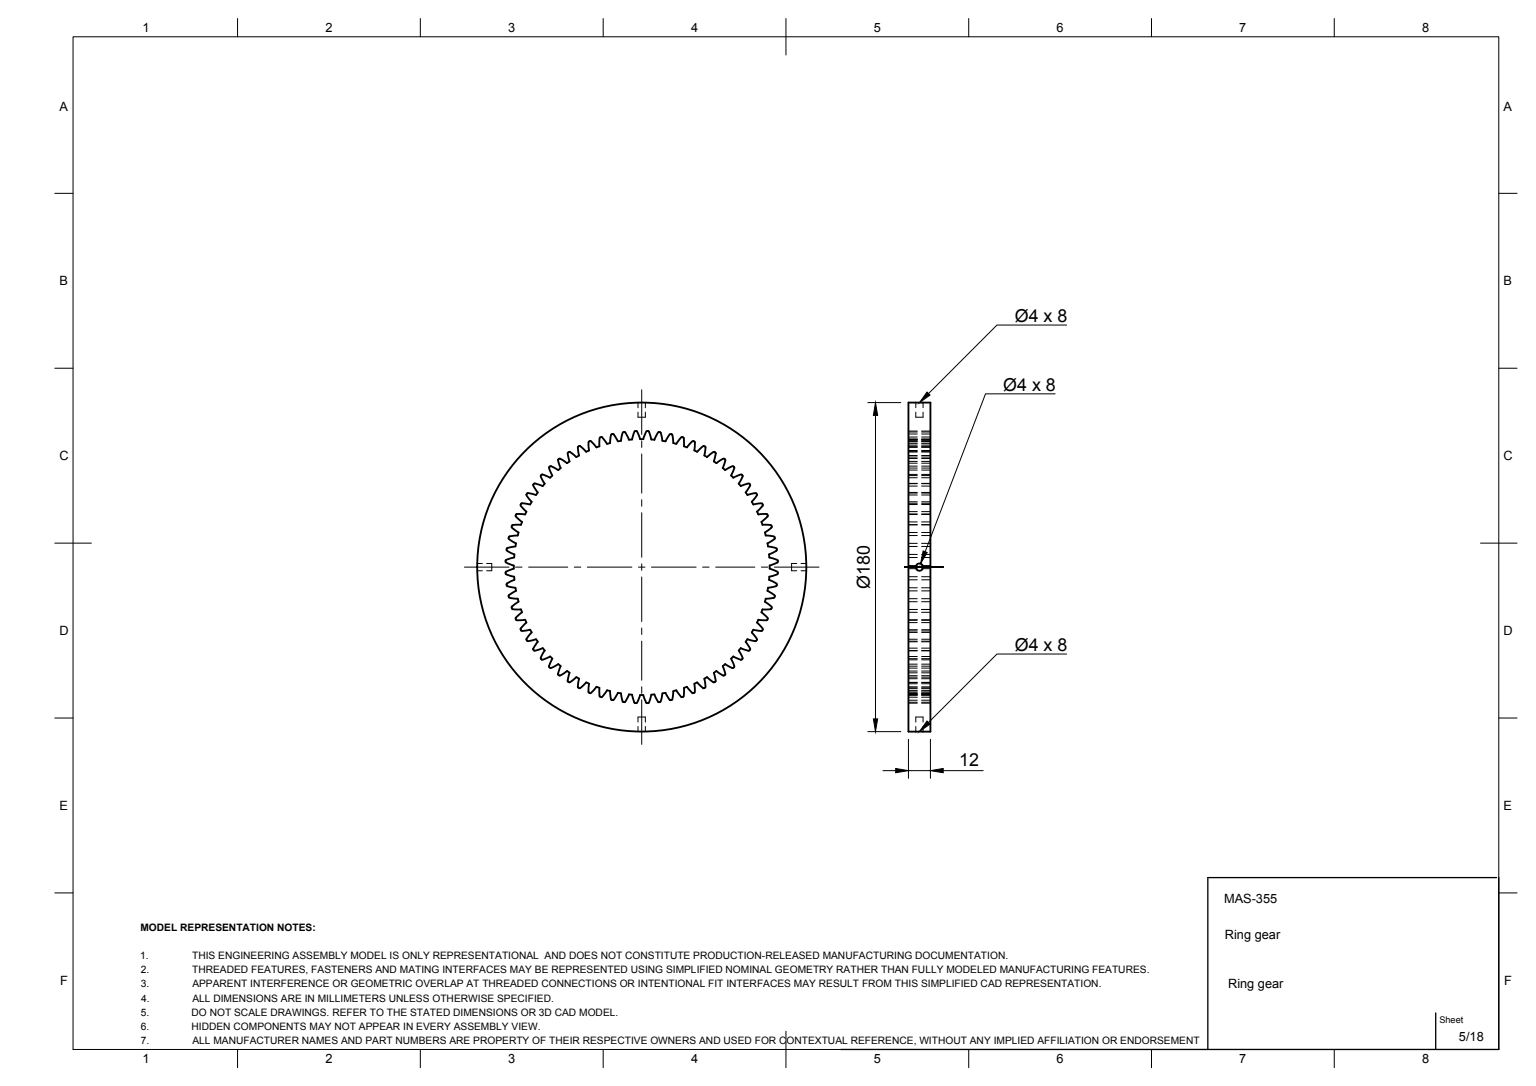
ISO-10303-21;
HEADER;
/* Generated by software containing ST-Developer
 * from STEP Tools, Inc. (www.steptools.com) 
 */

FILE_DESCRIPTION(
/* description */ ('Independent two-stage fixed-ring planetary gearbox,24/24/72 teeth,mod
ule2,20deg involutes,three planets per stage,4:1 x4:1=16:1. Native cut
-space/fillet/pattern tooth profiles derived from reusable gear blanks
; shared sun/planet/ring/carrier parts across both stages. Captured br
onze-journal input/carriers, headed retained planet pins, keyed inters
tage drive and modular keyed output interface. Native ideal gear links
; no torque, precision grade, production backlash/fits, lubrication, s
peed or life rating.'),
/* implementation_level */ '2;1');

FILE_NAME(
/* name */ 'Ring gear.step',
/* time_stamp */ '2026-11-08T19:10:00-08:00',
/* author */ (''),
/* organization */ (''),
/* preprocessor_version */ 'ST-DEVELOPER v20.2',
/* originating_system */ 'Autodesk Translation Framework v15.17.0.0',
/* authorisation */ '');

FILE_SCHEMA (('AUTOMOTIVE_DESIGN { 1 0 10303 214 3 1 1 }'));
ENDSEC;

DATA;
#10=MECHANICAL_DESIGN_GEOMETRIC_PRESENTATION_REPRESENTATION('',(#1167),#259224);
#403=(
BOUNDED_CURVE()
B_SPLINE_CURVE(5,(#53033,#53034,#53035,#53036,#53037,#53038,#53039,#53040,
#53041,#53042,#53043,#53044,#53045,#53046,#53047,#53048,#53049,#53050,#53051,
#53052,#53053,#53054,#53055,#53056,#53057,#53058,#53059,#53060,#53061,#53062,
#53063,#53064,#53065,#53066,#53067,#53068,#53069,#53070,#53071,#53072,#53073,
#53074,#53075,#53076,#53077,#53078,#53079,#53080,#53081,#53082,#53083,#53084,
#53085,#53086,#53087,#53088,#53089,#53090,#53091,#53092,#53093,#53094,#53095,
#53096,#53097,#53098,#53099,#53100,#53101,#53102,#53103,#53104,#53105,#53106,
#53107,#53108,#53109,#53110,#53111,#53112,#53113,#53114,#53115,#53116,#53117,
#53118,#53119,#53120,#53121,#53122,#53123,#53124,#53125,#53126,#53127,#53128,
#53129,#53130,#53131,#53132,#53133,#53134,#53135,#53136,#53137,#53138,#53139,
#53140,#53141,#53142,#53143,#53144,#53145,#53146,#53147,#53148,#53149,#53150,
#53151,#53152,#53153,#53154,#53155,#53156,#53157,#53158,#53159,#53160,#53161,
#53162,#53163,#53164,#53165,#53166,#53167,#53168,#53169,#53170,#53171,#53172,
#53173,#53174,#53175,#53176,#53177,#53178,#53179,#53180,#53181,#53182,#53183,
#53184,#53185,#53186,#53187,#53188,#53189,#53190,#53191,#53192,#53193,#53194,
#53195,#53196,#53197,#53198,#53199,#53200,#53201,#53202,#53203,#53204,#53205,
#53206,#53207,#53208,#53209,#53210,#53211,#53212,#53213,#53214,#53215,#53216,
#53217,#53218,#53219,#53220,#53221,#53222,#53223,#53224,#53225,#53226),
 .UNSPECIFIED.,.F.,.F.)
B_SPLINE_CURVE_WITH_KNOTS((6,1,1,1,1,1,1,1,1,1,1,1,1,1,1,1,1,1,1,1,1,1,
1,1,1,1,1,1,1,1,1,1,1,1,1,1,1,1,1,1,1,1,1,1,1,1,1,1,1,1,1,1,1,1,1,1,1,1,
1,1,1,1,1,1,1,1,1,1,1,1,1,1,1,1,1,1,1,1,1,1,1,1,1,1,1,1,1,1,1,1,1,1,1,1,
1,1,1,1,1,1,1,1,1,1,1,1,1,1,1,1,1,1,1,1,1,1,1,1,1,1,1,1,1,1,1,1,1,1,1,1,
1,1,1,1,1,1,1,1,1,1,1,1,1,1,1,1,1,1,1,1,1,1,1,1,1,1,1,1,1,1,1,1,1,1,1,1,
1,1,1,1,1,1,1,1,1,1,1,1,1,1,1,1,1,1,1,1,1,1,1,6),(0.,0.005,0.01,0.015,0.02,
0.025,0.03,0.035,0.04,0.045,0.05,0.055,0.06,0.065,0.07,0.075,0.08,0.085,
0.09,0.095,0.1,0.105,0.11,0.115,0.12,0.125,0.13,0.135,0.14,0.145,0.15,0.155,
0.16,0.165,0.17,0.175,0.18,0.185,0.19,0.195,0.2,0.205,0.21,0.215,0.22,0.225,
0.23,0.235,0.24,0.245,0.25,0.255,0.26,0.265,0.27,0.275,0.28,0.285,0.29,
0.295,0.3,0.305,0.31,0.315,0.32,0.325,0.33,0.335,0.34,0.345,0.35,0.355,
0.36,0.365,0.37,0.375,0.38,0.385,0.39,0.395,0.4,0.405,0.41,0.415,0.42,0.425,
0.43,0.435,0.44,0.445,0.45,0.455,0.46,0.465,0.47,0.475,0.48,0.485,0.49,
0.495,0.5,0.505,0.51,0.515,0.52,0.525,0.53,0.535,0.54,0.545,0.55,0.555,
0.56,0.565,0.57,0.575,0.58,0.585,0.59,0.595,0.6,0.605,0.61,0.615,0.62,0.625,
0.63,0.635,0.64,0.645,0.65,0.655,0.66,0.665,0.67,0.675,0.68,0.685,0.690000000000001,
0.695000000000001,0.700000000000001,0.705000000000001,0.710000000000001,
0.715000000000001,0.720000000000001,0.725000000000001,0.730000000000001,
0.735000000000001,0.740000000000001,0.745000000000001,0.750000000000001,
0.755000000000001,0.760000000000001,0.765000000000001,0.770000000000001,
0.775000000000001,0.780000000000001,0.785000000000001,0.790000000000001,
0.795000000000001,0.800000000000001,0.805000000000001,0.810000000000001,
0.815000000000001,0.820000000000001,0.825000000000001,0.830000000000001,
0.835000000000001,0.840000000000001,0.845000000000001,0.850000000000001,
0.855000000000001,0.860000000000001,0.865000000000001,0.870000000000001,
0.875000000000001,0.880000000000001,0.885000000000001,0.890000000000001,
0.895000000000001,0.900000000000001,0.905000000000001,0.910000000000001,
0.915000000000001,0.920000000000001,0.925000000000001,0.930000000000001,
0.935000000000001,0.940000000000001,0.941429844431396),.UNSPECIFIED.)
CURVE()
GEOMETRIC_REPRESENTATION_ITEM()
RATIONAL_B_SPLINE_CURVE((1.,1.,1.,1.,1.,1.,1.,1.,1.,1.,1.,1.,1.,1.,1.,1.,
1.,1.,1.,1.,1.,1.,1.,1.,1.,1.,1.,1.,1.,1.,1.,1.,1.,1.,1.,1.,1.,1.,1.,1.,
1.,1.,1.,1.,1.,1.,1.,1.,1.,1.,1.,1.,1.,1.,1.,1.,1.,1.,1.,1.,1.,1.,1.,1.,
1.,1.,1.,1.,1.,1.,1.,1.,1.,1.,1.,1.,1.,1.,1.,1.,1.,1.,1.,1.,1.,1.,1.,1.,
1.,1.,1.,1.,1.,1.,1.,1.,1.,1.,1.,1.,1.,1.,1.,1.,1.,1.,1.,1.,1.,1.,1.,1.,
1.,1.,1.,1.,1.,1.,1.,1.,1.,1.,1.,1.,1.,1.,1.,1.,1.,1.,1.,1.,1.,1.,1.,1.,
1.,1.,1.,1.,1.,1.,1.,1.,1.,1.,1.,1.,1.,1.,1.,1.,1.,1.,1.,1.,1.,1.,1.,1.,
1.,1.,1.,1.,1.,1.,1.,1.,1.,1.,1.,1.,1.,1.,1.,1.,1.,1.,1.,1.,1.,1.,1.,1.,
1.,1.,1.,1.,1.,1.,1.,1.,1.,1.))
REPRESENTATION_ITEM('')
);
#404=(
BOUNDED_CURVE()
B_SPLINE_CURVE(5,(#53229,#53230,#53231,#53232,#53233,#53234,#53235,#53236,
#53237,#53238,#53239,#53240,#53241,#53242,#53243,#53244,#53245,#53246,#53247,
#53248,#53249,#53250,#53251,#53252,#53253,#53254,#53255,#53256,#53257,#53258,
#53259,#53260,#53261,#53262,#53263,#53264,#53265,#53266,#53267,#53268,#53269,
#53270,#53271,#53272,#53273,#53274,#53275,#53276,#53277,#53278,#53279,#53280,
#53281,#53282,#53283,#53284,#53285,#53286,#53287,#53288,#53289,#53290,#53291,
#53292,#53293,#53294,#53295,#53296,#53297,#53298,#53299,#53300,#53301,#53302,
#53303,#53304,#53305,#53306,#53307,#53308,#53309,#53310,#53311,#53312,#53313,
#53314,#53315,#53316,#53317,#53318,#53319,#53320,#53321,#53322,#53323,#53324,
#53325,#53326,#53327,#53328,#53329,#53330,#53331,#53332,#53333,#53334,#53335,
#53336,#53337,#53338,#53339,#53340,#53341,#53342,#53343,#53344,#53345,#53346,
#53347,#53348,#53349,#53350,#53351,#53352,#53353,#53354,#53355,#53356,#53357,
#53358,#53359,#53360,#53361,#53362,#53363,#53364,#53365,#53366,#53367,#53368,
#53369,#53370,#53371,#53372,#53373,#53374,#53375,#53376,#53377,#53378,#53379,
#53380,#53381,#53382,#53383,#53384,#53385,#53386,#53387,#53388,#53389,#53390,
#53391,#53392,#53393,#53394,#53395,#53396,#53397,#53398,#53399,#53400,#53401,
#53402,#53403,#53404,#53405,#53406,#53407,#53408,#53409,#53410,#53411,#53412,
#53413,#53414,#53415,#53416,#53417,#53418,#53419,#53420,#53421,#53422),
 .UNSPECIFIED.,.F.,.F.)
B_SPLINE_CURVE_WITH_KNOTS((6,1,1,1,1,1,1,1,1,1,1,1,1,1,1,1,1,1,1,1,1,1,
1,1,1,1,1,1,1,1,1,1,1,1,1,1,1,1,1,1,1,1,1,1,1,1,1,1,1,1,1,1,1,1,1,1,1,1,
1,1,1,1,1,1,1,1,1,1,1,1,1,1,1,1,1,1,1,1,1,1,1,1,1,1,1,1,1,1,1,1,1,1,1,1,
1,1,1,1,1,1,1,1,1,1,1,1,1,1,1,1,1,1,1,1,1,1,1,1,1,1,1,1,1,1,1,1,1,1,1,1,
1,1,1,1,1,1,1,1,1,1,1,1,1,1,1,1,1,1,1,1,1,1,1,1,1,1,1,1,1,1,1,1,1,1,1,1,
1,1,1,1,1,1,1,1,1,1,1,1,1,1,1,1,1,1,1,1,1,1,1,6),(-0.941429844431396,-0.940000000000001,
-0.935000000000001,-0.930000000000001,-0.925000000000001,-0.920000000000001,
-0.915000000000001,-0.910000000000001,-0.905000000000001,-0.900000000000001,
-0.895000000000001,-0.890000000000001,-0.885000000000001,-0.880000000000001,
-0.875000000000001,-0.870000000000001,-0.865000000000001,-0.860000000000001,
-0.855000000000001,-0.850000000000001,-0.845000000000001,-0.840000000000001,
-0.835000000000001,-0.830000000000001,-0.825000000000001,-0.820000000000001,
-0.815000000000001,-0.810000000000001,-0.805000000000001,-0.800000000000001,
-0.795000000000001,-0.790000000000001,-0.785000000000001,-0.780000000000001,
-0.775000000000001,-0.770000000000001,-0.765000000000001,-0.760000000000001,
-0.755000000000001,-0.750000000000001,-0.745000000000001,-0.740000000000001,
-0.735000000000001,-0.730000000000001,-0.725000000000001,-0.720000000000001,
-0.715000000000001,-0.710000000000001,-0.705000000000001,-0.700000000000001,
-0.695000000000001,-0.690000000000001,-0.685,-0.68,-0.675,-0.67,-0.665,
-0.66,-0.655,-0.65,-0.645,-0.64,-0.635,-0.63,-0.625,-0.62,-0.615,-0.61,
-0.605,-0.6,-0.595,-0.59,-0.585,-0.58,-0.575,-0.57,-0.565,-0.56,-0.555,
-0.55,-0.545,-0.54,-0.535,-0.53,-0.525,-0.52,-0.515,-0.51,-0.505,-0.5,-0.495,
-0.49,-0.485,-0.48,-0.475,-0.47,-0.465,-0.46,-0.455,-0.45,-0.445,-0.44,
-0.435,-0.43,-0.425,-0.42,-0.415,-0.41,-0.405,-0.4,-0.395,-0.39,-0.385,
-0.38,-0.375,-0.37,-0.365,-0.36,-0.355,-0.35,-0.345,-0.34,-0.335,-0.33,
-0.325,-0.32,-0.315,-0.31,-0.305,-0.3,-0.295,-0.29,-0.285,-0.28,-0.275,
-0.27,-0.265,-0.26,-0.255,-0.25,-0.245,-0.24,-0.235,-0.23,-0.225,-0.22,
-0.215,-0.21,-0.205,-0.2,-0.195,-0.19,-0.185,-0.18,-0.175,-0.17,-0.165,
-0.16,-0.155,-0.15,-0.145,-0.14,-0.135,-0.13,-0.125,-0.12,-0.115,-0.11,
-0.105,-0.1,-0.095,-0.09,-0.085,-0.08,-0.075,-0.07,-0.065,-0.06,-0.055,
-0.05,-0.045,-0.04,-0.035,-0.03,-0.025,-0.02,-0.015,-0.01,-0.005,0.),
 .UNSPECIFIED.)
CURVE()
GEOMETRIC_REPRESENTATION_ITEM()
RATIONAL_B_SPLINE_CURVE((1.,1.,1.,1.,1.,1.,1.,1.,1.,1.,1.,1.,1.,1.,1.,1.,
1.,1.,1.,1.,1.,1.,1.,1.,1.,1.,1.,1.,1.,1.,1.,1.,1.,1.,1.,1.,1.,1.,1.,1.,
1.,1.,1.,1.,1.,1.,1.,1.,1.,1.,1.,1.,1.,1.,1.,1.,1.,1.,1.,1.,1.,1.,1.,1.,
1.,1.,1.,1.,1.,1.,1.,1.,1.,1.,1.,1.,1.,1.,1.,1.,1.,1.,1.,1.,1.,1.,1.,1.,
1.,1.,1.,1.,1.,1.,1.,1.,1.,1.,1.,1.,1.,1.,1.,1.,1.,1.,1.,1.,1.,1.,1.,1.,
1.,1.,1.,1.,1.,1.,1.,1.,1.,1.,1.,1.,1.,1.,1.,1.,1.,1.,1.,1.,1.,1.,1.,1.,
1.,1.,1.,1.,1.,1.,1.,1.,1.,1.,1.,1.,1.,1.,1.,1.,1.,1.,1.,1.,1.,1.,1.,1.,
1.,1.,1.,1.,1.,1.,1.,1.,1.,1.,1.,1.,1.,1.,1.,1.,1.,1.,1.,1.,1.,1.,1.,1.,
1.,1.,1.,1.,1.,1.,1.,1.,1.,1.))
REPRESENTATION_ITEM('')
);
#405=(
BOUNDED_CURVE()
B_SPLINE_CURVE(5,(#53929,#53930,#53931,#53932,#53933,#53934,#53935,#53936,
#53937,#53938,#53939,#53940,#53941,#53942,#53943,#53944,#53945,#53946,#53947,
#53948,#53949,#53950,#53951,#53952,#53953,#53954,#53955,#53956,#53957,#53958,
#53959,#53960,#53961,#53962,#53963,#53964,#53965,#53966,#53967,#53968,#53969,
#53970,#53971,#53972,#53973,#53974,#53975,#53976,#53977,#53978,#53979,#53980,
#53981,#53982,#53983,#53984,#53985,#53986,#53987,#53988,#53989,#53990,#53991,
#53992,#53993,#53994,#53995,#53996,#53997,#53998,#53999,#54000,#54001,#54002,
#54003,#54004,#54005,#54006,#54007,#54008,#54009,#54010,#54011,#54012,#54013,
#54014,#54015,#54016,#54017,#54018,#54019,#54020,#54021,#54022,#54023,#54024,
#54025,#54026,#54027,#54028,#54029,#54030,#54031,#54032,#54033,#54034,#54035,
#54036,#54037,#54038,#54039,#54040,#54041,#54042,#54043,#54044,#54045,#54046,
#54047,#54048,#54049,#54050,#54051,#54052,#54053,#54054,#54055,#54056,#54057,
#54058,#54059,#54060,#54061,#54062,#54063,#54064,#54065,#54066,#54067,#54068,
#54069,#54070,#54071,#54072,#54073,#54074,#54075,#54076,#54077,#54078,#54079,
#54080,#54081,#54082,#54083,#54084,#54085,#54086,#54087,#54088,#54089,#54090,
#54091,#54092,#54093,#54094,#54095,#54096,#54097,#54098,#54099,#54100,#54101,
#54102,#54103,#54104,#54105,#54106,#54107,#54108,#54109,#54110,#54111,#54112,
#54113,#54114,#54115,#54116,#54117,#54118,#54119,#54120,#54121,#54122),
 .UNSPECIFIED.,.F.,.F.)
B_SPLINE_CURVE_WITH_KNOTS((6,1,1,1,1,1,1,1,1,1,1,1,1,1,1,1,1,1,1,1,1,1,
1,1,1,1,1,1,1,1,1,1,1,1,1,1,1,1,1,1,1,1,1,1,1,1,1,1,1,1,1,1,1,1,1,1,1,1,
1,1,1,1,1,1,1,1,1,1,1,1,1,1,1,1,1,1,1,1,1,1,1,1,1,1,1,1,1,1,1,1,1,1,1,1,
1,1,1,1,1,1,1,1,1,1,1,1,1,1,1,1,1,1,1,1,1,1,1,1,1,1,1,1,1,1,1,1,1,1,1,1,
1,1,1,1,1,1,1,1,1,1,1,1,1,1,1,1,1,1,1,1,1,1,1,1,1,1,1,1,1,1,1,1,1,1,1,1,
1,1,1,1,1,1,1,1,1,1,1,1,1,1,1,1,1,1,1,1,1,1,1,6),(0.,0.005,0.01,0.015,0.02,
0.025,0.03,0.035,0.04,0.045,0.05,0.055,0.06,0.065,0.07,0.075,0.08,0.085,
0.09,0.095,0.1,0.105,0.11,0.115,0.12,0.125,0.13,0.135,0.14,0.145,0.15,0.155,
0.16,0.165,0.17,0.175,0.18,0.185,0.19,0.195,0.2,0.205,0.21,0.215,0.22,0.225,
0.23,0.235,0.24,0.245,0.25,0.255,0.26,0.265,0.27,0.275,0.28,0.285,0.29,
0.295,0.3,0.305,0.31,0.315,0.32,0.325,0.33,0.335,0.34,0.345,0.35,0.355,
0.36,0.365,0.37,0.375,0.38,0.385,0.39,0.395,0.4,0.405,0.41,0.415,0.42,0.425,
0.43,0.435,0.44,0.445,0.45,0.455,0.46,0.465,0.47,0.475,0.48,0.485,0.49,
0.495,0.5,0.505,0.51,0.515,0.52,0.525,0.53,0.535,0.54,0.545,0.55,0.555,
0.56,0.565,0.57,0.575,0.58,0.585,0.59,0.595,0.6,0.605,0.61,0.615,0.62,0.625,
0.63,0.635,0.64,0.645,0.65,0.655,0.66,0.665,0.67,0.675,0.68,0.685,0.690000000000001,
0.695000000000001,0.700000000000001,0.705000000000001,0.710000000000001,
0.715000000000001,0.720000000000001,0.725000000000001,0.730000000000001,
0.735000000000001,0.740000000000001,0.745000000000001,0.750000000000001,
0.755000000000001,0.760000000000001,0.765000000000001,0.770000000000001,
0.775000000000001,0.780000000000001,0.785000000000001,0.790000000000001,
0.795000000000001,0.800000000000001,0.805000000000001,0.810000000000001,
0.815000000000001,0.820000000000001,0.825000000000001,0.830000000000001,
0.835000000000001,0.840000000000001,0.845000000000001,0.850000000000001,
0.855000000000001,0.860000000000001,0.865000000000001,0.870000000000001,
0.875000000000001,0.880000000000001,0.885000000000001,0.890000000000001,
0.895000000000001,0.900000000000001,0.905000000000001,0.910000000000001,
0.915000000000001,0.920000000000001,0.925000000000001,0.930000000000001,
0.935000000000001,0.940000000000001,0.941429844431388),.UNSPECIFIED.)
CURVE()
GEOMETRIC_REPRESENTATION_ITEM()
RATIONAL_B_SPLINE_CURVE((1.,1.,1.,1.,1.,1.,1.,1.,1.,1.,1.,1.,1.,1.,1.,1.,
1.,1.,1.,1.,1.,1.,1.,1.,1.,1.,1.,1.,1.,1.,1.,1.,1.,1.,1.,1.,1.,1.,1.,1.,
1.,1.,1.,1.,1.,1.,1.,1.,1.,1.,1.,1.,1.,1.,1.,1.,1.,1.,1.,1.,1.,1.,1.,1.,
1.,1.,1.,1.,1.,1.,1.,1.,1.,1.,1.,1.,1.,1.,1.,1.,1.,1.,1.,1.,1.,1.,1.,1.,
1.,1.,1.,1.,1.,1.,1.,1.,1.,1.,1.,1.,1.,1.,1.,1.,1.,1.,1.,1.,1.,1.,1.,1.,
1.,1.,1.,1.,1.,1.,1.,1.,1.,1.,1.,1.,1.,1.,1.,1.,1.,1.,1.,1.,1.,1.,1.,1.,
1.,1.,1.,1.,1.,1.,1.,1.,1.,1.,1.,1.,1.,1.,1.,1.,1.,1.,1.,1.,1.,1.,1.,1.,
1.,1.,1.,1.,1.,1.,1.,1.,1.,1.,1.,1.,1.,1.,1.,1.,1.,1.,1.,1.,1.,1.,1.,1.,
1.,1.,1.,1.,1.,1.,1.,1.,1.,1.))
REPRESENTATION_ITEM('')
);
#406=(
BOUNDED_CURVE()
B_SPLINE_CURVE(5,(#54125,#54126,#54127,#54128,#54129,#54130,#54131,#54132,
#54133,#54134,#54135,#54136,#54137,#54138,#54139,#54140,#54141,#54142,#54143,
#54144,#54145,#54146,#54147,#54148,#54149,#54150,#54151,#54152,#54153,#54154,
#54155,#54156,#54157,#54158,#54159,#54160,#54161,#54162,#54163,#54164,#54165,
#54166,#54167,#54168,#54169,#54170,#54171,#54172,#54173,#54174,#54175,#54176,
#54177,#54178,#54179,#54180,#54181,#54182,#54183,#54184,#54185,#54186,#54187,
#54188,#54189,#54190,#54191,#54192,#54193,#54194,#54195,#54196,#54197,#54198,
#54199,#54200,#54201,#54202,#54203,#54204,#54205,#54206,#54207,#54208,#54209,
#54210,#54211,#54212,#54213,#54214,#54215,#54216,#54217,#54218,#54219,#54220,
#54221,#54222,#54223,#54224,#54225,#54226,#54227,#54228,#54229,#54230,#54231,
#54232,#54233,#54234,#54235,#54236,#54237,#54238,#54239,#54240,#54241,#54242,
#54243,#54244,#54245,#54246,#54247,#54248,#54249,#54250,#54251,#54252,#54253,
#54254,#54255,#54256,#54257,#54258,#54259,#54260,#54261,#54262,#54263,#54264,
#54265,#54266,#54267,#54268,#54269,#54270,#54271,#54272,#54273,#54274,#54275,
#54276,#54277,#54278,#54279,#54280,#54281,#54282,#54283,#54284,#54285,#54286,
#54287,#54288,#54289,#54290,#54291,#54292,#54293,#54294,#54295,#54296,#54297,
#54298,#54299,#54300,#54301,#54302,#54303,#54304,#54305,#54306,#54307,#54308,
#54309,#54310,#54311,#54312,#54313,#54314,#54315,#54316,#54317,#54318),
 .UNSPECIFIED.,.F.,.F.)
B_SPLINE_CURVE_WITH_KNOTS((6,1,1,1,1,1,1,1,1,1,1,1,1,1,1,1,1,1,1,1,1,1,
1,1,1,1,1,1,1,1,1,1,1,1,1,1,1,1,1,1,1,1,1,1,1,1,1,1,1,1,1,1,1,1,1,1,1,1,
1,1,1,1,1,1,1,1,1,1,1,1,1,1,1,1,1,1,1,1,1,1,1,1,1,1,1,1,1,1,1,1,1,1,1,1,
1,1,1,1,1,1,1,1,1,1,1,1,1,1,1,1,1,1,1,1,1,1,1,1,1,1,1,1,1,1,1,1,1,1,1,1,
1,1,1,1,1,1,1,1,1,1,1,1,1,1,1,1,1,1,1,1,1,1,1,1,1,1,1,1,1,1,1,1,1,1,1,1,
1,1,1,1,1,1,1,1,1,1,1,1,1,1,1,1,1,1,1,1,1,1,1,6),(-0.941429844431391,-0.940000000000001,
-0.935000000000001,-0.930000000000001,-0.925000000000001,-0.920000000000001,
-0.915000000000001,-0.910000000000001,-0.905000000000001,-0.900000000000001,
-0.895000000000001,-0.890000000000001,-0.885000000000001,-0.880000000000001,
-0.875000000000001,-0.870000000000001,-0.865000000000001,-0.860000000000001,
-0.855000000000001,-0.850000000000001,-0.845000000000001,-0.840000000000001,
-0.835000000000001,-0.830000000000001,-0.825000000000001,-0.820000000000001,
-0.815000000000001,-0.810000000000001,-0.805000000000001,-0.800000000000001,
-0.795000000000001,-0.790000000000001,-0.785000000000001,-0.780000000000001,
-0.775000000000001,-0.770000000000001,-0.765000000000001,-0.760000000000001,
-0.755000000000001,-0.750000000000001,-0.745000000000001,-0.740000000000001,
-0.735000000000001,-0.730000000000001,-0.725000000000001,-0.720000000000001,
-0.715000000000001,-0.710000000000001,-0.705000000000001,-0.700000000000001,
-0.695000000000001,-0.690000000000001,-0.685,-0.68,-0.675,-0.67,-0.665,
-0.66,-0.655,-0.65,-0.645,-0.64,-0.635,-0.63,-0.625,-0.62,-0.615,-0.61,
-0.605,-0.6,-0.595,-0.59,-0.585,-0.58,-0.575,-0.57,-0.565,-0.56,-0.555,
-0.55,-0.545,-0.54,-0.535,-0.53,-0.525,-0.52,-0.515,-0.51,-0.505,-0.5,-0.495,
-0.49,-0.485,-0.48,-0.475,-0.47,-0.465,-0.46,-0.455,-0.45,-0.445,-0.44,
-0.435,-0.43,-0.425,-0.42,-0.415,-0.41,-0.405,-0.4,-0.395,-0.39,-0.385,
-0.38,-0.375,-0.37,-0.365,-0.36,-0.355,-0.35,-0.345,-0.34,-0.335,-0.33,
-0.325,-0.32,-0.315,-0.31,-0.305,-0.3,-0.295,-0.29,-0.285,-0.28,-0.275,
-0.27,-0.265,-0.26,-0.255,-0.25,-0.245,-0.24,-0.235,-0.23,-0.225,-0.22,
-0.215,-0.21,-0.205,-0.2,-0.195,-0.19,-0.185,-0.18,-0.175,-0.17,-0.165,
-0.16,-0.155,-0.15,-0.145,-0.14,-0.135,-0.13,-0.125,-0.12,-0.115,-0.11,
-0.105,-0.1,-0.095,-0.09,-0.085,-0.08,-0.075,-0.07,-0.065,-0.06,-0.055,
-0.05,-0.045,-0.04,-0.035,-0.03,-0.025,-0.02,-0.015,-0.01,-0.005,0.),
 .UNSPECIFIED.)
CURVE()
GEOMETRIC_REPRESENTATION_ITEM()
RATIONAL_B_SPLINE_CURVE((1.,1.,1.,1.,1.,1.,1.,1.,1.,1.,1.,1.,1.,1.,1.,1.,
1.,1.,1.,1.,1.,1.,1.,1.,1.,1.,1.,1.,1.,1.,1.,1.,1.,1.,1.,1.,1.,1.,1.,1.,
1.,1.,1.,1.,1.,1.,1.,1.,1.,1.,1.,1.,1.,1.,1.,1.,1.,1.,1.,1.,1.,1.,1.,1.,
1.,1.,1.,1.,1.,1.,1.,1.,1.,1.,1.,1.,1.,1.,1.,1.,1.,1.,1.,1.,1.,1.,1.,1.,
1.,1.,1.,1.,1.,1.,1.,1.,1.,1.,1.,1.,1.,1.,1.,1.,1.,1.,1.,1.,1.,1.,1.,1.,
1.,1.,1.,1.,1.,1.,1.,1.,1.,1.,1.,1.,1.,1.,1.,1.,1.,1.,1.,1.,1.,1.,1.,1.,
1.,1.,1.,1.,1.,1.,1.,1.,1.,1.,1.,1.,1.,1.,1.,1.,1.,1.,1.,1.,1.,1.,1.,1.,
1.,1.,1.,1.,1.,1.,1.,1.,1.,1.,1.,1.,1.,1.,1.,1.,1.,1.,1.,1.,1.,1.,1.,1.,
1.,1.,1.,1.,1.,1.,1.,1.,1.,1.))
REPRESENTATION_ITEM('')
);
#407=(
BOUNDED_CURVE()
B_SPLINE_CURVE(5,(#54825,#54826,#54827,#54828,#54829,#54830,#54831,#54832,
#54833,#54834,#54835,#54836,#54837,#54838,#54839,#54840,#54841,#54842,#54843,
#54844,#54845,#54846,#54847,#54848,#54849,#54850,#54851,#54852,#54853,#54854,
#54855,#54856,#54857,#54858,#54859,#54860,#54861,#54862,#54863,#54864,#54865,
#54866,#54867,#54868,#54869,#54870,#54871,#54872,#54873,#54874,#54875,#54876,
#54877,#54878,#54879,#54880,#54881,#54882,#54883,#54884,#54885,#54886,#54887,
#54888,#54889,#54890,#54891,#54892,#54893,#54894,#54895,#54896,#54897,#54898,
#54899,#54900,#54901,#54902,#54903,#54904,#54905,#54906,#54907,#54908,#54909,
#54910,#54911,#54912,#54913,#54914,#54915,#54916,#54917,#54918,#54919,#54920,
#54921,#54922,#54923,#54924,#54925,#54926,#54927,#54928,#54929,#54930,#54931,
#54932,#54933,#54934,#54935,#54936,#54937,#54938,#54939,#54940,#54941,#54942,
#54943,#54944,#54945,#54946,#54947,#54948,#54949,#54950,#54951,#54952,#54953,
#54954,#54955,#54956,#54957,#54958,#54959,#54960,#54961,#54962,#54963,#54964,
#54965,#54966,#54967,#54968,#54969,#54970,#54971,#54972,#54973,#54974,#54975,
#54976,#54977,#54978,#54979,#54980,#54981,#54982,#54983,#54984,#54985,#54986,
#54987,#54988,#54989,#54990,#54991,#54992,#54993,#54994,#54995,#54996,#54997,
#54998,#54999,#55000,#55001,#55002,#55003,#55004,#55005,#55006,#55007,#55008,
#55009,#55010,#55011,#55012,#55013,#55014,#55015,#55016,#55017,#55018),
 .UNSPECIFIED.,.F.,.F.)
B_SPLINE_CURVE_WITH_KNOTS((6,1,1,1,1,1,1,1,1,1,1,1,1,1,1,1,1,1,1,1,1,1,
1,1,1,1,1,1,1,1,1,1,1,1,1,1,1,1,1,1,1,1,1,1,1,1,1,1,1,1,1,1,1,1,1,1,1,1,
1,1,1,1,1,1,1,1,1,1,1,1,1,1,1,1,1,1,1,1,1,1,1,1,1,1,1,1,1,1,1,1,1,1,1,1,
1,1,1,1,1,1,1,1,1,1,1,1,1,1,1,1,1,1,1,1,1,1,1,1,1,1,1,1,1,1,1,1,1,1,1,1,
1,1,1,1,1,1,1,1,1,1,1,1,1,1,1,1,1,1,1,1,1,1,1,1,1,1,1,1,1,1,1,1,1,1,1,1,
1,1,1,1,1,1,1,1,1,1,1,1,1,1,1,1,1,1,1,1,1,1,1,6),(0.,0.005,0.01,0.015,0.02,
0.025,0.03,0.035,0.04,0.045,0.05,0.055,0.06,0.065,0.07,0.075,0.08,0.085,
0.09,0.095,0.1,0.105,0.11,0.115,0.12,0.125,0.13,0.135,0.14,0.145,0.15,0.155,
0.16,0.165,0.17,0.175,0.18,0.185,0.19,0.195,0.2,0.205,0.21,0.215,0.22,0.225,
0.23,0.235,0.24,0.245,0.25,0.255,0.26,0.265,0.27,0.275,0.28,0.285,0.29,
0.295,0.3,0.305,0.31,0.315,0.32,0.325,0.33,0.335,0.34,0.345,0.35,0.355,
0.36,0.365,0.37,0.375,0.38,0.385,0.39,0.395,0.4,0.405,0.41,0.415,0.42,0.425,
0.43,0.435,0.44,0.445,0.45,0.455,0.46,0.465,0.47,0.475,0.48,0.485,0.49,
0.495,0.5,0.505,0.51,0.515,0.52,0.525,0.53,0.535,0.54,0.545,0.55,0.555,
0.56,0.565,0.57,0.575,0.58,0.585,0.59,0.595,0.6,0.605,0.61,0.615,0.62,0.625,
0.63,0.635,0.64,0.645,0.65,0.655,0.66,0.665,0.67,0.675,0.68,0.685,0.690000000000001,
0.695000000000001,0.700000000000001,0.705000000000001,0.710000000000001,
0.715000000000001,0.720000000000001,0.725000000000001,0.730000000000001,
0.735000000000001,0.740000000000001,0.745000000000001,0.750000000000001,
0.755000000000001,0.760000000000001,0.765000000000001,0.770000000000001,
0.775000000000001,0.780000000000001,0.785000000000001,0.790000000000001,
0.795000000000001,0.800000000000001,0.805000000000001,0.810000000000001,
0.815000000000001,0.820000000000001,0.825000000000001,0.830000000000001,
0.835000000000001,0.840000000000001,0.845000000000001,0.850000000000001,
0.855000000000001,0.860000000000001,0.865000000000001,0.870000000000001,
0.875000000000001,0.880000000000001,0.885000000000001,0.890000000000001,
0.895000000000001,0.900000000000001,0.905000000000001,0.910000000000001,
0.915000000000001,0.920000000000001,0.925000000000001,0.930000000000001,
0.935000000000001,0.940000000000001,0.941429844431439),.UNSPECIFIED.)
CURVE()
GEOMETRIC_REPRESENTATION_ITEM()
RATIONAL_B_SPLINE_CURVE((1.,1.,1.,1.,1.,1.,1.,1.,1.,1.,1.,1.,1.,1.,1.,1.,
1.,1.,1.,1.,1.,1.,1.,1.,1.,1.,1.,1.,1.,1.,1.,1.,1.,1.,1.,1.,1.,1.,1.,1.,
1.,1.,1.,1.,1.,1.,1.,1.,1.,1.,1.,1.,1.,1.,1.,1.,1.,1.,1.,1.,1.,1.,1.,1.,
1.,1.,1.,1.,1.,1.,1.,1.,1.,1.,1.,1.,1.,1.,1.,1.,1.,1.,1.,1.,1.,1.,1.,1.,
1.,1.,1.,1.,1.,1.,1.,1.,1.,1.,1.,1.,1.,1.,1.,1.,1.,1.,1.,1.,1.,1.,1.,1.,
1.,1.,1.,1.,1.,1.,1.,1.,1.,1.,1.,1.,1.,1.,1.,1.,1.,1.,1.,1.,1.,1.,1.,1.,
1.,1.,1.,1.,1.,1.,1.,1.,1.,1.,1.,1.,1.,1.,1.,1.,1.,1.,1.,1.,1.,1.,1.,1.,
1.,1.,1.,1.,1.,1.,1.,1.,1.,1.,1.,1.,1.,1.,1.,1.,1.,1.,1.,1.,1.,1.,1.,1.,
1.,1.,1.,1.,1.,1.,1.,1.,1.,1.))
REPRESENTATION_ITEM('')
);
#408=(
BOUNDED_CURVE()
B_SPLINE_CURVE(5,(#55021,#55022,#55023,#55024,#55025,#55026,#55027,#55028,
#55029,#55030,#55031,#55032,#55033,#55034,#55035,#55036,#55037,#55038,#55039,
#55040,#55041,#55042,#55043,#55044,#55045,#55046,#55047,#55048,#55049,#55050,
#55051,#55052,#55053,#55054,#55055,#55056,#55057,#55058,#55059,#55060,#55061,
#55062,#55063,#55064,#55065,#55066,#55067,#55068,#55069,#55070,#55071,#55072,
#55073,#55074,#55075,#55076,#55077,#55078,#55079,#55080,#55081,#55082,#55083,
#55084,#55085,#55086,#55087,#55088,#55089,#55090,#55091,#55092,#55093,#55094,
#55095,#55096,#55097,#55098,#55099,#55100,#55101,#55102,#55103,#55104,#55105,
#55106,#55107,#55108,#55109,#55110,#55111,#55112,#55113,#55114,#55115,#55116,
#55117,#55118,#55119,#55120,#55121,#55122,#55123,#55124,#55125,#55126,#55127,
#55128,#55129,#55130,#55131,#55132,#55133,#55134,#55135,#55136,#55137,#55138,
#55139,#55140,#55141,#55142,#55143,#55144,#55145,#55146,#55147,#55148,#55149,
#55150,#55151,#55152,#55153,#55154,#55155,#55156,#55157,#55158,#55159,#55160,
#55161,#55162,#55163,#55164,#55165,#55166,#55167,#55168,#55169,#55170,#55171,
#55172,#55173,#55174,#55175,#55176,#55177,#55178,#55179,#55180,#55181,#55182,
#55183,#55184,#55185,#55186,#55187,#55188,#55189,#55190,#55191,#55192,#55193,
#55194,#55195,#55196,#55197,#55198,#55199,#55200,#55201,#55202,#55203,#55204,
#55205,#55206,#55207,#55208,#55209,#55210,#55211,#55212,#55213,#55214),
 .UNSPECIFIED.,.F.,.F.)
B_SPLINE_CURVE_WITH_KNOTS((6,1,1,1,1,1,1,1,1,1,1,1,1,1,1,1,1,1,1,1,1,1,
1,1,1,1,1,1,1,1,1,1,1,1,1,1,1,1,1,1,1,1,1,1,1,1,1,1,1,1,1,1,1,1,1,1,1,1,
1,1,1,1,1,1,1,1,1,1,1,1,1,1,1,1,1,1,1,1,1,1,1,1,1,1,1,1,1,1,1,1,1,1,1,1,
1,1,1,1,1,1,1,1,1,1,1,1,1,1,1,1,1,1,1,1,1,1,1,1,1,1,1,1,1,1,1,1,1,1,1,1,
1,1,1,1,1,1,1,1,1,1,1,1,1,1,1,1,1,1,1,1,1,1,1,1,1,1,1,1,1,1,1,1,1,1,1,1,
1,1,1,1,1,1,1,1,1,1,1,1,1,1,1,1,1,1,1,1,1,1,1,6),(-0.941429844431442,-0.940000000000001,
-0.935000000000001,-0.930000000000001,-0.925000000000001,-0.920000000000001,
-0.915000000000001,-0.910000000000001,-0.905000000000001,-0.900000000000001,
-0.895000000000001,-0.890000000000001,-0.885000000000001,-0.880000000000001,
-0.875000000000001,-0.870000000000001,-0.865000000000001,-0.860000000000001,
-0.855000000000001,-0.850000000000001,-0.845000000000001,-0.840000000000001,
-0.835000000000001,-0.830000000000001,-0.825000000000001,-0.820000000000001,
-0.815000000000001,-0.810000000000001,-0.805000000000001,-0.800000000000001,
-0.795000000000001,-0.790000000000001,-0.785000000000001,-0.780000000000001,
-0.775000000000001,-0.770000000000001,-0.765000000000001,-0.760000000000001,
-0.755000000000001,-0.750000000000001,-0.745000000000001,-0.740000000000001,
-0.735000000000001,-0.730000000000001,-0.725000000000001,-0.720000000000001,
-0.715000000000001,-0.710000000000001,-0.705000000000001,-0.700000000000001,
-0.695000000000001,-0.690000000000001,-0.685,-0.68,-0.675,-0.67,-0.665,
-0.66,-0.655,-0.65,-0.645,-0.64,-0.635,-0.63,-0.625,-0.62,-0.615,-0.61,
-0.605,-0.6,-0.595,-0.59,-0.585,-0.58,-0.575,-0.57,-0.565,-0.56,-0.555,
-0.55,-0.545,-0.54,-0.535,-0.53,-0.525,-0.52,-0.515,-0.51,-0.505,-0.5,-0.495,
-0.49,-0.485,-0.48,-0.475,-0.47,-0.465,-0.46,-0.455,-0.45,-0.445,-0.44,
-0.435,-0.43,-0.425,-0.42,-0.415,-0.41,-0.405,-0.4,-0.395,-0.39,-0.385,
-0.38,-0.375,-0.37,-0.365,-0.36,-0.355,-0.35,-0.345,-0.34,-0.335,-0.33,
-0.325,-0.32,-0.315,-0.31,-0.305,-0.3,-0.295,-0.29,-0.285,-0.28,-0.275,
-0.27,-0.265,-0.26,-0.255,-0.25,-0.245,-0.24,-0.235,-0.23,-0.225,-0.22,
-0.215,-0.21,-0.205,-0.2,-0.195,-0.19,-0.185,-0.18,-0.175,-0.17,-0.165,
-0.16,-0.155,-0.15,-0.145,-0.14,-0.135,-0.13,-0.125,-0.12,-0.115,-0.11,
-0.105,-0.1,-0.095,-0.09,-0.085,-0.08,-0.075,-0.07,-0.065,-0.06,-0.055,
-0.05,-0.045,-0.04,-0.035,-0.03,-0.025,-0.02,-0.015,-0.01,-0.005,0.),
 .UNSPECIFIED.)
CURVE()
GEOMETRIC_REPRESENTATION_ITEM()
RATIONAL_B_SPLINE_CURVE((1.,1.,1.,1.,1.,1.,1.,1.,1.,1.,1.,1.,1.,1.,1.,1.,
1.,1.,1.,1.,1.,1.,1.,1.,1.,1.,1.,1.,1.,1.,1.,1.,1.,1.,1.,1.,1.,1.,1.,1.,
1.,1.,1.,1.,1.,1.,1.,1.,1.,1.,1.,1.,1.,1.,1.,1.,1.,1.,1.,1.,1.,1.,1.,1.,
1.,1.,1.,1.,1.,1.,1.,1.,1.,1.,1.,1.,1.,1.,1.,1.,1.,1.,1.,1.,1.,1.,1.,1.,
1.,1.,1.,1.,1.,1.,1.,1.,1.,1.,1.,1.,1.,1.,1.,1.,1.,1.,1.,1.,1.,1.,1.,1.,
1.,1.,1.,1.,1.,1.,1.,1.,1.,1.,1.,1.,1.,1.,1.,1.,1.,1.,1.,1.,1.,1.,1.,1.,
1.,1.,1.,1.,1.,1.,1.,1.,1.,1.,1.,1.,1.,1.,1.,1.,1.,1.,1.,1.,1.,1.,1.,1.,
1.,1.,1.,1.,1.,1.,1.,1.,1.,1.,1.,1.,1.,1.,1.,1.,1.,1.,1.,1.,1.,1.,1.,1.,
1.,1.,1.,1.,1.,1.,1.,1.,1.,1.))
REPRESENTATION_ITEM('')
);
#409=(
BOUNDED_CURVE()
B_SPLINE_CURVE(5,(#55721,#55722,#55723,#55724,#55725,#55726,#55727,#55728,
#55729,#55730,#55731,#55732,#55733,#55734,#55735,#55736,#55737,#55738,#55739,
#55740,#55741,#55742,#55743,#55744,#55745,#55746,#55747,#55748,#55749,#55750,
#55751,#55752,#55753,#55754,#55755,#55756,#55757,#55758,#55759,#55760,#55761,
#55762,#55763,#55764,#55765,#55766,#55767,#55768,#55769,#55770,#55771,#55772,
#55773,#55774,#55775,#55776,#55777,#55778,#55779,#55780,#55781,#55782,#55783,
#55784,#55785,#55786,#55787,#55788,#55789,#55790,#55791,#55792,#55793,#55794,
#55795,#55796,#55797,#55798,#55799,#55800,#55801,#55802,#55803,#55804,#55805,
#55806,#55807,#55808,#55809,#55810,#55811,#55812,#55813,#55814,#55815,#55816,
#55817,#55818,#55819,#55820,#55821,#55822,#55823,#55824,#55825,#55826,#55827,
#55828,#55829,#55830,#55831,#55832,#55833,#55834,#55835,#55836,#55837,#55838,
#55839,#55840,#55841,#55842,#55843,#55844,#55845,#55846,#55847,#55848,#55849,
#55850,#55851,#55852,#55853,#55854,#55855,#55856,#55857,#55858,#55859,#55860,
#55861,#55862,#55863,#55864,#55865,#55866,#55867,#55868,#55869,#55870,#55871,
#55872,#55873,#55874,#55875,#55876,#55877,#55878,#55879,#55880,#55881,#55882,
#55883,#55884,#55885,#55886,#55887,#55888,#55889,#55890,#55891,#55892,#55893,
#55894,#55895,#55896,#55897,#55898,#55899,#55900,#55901,#55902,#55903,#55904,
#55905,#55906,#55907,#55908,#55909,#55910,#55911,#55912,#55913,#55914),
 .UNSPECIFIED.,.F.,.F.)
B_SPLINE_CURVE_WITH_KNOTS((6,1,1,1,1,1,1,1,1,1,1,1,1,1,1,1,1,1,1,1,1,1,
1,1,1,1,1,1,1,1,1,1,1,1,1,1,1,1,1,1,1,1,1,1,1,1,1,1,1,1,1,1,1,1,1,1,1,1,
1,1,1,1,1,1,1,1,1,1,1,1,1,1,1,1,1,1,1,1,1,1,1,1,1,1,1,1,1,1,1,1,1,1,1,1,
1,1,1,1,1,1,1,1,1,1,1,1,1,1,1,1,1,1,1,1,1,1,1,1,1,1,1,1,1,1,1,1,1,1,1,1,
1,1,1,1,1,1,1,1,1,1,1,1,1,1,1,1,1,1,1,1,1,1,1,1,1,1,1,1,1,1,1,1,1,1,1,1,
1,1,1,1,1,1,1,1,1,1,1,1,1,1,1,1,1,1,1,1,1,1,1,6),(0.,0.005,0.01,0.015,0.02,
0.025,0.03,0.035,0.04,0.045,0.05,0.055,0.06,0.065,0.07,0.075,0.08,0.085,
0.09,0.095,0.1,0.105,0.11,0.115,0.12,0.125,0.13,0.135,0.14,0.145,0.15,0.155,
0.16,0.165,0.17,0.175,0.18,0.185,0.19,0.195,0.2,0.205,0.21,0.215,0.22,0.225,
0.23,0.235,0.24,0.245,0.25,0.255,0.26,0.265,0.27,0.275,0.28,0.285,0.29,
0.295,0.3,0.305,0.31,0.315,0.32,0.325,0.33,0.335,0.34,0.345,0.35,0.355,
0.36,0.365,0.37,0.375,0.38,0.385,0.39,0.395,0.4,0.405,0.41,0.415,0.42,0.425,
0.43,0.435,0.44,0.445,0.45,0.455,0.46,0.465,0.47,0.475,0.48,0.485,0.49,
0.495,0.5,0.505,0.51,0.515,0.52,0.525,0.53,0.535,0.54,0.545,0.55,0.555,
0.56,0.565,0.57,0.575,0.58,0.585,0.59,0.595,0.6,0.605,0.61,0.615,0.62,0.625,
0.63,0.635,0.64,0.645,0.65,0.655,0.66,0.665,0.67,0.675,0.68,0.685,0.690000000000001,
0.695000000000001,0.700000000000001,0.705000000000001,0.710000000000001,
0.715000000000001,0.720000000000001,0.725000000000001,0.730000000000001,
0.735000000000001,0.740000000000001,0.745000000000001,0.750000000000001,
0.755000000000001,0.760000000000001,0.765000000000001,0.770000000000001,
0.775000000000001,0.780000000000001,0.785000000000001,0.790000000000001,
0.795000000000001,0.800000000000001,0.805000000000001,0.810000000000001,
0.815000000000001,0.820000000000001,0.825000000000001,0.830000000000001,
0.835000000000001,0.840000000000001,0.845000000000001,0.850000000000001,
0.855000000000001,0.860000000000001,0.865000000000001,0.870000000000001,
0.875000000000001,0.880000000000001,0.885000000000001,0.890000000000001,
0.895000000000001,0.900000000000001,0.905000000000001,0.910000000000001,
0.915000000000001,0.920000000000001,0.925000000000001,0.930000000000001,
0.935000000000001,0.940000000000001,0.941429844431425),.UNSPECIFIED.)
CURVE()
GEOMETRIC_REPRESENTATION_ITEM()
RATIONAL_B_SPLINE_CURVE((1.,1.,1.,1.,1.,1.,1.,1.,1.,1.,1.,1.,1.,1.,1.,1.,
1.,1.,1.,1.,1.,1.,1.,1.,1.,1.,1.,1.,1.,1.,1.,1.,1.,1.,1.,1.,1.,1.,1.,1.,
1.,1.,1.,1.,1.,1.,1.,1.,1.,1.,1.,1.,1.,1.,1.,1.,1.,1.,1.,1.,1.,1.,1.,1.,
1.,1.,1.,1.,1.,1.,1.,1.,1.,1.,1.,1.,1.,1.,1.,1.,1.,1.,1.,1.,1.,1.,1.,1.,
1.,1.,1.,1.,1.,1.,1.,1.,1.,1.,1.,1.,1.,1.,1.,1.,1.,1.,1.,1.,1.,1.,1.,1.,
1.,1.,1.,1.,1.,1.,1.,1.,1.,1.,1.,1.,1.,1.,1.,1.,1.,1.,1.,1.,1.,1.,1.,1.,
1.,1.,1.,1.,1.,1.,1.,1.,1.,1.,1.,1.,1.,1.,1.,1.,1.,1.,1.,1.,1.,1.,1.,1.,
1.,1.,1.,1.,1.,1.,1.,1.,1.,1.,1.,1.,1.,1.,1.,1.,1.,1.,1.,1.,1.,1.,1.,1.,
1.,1.,1.,1.,1.,1.,1.,1.,1.,1.))
REPRESENTATION_ITEM('')
);
#410=(
BOUNDED_CURVE()
B_SPLINE_CURVE(5,(#55917,#55918,#55919,#55920,#55921,#55922,#55923,#55924,
#55925,#55926,#55927,#55928,#55929,#55930,#55931,#55932,#55933,#55934,#55935,
#55936,#55937,#55938,#55939,#55940,#55941,#55942,#55943,#55944,#55945,#55946,
#55947,#55948,#55949,#55950,#55951,#55952,#55953,#55954,#55955,#55956,#55957,
#55958,#55959,#55960,#55961,#55962,#55963,#55964,#55965,#55966,#55967,#55968,
#55969,#55970,#55971,#55972,#55973,#55974,#55975,#55976,#55977,#55978,#55979,
#55980,#55981,#55982,#55983,#55984,#55985,#55986,#55987,#55988,#55989,#55990,
#55991,#55992,#55993,#55994,#55995,#55996,#55997,#55998,#55999,#56000,#56001,
#56002,#56003,#56004,#56005,#56006,#56007,#56008,#56009,#56010,#56011,#56012,
#56013,#56014,#56015,#56016,#56017,#56018,#56019,#56020,#56021,#56022,#56023,
#56024,#56025,#56026,#56027,#56028,#56029,#56030,#56031,#56032,#56033,#56034,
#56035,#56036,#56037,#56038,#56039,#56040,#56041,#56042,#56043,#56044,#56045,
#56046,#56047,#56048,#56049,#56050,#56051,#56052,#56053,#56054,#56055,#56056,
#56057,#56058,#56059,#56060,#56061,#56062,#56063,#56064,#56065,#56066,#56067,
#56068,#56069,#56070,#56071,#56072,#56073,#56074,#56075,#56076,#56077,#56078,
#56079,#56080,#56081,#56082,#56083,#56084,#56085,#56086,#56087,#56088,#56089,
#56090,#56091,#56092,#56093,#56094,#56095,#56096,#56097,#56098,#56099,#56100,
#56101,#56102,#56103,#56104,#56105,#56106,#56107,#56108,#56109,#56110),
 .UNSPECIFIED.,.F.,.F.)
B_SPLINE_CURVE_WITH_KNOTS((6,1,1,1,1,1,1,1,1,1,1,1,1,1,1,1,1,1,1,1,1,1,
1,1,1,1,1,1,1,1,1,1,1,1,1,1,1,1,1,1,1,1,1,1,1,1,1,1,1,1,1,1,1,1,1,1,1,1,
1,1,1,1,1,1,1,1,1,1,1,1,1,1,1,1,1,1,1,1,1,1,1,1,1,1,1,1,1,1,1,1,1,1,1,1,
1,1,1,1,1,1,1,1,1,1,1,1,1,1,1,1,1,1,1,1,1,1,1,1,1,1,1,1,1,1,1,1,1,1,1,1,
1,1,1,1,1,1,1,1,1,1,1,1,1,1,1,1,1,1,1,1,1,1,1,1,1,1,1,1,1,1,1,1,1,1,1,1,
1,1,1,1,1,1,1,1,1,1,1,1,1,1,1,1,1,1,1,1,1,1,1,6),(-0.941429844431423,-0.940000000000001,
-0.935000000000001,-0.930000000000001,-0.925000000000001,-0.920000000000001,
-0.915000000000001,-0.910000000000001,-0.905000000000001,-0.900000000000001,
-0.895000000000001,-0.890000000000001,-0.885000000000001,-0.880000000000001,
-0.875000000000001,-0.870000000000001,-0.865000000000001,-0.860000000000001,
-0.855000000000001,-0.850000000000001,-0.845000000000001,-0.840000000000001,
-0.835000000000001,-0.830000000000001,-0.825000000000001,-0.820000000000001,
-0.815000000000001,-0.810000000000001,-0.805000000000001,-0.800000000000001,
-0.795000000000001,-0.790000000000001,-0.785000000000001,-0.780000000000001,
-0.775000000000001,-0.770000000000001,-0.765000000000001,-0.760000000000001,
-0.755000000000001,-0.750000000000001,-0.745000000000001,-0.740000000000001,
-0.735000000000001,-0.730000000000001,-0.725000000000001,-0.720000000000001,
-0.715000000000001,-0.710000000000001,-0.705000000000001,-0.700000000000001,
-0.695000000000001,-0.690000000000001,-0.685,-0.68,-0.675,-0.67,-0.665,
-0.66,-0.655,-0.65,-0.645,-0.64,-0.635,-0.63,-0.625,-0.62,-0.615,-0.61,
-0.605,-0.6,-0.595,-0.59,-0.585,-0.58,-0.575,-0.57,-0.565,-0.56,-0.555,
-0.55,-0.545,-0.54,-0.535,-0.53,-0.525,-0.52,-0.515,-0.51,-0.505,-0.5,-0.495,
-0.49,-0.485,-0.48,-0.475,-0.47,-0.465,-0.46,-0.455,-0.45,-0.445,-0.44,
-0.435,-0.43,-0.425,-0.42,-0.415,-0.41,-0.405,-0.4,-0.395,-0.39,-0.385,
-0.38,-0.375,-0.37,-0.365,-0.36,-0.355,-0.35,-0.345,-0.34,-0.335,-0.33,
-0.325,-0.32,-0.315,-0.31,-0.305,-0.3,-0.295,-0.29,-0.285,-0.28,-0.275,
-0.27,-0.265,-0.26,-0.255,-0.25,-0.245,-0.24,-0.235,-0.23,-0.225,-0.22,
-0.215,-0.21,-0.205,-0.2,-0.195,-0.19,-0.185,-0.18,-0.175,-0.17,-0.165,
-0.16,-0.155,-0.15,-0.145,-0.14,-0.135,-0.13,-0.125,-0.12,-0.115,-0.11,
-0.105,-0.1,-0.095,-0.09,-0.085,-0.08,-0.075,-0.07,-0.065,-0.06,-0.055,
-0.05,-0.045,-0.04,-0.035,-0.03,-0.025,-0.02,-0.015,-0.01,-0.005,0.),
 .UNSPECIFIED.)
CURVE()
GEOMETRIC_REPRESENTATION_ITEM()
RATIONAL_B_SPLINE_CURVE((1.,1.,1.,1.,1.,1.,1.,1.,1.,1.,1.,1.,1.,1.,1.,1.,
1.,1.,1.,1.,1.,1.,1.,1.,1.,1.,1.,1.,1.,1.,1.,1.,1.,1.,1.,1.,1.,1.,1.,1.,
1.,1.,1.,1.,1.,1.,1.,1.,1.,1.,1.,1.,1.,1.,1.,1.,1.,1.,1.,1.,1.,1.,1.,1.,
1.,1.,1.,1.,1.,1.,1.,1.,1.,1.,1.,1.,1.,1.,1.,1.,1.,1.,1.,1.,1.,1.,1.,1.,
1.,1.,1.,1.,1.,1.,1.,1.,1.,1.,1.,1.,1.,1.,1.,1.,1.,1.,1.,1.,1.,1.,1.,1.,
1.,1.,1.,1.,1.,1.,1.,1.,1.,1.,1.,1.,1.,1.,1.,1.,1.,1.,1.,1.,1.,1.,1.,1.,
1.,1.,1.,1.,1.,1.,1.,1.,1.,1.,1.,1.,1.,1.,1.,1.,1.,1.,1.,1.,1.,1.,1.,1.,
1.,1.,1.,1.,1.,1.,1.,1.,1.,1.,1.,1.,1.,1.,1.,1.,1.,1.,1.,1.,1.,1.,1.,1.,
1.,1.,1.,1.,1.,1.,1.,1.,1.,1.))
REPRESENTATION_ITEM('')
);
#411=(
BOUNDED_CURVE()
B_SPLINE_CURVE(5,(#56617,#56618,#56619,#56620,#56621,#56622,#56623,#56624,
#56625,#56626,#56627,#56628,#56629,#56630,#56631,#56632,#56633,#56634,#56635,
#56636,#56637,#56638,#56639,#56640,#56641,#56642,#56643,#56644,#56645,#56646,
#56647,#56648,#56649,#56650,#56651,#56652,#56653,#56654,#56655,#56656,#56657,
#56658,#56659,#56660,#56661,#56662,#56663,#56664,#56665,#56666,#56667,#56668,
#56669,#56670,#56671,#56672,#56673,#56674,#56675,#56676,#56677,#56678,#56679,
#56680,#56681,#56682,#56683,#56684,#56685,#56686,#56687,#56688,#56689,#56690,
#56691,#56692,#56693,#56694,#56695,#56696,#56697,#56698,#56699,#56700,#56701,
#56702,#56703,#56704,#56705,#56706,#56707,#56708,#56709,#56710,#56711,#56712,
#56713,#56714,#56715,#56716,#56717,#56718,#56719,#56720,#56721,#56722,#56723,
#56724,#56725,#56726,#56727,#56728,#56729,#56730,#56731,#56732,#56733,#56734,
#56735,#56736,#56737,#56738,#56739,#56740,#56741,#56742,#56743,#56744,#56745,
#56746,#56747,#56748,#56749,#56750,#56751,#56752,#56753,#56754,#56755,#56756,
#56757,#56758,#56759,#56760,#56761,#56762,#56763,#56764,#56765,#56766,#56767,
#56768,#56769,#56770,#56771,#56772,#56773,#56774,#56775,#56776,#56777,#56778,
#56779,#56780,#56781,#56782,#56783,#56784,#56785,#56786,#56787,#56788,#56789,
#56790,#56791,#56792,#56793,#56794,#56795,#56796,#56797,#56798,#56799,#56800,
#56801,#56802,#56803,#56804,#56805,#56806,#56807,#56808,#56809,#56810),
 .UNSPECIFIED.,.F.,.F.)
B_SPLINE_CURVE_WITH_KNOTS((6,1,1,1,1,1,1,1,1,1,1,1,1,1,1,1,1,1,1,1,1,1,
1,1,1,1,1,1,1,1,1,1,1,1,1,1,1,1,1,1,1,1,1,1,1,1,1,1,1,1,1,1,1,1,1,1,1,1,
1,1,1,1,1,1,1,1,1,1,1,1,1,1,1,1,1,1,1,1,1,1,1,1,1,1,1,1,1,1,1,1,1,1,1,1,
1,1,1,1,1,1,1,1,1,1,1,1,1,1,1,1,1,1,1,1,1,1,1,1,1,1,1,1,1,1,1,1,1,1,1,1,
1,1,1,1,1,1,1,1,1,1,1,1,1,1,1,1,1,1,1,1,1,1,1,1,1,1,1,1,1,1,1,1,1,1,1,1,
1,1,1,1,1,1,1,1,1,1,1,1,1,1,1,1,1,1,1,1,1,1,1,6),(0.,0.005,0.01,0.015,0.02,
0.025,0.03,0.035,0.04,0.045,0.05,0.055,0.06,0.065,0.07,0.075,0.08,0.085,
0.09,0.095,0.1,0.105,0.11,0.115,0.12,0.125,0.13,0.135,0.14,0.145,0.15,0.155,
0.16,0.165,0.17,0.175,0.18,0.185,0.19,0.195,0.2,0.205,0.21,0.215,0.22,0.225,
0.23,0.235,0.24,0.245,0.25,0.255,0.26,0.265,0.27,0.275,0.28,0.285,0.29,
0.295,0.3,0.305,0.31,0.315,0.32,0.325,0.33,0.335,0.34,0.345,0.35,0.355,
0.36,0.365,0.37,0.375,0.38,0.385,0.39,0.395,0.4,0.405,0.41,0.415,0.42,0.425,
0.43,0.435,0.44,0.445,0.45,0.455,0.46,0.465,0.47,0.475,0.48,0.485,0.49,
0.495,0.5,0.505,0.51,0.515,0.52,0.525,0.53,0.535,0.54,0.545,0.55,0.555,
0.56,0.565,0.57,0.575,0.58,0.585,0.59,0.595,0.6,0.605,0.61,0.615,0.62,0.625,
0.63,0.635,0.64,0.645,0.65,0.655,0.66,0.665,0.67,0.675,0.68,0.685,0.690000000000001,
0.695000000000001,0.700000000000001,0.705000000000001,0.710000000000001,
0.715000000000001,0.720000000000001,0.725000000000001,0.730000000000001,
0.735000000000001,0.740000000000001,0.745000000000001,0.750000000000001,
0.755000000000001,0.760000000000001,0.765000000000001,0.770000000000001,
0.775000000000001,0.780000000000001,0.785000000000001,0.790000000000001,
0.795000000000001,0.800000000000001,0.805000000000001,0.810000000000001,
0.815000000000001,0.820000000000001,0.825000000000001,0.830000000000001,
0.835000000000001,0.840000000000001,0.845000000000001,0.850000000000001,
0.855000000000001,0.860000000000001,0.865000000000001,0.870000000000001,
0.875000000000001,0.880000000000001,0.885000000000001,0.890000000000001,
0.895000000000001,0.900000000000001,0.905000000000001,0.910000000000001,
0.915000000000001,0.920000000000001,0.925000000000001,0.930000000000001,
0.935000000000001,0.940000000000001,0.941429844431363),.UNSPECIFIED.)
CURVE()
GEOMETRIC_REPRESENTATION_ITEM()
RATIONAL_B_SPLINE_CURVE((1.,1.,1.,1.,1.,1.,1.,1.,1.,1.,1.,1.,1.,1.,1.,1.,
1.,1.,1.,1.,1.,1.,1.,1.,1.,1.,1.,1.,1.,1.,1.,1.,1.,1.,1.,1.,1.,1.,1.,1.,
1.,1.,1.,1.,1.,1.,1.,1.,1.,1.,1.,1.,1.,1.,1.,1.,1.,1.,1.,1.,1.,1.,1.,1.,
1.,1.,1.,1.,1.,1.,1.,1.,1.,1.,1.,1.,1.,1.,1.,1.,1.,1.,1.,1.,1.,1.,1.,1.,
1.,1.,1.,1.,1.,1.,1.,1.,1.,1.,1.,1.,1.,1.,1.,1.,1.,1.,1.,1.,1.,1.,1.,1.,
1.,1.,1.,1.,1.,1.,1.,1.,1.,1.,1.,1.,1.,1.,1.,1.,1.,1.,1.,1.,1.,1.,1.,1.,
1.,1.,1.,1.,1.,1.,1.,1.,1.,1.,1.,1.,1.,1.,1.,1.,1.,1.,1.,1.,1.,1.,1.,1.,
1.,1.,1.,1.,1.,1.,1.,1.,1.,1.,1.,1.,1.,1.,1.,1.,1.,1.,1.,1.,1.,1.,1.,1.,
1.,1.,1.,1.,1.,1.,1.,1.,1.,1.))
REPRESENTATION_ITEM('')
);
#412=(
BOUNDED_CURVE()
B_SPLINE_CURVE(5,(#56813,#56814,#56815,#56816,#56817,#56818,#56819,#56820,
#56821,#56822,#56823,#56824,#56825,#56826,#56827,#56828,#56829,#56830,#56831,
#56832,#56833,#56834,#56835,#56836,#56837,#56838,#56839,#56840,#56841,#56842,
#56843,#56844,#56845,#56846,#56847,#56848,#56849,#56850,#56851,#56852,#56853,
#56854,#56855,#56856,#56857,#56858,#56859,#56860,#56861,#56862,#56863,#56864,
#56865,#56866,#56867,#56868,#56869,#56870,#56871,#56872,#56873,#56874,#56875,
#56876,#56877,#56878,#56879,#56880,#56881,#56882,#56883,#56884,#56885,#56886,
#56887,#56888,#56889,#56890,#56891,#56892,#56893,#56894,#56895,#56896,#56897,
#56898,#56899,#56900,#56901,#56902,#56903,#56904,#56905,#56906,#56907,#56908,
#56909,#56910,#56911,#56912,#56913,#56914,#56915,#56916,#56917,#56918,#56919,
#56920,#56921,#56922,#56923,#56924,#56925,#56926,#56927,#56928,#56929,#56930,
#56931,#56932,#56933,#56934,#56935,#56936,#56937,#56938,#56939,#56940,#56941,
#56942,#56943,#56944,#56945,#56946,#56947,#56948,#56949,#56950,#56951,#56952,
#56953,#56954,#56955,#56956,#56957,#56958,#56959,#56960,#56961,#56962,#56963,
#56964,#56965,#56966,#56967,#56968,#56969,#56970,#56971,#56972,#56973,#56974,
#56975,#56976,#56977,#56978,#56979,#56980,#56981,#56982,#56983,#56984,#56985,
#56986,#56987,#56988,#56989,#56990,#56991,#56992,#56993,#56994,#56995,#56996,
#56997,#56998,#56999,#57000,#57001,#57002,#57003,#57004,#57005,#57006),
 .UNSPECIFIED.,.F.,.F.)
B_SPLINE_CURVE_WITH_KNOTS((6,1,1,1,1,1,1,1,1,1,1,1,1,1,1,1,1,1,1,1,1,1,
1,1,1,1,1,1,1,1,1,1,1,1,1,1,1,1,1,1,1,1,1,1,1,1,1,1,1,1,1,1,1,1,1,1,1,1,
1,1,1,1,1,1,1,1,1,1,1,1,1,1,1,1,1,1,1,1,1,1,1,1,1,1,1,1,1,1,1,1,1,1,1,1,
1,1,1,1,1,1,1,1,1,1,1,1,1,1,1,1,1,1,1,1,1,1,1,1,1,1,1,1,1,1,1,1,1,1,1,1,
1,1,1,1,1,1,1,1,1,1,1,1,1,1,1,1,1,1,1,1,1,1,1,1,1,1,1,1,1,1,1,1,1,1,1,1,
1,1,1,1,1,1,1,1,1,1,1,1,1,1,1,1,1,1,1,1,1,1,1,6),(-0.941429844431365,-0.940000000000001,
-0.935000000000001,-0.930000000000001,-0.925000000000001,-0.920000000000001,
-0.915000000000001,-0.910000000000001,-0.905000000000001,-0.900000000000001,
-0.895000000000001,-0.890000000000001,-0.885000000000001,-0.880000000000001,
-0.875000000000001,-0.870000000000001,-0.865000000000001,-0.860000000000001,
-0.855000000000001,-0.850000000000001,-0.845000000000001,-0.840000000000001,
-0.835000000000001,-0.830000000000001,-0.825000000000001,-0.820000000000001,
-0.815000000000001,-0.810000000000001,-0.805000000000001,-0.800000000000001,
-0.795000000000001,-0.790000000000001,-0.785000000000001,-0.780000000000001,
-0.775000000000001,-0.770000000000001,-0.765000000000001,-0.760000000000001,
-0.755000000000001,-0.750000000000001,-0.745000000000001,-0.740000000000001,
-0.735000000000001,-0.730000000000001,-0.725000000000001,-0.720000000000001,
-0.715000000000001,-0.710000000000001,-0.705000000000001,-0.700000000000001,
-0.695000000000001,-0.690000000000001,-0.685,-0.68,-0.675,-0.67,-0.665,
-0.66,-0.655,-0.65,-0.645,-0.64,-0.635,-0.63,-0.625,-0.62,-0.615,-0.61,
-0.605,-0.6,-0.595,-0.59,-0.585,-0.58,-0.575,-0.57,-0.565,-0.56,-0.555,
-0.55,-0.545,-0.54,-0.535,-0.53,-0.525,-0.52,-0.515,-0.51,-0.505,-0.5,-0.495,
-0.49,-0.485,-0.48,-0.475,-0.47,-0.465,-0.46,-0.455,-0.45,-0.445,-0.44,
-0.435,-0.43,-0.425,-0.42,-0.415,-0.41,-0.405,-0.4,-0.395,-0.39,-0.385,
-0.38,-0.375,-0.37,-0.365,-0.36,-0.355,-0.35,-0.345,-0.34,-0.335,-0.33,
-0.325,-0.32,-0.315,-0.31,-0.305,-0.3,-0.295,-0.29,-0.285,-0.28,-0.275,
-0.27,-0.265,-0.26,-0.255,-0.25,-0.245,-0.24,-0.235,-0.23,-0.225,-0.22,
-0.215,-0.21,-0.205,-0.2,-0.195,-0.19,-0.185,-0.18,-0.175,-0.17,-0.165,
-0.16,-0.155,-0.15,-0.145,-0.14,-0.135,-0.13,-0.125,-0.12,-0.115,-0.11,
-0.105,-0.1,-0.095,-0.09,-0.085,-0.08,-0.075,-0.07,-0.065,-0.06,-0.055,
-0.05,-0.045,-0.04,-0.035,-0.03,-0.025,-0.02,-0.015,-0.01,-0.005,0.),
 .UNSPECIFIED.)
CURVE()
GEOMETRIC_REPRESENTATION_ITEM()
RATIONAL_B_SPLINE_CURVE((1.,1.,1.,1.,1.,1.,1.,1.,1.,1.,1.,1.,1.,1.,1.,1.,
1.,1.,1.,1.,1.,1.,1.,1.,1.,1.,1.,1.,1.,1.,1.,1.,1.,1.,1.,1.,1.,1.,1.,1.,
1.,1.,1.,1.,1.,1.,1.,1.,1.,1.,1.,1.,1.,1.,1.,1.,1.,1.,1.,1.,1.,1.,1.,1.,
1.,1.,1.,1.,1.,1.,1.,1.,1.,1.,1.,1.,1.,1.,1.,1.,1.,1.,1.,1.,1.,1.,1.,1.,
1.,1.,1.,1.,1.,1.,1.,1.,1.,1.,1.,1.,1.,1.,1.,1.,1.,1.,1.,1.,1.,1.,1.,1.,
1.,1.,1.,1.,1.,1.,1.,1.,1.,1.,1.,1.,1.,1.,1.,1.,1.,1.,1.,1.,1.,1.,1.,1.,
1.,1.,1.,1.,1.,1.,1.,1.,1.,1.,1.,1.,1.,1.,1.,1.,1.,1.,1.,1.,1.,1.,1.,1.,
1.,1.,1.,1.,1.,1.,1.,1.,1.,1.,1.,1.,1.,1.,1.,1.,1.,1.,1.,1.,1.,1.,1.,1.,
1.,1.,1.,1.,1.,1.,1.,1.,1.,1.))
REPRESENTATION_ITEM('')
);
#413=(
BOUNDED_CURVE()
B_SPLINE_CURVE(5,(#57513,#57514,#57515,#57516,#57517,#57518,#57519,#57520,
#57521,#57522,#57523,#57524,#57525,#57526,#57527,#57528,#57529,#57530,#57531,
#57532,#57533,#57534,#57535,#57536,#57537,#57538,#57539,#57540,#57541,#57542,
#57543,#57544,#57545,#57546,#57547,#57548,#57549,#57550,#57551,#57552,#57553,
#57554,#57555,#57556,#57557,#57558,#57559,#57560,#57561,#57562,#57563,#57564,
#57565,#57566,#57567,#57568,#57569,#57570,#57571,#57572,#57573,#57574,#57575,
#57576,#57577,#57578,#57579,#57580,#57581,#57582,#57583,#57584,#57585,#57586,
#57587,#57588,#57589,#57590,#57591,#57592,#57593,#57594,#57595,#57596,#57597,
#57598,#57599,#57600,#57601,#57602,#57603,#57604,#57605,#57606,#57607,#57608,
#57609,#57610,#57611,#57612,#57613,#57614,#57615,#57616,#57617,#57618,#57619,
#57620,#57621,#57622,#57623,#57624,#57625,#57626,#57627,#57628,#57629,#57630,
#57631,#57632,#57633,#57634,#57635,#57636,#57637,#57638,#57639,#57640,#57641,
#57642,#57643,#57644,#57645,#57646,#57647,#57648,#57649,#57650,#57651,#57652,
#57653,#57654,#57655,#57656,#57657,#57658,#57659,#57660,#57661,#57662,#57663,
#57664,#57665,#57666,#57667,#57668,#57669,#57670,#57671,#57672,#57673,#57674,
#57675,#57676,#57677,#57678,#57679,#57680,#57681,#57682,#57683,#57684,#57685,
#57686,#57687,#57688,#57689,#57690,#57691,#57692,#57693,#57694,#57695,#57696,
#57697,#57698,#57699,#57700,#57701,#57702,#57703,#57704,#57705,#57706),
 .UNSPECIFIED.,.F.,.F.)
B_SPLINE_CURVE_WITH_KNOTS((6,1,1,1,1,1,1,1,1,1,1,1,1,1,1,1,1,1,1,1,1,1,
1,1,1,1,1,1,1,1,1,1,1,1,1,1,1,1,1,1,1,1,1,1,1,1,1,1,1,1,1,1,1,1,1,1,1,1,
1,1,1,1,1,1,1,1,1,1,1,1,1,1,1,1,1,1,1,1,1,1,1,1,1,1,1,1,1,1,1,1,1,1,1,1,
1,1,1,1,1,1,1,1,1,1,1,1,1,1,1,1,1,1,1,1,1,1,1,1,1,1,1,1,1,1,1,1,1,1,1,1,
1,1,1,1,1,1,1,1,1,1,1,1,1,1,1,1,1,1,1,1,1,1,1,1,1,1,1,1,1,1,1,1,1,1,1,1,
1,1,1,1,1,1,1,1,1,1,1,1,1,1,1,1,1,1,1,1,1,1,1,6),(0.,0.005,0.01,0.015,0.02,
0.025,0.03,0.035,0.04,0.045,0.05,0.055,0.06,0.065,0.07,0.075,0.08,0.085,
0.09,0.095,0.1,0.105,0.11,0.115,0.12,0.125,0.13,0.135,0.14,0.145,0.15,0.155,
0.16,0.165,0.17,0.175,0.18,0.185,0.19,0.195,0.2,0.205,0.21,0.215,0.22,0.225,
0.23,0.235,0.24,0.245,0.25,0.255,0.26,0.265,0.27,0.275,0.28,0.285,0.29,
0.295,0.3,0.305,0.31,0.315,0.32,0.325,0.33,0.335,0.34,0.345,0.35,0.355,
0.36,0.365,0.37,0.375,0.38,0.385,0.39,0.395,0.4,0.405,0.41,0.415,0.42,0.425,
0.43,0.435,0.44,0.445,0.45,0.455,0.46,0.465,0.47,0.475,0.48,0.485,0.49,
0.495,0.5,0.505,0.51,0.515,0.52,0.525,0.53,0.535,0.54,0.545,0.55,0.555,
0.56,0.565,0.57,0.575,0.58,0.585,0.59,0.595,0.6,0.605,0.61,0.615,0.62,0.625,
0.63,0.635,0.64,0.645,0.65,0.655,0.66,0.665,0.67,0.675,0.68,0.685,0.690000000000001,
0.695000000000001,0.700000000000001,0.705000000000001,0.710000000000001,
0.715000000000001,0.720000000000001,0.725000000000001,0.730000000000001,
0.735000000000001,0.740000000000001,0.745000000000001,0.750000000000001,
0.755000000000001,0.760000000000001,0.765000000000001,0.770000000000001,
0.775000000000001,0.780000000000001,0.785000000000001,0.790000000000001,
0.795000000000001,0.800000000000001,0.805000000000001,0.810000000000001,
0.815000000000001,0.820000000000001,0.825000000000001,0.830000000000001,
0.835000000000001,0.840000000000001,0.845000000000001,0.850000000000001,
0.855000000000001,0.860000000000001,0.865000000000001,0.870000000000001,
0.875000000000001,0.880000000000001,0.885000000000001,0.890000000000001,
0.895000000000001,0.900000000000001,0.905000000000001,0.910000000000001,
0.915000000000001,0.920000000000001,0.925000000000001,0.930000000000001,
0.935000000000001,0.940000000000001,0.941429844431354),.UNSPECIFIED.)
CURVE()
GEOMETRIC_REPRESENTATION_ITEM()
RATIONAL_B_SPLINE_CURVE((1.,1.,1.,1.,1.,1.,1.,1.,1.,1.,1.,1.,1.,1.,1.,1.,
1.,1.,1.,1.,1.,1.,1.,1.,1.,1.,1.,1.,1.,1.,1.,1.,1.,1.,1.,1.,1.,1.,1.,1.,
1.,1.,1.,1.,1.,1.,1.,1.,1.,1.,1.,1.,1.,1.,1.,1.,1.,1.,1.,1.,1.,1.,1.,1.,
1.,1.,1.,1.,1.,1.,1.,1.,1.,1.,1.,1.,1.,1.,1.,1.,1.,1.,1.,1.,1.,1.,1.,1.,
1.,1.,1.,1.,1.,1.,1.,1.,1.,1.,1.,1.,1.,1.,1.,1.,1.,1.,1.,1.,1.,1.,1.,1.,
1.,1.,1.,1.,1.,1.,1.,1.,1.,1.,1.,1.,1.,1.,1.,1.,1.,1.,1.,1.,1.,1.,1.,1.,
1.,1.,1.,1.,1.,1.,1.,1.,1.,1.,1.,1.,1.,1.,1.,1.,1.,1.,1.,1.,1.,1.,1.,1.,
1.,1.,1.,1.,1.,1.,1.,1.,1.,1.,1.,1.,1.,1.,1.,1.,1.,1.,1.,1.,1.,1.,1.,1.,
1.,1.,1.,1.,1.,1.,1.,1.,1.,1.))
REPRESENTATION_ITEM('')
);
#414=(
BOUNDED_CURVE()
B_SPLINE_CURVE(5,(#57709,#57710,#57711,#57712,#57713,#57714,#57715,#57716,
#57717,#57718,#57719,#57720,#57721,#57722,#57723,#57724,#57725,#57726,#57727,
#57728,#57729,#57730,#57731,#57732,#57733,#57734,#57735,#57736,#57737,#57738,
#57739,#57740,#57741,#57742,#57743,#57744,#57745,#57746,#57747,#57748,#57749,
#57750,#57751,#57752,#57753,#57754,#57755,#57756,#57757,#57758,#57759,#57760,
#57761,#57762,#57763,#57764,#57765,#57766,#57767,#57768,#57769,#57770,#57771,
#57772,#57773,#57774,#57775,#57776,#57777,#57778,#57779,#57780,#57781,#57782,
#57783,#57784,#57785,#57786,#57787,#57788,#57789,#57790,#57791,#57792,#57793,
#57794,#57795,#57796,#57797,#57798,#57799,#57800,#57801,#57802,#57803,#57804,
#57805,#57806,#57807,#57808,#57809,#57810,#57811,#57812,#57813,#57814,#57815,
#57816,#57817,#57818,#57819,#57820,#57821,#57822,#57823,#57824,#57825,#57826,
#57827,#57828,#57829,#57830,#57831,#57832,#57833,#57834,#57835,#57836,#57837,
#57838,#57839,#57840,#57841,#57842,#57843,#57844,#57845,#57846,#57847,#57848,
#57849,#57850,#57851,#57852,#57853,#57854,#57855,#57856,#57857,#57858,#57859,
#57860,#57861,#57862,#57863,#57864,#57865,#57866,#57867,#57868,#57869,#57870,
#57871,#57872,#57873,#57874,#57875,#57876,#57877,#57878,#57879,#57880,#57881,
#57882,#57883,#57884,#57885,#57886,#57887,#57888,#57889,#57890,#57891,#57892,
#57893,#57894,#57895,#57896,#57897,#57898,#57899,#57900,#57901,#57902),
 .UNSPECIFIED.,.F.,.F.)
B_SPLINE_CURVE_WITH_KNOTS((6,1,1,1,1,1,1,1,1,1,1,1,1,1,1,1,1,1,1,1,1,1,
1,1,1,1,1,1,1,1,1,1,1,1,1,1,1,1,1,1,1,1,1,1,1,1,1,1,1,1,1,1,1,1,1,1,1,1,
1,1,1,1,1,1,1,1,1,1,1,1,1,1,1,1,1,1,1,1,1,1,1,1,1,1,1,1,1,1,1,1,1,1,1,1,
1,1,1,1,1,1,1,1,1,1,1,1,1,1,1,1,1,1,1,1,1,1,1,1,1,1,1,1,1,1,1,1,1,1,1,1,
1,1,1,1,1,1,1,1,1,1,1,1,1,1,1,1,1,1,1,1,1,1,1,1,1,1,1,1,1,1,1,1,1,1,1,1,
1,1,1,1,1,1,1,1,1,1,1,1,1,1,1,1,1,1,1,1,1,1,1,6),(-0.941429844431354,-0.940000000000001,
-0.935000000000001,-0.930000000000001,-0.925000000000001,-0.920000000000001,
-0.915000000000001,-0.910000000000001,-0.905000000000001,-0.900000000000001,
-0.895000000000001,-0.890000000000001,-0.885000000000001,-0.880000000000001,
-0.875000000000001,-0.870000000000001,-0.865000000000001,-0.860000000000001,
-0.855000000000001,-0.850000000000001,-0.845000000000001,-0.840000000000001,
-0.835000000000001,-0.830000000000001,-0.825000000000001,-0.820000000000001,
-0.815000000000001,-0.810000000000001,-0.805000000000001,-0.800000000000001,
-0.795000000000001,-0.790000000000001,-0.785000000000001,-0.780000000000001,
-0.775000000000001,-0.770000000000001,-0.765000000000001,-0.760000000000001,
-0.755000000000001,-0.750000000000001,-0.745000000000001,-0.740000000000001,
-0.735000000000001,-0.730000000000001,-0.725000000000001,-0.720000000000001,
-0.715000000000001,-0.710000000000001,-0.705000000000001,-0.700000000000001,
-0.695000000000001,-0.690000000000001,-0.685,-0.68,-0.675,-0.67,-0.665,
-0.66,-0.655,-0.65,-0.645,-0.64,-0.635,-0.63,-0.625,-0.62,-0.615,-0.61,
-0.605,-0.6,-0.595,-0.59,-0.585,-0.58,-0.575,-0.57,-0.565,-0.56,-0.555,
-0.55,-0.545,-0.54,-0.535,-0.53,-0.525,-0.52,-0.515,-0.51,-0.505,-0.5,-0.495,
-0.49,-0.485,-0.48,-0.475,-0.47,-0.465,-0.46,-0.455,-0.45,-0.445,-0.44,
-0.435,-0.43,-0.425,-0.42,-0.415,-0.41,-0.405,-0.4,-0.395,-0.39,-0.385,
-0.38,-0.375,-0.37,-0.365,-0.36,-0.355,-0.35,-0.345,-0.34,-0.335,-0.33,
-0.325,-0.32,-0.315,-0.31,-0.305,-0.3,-0.295,-0.29,-0.285,-0.28,-0.275,
-0.27,-0.265,-0.26,-0.255,-0.25,-0.245,-0.24,-0.235,-0.23,-0.225,-0.22,
-0.215,-0.21,-0.205,-0.2,-0.195,-0.19,-0.185,-0.18,-0.175,-0.17,-0.165,
-0.16,-0.155,-0.15,-0.145,-0.14,-0.135,-0.13,-0.125,-0.12,-0.115,-0.11,
-0.105,-0.1,-0.095,-0.09,-0.085,-0.08,-0.075,-0.07,-0.065,-0.06,-0.055,
-0.05,-0.045,-0.04,-0.035,-0.03,-0.025,-0.02,-0.015,-0.01,-0.005,0.),
 .UNSPECIFIED.)
CURVE()
GEOMETRIC_REPRESENTATION_ITEM()
RATIONAL_B_SPLINE_CURVE((1.,1.,1.,1.,1.,1.,1.,1.,1.,1.,1.,1.,1.,1.,1.,1.,
1.,1.,1.,1.,1.,1.,1.,1.,1.,1.,1.,1.,1.,1.,1.,1.,1.,1.,1.,1.,1.,1.,1.,1.,
1.,1.,1.,1.,1.,1.,1.,1.,1.,1.,1.,1.,1.,1.,1.,1.,1.,1.,1.,1.,1.,1.,1.,1.,
1.,1.,1.,1.,1.,1.,1.,1.,1.,1.,1.,1.,1.,1.,1.,1.,1.,1.,1.,1.,1.,1.,1.,1.,
1.,1.,1.,1.,1.,1.,1.,1.,1.,1.,1.,1.,1.,1.,1.,1.,1.,1.,1.,1.,1.,1.,1.,1.,
1.,1.,1.,1.,1.,1.,1.,1.,1.,1.,1.,1.,1.,1.,1.,1.,1.,1.,1.,1.,1.,1.,1.,1.,
1.,1.,1.,1.,1.,1.,1.,1.,1.,1.,1.,1.,1.,1.,1.,1.,1.,1.,1.,1.,1.,1.,1.,1.,
1.,1.,1.,1.,1.,1.,1.,1.,1.,1.,1.,1.,1.,1.,1.,1.,1.,1.,1.,1.,1.,1.,1.,1.,
1.,1.,1.,1.,1.,1.,1.,1.,1.,1.))
REPRESENTATION_ITEM('')
);
#415=(
BOUNDED_CURVE()
B_SPLINE_CURVE(5,(#58409,#58410,#58411,#58412,#58413,#58414,#58415,#58416,
#58417,#58418,#58419,#58420,#58421,#58422,#58423,#58424,#58425,#58426,#58427,
#58428,#58429,#58430,#58431,#58432,#58433,#58434,#58435,#58436,#58437,#58438,
#58439,#58440,#58441,#58442,#58443,#58444,#58445,#58446,#58447,#58448,#58449,
#58450,#58451,#58452,#58453,#58454,#58455,#58456,#58457,#58458,#58459,#58460,
#58461,#58462,#58463,#58464,#58465,#58466,#58467,#58468,#58469,#58470,#58471,
#58472,#58473,#58474,#58475,#58476,#58477,#58478,#58479,#58480,#58481,#58482,
#58483,#58484,#58485,#58486,#58487,#58488,#58489,#58490,#58491,#58492,#58493,
#58494,#58495,#58496,#58497,#58498,#58499,#58500,#58501,#58502,#58503,#58504,
#58505,#58506,#58507,#58508,#58509,#58510,#58511,#58512,#58513,#58514,#58515,
#58516,#58517,#58518,#58519,#58520,#58521,#58522,#58523,#58524,#58525,#58526,
#58527,#58528,#58529,#58530,#58531,#58532,#58533,#58534,#58535,#58536,#58537,
#58538,#58539,#58540,#58541,#58542,#58543,#58544,#58545,#58546,#58547,#58548,
#58549,#58550,#58551,#58552,#58553,#58554,#58555,#58556,#58557,#58558,#58559,
#58560,#58561,#58562,#58563,#58564,#58565,#58566,#58567,#58568,#58569,#58570,
#58571,#58572,#58573,#58574,#58575,#58576,#58577,#58578,#58579,#58580,#58581,
#58582,#58583,#58584,#58585,#58586,#58587,#58588,#58589,#58590,#58591,#58592,
#58593,#58594,#58595,#58596,#58597,#58598,#58599,#58600,#58601,#58602),
 .UNSPECIFIED.,.F.,.F.)
B_SPLINE_CURVE_WITH_KNOTS((6,1,1,1,1,1,1,1,1,1,1,1,1,1,1,1,1,1,1,1,1,1,
1,1,1,1,1,1,1,1,1,1,1,1,1,1,1,1,1,1,1,1,1,1,1,1,1,1,1,1,1,1,1,1,1,1,1,1,
1,1,1,1,1,1,1,1,1,1,1,1,1,1,1,1,1,1,1,1,1,1,1,1,1,1,1,1,1,1,1,1,1,1,1,1,
1,1,1,1,1,1,1,1,1,1,1,1,1,1,1,1,1,1,1,1,1,1,1,1,1,1,1,1,1,1,1,1,1,1,1,1,
1,1,1,1,1,1,1,1,1,1,1,1,1,1,1,1,1,1,1,1,1,1,1,1,1,1,1,1,1,1,1,1,1,1,1,1,
1,1,1,1,1,1,1,1,1,1,1,1,1,1,1,1,1,1,1,1,1,1,1,6),(0.,0.005,0.01,0.015,0.02,
0.025,0.03,0.035,0.04,0.045,0.05,0.055,0.06,0.065,0.07,0.075,0.08,0.085,
0.09,0.095,0.1,0.105,0.11,0.115,0.12,0.125,0.13,0.135,0.14,0.145,0.15,0.155,
0.16,0.165,0.17,0.175,0.18,0.185,0.19,0.195,0.2,0.205,0.21,0.215,0.22,0.225,
0.23,0.235,0.24,0.245,0.25,0.255,0.26,0.265,0.27,0.275,0.28,0.285,0.29,
0.295,0.3,0.305,0.31,0.315,0.32,0.325,0.33,0.335,0.34,0.345,0.35,0.355,
0.36,0.365,0.37,0.375,0.38,0.385,0.39,0.395,0.4,0.405,0.41,0.415,0.42,0.425,
0.43,0.435,0.44,0.445,0.45,0.455,0.46,0.465,0.47,0.475,0.48,0.485,0.49,
0.495,0.5,0.505,0.51,0.515,0.52,0.525,0.53,0.535,0.54,0.545,0.55,0.555,
0.56,0.565,0.57,0.575,0.58,0.585,0.59,0.595,0.6,0.605,0.61,0.615,0.62,0.625,
0.63,0.635,0.64,0.645,0.65,0.655,0.66,0.665,0.67,0.675,0.68,0.685,0.690000000000001,
0.695000000000001,0.700000000000001,0.705000000000001,0.710000000000001,
0.715000000000001,0.720000000000001,0.725000000000001,0.730000000000001,
0.735000000000001,0.740000000000001,0.745000000000001,0.750000000000001,
0.755000000000001,0.760000000000001,0.765000000000001,0.770000000000001,
0.775000000000001,0.780000000000001,0.785000000000001,0.790000000000001,
0.795000000000001,0.800000000000001,0.805000000000001,0.810000000000001,
0.815000000000001,0.820000000000001,0.825000000000001,0.830000000000001,
0.835000000000001,0.840000000000001,0.845000000000001,0.850000000000001,
0.855000000000001,0.860000000000001,0.865000000000001,0.870000000000001,
0.875000000000001,0.880000000000001,0.885000000000001,0.890000000000001,
0.895000000000001,0.900000000000001,0.905000000000001,0.910000000000001,
0.915000000000001,0.920000000000001,0.925000000000001,0.930000000000001,
0.935000000000001,0.940000000000001,0.941429844431335),.UNSPECIFIED.)
CURVE()
GEOMETRIC_REPRESENTATION_ITEM()
RATIONAL_B_SPLINE_CURVE((1.,1.,1.,1.,1.,1.,1.,1.,1.,1.,1.,1.,1.,1.,1.,1.,
1.,1.,1.,1.,1.,1.,1.,1.,1.,1.,1.,1.,1.,1.,1.,1.,1.,1.,1.,1.,1.,1.,1.,1.,
1.,1.,1.,1.,1.,1.,1.,1.,1.,1.,1.,1.,1.,1.,1.,1.,1.,1.,1.,1.,1.,1.,1.,1.,
1.,1.,1.,1.,1.,1.,1.,1.,1.,1.,1.,1.,1.,1.,1.,1.,1.,1.,1.,1.,1.,1.,1.,1.,
1.,1.,1.,1.,1.,1.,1.,1.,1.,1.,1.,1.,1.,1.,1.,1.,1.,1.,1.,1.,1.,1.,1.,1.,
1.,1.,1.,1.,1.,1.,1.,1.,1.,1.,1.,1.,1.,1.,1.,1.,1.,1.,1.,1.,1.,1.,1.,1.,
1.,1.,1.,1.,1.,1.,1.,1.,1.,1.,1.,1.,1.,1.,1.,1.,1.,1.,1.,1.,1.,1.,1.,1.,
1.,1.,1.,1.,1.,1.,1.,1.,1.,1.,1.,1.,1.,1.,1.,1.,1.,1.,1.,1.,1.,1.,1.,1.,
1.,1.,1.,1.,1.,1.,1.,1.,1.,1.))
REPRESENTATION_ITEM('')
);
#416=(
BOUNDED_CURVE()
B_SPLINE_CURVE(5,(#58605,#58606,#58607,#58608,#58609,#58610,#58611,#58612,
#58613,#58614,#58615,#58616,#58617,#58618,#58619,#58620,#58621,#58622,#58623,
#58624,#58625,#58626,#58627,#58628,#58629,#58630,#58631,#58632,#58633,#58634,
#58635,#58636,#58637,#58638,#58639,#58640,#58641,#58642,#58643,#58644,#58645,
#58646,#58647,#58648,#58649,#58650,#58651,#58652,#58653,#58654,#58655,#58656,
#58657,#58658,#58659,#58660,#58661,#58662,#58663,#58664,#58665,#58666,#58667,
#58668,#58669,#58670,#58671,#58672,#58673,#58674,#58675,#58676,#58677,#58678,
#58679,#58680,#58681,#58682,#58683,#58684,#58685,#58686,#58687,#58688,#58689,
#58690,#58691,#58692,#58693,#58694,#58695,#58696,#58697,#58698,#58699,#58700,
#58701,#58702,#58703,#58704,#58705,#58706,#58707,#58708,#58709,#58710,#58711,
#58712,#58713,#58714,#58715,#58716,#58717,#58718,#58719,#58720,#58721,#58722,
#58723,#58724,#58725,#58726,#58727,#58728,#58729,#58730,#58731,#58732,#58733,
#58734,#58735,#58736,#58737,#58738,#58739,#58740,#58741,#58742,#58743,#58744,
#58745,#58746,#58747,#58748,#58749,#58750,#58751,#58752,#58753,#58754,#58755,
#58756,#58757,#58758,#58759,#58760,#58761,#58762,#58763,#58764,#58765,#58766,
#58767,#58768,#58769,#58770,#58771,#58772,#58773,#58774,#58775,#58776,#58777,
#58778,#58779,#58780,#58781,#58782,#58783,#58784,#58785,#58786,#58787,#58788,
#58789,#58790,#58791,#58792,#58793,#58794,#58795,#58796,#58797,#58798),
 .UNSPECIFIED.,.F.,.F.)
B_SPLINE_CURVE_WITH_KNOTS((6,1,1,1,1,1,1,1,1,1,1,1,1,1,1,1,1,1,1,1,1,1,
1,1,1,1,1,1,1,1,1,1,1,1,1,1,1,1,1,1,1,1,1,1,1,1,1,1,1,1,1,1,1,1,1,1,1,1,
1,1,1,1,1,1,1,1,1,1,1,1,1,1,1,1,1,1,1,1,1,1,1,1,1,1,1,1,1,1,1,1,1,1,1,1,
1,1,1,1,1,1,1,1,1,1,1,1,1,1,1,1,1,1,1,1,1,1,1,1,1,1,1,1,1,1,1,1,1,1,1,1,
1,1,1,1,1,1,1,1,1,1,1,1,1,1,1,1,1,1,1,1,1,1,1,1,1,1,1,1,1,1,1,1,1,1,1,1,
1,1,1,1,1,1,1,1,1,1,1,1,1,1,1,1,1,1,1,1,1,1,1,6),(-0.941429844431332,-0.940000000000001,
-0.935000000000001,-0.930000000000001,-0.925000000000001,-0.920000000000001,
-0.915000000000001,-0.910000000000001,-0.905000000000001,-0.900000000000001,
-0.895000000000001,-0.890000000000001,-0.885000000000001,-0.880000000000001,
-0.875000000000001,-0.870000000000001,-0.865000000000001,-0.860000000000001,
-0.855000000000001,-0.850000000000001,-0.845000000000001,-0.840000000000001,
-0.835000000000001,-0.830000000000001,-0.825000000000001,-0.820000000000001,
-0.815000000000001,-0.810000000000001,-0.805000000000001,-0.800000000000001,
-0.795000000000001,-0.790000000000001,-0.785000000000001,-0.780000000000001,
-0.775000000000001,-0.770000000000001,-0.765000000000001,-0.760000000000001,
-0.755000000000001,-0.750000000000001,-0.745000000000001,-0.740000000000001,
-0.735000000000001,-0.730000000000001,-0.725000000000001,-0.720000000000001,
-0.715000000000001,-0.710000000000001,-0.705000000000001,-0.700000000000001,
-0.695000000000001,-0.690000000000001,-0.685,-0.68,-0.675,-0.67,-0.665,
-0.66,-0.655,-0.65,-0.645,-0.64,-0.635,-0.63,-0.625,-0.62,-0.615,-0.61,
-0.605,-0.6,-0.595,-0.59,-0.585,-0.58,-0.575,-0.57,-0.565,-0.56,-0.555,
-0.55,-0.545,-0.54,-0.535,-0.53,-0.525,-0.52,-0.515,-0.51,-0.505,-0.5,-0.495,
-0.49,-0.485,-0.48,-0.475,-0.47,-0.465,-0.46,-0.455,-0.45,-0.445,-0.44,
-0.435,-0.43,-0.425,-0.42,-0.415,-0.41,-0.405,-0.4,-0.395,-0.39,-0.385,
-0.38,-0.375,-0.37,-0.365,-0.36,-0.355,-0.35,-0.345,-0.34,-0.335,-0.33,
-0.325,-0.32,-0.315,-0.31,-0.305,-0.3,-0.295,-0.29,-0.285,-0.28,-0.275,
-0.27,-0.265,-0.26,-0.255,-0.25,-0.245,-0.24,-0.235,-0.23,-0.225,-0.22,
-0.215,-0.21,-0.205,-0.2,-0.195,-0.19,-0.185,-0.18,-0.175,-0.17,-0.165,
-0.16,-0.155,-0.15,-0.145,-0.14,-0.135,-0.13,-0.125,-0.12,-0.115,-0.11,
-0.105,-0.1,-0.095,-0.09,-0.085,-0.08,-0.075,-0.07,-0.065,-0.06,-0.055,
-0.05,-0.045,-0.04,-0.035,-0.03,-0.025,-0.02,-0.015,-0.01,-0.005,0.),
 .UNSPECIFIED.)
CURVE()
GEOMETRIC_REPRESENTATION_ITEM()
RATIONAL_B_SPLINE_CURVE((1.,1.,1.,1.,1.,1.,1.,1.,1.,1.,1.,1.,1.,1.,1.,1.,
1.,1.,1.,1.,1.,1.,1.,1.,1.,1.,1.,1.,1.,1.,1.,1.,1.,1.,1.,1.,1.,1.,1.,1.,
1.,1.,1.,1.,1.,1.,1.,1.,1.,1.,1.,1.,1.,1.,1.,1.,1.,1.,1.,1.,1.,1.,1.,1.,
1.,1.,1.,1.,1.,1.,1.,1.,1.,1.,1.,1.,1.,1.,1.,1.,1.,1.,1.,1.,1.,1.,1.,1.,
1.,1.,1.,1.,1.,1.,1.,1.,1.,1.,1.,1.,1.,1.,1.,1.,1.,1.,1.,1.,1.,1.,1.,1.,
1.,1.,1.,1.,1.,1.,1.,1.,1.,1.,1.,1.,1.,1.,1.,1.,1.,1.,1.,1.,1.,1.,1.,1.,
1.,1.,1.,1.,1.,1.,1.,1.,1.,1.,1.,1.,1.,1.,1.,1.,1.,1.,1.,1.,1.,1.,1.,1.,
1.,1.,1.,1.,1.,1.,1.,1.,1.,1.,1.,1.,1.,1.,1.,1.,1.,1.,1.,1.,1.,1.,1.,1.,
1.,1.,1.,1.,1.,1.,1.,1.,1.,1.))
REPRESENTATION_ITEM('')
);
#417=(
BOUNDED_CURVE()
B_SPLINE_CURVE(5,(#59305,#59306,#59307,#59308,#59309,#59310,#59311,#59312,
#59313,#59314,#59315,#59316,#59317,#59318,#59319,#59320,#59321,#59322,#59323,
#59324,#59325,#59326,#59327,#59328,#59329,#59330,#59331,#59332,#59333,#59334,
#59335,#59336,#59337,#59338,#59339,#59340,#59341,#59342,#59343,#59344,#59345,
#59346,#59347,#59348,#59349,#59350,#59351,#59352,#59353,#59354,#59355,#59356,
#59357,#59358,#59359,#59360,#59361,#59362,#59363,#59364,#59365,#59366,#59367,
#59368,#59369,#59370,#59371,#59372,#59373,#59374,#59375,#59376,#59377,#59378,
#59379,#59380,#59381,#59382,#59383,#59384,#59385,#59386,#59387,#59388,#59389,
#59390,#59391,#59392,#59393,#59394,#59395,#59396,#59397,#59398,#59399,#59400,
#59401,#59402,#59403,#59404,#59405,#59406,#59407,#59408,#59409,#59410,#59411,
#59412,#59413,#59414,#59415,#59416,#59417,#59418,#59419,#59420,#59421,#59422,
#59423,#59424,#59425,#59426,#59427,#59428,#59429,#59430,#59431,#59432,#59433,
#59434,#59435,#59436,#59437,#59438,#59439,#59440,#59441,#59442,#59443,#59444,
#59445,#59446,#59447,#59448,#59449,#59450,#59451,#59452,#59453,#59454,#59455,
#59456,#59457,#59458,#59459,#59460,#59461,#59462,#59463,#59464,#59465,#59466,
#59467,#59468,#59469,#59470,#59471,#59472,#59473,#59474,#59475,#59476,#59477,
#59478,#59479,#59480,#59481,#59482,#59483,#59484,#59485,#59486,#59487,#59488,
#59489,#59490,#59491,#59492,#59493,#59494,#59495,#59496,#59497,#59498),
 .UNSPECIFIED.,.F.,.F.)
B_SPLINE_CURVE_WITH_KNOTS((6,1,1,1,1,1,1,1,1,1,1,1,1,1,1,1,1,1,1,1,1,1,
1,1,1,1,1,1,1,1,1,1,1,1,1,1,1,1,1,1,1,1,1,1,1,1,1,1,1,1,1,1,1,1,1,1,1,1,
1,1,1,1,1,1,1,1,1,1,1,1,1,1,1,1,1,1,1,1,1,1,1,1,1,1,1,1,1,1,1,1,1,1,1,1,
1,1,1,1,1,1,1,1,1,1,1,1,1,1,1,1,1,1,1,1,1,1,1,1,1,1,1,1,1,1,1,1,1,1,1,1,
1,1,1,1,1,1,1,1,1,1,1,1,1,1,1,1,1,1,1,1,1,1,1,1,1,1,1,1,1,1,1,1,1,1,1,1,
1,1,1,1,1,1,1,1,1,1,1,1,1,1,1,1,1,1,1,1,1,1,1,6),(0.,0.005,0.01,0.015,0.02,
0.025,0.03,0.035,0.04,0.045,0.05,0.055,0.06,0.065,0.07,0.075,0.08,0.085,
0.09,0.095,0.1,0.105,0.11,0.115,0.12,0.125,0.13,0.135,0.14,0.145,0.15,0.155,
0.16,0.165,0.17,0.175,0.18,0.185,0.19,0.195,0.2,0.205,0.21,0.215,0.22,0.225,
0.23,0.235,0.24,0.245,0.25,0.255,0.26,0.265,0.27,0.275,0.28,0.285,0.29,
0.295,0.3,0.305,0.31,0.315,0.32,0.325,0.33,0.335,0.34,0.345,0.35,0.355,
0.36,0.365,0.37,0.375,0.38,0.385,0.39,0.395,0.4,0.405,0.41,0.415,0.42,0.425,
0.43,0.435,0.44,0.445,0.45,0.455,0.46,0.465,0.47,0.475,0.48,0.485,0.49,
0.495,0.5,0.505,0.51,0.515,0.52,0.525,0.53,0.535,0.54,0.545,0.55,0.555,
0.56,0.565,0.57,0.575,0.58,0.585,0.59,0.595,0.6,0.605,0.61,0.615,0.62,0.625,
0.63,0.635,0.64,0.645,0.65,0.655,0.66,0.665,0.67,0.675,0.68,0.685,0.690000000000001,
0.695000000000001,0.700000000000001,0.705000000000001,0.710000000000001,
0.715000000000001,0.720000000000001,0.725000000000001,0.730000000000001,
0.735000000000001,0.740000000000001,0.745000000000001,0.750000000000001,
0.755000000000001,0.760000000000001,0.765000000000001,0.770000000000001,
0.775000000000001,0.780000000000001,0.785000000000001,0.790000000000001,
0.795000000000001,0.800000000000001,0.805000000000001,0.810000000000001,
0.815000000000001,0.820000000000001,0.825000000000001,0.830000000000001,
0.835000000000001,0.840000000000001,0.845000000000001,0.850000000000001,
0.855000000000001,0.860000000000001,0.865000000000001,0.870000000000001,
0.875000000000001,0.880000000000001,0.885000000000001,0.890000000000001,
0.895000000000001,0.900000000000001,0.905000000000001,0.910000000000001,
0.915000000000001,0.920000000000001,0.925000000000001,0.930000000000001,
0.935000000000001,0.940000000000001,0.941429844431367),.UNSPECIFIED.)
CURVE()
GEOMETRIC_REPRESENTATION_ITEM()
RATIONAL_B_SPLINE_CURVE((1.,1.,1.,1.,1.,1.,1.,1.,1.,1.,1.,1.,1.,1.,1.,1.,
1.,1.,1.,1.,1.,1.,1.,1.,1.,1.,1.,1.,1.,1.,1.,1.,1.,1.,1.,1.,1.,1.,1.,1.,
1.,1.,1.,1.,1.,1.,1.,1.,1.,1.,1.,1.,1.,1.,1.,1.,1.,1.,1.,1.,1.,1.,1.,1.,
1.,1.,1.,1.,1.,1.,1.,1.,1.,1.,1.,1.,1.,1.,1.,1.,1.,1.,1.,1.,1.,1.,1.,1.,
1.,1.,1.,1.,1.,1.,1.,1.,1.,1.,1.,1.,1.,1.,1.,1.,1.,1.,1.,1.,1.,1.,1.,1.,
1.,1.,1.,1.,1.,1.,1.,1.,1.,1.,1.,1.,1.,1.,1.,1.,1.,1.,1.,1.,1.,1.,1.,1.,
1.,1.,1.,1.,1.,1.,1.,1.,1.,1.,1.,1.,1.,1.,1.,1.,1.,1.,1.,1.,1.,1.,1.,1.,
1.,1.,1.,1.,1.,1.,1.,1.,1.,1.,1.,1.,1.,1.,1.,1.,1.,1.,1.,1.,1.,1.,1.,1.,
1.,1.,1.,1.,1.,1.,1.,1.,1.,1.))
REPRESENTATION_ITEM('')
);
#418=(
BOUNDED_CURVE()
B_SPLINE_CURVE(5,(#59501,#59502,#59503,#59504,#59505,#59506,#59507,#59508,
#59509,#59510,#59511,#59512,#59513,#59514,#59515,#59516,#59517,#59518,#59519,
#59520,#59521,#59522,#59523,#59524,#59525,#59526,#59527,#59528,#59529,#59530,
#59531,#59532,#59533,#59534,#59535,#59536,#59537,#59538,#59539,#59540,#59541,
#59542,#59543,#59544,#59545,#59546,#59547,#59548,#59549,#59550,#59551,#59552,
#59553,#59554,#59555,#59556,#59557,#59558,#59559,#59560,#59561,#59562,#59563,
#59564,#59565,#59566,#59567,#59568,#59569,#59570,#59571,#59572,#59573,#59574,
#59575,#59576,#59577,#59578,#59579,#59580,#59581,#59582,#59583,#59584,#59585,
#59586,#59587,#59588,#59589,#59590,#59591,#59592,#59593,#59594,#59595,#59596,
#59597,#59598,#59599,#59600,#59601,#59602,#59603,#59604,#59605,#59606,#59607,
#59608,#59609,#59610,#59611,#59612,#59613,#59614,#59615,#59616,#59617,#59618,
#59619,#59620,#59621,#59622,#59623,#59624,#59625,#59626,#59627,#59628,#59629,
#59630,#59631,#59632,#59633,#59634,#59635,#59636,#59637,#59638,#59639,#59640,
#59641,#59642,#59643,#59644,#59645,#59646,#59647,#59648,#59649,#59650,#59651,
#59652,#59653,#59654,#59655,#59656,#59657,#59658,#59659,#59660,#59661,#59662,
#59663,#59664,#59665,#59666,#59667,#59668,#59669,#59670,#59671,#59672,#59673,
#59674,#59675,#59676,#59677,#59678,#59679,#59680,#59681,#59682,#59683,#59684,
#59685,#59686,#59687,#59688,#59689,#59690,#59691,#59692,#59693,#59694),
 .UNSPECIFIED.,.F.,.F.)
B_SPLINE_CURVE_WITH_KNOTS((6,1,1,1,1,1,1,1,1,1,1,1,1,1,1,1,1,1,1,1,1,1,
1,1,1,1,1,1,1,1,1,1,1,1,1,1,1,1,1,1,1,1,1,1,1,1,1,1,1,1,1,1,1,1,1,1,1,1,
1,1,1,1,1,1,1,1,1,1,1,1,1,1,1,1,1,1,1,1,1,1,1,1,1,1,1,1,1,1,1,1,1,1,1,1,
1,1,1,1,1,1,1,1,1,1,1,1,1,1,1,1,1,1,1,1,1,1,1,1,1,1,1,1,1,1,1,1,1,1,1,1,
1,1,1,1,1,1,1,1,1,1,1,1,1,1,1,1,1,1,1,1,1,1,1,1,1,1,1,1,1,1,1,1,1,1,1,1,
1,1,1,1,1,1,1,1,1,1,1,1,1,1,1,1,1,1,1,1,1,1,1,6),(-0.941429844431342,-0.940000000000001,
-0.935000000000001,-0.930000000000001,-0.925000000000001,-0.920000000000001,
-0.915000000000001,-0.910000000000001,-0.905000000000001,-0.900000000000001,
-0.895000000000001,-0.890000000000001,-0.885000000000001,-0.880000000000001,
-0.875000000000001,-0.870000000000001,-0.865000000000001,-0.860000000000001,
-0.855000000000001,-0.850000000000001,-0.845000000000001,-0.840000000000001,
-0.835000000000001,-0.830000000000001,-0.825000000000001,-0.820000000000001,
-0.815000000000001,-0.810000000000001,-0.805000000000001,-0.800000000000001,
-0.795000000000001,-0.790000000000001,-0.785000000000001,-0.780000000000001,
-0.775000000000001,-0.770000000000001,-0.765000000000001,-0.760000000000001,
-0.755000000000001,-0.750000000000001,-0.745000000000001,-0.740000000000001,
-0.735000000000001,-0.730000000000001,-0.725000000000001,-0.720000000000001,
-0.715000000000001,-0.710000000000001,-0.705000000000001,-0.700000000000001,
-0.695000000000001,-0.690000000000001,-0.685,-0.68,-0.675,-0.67,-0.665,
-0.66,-0.655,-0.65,-0.645,-0.64,-0.635,-0.63,-0.625,-0.62,-0.615,-0.61,
-0.605,-0.6,-0.595,-0.59,-0.585,-0.58,-0.575,-0.57,-0.565,-0.56,-0.555,
-0.55,-0.545,-0.54,-0.535,-0.53,-0.525,-0.52,-0.515,-0.51,-0.505,-0.5,-0.495,
-0.49,-0.485,-0.48,-0.475,-0.47,-0.465,-0.46,-0.455,-0.45,-0.445,-0.44,
-0.435,-0.43,-0.425,-0.42,-0.415,-0.41,-0.405,-0.4,-0.395,-0.39,-0.385,
-0.38,-0.375,-0.37,-0.365,-0.36,-0.355,-0.35,-0.345,-0.34,-0.335,-0.33,
-0.325,-0.32,-0.315,-0.31,-0.305,-0.3,-0.295,-0.29,-0.285,-0.28,-0.275,
-0.27,-0.265,-0.26,-0.255,-0.25,-0.245,-0.24,-0.235,-0.23,-0.225,-0.22,
-0.215,-0.21,-0.205,-0.2,-0.195,-0.19,-0.185,-0.18,-0.175,-0.17,-0.165,
-0.16,-0.155,-0.15,-0.145,-0.14,-0.135,-0.13,-0.125,-0.12,-0.115,-0.11,
-0.105,-0.1,-0.095,-0.09,-0.085,-0.08,-0.075,-0.07,-0.065,-0.06,-0.055,
-0.05,-0.045,-0.04,-0.035,-0.03,-0.025,-0.02,-0.015,-0.01,-0.005,0.),
 .UNSPECIFIED.)
CURVE()
GEOMETRIC_REPRESENTATION_ITEM()
RATIONAL_B_SPLINE_CURVE((1.,1.,1.,1.,1.,1.,1.,1.,1.,1.,1.,1.,1.,1.,1.,1.,
1.,1.,1.,1.,1.,1.,1.,1.,1.,1.,1.,1.,1.,1.,1.,1.,1.,1.,1.,1.,1.,1.,1.,1.,
1.,1.,1.,1.,1.,1.,1.,1.,1.,1.,1.,1.,1.,1.,1.,1.,1.,1.,1.,1.,1.,1.,1.,1.,
1.,1.,1.,1.,1.,1.,1.,1.,1.,1.,1.,1.,1.,1.,1.,1.,1.,1.,1.,1.,1.,1.,1.,1.,
1.,1.,1.,1.,1.,1.,1.,1.,1.,1.,1.,1.,1.,1.,1.,1.,1.,1.,1.,1.,1.,1.,1.,1.,
1.,1.,1.,1.,1.,1.,1.,1.,1.,1.,1.,1.,1.,1.,1.,1.,1.,1.,1.,1.,1.,1.,1.,1.,
1.,1.,1.,1.,1.,1.,1.,1.,1.,1.,1.,1.,1.,1.,1.,1.,1.,1.,1.,1.,1.,1.,1.,1.,
1.,1.,1.,1.,1.,1.,1.,1.,1.,1.,1.,1.,1.,1.,1.,1.,1.,1.,1.,1.,1.,1.,1.,1.,
1.,1.,1.,1.,1.,1.,1.,1.,1.,1.))
REPRESENTATION_ITEM('')
);
#419=(
BOUNDED_CURVE()
B_SPLINE_CURVE(5,(#60201,#60202,#60203,#60204,#60205,#60206,#60207,#60208,
#60209,#60210,#60211,#60212,#60213,#60214,#60215,#60216,#60217,#60218,#60219,
#60220,#60221,#60222,#60223,#60224,#60225,#60226,#60227,#60228,#60229,#60230,
#60231,#60232,#60233,#60234,#60235,#60236,#60237,#60238,#60239,#60240,#60241,
#60242,#60243,#60244,#60245,#60246,#60247,#60248,#60249,#60250,#60251,#60252,
#60253,#60254,#60255,#60256,#60257,#60258,#60259,#60260,#60261,#60262,#60263,
#60264,#60265,#60266,#60267,#60268,#60269,#60270,#60271,#60272,#60273,#60274,
#60275,#60276,#60277,#60278,#60279,#60280,#60281,#60282,#60283,#60284,#60285,
#60286,#60287,#60288,#60289,#60290,#60291,#60292,#60293,#60294,#60295,#60296,
#60297,#60298,#60299,#60300,#60301,#60302,#60303,#60304,#60305,#60306,#60307,
#60308,#60309,#60310,#60311,#60312,#60313,#60314,#60315,#60316,#60317,#60318,
#60319,#60320,#60321,#60322,#60323,#60324,#60325,#60326,#60327,#60328,#60329,
#60330,#60331,#60332,#60333,#60334,#60335,#60336,#60337,#60338,#60339,#60340,
#60341,#60342,#60343,#60344,#60345,#60346,#60347,#60348,#60349,#60350,#60351,
#60352,#60353,#60354,#60355,#60356,#60357,#60358,#60359,#60360,#60361,#60362,
#60363,#60364,#60365,#60366,#60367,#60368,#60369,#60370,#60371,#60372,#60373,
#60374,#60375,#60376,#60377,#60378,#60379,#60380,#60381,#60382,#60383,#60384,
#60385,#60386,#60387,#60388,#60389,#60390,#60391,#60392,#60393,#60394),
 .UNSPECIFIED.,.F.,.F.)
B_SPLINE_CURVE_WITH_KNOTS((6,1,1,1,1,1,1,1,1,1,1,1,1,1,1,1,1,1,1,1,1,1,
1,1,1,1,1,1,1,1,1,1,1,1,1,1,1,1,1,1,1,1,1,1,1,1,1,1,1,1,1,1,1,1,1,1,1,1,
1,1,1,1,1,1,1,1,1,1,1,1,1,1,1,1,1,1,1,1,1,1,1,1,1,1,1,1,1,1,1,1,1,1,1,1,
1,1,1,1,1,1,1,1,1,1,1,1,1,1,1,1,1,1,1,1,1,1,1,1,1,1,1,1,1,1,1,1,1,1,1,1,
1,1,1,1,1,1,1,1,1,1,1,1,1,1,1,1,1,1,1,1,1,1,1,1,1,1,1,1,1,1,1,1,1,1,1,1,
1,1,1,1,1,1,1,1,1,1,1,1,1,1,1,1,1,1,1,1,1,1,1,6),(0.,0.005,0.01,0.015,0.02,
0.025,0.03,0.035,0.04,0.045,0.05,0.055,0.06,0.065,0.07,0.075,0.08,0.085,
0.09,0.095,0.1,0.105,0.11,0.115,0.12,0.125,0.13,0.135,0.14,0.145,0.15,0.155,
0.16,0.165,0.17,0.175,0.18,0.185,0.19,0.195,0.2,0.205,0.21,0.215,0.22,0.225,
0.23,0.235,0.24,0.245,0.25,0.255,0.26,0.265,0.27,0.275,0.28,0.285,0.29,
0.295,0.3,0.305,0.31,0.315,0.32,0.325,0.33,0.335,0.34,0.345,0.35,0.355,
0.36,0.365,0.37,0.375,0.38,0.385,0.39,0.395,0.4,0.405,0.41,0.415,0.42,0.425,
0.43,0.435,0.44,0.445,0.45,0.455,0.46,0.465,0.47,0.475,0.48,0.485,0.49,
0.495,0.5,0.505,0.51,0.515,0.52,0.525,0.53,0.535,0.54,0.545,0.55,0.555,
0.56,0.565,0.57,0.575,0.58,0.585,0.59,0.595,0.6,0.605,0.61,0.615,0.62,0.625,
0.63,0.635,0.64,0.645,0.65,0.655,0.66,0.665,0.67,0.675,0.68,0.685,0.690000000000001,
0.695000000000001,0.700000000000001,0.705000000000001,0.710000000000001,
0.715000000000001,0.720000000000001,0.725000000000001,0.730000000000001,
0.735000000000001,0.740000000000001,0.745000000000001,0.750000000000001,
0.755000000000001,0.760000000000001,0.765000000000001,0.770000000000001,
0.775000000000001,0.780000000000001,0.785000000000001,0.790000000000001,
0.795000000000001,0.800000000000001,0.805000000000001,0.810000000000001,
0.815000000000001,0.820000000000001,0.825000000000001,0.830000000000001,
0.835000000000001,0.840000000000001,0.845000000000001,0.850000000000001,
0.855000000000001,0.860000000000001,0.865000000000001,0.870000000000001,
0.875000000000001,0.880000000000001,0.885000000000001,0.890000000000001,
0.895000000000001,0.900000000000001,0.905000000000001,0.910000000000001,
0.915000000000001,0.920000000000001,0.925000000000001,0.930000000000001,
0.935000000000001,0.940000000000001,0.941429844431369),.UNSPECIFIED.)
CURVE()
GEOMETRIC_REPRESENTATION_ITEM()
RATIONAL_B_SPLINE_CURVE((1.,1.,1.,1.,1.,1.,1.,1.,1.,1.,1.,1.,1.,1.,1.,1.,
1.,1.,1.,1.,1.,1.,1.,1.,1.,1.,1.,1.,1.,1.,1.,1.,1.,1.,1.,1.,1.,1.,1.,1.,
1.,1.,1.,1.,1.,1.,1.,1.,1.,1.,1.,1.,1.,1.,1.,1.,1.,1.,1.,1.,1.,1.,1.,1.,
1.,1.,1.,1.,1.,1.,1.,1.,1.,1.,1.,1.,1.,1.,1.,1.,1.,1.,1.,1.,1.,1.,1.,1.,
1.,1.,1.,1.,1.,1.,1.,1.,1.,1.,1.,1.,1.,1.,1.,1.,1.,1.,1.,1.,1.,1.,1.,1.,
1.,1.,1.,1.,1.,1.,1.,1.,1.,1.,1.,1.,1.,1.,1.,1.,1.,1.,1.,1.,1.,1.,1.,1.,
1.,1.,1.,1.,1.,1.,1.,1.,1.,1.,1.,1.,1.,1.,1.,1.,1.,1.,1.,1.,1.,1.,1.,1.,
1.,1.,1.,1.,1.,1.,1.,1.,1.,1.,1.,1.,1.,1.,1.,1.,1.,1.,1.,1.,1.,1.,1.,1.,
1.,1.,1.,1.,1.,1.,1.,1.,1.,1.))
REPRESENTATION_ITEM('')
);
#420=(
BOUNDED_CURVE()
B_SPLINE_CURVE(5,(#60397,#60398,#60399,#60400,#60401,#60402,#60403,#60404,
#60405,#60406,#60407,#60408,#60409,#60410,#60411,#60412,#60413,#60414,#60415,
#60416,#60417,#60418,#60419,#60420,#60421,#60422,#60423,#60424,#60425,#60426,
#60427,#60428,#60429,#60430,#60431,#60432,#60433,#60434,#60435,#60436,#60437,
#60438,#60439,#60440,#60441,#60442,#60443,#60444,#60445,#60446,#60447,#60448,
#60449,#60450,#60451,#60452,#60453,#60454,#60455,#60456,#60457,#60458,#60459,
#60460,#60461,#60462,#60463,#60464,#60465,#60466,#60467,#60468,#60469,#60470,
#60471,#60472,#60473,#60474,#60475,#60476,#60477,#60478,#60479,#60480,#60481,
#60482,#60483,#60484,#60485,#60486,#60487,#60488,#60489,#60490,#60491,#60492,
#60493,#60494,#60495,#60496,#60497,#60498,#60499,#60500,#60501,#60502,#60503,
#60504,#60505,#60506,#60507,#60508,#60509,#60510,#60511,#60512,#60513,#60514,
#60515,#60516,#60517,#60518,#60519,#60520,#60521,#60522,#60523,#60524,#60525,
#60526,#60527,#60528,#60529,#60530,#60531,#60532,#60533,#60534,#60535,#60536,
#60537,#60538,#60539,#60540,#60541,#60542,#60543,#60544,#60545,#60546,#60547,
#60548,#60549,#60550,#60551,#60552,#60553,#60554,#60555,#60556,#60557,#60558,
#60559,#60560,#60561,#60562,#60563,#60564,#60565,#60566,#60567,#60568,#60569,
#60570,#60571,#60572,#60573,#60574,#60575,#60576,#60577,#60578,#60579,#60580,
#60581,#60582,#60583,#60584,#60585,#60586,#60587,#60588,#60589,#60590),
 .UNSPECIFIED.,.F.,.F.)
B_SPLINE_CURVE_WITH_KNOTS((6,1,1,1,1,1,1,1,1,1,1,1,1,1,1,1,1,1,1,1,1,1,
1,1,1,1,1,1,1,1,1,1,1,1,1,1,1,1,1,1,1,1,1,1,1,1,1,1,1,1,1,1,1,1,1,1,1,1,
1,1,1,1,1,1,1,1,1,1,1,1,1,1,1,1,1,1,1,1,1,1,1,1,1,1,1,1,1,1,1,1,1,1,1,1,
1,1,1,1,1,1,1,1,1,1,1,1,1,1,1,1,1,1,1,1,1,1,1,1,1,1,1,1,1,1,1,1,1,1,1,1,
1,1,1,1,1,1,1,1,1,1,1,1,1,1,1,1,1,1,1,1,1,1,1,1,1,1,1,1,1,1,1,1,1,1,1,1,
1,1,1,1,1,1,1,1,1,1,1,1,1,1,1,1,1,1,1,1,1,1,1,6),(-0.941429844431369,-0.940000000000001,
-0.935000000000001,-0.930000000000001,-0.925000000000001,-0.920000000000001,
-0.915000000000001,-0.910000000000001,-0.905000000000001,-0.900000000000001,
-0.895000000000001,-0.890000000000001,-0.885000000000001,-0.880000000000001,
-0.875000000000001,-0.870000000000001,-0.865000000000001,-0.860000000000001,
-0.855000000000001,-0.850000000000001,-0.845000000000001,-0.840000000000001,
-0.835000000000001,-0.830000000000001,-0.825000000000001,-0.820000000000001,
-0.815000000000001,-0.810000000000001,-0.805000000000001,-0.800000000000001,
-0.795000000000001,-0.790000000000001,-0.785000000000001,-0.780000000000001,
-0.775000000000001,-0.770000000000001,-0.765000000000001,-0.760000000000001,
-0.755000000000001,-0.750000000000001,-0.745000000000001,-0.740000000000001,
-0.735000000000001,-0.730000000000001,-0.725000000000001,-0.720000000000001,
-0.715000000000001,-0.710000000000001,-0.705000000000001,-0.700000000000001,
-0.695000000000001,-0.690000000000001,-0.685,-0.68,-0.675,-0.67,-0.665,
-0.66,-0.655,-0.65,-0.645,-0.64,-0.635,-0.63,-0.625,-0.62,-0.615,-0.61,
-0.605,-0.6,-0.595,-0.59,-0.585,-0.58,-0.575,-0.57,-0.565,-0.56,-0.555,
-0.55,-0.545,-0.54,-0.535,-0.53,-0.525,-0.52,-0.515,-0.51,-0.505,-0.5,-0.495,
-0.49,-0.485,-0.48,-0.475,-0.47,-0.465,-0.46,-0.455,-0.45,-0.445,-0.44,
-0.435,-0.43,-0.425,-0.42,-0.415,-0.41,-0.405,-0.4,-0.395,-0.39,-0.385,
-0.38,-0.375,-0.37,-0.365,-0.36,-0.355,-0.35,-0.345,-0.34,-0.335,-0.33,
-0.325,-0.32,-0.315,-0.31,-0.305,-0.3,-0.295,-0.29,-0.285,-0.28,-0.275,
-0.27,-0.265,-0.26,-0.255,-0.25,-0.245,-0.24,-0.235,-0.23,-0.225,-0.22,
-0.215,-0.21,-0.205,-0.2,-0.195,-0.19,-0.185,-0.18,-0.175,-0.17,-0.165,
-0.16,-0.155,-0.15,-0.145,-0.14,-0.135,-0.13,-0.125,-0.12,-0.115,-0.11,
-0.105,-0.1,-0.095,-0.09,-0.085,-0.08,-0.075,-0.07,-0.065,-0.06,-0.055,
-0.05,-0.045,-0.04,-0.035,-0.03,-0.025,-0.02,-0.015,-0.01,-0.005,0.),
 .UNSPECIFIED.)
CURVE()
GEOMETRIC_REPRESENTATION_ITEM()
RATIONAL_B_SPLINE_CURVE((1.,1.,1.,1.,1.,1.,1.,1.,1.,1.,1.,1.,1.,1.,1.,1.,
1.,1.,1.,1.,1.,1.,1.,1.,1.,1.,1.,1.,1.,1.,1.,1.,1.,1.,1.,1.,1.,1.,1.,1.,
1.,1.,1.,1.,1.,1.,1.,1.,1.,1.,1.,1.,1.,1.,1.,1.,1.,1.,1.,1.,1.,1.,1.,1.,
1.,1.,1.,1.,1.,1.,1.,1.,1.,1.,1.,1.,1.,1.,1.,1.,1.,1.,1.,1.,1.,1.,1.,1.,
1.,1.,1.,1.,1.,1.,1.,1.,1.,1.,1.,1.,1.,1.,1.,1.,1.,1.,1.,1.,1.,1.,1.,1.,
1.,1.,1.,1.,1.,1.,1.,1.,1.,1.,1.,1.,1.,1.,1.,1.,1.,1.,1.,1.,1.,1.,1.,1.,
1.,1.,1.,1.,1.,1.,1.,1.,1.,1.,1.,1.,1.,1.,1.,1.,1.,1.,1.,1.,1.,1.,1.,1.,
1.,1.,1.,1.,1.,1.,1.,1.,1.,1.,1.,1.,1.,1.,1.,1.,1.,1.,1.,1.,1.,1.,1.,1.,
1.,1.,1.,1.,1.,1.,1.,1.,1.,1.))
REPRESENTATION_ITEM('')
);
#421=(
BOUNDED_CURVE()
B_SPLINE_CURVE(5,(#61097,#61098,#61099,#61100,#61101,#61102,#61103,#61104,
#61105,#61106,#61107,#61108,#61109,#61110,#61111,#61112,#61113,#61114,#61115,
#61116,#61117,#61118,#61119,#61120,#61121,#61122,#61123,#61124,#61125,#61126,
#61127,#61128,#61129,#61130,#61131,#61132,#61133,#61134,#61135,#61136,#61137,
#61138,#61139,#61140,#61141,#61142,#61143,#61144,#61145,#61146,#61147,#61148,
#61149,#61150,#61151,#61152,#61153,#61154,#61155,#61156,#61157,#61158,#61159,
#61160,#61161,#61162,#61163,#61164,#61165,#61166,#61167,#61168,#61169,#61170,
#61171,#61172,#61173,#61174,#61175,#61176,#61177,#61178,#61179,#61180,#61181,
#61182,#61183,#61184,#61185,#61186,#61187,#61188,#61189,#61190,#61191,#61192,
#61193,#61194,#61195,#61196,#61197,#61198,#61199,#61200,#61201,#61202,#61203,
#61204,#61205,#61206,#61207,#61208,#61209,#61210,#61211,#61212,#61213,#61214,
#61215,#61216,#61217,#61218,#61219,#61220,#61221,#61222,#61223,#61224,#61225,
#61226,#61227,#61228,#61229,#61230,#61231,#61232,#61233,#61234,#61235,#61236,
#61237,#61238,#61239,#61240,#61241,#61242,#61243,#61244,#61245,#61246,#61247,
#61248,#61249,#61250,#61251,#61252,#61253,#61254,#61255,#61256,#61257,#61258,
#61259,#61260,#61261,#61262,#61263,#61264,#61265,#61266,#61267,#61268,#61269,
#61270,#61271,#61272,#61273,#61274,#61275,#61276,#61277,#61278,#61279,#61280,
#61281,#61282,#61283,#61284,#61285,#61286,#61287,#61288,#61289,#61290),
 .UNSPECIFIED.,.F.,.F.)
B_SPLINE_CURVE_WITH_KNOTS((6,1,1,1,1,1,1,1,1,1,1,1,1,1,1,1,1,1,1,1,1,1,
1,1,1,1,1,1,1,1,1,1,1,1,1,1,1,1,1,1,1,1,1,1,1,1,1,1,1,1,1,1,1,1,1,1,1,1,
1,1,1,1,1,1,1,1,1,1,1,1,1,1,1,1,1,1,1,1,1,1,1,1,1,1,1,1,1,1,1,1,1,1,1,1,
1,1,1,1,1,1,1,1,1,1,1,1,1,1,1,1,1,1,1,1,1,1,1,1,1,1,1,1,1,1,1,1,1,1,1,1,
1,1,1,1,1,1,1,1,1,1,1,1,1,1,1,1,1,1,1,1,1,1,1,1,1,1,1,1,1,1,1,1,1,1,1,1,
1,1,1,1,1,1,1,1,1,1,1,1,1,1,1,1,1,1,1,1,1,1,1,6),(0.,0.005,0.01,0.015,0.02,
0.025,0.03,0.035,0.04,0.045,0.05,0.055,0.06,0.065,0.07,0.075,0.08,0.085,
0.09,0.095,0.1,0.105,0.11,0.115,0.12,0.125,0.13,0.135,0.14,0.145,0.15,0.155,
0.16,0.165,0.17,0.175,0.18,0.185,0.19,0.195,0.2,0.205,0.21,0.215,0.22,0.225,
0.23,0.235,0.24,0.245,0.25,0.255,0.26,0.265,0.27,0.275,0.28,0.285,0.29,
0.295,0.3,0.305,0.31,0.315,0.32,0.325,0.33,0.335,0.34,0.345,0.35,0.355,
0.36,0.365,0.37,0.375,0.38,0.385,0.39,0.395,0.4,0.405,0.41,0.415,0.42,0.425,
0.43,0.435,0.44,0.445,0.45,0.455,0.46,0.465,0.47,0.475,0.48,0.485,0.49,
0.495,0.5,0.505,0.51,0.515,0.52,0.525,0.53,0.535,0.54,0.545,0.55,0.555,
0.56,0.565,0.57,0.575,0.58,0.585,0.59,0.595,0.6,0.605,0.61,0.615,0.62,0.625,
0.63,0.635,0.64,0.645,0.65,0.655,0.66,0.665,0.67,0.675,0.68,0.685,0.690000000000001,
0.695000000000001,0.700000000000001,0.705000000000001,0.710000000000001,
0.715000000000001,0.720000000000001,0.725000000000001,0.730000000000001,
0.735000000000001,0.740000000000001,0.745000000000001,0.750000000000001,
0.755000000000001,0.760000000000001,0.765000000000001,0.770000000000001,
0.775000000000001,0.780000000000001,0.785000000000001,0.790000000000001,
0.795000000000001,0.800000000000001,0.805000000000001,0.810000000000001,
0.815000000000001,0.820000000000001,0.825000000000001,0.830000000000001,
0.835000000000001,0.840000000000001,0.845000000000001,0.850000000000001,
0.855000000000001,0.860000000000001,0.865000000000001,0.870000000000001,
0.875000000000001,0.880000000000001,0.885000000000001,0.890000000000001,
0.895000000000001,0.900000000000001,0.905000000000001,0.910000000000001,
0.915000000000001,0.920000000000001,0.925000000000001,0.930000000000001,
0.935000000000001,0.940000000000001,0.941429844431463),.UNSPECIFIED.)
CURVE()
GEOMETRIC_REPRESENTATION_ITEM()
RATIONAL_B_SPLINE_CURVE((1.,1.,1.,1.,1.,1.,1.,1.,1.,1.,1.,1.,1.,1.,1.,1.,
1.,1.,1.,1.,1.,1.,1.,1.,1.,1.,1.,1.,1.,1.,1.,1.,1.,1.,1.,1.,1.,1.,1.,1.,
1.,1.,1.,1.,1.,1.,1.,1.,1.,1.,1.,1.,1.,1.,1.,1.,1.,1.,1.,1.,1.,1.,1.,1.,
1.,1.,1.,1.,1.,1.,1.,1.,1.,1.,1.,1.,1.,1.,1.,1.,1.,1.,1.,1.,1.,1.,1.,1.,
1.,1.,1.,1.,1.,1.,1.,1.,1.,1.,1.,1.,1.,1.,1.,1.,1.,1.,1.,1.,1.,1.,1.,1.,
1.,1.,1.,1.,1.,1.,1.,1.,1.,1.,1.,1.,1.,1.,1.,1.,1.,1.,1.,1.,1.,1.,1.,1.,
1.,1.,1.,1.,1.,1.,1.,1.,1.,1.,1.,1.,1.,1.,1.,1.,1.,1.,1.,1.,1.,1.,1.,1.,
1.,1.,1.,1.,1.,1.,1.,1.,1.,1.,1.,1.,1.,1.,1.,1.,1.,1.,1.,1.,1.,1.,1.,1.,
1.,1.,1.,1.,1.,1.,1.,1.,1.,1.))
REPRESENTATION_ITEM('')
);
#422=(
BOUNDED_CURVE()
B_SPLINE_CURVE(5,(#61293,#61294,#61295,#61296,#61297,#61298,#61299,#61300,
#61301,#61302,#61303,#61304,#61305,#61306,#61307,#61308,#61309,#61310,#61311,
#61312,#61313,#61314,#61315,#61316,#61317,#61318,#61319,#61320,#61321,#61322,
#61323,#61324,#61325,#61326,#61327,#61328,#61329,#61330,#61331,#61332,#61333,
#61334,#61335,#61336,#61337,#61338,#61339,#61340,#61341,#61342,#61343,#61344,
#61345,#61346,#61347,#61348,#61349,#61350,#61351,#61352,#61353,#61354,#61355,
#61356,#61357,#61358,#61359,#61360,#61361,#61362,#61363,#61364,#61365,#61366,
#61367,#61368,#61369,#61370,#61371,#61372,#61373,#61374,#61375,#61376,#61377,
#61378,#61379,#61380,#61381,#61382,#61383,#61384,#61385,#61386,#61387,#61388,
#61389,#61390,#61391,#61392,#61393,#61394,#61395,#61396,#61397,#61398,#61399,
#61400,#61401,#61402,#61403,#61404,#61405,#61406,#61407,#61408,#61409,#61410,
#61411,#61412,#61413,#61414,#61415,#61416,#61417,#61418,#61419,#61420,#61421,
#61422,#61423,#61424,#61425,#61426,#61427,#61428,#61429,#61430,#61431,#61432,
#61433,#61434,#61435,#61436,#61437,#61438,#61439,#61440,#61441,#61442,#61443,
#61444,#61445,#61446,#61447,#61448,#61449,#61450,#61451,#61452,#61453,#61454,
#61455,#61456,#61457,#61458,#61459,#61460,#61461,#61462,#61463,#61464,#61465,
#61466,#61467,#61468,#61469,#61470,#61471,#61472,#61473,#61474,#61475,#61476,
#61477,#61478,#61479,#61480,#61481,#61482,#61483,#61484,#61485,#61486),
 .UNSPECIFIED.,.F.,.F.)
B_SPLINE_CURVE_WITH_KNOTS((6,1,1,1,1,1,1,1,1,1,1,1,1,1,1,1,1,1,1,1,1,1,
1,1,1,1,1,1,1,1,1,1,1,1,1,1,1,1,1,1,1,1,1,1,1,1,1,1,1,1,1,1,1,1,1,1,1,1,
1,1,1,1,1,1,1,1,1,1,1,1,1,1,1,1,1,1,1,1,1,1,1,1,1,1,1,1,1,1,1,1,1,1,1,1,
1,1,1,1,1,1,1,1,1,1,1,1,1,1,1,1,1,1,1,1,1,1,1,1,1,1,1,1,1,1,1,1,1,1,1,1,
1,1,1,1,1,1,1,1,1,1,1,1,1,1,1,1,1,1,1,1,1,1,1,1,1,1,1,1,1,1,1,1,1,1,1,1,
1,1,1,1,1,1,1,1,1,1,1,1,1,1,1,1,1,1,1,1,1,1,1,6),(-0.941429844431463,-0.940000000000001,
-0.935000000000001,-0.930000000000001,-0.925000000000001,-0.920000000000001,
-0.915000000000001,-0.910000000000001,-0.905000000000001,-0.900000000000001,
-0.895000000000001,-0.890000000000001,-0.885000000000001,-0.880000000000001,
-0.875000000000001,-0.870000000000001,-0.865000000000001,-0.860000000000001,
-0.855000000000001,-0.850000000000001,-0.845000000000001,-0.840000000000001,
-0.835000000000001,-0.830000000000001,-0.825000000000001,-0.820000000000001,
-0.815000000000001,-0.810000000000001,-0.805000000000001,-0.800000000000001,
-0.795000000000001,-0.790000000000001,-0.785000000000001,-0.780000000000001,
-0.775000000000001,-0.770000000000001,-0.765000000000001,-0.760000000000001,
-0.755000000000001,-0.750000000000001,-0.745000000000001,-0.740000000000001,
-0.735000000000001,-0.730000000000001,-0.725000000000001,-0.720000000000001,
-0.715000000000001,-0.710000000000001,-0.705000000000001,-0.700000000000001,
-0.695000000000001,-0.690000000000001,-0.685,-0.68,-0.675,-0.67,-0.665,
-0.66,-0.655,-0.65,-0.645,-0.64,-0.635,-0.63,-0.625,-0.62,-0.615,-0.61,
-0.605,-0.6,-0.595,-0.59,-0.585,-0.58,-0.575,-0.57,-0.565,-0.56,-0.555,
-0.55,-0.545,-0.54,-0.535,-0.53,-0.525,-0.52,-0.515,-0.51,-0.505,-0.5,-0.495,
-0.49,-0.485,-0.48,-0.475,-0.47,-0.465,-0.46,-0.455,-0.45,-0.445,-0.44,
-0.435,-0.43,-0.425,-0.42,-0.415,-0.41,-0.405,-0.4,-0.395,-0.39,-0.385,
-0.38,-0.375,-0.37,-0.365,-0.36,-0.355,-0.35,-0.345,-0.34,-0.335,-0.33,
-0.325,-0.32,-0.315,-0.31,-0.305,-0.3,-0.295,-0.29,-0.285,-0.28,-0.275,
-0.27,-0.265,-0.26,-0.255,-0.25,-0.245,-0.24,-0.235,-0.23,-0.225,-0.22,
-0.215,-0.21,-0.205,-0.2,-0.195,-0.19,-0.185,-0.18,-0.175,-0.17,-0.165,
-0.16,-0.155,-0.15,-0.145,-0.14,-0.135,-0.13,-0.125,-0.12,-0.115,-0.11,
-0.105,-0.1,-0.095,-0.09,-0.085,-0.08,-0.075,-0.07,-0.065,-0.06,-0.055,
-0.05,-0.045,-0.04,-0.035,-0.03,-0.025,-0.02,-0.015,-0.01,-0.005,0.),
 .UNSPECIFIED.)
CURVE()
GEOMETRIC_REPRESENTATION_ITEM()
RATIONAL_B_SPLINE_CURVE((1.,1.,1.,1.,1.,1.,1.,1.,1.,1.,1.,1.,1.,1.,1.,1.,
1.,1.,1.,1.,1.,1.,1.,1.,1.,1.,1.,1.,1.,1.,1.,1.,1.,1.,1.,1.,1.,1.,1.,1.,
1.,1.,1.,1.,1.,1.,1.,1.,1.,1.,1.,1.,1.,1.,1.,1.,1.,1.,1.,1.,1.,1.,1.,1.,
1.,1.,1.,1.,1.,1.,1.,1.,1.,1.,1.,1.,1.,1.,1.,1.,1.,1.,1.,1.,1.,1.,1.,1.,
1.,1.,1.,1.,1.,1.,1.,1.,1.,1.,1.,1.,1.,1.,1.,1.,1.,1.,1.,1.,1.,1.,1.,1.,
1.,1.,1.,1.,1.,1.,1.,1.,1.,1.,1.,1.,1.,1.,1.,1.,1.,1.,1.,1.,1.,1.,1.,1.,
1.,1.,1.,1.,1.,1.,1.,1.,1.,1.,1.,1.,1.,1.,1.,1.,1.,1.,1.,1.,1.,1.,1.,1.,
1.,1.,1.,1.,1.,1.,1.,1.,1.,1.,1.,1.,1.,1.,1.,1.,1.,1.,1.,1.,1.,1.,1.,1.,
1.,1.,1.,1.,1.,1.,1.,1.,1.,1.))
REPRESENTATION_ITEM('')
);
#423=(
BOUNDED_CURVE()
B_SPLINE_CURVE(5,(#61993,#61994,#61995,#61996,#61997,#61998,#61999,#62000,
#62001,#62002,#62003,#62004,#62005,#62006,#62007,#62008,#62009,#62010,#62011,
#62012,#62013,#62014,#62015,#62016,#62017,#62018,#62019,#62020,#62021,#62022,
#62023,#62024,#62025,#62026,#62027,#62028,#62029,#62030,#62031,#62032,#62033,
#62034,#62035,#62036,#62037,#62038,#62039,#62040,#62041,#62042,#62043,#62044,
#62045,#62046,#62047,#62048,#62049,#62050,#62051,#62052,#62053,#62054,#62055,
#62056,#62057,#62058,#62059,#62060,#62061,#62062,#62063,#62064,#62065,#62066,
#62067,#62068,#62069,#62070,#62071,#62072,#62073,#62074,#62075,#62076,#62077,
#62078,#62079,#62080,#62081,#62082,#62083,#62084,#62085,#62086,#62087,#62088,
#62089,#62090,#62091,#62092,#62093,#62094,#62095,#62096,#62097,#62098,#62099,
#62100,#62101,#62102,#62103,#62104,#62105,#62106,#62107,#62108,#62109,#62110,
#62111,#62112,#62113,#62114,#62115,#62116,#62117,#62118,#62119,#62120,#62121,
#62122,#62123,#62124,#62125,#62126,#62127,#62128,#62129,#62130,#62131,#62132,
#62133,#62134,#62135,#62136,#62137,#62138,#62139,#62140,#62141,#62142,#62143,
#62144,#62145,#62146,#62147,#62148,#62149,#62150,#62151,#62152,#62153,#62154,
#62155,#62156,#62157,#62158,#62159,#62160,#62161,#62162,#62163,#62164,#62165,
#62166,#62167,#62168,#62169,#62170,#62171,#62172,#62173,#62174,#62175,#62176,
#62177,#62178,#62179,#62180,#62181,#62182,#62183,#62184,#62185,#62186),
 .UNSPECIFIED.,.F.,.F.)
B_SPLINE_CURVE_WITH_KNOTS((6,1,1,1,1,1,1,1,1,1,1,1,1,1,1,1,1,1,1,1,1,1,
1,1,1,1,1,1,1,1,1,1,1,1,1,1,1,1,1,1,1,1,1,1,1,1,1,1,1,1,1,1,1,1,1,1,1,1,
1,1,1,1,1,1,1,1,1,1,1,1,1,1,1,1,1,1,1,1,1,1,1,1,1,1,1,1,1,1,1,1,1,1,1,1,
1,1,1,1,1,1,1,1,1,1,1,1,1,1,1,1,1,1,1,1,1,1,1,1,1,1,1,1,1,1,1,1,1,1,1,1,
1,1,1,1,1,1,1,1,1,1,1,1,1,1,1,1,1,1,1,1,1,1,1,1,1,1,1,1,1,1,1,1,1,1,1,1,
1,1,1,1,1,1,1,1,1,1,1,1,1,1,1,1,1,1,1,1,1,1,1,6),(0.,0.005,0.01,0.015,0.02,
0.025,0.03,0.035,0.04,0.045,0.05,0.055,0.06,0.065,0.07,0.075,0.08,0.085,
0.09,0.095,0.1,0.105,0.11,0.115,0.12,0.125,0.13,0.135,0.14,0.145,0.15,0.155,
0.16,0.165,0.17,0.175,0.18,0.185,0.19,0.195,0.2,0.205,0.21,0.215,0.22,0.225,
0.23,0.235,0.24,0.245,0.25,0.255,0.26,0.265,0.27,0.275,0.28,0.285,0.29,
0.295,0.3,0.305,0.31,0.315,0.32,0.325,0.33,0.335,0.34,0.345,0.35,0.355,
0.36,0.365,0.37,0.375,0.38,0.385,0.39,0.395,0.4,0.405,0.41,0.415,0.42,0.425,
0.43,0.435,0.44,0.445,0.45,0.455,0.46,0.465,0.47,0.475,0.48,0.485,0.49,
0.495,0.5,0.505,0.51,0.515,0.52,0.525,0.53,0.535,0.54,0.545,0.55,0.555,
0.56,0.565,0.57,0.575,0.58,0.585,0.59,0.595,0.6,0.605,0.61,0.615,0.62,0.625,
0.63,0.635,0.64,0.645,0.65,0.655,0.66,0.665,0.67,0.675,0.68,0.685,0.690000000000001,
0.695000000000001,0.700000000000001,0.705000000000001,0.710000000000001,
0.715000000000001,0.720000000000001,0.725000000000001,0.730000000000001,
0.735000000000001,0.740000000000001,0.745000000000001,0.750000000000001,
0.755000000000001,0.760000000000001,0.765000000000001,0.770000000000001,
0.775000000000001,0.780000000000001,0.785000000000001,0.790000000000001,
0.795000000000001,0.800000000000001,0.805000000000001,0.810000000000001,
0.815000000000001,0.820000000000001,0.825000000000001,0.830000000000001,
0.835000000000001,0.840000000000001,0.845000000000001,0.850000000000001,
0.855000000000001,0.860000000000001,0.865000000000001,0.870000000000001,
0.875000000000001,0.880000000000001,0.885000000000001,0.890000000000001,
0.895000000000001,0.900000000000001,0.905000000000001,0.910000000000001,
0.915000000000001,0.920000000000001,0.925000000000001,0.930000000000001,
0.935000000000001,0.940000000000001,0.941429844431297),.UNSPECIFIED.)
CURVE()
GEOMETRIC_REPRESENTATION_ITEM()
RATIONAL_B_SPLINE_CURVE((1.,1.,1.,1.,1.,1.,1.,1.,1.,1.,1.,1.,1.,1.,1.,1.,
1.,1.,1.,1.,1.,1.,1.,1.,1.,1.,1.,1.,1.,1.,1.,1.,1.,1.,1.,1.,1.,1.,1.,1.,
1.,1.,1.,1.,1.,1.,1.,1.,1.,1.,1.,1.,1.,1.,1.,1.,1.,1.,1.,1.,1.,1.,1.,1.,
1.,1.,1.,1.,1.,1.,1.,1.,1.,1.,1.,1.,1.,1.,1.,1.,1.,1.,1.,1.,1.,1.,1.,1.,
1.,1.,1.,1.,1.,1.,1.,1.,1.,1.,1.,1.,1.,1.,1.,1.,1.,1.,1.,1.,1.,1.,1.,1.,
1.,1.,1.,1.,1.,1.,1.,1.,1.,1.,1.,1.,1.,1.,1.,1.,1.,1.,1.,1.,1.,1.,1.,1.,
1.,1.,1.,1.,1.,1.,1.,1.,1.,1.,1.,1.,1.,1.,1.,1.,1.,1.,1.,1.,1.,1.,1.,1.,
1.,1.,1.,1.,1.,1.,1.,1.,1.,1.,1.,1.,1.,1.,1.,1.,1.,1.,1.,1.,1.,1.,1.,1.,
1.,1.,1.,1.,1.,1.,1.,1.,1.,1.))
REPRESENTATION_ITEM('')
);
#424=(
BOUNDED_CURVE()
B_SPLINE_CURVE(5,(#62189,#62190,#62191,#62192,#62193,#62194,#62195,#62196,
#62197,#62198,#62199,#62200,#62201,#62202,#62203,#62204,#62205,#62206,#62207,
#62208,#62209,#62210,#62211,#62212,#62213,#62214,#62215,#62216,#62217,#62218,
#62219,#62220,#62221,#62222,#62223,#62224,#62225,#62226,#62227,#62228,#62229,
#62230,#62231,#62232,#62233,#62234,#62235,#62236,#62237,#62238,#62239,#62240,
#62241,#62242,#62243,#62244,#62245,#62246,#62247,#62248,#62249,#62250,#62251,
#62252,#62253,#62254,#62255,#62256,#62257,#62258,#62259,#62260,#62261,#62262,
#62263,#62264,#62265,#62266,#62267,#62268,#62269,#62270,#62271,#62272,#62273,
#62274,#62275,#62276,#62277,#62278,#62279,#62280,#62281,#62282,#62283,#62284,
#62285,#62286,#62287,#62288,#62289,#62290,#62291,#62292,#62293,#62294,#62295,
#62296,#62297,#62298,#62299,#62300,#62301,#62302,#62303,#62304,#62305,#62306,
#62307,#62308,#62309,#62310,#62311,#62312,#62313,#62314,#62315,#62316,#62317,
#62318,#62319,#62320,#62321,#62322,#62323,#62324,#62325,#62326,#62327,#62328,
#62329,#62330,#62331,#62332,#62333,#62334,#62335,#62336,#62337,#62338,#62339,
#62340,#62341,#62342,#62343,#62344,#62345,#62346,#62347,#62348,#62349,#62350,
#62351,#62352,#62353,#62354,#62355,#62356,#62357,#62358,#62359,#62360,#62361,
#62362,#62363,#62364,#62365,#62366,#62367,#62368,#62369,#62370,#62371,#62372,
#62373,#62374,#62375,#62376,#62377,#62378,#62379,#62380,#62381,#62382),
 .UNSPECIFIED.,.F.,.F.)
B_SPLINE_CURVE_WITH_KNOTS((6,1,1,1,1,1,1,1,1,1,1,1,1,1,1,1,1,1,1,1,1,1,
1,1,1,1,1,1,1,1,1,1,1,1,1,1,1,1,1,1,1,1,1,1,1,1,1,1,1,1,1,1,1,1,1,1,1,1,
1,1,1,1,1,1,1,1,1,1,1,1,1,1,1,1,1,1,1,1,1,1,1,1,1,1,1,1,1,1,1,1,1,1,1,1,
1,1,1,1,1,1,1,1,1,1,1,1,1,1,1,1,1,1,1,1,1,1,1,1,1,1,1,1,1,1,1,1,1,1,1,1,
1,1,1,1,1,1,1,1,1,1,1,1,1,1,1,1,1,1,1,1,1,1,1,1,1,1,1,1,1,1,1,1,1,1,1,1,
1,1,1,1,1,1,1,1,1,1,1,1,1,1,1,1,1,1,1,1,1,1,1,6),(-0.941429844431289,-0.940000000000001,
-0.935000000000001,-0.930000000000001,-0.925000000000001,-0.920000000000001,
-0.915000000000001,-0.910000000000001,-0.905000000000001,-0.900000000000001,
-0.895000000000001,-0.890000000000001,-0.885000000000001,-0.880000000000001,
-0.875000000000001,-0.870000000000001,-0.865000000000001,-0.860000000000001,
-0.855000000000001,-0.850000000000001,-0.845000000000001,-0.840000000000001,
-0.835000000000001,-0.830000000000001,-0.825000000000001,-0.820000000000001,
-0.815000000000001,-0.810000000000001,-0.805000000000001,-0.800000000000001,
-0.795000000000001,-0.790000000000001,-0.785000000000001,-0.780000000000001,
-0.775000000000001,-0.770000000000001,-0.765000000000001,-0.760000000000001,
-0.755000000000001,-0.750000000000001,-0.745000000000001,-0.740000000000001,
-0.735000000000001,-0.730000000000001,-0.725000000000001,-0.720000000000001,
-0.715000000000001,-0.710000000000001,-0.705000000000001,-0.700000000000001,
-0.695000000000001,-0.690000000000001,-0.685,-0.68,-0.675,-0.67,-0.665,
-0.66,-0.655,-0.65,-0.645,-0.64,-0.635,-0.63,-0.625,-0.62,-0.615,-0.61,
-0.605,-0.6,-0.595,-0.59,-0.585,-0.58,-0.575,-0.57,-0.565,-0.56,-0.555,
-0.55,-0.545,-0.54,-0.535,-0.53,-0.525,-0.52,-0.515,-0.51,-0.505,-0.5,-0.495,
-0.49,-0.485,-0.48,-0.475,-0.47,-0.465,-0.46,-0.455,-0.45,-0.445,-0.44,
-0.435,-0.43,-0.425,-0.42,-0.415,-0.41,-0.405,-0.4,-0.395,-0.39,-0.385,
-0.38,-0.375,-0.37,-0.365,-0.36,-0.355,-0.35,-0.345,-0.34,-0.335,-0.33,
-0.325,-0.32,-0.315,-0.31,-0.305,-0.3,-0.295,-0.29,-0.285,-0.28,-0.275,
-0.27,-0.265,-0.26,-0.255,-0.25,-0.245,-0.24,-0.235,-0.23,-0.225,-0.22,
-0.215,-0.21,-0.205,-0.2,-0.195,-0.19,-0.185,-0.18,-0.175,-0.17,-0.165,
-0.16,-0.155,-0.15,-0.145,-0.14,-0.135,-0.13,-0.125,-0.12,-0.115,-0.11,
-0.105,-0.1,-0.095,-0.09,-0.085,-0.08,-0.075,-0.07,-0.065,-0.06,-0.055,
-0.05,-0.045,-0.04,-0.035,-0.03,-0.025,-0.02,-0.015,-0.01,-0.005,0.),
 .UNSPECIFIED.)
CURVE()
GEOMETRIC_REPRESENTATION_ITEM()
RATIONAL_B_SPLINE_CURVE((1.,1.,1.,1.,1.,1.,1.,1.,1.,1.,1.,1.,1.,1.,1.,1.,
1.,1.,1.,1.,1.,1.,1.,1.,1.,1.,1.,1.,1.,1.,1.,1.,1.,1.,1.,1.,1.,1.,1.,1.,
1.,1.,1.,1.,1.,1.,1.,1.,1.,1.,1.,1.,1.,1.,1.,1.,1.,1.,1.,1.,1.,1.,1.,1.,
1.,1.,1.,1.,1.,1.,1.,1.,1.,1.,1.,1.,1.,1.,1.,1.,1.,1.,1.,1.,1.,1.,1.,1.,
1.,1.,1.,1.,1.,1.,1.,1.,1.,1.,1.,1.,1.,1.,1.,1.,1.,1.,1.,1.,1.,1.,1.,1.,
1.,1.,1.,1.,1.,1.,1.,1.,1.,1.,1.,1.,1.,1.,1.,1.,1.,1.,1.,1.,1.,1.,1.,1.,
1.,1.,1.,1.,1.,1.,1.,1.,1.,1.,1.,1.,1.,1.,1.,1.,1.,1.,1.,1.,1.,1.,1.,1.,
1.,1.,1.,1.,1.,1.,1.,1.,1.,1.,1.,1.,1.,1.,1.,1.,1.,1.,1.,1.,1.,1.,1.,1.,
1.,1.,1.,1.,1.,1.,1.,1.,1.,1.))
REPRESENTATION_ITEM('')
);
#425=(
BOUNDED_CURVE()
B_SPLINE_CURVE(5,(#62889,#62890,#62891,#62892,#62893,#62894,#62895,#62896,
#62897,#62898,#62899,#62900,#62901,#62902,#62903,#62904,#62905,#62906,#62907,
#62908,#62909,#62910,#62911,#62912,#62913,#62914,#62915,#62916,#62917,#62918,
#62919,#62920,#62921,#62922,#62923,#62924,#62925,#62926,#62927,#62928,#62929,
#62930,#62931,#62932,#62933,#62934,#62935,#62936,#62937,#62938,#62939,#62940,
#62941,#62942,#62943,#62944,#62945,#62946,#62947,#62948,#62949,#62950,#62951,
#62952,#62953,#62954,#62955,#62956,#62957,#62958,#62959,#62960,#62961,#62962,
#62963,#62964,#62965,#62966,#62967,#62968,#62969,#62970,#62971,#62972,#62973,
#62974,#62975,#62976,#62977,#62978,#62979,#62980,#62981,#62982,#62983,#62984,
#62985,#62986,#62987,#62988,#62989,#62990,#62991,#62992,#62993,#62994,#62995,
#62996,#62997,#62998,#62999,#63000,#63001,#63002,#63003,#63004,#63005,#63006,
#63007,#63008,#63009,#63010,#63011,#63012,#63013,#63014,#63015,#63016,#63017,
#63018,#63019,#63020,#63021,#63022,#63023,#63024,#63025,#63026,#63027,#63028,
#63029,#63030,#63031,#63032,#63033,#63034,#63035,#63036,#63037,#63038,#63039,
#63040,#63041,#63042,#63043,#63044,#63045,#63046,#63047,#63048,#63049,#63050,
#63051,#63052,#63053,#63054,#63055,#63056,#63057,#63058,#63059,#63060,#63061,
#63062,#63063,#63064,#63065,#63066,#63067,#63068,#63069,#63070,#63071,#63072,
#63073,#63074,#63075,#63076,#63077,#63078,#63079,#63080,#63081,#63082),
 .UNSPECIFIED.,.F.,.F.)
B_SPLINE_CURVE_WITH_KNOTS((6,1,1,1,1,1,1,1,1,1,1,1,1,1,1,1,1,1,1,1,1,1,
1,1,1,1,1,1,1,1,1,1,1,1,1,1,1,1,1,1,1,1,1,1,1,1,1,1,1,1,1,1,1,1,1,1,1,1,
1,1,1,1,1,1,1,1,1,1,1,1,1,1,1,1,1,1,1,1,1,1,1,1,1,1,1,1,1,1,1,1,1,1,1,1,
1,1,1,1,1,1,1,1,1,1,1,1,1,1,1,1,1,1,1,1,1,1,1,1,1,1,1,1,1,1,1,1,1,1,1,1,
1,1,1,1,1,1,1,1,1,1,1,1,1,1,1,1,1,1,1,1,1,1,1,1,1,1,1,1,1,1,1,1,1,1,1,1,
1,1,1,1,1,1,1,1,1,1,1,1,1,1,1,1,1,1,1,1,1,1,1,6),(0.,0.005,0.01,0.015,0.02,
0.025,0.03,0.035,0.04,0.045,0.05,0.055,0.06,0.065,0.07,0.075,0.08,0.085,
0.09,0.095,0.1,0.105,0.11,0.115,0.12,0.125,0.13,0.135,0.14,0.145,0.15,0.155,
0.16,0.165,0.17,0.175,0.18,0.185,0.19,0.195,0.2,0.205,0.21,0.215,0.22,0.225,
0.23,0.235,0.24,0.245,0.25,0.255,0.26,0.265,0.27,0.275,0.28,0.285,0.29,
0.295,0.3,0.305,0.31,0.315,0.32,0.325,0.33,0.335,0.34,0.345,0.35,0.355,
0.36,0.365,0.37,0.375,0.38,0.385,0.39,0.395,0.4,0.405,0.41,0.415,0.42,0.425,
0.43,0.435,0.44,0.445,0.45,0.455,0.46,0.465,0.47,0.475,0.48,0.485,0.49,
0.495,0.5,0.505,0.51,0.515,0.52,0.525,0.53,0.535,0.54,0.545,0.55,0.555,
0.56,0.565,0.57,0.575,0.58,0.585,0.59,0.595,0.6,0.605,0.61,0.615,0.62,0.625,
0.63,0.635,0.64,0.645,0.65,0.655,0.66,0.665,0.67,0.675,0.68,0.685,0.690000000000001,
0.695000000000001,0.700000000000001,0.705000000000001,0.710000000000001,
0.715000000000001,0.720000000000001,0.725000000000001,0.730000000000001,
0.735000000000001,0.740000000000001,0.745000000000001,0.750000000000001,
0.755000000000001,0.760000000000001,0.765000000000001,0.770000000000001,
0.775000000000001,0.780000000000001,0.785000000000001,0.790000000000001,
0.795000000000001,0.800000000000001,0.805000000000001,0.810000000000001,
0.815000000000001,0.820000000000001,0.825000000000001,0.830000000000001,
0.835000000000001,0.840000000000001,0.845000000000001,0.850000000000001,
0.855000000000001,0.860000000000001,0.865000000000001,0.870000000000001,
0.875000000000001,0.880000000000001,0.885000000000001,0.890000000000001,
0.895000000000001,0.900000000000001,0.905000000000001,0.910000000000001,
0.915000000000001,0.920000000000001,0.925000000000001,0.930000000000001,
0.935000000000001,0.940000000000001,0.941429844431249),.UNSPECIFIED.)
CURVE()
GEOMETRIC_REPRESENTATION_ITEM()
RATIONAL_B_SPLINE_CURVE((1.,1.,1.,1.,1.,1.,1.,1.,1.,1.,1.,1.,1.,1.,1.,1.,
1.,1.,1.,1.,1.,1.,1.,1.,1.,1.,1.,1.,1.,1.,1.,1.,1.,1.,1.,1.,1.,1.,1.,1.,
1.,1.,1.,1.,1.,1.,1.,1.,1.,1.,1.,1.,1.,1.,1.,1.,1.,1.,1.,1.,1.,1.,1.,1.,
1.,1.,1.,1.,1.,1.,1.,1.,1.,1.,1.,1.,1.,1.,1.,1.,1.,1.,1.,1.,1.,1.,1.,1.,
1.,1.,1.,1.,1.,1.,1.,1.,1.,1.,1.,1.,1.,1.,1.,1.,1.,1.,1.,1.,1.,1.,1.,1.,
1.,1.,1.,1.,1.,1.,1.,1.,1.,1.,1.,1.,1.,1.,1.,1.,1.,1.,1.,1.,1.,1.,1.,1.,
1.,1.,1.,1.,1.,1.,1.,1.,1.,1.,1.,1.,1.,1.,1.,1.,1.,1.,1.,1.,1.,1.,1.,1.,
1.,1.,1.,1.,1.,1.,1.,1.,1.,1.,1.,1.,1.,1.,1.,1.,1.,1.,1.,1.,1.,1.,1.,1.,
1.,1.,1.,1.,1.,1.,1.,1.,1.,1.))
REPRESENTATION_ITEM('')
);
#426=(
BOUNDED_CURVE()
B_SPLINE_CURVE(5,(#63085,#63086,#63087,#63088,#63089,#63090,#63091,#63092,
#63093,#63094,#63095,#63096,#63097,#63098,#63099,#63100,#63101,#63102,#63103,
#63104,#63105,#63106,#63107,#63108,#63109,#63110,#63111,#63112,#63113,#63114,
#63115,#63116,#63117,#63118,#63119,#63120,#63121,#63122,#63123,#63124,#63125,
#63126,#63127,#63128,#63129,#63130,#63131,#63132,#63133,#63134,#63135,#63136,
#63137,#63138,#63139,#63140,#63141,#63142,#63143,#63144,#63145,#63146,#63147,
#63148,#63149,#63150,#63151,#63152,#63153,#63154,#63155,#63156,#63157,#63158,
#63159,#63160,#63161,#63162,#63163,#63164,#63165,#63166,#63167,#63168,#63169,
#63170,#63171,#63172,#63173,#63174,#63175,#63176,#63177,#63178,#63179,#63180,
#63181,#63182,#63183,#63184,#63185,#63186,#63187,#63188,#63189,#63190,#63191,
#63192,#63193,#63194,#63195,#63196,#63197,#63198,#63199,#63200,#63201,#63202,
#63203,#63204,#63205,#63206,#63207,#63208,#63209,#63210,#63211,#63212,#63213,
#63214,#63215,#63216,#63217,#63218,#63219,#63220,#63221,#63222,#63223,#63224,
#63225,#63226,#63227,#63228,#63229,#63230,#63231,#63232,#63233,#63234,#63235,
#63236,#63237,#63238,#63239,#63240,#63241,#63242,#63243,#63244,#63245,#63246,
#63247,#63248,#63249,#63250,#63251,#63252,#63253,#63254,#63255,#63256,#63257,
#63258,#63259,#63260,#63261,#63262,#63263,#63264,#63265,#63266,#63267,#63268,
#63269,#63270,#63271,#63272,#63273,#63274,#63275,#63276,#63277,#63278),
 .UNSPECIFIED.,.F.,.F.)
B_SPLINE_CURVE_WITH_KNOTS((6,1,1,1,1,1,1,1,1,1,1,1,1,1,1,1,1,1,1,1,1,1,
1,1,1,1,1,1,1,1,1,1,1,1,1,1,1,1,1,1,1,1,1,1,1,1,1,1,1,1,1,1,1,1,1,1,1,1,
1,1,1,1,1,1,1,1,1,1,1,1,1,1,1,1,1,1,1,1,1,1,1,1,1,1,1,1,1,1,1,1,1,1,1,1,
1,1,1,1,1,1,1,1,1,1,1,1,1,1,1,1,1,1,1,1,1,1,1,1,1,1,1,1,1,1,1,1,1,1,1,1,
1,1,1,1,1,1,1,1,1,1,1,1,1,1,1,1,1,1,1,1,1,1,1,1,1,1,1,1,1,1,1,1,1,1,1,1,
1,1,1,1,1,1,1,1,1,1,1,1,1,1,1,1,1,1,1,1,1,1,1,6),(-0.94142984443124,-0.940000000000001,
-0.935000000000001,-0.930000000000001,-0.925000000000001,-0.920000000000001,
-0.915000000000001,-0.910000000000001,-0.905000000000001,-0.900000000000001,
-0.895000000000001,-0.890000000000001,-0.885000000000001,-0.880000000000001,
-0.875000000000001,-0.870000000000001,-0.865000000000001,-0.860000000000001,
-0.855000000000001,-0.850000000000001,-0.845000000000001,-0.840000000000001,
-0.835000000000001,-0.830000000000001,-0.825000000000001,-0.820000000000001,
-0.815000000000001,-0.810000000000001,-0.805000000000001,-0.800000000000001,
-0.795000000000001,-0.790000000000001,-0.785000000000001,-0.780000000000001,
-0.775000000000001,-0.770000000000001,-0.765000000000001,-0.760000000000001,
-0.755000000000001,-0.750000000000001,-0.745000000000001,-0.740000000000001,
-0.735000000000001,-0.730000000000001,-0.725000000000001,-0.720000000000001,
-0.715000000000001,-0.710000000000001,-0.705000000000001,-0.700000000000001,
-0.695000000000001,-0.690000000000001,-0.685,-0.68,-0.675,-0.67,-0.665,
-0.66,-0.655,-0.65,-0.645,-0.64,-0.635,-0.63,-0.625,-0.62,-0.615,-0.61,
-0.605,-0.6,-0.595,-0.59,-0.585,-0.58,-0.575,-0.57,-0.565,-0.56,-0.555,
-0.55,-0.545,-0.54,-0.535,-0.53,-0.525,-0.52,-0.515,-0.51,-0.505,-0.5,-0.495,
-0.49,-0.485,-0.48,-0.475,-0.47,-0.465,-0.46,-0.455,-0.45,-0.445,-0.44,
-0.435,-0.43,-0.425,-0.42,-0.415,-0.41,-0.405,-0.4,-0.395,-0.39,-0.385,
-0.38,-0.375,-0.37,-0.365,-0.36,-0.355,-0.35,-0.345,-0.34,-0.335,-0.33,
-0.325,-0.32,-0.315,-0.31,-0.305,-0.3,-0.295,-0.29,-0.285,-0.28,-0.275,
-0.27,-0.265,-0.26,-0.255,-0.25,-0.245,-0.24,-0.235,-0.23,-0.225,-0.22,
-0.215,-0.21,-0.205,-0.2,-0.195,-0.19,-0.185,-0.18,-0.175,-0.17,-0.165,
-0.16,-0.155,-0.15,-0.145,-0.14,-0.135,-0.13,-0.125,-0.12,-0.115,-0.11,
-0.105,-0.1,-0.095,-0.09,-0.085,-0.08,-0.075,-0.07,-0.065,-0.06,-0.055,
-0.05,-0.045,-0.04,-0.035,-0.03,-0.025,-0.02,-0.015,-0.01,-0.005,0.),
 .UNSPECIFIED.)
CURVE()
GEOMETRIC_REPRESENTATION_ITEM()
RATIONAL_B_SPLINE_CURVE((1.,1.,1.,1.,1.,1.,1.,1.,1.,1.,1.,1.,1.,1.,1.,1.,
1.,1.,1.,1.,1.,1.,1.,1.,1.,1.,1.,1.,1.,1.,1.,1.,1.,1.,1.,1.,1.,1.,1.,1.,
1.,1.,1.,1.,1.,1.,1.,1.,1.,1.,1.,1.,1.,1.,1.,1.,1.,1.,1.,1.,1.,1.,1.,1.,
1.,1.,1.,1.,1.,1.,1.,1.,1.,1.,1.,1.,1.,1.,1.,1.,1.,1.,1.,1.,1.,1.,1.,1.,
1.,1.,1.,1.,1.,1.,1.,1.,1.,1.,1.,1.,1.,1.,1.,1.,1.,1.,1.,1.,1.,1.,1.,1.,
1.,1.,1.,1.,1.,1.,1.,1.,1.,1.,1.,1.,1.,1.,1.,1.,1.,1.,1.,1.,1.,1.,1.,1.,
1.,1.,1.,1.,1.,1.,1.,1.,1.,1.,1.,1.,1.,1.,1.,1.,1.,1.,1.,1.,1.,1.,1.,1.,
1.,1.,1.,1.,1.,1.,1.,1.,1.,1.,1.,1.,1.,1.,1.,1.,1.,1.,1.,1.,1.,1.,1.,1.,
1.,1.,1.,1.,1.,1.,1.,1.,1.,1.))
REPRESENTATION_ITEM('')
);
#427=(
BOUNDED_CURVE()
B_SPLINE_CURVE(5,(#63785,#63786,#63787,#63788,#63789,#63790,#63791,#63792,
#63793,#63794,#63795,#63796,#63797,#63798,#63799,#63800,#63801,#63802,#63803,
#63804,#63805,#63806,#63807,#63808,#63809,#63810,#63811,#63812,#63813,#63814,
#63815,#63816,#63817,#63818,#63819,#63820,#63821,#63822,#63823,#63824,#63825,
#63826,#63827,#63828,#63829,#63830,#63831,#63832,#63833,#63834,#63835,#63836,
#63837,#63838,#63839,#63840,#63841,#63842,#63843,#63844,#63845,#63846,#63847,
#63848,#63849,#63850,#63851,#63852,#63853,#63854,#63855,#63856,#63857,#63858,
#63859,#63860,#63861,#63862,#63863,#63864,#63865,#63866,#63867,#63868,#63869,
#63870,#63871,#63872,#63873,#63874,#63875,#63876,#63877,#63878,#63879,#63880,
#63881,#63882,#63883,#63884,#63885,#63886,#63887,#63888,#63889,#63890,#63891,
#63892,#63893,#63894,#63895,#63896,#63897,#63898,#63899,#63900,#63901,#63902,
#63903,#63904,#63905,#63906,#63907,#63908,#63909,#63910,#63911,#63912,#63913,
#63914,#63915,#63916,#63917,#63918,#63919,#63920,#63921,#63922,#63923,#63924,
#63925,#63926,#63927,#63928,#63929,#63930,#63931,#63932,#63933,#63934,#63935,
#63936,#63937,#63938,#63939,#63940,#63941,#63942,#63943,#63944,#63945,#63946,
#63947,#63948,#63949,#63950,#63951,#63952,#63953,#63954,#63955,#63956,#63957,
#63958,#63959,#63960,#63961,#63962,#63963,#63964,#63965,#63966,#63967,#63968,
#63969,#63970,#63971,#63972,#63973,#63974,#63975,#63976,#63977,#63978),
 .UNSPECIFIED.,.F.,.F.)
B_SPLINE_CURVE_WITH_KNOTS((6,1,1,1,1,1,1,1,1,1,1,1,1,1,1,1,1,1,1,1,1,1,
1,1,1,1,1,1,1,1,1,1,1,1,1,1,1,1,1,1,1,1,1,1,1,1,1,1,1,1,1,1,1,1,1,1,1,1,
1,1,1,1,1,1,1,1,1,1,1,1,1,1,1,1,1,1,1,1,1,1,1,1,1,1,1,1,1,1,1,1,1,1,1,1,
1,1,1,1,1,1,1,1,1,1,1,1,1,1,1,1,1,1,1,1,1,1,1,1,1,1,1,1,1,1,1,1,1,1,1,1,
1,1,1,1,1,1,1,1,1,1,1,1,1,1,1,1,1,1,1,1,1,1,1,1,1,1,1,1,1,1,1,1,1,1,1,1,
1,1,1,1,1,1,1,1,1,1,1,1,1,1,1,1,1,1,1,1,1,1,1,6),(0.,0.005,0.01,0.015,0.02,
0.025,0.03,0.035,0.04,0.045,0.05,0.055,0.06,0.065,0.07,0.075,0.08,0.085,
0.09,0.095,0.1,0.105,0.11,0.115,0.12,0.125,0.13,0.135,0.14,0.145,0.15,0.155,
0.16,0.165,0.17,0.175,0.18,0.185,0.19,0.195,0.2,0.205,0.21,0.215,0.22,0.225,
0.23,0.235,0.24,0.245,0.25,0.255,0.26,0.265,0.27,0.275,0.28,0.285,0.29,
0.295,0.3,0.305,0.31,0.315,0.32,0.325,0.33,0.335,0.34,0.345,0.35,0.355,
0.36,0.365,0.37,0.375,0.38,0.385,0.39,0.395,0.4,0.405,0.41,0.415,0.42,0.425,
0.43,0.435,0.44,0.445,0.45,0.455,0.46,0.465,0.47,0.475,0.48,0.485,0.49,
0.495,0.5,0.505,0.51,0.515,0.52,0.525,0.53,0.535,0.54,0.545,0.55,0.555,
0.56,0.565,0.57,0.575,0.58,0.585,0.59,0.595,0.6,0.605,0.61,0.615,0.62,0.625,
0.63,0.635,0.64,0.645,0.65,0.655,0.66,0.665,0.67,0.675,0.68,0.685,0.690000000000001,
0.695000000000001,0.700000000000001,0.705000000000001,0.710000000000001,
0.715000000000001,0.720000000000001,0.725000000000001,0.730000000000001,
0.735000000000001,0.740000000000001,0.745000000000001,0.750000000000001,
0.755000000000001,0.760000000000001,0.765000000000001,0.770000000000001,
0.775000000000001,0.780000000000001,0.785000000000001,0.790000000000001,
0.795000000000001,0.800000000000001,0.805000000000001,0.810000000000001,
0.815000000000001,0.820000000000001,0.825000000000001,0.830000000000001,
0.835000000000001,0.840000000000001,0.845000000000001,0.850000000000001,
0.855000000000001,0.860000000000001,0.865000000000001,0.870000000000001,
0.875000000000001,0.880000000000001,0.885000000000001,0.890000000000001,
0.895000000000001,0.900000000000001,0.905000000000001,0.910000000000001,
0.915000000000001,0.920000000000001,0.925000000000001,0.930000000000001,
0.935000000000001,0.940000000000001,0.941429844431314),.UNSPECIFIED.)
CURVE()
GEOMETRIC_REPRESENTATION_ITEM()
RATIONAL_B_SPLINE_CURVE((1.,1.,1.,1.,1.,1.,1.,1.,1.,1.,1.,1.,1.,1.,1.,1.,
1.,1.,1.,1.,1.,1.,1.,1.,1.,1.,1.,1.,1.,1.,1.,1.,1.,1.,1.,1.,1.,1.,1.,1.,
1.,1.,1.,1.,1.,1.,1.,1.,1.,1.,1.,1.,1.,1.,1.,1.,1.,1.,1.,1.,1.,1.,1.,1.,
1.,1.,1.,1.,1.,1.,1.,1.,1.,1.,1.,1.,1.,1.,1.,1.,1.,1.,1.,1.,1.,1.,1.,1.,
1.,1.,1.,1.,1.,1.,1.,1.,1.,1.,1.,1.,1.,1.,1.,1.,1.,1.,1.,1.,1.,1.,1.,1.,
1.,1.,1.,1.,1.,1.,1.,1.,1.,1.,1.,1.,1.,1.,1.,1.,1.,1.,1.,1.,1.,1.,1.,1.,
1.,1.,1.,1.,1.,1.,1.,1.,1.,1.,1.,1.,1.,1.,1.,1.,1.,1.,1.,1.,1.,1.,1.,1.,
1.,1.,1.,1.,1.,1.,1.,1.,1.,1.,1.,1.,1.,1.,1.,1.,1.,1.,1.,1.,1.,1.,1.,1.,
1.,1.,1.,1.,1.,1.,1.,1.,1.,1.))
REPRESENTATION_ITEM('')
);
#428=(
BOUNDED_CURVE()
B_SPLINE_CURVE(5,(#63981,#63982,#63983,#63984,#63985,#63986,#63987,#63988,
#63989,#63990,#63991,#63992,#63993,#63994,#63995,#63996,#63997,#63998,#63999,
#64000,#64001,#64002,#64003,#64004,#64005,#64006,#64007,#64008,#64009,#64010,
#64011,#64012,#64013,#64014,#64015,#64016,#64017,#64018,#64019,#64020,#64021,
#64022,#64023,#64024,#64025,#64026,#64027,#64028,#64029,#64030,#64031,#64032,
#64033,#64034,#64035,#64036,#64037,#64038,#64039,#64040,#64041,#64042,#64043,
#64044,#64045,#64046,#64047,#64048,#64049,#64050,#64051,#64052,#64053,#64054,
#64055,#64056,#64057,#64058,#64059,#64060,#64061,#64062,#64063,#64064,#64065,
#64066,#64067,#64068,#64069,#64070,#64071,#64072,#64073,#64074,#64075,#64076,
#64077,#64078,#64079,#64080,#64081,#64082,#64083,#64084,#64085,#64086,#64087,
#64088,#64089,#64090,#64091,#64092,#64093,#64094,#64095,#64096,#64097,#64098,
#64099,#64100,#64101,#64102,#64103,#64104,#64105,#64106,#64107,#64108,#64109,
#64110,#64111,#64112,#64113,#64114,#64115,#64116,#64117,#64118,#64119,#64120,
#64121,#64122,#64123,#64124,#64125,#64126,#64127,#64128,#64129,#64130,#64131,
#64132,#64133,#64134,#64135,#64136,#64137,#64138,#64139,#64140,#64141,#64142,
#64143,#64144,#64145,#64146,#64147,#64148,#64149,#64150,#64151,#64152,#64153,
#64154,#64155,#64156,#64157,#64158,#64159,#64160,#64161,#64162,#64163,#64164,
#64165,#64166,#64167,#64168,#64169,#64170,#64171,#64172,#64173,#64174),
 .UNSPECIFIED.,.F.,.F.)
B_SPLINE_CURVE_WITH_KNOTS((6,1,1,1,1,1,1,1,1,1,1,1,1,1,1,1,1,1,1,1,1,1,
1,1,1,1,1,1,1,1,1,1,1,1,1,1,1,1,1,1,1,1,1,1,1,1,1,1,1,1,1,1,1,1,1,1,1,1,
1,1,1,1,1,1,1,1,1,1,1,1,1,1,1,1,1,1,1,1,1,1,1,1,1,1,1,1,1,1,1,1,1,1,1,1,
1,1,1,1,1,1,1,1,1,1,1,1,1,1,1,1,1,1,1,1,1,1,1,1,1,1,1,1,1,1,1,1,1,1,1,1,
1,1,1,1,1,1,1,1,1,1,1,1,1,1,1,1,1,1,1,1,1,1,1,1,1,1,1,1,1,1,1,1,1,1,1,1,
1,1,1,1,1,1,1,1,1,1,1,1,1,1,1,1,1,1,1,1,1,1,1,6),(-0.941429844431327,-0.940000000000001,
-0.935000000000001,-0.930000000000001,-0.925000000000001,-0.920000000000001,
-0.915000000000001,-0.910000000000001,-0.905000000000001,-0.900000000000001,
-0.895000000000001,-0.890000000000001,-0.885000000000001,-0.880000000000001,
-0.875000000000001,-0.870000000000001,-0.865000000000001,-0.860000000000001,
-0.855000000000001,-0.850000000000001,-0.845000000000001,-0.840000000000001,
-0.835000000000001,-0.830000000000001,-0.825000000000001,-0.820000000000001,
-0.815000000000001,-0.810000000000001,-0.805000000000001,-0.800000000000001,
-0.795000000000001,-0.790000000000001,-0.785000000000001,-0.780000000000001,
-0.775000000000001,-0.770000000000001,-0.765000000000001,-0.760000000000001,
-0.755000000000001,-0.750000000000001,-0.745000000000001,-0.740000000000001,
-0.735000000000001,-0.730000000000001,-0.725000000000001,-0.720000000000001,
-0.715000000000001,-0.710000000000001,-0.705000000000001,-0.700000000000001,
-0.695000000000001,-0.690000000000001,-0.685,-0.68,-0.675,-0.67,-0.665,
-0.66,-0.655,-0.65,-0.645,-0.64,-0.635,-0.63,-0.625,-0.62,-0.615,-0.61,
-0.605,-0.6,-0.595,-0.59,-0.585,-0.58,-0.575,-0.57,-0.565,-0.56,-0.555,
-0.55,-0.545,-0.54,-0.535,-0.53,-0.525,-0.52,-0.515,-0.51,-0.505,-0.5,-0.495,
-0.49,-0.485,-0.48,-0.475,-0.47,-0.465,-0.46,-0.455,-0.45,-0.445,-0.44,
-0.435,-0.43,-0.425,-0.42,-0.415,-0.41,-0.405,-0.4,-0.395,-0.39,-0.385,
-0.38,-0.375,-0.37,-0.365,-0.36,-0.355,-0.35,-0.345,-0.34,-0.335,-0.33,
-0.325,-0.32,-0.315,-0.31,-0.305,-0.3,-0.295,-0.29,-0.285,-0.28,-0.275,
-0.27,-0.265,-0.26,-0.255,-0.25,-0.245,-0.24,-0.235,-0.23,-0.225,-0.22,
-0.215,-0.21,-0.205,-0.2,-0.195,-0.19,-0.185,-0.18,-0.175,-0.17,-0.165,
-0.16,-0.155,-0.15,-0.145,-0.14,-0.135,-0.13,-0.125,-0.12,-0.115,-0.11,
-0.105,-0.1,-0.095,-0.09,-0.085,-0.08,-0.075,-0.07,-0.065,-0.06,-0.055,
-0.05,-0.045,-0.04,-0.035,-0.03,-0.025,-0.02,-0.015,-0.01,-0.005,0.),
 .UNSPECIFIED.)
CURVE()
GEOMETRIC_REPRESENTATION_ITEM()
RATIONAL_B_SPLINE_CURVE((1.,1.,1.,1.,1.,1.,1.,1.,1.,1.,1.,1.,1.,1.,1.,1.,
1.,1.,1.,1.,1.,1.,1.,1.,1.,1.,1.,1.,1.,1.,1.,1.,1.,1.,1.,1.,1.,1.,1.,1.,
1.,1.,1.,1.,1.,1.,1.,1.,1.,1.,1.,1.,1.,1.,1.,1.,1.,1.,1.,1.,1.,1.,1.,1.,
1.,1.,1.,1.,1.,1.,1.,1.,1.,1.,1.,1.,1.,1.,1.,1.,1.,1.,1.,1.,1.,1.,1.,1.,
1.,1.,1.,1.,1.,1.,1.,1.,1.,1.,1.,1.,1.,1.,1.,1.,1.,1.,1.,1.,1.,1.,1.,1.,
1.,1.,1.,1.,1.,1.,1.,1.,1.,1.,1.,1.,1.,1.,1.,1.,1.,1.,1.,1.,1.,1.,1.,1.,
1.,1.,1.,1.,1.,1.,1.,1.,1.,1.,1.,1.,1.,1.,1.,1.,1.,1.,1.,1.,1.,1.,1.,1.,
1.,1.,1.,1.,1.,1.,1.,1.,1.,1.,1.,1.,1.,1.,1.,1.,1.,1.,1.,1.,1.,1.,1.,1.,
1.,1.,1.,1.,1.,1.,1.,1.,1.,1.))
REPRESENTATION_ITEM('')
);
#429=(
BOUNDED_CURVE()
B_SPLINE_CURVE(5,(#64681,#64682,#64683,#64684,#64685,#64686,#64687,#64688,
#64689,#64690,#64691,#64692,#64693,#64694,#64695,#64696,#64697,#64698,#64699,
#64700,#64701,#64702,#64703,#64704,#64705,#64706,#64707,#64708,#64709,#64710,
#64711,#64712,#64713,#64714,#64715,#64716,#64717,#64718,#64719,#64720,#64721,
#64722,#64723,#64724,#64725,#64726,#64727,#64728,#64729,#64730,#64731,#64732,
#64733,#64734,#64735,#64736,#64737,#64738,#64739,#64740,#64741,#64742,#64743,
#64744,#64745,#64746,#64747,#64748,#64749,#64750,#64751,#64752,#64753,#64754,
#64755,#64756,#64757,#64758,#64759,#64760,#64761,#64762,#64763,#64764,#64765,
#64766,#64767,#64768,#64769,#64770,#64771,#64772,#64773,#64774,#64775,#64776,
#64777,#64778,#64779,#64780,#64781,#64782,#64783,#64784,#64785,#64786,#64787,
#64788,#64789,#64790,#64791,#64792,#64793,#64794,#64795,#64796,#64797,#64798,
#64799,#64800,#64801,#64802,#64803,#64804,#64805,#64806,#64807,#64808,#64809,
#64810,#64811,#64812,#64813,#64814,#64815,#64816,#64817,#64818,#64819,#64820,
#64821,#64822,#64823,#64824,#64825,#64826,#64827,#64828,#64829,#64830,#64831,
#64832,#64833,#64834,#64835,#64836,#64837,#64838,#64839,#64840,#64841,#64842,
#64843,#64844,#64845,#64846,#64847,#64848,#64849,#64850,#64851,#64852,#64853,
#64854,#64855,#64856,#64857,#64858,#64859,#64860,#64861,#64862,#64863,#64864,
#64865,#64866,#64867,#64868,#64869,#64870,#64871,#64872,#64873,#64874),
 .UNSPECIFIED.,.F.,.F.)
B_SPLINE_CURVE_WITH_KNOTS((6,1,1,1,1,1,1,1,1,1,1,1,1,1,1,1,1,1,1,1,1,1,
1,1,1,1,1,1,1,1,1,1,1,1,1,1,1,1,1,1,1,1,1,1,1,1,1,1,1,1,1,1,1,1,1,1,1,1,
1,1,1,1,1,1,1,1,1,1,1,1,1,1,1,1,1,1,1,1,1,1,1,1,1,1,1,1,1,1,1,1,1,1,1,1,
1,1,1,1,1,1,1,1,1,1,1,1,1,1,1,1,1,1,1,1,1,1,1,1,1,1,1,1,1,1,1,1,1,1,1,1,
1,1,1,1,1,1,1,1,1,1,1,1,1,1,1,1,1,1,1,1,1,1,1,1,1,1,1,1,1,1,1,1,1,1,1,1,
1,1,1,1,1,1,1,1,1,1,1,1,1,1,1,1,1,1,1,1,1,1,1,6),(0.,0.005,0.01,0.015,0.02,
0.025,0.03,0.035,0.04,0.045,0.05,0.055,0.06,0.065,0.07,0.075,0.08,0.085,
0.09,0.095,0.1,0.105,0.11,0.115,0.12,0.125,0.13,0.135,0.14,0.145,0.15,0.155,
0.16,0.165,0.17,0.175,0.18,0.185,0.19,0.195,0.2,0.205,0.21,0.215,0.22,0.225,
0.23,0.235,0.24,0.245,0.25,0.255,0.26,0.265,0.27,0.275,0.28,0.285,0.29,
0.295,0.3,0.305,0.31,0.315,0.32,0.325,0.33,0.335,0.34,0.345,0.35,0.355,
0.36,0.365,0.37,0.375,0.38,0.385,0.39,0.395,0.4,0.405,0.41,0.415,0.42,0.425,
0.43,0.435,0.44,0.445,0.45,0.455,0.46,0.465,0.47,0.475,0.48,0.485,0.49,
0.495,0.5,0.505,0.51,0.515,0.52,0.525,0.53,0.535,0.54,0.545,0.55,0.555,
0.56,0.565,0.57,0.575,0.58,0.585,0.59,0.595,0.6,0.605,0.61,0.615,0.62,0.625,
0.63,0.635,0.64,0.645,0.65,0.655,0.66,0.665,0.67,0.675,0.68,0.685,0.690000000000001,
0.695000000000001,0.700000000000001,0.705000000000001,0.710000000000001,
0.715000000000001,0.720000000000001,0.725000000000001,0.730000000000001,
0.735000000000001,0.740000000000001,0.745000000000001,0.750000000000001,
0.755000000000001,0.760000000000001,0.765000000000001,0.770000000000001,
0.775000000000001,0.780000000000001,0.785000000000001,0.790000000000001,
0.795000000000001,0.800000000000001,0.805000000000001,0.810000000000001,
0.815000000000001,0.820000000000001,0.825000000000001,0.830000000000001,
0.835000000000001,0.840000000000001,0.845000000000001,0.850000000000001,
0.855000000000001,0.860000000000001,0.865000000000001,0.870000000000001,
0.875000000000001,0.880000000000001,0.885000000000001,0.890000000000001,
0.895000000000001,0.900000000000001,0.905000000000001,0.910000000000001,
0.915000000000001,0.920000000000001,0.925000000000001,0.930000000000001,
0.935000000000001,0.940000000000001,0.941429844431384),.UNSPECIFIED.)
CURVE()
GEOMETRIC_REPRESENTATION_ITEM()
RATIONAL_B_SPLINE_CURVE((1.,1.,1.,1.,1.,1.,1.,1.,1.,1.,1.,1.,1.,1.,1.,1.,
1.,1.,1.,1.,1.,1.,1.,1.,1.,1.,1.,1.,1.,1.,1.,1.,1.,1.,1.,1.,1.,1.,1.,1.,
1.,1.,1.,1.,1.,1.,1.,1.,1.,1.,1.,1.,1.,1.,1.,1.,1.,1.,1.,1.,1.,1.,1.,1.,
1.,1.,1.,1.,1.,1.,1.,1.,1.,1.,1.,1.,1.,1.,1.,1.,1.,1.,1.,1.,1.,1.,1.,1.,
1.,1.,1.,1.,1.,1.,1.,1.,1.,1.,1.,1.,1.,1.,1.,1.,1.,1.,1.,1.,1.,1.,1.,1.,
1.,1.,1.,1.,1.,1.,1.,1.,1.,1.,1.,1.,1.,1.,1.,1.,1.,1.,1.,1.,1.,1.,1.,1.,
1.,1.,1.,1.,1.,1.,1.,1.,1.,1.,1.,1.,1.,1.,1.,1.,1.,1.,1.,1.,1.,1.,1.,1.,
1.,1.,1.,1.,1.,1.,1.,1.,1.,1.,1.,1.,1.,1.,1.,1.,1.,1.,1.,1.,1.,1.,1.,1.,
1.,1.,1.,1.,1.,1.,1.,1.,1.,1.))
REPRESENTATION_ITEM('')
);
#430=(
BOUNDED_CURVE()
B_SPLINE_CURVE(5,(#64877,#64878,#64879,#64880,#64881,#64882,#64883,#64884,
#64885,#64886,#64887,#64888,#64889,#64890,#64891,#64892,#64893,#64894,#64895,
#64896,#64897,#64898,#64899,#64900,#64901,#64902,#64903,#64904,#64905,#64906,
#64907,#64908,#64909,#64910,#64911,#64912,#64913,#64914,#64915,#64916,#64917,
#64918,#64919,#64920,#64921,#64922,#64923,#64924,#64925,#64926,#64927,#64928,
#64929,#64930,#64931,#64932,#64933,#64934,#64935,#64936,#64937,#64938,#64939,
#64940,#64941,#64942,#64943,#64944,#64945,#64946,#64947,#64948,#64949,#64950,
#64951,#64952,#64953,#64954,#64955,#64956,#64957,#64958,#64959,#64960,#64961,
#64962,#64963,#64964,#64965,#64966,#64967,#64968,#64969,#64970,#64971,#64972,
#64973,#64974,#64975,#64976,#64977,#64978,#64979,#64980,#64981,#64982,#64983,
#64984,#64985,#64986,#64987,#64988,#64989,#64990,#64991,#64992,#64993,#64994,
#64995,#64996,#64997,#64998,#64999,#65000,#65001,#65002,#65003,#65004,#65005,
#65006,#65007,#65008,#65009,#65010,#65011,#65012,#65013,#65014,#65015,#65016,
#65017,#65018,#65019,#65020,#65021,#65022,#65023,#65024,#65025,#65026,#65027,
#65028,#65029,#65030,#65031,#65032,#65033,#65034,#65035,#65036,#65037,#65038,
#65039,#65040,#65041,#65042,#65043,#65044,#65045,#65046,#65047,#65048,#65049,
#65050,#65051,#65052,#65053,#65054,#65055,#65056,#65057,#65058,#65059,#65060,
#65061,#65062,#65063,#65064,#65065,#65066,#65067,#65068,#65069,#65070),
 .UNSPECIFIED.,.F.,.F.)
B_SPLINE_CURVE_WITH_KNOTS((6,1,1,1,1,1,1,1,1,1,1,1,1,1,1,1,1,1,1,1,1,1,
1,1,1,1,1,1,1,1,1,1,1,1,1,1,1,1,1,1,1,1,1,1,1,1,1,1,1,1,1,1,1,1,1,1,1,1,
1,1,1,1,1,1,1,1,1,1,1,1,1,1,1,1,1,1,1,1,1,1,1,1,1,1,1,1,1,1,1,1,1,1,1,1,
1,1,1,1,1,1,1,1,1,1,1,1,1,1,1,1,1,1,1,1,1,1,1,1,1,1,1,1,1,1,1,1,1,1,1,1,
1,1,1,1,1,1,1,1,1,1,1,1,1,1,1,1,1,1,1,1,1,1,1,1,1,1,1,1,1,1,1,1,1,1,1,1,
1,1,1,1,1,1,1,1,1,1,1,1,1,1,1,1,1,1,1,1,1,1,1,6),(-0.941429844431384,-0.940000000000001,
-0.935000000000001,-0.930000000000001,-0.925000000000001,-0.920000000000001,
-0.915000000000001,-0.910000000000001,-0.905000000000001,-0.900000000000001,
-0.895000000000001,-0.890000000000001,-0.885000000000001,-0.880000000000001,
-0.875000000000001,-0.870000000000001,-0.865000000000001,-0.860000000000001,
-0.855000000000001,-0.850000000000001,-0.845000000000001,-0.840000000000001,
-0.835000000000001,-0.830000000000001,-0.825000000000001,-0.820000000000001,
-0.815000000000001,-0.810000000000001,-0.805000000000001,-0.800000000000001,
-0.795000000000001,-0.790000000000001,-0.785000000000001,-0.780000000000001,
-0.775000000000001,-0.770000000000001,-0.765000000000001,-0.760000000000001,
-0.755000000000001,-0.750000000000001,-0.745000000000001,-0.740000000000001,
-0.735000000000001,-0.730000000000001,-0.725000000000001,-0.720000000000001,
-0.715000000000001,-0.710000000000001,-0.705000000000001,-0.700000000000001,
-0.695000000000001,-0.690000000000001,-0.685,-0.68,-0.675,-0.67,-0.665,
-0.66,-0.655,-0.65,-0.645,-0.64,-0.635,-0.63,-0.625,-0.62,-0.615,-0.61,
-0.605,-0.6,-0.595,-0.59,-0.585,-0.58,-0.575,-0.57,-0.565,-0.56,-0.555,
-0.55,-0.545,-0.54,-0.535,-0.53,-0.525,-0.52,-0.515,-0.51,-0.505,-0.5,-0.495,
-0.49,-0.485,-0.48,-0.475,-0.47,-0.465,-0.46,-0.455,-0.45,-0.445,-0.44,
-0.435,-0.43,-0.425,-0.42,-0.415,-0.41,-0.405,-0.4,-0.395,-0.39,-0.385,
-0.38,-0.375,-0.37,-0.365,-0.36,-0.355,-0.35,-0.345,-0.34,-0.335,-0.33,
-0.325,-0.32,-0.315,-0.31,-0.305,-0.3,-0.295,-0.29,-0.285,-0.28,-0.275,
-0.27,-0.265,-0.26,-0.255,-0.25,-0.245,-0.24,-0.235,-0.23,-0.225,-0.22,
-0.215,-0.21,-0.205,-0.2,-0.195,-0.19,-0.185,-0.18,-0.175,-0.17,-0.165,
-0.16,-0.155,-0.15,-0.145,-0.14,-0.135,-0.13,-0.125,-0.12,-0.115,-0.11,
-0.105,-0.1,-0.095,-0.09,-0.085,-0.08,-0.075,-0.07,-0.065,-0.06,-0.055,
-0.05,-0.045,-0.04,-0.035,-0.03,-0.025,-0.02,-0.015,-0.01,-0.005,0.),
 .UNSPECIFIED.)
CURVE()
GEOMETRIC_REPRESENTATION_ITEM()
RATIONAL_B_SPLINE_CURVE((1.,1.,1.,1.,1.,1.,1.,1.,1.,1.,1.,1.,1.,1.,1.,1.,
1.,1.,1.,1.,1.,1.,1.,1.,1.,1.,1.,1.,1.,1.,1.,1.,1.,1.,1.,1.,1.,1.,1.,1.,
1.,1.,1.,1.,1.,1.,1.,1.,1.,1.,1.,1.,1.,1.,1.,1.,1.,1.,1.,1.,1.,1.,1.,1.,
1.,1.,1.,1.,1.,1.,1.,1.,1.,1.,1.,1.,1.,1.,1.,1.,1.,1.,1.,1.,1.,1.,1.,1.,
1.,1.,1.,1.,1.,1.,1.,1.,1.,1.,1.,1.,1.,1.,1.,1.,1.,1.,1.,1.,1.,1.,1.,1.,
1.,1.,1.,1.,1.,1.,1.,1.,1.,1.,1.,1.,1.,1.,1.,1.,1.,1.,1.,1.,1.,1.,1.,1.,
1.,1.,1.,1.,1.,1.,1.,1.,1.,1.,1.,1.,1.,1.,1.,1.,1.,1.,1.,1.,1.,1.,1.,1.,
1.,1.,1.,1.,1.,1.,1.,1.,1.,1.,1.,1.,1.,1.,1.,1.,1.,1.,1.,1.,1.,1.,1.,1.,
1.,1.,1.,1.,1.,1.,1.,1.,1.,1.))
REPRESENTATION_ITEM('')
);
#431=(
BOUNDED_CURVE()
B_SPLINE_CURVE(5,(#65577,#65578,#65579,#65580,#65581,#65582,#65583,#65584,
#65585,#65586,#65587,#65588,#65589,#65590,#65591,#65592,#65593,#65594,#65595,
#65596,#65597,#65598,#65599,#65600,#65601,#65602,#65603,#65604,#65605,#65606,
#65607,#65608,#65609,#65610,#65611,#65612,#65613,#65614,#65615,#65616,#65617,
#65618,#65619,#65620,#65621,#65622,#65623,#65624,#65625,#65626,#65627,#65628,
#65629,#65630,#65631,#65632,#65633,#65634,#65635,#65636,#65637,#65638,#65639,
#65640,#65641,#65642,#65643,#65644,#65645,#65646,#65647,#65648,#65649,#65650,
#65651,#65652,#65653,#65654,#65655,#65656,#65657,#65658,#65659,#65660,#65661,
#65662,#65663,#65664,#65665,#65666,#65667,#65668,#65669,#65670,#65671,#65672,
#65673,#65674,#65675,#65676,#65677,#65678,#65679,#65680,#65681,#65682,#65683,
#65684,#65685,#65686,#65687,#65688,#65689,#65690,#65691,#65692,#65693,#65694,
#65695,#65696,#65697,#65698,#65699,#65700,#65701,#65702,#65703,#65704,#65705,
#65706,#65707,#65708,#65709,#65710,#65711,#65712,#65713,#65714,#65715,#65716,
#65717,#65718,#65719,#65720,#65721,#65722,#65723,#65724,#65725,#65726,#65727,
#65728,#65729,#65730,#65731,#65732,#65733,#65734,#65735,#65736,#65737,#65738,
#65739,#65740,#65741,#65742,#65743,#65744,#65745,#65746,#65747,#65748,#65749,
#65750,#65751,#65752,#65753,#65754,#65755,#65756,#65757,#65758,#65759,#65760,
#65761,#65762,#65763,#65764,#65765,#65766,#65767,#65768,#65769,#65770),
 .UNSPECIFIED.,.F.,.F.)
B_SPLINE_CURVE_WITH_KNOTS((6,1,1,1,1,1,1,1,1,1,1,1,1,1,1,1,1,1,1,1,1,1,
1,1,1,1,1,1,1,1,1,1,1,1,1,1,1,1,1,1,1,1,1,1,1,1,1,1,1,1,1,1,1,1,1,1,1,1,
1,1,1,1,1,1,1,1,1,1,1,1,1,1,1,1,1,1,1,1,1,1,1,1,1,1,1,1,1,1,1,1,1,1,1,1,
1,1,1,1,1,1,1,1,1,1,1,1,1,1,1,1,1,1,1,1,1,1,1,1,1,1,1,1,1,1,1,1,1,1,1,1,
1,1,1,1,1,1,1,1,1,1,1,1,1,1,1,1,1,1,1,1,1,1,1,1,1,1,1,1,1,1,1,1,1,1,1,1,
1,1,1,1,1,1,1,1,1,1,1,1,1,1,1,1,1,1,1,1,1,1,1,6),(0.,0.005,0.01,0.015,0.02,
0.025,0.03,0.035,0.04,0.045,0.05,0.055,0.06,0.065,0.07,0.075,0.08,0.085,
0.09,0.095,0.1,0.105,0.11,0.115,0.12,0.125,0.13,0.135,0.14,0.145,0.15,0.155,
0.16,0.165,0.17,0.175,0.18,0.185,0.19,0.195,0.2,0.205,0.21,0.215,0.22,0.225,
0.23,0.235,0.24,0.245,0.25,0.255,0.26,0.265,0.27,0.275,0.28,0.285,0.29,
0.295,0.3,0.305,0.31,0.315,0.32,0.325,0.33,0.335,0.34,0.345,0.35,0.355,
0.36,0.365,0.37,0.375,0.38,0.385,0.39,0.395,0.4,0.405,0.41,0.415,0.42,0.425,
0.43,0.435,0.44,0.445,0.45,0.455,0.46,0.465,0.47,0.475,0.48,0.485,0.49,
0.495,0.5,0.505,0.51,0.515,0.52,0.525,0.53,0.535,0.54,0.545,0.55,0.555,
0.56,0.565,0.57,0.575,0.58,0.585,0.59,0.595,0.6,0.605,0.61,0.615,0.62,0.625,
0.63,0.635,0.64,0.645,0.65,0.655,0.66,0.665,0.67,0.675,0.68,0.685,0.690000000000001,
0.695000000000001,0.700000000000001,0.705000000000001,0.710000000000001,
0.715000000000001,0.720000000000001,0.725000000000001,0.730000000000001,
0.735000000000001,0.740000000000001,0.745000000000001,0.750000000000001,
0.755000000000001,0.760000000000001,0.765000000000001,0.770000000000001,
0.775000000000001,0.780000000000001,0.785000000000001,0.790000000000001,
0.795000000000001,0.800000000000001,0.805000000000001,0.810000000000001,
0.815000000000001,0.820000000000001,0.825000000000001,0.830000000000001,
0.835000000000001,0.840000000000001,0.845000000000001,0.850000000000001,
0.855000000000001,0.860000000000001,0.865000000000001,0.870000000000001,
0.875000000000001,0.880000000000001,0.885000000000001,0.890000000000001,
0.895000000000001,0.900000000000001,0.905000000000001,0.910000000000001,
0.915000000000001,0.920000000000001,0.925000000000001,0.930000000000001,
0.935000000000001,0.940000000000001,0.941429844431397),.UNSPECIFIED.)
CURVE()
GEOMETRIC_REPRESENTATION_ITEM()
RATIONAL_B_SPLINE_CURVE((1.,1.,1.,1.,1.,1.,1.,1.,1.,1.,1.,1.,1.,1.,1.,1.,
1.,1.,1.,1.,1.,1.,1.,1.,1.,1.,1.,1.,1.,1.,1.,1.,1.,1.,1.,1.,1.,1.,1.,1.,
1.,1.,1.,1.,1.,1.,1.,1.,1.,1.,1.,1.,1.,1.,1.,1.,1.,1.,1.,1.,1.,1.,1.,1.,
1.,1.,1.,1.,1.,1.,1.,1.,1.,1.,1.,1.,1.,1.,1.,1.,1.,1.,1.,1.,1.,1.,1.,1.,
1.,1.,1.,1.,1.,1.,1.,1.,1.,1.,1.,1.,1.,1.,1.,1.,1.,1.,1.,1.,1.,1.,1.,1.,
1.,1.,1.,1.,1.,1.,1.,1.,1.,1.,1.,1.,1.,1.,1.,1.,1.,1.,1.,1.,1.,1.,1.,1.,
1.,1.,1.,1.,1.,1.,1.,1.,1.,1.,1.,1.,1.,1.,1.,1.,1.,1.,1.,1.,1.,1.,1.,1.,
1.,1.,1.,1.,1.,1.,1.,1.,1.,1.,1.,1.,1.,1.,1.,1.,1.,1.,1.,1.,1.,1.,1.,1.,
1.,1.,1.,1.,1.,1.,1.,1.,1.,1.))
REPRESENTATION_ITEM('')
);
#432=(
BOUNDED_CURVE()
B_SPLINE_CURVE(5,(#65773,#65774,#65775,#65776,#65777,#65778,#65779,#65780,
#65781,#65782,#65783,#65784,#65785,#65786,#65787,#65788,#65789,#65790,#65791,
#65792,#65793,#65794,#65795,#65796,#65797,#65798,#65799,#65800,#65801,#65802,
#65803,#65804,#65805,#65806,#65807,#65808,#65809,#65810,#65811,#65812,#65813,
#65814,#65815,#65816,#65817,#65818,#65819,#65820,#65821,#65822,#65823,#65824,
#65825,#65826,#65827,#65828,#65829,#65830,#65831,#65832,#65833,#65834,#65835,
#65836,#65837,#65838,#65839,#65840,#65841,#65842,#65843,#65844,#65845,#65846,
#65847,#65848,#65849,#65850,#65851,#65852,#65853,#65854,#65855,#65856,#65857,
#65858,#65859,#65860,#65861,#65862,#65863,#65864,#65865,#65866,#65867,#65868,
#65869,#65870,#65871,#65872,#65873,#65874,#65875,#65876,#65877,#65878,#65879,
#65880,#65881,#65882,#65883,#65884,#65885,#65886,#65887,#65888,#65889,#65890,
#65891,#65892,#65893,#65894,#65895,#65896,#65897,#65898,#65899,#65900,#65901,
#65902,#65903,#65904,#65905,#65906,#65907,#65908,#65909,#65910,#65911,#65912,
#65913,#65914,#65915,#65916,#65917,#65918,#65919,#65920,#65921,#65922,#65923,
#65924,#65925,#65926,#65927,#65928,#65929,#65930,#65931,#65932,#65933,#65934,
#65935,#65936,#65937,#65938,#65939,#65940,#65941,#65942,#65943,#65944,#65945,
#65946,#65947,#65948,#65949,#65950,#65951,#65952,#65953,#65954,#65955,#65956,
#65957,#65958,#65959,#65960,#65961,#65962,#65963,#65964,#65965,#65966),
 .UNSPECIFIED.,.F.,.F.)
B_SPLINE_CURVE_WITH_KNOTS((6,1,1,1,1,1,1,1,1,1,1,1,1,1,1,1,1,1,1,1,1,1,
1,1,1,1,1,1,1,1,1,1,1,1,1,1,1,1,1,1,1,1,1,1,1,1,1,1,1,1,1,1,1,1,1,1,1,1,
1,1,1,1,1,1,1,1,1,1,1,1,1,1,1,1,1,1,1,1,1,1,1,1,1,1,1,1,1,1,1,1,1,1,1,1,
1,1,1,1,1,1,1,1,1,1,1,1,1,1,1,1,1,1,1,1,1,1,1,1,1,1,1,1,1,1,1,1,1,1,1,1,
1,1,1,1,1,1,1,1,1,1,1,1,1,1,1,1,1,1,1,1,1,1,1,1,1,1,1,1,1,1,1,1,1,1,1,1,
1,1,1,1,1,1,1,1,1,1,1,1,1,1,1,1,1,1,1,1,1,1,1,6),(-0.941429844431399,-0.940000000000001,
-0.935000000000001,-0.930000000000001,-0.925000000000001,-0.920000000000001,
-0.915000000000001,-0.910000000000001,-0.905000000000001,-0.900000000000001,
-0.895000000000001,-0.890000000000001,-0.885000000000001,-0.880000000000001,
-0.875000000000001,-0.870000000000001,-0.865000000000001,-0.860000000000001,
-0.855000000000001,-0.850000000000001,-0.845000000000001,-0.840000000000001,
-0.835000000000001,-0.830000000000001,-0.825000000000001,-0.820000000000001,
-0.815000000000001,-0.810000000000001,-0.805000000000001,-0.800000000000001,
-0.795000000000001,-0.790000000000001,-0.785000000000001,-0.780000000000001,
-0.775000000000001,-0.770000000000001,-0.765000000000001,-0.760000000000001,
-0.755000000000001,-0.750000000000001,-0.745000000000001,-0.740000000000001,
-0.735000000000001,-0.730000000000001,-0.725000000000001,-0.720000000000001,
-0.715000000000001,-0.710000000000001,-0.705000000000001,-0.700000000000001,
-0.695000000000001,-0.690000000000001,-0.685,-0.68,-0.675,-0.67,-0.665,
-0.66,-0.655,-0.65,-0.645,-0.64,-0.635,-0.63,-0.625,-0.62,-0.615,-0.61,
-0.605,-0.6,-0.595,-0.59,-0.585,-0.58,-0.575,-0.57,-0.565,-0.56,-0.555,
-0.55,-0.545,-0.54,-0.535,-0.53,-0.525,-0.52,-0.515,-0.51,-0.505,-0.5,-0.495,
-0.49,-0.485,-0.48,-0.475,-0.47,-0.465,-0.46,-0.455,-0.45,-0.445,-0.44,
-0.435,-0.43,-0.425,-0.42,-0.415,-0.41,-0.405,-0.4,-0.395,-0.39,-0.385,
-0.38,-0.375,-0.37,-0.365,-0.36,-0.355,-0.35,-0.345,-0.34,-0.335,-0.33,
-0.325,-0.32,-0.315,-0.31,-0.305,-0.3,-0.295,-0.29,-0.285,-0.28,-0.275,
-0.27,-0.265,-0.26,-0.255,-0.25,-0.245,-0.24,-0.235,-0.23,-0.225,-0.22,
-0.215,-0.21,-0.205,-0.2,-0.195,-0.19,-0.185,-0.18,-0.175,-0.17,-0.165,
-0.16,-0.155,-0.15,-0.145,-0.14,-0.135,-0.13,-0.125,-0.12,-0.115,-0.11,
-0.105,-0.1,-0.095,-0.09,-0.085,-0.08,-0.075,-0.07,-0.065,-0.06,-0.055,
-0.05,-0.045,-0.04,-0.035,-0.03,-0.025,-0.02,-0.015,-0.01,-0.005,0.),
 .UNSPECIFIED.)
CURVE()
GEOMETRIC_REPRESENTATION_ITEM()
RATIONAL_B_SPLINE_CURVE((1.,1.,1.,1.,1.,1.,1.,1.,1.,1.,1.,1.,1.,1.,1.,1.,
1.,1.,1.,1.,1.,1.,1.,1.,1.,1.,1.,1.,1.,1.,1.,1.,1.,1.,1.,1.,1.,1.,1.,1.,
1.,1.,1.,1.,1.,1.,1.,1.,1.,1.,1.,1.,1.,1.,1.,1.,1.,1.,1.,1.,1.,1.,1.,1.,
1.,1.,1.,1.,1.,1.,1.,1.,1.,1.,1.,1.,1.,1.,1.,1.,1.,1.,1.,1.,1.,1.,1.,1.,
1.,1.,1.,1.,1.,1.,1.,1.,1.,1.,1.,1.,1.,1.,1.,1.,1.,1.,1.,1.,1.,1.,1.,1.,
1.,1.,1.,1.,1.,1.,1.,1.,1.,1.,1.,1.,1.,1.,1.,1.,1.,1.,1.,1.,1.,1.,1.,1.,
1.,1.,1.,1.,1.,1.,1.,1.,1.,1.,1.,1.,1.,1.,1.,1.,1.,1.,1.,1.,1.,1.,1.,1.,
1.,1.,1.,1.,1.,1.,1.,1.,1.,1.,1.,1.,1.,1.,1.,1.,1.,1.,1.,1.,1.,1.,1.,1.,
1.,1.,1.,1.,1.,1.,1.,1.,1.,1.))
REPRESENTATION_ITEM('')
);
#433=(
BOUNDED_CURVE()
B_SPLINE_CURVE(5,(#66473,#66474,#66475,#66476,#66477,#66478,#66479,#66480,
#66481,#66482,#66483,#66484,#66485,#66486,#66487,#66488,#66489,#66490,#66491,
#66492,#66493,#66494,#66495,#66496,#66497,#66498,#66499,#66500,#66501,#66502,
#66503,#66504,#66505,#66506,#66507,#66508,#66509,#66510,#66511,#66512,#66513,
#66514,#66515,#66516,#66517,#66518,#66519,#66520,#66521,#66522,#66523,#66524,
#66525,#66526,#66527,#66528,#66529,#66530,#66531,#66532,#66533,#66534,#66535,
#66536,#66537,#66538,#66539,#66540,#66541,#66542,#66543,#66544,#66545,#66546,
#66547,#66548,#66549,#66550,#66551,#66552,#66553,#66554,#66555,#66556,#66557,
#66558,#66559,#66560,#66561,#66562,#66563,#66564,#66565,#66566,#66567,#66568,
#66569,#66570,#66571,#66572,#66573,#66574,#66575,#66576,#66577,#66578,#66579,
#66580,#66581,#66582,#66583,#66584,#66585,#66586,#66587,#66588,#66589,#66590,
#66591,#66592,#66593,#66594,#66595,#66596,#66597,#66598,#66599,#66600,#66601,
#66602,#66603,#66604,#66605,#66606,#66607,#66608,#66609,#66610,#66611,#66612,
#66613,#66614,#66615,#66616,#66617,#66618,#66619,#66620,#66621,#66622,#66623,
#66624,#66625,#66626,#66627,#66628,#66629,#66630,#66631,#66632,#66633,#66634,
#66635,#66636,#66637,#66638,#66639,#66640,#66641,#66642,#66643,#66644,#66645,
#66646,#66647,#66648,#66649,#66650,#66651,#66652,#66653,#66654,#66655,#66656,
#66657,#66658,#66659,#66660,#66661,#66662,#66663,#66664,#66665,#66666),
 .UNSPECIFIED.,.F.,.F.)
B_SPLINE_CURVE_WITH_KNOTS((6,1,1,1,1,1,1,1,1,1,1,1,1,1,1,1,1,1,1,1,1,1,
1,1,1,1,1,1,1,1,1,1,1,1,1,1,1,1,1,1,1,1,1,1,1,1,1,1,1,1,1,1,1,1,1,1,1,1,
1,1,1,1,1,1,1,1,1,1,1,1,1,1,1,1,1,1,1,1,1,1,1,1,1,1,1,1,1,1,1,1,1,1,1,1,
1,1,1,1,1,1,1,1,1,1,1,1,1,1,1,1,1,1,1,1,1,1,1,1,1,1,1,1,1,1,1,1,1,1,1,1,
1,1,1,1,1,1,1,1,1,1,1,1,1,1,1,1,1,1,1,1,1,1,1,1,1,1,1,1,1,1,1,1,1,1,1,1,
1,1,1,1,1,1,1,1,1,1,1,1,1,1,1,1,1,1,1,1,1,1,1,6),(0.,0.005,0.01,0.015,0.02,
0.025,0.03,0.035,0.04,0.045,0.05,0.055,0.06,0.065,0.07,0.075,0.08,0.085,
0.09,0.095,0.1,0.105,0.11,0.115,0.12,0.125,0.13,0.135,0.14,0.145,0.15,0.155,
0.16,0.165,0.17,0.175,0.18,0.185,0.19,0.195,0.2,0.205,0.21,0.215,0.22,0.225,
0.23,0.235,0.24,0.245,0.25,0.255,0.26,0.265,0.27,0.275,0.28,0.285,0.29,
0.295,0.3,0.305,0.31,0.315,0.32,0.325,0.33,0.335,0.34,0.345,0.35,0.355,
0.36,0.365,0.37,0.375,0.38,0.385,0.39,0.395,0.4,0.405,0.41,0.415,0.42,0.425,
0.43,0.435,0.44,0.445,0.45,0.455,0.46,0.465,0.47,0.475,0.48,0.485,0.49,
0.495,0.5,0.505,0.51,0.515,0.52,0.525,0.53,0.535,0.54,0.545,0.55,0.555,
0.56,0.565,0.57,0.575,0.58,0.585,0.59,0.595,0.6,0.605,0.61,0.615,0.62,0.625,
0.63,0.635,0.64,0.645,0.65,0.655,0.66,0.665,0.67,0.675,0.68,0.685,0.690000000000001,
0.695000000000001,0.700000000000001,0.705000000000001,0.710000000000001,
0.715000000000001,0.720000000000001,0.725000000000001,0.730000000000001,
0.735000000000001,0.740000000000001,0.745000000000001,0.750000000000001,
0.755000000000001,0.760000000000001,0.765000000000001,0.770000000000001,
0.775000000000001,0.780000000000001,0.785000000000001,0.790000000000001,
0.795000000000001,0.800000000000001,0.805000000000001,0.810000000000001,
0.815000000000001,0.820000000000001,0.825000000000001,0.830000000000001,
0.835000000000001,0.840000000000001,0.845000000000001,0.850000000000001,
0.855000000000001,0.860000000000001,0.865000000000001,0.870000000000001,
0.875000000000001,0.880000000000001,0.885000000000001,0.890000000000001,
0.895000000000001,0.900000000000001,0.905000000000001,0.910000000000001,
0.915000000000001,0.920000000000001,0.925000000000001,0.930000000000001,
0.935000000000001,0.940000000000001,0.941429844431383),.UNSPECIFIED.)
CURVE()
GEOMETRIC_REPRESENTATION_ITEM()
RATIONAL_B_SPLINE_CURVE((1.,1.,1.,1.,1.,1.,1.,1.,1.,1.,1.,1.,1.,1.,1.,1.,
1.,1.,1.,1.,1.,1.,1.,1.,1.,1.,1.,1.,1.,1.,1.,1.,1.,1.,1.,1.,1.,1.,1.,1.,
1.,1.,1.,1.,1.,1.,1.,1.,1.,1.,1.,1.,1.,1.,1.,1.,1.,1.,1.,1.,1.,1.,1.,1.,
1.,1.,1.,1.,1.,1.,1.,1.,1.,1.,1.,1.,1.,1.,1.,1.,1.,1.,1.,1.,1.,1.,1.,1.,
1.,1.,1.,1.,1.,1.,1.,1.,1.,1.,1.,1.,1.,1.,1.,1.,1.,1.,1.,1.,1.,1.,1.,1.,
1.,1.,1.,1.,1.,1.,1.,1.,1.,1.,1.,1.,1.,1.,1.,1.,1.,1.,1.,1.,1.,1.,1.,1.,
1.,1.,1.,1.,1.,1.,1.,1.,1.,1.,1.,1.,1.,1.,1.,1.,1.,1.,1.,1.,1.,1.,1.,1.,
1.,1.,1.,1.,1.,1.,1.,1.,1.,1.,1.,1.,1.,1.,1.,1.,1.,1.,1.,1.,1.,1.,1.,1.,
1.,1.,1.,1.,1.,1.,1.,1.,1.,1.))
REPRESENTATION_ITEM('')
);
#434=(
BOUNDED_CURVE()
B_SPLINE_CURVE(5,(#66669,#66670,#66671,#66672,#66673,#66674,#66675,#66676,
#66677,#66678,#66679,#66680,#66681,#66682,#66683,#66684,#66685,#66686,#66687,
#66688,#66689,#66690,#66691,#66692,#66693,#66694,#66695,#66696,#66697,#66698,
#66699,#66700,#66701,#66702,#66703,#66704,#66705,#66706,#66707,#66708,#66709,
#66710,#66711,#66712,#66713,#66714,#66715,#66716,#66717,#66718,#66719,#66720,
#66721,#66722,#66723,#66724,#66725,#66726,#66727,#66728,#66729,#66730,#66731,
#66732,#66733,#66734,#66735,#66736,#66737,#66738,#66739,#66740,#66741,#66742,
#66743,#66744,#66745,#66746,#66747,#66748,#66749,#66750,#66751,#66752,#66753,
#66754,#66755,#66756,#66757,#66758,#66759,#66760,#66761,#66762,#66763,#66764,
#66765,#66766,#66767,#66768,#66769,#66770,#66771,#66772,#66773,#66774,#66775,
#66776,#66777,#66778,#66779,#66780,#66781,#66782,#66783,#66784,#66785,#66786,
#66787,#66788,#66789,#66790,#66791,#66792,#66793,#66794,#66795,#66796,#66797,
#66798,#66799,#66800,#66801,#66802,#66803,#66804,#66805,#66806,#66807,#66808,
#66809,#66810,#66811,#66812,#66813,#66814,#66815,#66816,#66817,#66818,#66819,
#66820,#66821,#66822,#66823,#66824,#66825,#66826,#66827,#66828,#66829,#66830,
#66831,#66832,#66833,#66834,#66835,#66836,#66837,#66838,#66839,#66840,#66841,
#66842,#66843,#66844,#66845,#66846,#66847,#66848,#66849,#66850,#66851,#66852,
#66853,#66854,#66855,#66856,#66857,#66858,#66859,#66860,#66861,#66862),
 .UNSPECIFIED.,.F.,.F.)
B_SPLINE_CURVE_WITH_KNOTS((6,1,1,1,1,1,1,1,1,1,1,1,1,1,1,1,1,1,1,1,1,1,
1,1,1,1,1,1,1,1,1,1,1,1,1,1,1,1,1,1,1,1,1,1,1,1,1,1,1,1,1,1,1,1,1,1,1,1,
1,1,1,1,1,1,1,1,1,1,1,1,1,1,1,1,1,1,1,1,1,1,1,1,1,1,1,1,1,1,1,1,1,1,1,1,
1,1,1,1,1,1,1,1,1,1,1,1,1,1,1,1,1,1,1,1,1,1,1,1,1,1,1,1,1,1,1,1,1,1,1,1,
1,1,1,1,1,1,1,1,1,1,1,1,1,1,1,1,1,1,1,1,1,1,1,1,1,1,1,1,1,1,1,1,1,1,1,1,
1,1,1,1,1,1,1,1,1,1,1,1,1,1,1,1,1,1,1,1,1,1,1,6),(-0.941429844431371,-0.940000000000001,
-0.935000000000001,-0.930000000000001,-0.925000000000001,-0.920000000000001,
-0.915000000000001,-0.910000000000001,-0.905000000000001,-0.900000000000001,
-0.895000000000001,-0.890000000000001,-0.885000000000001,-0.880000000000001,
-0.875000000000001,-0.870000000000001,-0.865000000000001,-0.860000000000001,
-0.855000000000001,-0.850000000000001,-0.845000000000001,-0.840000000000001,
-0.835000000000001,-0.830000000000001,-0.825000000000001,-0.820000000000001,
-0.815000000000001,-0.810000000000001,-0.805000000000001,-0.800000000000001,
-0.795000000000001,-0.790000000000001,-0.785000000000001,-0.780000000000001,
-0.775000000000001,-0.770000000000001,-0.765000000000001,-0.760000000000001,
-0.755000000000001,-0.750000000000001,-0.745000000000001,-0.740000000000001,
-0.735000000000001,-0.730000000000001,-0.725000000000001,-0.720000000000001,
-0.715000000000001,-0.710000000000001,-0.705000000000001,-0.700000000000001,
-0.695000000000001,-0.690000000000001,-0.685,-0.68,-0.675,-0.67,-0.665,
-0.66,-0.655,-0.65,-0.645,-0.64,-0.635,-0.63,-0.625,-0.62,-0.615,-0.61,
-0.605,-0.6,-0.595,-0.59,-0.585,-0.58,-0.575,-0.57,-0.565,-0.56,-0.555,
-0.55,-0.545,-0.54,-0.535,-0.53,-0.525,-0.52,-0.515,-0.51,-0.505,-0.5,-0.495,
-0.49,-0.485,-0.48,-0.475,-0.47,-0.465,-0.46,-0.455,-0.45,-0.445,-0.44,
-0.435,-0.43,-0.425,-0.42,-0.415,-0.41,-0.405,-0.4,-0.395,-0.39,-0.385,
-0.38,-0.375,-0.37,-0.365,-0.36,-0.355,-0.35,-0.345,-0.34,-0.335,-0.33,
-0.325,-0.32,-0.315,-0.31,-0.305,-0.3,-0.295,-0.29,-0.285,-0.28,-0.275,
-0.27,-0.265,-0.26,-0.255,-0.25,-0.245,-0.24,-0.235,-0.23,-0.225,-0.22,
-0.215,-0.21,-0.205,-0.2,-0.195,-0.19,-0.185,-0.18,-0.175,-0.17,-0.165,
-0.16,-0.155,-0.15,-0.145,-0.14,-0.135,-0.13,-0.125,-0.12,-0.115,-0.11,
-0.105,-0.1,-0.095,-0.09,-0.085,-0.08,-0.075,-0.07,-0.065,-0.06,-0.055,
-0.05,-0.045,-0.04,-0.035,-0.03,-0.025,-0.02,-0.015,-0.01,-0.005,0.),
 .UNSPECIFIED.)
CURVE()
GEOMETRIC_REPRESENTATION_ITEM()
RATIONAL_B_SPLINE_CURVE((1.,1.,1.,1.,1.,1.,1.,1.,1.,1.,1.,1.,1.,1.,1.,1.,
1.,1.,1.,1.,1.,1.,1.,1.,1.,1.,1.,1.,1.,1.,1.,1.,1.,1.,1.,1.,1.,1.,1.,1.,
1.,1.,1.,1.,1.,1.,1.,1.,1.,1.,1.,1.,1.,1.,1.,1.,1.,1.,1.,1.,1.,1.,1.,1.,
1.,1.,1.,1.,1.,1.,1.,1.,1.,1.,1.,1.,1.,1.,1.,1.,1.,1.,1.,1.,1.,1.,1.,1.,
1.,1.,1.,1.,1.,1.,1.,1.,1.,1.,1.,1.,1.,1.,1.,1.,1.,1.,1.,1.,1.,1.,1.,1.,
1.,1.,1.,1.,1.,1.,1.,1.,1.,1.,1.,1.,1.,1.,1.,1.,1.,1.,1.,1.,1.,1.,1.,1.,
1.,1.,1.,1.,1.,1.,1.,1.,1.,1.,1.,1.,1.,1.,1.,1.,1.,1.,1.,1.,1.,1.,1.,1.,
1.,1.,1.,1.,1.,1.,1.,1.,1.,1.,1.,1.,1.,1.,1.,1.,1.,1.,1.,1.,1.,1.,1.,1.,
1.,1.,1.,1.,1.,1.,1.,1.,1.,1.))
REPRESENTATION_ITEM('')
);
#435=(
BOUNDED_CURVE()
B_SPLINE_CURVE(5,(#67369,#67370,#67371,#67372,#67373,#67374,#67375,#67376,
#67377,#67378,#67379,#67380,#67381,#67382,#67383,#67384,#67385,#67386,#67387,
#67388,#67389,#67390,#67391,#67392,#67393,#67394,#67395,#67396,#67397,#67398,
#67399,#67400,#67401,#67402,#67403,#67404,#67405,#67406,#67407,#67408,#67409,
#67410,#67411,#67412,#67413,#67414,#67415,#67416,#67417,#67418,#67419,#67420,
#67421,#67422,#67423,#67424,#67425,#67426,#67427,#67428,#67429,#67430,#67431,
#67432,#67433,#67434,#67435,#67436,#67437,#67438,#67439,#67440,#67441,#67442,
#67443,#67444,#67445,#67446,#67447,#67448,#67449,#67450,#67451,#67452,#67453,
#67454,#67455,#67456,#67457,#67458,#67459,#67460,#67461,#67462,#67463,#67464,
#67465,#67466,#67467,#67468,#67469,#67470,#67471,#67472,#67473,#67474,#67475,
#67476,#67477,#67478,#67479,#67480,#67481,#67482,#67483,#67484,#67485,#67486,
#67487,#67488,#67489,#67490,#67491,#67492,#67493,#67494,#67495,#67496,#67497,
#67498,#67499,#67500,#67501,#67502,#67503,#67504,#67505,#67506,#67507,#67508,
#67509,#67510,#67511,#67512,#67513,#67514,#67515,#67516,#67517,#67518,#67519,
#67520,#67521,#67522,#67523,#67524,#67525,#67526,#67527,#67528,#67529,#67530,
#67531,#67532,#67533,#67534,#67535,#67536,#67537,#67538,#67539,#67540,#67541,
#67542,#67543,#67544,#67545,#67546,#67547,#67548,#67549,#67550,#67551,#67552,
#67553,#67554,#67555,#67556,#67557,#67558,#67559,#67560,#67561,#67562),
 .UNSPECIFIED.,.F.,.F.)
B_SPLINE_CURVE_WITH_KNOTS((6,1,1,1,1,1,1,1,1,1,1,1,1,1,1,1,1,1,1,1,1,1,
1,1,1,1,1,1,1,1,1,1,1,1,1,1,1,1,1,1,1,1,1,1,1,1,1,1,1,1,1,1,1,1,1,1,1,1,
1,1,1,1,1,1,1,1,1,1,1,1,1,1,1,1,1,1,1,1,1,1,1,1,1,1,1,1,1,1,1,1,1,1,1,1,
1,1,1,1,1,1,1,1,1,1,1,1,1,1,1,1,1,1,1,1,1,1,1,1,1,1,1,1,1,1,1,1,1,1,1,1,
1,1,1,1,1,1,1,1,1,1,1,1,1,1,1,1,1,1,1,1,1,1,1,1,1,1,1,1,1,1,1,1,1,1,1,1,
1,1,1,1,1,1,1,1,1,1,1,1,1,1,1,1,1,1,1,1,1,1,1,6),(0.,0.005,0.01,0.015,0.02,
0.025,0.03,0.035,0.04,0.045,0.05,0.055,0.06,0.065,0.07,0.075,0.08,0.085,
0.09,0.095,0.1,0.105,0.11,0.115,0.12,0.125,0.13,0.135,0.14,0.145,0.15,0.155,
0.16,0.165,0.17,0.175,0.18,0.185,0.19,0.195,0.2,0.205,0.21,0.215,0.22,0.225,
0.23,0.235,0.24,0.245,0.25,0.255,0.26,0.265,0.27,0.275,0.28,0.285,0.29,
0.295,0.3,0.305,0.31,0.315,0.32,0.325,0.33,0.335,0.34,0.345,0.35,0.355,
0.36,0.365,0.37,0.375,0.38,0.385,0.39,0.395,0.4,0.405,0.41,0.415,0.42,0.425,
0.43,0.435,0.44,0.445,0.45,0.455,0.46,0.465,0.47,0.475,0.48,0.485,0.49,
0.495,0.5,0.505,0.51,0.515,0.52,0.525,0.53,0.535,0.54,0.545,0.55,0.555,
0.56,0.565,0.57,0.575,0.58,0.585,0.59,0.595,0.6,0.605,0.61,0.615,0.62,0.625,
0.63,0.635,0.64,0.645,0.65,0.655,0.66,0.665,0.67,0.675,0.68,0.685,0.690000000000001,
0.695000000000001,0.700000000000001,0.705000000000001,0.710000000000001,
0.715000000000001,0.720000000000001,0.725000000000001,0.730000000000001,
0.735000000000001,0.740000000000001,0.745000000000001,0.750000000000001,
0.755000000000001,0.760000000000001,0.765000000000001,0.770000000000001,
0.775000000000001,0.780000000000001,0.785000000000001,0.790000000000001,
0.795000000000001,0.800000000000001,0.805000000000001,0.810000000000001,
0.815000000000001,0.820000000000001,0.825000000000001,0.830000000000001,
0.835000000000001,0.840000000000001,0.845000000000001,0.850000000000001,
0.855000000000001,0.860000000000001,0.865000000000001,0.870000000000001,
0.875000000000001,0.880000000000001,0.885000000000001,0.890000000000001,
0.895000000000001,0.900000000000001,0.905000000000001,0.910000000000001,
0.915000000000001,0.920000000000001,0.925000000000001,0.930000000000001,
0.935000000000001,0.940000000000001,0.941429844431383),.UNSPECIFIED.)
CURVE()
GEOMETRIC_REPRESENTATION_ITEM()
RATIONAL_B_SPLINE_CURVE((1.,1.,1.,1.,1.,1.,1.,1.,1.,1.,1.,1.,1.,1.,1.,1.,
1.,1.,1.,1.,1.,1.,1.,1.,1.,1.,1.,1.,1.,1.,1.,1.,1.,1.,1.,1.,1.,1.,1.,1.,
1.,1.,1.,1.,1.,1.,1.,1.,1.,1.,1.,1.,1.,1.,1.,1.,1.,1.,1.,1.,1.,1.,1.,1.,
1.,1.,1.,1.,1.,1.,1.,1.,1.,1.,1.,1.,1.,1.,1.,1.,1.,1.,1.,1.,1.,1.,1.,1.,
1.,1.,1.,1.,1.,1.,1.,1.,1.,1.,1.,1.,1.,1.,1.,1.,1.,1.,1.,1.,1.,1.,1.,1.,
1.,1.,1.,1.,1.,1.,1.,1.,1.,1.,1.,1.,1.,1.,1.,1.,1.,1.,1.,1.,1.,1.,1.,1.,
1.,1.,1.,1.,1.,1.,1.,1.,1.,1.,1.,1.,1.,1.,1.,1.,1.,1.,1.,1.,1.,1.,1.,1.,
1.,1.,1.,1.,1.,1.,1.,1.,1.,1.,1.,1.,1.,1.,1.,1.,1.,1.,1.,1.,1.,1.,1.,1.,
1.,1.,1.,1.,1.,1.,1.,1.,1.,1.))
REPRESENTATION_ITEM('')
);
#436=(
BOUNDED_CURVE()
B_SPLINE_CURVE(5,(#67565,#67566,#67567,#67568,#67569,#67570,#67571,#67572,
#67573,#67574,#67575,#67576,#67577,#67578,#67579,#67580,#67581,#67582,#67583,
#67584,#67585,#67586,#67587,#67588,#67589,#67590,#67591,#67592,#67593,#67594,
#67595,#67596,#67597,#67598,#67599,#67600,#67601,#67602,#67603,#67604,#67605,
#67606,#67607,#67608,#67609,#67610,#67611,#67612,#67613,#67614,#67615,#67616,
#67617,#67618,#67619,#67620,#67621,#67622,#67623,#67624,#67625,#67626,#67627,
#67628,#67629,#67630,#67631,#67632,#67633,#67634,#67635,#67636,#67637,#67638,
#67639,#67640,#67641,#67642,#67643,#67644,#67645,#67646,#67647,#67648,#67649,
#67650,#67651,#67652,#67653,#67654,#67655,#67656,#67657,#67658,#67659,#67660,
#67661,#67662,#67663,#67664,#67665,#67666,#67667,#67668,#67669,#67670,#67671,
#67672,#67673,#67674,#67675,#67676,#67677,#67678,#67679,#67680,#67681,#67682,
#67683,#67684,#67685,#67686,#67687,#67688,#67689,#67690,#67691,#67692,#67693,
#67694,#67695,#67696,#67697,#67698,#67699,#67700,#67701,#67702,#67703,#67704,
#67705,#67706,#67707,#67708,#67709,#67710,#67711,#67712,#67713,#67714,#67715,
#67716,#67717,#67718,#67719,#67720,#67721,#67722,#67723,#67724,#67725,#67726,
#67727,#67728,#67729,#67730,#67731,#67732,#67733,#67734,#67735,#67736,#67737,
#67738,#67739,#67740,#67741,#67742,#67743,#67744,#67745,#67746,#67747,#67748,
#67749,#67750,#67751,#67752,#67753,#67754,#67755,#67756,#67757,#67758),
 .UNSPECIFIED.,.F.,.F.)
B_SPLINE_CURVE_WITH_KNOTS((6,1,1,1,1,1,1,1,1,1,1,1,1,1,1,1,1,1,1,1,1,1,
1,1,1,1,1,1,1,1,1,1,1,1,1,1,1,1,1,1,1,1,1,1,1,1,1,1,1,1,1,1,1,1,1,1,1,1,
1,1,1,1,1,1,1,1,1,1,1,1,1,1,1,1,1,1,1,1,1,1,1,1,1,1,1,1,1,1,1,1,1,1,1,1,
1,1,1,1,1,1,1,1,1,1,1,1,1,1,1,1,1,1,1,1,1,1,1,1,1,1,1,1,1,1,1,1,1,1,1,1,
1,1,1,1,1,1,1,1,1,1,1,1,1,1,1,1,1,1,1,1,1,1,1,1,1,1,1,1,1,1,1,1,1,1,1,1,
1,1,1,1,1,1,1,1,1,1,1,1,1,1,1,1,1,1,1,1,1,1,1,6),(-0.941429844431383,-0.940000000000001,
-0.935000000000001,-0.930000000000001,-0.925000000000001,-0.920000000000001,
-0.915000000000001,-0.910000000000001,-0.905000000000001,-0.900000000000001,
-0.895000000000001,-0.890000000000001,-0.885000000000001,-0.880000000000001,
-0.875000000000001,-0.870000000000001,-0.865000000000001,-0.860000000000001,
-0.855000000000001,-0.850000000000001,-0.845000000000001,-0.840000000000001,
-0.835000000000001,-0.830000000000001,-0.825000000000001,-0.820000000000001,
-0.815000000000001,-0.810000000000001,-0.805000000000001,-0.800000000000001,
-0.795000000000001,-0.790000000000001,-0.785000000000001,-0.780000000000001,
-0.775000000000001,-0.770000000000001,-0.765000000000001,-0.760000000000001,
-0.755000000000001,-0.750000000000001,-0.745000000000001,-0.740000000000001,
-0.735000000000001,-0.730000000000001,-0.725000000000001,-0.720000000000001,
-0.715000000000001,-0.710000000000001,-0.705000000000001,-0.700000000000001,
-0.695000000000001,-0.690000000000001,-0.685,-0.68,-0.675,-0.67,-0.665,
-0.66,-0.655,-0.65,-0.645,-0.64,-0.635,-0.63,-0.625,-0.62,-0.615,-0.61,
-0.605,-0.6,-0.595,-0.59,-0.585,-0.58,-0.575,-0.57,-0.565,-0.56,-0.555,
-0.55,-0.545,-0.54,-0.535,-0.53,-0.525,-0.52,-0.515,-0.51,-0.505,-0.5,-0.495,
-0.49,-0.485,-0.48,-0.475,-0.47,-0.465,-0.46,-0.455,-0.45,-0.445,-0.44,
-0.435,-0.43,-0.425,-0.42,-0.415,-0.41,-0.405,-0.4,-0.395,-0.39,-0.385,
-0.38,-0.375,-0.37,-0.365,-0.36,-0.355,-0.35,-0.345,-0.34,-0.335,-0.33,
-0.325,-0.32,-0.315,-0.31,-0.305,-0.3,-0.295,-0.29,-0.285,-0.28,-0.275,
-0.27,-0.265,-0.26,-0.255,-0.25,-0.245,-0.24,-0.235,-0.23,-0.225,-0.22,
-0.215,-0.21,-0.205,-0.2,-0.195,-0.19,-0.185,-0.18,-0.175,-0.17,-0.165,
-0.16,-0.155,-0.15,-0.145,-0.14,-0.135,-0.13,-0.125,-0.12,-0.115,-0.11,
-0.105,-0.1,-0.095,-0.09,-0.085,-0.08,-0.075,-0.07,-0.065,-0.06,-0.055,
-0.05,-0.045,-0.04,-0.035,-0.03,-0.025,-0.02,-0.015,-0.01,-0.005,0.),
 .UNSPECIFIED.)
CURVE()
GEOMETRIC_REPRESENTATION_ITEM()
RATIONAL_B_SPLINE_CURVE((1.,1.,1.,1.,1.,1.,1.,1.,1.,1.,1.,1.,1.,1.,1.,1.,
1.,1.,1.,1.,1.,1.,1.,1.,1.,1.,1.,1.,1.,1.,1.,1.,1.,1.,1.,1.,1.,1.,1.,1.,
1.,1.,1.,1.,1.,1.,1.,1.,1.,1.,1.,1.,1.,1.,1.,1.,1.,1.,1.,1.,1.,1.,1.,1.,
1.,1.,1.,1.,1.,1.,1.,1.,1.,1.,1.,1.,1.,1.,1.,1.,1.,1.,1.,1.,1.,1.,1.,1.,
1.,1.,1.,1.,1.,1.,1.,1.,1.,1.,1.,1.,1.,1.,1.,1.,1.,1.,1.,1.,1.,1.,1.,1.,
1.,1.,1.,1.,1.,1.,1.,1.,1.,1.,1.,1.,1.,1.,1.,1.,1.,1.,1.,1.,1.,1.,1.,1.,
1.,1.,1.,1.,1.,1.,1.,1.,1.,1.,1.,1.,1.,1.,1.,1.,1.,1.,1.,1.,1.,1.,1.,1.,
1.,1.,1.,1.,1.,1.,1.,1.,1.,1.,1.,1.,1.,1.,1.,1.,1.,1.,1.,1.,1.,1.,1.,1.,
1.,1.,1.,1.,1.,1.,1.,1.,1.,1.))
REPRESENTATION_ITEM('')
);
#437=(
BOUNDED_CURVE()
B_SPLINE_CURVE(5,(#68265,#68266,#68267,#68268,#68269,#68270,#68271,#68272,
#68273,#68274,#68275,#68276,#68277,#68278,#68279,#68280,#68281,#68282,#68283,
#68284,#68285,#68286,#68287,#68288,#68289,#68290,#68291,#68292,#68293,#68294,
#68295,#68296,#68297,#68298,#68299,#68300,#68301,#68302,#68303,#68304,#68305,
#68306,#68307,#68308,#68309,#68310,#68311,#68312,#68313,#68314,#68315,#68316,
#68317,#68318,#68319,#68320,#68321,#68322,#68323,#68324,#68325,#68326,#68327,
#68328,#68329,#68330,#68331,#68332,#68333,#68334,#68335,#68336,#68337,#68338,
#68339,#68340,#68341,#68342,#68343,#68344,#68345,#68346,#68347,#68348,#68349,
#68350,#68351,#68352,#68353,#68354,#68355,#68356,#68357,#68358,#68359,#68360,
#68361,#68362,#68363,#68364,#68365,#68366,#68367,#68368,#68369,#68370,#68371,
#68372,#68373,#68374,#68375,#68376,#68377,#68378,#68379,#68380,#68381,#68382,
#68383,#68384,#68385,#68386,#68387,#68388,#68389,#68390,#68391,#68392,#68393,
#68394,#68395,#68396,#68397,#68398,#68399,#68400,#68401,#68402,#68403,#68404,
#68405,#68406,#68407,#68408,#68409,#68410,#68411,#68412,#68413,#68414,#68415,
#68416,#68417,#68418,#68419,#68420,#68421,#68422,#68423,#68424,#68425,#68426,
#68427,#68428,#68429,#68430,#68431,#68432,#68433,#68434,#68435,#68436,#68437,
#68438,#68439,#68440,#68441,#68442,#68443,#68444,#68445,#68446,#68447,#68448,
#68449,#68450,#68451,#68452,#68453,#68454,#68455,#68456,#68457,#68458),
 .UNSPECIFIED.,.F.,.F.)
B_SPLINE_CURVE_WITH_KNOTS((6,1,1,1,1,1,1,1,1,1,1,1,1,1,1,1,1,1,1,1,1,1,
1,1,1,1,1,1,1,1,1,1,1,1,1,1,1,1,1,1,1,1,1,1,1,1,1,1,1,1,1,1,1,1,1,1,1,1,
1,1,1,1,1,1,1,1,1,1,1,1,1,1,1,1,1,1,1,1,1,1,1,1,1,1,1,1,1,1,1,1,1,1,1,1,
1,1,1,1,1,1,1,1,1,1,1,1,1,1,1,1,1,1,1,1,1,1,1,1,1,1,1,1,1,1,1,1,1,1,1,1,
1,1,1,1,1,1,1,1,1,1,1,1,1,1,1,1,1,1,1,1,1,1,1,1,1,1,1,1,1,1,1,1,1,1,1,1,
1,1,1,1,1,1,1,1,1,1,1,1,1,1,1,1,1,1,1,1,1,1,1,6),(0.,0.005,0.01,0.015,0.02,
0.025,0.03,0.035,0.04,0.045,0.05,0.055,0.06,0.065,0.07,0.075,0.08,0.085,
0.09,0.095,0.1,0.105,0.11,0.115,0.12,0.125,0.13,0.135,0.14,0.145,0.15,0.155,
0.16,0.165,0.17,0.175,0.18,0.185,0.19,0.195,0.2,0.205,0.21,0.215,0.22,0.225,
0.23,0.235,0.24,0.245,0.25,0.255,0.26,0.265,0.27,0.275,0.28,0.285,0.29,
0.295,0.3,0.305,0.31,0.315,0.32,0.325,0.33,0.335,0.34,0.345,0.35,0.355,
0.36,0.365,0.37,0.375,0.38,0.385,0.39,0.395,0.4,0.405,0.41,0.415,0.42,0.425,
0.43,0.435,0.44,0.445,0.45,0.455,0.46,0.465,0.47,0.475,0.48,0.485,0.49,
0.495,0.5,0.505,0.51,0.515,0.52,0.525,0.53,0.535,0.54,0.545,0.55,0.555,
0.56,0.565,0.57,0.575,0.58,0.585,0.59,0.595,0.6,0.605,0.61,0.615,0.62,0.625,
0.63,0.635,0.64,0.645,0.65,0.655,0.66,0.665,0.67,0.675,0.68,0.685,0.690000000000001,
0.695000000000001,0.700000000000001,0.705000000000001,0.710000000000001,
0.715000000000001,0.720000000000001,0.725000000000001,0.730000000000001,
0.735000000000001,0.740000000000001,0.745000000000001,0.750000000000001,
0.755000000000001,0.760000000000001,0.765000000000001,0.770000000000001,
0.775000000000001,0.780000000000001,0.785000000000001,0.790000000000001,
0.795000000000001,0.800000000000001,0.805000000000001,0.810000000000001,
0.815000000000001,0.820000000000001,0.825000000000001,0.830000000000001,
0.835000000000001,0.840000000000001,0.845000000000001,0.850000000000001,
0.855000000000001,0.860000000000001,0.865000000000001,0.870000000000001,
0.875000000000001,0.880000000000001,0.885000000000001,0.890000000000001,
0.895000000000001,0.900000000000001,0.905000000000001,0.910000000000001,
0.915000000000001,0.920000000000001,0.925000000000001,0.930000000000001,
0.935000000000001,0.940000000000001,0.941429844431453),.UNSPECIFIED.)
CURVE()
GEOMETRIC_REPRESENTATION_ITEM()
RATIONAL_B_SPLINE_CURVE((1.,1.,1.,1.,1.,1.,1.,1.,1.,1.,1.,1.,1.,1.,1.,1.,
1.,1.,1.,1.,1.,1.,1.,1.,1.,1.,1.,1.,1.,1.,1.,1.,1.,1.,1.,1.,1.,1.,1.,1.,
1.,1.,1.,1.,1.,1.,1.,1.,1.,1.,1.,1.,1.,1.,1.,1.,1.,1.,1.,1.,1.,1.,1.,1.,
1.,1.,1.,1.,1.,1.,1.,1.,1.,1.,1.,1.,1.,1.,1.,1.,1.,1.,1.,1.,1.,1.,1.,1.,
1.,1.,1.,1.,1.,1.,1.,1.,1.,1.,1.,1.,1.,1.,1.,1.,1.,1.,1.,1.,1.,1.,1.,1.,
1.,1.,1.,1.,1.,1.,1.,1.,1.,1.,1.,1.,1.,1.,1.,1.,1.,1.,1.,1.,1.,1.,1.,1.,
1.,1.,1.,1.,1.,1.,1.,1.,1.,1.,1.,1.,1.,1.,1.,1.,1.,1.,1.,1.,1.,1.,1.,1.,
1.,1.,1.,1.,1.,1.,1.,1.,1.,1.,1.,1.,1.,1.,1.,1.,1.,1.,1.,1.,1.,1.,1.,1.,
1.,1.,1.,1.,1.,1.,1.,1.,1.,1.))
REPRESENTATION_ITEM('')
);
#438=(
BOUNDED_CURVE()
B_SPLINE_CURVE(5,(#68461,#68462,#68463,#68464,#68465,#68466,#68467,#68468,
#68469,#68470,#68471,#68472,#68473,#68474,#68475,#68476,#68477,#68478,#68479,
#68480,#68481,#68482,#68483,#68484,#68485,#68486,#68487,#68488,#68489,#68490,
#68491,#68492,#68493,#68494,#68495,#68496,#68497,#68498,#68499,#68500,#68501,
#68502,#68503,#68504,#68505,#68506,#68507,#68508,#68509,#68510,#68511,#68512,
#68513,#68514,#68515,#68516,#68517,#68518,#68519,#68520,#68521,#68522,#68523,
#68524,#68525,#68526,#68527,#68528,#68529,#68530,#68531,#68532,#68533,#68534,
#68535,#68536,#68537,#68538,#68539,#68540,#68541,#68542,#68543,#68544,#68545,
#68546,#68547,#68548,#68549,#68550,#68551,#68552,#68553,#68554,#68555,#68556,
#68557,#68558,#68559,#68560,#68561,#68562,#68563,#68564,#68565,#68566,#68567,
#68568,#68569,#68570,#68571,#68572,#68573,#68574,#68575,#68576,#68577,#68578,
#68579,#68580,#68581,#68582,#68583,#68584,#68585,#68586,#68587,#68588,#68589,
#68590,#68591,#68592,#68593,#68594,#68595,#68596,#68597,#68598,#68599,#68600,
#68601,#68602,#68603,#68604,#68605,#68606,#68607,#68608,#68609,#68610,#68611,
#68612,#68613,#68614,#68615,#68616,#68617,#68618,#68619,#68620,#68621,#68622,
#68623,#68624,#68625,#68626,#68627,#68628,#68629,#68630,#68631,#68632,#68633,
#68634,#68635,#68636,#68637,#68638,#68639,#68640,#68641,#68642,#68643,#68644,
#68645,#68646,#68647,#68648,#68649,#68650,#68651,#68652,#68653,#68654),
 .UNSPECIFIED.,.F.,.F.)
B_SPLINE_CURVE_WITH_KNOTS((6,1,1,1,1,1,1,1,1,1,1,1,1,1,1,1,1,1,1,1,1,1,
1,1,1,1,1,1,1,1,1,1,1,1,1,1,1,1,1,1,1,1,1,1,1,1,1,1,1,1,1,1,1,1,1,1,1,1,
1,1,1,1,1,1,1,1,1,1,1,1,1,1,1,1,1,1,1,1,1,1,1,1,1,1,1,1,1,1,1,1,1,1,1,1,
1,1,1,1,1,1,1,1,1,1,1,1,1,1,1,1,1,1,1,1,1,1,1,1,1,1,1,1,1,1,1,1,1,1,1,1,
1,1,1,1,1,1,1,1,1,1,1,1,1,1,1,1,1,1,1,1,1,1,1,1,1,1,1,1,1,1,1,1,1,1,1,1,
1,1,1,1,1,1,1,1,1,1,1,1,1,1,1,1,1,1,1,1,1,1,1,6),(-0.941429844431454,-0.940000000000001,
-0.935000000000001,-0.930000000000001,-0.925000000000001,-0.920000000000001,
-0.915000000000001,-0.910000000000001,-0.905000000000001,-0.900000000000001,
-0.895000000000001,-0.890000000000001,-0.885000000000001,-0.880000000000001,
-0.875000000000001,-0.870000000000001,-0.865000000000001,-0.860000000000001,
-0.855000000000001,-0.850000000000001,-0.845000000000001,-0.840000000000001,
-0.835000000000001,-0.830000000000001,-0.825000000000001,-0.820000000000001,
-0.815000000000001,-0.810000000000001,-0.805000000000001,-0.800000000000001,
-0.795000000000001,-0.790000000000001,-0.785000000000001,-0.780000000000001,
-0.775000000000001,-0.770000000000001,-0.765000000000001,-0.760000000000001,
-0.755000000000001,-0.750000000000001,-0.745000000000001,-0.740000000000001,
-0.735000000000001,-0.730000000000001,-0.725000000000001,-0.720000000000001,
-0.715000000000001,-0.710000000000001,-0.705000000000001,-0.700000000000001,
-0.695000000000001,-0.690000000000001,-0.685,-0.68,-0.675,-0.67,-0.665,
-0.66,-0.655,-0.65,-0.645,-0.64,-0.635,-0.63,-0.625,-0.62,-0.615,-0.61,
-0.605,-0.6,-0.595,-0.59,-0.585,-0.58,-0.575,-0.57,-0.565,-0.56,-0.555,
-0.55,-0.545,-0.54,-0.535,-0.53,-0.525,-0.52,-0.515,-0.51,-0.505,-0.5,-0.495,
-0.49,-0.485,-0.48,-0.475,-0.47,-0.465,-0.46,-0.455,-0.45,-0.445,-0.44,
-0.435,-0.43,-0.425,-0.42,-0.415,-0.41,-0.405,-0.4,-0.395,-0.39,-0.385,
-0.38,-0.375,-0.37,-0.365,-0.36,-0.355,-0.35,-0.345,-0.34,-0.335,-0.33,
-0.325,-0.32,-0.315,-0.31,-0.305,-0.3,-0.295,-0.29,-0.285,-0.28,-0.275,
-0.27,-0.265,-0.26,-0.255,-0.25,-0.245,-0.24,-0.235,-0.23,-0.225,-0.22,
-0.215,-0.21,-0.205,-0.2,-0.195,-0.19,-0.185,-0.18,-0.175,-0.17,-0.165,
-0.16,-0.155,-0.15,-0.145,-0.14,-0.135,-0.13,-0.125,-0.12,-0.115,-0.11,
-0.105,-0.1,-0.095,-0.09,-0.085,-0.08,-0.075,-0.07,-0.065,-0.06,-0.055,
-0.05,-0.045,-0.04,-0.035,-0.03,-0.025,-0.02,-0.015,-0.01,-0.005,0.),
 .UNSPECIFIED.)
CURVE()
GEOMETRIC_REPRESENTATION_ITEM()
RATIONAL_B_SPLINE_CURVE((1.,1.,1.,1.,1.,1.,1.,1.,1.,1.,1.,1.,1.,1.,1.,1.,
1.,1.,1.,1.,1.,1.,1.,1.,1.,1.,1.,1.,1.,1.,1.,1.,1.,1.,1.,1.,1.,1.,1.,1.,
1.,1.,1.,1.,1.,1.,1.,1.,1.,1.,1.,1.,1.,1.,1.,1.,1.,1.,1.,1.,1.,1.,1.,1.,
1.,1.,1.,1.,1.,1.,1.,1.,1.,1.,1.,1.,1.,1.,1.,1.,1.,1.,1.,1.,1.,1.,1.,1.,
1.,1.,1.,1.,1.,1.,1.,1.,1.,1.,1.,1.,1.,1.,1.,1.,1.,1.,1.,1.,1.,1.,1.,1.,
1.,1.,1.,1.,1.,1.,1.,1.,1.,1.,1.,1.,1.,1.,1.,1.,1.,1.,1.,1.,1.,1.,1.,1.,
1.,1.,1.,1.,1.,1.,1.,1.,1.,1.,1.,1.,1.,1.,1.,1.,1.,1.,1.,1.,1.,1.,1.,1.,
1.,1.,1.,1.,1.,1.,1.,1.,1.,1.,1.,1.,1.,1.,1.,1.,1.,1.,1.,1.,1.,1.,1.,1.,
1.,1.,1.,1.,1.,1.,1.,1.,1.,1.))
REPRESENTATION_ITEM('')
);
#439=(
BOUNDED_CURVE()
B_SPLINE_CURVE(5,(#69161,#69162,#69163,#69164,#69165,#69166,#69167,#69168,
#69169,#69170,#69171,#69172,#69173,#69174,#69175,#69176,#69177,#69178,#69179,
#69180,#69181,#69182,#69183,#69184,#69185,#69186,#69187,#69188,#69189,#69190,
#69191,#69192,#69193,#69194,#69195,#69196,#69197,#69198,#69199,#69200,#69201,
#69202,#69203,#69204,#69205,#69206,#69207,#69208,#69209,#69210,#69211,#69212,
#69213,#69214,#69215,#69216,#69217,#69218,#69219,#69220,#69221,#69222,#69223,
#69224,#69225,#69226,#69227,#69228,#69229,#69230,#69231,#69232,#69233,#69234,
#69235,#69236,#69237,#69238,#69239,#69240,#69241,#69242,#69243,#69244,#69245,
#69246,#69247,#69248,#69249,#69250,#69251,#69252,#69253,#69254,#69255,#69256,
#69257,#69258,#69259,#69260,#69261,#69262,#69263,#69264,#69265,#69266,#69267,
#69268,#69269,#69270,#69271,#69272,#69273,#69274,#69275,#69276,#69277,#69278,
#69279,#69280,#69281,#69282,#69283,#69284,#69285,#69286,#69287,#69288,#69289,
#69290,#69291,#69292,#69293,#69294,#69295,#69296,#69297,#69298,#69299,#69300,
#69301,#69302,#69303,#69304,#69305,#69306,#69307,#69308,#69309,#69310,#69311,
#69312,#69313,#69314,#69315,#69316,#69317,#69318,#69319,#69320,#69321,#69322,
#69323,#69324,#69325,#69326,#69327,#69328,#69329,#69330,#69331,#69332,#69333,
#69334,#69335,#69336,#69337,#69338,#69339,#69340,#69341,#69342,#69343,#69344,
#69345,#69346,#69347,#69348,#69349,#69350,#69351,#69352,#69353,#69354),
 .UNSPECIFIED.,.F.,.F.)
B_SPLINE_CURVE_WITH_KNOTS((6,1,1,1,1,1,1,1,1,1,1,1,1,1,1,1,1,1,1,1,1,1,
1,1,1,1,1,1,1,1,1,1,1,1,1,1,1,1,1,1,1,1,1,1,1,1,1,1,1,1,1,1,1,1,1,1,1,1,
1,1,1,1,1,1,1,1,1,1,1,1,1,1,1,1,1,1,1,1,1,1,1,1,1,1,1,1,1,1,1,1,1,1,1,1,
1,1,1,1,1,1,1,1,1,1,1,1,1,1,1,1,1,1,1,1,1,1,1,1,1,1,1,1,1,1,1,1,1,1,1,1,
1,1,1,1,1,1,1,1,1,1,1,1,1,1,1,1,1,1,1,1,1,1,1,1,1,1,1,1,1,1,1,1,1,1,1,1,
1,1,1,1,1,1,1,1,1,1,1,1,1,1,1,1,1,1,1,1,1,1,1,6),(0.,0.005,0.01,0.015,0.02,
0.025,0.03,0.035,0.04,0.045,0.05,0.055,0.06,0.065,0.07,0.075,0.08,0.085,
0.09,0.095,0.1,0.105,0.11,0.115,0.12,0.125,0.13,0.135,0.14,0.145,0.15,0.155,
0.16,0.165,0.17,0.175,0.18,0.185,0.19,0.195,0.2,0.205,0.21,0.215,0.22,0.225,
0.23,0.235,0.24,0.245,0.25,0.255,0.26,0.265,0.27,0.275,0.28,0.285,0.29,
0.295,0.3,0.305,0.31,0.315,0.32,0.325,0.33,0.335,0.34,0.345,0.35,0.355,
0.36,0.365,0.37,0.375,0.38,0.385,0.39,0.395,0.4,0.405,0.41,0.415,0.42,0.425,
0.43,0.435,0.44,0.445,0.45,0.455,0.46,0.465,0.47,0.475,0.48,0.485,0.49,
0.495,0.5,0.505,0.51,0.515,0.52,0.525,0.53,0.535,0.54,0.545,0.55,0.555,
0.56,0.565,0.57,0.575,0.58,0.585,0.59,0.595,0.6,0.605,0.61,0.615,0.62,0.625,
0.63,0.635,0.64,0.645,0.65,0.655,0.66,0.665,0.67,0.675,0.68,0.685,0.690000000000001,
0.695000000000001,0.700000000000001,0.705000000000001,0.710000000000001,
0.715000000000001,0.720000000000001,0.725000000000001,0.730000000000001,
0.735000000000001,0.740000000000001,0.745000000000001,0.750000000000001,
0.755000000000001,0.760000000000001,0.765000000000001,0.770000000000001,
0.775000000000001,0.780000000000001,0.785000000000001,0.790000000000001,
0.795000000000001,0.800000000000001,0.805000000000001,0.810000000000001,
0.815000000000001,0.820000000000001,0.825000000000001,0.830000000000001,
0.835000000000001,0.840000000000001,0.845000000000001,0.850000000000001,
0.855000000000001,0.860000000000001,0.865000000000001,0.870000000000001,
0.875000000000001,0.880000000000001,0.885000000000001,0.890000000000001,
0.895000000000001,0.900000000000001,0.905000000000001,0.910000000000001,
0.915000000000001,0.920000000000001,0.925000000000001,0.930000000000001,
0.935000000000001,0.940000000000001,0.941429844431382),.UNSPECIFIED.)
CURVE()
GEOMETRIC_REPRESENTATION_ITEM()
RATIONAL_B_SPLINE_CURVE((1.,1.,1.,1.,1.,1.,1.,1.,1.,1.,1.,1.,1.,1.,1.,1.,
1.,1.,1.,1.,1.,1.,1.,1.,1.,1.,1.,1.,1.,1.,1.,1.,1.,1.,1.,1.,1.,1.,1.,1.,
1.,1.,1.,1.,1.,1.,1.,1.,1.,1.,1.,1.,1.,1.,1.,1.,1.,1.,1.,1.,1.,1.,1.,1.,
1.,1.,1.,1.,1.,1.,1.,1.,1.,1.,1.,1.,1.,1.,1.,1.,1.,1.,1.,1.,1.,1.,1.,1.,
1.,1.,1.,1.,1.,1.,1.,1.,1.,1.,1.,1.,1.,1.,1.,1.,1.,1.,1.,1.,1.,1.,1.,1.,
1.,1.,1.,1.,1.,1.,1.,1.,1.,1.,1.,1.,1.,1.,1.,1.,1.,1.,1.,1.,1.,1.,1.,1.,
1.,1.,1.,1.,1.,1.,1.,1.,1.,1.,1.,1.,1.,1.,1.,1.,1.,1.,1.,1.,1.,1.,1.,1.,
1.,1.,1.,1.,1.,1.,1.,1.,1.,1.,1.,1.,1.,1.,1.,1.,1.,1.,1.,1.,1.,1.,1.,1.,
1.,1.,1.,1.,1.,1.,1.,1.,1.,1.))
REPRESENTATION_ITEM('')
);
#440=(
BOUNDED_CURVE()
B_SPLINE_CURVE(5,(#69357,#69358,#69359,#69360,#69361,#69362,#69363,#69364,
#69365,#69366,#69367,#69368,#69369,#69370,#69371,#69372,#69373,#69374,#69375,
#69376,#69377,#69378,#69379,#69380,#69381,#69382,#69383,#69384,#69385,#69386,
#69387,#69388,#69389,#69390,#69391,#69392,#69393,#69394,#69395,#69396,#69397,
#69398,#69399,#69400,#69401,#69402,#69403,#69404,#69405,#69406,#69407,#69408,
#69409,#69410,#69411,#69412,#69413,#69414,#69415,#69416,#69417,#69418,#69419,
#69420,#69421,#69422,#69423,#69424,#69425,#69426,#69427,#69428,#69429,#69430,
#69431,#69432,#69433,#69434,#69435,#69436,#69437,#69438,#69439,#69440,#69441,
#69442,#69443,#69444,#69445,#69446,#69447,#69448,#69449,#69450,#69451,#69452,
#69453,#69454,#69455,#69456,#69457,#69458,#69459,#69460,#69461,#69462,#69463,
#69464,#69465,#69466,#69467,#69468,#69469,#69470,#69471,#69472,#69473,#69474,
#69475,#69476,#69477,#69478,#69479,#69480,#69481,#69482,#69483,#69484,#69485,
#69486,#69487,#69488,#69489,#69490,#69491,#69492,#69493,#69494,#69495,#69496,
#69497,#69498,#69499,#69500,#69501,#69502,#69503,#69504,#69505,#69506,#69507,
#69508,#69509,#69510,#69511,#69512,#69513,#69514,#69515,#69516,#69517,#69518,
#69519,#69520,#69521,#69522,#69523,#69524,#69525,#69526,#69527,#69528,#69529,
#69530,#69531,#69532,#69533,#69534,#69535,#69536,#69537,#69538,#69539,#69540,
#69541,#69542,#69543,#69544,#69545,#69546,#69547,#69548,#69549,#69550),
 .UNSPECIFIED.,.F.,.F.)
B_SPLINE_CURVE_WITH_KNOTS((6,1,1,1,1,1,1,1,1,1,1,1,1,1,1,1,1,1,1,1,1,1,
1,1,1,1,1,1,1,1,1,1,1,1,1,1,1,1,1,1,1,1,1,1,1,1,1,1,1,1,1,1,1,1,1,1,1,1,
1,1,1,1,1,1,1,1,1,1,1,1,1,1,1,1,1,1,1,1,1,1,1,1,1,1,1,1,1,1,1,1,1,1,1,1,
1,1,1,1,1,1,1,1,1,1,1,1,1,1,1,1,1,1,1,1,1,1,1,1,1,1,1,1,1,1,1,1,1,1,1,1,
1,1,1,1,1,1,1,1,1,1,1,1,1,1,1,1,1,1,1,1,1,1,1,1,1,1,1,1,1,1,1,1,1,1,1,1,
1,1,1,1,1,1,1,1,1,1,1,1,1,1,1,1,1,1,1,1,1,1,1,6),(-0.941429844431382,-0.940000000000001,
-0.935000000000001,-0.930000000000001,-0.925000000000001,-0.920000000000001,
-0.915000000000001,-0.910000000000001,-0.905000000000001,-0.900000000000001,
-0.895000000000001,-0.890000000000001,-0.885000000000001,-0.880000000000001,
-0.875000000000001,-0.870000000000001,-0.865000000000001,-0.860000000000001,
-0.855000000000001,-0.850000000000001,-0.845000000000001,-0.840000000000001,
-0.835000000000001,-0.830000000000001,-0.825000000000001,-0.820000000000001,
-0.815000000000001,-0.810000000000001,-0.805000000000001,-0.800000000000001,
-0.795000000000001,-0.790000000000001,-0.785000000000001,-0.780000000000001,
-0.775000000000001,-0.770000000000001,-0.765000000000001,-0.760000000000001,
-0.755000000000001,-0.750000000000001,-0.745000000000001,-0.740000000000001,
-0.735000000000001,-0.730000000000001,-0.725000000000001,-0.720000000000001,
-0.715000000000001,-0.710000000000001,-0.705000000000001,-0.700000000000001,
-0.695000000000001,-0.690000000000001,-0.685,-0.68,-0.675,-0.67,-0.665,
-0.66,-0.655,-0.65,-0.645,-0.64,-0.635,-0.63,-0.625,-0.62,-0.615,-0.61,
-0.605,-0.6,-0.595,-0.59,-0.585,-0.58,-0.575,-0.57,-0.565,-0.56,-0.555,
-0.55,-0.545,-0.54,-0.535,-0.53,-0.525,-0.52,-0.515,-0.51,-0.505,-0.5,-0.495,
-0.49,-0.485,-0.48,-0.475,-0.47,-0.465,-0.46,-0.455,-0.45,-0.445,-0.44,
-0.435,-0.43,-0.425,-0.42,-0.415,-0.41,-0.405,-0.4,-0.395,-0.39,-0.385,
-0.38,-0.375,-0.37,-0.365,-0.36,-0.355,-0.35,-0.345,-0.34,-0.335,-0.33,
-0.325,-0.32,-0.315,-0.31,-0.305,-0.3,-0.295,-0.29,-0.285,-0.28,-0.275,
-0.27,-0.265,-0.26,-0.255,-0.25,-0.245,-0.24,-0.235,-0.23,-0.225,-0.22,
-0.215,-0.21,-0.205,-0.2,-0.195,-0.19,-0.185,-0.18,-0.175,-0.17,-0.165,
-0.16,-0.155,-0.15,-0.145,-0.14,-0.135,-0.13,-0.125,-0.12,-0.115,-0.11,
-0.105,-0.1,-0.095,-0.09,-0.085,-0.08,-0.075,-0.07,-0.065,-0.06,-0.055,
-0.05,-0.045,-0.04,-0.035,-0.03,-0.025,-0.02,-0.015,-0.01,-0.005,0.),
 .UNSPECIFIED.)
CURVE()
GEOMETRIC_REPRESENTATION_ITEM()
RATIONAL_B_SPLINE_CURVE((1.,1.,1.,1.,1.,1.,1.,1.,1.,1.,1.,1.,1.,1.,1.,1.,
1.,1.,1.,1.,1.,1.,1.,1.,1.,1.,1.,1.,1.,1.,1.,1.,1.,1.,1.,1.,1.,1.,1.,1.,
1.,1.,1.,1.,1.,1.,1.,1.,1.,1.,1.,1.,1.,1.,1.,1.,1.,1.,1.,1.,1.,1.,1.,1.,
1.,1.,1.,1.,1.,1.,1.,1.,1.,1.,1.,1.,1.,1.,1.,1.,1.,1.,1.,1.,1.,1.,1.,1.,
1.,1.,1.,1.,1.,1.,1.,1.,1.,1.,1.,1.,1.,1.,1.,1.,1.,1.,1.,1.,1.,1.,1.,1.,
1.,1.,1.,1.,1.,1.,1.,1.,1.,1.,1.,1.,1.,1.,1.,1.,1.,1.,1.,1.,1.,1.,1.,1.,
1.,1.,1.,1.,1.,1.,1.,1.,1.,1.,1.,1.,1.,1.,1.,1.,1.,1.,1.,1.,1.,1.,1.,1.,
1.,1.,1.,1.,1.,1.,1.,1.,1.,1.,1.,1.,1.,1.,1.,1.,1.,1.,1.,1.,1.,1.,1.,1.,
1.,1.,1.,1.,1.,1.,1.,1.,1.,1.))
REPRESENTATION_ITEM('')
);
#441=(
BOUNDED_CURVE()
B_SPLINE_CURVE(5,(#70057,#70058,#70059,#70060,#70061,#70062,#70063,#70064,
#70065,#70066,#70067,#70068,#70069,#70070,#70071,#70072,#70073,#70074,#70075,
#70076,#70077,#70078,#70079,#70080,#70081,#70082,#70083,#70084,#70085,#70086,
#70087,#70088,#70089,#70090,#70091,#70092,#70093,#70094,#70095,#70096,#70097,
#70098,#70099,#70100,#70101,#70102,#70103,#70104,#70105,#70106,#70107,#70108,
#70109,#70110,#70111,#70112,#70113,#70114,#70115,#70116,#70117,#70118,#70119,
#70120,#70121,#70122,#70123,#70124,#70125,#70126,#70127,#70128,#70129,#70130,
#70131,#70132,#70133,#70134,#70135,#70136,#70137,#70138,#70139,#70140,#70141,
#70142,#70143,#70144,#70145,#70146,#70147,#70148,#70149,#70150,#70151,#70152,
#70153,#70154,#70155,#70156,#70157,#70158,#70159,#70160,#70161,#70162,#70163,
#70164,#70165,#70166,#70167,#70168,#70169,#70170,#70171,#70172,#70173,#70174,
#70175,#70176,#70177,#70178,#70179,#70180,#70181,#70182,#70183,#70184,#70185,
#70186,#70187,#70188,#70189,#70190,#70191,#70192,#70193,#70194,#70195,#70196,
#70197,#70198,#70199,#70200,#70201,#70202,#70203,#70204,#70205,#70206,#70207,
#70208,#70209,#70210,#70211,#70212,#70213,#70214,#70215,#70216,#70217,#70218,
#70219,#70220,#70221,#70222,#70223,#70224,#70225,#70226,#70227,#70228,#70229,
#70230,#70231,#70232,#70233,#70234,#70235,#70236,#70237,#70238,#70239,#70240,
#70241,#70242,#70243,#70244,#70245,#70246,#70247,#70248,#70249,#70250),
 .UNSPECIFIED.,.F.,.F.)
B_SPLINE_CURVE_WITH_KNOTS((6,1,1,1,1,1,1,1,1,1,1,1,1,1,1,1,1,1,1,1,1,1,
1,1,1,1,1,1,1,1,1,1,1,1,1,1,1,1,1,1,1,1,1,1,1,1,1,1,1,1,1,1,1,1,1,1,1,1,
1,1,1,1,1,1,1,1,1,1,1,1,1,1,1,1,1,1,1,1,1,1,1,1,1,1,1,1,1,1,1,1,1,1,1,1,
1,1,1,1,1,1,1,1,1,1,1,1,1,1,1,1,1,1,1,1,1,1,1,1,1,1,1,1,1,1,1,1,1,1,1,1,
1,1,1,1,1,1,1,1,1,1,1,1,1,1,1,1,1,1,1,1,1,1,1,1,1,1,1,1,1,1,1,1,1,1,1,1,
1,1,1,1,1,1,1,1,1,1,1,1,1,1,1,1,1,1,1,1,1,1,1,6),(0.,0.005,0.01,0.015,0.02,
0.025,0.03,0.035,0.04,0.045,0.05,0.055,0.06,0.065,0.07,0.075,0.08,0.085,
0.09,0.095,0.1,0.105,0.11,0.115,0.12,0.125,0.13,0.135,0.14,0.145,0.15,0.155,
0.16,0.165,0.17,0.175,0.18,0.185,0.19,0.195,0.2,0.205,0.21,0.215,0.22,0.225,
0.23,0.235,0.24,0.245,0.25,0.255,0.26,0.265,0.27,0.275,0.28,0.285,0.29,
0.295,0.3,0.305,0.31,0.315,0.32,0.325,0.33,0.335,0.34,0.345,0.35,0.355,
0.36,0.365,0.37,0.375,0.38,0.385,0.39,0.395,0.4,0.405,0.41,0.415,0.42,0.425,
0.43,0.435,0.44,0.445,0.45,0.455,0.46,0.465,0.47,0.475,0.48,0.485,0.49,
0.495,0.5,0.505,0.51,0.515,0.52,0.525,0.53,0.535,0.54,0.545,0.55,0.555,
0.56,0.565,0.57,0.575,0.58,0.585,0.59,0.595,0.6,0.605,0.61,0.615,0.62,0.625,
0.63,0.635,0.64,0.645,0.65,0.655,0.66,0.665,0.67,0.675,0.68,0.685,0.690000000000001,
0.695000000000001,0.700000000000001,0.705000000000001,0.710000000000001,
0.715000000000001,0.720000000000001,0.725000000000001,0.730000000000001,
0.735000000000001,0.740000000000001,0.745000000000001,0.750000000000001,
0.755000000000001,0.760000000000001,0.765000000000001,0.770000000000001,
0.775000000000001,0.780000000000001,0.785000000000001,0.790000000000001,
0.795000000000001,0.800000000000001,0.805000000000001,0.810000000000001,
0.815000000000001,0.820000000000001,0.825000000000001,0.830000000000001,
0.835000000000001,0.840000000000001,0.845000000000001,0.850000000000001,
0.855000000000001,0.860000000000001,0.865000000000001,0.870000000000001,
0.875000000000001,0.880000000000001,0.885000000000001,0.890000000000001,
0.895000000000001,0.900000000000001,0.905000000000001,0.910000000000001,
0.915000000000001,0.920000000000001,0.925000000000001,0.930000000000001,
0.935000000000001,0.940000000000001,0.941429844431395),.UNSPECIFIED.)
CURVE()
GEOMETRIC_REPRESENTATION_ITEM()
RATIONAL_B_SPLINE_CURVE((1.,1.,1.,1.,1.,1.,1.,1.,1.,1.,1.,1.,1.,1.,1.,1.,
1.,1.,1.,1.,1.,1.,1.,1.,1.,1.,1.,1.,1.,1.,1.,1.,1.,1.,1.,1.,1.,1.,1.,1.,
1.,1.,1.,1.,1.,1.,1.,1.,1.,1.,1.,1.,1.,1.,1.,1.,1.,1.,1.,1.,1.,1.,1.,1.,
1.,1.,1.,1.,1.,1.,1.,1.,1.,1.,1.,1.,1.,1.,1.,1.,1.,1.,1.,1.,1.,1.,1.,1.,
1.,1.,1.,1.,1.,1.,1.,1.,1.,1.,1.,1.,1.,1.,1.,1.,1.,1.,1.,1.,1.,1.,1.,1.,
1.,1.,1.,1.,1.,1.,1.,1.,1.,1.,1.,1.,1.,1.,1.,1.,1.,1.,1.,1.,1.,1.,1.,1.,
1.,1.,1.,1.,1.,1.,1.,1.,1.,1.,1.,1.,1.,1.,1.,1.,1.,1.,1.,1.,1.,1.,1.,1.,
1.,1.,1.,1.,1.,1.,1.,1.,1.,1.,1.,1.,1.,1.,1.,1.,1.,1.,1.,1.,1.,1.,1.,1.,
1.,1.,1.,1.,1.,1.,1.,1.,1.,1.))
REPRESENTATION_ITEM('')
);
#442=(
BOUNDED_CURVE()
B_SPLINE_CURVE(5,(#70253,#70254,#70255,#70256,#70257,#70258,#70259,#70260,
#70261,#70262,#70263,#70264,#70265,#70266,#70267,#70268,#70269,#70270,#70271,
#70272,#70273,#70274,#70275,#70276,#70277,#70278,#70279,#70280,#70281,#70282,
#70283,#70284,#70285,#70286,#70287,#70288,#70289,#70290,#70291,#70292,#70293,
#70294,#70295,#70296,#70297,#70298,#70299,#70300,#70301,#70302,#70303,#70304,
#70305,#70306,#70307,#70308,#70309,#70310,#70311,#70312,#70313,#70314,#70315,
#70316,#70317,#70318,#70319,#70320,#70321,#70322,#70323,#70324,#70325,#70326,
#70327,#70328,#70329,#70330,#70331,#70332,#70333,#70334,#70335,#70336,#70337,
#70338,#70339,#70340,#70341,#70342,#70343,#70344,#70345,#70346,#70347,#70348,
#70349,#70350,#70351,#70352,#70353,#70354,#70355,#70356,#70357,#70358,#70359,
#70360,#70361,#70362,#70363,#70364,#70365,#70366,#70367,#70368,#70369,#70370,
#70371,#70372,#70373,#70374,#70375,#70376,#70377,#70378,#70379,#70380,#70381,
#70382,#70383,#70384,#70385,#70386,#70387,#70388,#70389,#70390,#70391,#70392,
#70393,#70394,#70395,#70396,#70397,#70398,#70399,#70400,#70401,#70402,#70403,
#70404,#70405,#70406,#70407,#70408,#70409,#70410,#70411,#70412,#70413,#70414,
#70415,#70416,#70417,#70418,#70419,#70420,#70421,#70422,#70423,#70424,#70425,
#70426,#70427,#70428,#70429,#70430,#70431,#70432,#70433,#70434,#70435,#70436,
#70437,#70438,#70439,#70440,#70441,#70442,#70443,#70444,#70445,#70446),
 .UNSPECIFIED.,.F.,.F.)
B_SPLINE_CURVE_WITH_KNOTS((6,1,1,1,1,1,1,1,1,1,1,1,1,1,1,1,1,1,1,1,1,1,
1,1,1,1,1,1,1,1,1,1,1,1,1,1,1,1,1,1,1,1,1,1,1,1,1,1,1,1,1,1,1,1,1,1,1,1,
1,1,1,1,1,1,1,1,1,1,1,1,1,1,1,1,1,1,1,1,1,1,1,1,1,1,1,1,1,1,1,1,1,1,1,1,
1,1,1,1,1,1,1,1,1,1,1,1,1,1,1,1,1,1,1,1,1,1,1,1,1,1,1,1,1,1,1,1,1,1,1,1,
1,1,1,1,1,1,1,1,1,1,1,1,1,1,1,1,1,1,1,1,1,1,1,1,1,1,1,1,1,1,1,1,1,1,1,1,
1,1,1,1,1,1,1,1,1,1,1,1,1,1,1,1,1,1,1,1,1,1,1,6),(-0.941429844431395,-0.940000000000001,
-0.935000000000001,-0.930000000000001,-0.925000000000001,-0.920000000000001,
-0.915000000000001,-0.910000000000001,-0.905000000000001,-0.900000000000001,
-0.895000000000001,-0.890000000000001,-0.885000000000001,-0.880000000000001,
-0.875000000000001,-0.870000000000001,-0.865000000000001,-0.860000000000001,
-0.855000000000001,-0.850000000000001,-0.845000000000001,-0.840000000000001,
-0.835000000000001,-0.830000000000001,-0.825000000000001,-0.820000000000001,
-0.815000000000001,-0.810000000000001,-0.805000000000001,-0.800000000000001,
-0.795000000000001,-0.790000000000001,-0.785000000000001,-0.780000000000001,
-0.775000000000001,-0.770000000000001,-0.765000000000001,-0.760000000000001,
-0.755000000000001,-0.750000000000001,-0.745000000000001,-0.740000000000001,
-0.735000000000001,-0.730000000000001,-0.725000000000001,-0.720000000000001,
-0.715000000000001,-0.710000000000001,-0.705000000000001,-0.700000000000001,
-0.695000000000001,-0.690000000000001,-0.685,-0.68,-0.675,-0.67,-0.665,
-0.66,-0.655,-0.65,-0.645,-0.64,-0.635,-0.63,-0.625,-0.62,-0.615,-0.61,
-0.605,-0.6,-0.595,-0.59,-0.585,-0.58,-0.575,-0.57,-0.565,-0.56,-0.555,
-0.55,-0.545,-0.54,-0.535,-0.53,-0.525,-0.52,-0.515,-0.51,-0.505,-0.5,-0.495,
-0.49,-0.485,-0.48,-0.475,-0.47,-0.465,-0.46,-0.455,-0.45,-0.445,-0.44,
-0.435,-0.43,-0.425,-0.42,-0.415,-0.41,-0.405,-0.4,-0.395,-0.39,-0.385,
-0.38,-0.375,-0.37,-0.365,-0.36,-0.355,-0.35,-0.345,-0.34,-0.335,-0.33,
-0.325,-0.32,-0.315,-0.31,-0.305,-0.3,-0.295,-0.29,-0.285,-0.28,-0.275,
-0.27,-0.265,-0.26,-0.255,-0.25,-0.245,-0.24,-0.235,-0.23,-0.225,-0.22,
-0.215,-0.21,-0.205,-0.2,-0.195,-0.19,-0.185,-0.18,-0.175,-0.17,-0.165,
-0.16,-0.155,-0.15,-0.145,-0.14,-0.135,-0.13,-0.125,-0.12,-0.115,-0.11,
-0.105,-0.1,-0.095,-0.09,-0.085,-0.08,-0.075,-0.07,-0.065,-0.06,-0.055,
-0.05,-0.045,-0.04,-0.035,-0.03,-0.025,-0.02,-0.015,-0.01,-0.005,0.),
 .UNSPECIFIED.)
CURVE()
GEOMETRIC_REPRESENTATION_ITEM()
RATIONAL_B_SPLINE_CURVE((1.,1.,1.,1.,1.,1.,1.,1.,1.,1.,1.,1.,1.,1.,1.,1.,
1.,1.,1.,1.,1.,1.,1.,1.,1.,1.,1.,1.,1.,1.,1.,1.,1.,1.,1.,1.,1.,1.,1.,1.,
1.,1.,1.,1.,1.,1.,1.,1.,1.,1.,1.,1.,1.,1.,1.,1.,1.,1.,1.,1.,1.,1.,1.,1.,
1.,1.,1.,1.,1.,1.,1.,1.,1.,1.,1.,1.,1.,1.,1.,1.,1.,1.,1.,1.,1.,1.,1.,1.,
1.,1.,1.,1.,1.,1.,1.,1.,1.,1.,1.,1.,1.,1.,1.,1.,1.,1.,1.,1.,1.,1.,1.,1.,
1.,1.,1.,1.,1.,1.,1.,1.,1.,1.,1.,1.,1.,1.,1.,1.,1.,1.,1.,1.,1.,1.,1.,1.,
1.,1.,1.,1.,1.,1.,1.,1.,1.,1.,1.,1.,1.,1.,1.,1.,1.,1.,1.,1.,1.,1.,1.,1.,
1.,1.,1.,1.,1.,1.,1.,1.,1.,1.,1.,1.,1.,1.,1.,1.,1.,1.,1.,1.,1.,1.,1.,1.,
1.,1.,1.,1.,1.,1.,1.,1.,1.,1.))
REPRESENTATION_ITEM('')
);
#443=(
BOUNDED_CURVE()
B_SPLINE_CURVE(5,(#70953,#70954,#70955,#70956,#70957,#70958,#70959,#70960,
#70961,#70962,#70963,#70964,#70965,#70966,#70967,#70968,#70969,#70970,#70971,
#70972,#70973,#70974,#70975,#70976,#70977,#70978,#70979,#70980,#70981,#70982,
#70983,#70984,#70985,#70986,#70987,#70988,#70989,#70990,#70991,#70992,#70993,
#70994,#70995,#70996,#70997,#70998,#70999,#71000,#71001,#71002,#71003,#71004,
#71005,#71006,#71007,#71008,#71009,#71010,#71011,#71012,#71013,#71014,#71015,
#71016,#71017,#71018,#71019,#71020,#71021,#71022,#71023,#71024,#71025,#71026,
#71027,#71028,#71029,#71030,#71031,#71032,#71033,#71034,#71035,#71036,#71037,
#71038,#71039,#71040,#71041,#71042,#71043,#71044,#71045,#71046,#71047,#71048,
#71049,#71050,#71051,#71052,#71053,#71054,#71055,#71056,#71057,#71058,#71059,
#71060,#71061,#71062,#71063,#71064,#71065,#71066,#71067,#71068,#71069,#71070,
#71071,#71072,#71073,#71074,#71075,#71076,#71077,#71078,#71079,#71080,#71081,
#71082,#71083,#71084,#71085,#71086,#71087,#71088,#71089,#71090,#71091,#71092,
#71093,#71094,#71095,#71096,#71097,#71098,#71099,#71100,#71101,#71102,#71103,
#71104,#71105,#71106,#71107,#71108,#71109,#71110,#71111,#71112,#71113,#71114,
#71115,#71116,#71117,#71118,#71119,#71120,#71121,#71122,#71123,#71124,#71125,
#71126,#71127,#71128,#71129,#71130,#71131,#71132,#71133,#71134,#71135,#71136,
#71137,#71138,#71139,#71140,#71141,#71142,#71143,#71144,#71145,#71146),
 .UNSPECIFIED.,.F.,.F.)
B_SPLINE_CURVE_WITH_KNOTS((6,1,1,1,1,1,1,1,1,1,1,1,1,1,1,1,1,1,1,1,1,1,
1,1,1,1,1,1,1,1,1,1,1,1,1,1,1,1,1,1,1,1,1,1,1,1,1,1,1,1,1,1,1,1,1,1,1,1,
1,1,1,1,1,1,1,1,1,1,1,1,1,1,1,1,1,1,1,1,1,1,1,1,1,1,1,1,1,1,1,1,1,1,1,1,
1,1,1,1,1,1,1,1,1,1,1,1,1,1,1,1,1,1,1,1,1,1,1,1,1,1,1,1,1,1,1,1,1,1,1,1,
1,1,1,1,1,1,1,1,1,1,1,1,1,1,1,1,1,1,1,1,1,1,1,1,1,1,1,1,1,1,1,1,1,1,1,1,
1,1,1,1,1,1,1,1,1,1,1,1,1,1,1,1,1,1,1,1,1,1,1,6),(0.,0.005,0.01,0.015,0.02,
0.025,0.03,0.035,0.04,0.045,0.05,0.055,0.06,0.065,0.07,0.075,0.08,0.085,
0.09,0.095,0.1,0.105,0.11,0.115,0.12,0.125,0.13,0.135,0.14,0.145,0.15,0.155,
0.16,0.165,0.17,0.175,0.18,0.185,0.19,0.195,0.2,0.205,0.21,0.215,0.22,0.225,
0.23,0.235,0.24,0.245,0.25,0.255,0.26,0.265,0.27,0.275,0.28,0.285,0.29,
0.295,0.3,0.305,0.31,0.315,0.32,0.325,0.33,0.335,0.34,0.345,0.35,0.355,
0.36,0.365,0.37,0.375,0.38,0.385,0.39,0.395,0.4,0.405,0.41,0.415,0.42,0.425,
0.43,0.435,0.44,0.445,0.45,0.455,0.46,0.465,0.47,0.475,0.48,0.485,0.49,
0.495,0.5,0.505,0.51,0.515,0.52,0.525,0.53,0.535,0.54,0.545,0.55,0.555,
0.56,0.565,0.57,0.575,0.58,0.585,0.59,0.595,0.6,0.605,0.61,0.615,0.62,0.625,
0.63,0.635,0.64,0.645,0.65,0.655,0.66,0.665,0.67,0.675,0.68,0.685,0.690000000000001,
0.695000000000001,0.700000000000001,0.705000000000001,0.710000000000001,
0.715000000000001,0.720000000000001,0.725000000000001,0.730000000000001,
0.735000000000001,0.740000000000001,0.745000000000001,0.750000000000001,
0.755000000000001,0.760000000000001,0.765000000000001,0.770000000000001,
0.775000000000001,0.780000000000001,0.785000000000001,0.790000000000001,
0.795000000000001,0.800000000000001,0.805000000000001,0.810000000000001,
0.815000000000001,0.820000000000001,0.825000000000001,0.830000000000001,
0.835000000000001,0.840000000000001,0.845000000000001,0.850000000000001,
0.855000000000001,0.860000000000001,0.865000000000001,0.870000000000001,
0.875000000000001,0.880000000000001,0.885000000000001,0.890000000000001,
0.895000000000001,0.900000000000001,0.905000000000001,0.910000000000001,
0.915000000000001,0.920000000000001,0.925000000000001,0.930000000000001,
0.935000000000001,0.940000000000001,0.941429844431403),.UNSPECIFIED.)
CURVE()
GEOMETRIC_REPRESENTATION_ITEM()
RATIONAL_B_SPLINE_CURVE((1.,1.,1.,1.,1.,1.,1.,1.,1.,1.,1.,1.,1.,1.,1.,1.,
1.,1.,1.,1.,1.,1.,1.,1.,1.,1.,1.,1.,1.,1.,1.,1.,1.,1.,1.,1.,1.,1.,1.,1.,
1.,1.,1.,1.,1.,1.,1.,1.,1.,1.,1.,1.,1.,1.,1.,1.,1.,1.,1.,1.,1.,1.,1.,1.,
1.,1.,1.,1.,1.,1.,1.,1.,1.,1.,1.,1.,1.,1.,1.,1.,1.,1.,1.,1.,1.,1.,1.,1.,
1.,1.,1.,1.,1.,1.,1.,1.,1.,1.,1.,1.,1.,1.,1.,1.,1.,1.,1.,1.,1.,1.,1.,1.,
1.,1.,1.,1.,1.,1.,1.,1.,1.,1.,1.,1.,1.,1.,1.,1.,1.,1.,1.,1.,1.,1.,1.,1.,
1.,1.,1.,1.,1.,1.,1.,1.,1.,1.,1.,1.,1.,1.,1.,1.,1.,1.,1.,1.,1.,1.,1.,1.,
1.,1.,1.,1.,1.,1.,1.,1.,1.,1.,1.,1.,1.,1.,1.,1.,1.,1.,1.,1.,1.,1.,1.,1.,
1.,1.,1.,1.,1.,1.,1.,1.,1.,1.))
REPRESENTATION_ITEM('')
);
#444=(
BOUNDED_CURVE()
B_SPLINE_CURVE(5,(#71149,#71150,#71151,#71152,#71153,#71154,#71155,#71156,
#71157,#71158,#71159,#71160,#71161,#71162,#71163,#71164,#71165,#71166,#71167,
#71168,#71169,#71170,#71171,#71172,#71173,#71174,#71175,#71176,#71177,#71178,
#71179,#71180,#71181,#71182,#71183,#71184,#71185,#71186,#71187,#71188,#71189,
#71190,#71191,#71192,#71193,#71194,#71195,#71196,#71197,#71198,#71199,#71200,
#71201,#71202,#71203,#71204,#71205,#71206,#71207,#71208,#71209,#71210,#71211,
#71212,#71213,#71214,#71215,#71216,#71217,#71218,#71219,#71220,#71221,#71222,
#71223,#71224,#71225,#71226,#71227,#71228,#71229,#71230,#71231,#71232,#71233,
#71234,#71235,#71236,#71237,#71238,#71239,#71240,#71241,#71242,#71243,#71244,
#71245,#71246,#71247,#71248,#71249,#71250,#71251,#71252,#71253,#71254,#71255,
#71256,#71257,#71258,#71259,#71260,#71261,#71262,#71263,#71264,#71265,#71266,
#71267,#71268,#71269,#71270,#71271,#71272,#71273,#71274,#71275,#71276,#71277,
#71278,#71279,#71280,#71281,#71282,#71283,#71284,#71285,#71286,#71287,#71288,
#71289,#71290,#71291,#71292,#71293,#71294,#71295,#71296,#71297,#71298,#71299,
#71300,#71301,#71302,#71303,#71304,#71305,#71306,#71307,#71308,#71309,#71310,
#71311,#71312,#71313,#71314,#71315,#71316,#71317,#71318,#71319,#71320,#71321,
#71322,#71323,#71324,#71325,#71326,#71327,#71328,#71329,#71330,#71331,#71332,
#71333,#71334,#71335,#71336,#71337,#71338,#71339,#71340,#71341,#71342),
 .UNSPECIFIED.,.F.,.F.)
B_SPLINE_CURVE_WITH_KNOTS((6,1,1,1,1,1,1,1,1,1,1,1,1,1,1,1,1,1,1,1,1,1,
1,1,1,1,1,1,1,1,1,1,1,1,1,1,1,1,1,1,1,1,1,1,1,1,1,1,1,1,1,1,1,1,1,1,1,1,
1,1,1,1,1,1,1,1,1,1,1,1,1,1,1,1,1,1,1,1,1,1,1,1,1,1,1,1,1,1,1,1,1,1,1,1,
1,1,1,1,1,1,1,1,1,1,1,1,1,1,1,1,1,1,1,1,1,1,1,1,1,1,1,1,1,1,1,1,1,1,1,1,
1,1,1,1,1,1,1,1,1,1,1,1,1,1,1,1,1,1,1,1,1,1,1,1,1,1,1,1,1,1,1,1,1,1,1,1,
1,1,1,1,1,1,1,1,1,1,1,1,1,1,1,1,1,1,1,1,1,1,1,6),(-0.941429844431403,-0.940000000000001,
-0.935000000000001,-0.930000000000001,-0.925000000000001,-0.920000000000001,
-0.915000000000001,-0.910000000000001,-0.905000000000001,-0.900000000000001,
-0.895000000000001,-0.890000000000001,-0.885000000000001,-0.880000000000001,
-0.875000000000001,-0.870000000000001,-0.865000000000001,-0.860000000000001,
-0.855000000000001,-0.850000000000001,-0.845000000000001,-0.840000000000001,
-0.835000000000001,-0.830000000000001,-0.825000000000001,-0.820000000000001,
-0.815000000000001,-0.810000000000001,-0.805000000000001,-0.800000000000001,
-0.795000000000001,-0.790000000000001,-0.785000000000001,-0.780000000000001,
-0.775000000000001,-0.770000000000001,-0.765000000000001,-0.760000000000001,
-0.755000000000001,-0.750000000000001,-0.745000000000001,-0.740000000000001,
-0.735000000000001,-0.730000000000001,-0.725000000000001,-0.720000000000001,
-0.715000000000001,-0.710000000000001,-0.705000000000001,-0.700000000000001,
-0.695000000000001,-0.690000000000001,-0.685,-0.68,-0.675,-0.67,-0.665,
-0.66,-0.655,-0.65,-0.645,-0.64,-0.635,-0.63,-0.625,-0.62,-0.615,-0.61,
-0.605,-0.6,-0.595,-0.59,-0.585,-0.58,-0.575,-0.57,-0.565,-0.56,-0.555,
-0.55,-0.545,-0.54,-0.535,-0.53,-0.525,-0.52,-0.515,-0.51,-0.505,-0.5,-0.495,
-0.49,-0.485,-0.48,-0.475,-0.47,-0.465,-0.46,-0.455,-0.45,-0.445,-0.44,
-0.435,-0.43,-0.425,-0.42,-0.415,-0.41,-0.405,-0.4,-0.395,-0.39,-0.385,
-0.38,-0.375,-0.37,-0.365,-0.36,-0.355,-0.35,-0.345,-0.34,-0.335,-0.33,
-0.325,-0.32,-0.315,-0.31,-0.305,-0.3,-0.295,-0.29,-0.285,-0.28,-0.275,
-0.27,-0.265,-0.26,-0.255,-0.25,-0.245,-0.24,-0.235,-0.23,-0.225,-0.22,
-0.215,-0.21,-0.205,-0.2,-0.195,-0.19,-0.185,-0.18,-0.175,-0.17,-0.165,
-0.16,-0.155,-0.15,-0.145,-0.14,-0.135,-0.13,-0.125,-0.12,-0.115,-0.11,
-0.105,-0.1,-0.095,-0.09,-0.085,-0.08,-0.075,-0.07,-0.065,-0.06,-0.055,
-0.05,-0.045,-0.04,-0.035,-0.03,-0.025,-0.02,-0.015,-0.01,-0.005,0.),
 .UNSPECIFIED.)
CURVE()
GEOMETRIC_REPRESENTATION_ITEM()
RATIONAL_B_SPLINE_CURVE((1.,1.,1.,1.,1.,1.,1.,1.,1.,1.,1.,1.,1.,1.,1.,1.,
1.,1.,1.,1.,1.,1.,1.,1.,1.,1.,1.,1.,1.,1.,1.,1.,1.,1.,1.,1.,1.,1.,1.,1.,
1.,1.,1.,1.,1.,1.,1.,1.,1.,1.,1.,1.,1.,1.,1.,1.,1.,1.,1.,1.,1.,1.,1.,1.,
1.,1.,1.,1.,1.,1.,1.,1.,1.,1.,1.,1.,1.,1.,1.,1.,1.,1.,1.,1.,1.,1.,1.,1.,
1.,1.,1.,1.,1.,1.,1.,1.,1.,1.,1.,1.,1.,1.,1.,1.,1.,1.,1.,1.,1.,1.,1.,1.,
1.,1.,1.,1.,1.,1.,1.,1.,1.,1.,1.,1.,1.,1.,1.,1.,1.,1.,1.,1.,1.,1.,1.,1.,
1.,1.,1.,1.,1.,1.,1.,1.,1.,1.,1.,1.,1.,1.,1.,1.,1.,1.,1.,1.,1.,1.,1.,1.,
1.,1.,1.,1.,1.,1.,1.,1.,1.,1.,1.,1.,1.,1.,1.,1.,1.,1.,1.,1.,1.,1.,1.,1.,
1.,1.,1.,1.,1.,1.,1.,1.,1.,1.))
REPRESENTATION_ITEM('')
);
#445=(
BOUNDED_CURVE()
B_SPLINE_CURVE(5,(#71849,#71850,#71851,#71852,#71853,#71854,#71855,#71856,
#71857,#71858,#71859,#71860,#71861,#71862,#71863,#71864,#71865,#71866,#71867,
#71868,#71869,#71870,#71871,#71872,#71873,#71874,#71875,#71876,#71877,#71878,
#71879,#71880,#71881,#71882,#71883,#71884,#71885,#71886,#71887,#71888,#71889,
#71890,#71891,#71892,#71893,#71894,#71895,#71896,#71897,#71898,#71899,#71900,
#71901,#71902,#71903,#71904,#71905,#71906,#71907,#71908,#71909,#71910,#71911,
#71912,#71913,#71914,#71915,#71916,#71917,#71918,#71919,#71920,#71921,#71922,
#71923,#71924,#71925,#71926,#71927,#71928,#71929,#71930,#71931,#71932,#71933,
#71934,#71935,#71936,#71937,#71938,#71939,#71940,#71941,#71942,#71943,#71944,
#71945,#71946,#71947,#71948,#71949,#71950,#71951,#71952,#71953,#71954,#71955,
#71956,#71957,#71958,#71959,#71960,#71961,#71962,#71963,#71964,#71965,#71966,
#71967,#71968,#71969,#71970,#71971,#71972,#71973,#71974,#71975,#71976,#71977,
#71978,#71979,#71980,#71981,#71982,#71983,#71984,#71985,#71986,#71987,#71988,
#71989,#71990,#71991,#71992,#71993,#71994,#71995,#71996,#71997,#71998,#71999,
#72000,#72001,#72002,#72003,#72004,#72005,#72006,#72007,#72008,#72009,#72010,
#72011,#72012,#72013,#72014,#72015,#72016,#72017,#72018,#72019,#72020,#72021,
#72022,#72023,#72024,#72025,#72026,#72027,#72028,#72029,#72030,#72031,#72032,
#72033,#72034,#72035,#72036,#72037,#72038,#72039,#72040,#72041,#72042),
 .UNSPECIFIED.,.F.,.F.)
B_SPLINE_CURVE_WITH_KNOTS((6,1,1,1,1,1,1,1,1,1,1,1,1,1,1,1,1,1,1,1,1,1,
1,1,1,1,1,1,1,1,1,1,1,1,1,1,1,1,1,1,1,1,1,1,1,1,1,1,1,1,1,1,1,1,1,1,1,1,
1,1,1,1,1,1,1,1,1,1,1,1,1,1,1,1,1,1,1,1,1,1,1,1,1,1,1,1,1,1,1,1,1,1,1,1,
1,1,1,1,1,1,1,1,1,1,1,1,1,1,1,1,1,1,1,1,1,1,1,1,1,1,1,1,1,1,1,1,1,1,1,1,
1,1,1,1,1,1,1,1,1,1,1,1,1,1,1,1,1,1,1,1,1,1,1,1,1,1,1,1,1,1,1,1,1,1,1,1,
1,1,1,1,1,1,1,1,1,1,1,1,1,1,1,1,1,1,1,1,1,1,1,6),(0.,0.005,0.01,0.015,0.02,
0.025,0.03,0.035,0.04,0.045,0.05,0.055,0.06,0.065,0.07,0.075,0.08,0.085,
0.09,0.095,0.1,0.105,0.11,0.115,0.12,0.125,0.13,0.135,0.14,0.145,0.15,0.155,
0.16,0.165,0.17,0.175,0.18,0.185,0.19,0.195,0.2,0.205,0.21,0.215,0.22,0.225,
0.23,0.235,0.24,0.245,0.25,0.255,0.26,0.265,0.27,0.275,0.28,0.285,0.29,
0.295,0.3,0.305,0.31,0.315,0.32,0.325,0.33,0.335,0.34,0.345,0.35,0.355,
0.36,0.365,0.37,0.375,0.38,0.385,0.39,0.395,0.4,0.405,0.41,0.415,0.42,0.425,
0.43,0.435,0.44,0.445,0.45,0.455,0.46,0.465,0.47,0.475,0.48,0.485,0.49,
0.495,0.5,0.505,0.51,0.515,0.52,0.525,0.53,0.535,0.54,0.545,0.55,0.555,
0.56,0.565,0.57,0.575,0.58,0.585,0.59,0.595,0.6,0.605,0.61,0.615,0.62,0.625,
0.63,0.635,0.64,0.645,0.65,0.655,0.66,0.665,0.67,0.675,0.68,0.685,0.690000000000001,
0.695000000000001,0.700000000000001,0.705000000000001,0.710000000000001,
0.715000000000001,0.720000000000001,0.725000000000001,0.730000000000001,
0.735000000000001,0.740000000000001,0.745000000000001,0.750000000000001,
0.755000000000001,0.760000000000001,0.765000000000001,0.770000000000001,
0.775000000000001,0.780000000000001,0.785000000000001,0.790000000000001,
0.795000000000001,0.800000000000001,0.805000000000001,0.810000000000001,
0.815000000000001,0.820000000000001,0.825000000000001,0.830000000000001,
0.835000000000001,0.840000000000001,0.845000000000001,0.850000000000001,
0.855000000000001,0.860000000000001,0.865000000000001,0.870000000000001,
0.875000000000001,0.880000000000001,0.885000000000001,0.890000000000001,
0.895000000000001,0.900000000000001,0.905000000000001,0.910000000000001,
0.915000000000001,0.920000000000001,0.925000000000001,0.930000000000001,
0.935000000000001,0.940000000000001,0.941429844431412),.UNSPECIFIED.)
CURVE()
GEOMETRIC_REPRESENTATION_ITEM()
RATIONAL_B_SPLINE_CURVE((1.,1.,1.,1.,1.,1.,1.,1.,1.,1.,1.,1.,1.,1.,1.,1.,
1.,1.,1.,1.,1.,1.,1.,1.,1.,1.,1.,1.,1.,1.,1.,1.,1.,1.,1.,1.,1.,1.,1.,1.,
1.,1.,1.,1.,1.,1.,1.,1.,1.,1.,1.,1.,1.,1.,1.,1.,1.,1.,1.,1.,1.,1.,1.,1.,
1.,1.,1.,1.,1.,1.,1.,1.,1.,1.,1.,1.,1.,1.,1.,1.,1.,1.,1.,1.,1.,1.,1.,1.,
1.,1.,1.,1.,1.,1.,1.,1.,1.,1.,1.,1.,1.,1.,1.,1.,1.,1.,1.,1.,1.,1.,1.,1.,
1.,1.,1.,1.,1.,1.,1.,1.,1.,1.,1.,1.,1.,1.,1.,1.,1.,1.,1.,1.,1.,1.,1.,1.,
1.,1.,1.,1.,1.,1.,1.,1.,1.,1.,1.,1.,1.,1.,1.,1.,1.,1.,1.,1.,1.,1.,1.,1.,
1.,1.,1.,1.,1.,1.,1.,1.,1.,1.,1.,1.,1.,1.,1.,1.,1.,1.,1.,1.,1.,1.,1.,1.,
1.,1.,1.,1.,1.,1.,1.,1.,1.,1.))
REPRESENTATION_ITEM('')
);
#446=(
BOUNDED_CURVE()
B_SPLINE_CURVE(5,(#72045,#72046,#72047,#72048,#72049,#72050,#72051,#72052,
#72053,#72054,#72055,#72056,#72057,#72058,#72059,#72060,#72061,#72062,#72063,
#72064,#72065,#72066,#72067,#72068,#72069,#72070,#72071,#72072,#72073,#72074,
#72075,#72076,#72077,#72078,#72079,#72080,#72081,#72082,#72083,#72084,#72085,
#72086,#72087,#72088,#72089,#72090,#72091,#72092,#72093,#72094,#72095,#72096,
#72097,#72098,#72099,#72100,#72101,#72102,#72103,#72104,#72105,#72106,#72107,
#72108,#72109,#72110,#72111,#72112,#72113,#72114,#72115,#72116,#72117,#72118,
#72119,#72120,#72121,#72122,#72123,#72124,#72125,#72126,#72127,#72128,#72129,
#72130,#72131,#72132,#72133,#72134,#72135,#72136,#72137,#72138,#72139,#72140,
#72141,#72142,#72143,#72144,#72145,#72146,#72147,#72148,#72149,#72150,#72151,
#72152,#72153,#72154,#72155,#72156,#72157,#72158,#72159,#72160,#72161,#72162,
#72163,#72164,#72165,#72166,#72167,#72168,#72169,#72170,#72171,#72172,#72173,
#72174,#72175,#72176,#72177,#72178,#72179,#72180,#72181,#72182,#72183,#72184,
#72185,#72186,#72187,#72188,#72189,#72190,#72191,#72192,#72193,#72194,#72195,
#72196,#72197,#72198,#72199,#72200,#72201,#72202,#72203,#72204,#72205,#72206,
#72207,#72208,#72209,#72210,#72211,#72212,#72213,#72214,#72215,#72216,#72217,
#72218,#72219,#72220,#72221,#72222,#72223,#72224,#72225,#72226,#72227,#72228,
#72229,#72230,#72231,#72232,#72233,#72234,#72235,#72236,#72237,#72238),
 .UNSPECIFIED.,.F.,.F.)
B_SPLINE_CURVE_WITH_KNOTS((6,1,1,1,1,1,1,1,1,1,1,1,1,1,1,1,1,1,1,1,1,1,
1,1,1,1,1,1,1,1,1,1,1,1,1,1,1,1,1,1,1,1,1,1,1,1,1,1,1,1,1,1,1,1,1,1,1,1,
1,1,1,1,1,1,1,1,1,1,1,1,1,1,1,1,1,1,1,1,1,1,1,1,1,1,1,1,1,1,1,1,1,1,1,1,
1,1,1,1,1,1,1,1,1,1,1,1,1,1,1,1,1,1,1,1,1,1,1,1,1,1,1,1,1,1,1,1,1,1,1,1,
1,1,1,1,1,1,1,1,1,1,1,1,1,1,1,1,1,1,1,1,1,1,1,1,1,1,1,1,1,1,1,1,1,1,1,1,
1,1,1,1,1,1,1,1,1,1,1,1,1,1,1,1,1,1,1,1,1,1,1,6),(-0.941429844431412,-0.940000000000001,
-0.935000000000001,-0.930000000000001,-0.925000000000001,-0.920000000000001,
-0.915000000000001,-0.910000000000001,-0.905000000000001,-0.900000000000001,
-0.895000000000001,-0.890000000000001,-0.885000000000001,-0.880000000000001,
-0.875000000000001,-0.870000000000001,-0.865000000000001,-0.860000000000001,
-0.855000000000001,-0.850000000000001,-0.845000000000001,-0.840000000000001,
-0.835000000000001,-0.830000000000001,-0.825000000000001,-0.820000000000001,
-0.815000000000001,-0.810000000000001,-0.805000000000001,-0.800000000000001,
-0.795000000000001,-0.790000000000001,-0.785000000000001,-0.780000000000001,
-0.775000000000001,-0.770000000000001,-0.765000000000001,-0.760000000000001,
-0.755000000000001,-0.750000000000001,-0.745000000000001,-0.740000000000001,
-0.735000000000001,-0.730000000000001,-0.725000000000001,-0.720000000000001,
-0.715000000000001,-0.710000000000001,-0.705000000000001,-0.700000000000001,
-0.695000000000001,-0.690000000000001,-0.685,-0.68,-0.675,-0.67,-0.665,
-0.66,-0.655,-0.65,-0.645,-0.64,-0.635,-0.63,-0.625,-0.62,-0.615,-0.61,
-0.605,-0.6,-0.595,-0.59,-0.585,-0.58,-0.575,-0.57,-0.565,-0.56,-0.555,
-0.55,-0.545,-0.54,-0.535,-0.53,-0.525,-0.52,-0.515,-0.51,-0.505,-0.5,-0.495,
-0.49,-0.485,-0.48,-0.475,-0.47,-0.465,-0.46,-0.455,-0.45,-0.445,-0.44,
-0.435,-0.43,-0.425,-0.42,-0.415,-0.41,-0.405,-0.4,-0.395,-0.39,-0.385,
-0.38,-0.375,-0.37,-0.365,-0.36,-0.355,-0.35,-0.345,-0.34,-0.335,-0.33,
-0.325,-0.32,-0.315,-0.31,-0.305,-0.3,-0.295,-0.29,-0.285,-0.28,-0.275,
-0.27,-0.265,-0.26,-0.255,-0.25,-0.245,-0.24,-0.235,-0.23,-0.225,-0.22,
-0.215,-0.21,-0.205,-0.2,-0.195,-0.19,-0.185,-0.18,-0.175,-0.17,-0.165,
-0.16,-0.155,-0.15,-0.145,-0.14,-0.135,-0.13,-0.125,-0.12,-0.115,-0.11,
-0.105,-0.1,-0.095,-0.09,-0.085,-0.08,-0.075,-0.07,-0.065,-0.06,-0.055,
-0.05,-0.045,-0.04,-0.035,-0.03,-0.025,-0.02,-0.015,-0.01,-0.005,0.),
 .UNSPECIFIED.)
CURVE()
GEOMETRIC_REPRESENTATION_ITEM()
RATIONAL_B_SPLINE_CURVE((1.,1.,1.,1.,1.,1.,1.,1.,1.,1.,1.,1.,1.,1.,1.,1.,
1.,1.,1.,1.,1.,1.,1.,1.,1.,1.,1.,1.,1.,1.,1.,1.,1.,1.,1.,1.,1.,1.,1.,1.,
1.,1.,1.,1.,1.,1.,1.,1.,1.,1.,1.,1.,1.,1.,1.,1.,1.,1.,1.,1.,1.,1.,1.,1.,
1.,1.,1.,1.,1.,1.,1.,1.,1.,1.,1.,1.,1.,1.,1.,1.,1.,1.,1.,1.,1.,1.,1.,1.,
1.,1.,1.,1.,1.,1.,1.,1.,1.,1.,1.,1.,1.,1.,1.,1.,1.,1.,1.,1.,1.,1.,1.,1.,
1.,1.,1.,1.,1.,1.,1.,1.,1.,1.,1.,1.,1.,1.,1.,1.,1.,1.,1.,1.,1.,1.,1.,1.,
1.,1.,1.,1.,1.,1.,1.,1.,1.,1.,1.,1.,1.,1.,1.,1.,1.,1.,1.,1.,1.,1.,1.,1.,
1.,1.,1.,1.,1.,1.,1.,1.,1.,1.,1.,1.,1.,1.,1.,1.,1.,1.,1.,1.,1.,1.,1.,1.,
1.,1.,1.,1.,1.,1.,1.,1.,1.,1.))
REPRESENTATION_ITEM('')
);
#447=(
BOUNDED_CURVE()
B_SPLINE_CURVE(5,(#72745,#72746,#72747,#72748,#72749,#72750,#72751,#72752,
#72753,#72754,#72755,#72756,#72757,#72758,#72759,#72760,#72761,#72762,#72763,
#72764,#72765,#72766,#72767,#72768,#72769,#72770,#72771,#72772,#72773,#72774,
#72775,#72776,#72777,#72778,#72779,#72780,#72781,#72782,#72783,#72784,#72785,
#72786,#72787,#72788,#72789,#72790,#72791,#72792,#72793,#72794,#72795,#72796,
#72797,#72798,#72799,#72800,#72801,#72802,#72803,#72804,#72805,#72806,#72807,
#72808,#72809,#72810,#72811,#72812,#72813,#72814,#72815,#72816,#72817,#72818,
#72819,#72820,#72821,#72822,#72823,#72824,#72825,#72826,#72827,#72828,#72829,
#72830,#72831,#72832,#72833,#72834,#72835,#72836,#72837,#72838,#72839,#72840,
#72841,#72842,#72843,#72844,#72845,#72846,#72847,#72848,#72849,#72850,#72851,
#72852,#72853,#72854,#72855,#72856,#72857,#72858,#72859,#72860,#72861,#72862,
#72863,#72864,#72865,#72866,#72867,#72868,#72869,#72870,#72871,#72872,#72873,
#72874,#72875,#72876,#72877,#72878,#72879,#72880,#72881,#72882,#72883,#72884,
#72885,#72886,#72887,#72888,#72889,#72890,#72891,#72892,#72893,#72894,#72895,
#72896,#72897,#72898,#72899,#72900,#72901,#72902,#72903,#72904,#72905,#72906,
#72907,#72908,#72909,#72910,#72911,#72912,#72913,#72914,#72915,#72916,#72917,
#72918,#72919,#72920,#72921,#72922,#72923,#72924,#72925,#72926,#72927,#72928,
#72929,#72930,#72931,#72932,#72933,#72934,#72935,#72936,#72937,#72938),
 .UNSPECIFIED.,.F.,.F.)
B_SPLINE_CURVE_WITH_KNOTS((6,1,1,1,1,1,1,1,1,1,1,1,1,1,1,1,1,1,1,1,1,1,
1,1,1,1,1,1,1,1,1,1,1,1,1,1,1,1,1,1,1,1,1,1,1,1,1,1,1,1,1,1,1,1,1,1,1,1,
1,1,1,1,1,1,1,1,1,1,1,1,1,1,1,1,1,1,1,1,1,1,1,1,1,1,1,1,1,1,1,1,1,1,1,1,
1,1,1,1,1,1,1,1,1,1,1,1,1,1,1,1,1,1,1,1,1,1,1,1,1,1,1,1,1,1,1,1,1,1,1,1,
1,1,1,1,1,1,1,1,1,1,1,1,1,1,1,1,1,1,1,1,1,1,1,1,1,1,1,1,1,1,1,1,1,1,1,1,
1,1,1,1,1,1,1,1,1,1,1,1,1,1,1,1,1,1,1,1,1,1,1,6),(0.,0.005,0.01,0.015,0.02,
0.025,0.03,0.035,0.04,0.045,0.05,0.055,0.06,0.065,0.07,0.075,0.08,0.085,
0.09,0.095,0.1,0.105,0.11,0.115,0.12,0.125,0.13,0.135,0.14,0.145,0.15,0.155,
0.16,0.165,0.17,0.175,0.18,0.185,0.19,0.195,0.2,0.205,0.21,0.215,0.22,0.225,
0.23,0.235,0.24,0.245,0.25,0.255,0.26,0.265,0.27,0.275,0.28,0.285,0.29,
0.295,0.3,0.305,0.31,0.315,0.32,0.325,0.33,0.335,0.34,0.345,0.35,0.355,
0.36,0.365,0.37,0.375,0.38,0.385,0.39,0.395,0.4,0.405,0.41,0.415,0.42,0.425,
0.43,0.435,0.44,0.445,0.45,0.455,0.46,0.465,0.47,0.475,0.48,0.485,0.49,
0.495,0.5,0.505,0.51,0.515,0.52,0.525,0.53,0.535,0.54,0.545,0.55,0.555,
0.56,0.565,0.57,0.575,0.58,0.585,0.59,0.595,0.6,0.605,0.61,0.615,0.62,0.625,
0.63,0.635,0.64,0.645,0.65,0.655,0.66,0.665,0.67,0.675,0.68,0.685,0.690000000000001,
0.695000000000001,0.700000000000001,0.705000000000001,0.710000000000001,
0.715000000000001,0.720000000000001,0.725000000000001,0.730000000000001,
0.735000000000001,0.740000000000001,0.745000000000001,0.750000000000001,
0.755000000000001,0.760000000000001,0.765000000000001,0.770000000000001,
0.775000000000001,0.780000000000001,0.785000000000001,0.790000000000001,
0.795000000000001,0.800000000000001,0.805000000000001,0.810000000000001,
0.815000000000001,0.820000000000001,0.825000000000001,0.830000000000001,
0.835000000000001,0.840000000000001,0.845000000000001,0.850000000000001,
0.855000000000001,0.860000000000001,0.865000000000001,0.870000000000001,
0.875000000000001,0.880000000000001,0.885000000000001,0.890000000000001,
0.895000000000001,0.900000000000001,0.905000000000001,0.910000000000001,
0.915000000000001,0.920000000000001,0.925000000000001,0.930000000000001,
0.935000000000001,0.940000000000001,0.941429844431353),.UNSPECIFIED.)
CURVE()
GEOMETRIC_REPRESENTATION_ITEM()
RATIONAL_B_SPLINE_CURVE((1.,1.,1.,1.,1.,1.,1.,1.,1.,1.,1.,1.,1.,1.,1.,1.,
1.,1.,1.,1.,1.,1.,1.,1.,1.,1.,1.,1.,1.,1.,1.,1.,1.,1.,1.,1.,1.,1.,1.,1.,
1.,1.,1.,1.,1.,1.,1.,1.,1.,1.,1.,1.,1.,1.,1.,1.,1.,1.,1.,1.,1.,1.,1.,1.,
1.,1.,1.,1.,1.,1.,1.,1.,1.,1.,1.,1.,1.,1.,1.,1.,1.,1.,1.,1.,1.,1.,1.,1.,
1.,1.,1.,1.,1.,1.,1.,1.,1.,1.,1.,1.,1.,1.,1.,1.,1.,1.,1.,1.,1.,1.,1.,1.,
1.,1.,1.,1.,1.,1.,1.,1.,1.,1.,1.,1.,1.,1.,1.,1.,1.,1.,1.,1.,1.,1.,1.,1.,
1.,1.,1.,1.,1.,1.,1.,1.,1.,1.,1.,1.,1.,1.,1.,1.,1.,1.,1.,1.,1.,1.,1.,1.,
1.,1.,1.,1.,1.,1.,1.,1.,1.,1.,1.,1.,1.,1.,1.,1.,1.,1.,1.,1.,1.,1.,1.,1.,
1.,1.,1.,1.,1.,1.,1.,1.,1.,1.))
REPRESENTATION_ITEM('')
);
#448=(
BOUNDED_CURVE()
B_SPLINE_CURVE(5,(#72941,#72942,#72943,#72944,#72945,#72946,#72947,#72948,
#72949,#72950,#72951,#72952,#72953,#72954,#72955,#72956,#72957,#72958,#72959,
#72960,#72961,#72962,#72963,#72964,#72965,#72966,#72967,#72968,#72969,#72970,
#72971,#72972,#72973,#72974,#72975,#72976,#72977,#72978,#72979,#72980,#72981,
#72982,#72983,#72984,#72985,#72986,#72987,#72988,#72989,#72990,#72991,#72992,
#72993,#72994,#72995,#72996,#72997,#72998,#72999,#73000,#73001,#73002,#73003,
#73004,#73005,#73006,#73007,#73008,#73009,#73010,#73011,#73012,#73013,#73014,
#73015,#73016,#73017,#73018,#73019,#73020,#73021,#73022,#73023,#73024,#73025,
#73026,#73027,#73028,#73029,#73030,#73031,#73032,#73033,#73034,#73035,#73036,
#73037,#73038,#73039,#73040,#73041,#73042,#73043,#73044,#73045,#73046,#73047,
#73048,#73049,#73050,#73051,#73052,#73053,#73054,#73055,#73056,#73057,#73058,
#73059,#73060,#73061,#73062,#73063,#73064,#73065,#73066,#73067,#73068,#73069,
#73070,#73071,#73072,#73073,#73074,#73075,#73076,#73077,#73078,#73079,#73080,
#73081,#73082,#73083,#73084,#73085,#73086,#73087,#73088,#73089,#73090,#73091,
#73092,#73093,#73094,#73095,#73096,#73097,#73098,#73099,#73100,#73101,#73102,
#73103,#73104,#73105,#73106,#73107,#73108,#73109,#73110,#73111,#73112,#73113,
#73114,#73115,#73116,#73117,#73118,#73119,#73120,#73121,#73122,#73123,#73124,
#73125,#73126,#73127,#73128,#73129,#73130,#73131,#73132,#73133,#73134),
 .UNSPECIFIED.,.F.,.F.)
B_SPLINE_CURVE_WITH_KNOTS((6,1,1,1,1,1,1,1,1,1,1,1,1,1,1,1,1,1,1,1,1,1,
1,1,1,1,1,1,1,1,1,1,1,1,1,1,1,1,1,1,1,1,1,1,1,1,1,1,1,1,1,1,1,1,1,1,1,1,
1,1,1,1,1,1,1,1,1,1,1,1,1,1,1,1,1,1,1,1,1,1,1,1,1,1,1,1,1,1,1,1,1,1,1,1,
1,1,1,1,1,1,1,1,1,1,1,1,1,1,1,1,1,1,1,1,1,1,1,1,1,1,1,1,1,1,1,1,1,1,1,1,
1,1,1,1,1,1,1,1,1,1,1,1,1,1,1,1,1,1,1,1,1,1,1,1,1,1,1,1,1,1,1,1,1,1,1,1,
1,1,1,1,1,1,1,1,1,1,1,1,1,1,1,1,1,1,1,1,1,1,1,6),(-0.941429844431353,-0.940000000000001,
-0.935000000000001,-0.930000000000001,-0.925000000000001,-0.920000000000001,
-0.915000000000001,-0.910000000000001,-0.905000000000001,-0.900000000000001,
-0.895000000000001,-0.890000000000001,-0.885000000000001,-0.880000000000001,
-0.875000000000001,-0.870000000000001,-0.865000000000001,-0.860000000000001,
-0.855000000000001,-0.850000000000001,-0.845000000000001,-0.840000000000001,
-0.835000000000001,-0.830000000000001,-0.825000000000001,-0.820000000000001,
-0.815000000000001,-0.810000000000001,-0.805000000000001,-0.800000000000001,
-0.795000000000001,-0.790000000000001,-0.785000000000001,-0.780000000000001,
-0.775000000000001,-0.770000000000001,-0.765000000000001,-0.760000000000001,
-0.755000000000001,-0.750000000000001,-0.745000000000001,-0.740000000000001,
-0.735000000000001,-0.730000000000001,-0.725000000000001,-0.720000000000001,
-0.715000000000001,-0.710000000000001,-0.705000000000001,-0.700000000000001,
-0.695000000000001,-0.690000000000001,-0.685,-0.68,-0.675,-0.67,-0.665,
-0.66,-0.655,-0.65,-0.645,-0.64,-0.635,-0.63,-0.625,-0.62,-0.615,-0.61,
-0.605,-0.6,-0.595,-0.59,-0.585,-0.58,-0.575,-0.57,-0.565,-0.56,-0.555,
-0.55,-0.545,-0.54,-0.535,-0.53,-0.525,-0.52,-0.515,-0.51,-0.505,-0.5,-0.495,
-0.49,-0.485,-0.48,-0.475,-0.47,-0.465,-0.46,-0.455,-0.45,-0.445,-0.44,
-0.435,-0.43,-0.425,-0.42,-0.415,-0.41,-0.405,-0.4,-0.395,-0.39,-0.385,
-0.38,-0.375,-0.37,-0.365,-0.36,-0.355,-0.35,-0.345,-0.34,-0.335,-0.33,
-0.325,-0.32,-0.315,-0.31,-0.305,-0.3,-0.295,-0.29,-0.285,-0.28,-0.275,
-0.27,-0.265,-0.26,-0.255,-0.25,-0.245,-0.24,-0.235,-0.23,-0.225,-0.22,
-0.215,-0.21,-0.205,-0.2,-0.195,-0.19,-0.185,-0.18,-0.175,-0.17,-0.165,
-0.16,-0.155,-0.15,-0.145,-0.14,-0.135,-0.13,-0.125,-0.12,-0.115,-0.11,
-0.105,-0.1,-0.095,-0.09,-0.085,-0.08,-0.075,-0.07,-0.065,-0.06,-0.055,
-0.05,-0.045,-0.04,-0.035,-0.03,-0.025,-0.02,-0.015,-0.01,-0.005,0.),
 .UNSPECIFIED.)
CURVE()
GEOMETRIC_REPRESENTATION_ITEM()
RATIONAL_B_SPLINE_CURVE((1.,1.,1.,1.,1.,1.,1.,1.,1.,1.,1.,1.,1.,1.,1.,1.,
1.,1.,1.,1.,1.,1.,1.,1.,1.,1.,1.,1.,1.,1.,1.,1.,1.,1.,1.,1.,1.,1.,1.,1.,
1.,1.,1.,1.,1.,1.,1.,1.,1.,1.,1.,1.,1.,1.,1.,1.,1.,1.,1.,1.,1.,1.,1.,1.,
1.,1.,1.,1.,1.,1.,1.,1.,1.,1.,1.,1.,1.,1.,1.,1.,1.,1.,1.,1.,1.,1.,1.,1.,
1.,1.,1.,1.,1.,1.,1.,1.,1.,1.,1.,1.,1.,1.,1.,1.,1.,1.,1.,1.,1.,1.,1.,1.,
1.,1.,1.,1.,1.,1.,1.,1.,1.,1.,1.,1.,1.,1.,1.,1.,1.,1.,1.,1.,1.,1.,1.,1.,
1.,1.,1.,1.,1.,1.,1.,1.,1.,1.,1.,1.,1.,1.,1.,1.,1.,1.,1.,1.,1.,1.,1.,1.,
1.,1.,1.,1.,1.,1.,1.,1.,1.,1.,1.,1.,1.,1.,1.,1.,1.,1.,1.,1.,1.,1.,1.,1.,
1.,1.,1.,1.,1.,1.,1.,1.,1.,1.))
REPRESENTATION_ITEM('')
);
#449=(
BOUNDED_CURVE()
B_SPLINE_CURVE(5,(#73641,#73642,#73643,#73644,#73645,#73646,#73647,#73648,
#73649,#73650,#73651,#73652,#73653,#73654,#73655,#73656,#73657,#73658,#73659,
#73660,#73661,#73662,#73663,#73664,#73665,#73666,#73667,#73668,#73669,#73670,
#73671,#73672,#73673,#73674,#73675,#73676,#73677,#73678,#73679,#73680,#73681,
#73682,#73683,#73684,#73685,#73686,#73687,#73688,#73689,#73690,#73691,#73692,
#73693,#73694,#73695,#73696,#73697,#73698,#73699,#73700,#73701,#73702,#73703,
#73704,#73705,#73706,#73707,#73708,#73709,#73710,#73711,#73712,#73713,#73714,
#73715,#73716,#73717,#73718,#73719,#73720,#73721,#73722,#73723,#73724,#73725,
#73726,#73727,#73728,#73729,#73730,#73731,#73732,#73733,#73734,#73735,#73736,
#73737,#73738,#73739,#73740,#73741,#73742,#73743,#73744,#73745,#73746,#73747,
#73748,#73749,#73750,#73751,#73752,#73753,#73754,#73755,#73756,#73757,#73758,
#73759,#73760,#73761,#73762,#73763,#73764,#73765,#73766,#73767,#73768,#73769,
#73770,#73771,#73772,#73773,#73774,#73775,#73776,#73777,#73778,#73779,#73780,
#73781,#73782,#73783,#73784,#73785,#73786,#73787,#73788,#73789,#73790,#73791,
#73792,#73793,#73794,#73795,#73796,#73797,#73798,#73799,#73800,#73801,#73802,
#73803,#73804,#73805,#73806,#73807,#73808,#73809,#73810,#73811,#73812,#73813,
#73814,#73815,#73816,#73817,#73818,#73819,#73820,#73821,#73822,#73823,#73824,
#73825,#73826,#73827,#73828,#73829,#73830,#73831,#73832,#73833,#73834),
 .UNSPECIFIED.,.F.,.F.)
B_SPLINE_CURVE_WITH_KNOTS((6,1,1,1,1,1,1,1,1,1,1,1,1,1,1,1,1,1,1,1,1,1,
1,1,1,1,1,1,1,1,1,1,1,1,1,1,1,1,1,1,1,1,1,1,1,1,1,1,1,1,1,1,1,1,1,1,1,1,
1,1,1,1,1,1,1,1,1,1,1,1,1,1,1,1,1,1,1,1,1,1,1,1,1,1,1,1,1,1,1,1,1,1,1,1,
1,1,1,1,1,1,1,1,1,1,1,1,1,1,1,1,1,1,1,1,1,1,1,1,1,1,1,1,1,1,1,1,1,1,1,1,
1,1,1,1,1,1,1,1,1,1,1,1,1,1,1,1,1,1,1,1,1,1,1,1,1,1,1,1,1,1,1,1,1,1,1,1,
1,1,1,1,1,1,1,1,1,1,1,1,1,1,1,1,1,1,1,1,1,1,1,6),(0.,0.005,0.01,0.015,0.02,
0.025,0.03,0.035,0.04,0.045,0.05,0.055,0.06,0.065,0.07,0.075,0.08,0.085,
0.09,0.095,0.1,0.105,0.11,0.115,0.12,0.125,0.13,0.135,0.14,0.145,0.15,0.155,
0.16,0.165,0.17,0.175,0.18,0.185,0.19,0.195,0.2,0.205,0.21,0.215,0.22,0.225,
0.23,0.235,0.24,0.245,0.25,0.255,0.26,0.265,0.27,0.275,0.28,0.285,0.29,
0.295,0.3,0.305,0.31,0.315,0.32,0.325,0.33,0.335,0.34,0.345,0.35,0.355,
0.36,0.365,0.37,0.375,0.38,0.385,0.39,0.395,0.4,0.405,0.41,0.415,0.42,0.425,
0.43,0.435,0.44,0.445,0.45,0.455,0.46,0.465,0.47,0.475,0.48,0.485,0.49,
0.495,0.5,0.505,0.51,0.515,0.52,0.525,0.53,0.535,0.54,0.545,0.55,0.555,
0.56,0.565,0.57,0.575,0.58,0.585,0.59,0.595,0.6,0.605,0.61,0.615,0.62,0.625,
0.63,0.635,0.64,0.645,0.65,0.655,0.66,0.665,0.67,0.675,0.68,0.685,0.690000000000001,
0.695000000000001,0.700000000000001,0.705000000000001,0.710000000000001,
0.715000000000001,0.720000000000001,0.725000000000001,0.730000000000001,
0.735000000000001,0.740000000000001,0.745000000000001,0.750000000000001,
0.755000000000001,0.760000000000001,0.765000000000001,0.770000000000001,
0.775000000000001,0.780000000000001,0.785000000000001,0.790000000000001,
0.795000000000001,0.800000000000001,0.805000000000001,0.810000000000001,
0.815000000000001,0.820000000000001,0.825000000000001,0.830000000000001,
0.835000000000001,0.840000000000001,0.845000000000001,0.850000000000001,
0.855000000000001,0.860000000000001,0.865000000000001,0.870000000000001,
0.875000000000001,0.880000000000001,0.885000000000001,0.890000000000001,
0.895000000000001,0.900000000000001,0.905000000000001,0.910000000000001,
0.915000000000001,0.920000000000001,0.925000000000001,0.930000000000001,
0.935000000000001,0.940000000000001,0.941429844431354),.UNSPECIFIED.)
CURVE()
GEOMETRIC_REPRESENTATION_ITEM()
RATIONAL_B_SPLINE_CURVE((1.,1.,1.,1.,1.,1.,1.,1.,1.,1.,1.,1.,1.,1.,1.,1.,
1.,1.,1.,1.,1.,1.,1.,1.,1.,1.,1.,1.,1.,1.,1.,1.,1.,1.,1.,1.,1.,1.,1.,1.,
1.,1.,1.,1.,1.,1.,1.,1.,1.,1.,1.,1.,1.,1.,1.,1.,1.,1.,1.,1.,1.,1.,1.,1.,
1.,1.,1.,1.,1.,1.,1.,1.,1.,1.,1.,1.,1.,1.,1.,1.,1.,1.,1.,1.,1.,1.,1.,1.,
1.,1.,1.,1.,1.,1.,1.,1.,1.,1.,1.,1.,1.,1.,1.,1.,1.,1.,1.,1.,1.,1.,1.,1.,
1.,1.,1.,1.,1.,1.,1.,1.,1.,1.,1.,1.,1.,1.,1.,1.,1.,1.,1.,1.,1.,1.,1.,1.,
1.,1.,1.,1.,1.,1.,1.,1.,1.,1.,1.,1.,1.,1.,1.,1.,1.,1.,1.,1.,1.,1.,1.,1.,
1.,1.,1.,1.,1.,1.,1.,1.,1.,1.,1.,1.,1.,1.,1.,1.,1.,1.,1.,1.,1.,1.,1.,1.,
1.,1.,1.,1.,1.,1.,1.,1.,1.,1.))
REPRESENTATION_ITEM('')
);
#450=(
BOUNDED_CURVE()
B_SPLINE_CURVE(5,(#73837,#73838,#73839,#73840,#73841,#73842,#73843,#73844,
#73845,#73846,#73847,#73848,#73849,#73850,#73851,#73852,#73853,#73854,#73855,
#73856,#73857,#73858,#73859,#73860,#73861,#73862,#73863,#73864,#73865,#73866,
#73867,#73868,#73869,#73870,#73871,#73872,#73873,#73874,#73875,#73876,#73877,
#73878,#73879,#73880,#73881,#73882,#73883,#73884,#73885,#73886,#73887,#73888,
#73889,#73890,#73891,#73892,#73893,#73894,#73895,#73896,#73897,#73898,#73899,
#73900,#73901,#73902,#73903,#73904,#73905,#73906,#73907,#73908,#73909,#73910,
#73911,#73912,#73913,#73914,#73915,#73916,#73917,#73918,#73919,#73920,#73921,
#73922,#73923,#73924,#73925,#73926,#73927,#73928,#73929,#73930,#73931,#73932,
#73933,#73934,#73935,#73936,#73937,#73938,#73939,#73940,#73941,#73942,#73943,
#73944,#73945,#73946,#73947,#73948,#73949,#73950,#73951,#73952,#73953,#73954,
#73955,#73956,#73957,#73958,#73959,#73960,#73961,#73962,#73963,#73964,#73965,
#73966,#73967,#73968,#73969,#73970,#73971,#73972,#73973,#73974,#73975,#73976,
#73977,#73978,#73979,#73980,#73981,#73982,#73983,#73984,#73985,#73986,#73987,
#73988,#73989,#73990,#73991,#73992,#73993,#73994,#73995,#73996,#73997,#73998,
#73999,#74000,#74001,#74002,#74003,#74004,#74005,#74006,#74007,#74008,#74009,
#74010,#74011,#74012,#74013,#74014,#74015,#74016,#74017,#74018,#74019,#74020,
#74021,#74022,#74023,#74024,#74025,#74026,#74027,#74028,#74029,#74030),
 .UNSPECIFIED.,.F.,.F.)
B_SPLINE_CURVE_WITH_KNOTS((6,1,1,1,1,1,1,1,1,1,1,1,1,1,1,1,1,1,1,1,1,1,
1,1,1,1,1,1,1,1,1,1,1,1,1,1,1,1,1,1,1,1,1,1,1,1,1,1,1,1,1,1,1,1,1,1,1,1,
1,1,1,1,1,1,1,1,1,1,1,1,1,1,1,1,1,1,1,1,1,1,1,1,1,1,1,1,1,1,1,1,1,1,1,1,
1,1,1,1,1,1,1,1,1,1,1,1,1,1,1,1,1,1,1,1,1,1,1,1,1,1,1,1,1,1,1,1,1,1,1,1,
1,1,1,1,1,1,1,1,1,1,1,1,1,1,1,1,1,1,1,1,1,1,1,1,1,1,1,1,1,1,1,1,1,1,1,1,
1,1,1,1,1,1,1,1,1,1,1,1,1,1,1,1,1,1,1,1,1,1,1,6),(-0.941429844431354,-0.940000000000001,
-0.935000000000001,-0.930000000000001,-0.925000000000001,-0.920000000000001,
-0.915000000000001,-0.910000000000001,-0.905000000000001,-0.900000000000001,
-0.895000000000001,-0.890000000000001,-0.885000000000001,-0.880000000000001,
-0.875000000000001,-0.870000000000001,-0.865000000000001,-0.860000000000001,
-0.855000000000001,-0.850000000000001,-0.845000000000001,-0.840000000000001,
-0.835000000000001,-0.830000000000001,-0.825000000000001,-0.820000000000001,
-0.815000000000001,-0.810000000000001,-0.805000000000001,-0.800000000000001,
-0.795000000000001,-0.790000000000001,-0.785000000000001,-0.780000000000001,
-0.775000000000001,-0.770000000000001,-0.765000000000001,-0.760000000000001,
-0.755000000000001,-0.750000000000001,-0.745000000000001,-0.740000000000001,
-0.735000000000001,-0.730000000000001,-0.725000000000001,-0.720000000000001,
-0.715000000000001,-0.710000000000001,-0.705000000000001,-0.700000000000001,
-0.695000000000001,-0.690000000000001,-0.685,-0.68,-0.675,-0.67,-0.665,
-0.66,-0.655,-0.65,-0.645,-0.64,-0.635,-0.63,-0.625,-0.62,-0.615,-0.61,
-0.605,-0.6,-0.595,-0.59,-0.585,-0.58,-0.575,-0.57,-0.565,-0.56,-0.555,
-0.55,-0.545,-0.54,-0.535,-0.53,-0.525,-0.52,-0.515,-0.51,-0.505,-0.5,-0.495,
-0.49,-0.485,-0.48,-0.475,-0.47,-0.465,-0.46,-0.455,-0.45,-0.445,-0.44,
-0.435,-0.43,-0.425,-0.42,-0.415,-0.41,-0.405,-0.4,-0.395,-0.39,-0.385,
-0.38,-0.375,-0.37,-0.365,-0.36,-0.355,-0.35,-0.345,-0.34,-0.335,-0.33,
-0.325,-0.32,-0.315,-0.31,-0.305,-0.3,-0.295,-0.29,-0.285,-0.28,-0.275,
-0.27,-0.265,-0.26,-0.255,-0.25,-0.245,-0.24,-0.235,-0.23,-0.225,-0.22,
-0.215,-0.21,-0.205,-0.2,-0.195,-0.19,-0.185,-0.18,-0.175,-0.17,-0.165,
-0.16,-0.155,-0.15,-0.145,-0.14,-0.135,-0.13,-0.125,-0.12,-0.115,-0.11,
-0.105,-0.1,-0.095,-0.09,-0.085,-0.08,-0.075,-0.07,-0.065,-0.06,-0.055,
-0.05,-0.045,-0.04,-0.035,-0.03,-0.025,-0.02,-0.015,-0.01,-0.005,0.),
 .UNSPECIFIED.)
CURVE()
GEOMETRIC_REPRESENTATION_ITEM()
RATIONAL_B_SPLINE_CURVE((1.,1.,1.,1.,1.,1.,1.,1.,1.,1.,1.,1.,1.,1.,1.,1.,
1.,1.,1.,1.,1.,1.,1.,1.,1.,1.,1.,1.,1.,1.,1.,1.,1.,1.,1.,1.,1.,1.,1.,1.,
1.,1.,1.,1.,1.,1.,1.,1.,1.,1.,1.,1.,1.,1.,1.,1.,1.,1.,1.,1.,1.,1.,1.,1.,
1.,1.,1.,1.,1.,1.,1.,1.,1.,1.,1.,1.,1.,1.,1.,1.,1.,1.,1.,1.,1.,1.,1.,1.,
1.,1.,1.,1.,1.,1.,1.,1.,1.,1.,1.,1.,1.,1.,1.,1.,1.,1.,1.,1.,1.,1.,1.,1.,
1.,1.,1.,1.,1.,1.,1.,1.,1.,1.,1.,1.,1.,1.,1.,1.,1.,1.,1.,1.,1.,1.,1.,1.,
1.,1.,1.,1.,1.,1.,1.,1.,1.,1.,1.,1.,1.,1.,1.,1.,1.,1.,1.,1.,1.,1.,1.,1.,
1.,1.,1.,1.,1.,1.,1.,1.,1.,1.,1.,1.,1.,1.,1.,1.,1.,1.,1.,1.,1.,1.,1.,1.,
1.,1.,1.,1.,1.,1.,1.,1.,1.,1.))
REPRESENTATION_ITEM('')
);
#451=(
BOUNDED_CURVE()
B_SPLINE_CURVE(5,(#74537,#74538,#74539,#74540,#74541,#74542,#74543,#74544,
#74545,#74546,#74547,#74548,#74549,#74550,#74551,#74552,#74553,#74554,#74555,
#74556,#74557,#74558,#74559,#74560,#74561,#74562,#74563,#74564,#74565,#74566,
#74567,#74568,#74569,#74570,#74571,#74572,#74573,#74574,#74575,#74576,#74577,
#74578,#74579,#74580,#74581,#74582,#74583,#74584,#74585,#74586,#74587,#74588,
#74589,#74590,#74591,#74592,#74593,#74594,#74595,#74596,#74597,#74598,#74599,
#74600,#74601,#74602,#74603,#74604,#74605,#74606,#74607,#74608,#74609,#74610,
#74611,#74612,#74613,#74614,#74615,#74616,#74617,#74618,#74619,#74620,#74621,
#74622,#74623,#74624,#74625,#74626,#74627,#74628,#74629,#74630,#74631,#74632,
#74633,#74634,#74635,#74636,#74637,#74638,#74639,#74640,#74641,#74642,#74643,
#74644,#74645,#74646,#74647,#74648,#74649,#74650,#74651,#74652,#74653,#74654,
#74655,#74656,#74657,#74658,#74659,#74660,#74661,#74662,#74663,#74664,#74665,
#74666,#74667,#74668,#74669,#74670,#74671,#74672,#74673,#74674,#74675,#74676,
#74677,#74678,#74679,#74680,#74681,#74682,#74683,#74684,#74685,#74686,#74687,
#74688,#74689,#74690,#74691,#74692,#74693,#74694,#74695,#74696,#74697,#74698,
#74699,#74700,#74701,#74702,#74703,#74704,#74705,#74706,#74707,#74708,#74709,
#74710,#74711,#74712,#74713,#74714,#74715,#74716,#74717,#74718,#74719,#74720,
#74721,#74722,#74723,#74724,#74725,#74726,#74727,#74728,#74729,#74730),
 .UNSPECIFIED.,.F.,.F.)
B_SPLINE_CURVE_WITH_KNOTS((6,1,1,1,1,1,1,1,1,1,1,1,1,1,1,1,1,1,1,1,1,1,
1,1,1,1,1,1,1,1,1,1,1,1,1,1,1,1,1,1,1,1,1,1,1,1,1,1,1,1,1,1,1,1,1,1,1,1,
1,1,1,1,1,1,1,1,1,1,1,1,1,1,1,1,1,1,1,1,1,1,1,1,1,1,1,1,1,1,1,1,1,1,1,1,
1,1,1,1,1,1,1,1,1,1,1,1,1,1,1,1,1,1,1,1,1,1,1,1,1,1,1,1,1,1,1,1,1,1,1,1,
1,1,1,1,1,1,1,1,1,1,1,1,1,1,1,1,1,1,1,1,1,1,1,1,1,1,1,1,1,1,1,1,1,1,1,1,
1,1,1,1,1,1,1,1,1,1,1,1,1,1,1,1,1,1,1,1,1,1,1,6),(0.,0.005,0.01,0.015,0.02,
0.025,0.03,0.035,0.04,0.045,0.05,0.055,0.06,0.065,0.07,0.075,0.08,0.085,
0.09,0.095,0.1,0.105,0.11,0.115,0.12,0.125,0.13,0.135,0.14,0.145,0.15,0.155,
0.16,0.165,0.17,0.175,0.18,0.185,0.19,0.195,0.2,0.205,0.21,0.215,0.22,0.225,
0.23,0.235,0.24,0.245,0.25,0.255,0.26,0.265,0.27,0.275,0.28,0.285,0.29,
0.295,0.3,0.305,0.31,0.315,0.32,0.325,0.33,0.335,0.34,0.345,0.35,0.355,
0.36,0.365,0.37,0.375,0.38,0.385,0.39,0.395,0.4,0.405,0.41,0.415,0.42,0.425,
0.43,0.435,0.44,0.445,0.45,0.455,0.46,0.465,0.47,0.475,0.48,0.485,0.49,
0.495,0.5,0.505,0.51,0.515,0.52,0.525,0.53,0.535,0.54,0.545,0.55,0.555,
0.56,0.565,0.57,0.575,0.58,0.585,0.59,0.595,0.6,0.605,0.61,0.615,0.62,0.625,
0.63,0.635,0.64,0.645,0.65,0.655,0.66,0.665,0.67,0.675,0.68,0.685,0.690000000000001,
0.695000000000001,0.700000000000001,0.705000000000001,0.710000000000001,
0.715000000000001,0.720000000000001,0.725000000000001,0.730000000000001,
0.735000000000001,0.740000000000001,0.745000000000001,0.750000000000001,
0.755000000000001,0.760000000000001,0.765000000000001,0.770000000000001,
0.775000000000001,0.780000000000001,0.785000000000001,0.790000000000001,
0.795000000000001,0.800000000000001,0.805000000000001,0.810000000000001,
0.815000000000001,0.820000000000001,0.825000000000001,0.830000000000001,
0.835000000000001,0.840000000000001,0.845000000000001,0.850000000000001,
0.855000000000001,0.860000000000001,0.865000000000001,0.870000000000001,
0.875000000000001,0.880000000000001,0.885000000000001,0.890000000000001,
0.895000000000001,0.900000000000001,0.905000000000001,0.910000000000001,
0.915000000000001,0.920000000000001,0.925000000000001,0.930000000000001,
0.935000000000001,0.940000000000001,0.94142984443138),.UNSPECIFIED.)
CURVE()
GEOMETRIC_REPRESENTATION_ITEM()
RATIONAL_B_SPLINE_CURVE((1.,1.,1.,1.,1.,1.,1.,1.,1.,1.,1.,1.,1.,1.,1.,1.,
1.,1.,1.,1.,1.,1.,1.,1.,1.,1.,1.,1.,1.,1.,1.,1.,1.,1.,1.,1.,1.,1.,1.,1.,
1.,1.,1.,1.,1.,1.,1.,1.,1.,1.,1.,1.,1.,1.,1.,1.,1.,1.,1.,1.,1.,1.,1.,1.,
1.,1.,1.,1.,1.,1.,1.,1.,1.,1.,1.,1.,1.,1.,1.,1.,1.,1.,1.,1.,1.,1.,1.,1.,
1.,1.,1.,1.,1.,1.,1.,1.,1.,1.,1.,1.,1.,1.,1.,1.,1.,1.,1.,1.,1.,1.,1.,1.,
1.,1.,1.,1.,1.,1.,1.,1.,1.,1.,1.,1.,1.,1.,1.,1.,1.,1.,1.,1.,1.,1.,1.,1.,
1.,1.,1.,1.,1.,1.,1.,1.,1.,1.,1.,1.,1.,1.,1.,1.,1.,1.,1.,1.,1.,1.,1.,1.,
1.,1.,1.,1.,1.,1.,1.,1.,1.,1.,1.,1.,1.,1.,1.,1.,1.,1.,1.,1.,1.,1.,1.,1.,
1.,1.,1.,1.,1.,1.,1.,1.,1.,1.))
REPRESENTATION_ITEM('')
);
#452=(
BOUNDED_CURVE()
B_SPLINE_CURVE(5,(#74733,#74734,#74735,#74736,#74737,#74738,#74739,#74740,
#74741,#74742,#74743,#74744,#74745,#74746,#74747,#74748,#74749,#74750,#74751,
#74752,#74753,#74754,#74755,#74756,#74757,#74758,#74759,#74760,#74761,#74762,
#74763,#74764,#74765,#74766,#74767,#74768,#74769,#74770,#74771,#74772,#74773,
#74774,#74775,#74776,#74777,#74778,#74779,#74780,#74781,#74782,#74783,#74784,
#74785,#74786,#74787,#74788,#74789,#74790,#74791,#74792,#74793,#74794,#74795,
#74796,#74797,#74798,#74799,#74800,#74801,#74802,#74803,#74804,#74805,#74806,
#74807,#74808,#74809,#74810,#74811,#74812,#74813,#74814,#74815,#74816,#74817,
#74818,#74819,#74820,#74821,#74822,#74823,#74824,#74825,#74826,#74827,#74828,
#74829,#74830,#74831,#74832,#74833,#74834,#74835,#74836,#74837,#74838,#74839,
#74840,#74841,#74842,#74843,#74844,#74845,#74846,#74847,#74848,#74849,#74850,
#74851,#74852,#74853,#74854,#74855,#74856,#74857,#74858,#74859,#74860,#74861,
#74862,#74863,#74864,#74865,#74866,#74867,#74868,#74869,#74870,#74871,#74872,
#74873,#74874,#74875,#74876,#74877,#74878,#74879,#74880,#74881,#74882,#74883,
#74884,#74885,#74886,#74887,#74888,#74889,#74890,#74891,#74892,#74893,#74894,
#74895,#74896,#74897,#74898,#74899,#74900,#74901,#74902,#74903,#74904,#74905,
#74906,#74907,#74908,#74909,#74910,#74911,#74912,#74913,#74914,#74915,#74916,
#74917,#74918,#74919,#74920,#74921,#74922,#74923,#74924,#74925,#74926),
 .UNSPECIFIED.,.F.,.F.)
B_SPLINE_CURVE_WITH_KNOTS((6,1,1,1,1,1,1,1,1,1,1,1,1,1,1,1,1,1,1,1,1,1,
1,1,1,1,1,1,1,1,1,1,1,1,1,1,1,1,1,1,1,1,1,1,1,1,1,1,1,1,1,1,1,1,1,1,1,1,
1,1,1,1,1,1,1,1,1,1,1,1,1,1,1,1,1,1,1,1,1,1,1,1,1,1,1,1,1,1,1,1,1,1,1,1,
1,1,1,1,1,1,1,1,1,1,1,1,1,1,1,1,1,1,1,1,1,1,1,1,1,1,1,1,1,1,1,1,1,1,1,1,
1,1,1,1,1,1,1,1,1,1,1,1,1,1,1,1,1,1,1,1,1,1,1,1,1,1,1,1,1,1,1,1,1,1,1,1,
1,1,1,1,1,1,1,1,1,1,1,1,1,1,1,1,1,1,1,1,1,1,1,6),(-0.941429844431407,-0.940000000000001,
-0.935000000000001,-0.930000000000001,-0.925000000000001,-0.920000000000001,
-0.915000000000001,-0.910000000000001,-0.905000000000001,-0.900000000000001,
-0.895000000000001,-0.890000000000001,-0.885000000000001,-0.880000000000001,
-0.875000000000001,-0.870000000000001,-0.865000000000001,-0.860000000000001,
-0.855000000000001,-0.850000000000001,-0.845000000000001,-0.840000000000001,
-0.835000000000001,-0.830000000000001,-0.825000000000001,-0.820000000000001,
-0.815000000000001,-0.810000000000001,-0.805000000000001,-0.800000000000001,
-0.795000000000001,-0.790000000000001,-0.785000000000001,-0.780000000000001,
-0.775000000000001,-0.770000000000001,-0.765000000000001,-0.760000000000001,
-0.755000000000001,-0.750000000000001,-0.745000000000001,-0.740000000000001,
-0.735000000000001,-0.730000000000001,-0.725000000000001,-0.720000000000001,
-0.715000000000001,-0.710000000000001,-0.705000000000001,-0.700000000000001,
-0.695000000000001,-0.690000000000001,-0.685,-0.68,-0.675,-0.67,-0.665,
-0.66,-0.655,-0.65,-0.645,-0.64,-0.635,-0.63,-0.625,-0.62,-0.615,-0.61,
-0.605,-0.6,-0.595,-0.59,-0.585,-0.58,-0.575,-0.57,-0.565,-0.56,-0.555,
-0.55,-0.545,-0.54,-0.535,-0.53,-0.525,-0.52,-0.515,-0.51,-0.505,-0.5,-0.495,
-0.49,-0.485,-0.48,-0.475,-0.47,-0.465,-0.46,-0.455,-0.45,-0.445,-0.44,
-0.435,-0.43,-0.425,-0.42,-0.415,-0.41,-0.405,-0.4,-0.395,-0.39,-0.385,
-0.38,-0.375,-0.37,-0.365,-0.36,-0.355,-0.35,-0.345,-0.34,-0.335,-0.33,
-0.325,-0.32,-0.315,-0.31,-0.305,-0.3,-0.295,-0.29,-0.285,-0.28,-0.275,
-0.27,-0.265,-0.26,-0.255,-0.25,-0.245,-0.24,-0.235,-0.23,-0.225,-0.22,
-0.215,-0.21,-0.205,-0.2,-0.195,-0.19,-0.185,-0.18,-0.175,-0.17,-0.165,
-0.16,-0.155,-0.15,-0.145,-0.14,-0.135,-0.13,-0.125,-0.12,-0.115,-0.11,
-0.105,-0.1,-0.095,-0.09,-0.085,-0.08,-0.075,-0.07,-0.065,-0.06,-0.055,
-0.05,-0.045,-0.04,-0.035,-0.03,-0.025,-0.02,-0.015,-0.01,-0.005,0.),
 .UNSPECIFIED.)
CURVE()
GEOMETRIC_REPRESENTATION_ITEM()
RATIONAL_B_SPLINE_CURVE((1.,1.,1.,1.,1.,1.,1.,1.,1.,1.,1.,1.,1.,1.,1.,1.,
1.,1.,1.,1.,1.,1.,1.,1.,1.,1.,1.,1.,1.,1.,1.,1.,1.,1.,1.,1.,1.,1.,1.,1.,
1.,1.,1.,1.,1.,1.,1.,1.,1.,1.,1.,1.,1.,1.,1.,1.,1.,1.,1.,1.,1.,1.,1.,1.,
1.,1.,1.,1.,1.,1.,1.,1.,1.,1.,1.,1.,1.,1.,1.,1.,1.,1.,1.,1.,1.,1.,1.,1.,
1.,1.,1.,1.,1.,1.,1.,1.,1.,1.,1.,1.,1.,1.,1.,1.,1.,1.,1.,1.,1.,1.,1.,1.,
1.,1.,1.,1.,1.,1.,1.,1.,1.,1.,1.,1.,1.,1.,1.,1.,1.,1.,1.,1.,1.,1.,1.,1.,
1.,1.,1.,1.,1.,1.,1.,1.,1.,1.,1.,1.,1.,1.,1.,1.,1.,1.,1.,1.,1.,1.,1.,1.,
1.,1.,1.,1.,1.,1.,1.,1.,1.,1.,1.,1.,1.,1.,1.,1.,1.,1.,1.,1.,1.,1.,1.,1.,
1.,1.,1.,1.,1.,1.,1.,1.,1.,1.))
REPRESENTATION_ITEM('')
);
#453=(
BOUNDED_CURVE()
B_SPLINE_CURVE(5,(#75433,#75434,#75435,#75436,#75437,#75438,#75439,#75440,
#75441,#75442,#75443,#75444,#75445,#75446,#75447,#75448,#75449,#75450,#75451,
#75452,#75453,#75454,#75455,#75456,#75457,#75458,#75459,#75460,#75461,#75462,
#75463,#75464,#75465,#75466,#75467,#75468,#75469,#75470,#75471,#75472,#75473,
#75474,#75475,#75476,#75477,#75478,#75479,#75480,#75481,#75482,#75483,#75484,
#75485,#75486,#75487,#75488,#75489,#75490,#75491,#75492,#75493,#75494,#75495,
#75496,#75497,#75498,#75499,#75500,#75501,#75502,#75503,#75504,#75505,#75506,
#75507,#75508,#75509,#75510,#75511,#75512,#75513,#75514,#75515,#75516,#75517,
#75518,#75519,#75520,#75521,#75522,#75523,#75524,#75525,#75526,#75527,#75528,
#75529,#75530,#75531,#75532,#75533,#75534,#75535,#75536,#75537,#75538,#75539,
#75540,#75541,#75542,#75543,#75544,#75545,#75546,#75547,#75548,#75549,#75550,
#75551,#75552,#75553,#75554,#75555,#75556,#75557,#75558,#75559,#75560,#75561,
#75562,#75563,#75564,#75565,#75566,#75567,#75568,#75569,#75570,#75571,#75572,
#75573,#75574,#75575,#75576,#75577,#75578,#75579,#75580,#75581,#75582,#75583,
#75584,#75585,#75586,#75587,#75588,#75589,#75590,#75591,#75592,#75593,#75594,
#75595,#75596,#75597,#75598,#75599,#75600,#75601,#75602,#75603,#75604,#75605,
#75606,#75607,#75608,#75609,#75610,#75611,#75612,#75613,#75614,#75615,#75616,
#75617,#75618,#75619,#75620,#75621,#75622,#75623,#75624,#75625,#75626),
 .UNSPECIFIED.,.F.,.F.)
B_SPLINE_CURVE_WITH_KNOTS((6,1,1,1,1,1,1,1,1,1,1,1,1,1,1,1,1,1,1,1,1,1,
1,1,1,1,1,1,1,1,1,1,1,1,1,1,1,1,1,1,1,1,1,1,1,1,1,1,1,1,1,1,1,1,1,1,1,1,
1,1,1,1,1,1,1,1,1,1,1,1,1,1,1,1,1,1,1,1,1,1,1,1,1,1,1,1,1,1,1,1,1,1,1,1,
1,1,1,1,1,1,1,1,1,1,1,1,1,1,1,1,1,1,1,1,1,1,1,1,1,1,1,1,1,1,1,1,1,1,1,1,
1,1,1,1,1,1,1,1,1,1,1,1,1,1,1,1,1,1,1,1,1,1,1,1,1,1,1,1,1,1,1,1,1,1,1,1,
1,1,1,1,1,1,1,1,1,1,1,1,1,1,1,1,1,1,1,1,1,1,1,6),(0.,0.005,0.01,0.015,0.02,
0.025,0.03,0.035,0.04,0.045,0.05,0.055,0.06,0.065,0.07,0.075,0.08,0.085,
0.09,0.095,0.1,0.105,0.11,0.115,0.12,0.125,0.13,0.135,0.14,0.145,0.15,0.155,
0.16,0.165,0.17,0.175,0.18,0.185,0.19,0.195,0.2,0.205,0.21,0.215,0.22,0.225,
0.23,0.235,0.24,0.245,0.25,0.255,0.26,0.265,0.27,0.275,0.28,0.285,0.29,
0.295,0.3,0.305,0.31,0.315,0.32,0.325,0.33,0.335,0.34,0.345,0.35,0.355,
0.36,0.365,0.37,0.375,0.38,0.385,0.39,0.395,0.4,0.405,0.41,0.415,0.42,0.425,
0.43,0.435,0.44,0.445,0.45,0.455,0.46,0.465,0.47,0.475,0.48,0.485,0.49,
0.495,0.5,0.505,0.51,0.515,0.52,0.525,0.53,0.535,0.54,0.545,0.55,0.555,
0.56,0.565,0.57,0.575,0.58,0.585,0.59,0.595,0.6,0.605,0.61,0.615,0.62,0.625,
0.63,0.635,0.64,0.645,0.65,0.655,0.66,0.665,0.67,0.675,0.68,0.685,0.690000000000001,
0.695000000000001,0.700000000000001,0.705000000000001,0.710000000000001,
0.715000000000001,0.720000000000001,0.725000000000001,0.730000000000001,
0.735000000000001,0.740000000000001,0.745000000000001,0.750000000000001,
0.755000000000001,0.760000000000001,0.765000000000001,0.770000000000001,
0.775000000000001,0.780000000000001,0.785000000000001,0.790000000000001,
0.795000000000001,0.800000000000001,0.805000000000001,0.810000000000001,
0.815000000000001,0.820000000000001,0.825000000000001,0.830000000000001,
0.835000000000001,0.840000000000001,0.845000000000001,0.850000000000001,
0.855000000000001,0.860000000000001,0.865000000000001,0.870000000000001,
0.875000000000001,0.880000000000001,0.885000000000001,0.890000000000001,
0.895000000000001,0.900000000000001,0.905000000000001,0.910000000000001,
0.915000000000001,0.920000000000001,0.925000000000001,0.930000000000001,
0.935000000000001,0.940000000000001,0.941429844431403),.UNSPECIFIED.)
CURVE()
GEOMETRIC_REPRESENTATION_ITEM()
RATIONAL_B_SPLINE_CURVE((1.,1.,1.,1.,1.,1.,1.,1.,1.,1.,1.,1.,1.,1.,1.,1.,
1.,1.,1.,1.,1.,1.,1.,1.,1.,1.,1.,1.,1.,1.,1.,1.,1.,1.,1.,1.,1.,1.,1.,1.,
1.,1.,1.,1.,1.,1.,1.,1.,1.,1.,1.,1.,1.,1.,1.,1.,1.,1.,1.,1.,1.,1.,1.,1.,
1.,1.,1.,1.,1.,1.,1.,1.,1.,1.,1.,1.,1.,1.,1.,1.,1.,1.,1.,1.,1.,1.,1.,1.,
1.,1.,1.,1.,1.,1.,1.,1.,1.,1.,1.,1.,1.,1.,1.,1.,1.,1.,1.,1.,1.,1.,1.,1.,
1.,1.,1.,1.,1.,1.,1.,1.,1.,1.,1.,1.,1.,1.,1.,1.,1.,1.,1.,1.,1.,1.,1.,1.,
1.,1.,1.,1.,1.,1.,1.,1.,1.,1.,1.,1.,1.,1.,1.,1.,1.,1.,1.,1.,1.,1.,1.,1.,
1.,1.,1.,1.,1.,1.,1.,1.,1.,1.,1.,1.,1.,1.,1.,1.,1.,1.,1.,1.,1.,1.,1.,1.,
1.,1.,1.,1.,1.,1.,1.,1.,1.,1.))
REPRESENTATION_ITEM('')
);
#454=(
BOUNDED_CURVE()
B_SPLINE_CURVE(5,(#75629,#75630,#75631,#75632,#75633,#75634,#75635,#75636,
#75637,#75638,#75639,#75640,#75641,#75642,#75643,#75644,#75645,#75646,#75647,
#75648,#75649,#75650,#75651,#75652,#75653,#75654,#75655,#75656,#75657,#75658,
#75659,#75660,#75661,#75662,#75663,#75664,#75665,#75666,#75667,#75668,#75669,
#75670,#75671,#75672,#75673,#75674,#75675,#75676,#75677,#75678,#75679,#75680,
#75681,#75682,#75683,#75684,#75685,#75686,#75687,#75688,#75689,#75690,#75691,
#75692,#75693,#75694,#75695,#75696,#75697,#75698,#75699,#75700,#75701,#75702,
#75703,#75704,#75705,#75706,#75707,#75708,#75709,#75710,#75711,#75712,#75713,
#75714,#75715,#75716,#75717,#75718,#75719,#75720,#75721,#75722,#75723,#75724,
#75725,#75726,#75727,#75728,#75729,#75730,#75731,#75732,#75733,#75734,#75735,
#75736,#75737,#75738,#75739,#75740,#75741,#75742,#75743,#75744,#75745,#75746,
#75747,#75748,#75749,#75750,#75751,#75752,#75753,#75754,#75755,#75756,#75757,
#75758,#75759,#75760,#75761,#75762,#75763,#75764,#75765,#75766,#75767,#75768,
#75769,#75770,#75771,#75772,#75773,#75774,#75775,#75776,#75777,#75778,#75779,
#75780,#75781,#75782,#75783,#75784,#75785,#75786,#75787,#75788,#75789,#75790,
#75791,#75792,#75793,#75794,#75795,#75796,#75797,#75798,#75799,#75800,#75801,
#75802,#75803,#75804,#75805,#75806,#75807,#75808,#75809,#75810,#75811,#75812,
#75813,#75814,#75815,#75816,#75817,#75818,#75819,#75820,#75821,#75822),
 .UNSPECIFIED.,.F.,.F.)
B_SPLINE_CURVE_WITH_KNOTS((6,1,1,1,1,1,1,1,1,1,1,1,1,1,1,1,1,1,1,1,1,1,
1,1,1,1,1,1,1,1,1,1,1,1,1,1,1,1,1,1,1,1,1,1,1,1,1,1,1,1,1,1,1,1,1,1,1,1,
1,1,1,1,1,1,1,1,1,1,1,1,1,1,1,1,1,1,1,1,1,1,1,1,1,1,1,1,1,1,1,1,1,1,1,1,
1,1,1,1,1,1,1,1,1,1,1,1,1,1,1,1,1,1,1,1,1,1,1,1,1,1,1,1,1,1,1,1,1,1,1,1,
1,1,1,1,1,1,1,1,1,1,1,1,1,1,1,1,1,1,1,1,1,1,1,1,1,1,1,1,1,1,1,1,1,1,1,1,
1,1,1,1,1,1,1,1,1,1,1,1,1,1,1,1,1,1,1,1,1,1,1,6),(-0.941429844431386,-0.940000000000001,
-0.935000000000001,-0.930000000000001,-0.925000000000001,-0.920000000000001,
-0.915000000000001,-0.910000000000001,-0.905000000000001,-0.900000000000001,
-0.895000000000001,-0.890000000000001,-0.885000000000001,-0.880000000000001,
-0.875000000000001,-0.870000000000001,-0.865000000000001,-0.860000000000001,
-0.855000000000001,-0.850000000000001,-0.845000000000001,-0.840000000000001,
-0.835000000000001,-0.830000000000001,-0.825000000000001,-0.820000000000001,
-0.815000000000001,-0.810000000000001,-0.805000000000001,-0.800000000000001,
-0.795000000000001,-0.790000000000001,-0.785000000000001,-0.780000000000001,
-0.775000000000001,-0.770000000000001,-0.765000000000001,-0.760000000000001,
-0.755000000000001,-0.750000000000001,-0.745000000000001,-0.740000000000001,
-0.735000000000001,-0.730000000000001,-0.725000000000001,-0.720000000000001,
-0.715000000000001,-0.710000000000001,-0.705000000000001,-0.700000000000001,
-0.695000000000001,-0.690000000000001,-0.685,-0.68,-0.675,-0.67,-0.665,
-0.66,-0.655,-0.65,-0.645,-0.64,-0.635,-0.63,-0.625,-0.62,-0.615,-0.61,
-0.605,-0.6,-0.595,-0.59,-0.585,-0.58,-0.575,-0.57,-0.565,-0.56,-0.555,
-0.55,-0.545,-0.54,-0.535,-0.53,-0.525,-0.52,-0.515,-0.51,-0.505,-0.5,-0.495,
-0.49,-0.485,-0.48,-0.475,-0.47,-0.465,-0.46,-0.455,-0.45,-0.445,-0.44,
-0.435,-0.43,-0.425,-0.42,-0.415,-0.41,-0.405,-0.4,-0.395,-0.39,-0.385,
-0.38,-0.375,-0.37,-0.365,-0.36,-0.355,-0.35,-0.345,-0.34,-0.335,-0.33,
-0.325,-0.32,-0.315,-0.31,-0.305,-0.3,-0.295,-0.29,-0.285,-0.28,-0.275,
-0.27,-0.265,-0.26,-0.255,-0.25,-0.245,-0.24,-0.235,-0.23,-0.225,-0.22,
-0.215,-0.21,-0.205,-0.2,-0.195,-0.19,-0.185,-0.18,-0.175,-0.17,-0.165,
-0.16,-0.155,-0.15,-0.145,-0.14,-0.135,-0.13,-0.125,-0.12,-0.115,-0.11,
-0.105,-0.1,-0.095,-0.09,-0.085,-0.08,-0.075,-0.07,-0.065,-0.06,-0.055,
-0.05,-0.045,-0.04,-0.035,-0.03,-0.025,-0.02,-0.015,-0.01,-0.005,0.),
 .UNSPECIFIED.)
CURVE()
GEOMETRIC_REPRESENTATION_ITEM()
RATIONAL_B_SPLINE_CURVE((1.,1.,1.,1.,1.,1.,1.,1.,1.,1.,1.,1.,1.,1.,1.,1.,
1.,1.,1.,1.,1.,1.,1.,1.,1.,1.,1.,1.,1.,1.,1.,1.,1.,1.,1.,1.,1.,1.,1.,1.,
1.,1.,1.,1.,1.,1.,1.,1.,1.,1.,1.,1.,1.,1.,1.,1.,1.,1.,1.,1.,1.,1.,1.,1.,
1.,1.,1.,1.,1.,1.,1.,1.,1.,1.,1.,1.,1.,1.,1.,1.,1.,1.,1.,1.,1.,1.,1.,1.,
1.,1.,1.,1.,1.,1.,1.,1.,1.,1.,1.,1.,1.,1.,1.,1.,1.,1.,1.,1.,1.,1.,1.,1.,
1.,1.,1.,1.,1.,1.,1.,1.,1.,1.,1.,1.,1.,1.,1.,1.,1.,1.,1.,1.,1.,1.,1.,1.,
1.,1.,1.,1.,1.,1.,1.,1.,1.,1.,1.,1.,1.,1.,1.,1.,1.,1.,1.,1.,1.,1.,1.,1.,
1.,1.,1.,1.,1.,1.,1.,1.,1.,1.,1.,1.,1.,1.,1.,1.,1.,1.,1.,1.,1.,1.,1.,1.,
1.,1.,1.,1.,1.,1.,1.,1.,1.,1.))
REPRESENTATION_ITEM('')
);
#455=(
BOUNDED_CURVE()
B_SPLINE_CURVE(5,(#76329,#76330,#76331,#76332,#76333,#76334,#76335,#76336,
#76337,#76338,#76339,#76340,#76341,#76342,#76343,#76344,#76345,#76346,#76347,
#76348,#76349,#76350,#76351,#76352,#76353,#76354,#76355,#76356,#76357,#76358,
#76359,#76360,#76361,#76362,#76363,#76364,#76365,#76366,#76367,#76368,#76369,
#76370,#76371,#76372,#76373,#76374,#76375,#76376,#76377,#76378,#76379,#76380,
#76381,#76382,#76383,#76384,#76385,#76386,#76387,#76388,#76389,#76390,#76391,
#76392,#76393,#76394,#76395,#76396,#76397,#76398,#76399,#76400,#76401,#76402,
#76403,#76404,#76405,#76406,#76407,#76408,#76409,#76410,#76411,#76412,#76413,
#76414,#76415,#76416,#76417,#76418,#76419,#76420,#76421,#76422,#76423,#76424,
#76425,#76426,#76427,#76428,#76429,#76430,#76431,#76432,#76433,#76434,#76435,
#76436,#76437,#76438,#76439,#76440,#76441,#76442,#76443,#76444,#76445,#76446,
#76447,#76448,#76449,#76450,#76451,#76452,#76453,#76454,#76455,#76456,#76457,
#76458,#76459,#76460,#76461,#76462,#76463,#76464,#76465,#76466,#76467,#76468,
#76469,#76470,#76471,#76472,#76473,#76474,#76475,#76476,#76477,#76478,#76479,
#76480,#76481,#76482,#76483,#76484,#76485,#76486,#76487,#76488,#76489,#76490,
#76491,#76492,#76493,#76494,#76495,#76496,#76497,#76498,#76499,#76500,#76501,
#76502,#76503,#76504,#76505,#76506,#76507,#76508,#76509,#76510,#76511,#76512,
#76513,#76514,#76515,#76516,#76517,#76518,#76519,#76520,#76521,#76522),
 .UNSPECIFIED.,.F.,.F.)
B_SPLINE_CURVE_WITH_KNOTS((6,1,1,1,1,1,1,1,1,1,1,1,1,1,1,1,1,1,1,1,1,1,
1,1,1,1,1,1,1,1,1,1,1,1,1,1,1,1,1,1,1,1,1,1,1,1,1,1,1,1,1,1,1,1,1,1,1,1,
1,1,1,1,1,1,1,1,1,1,1,1,1,1,1,1,1,1,1,1,1,1,1,1,1,1,1,1,1,1,1,1,1,1,1,1,
1,1,1,1,1,1,1,1,1,1,1,1,1,1,1,1,1,1,1,1,1,1,1,1,1,1,1,1,1,1,1,1,1,1,1,1,
1,1,1,1,1,1,1,1,1,1,1,1,1,1,1,1,1,1,1,1,1,1,1,1,1,1,1,1,1,1,1,1,1,1,1,1,
1,1,1,1,1,1,1,1,1,1,1,1,1,1,1,1,1,1,1,1,1,1,1,6),(0.,0.005,0.01,0.015,0.02,
0.025,0.03,0.035,0.04,0.045,0.05,0.055,0.06,0.065,0.07,0.075,0.08,0.085,
0.09,0.095,0.1,0.105,0.11,0.115,0.12,0.125,0.13,0.135,0.14,0.145,0.15,0.155,
0.16,0.165,0.17,0.175,0.18,0.185,0.19,0.195,0.2,0.205,0.21,0.215,0.22,0.225,
0.23,0.235,0.24,0.245,0.25,0.255,0.26,0.265,0.27,0.275,0.28,0.285,0.29,
0.295,0.3,0.305,0.31,0.315,0.32,0.325,0.33,0.335,0.34,0.345,0.35,0.355,
0.36,0.365,0.37,0.375,0.38,0.385,0.39,0.395,0.4,0.405,0.41,0.415,0.42,0.425,
0.43,0.435,0.44,0.445,0.45,0.455,0.46,0.465,0.47,0.475,0.48,0.485,0.49,
0.495,0.5,0.505,0.51,0.515,0.52,0.525,0.53,0.535,0.54,0.545,0.55,0.555,
0.56,0.565,0.57,0.575,0.58,0.585,0.59,0.595,0.6,0.605,0.61,0.615,0.62,0.625,
0.63,0.635,0.64,0.645,0.65,0.655,0.66,0.665,0.67,0.675,0.68,0.685,0.690000000000001,
0.695000000000001,0.700000000000001,0.705000000000001,0.710000000000001,
0.715000000000001,0.720000000000001,0.725000000000001,0.730000000000001,
0.735000000000001,0.740000000000001,0.745000000000001,0.750000000000001,
0.755000000000001,0.760000000000001,0.765000000000001,0.770000000000001,
0.775000000000001,0.780000000000001,0.785000000000001,0.790000000000001,
0.795000000000001,0.800000000000001,0.805000000000001,0.810000000000001,
0.815000000000001,0.820000000000001,0.825000000000001,0.830000000000001,
0.835000000000001,0.840000000000001,0.845000000000001,0.850000000000001,
0.855000000000001,0.860000000000001,0.865000000000001,0.870000000000001,
0.875000000000001,0.880000000000001,0.885000000000001,0.890000000000001,
0.895000000000001,0.900000000000001,0.905000000000001,0.910000000000001,
0.915000000000001,0.920000000000001,0.925000000000001,0.930000000000001,
0.935000000000001,0.940000000000001,0.941429844431507),.UNSPECIFIED.)
CURVE()
GEOMETRIC_REPRESENTATION_ITEM()
RATIONAL_B_SPLINE_CURVE((1.,1.,1.,1.,1.,1.,1.,1.,1.,1.,1.,1.,1.,1.,1.,1.,
1.,1.,1.,1.,1.,1.,1.,1.,1.,1.,1.,1.,1.,1.,1.,1.,1.,1.,1.,1.,1.,1.,1.,1.,
1.,1.,1.,1.,1.,1.,1.,1.,1.,1.,1.,1.,1.,1.,1.,1.,1.,1.,1.,1.,1.,1.,1.,1.,
1.,1.,1.,1.,1.,1.,1.,1.,1.,1.,1.,1.,1.,1.,1.,1.,1.,1.,1.,1.,1.,1.,1.,1.,
1.,1.,1.,1.,1.,1.,1.,1.,1.,1.,1.,1.,1.,1.,1.,1.,1.,1.,1.,1.,1.,1.,1.,1.,
1.,1.,1.,1.,1.,1.,1.,1.,1.,1.,1.,1.,1.,1.,1.,1.,1.,1.,1.,1.,1.,1.,1.,1.,
1.,1.,1.,1.,1.,1.,1.,1.,1.,1.,1.,1.,1.,1.,1.,1.,1.,1.,1.,1.,1.,1.,1.,1.,
1.,1.,1.,1.,1.,1.,1.,1.,1.,1.,1.,1.,1.,1.,1.,1.,1.,1.,1.,1.,1.,1.,1.,1.,
1.,1.,1.,1.,1.,1.,1.,1.,1.,1.))
REPRESENTATION_ITEM('')
);
#456=(
BOUNDED_CURVE()
B_SPLINE_CURVE(5,(#76525,#76526,#76527,#76528,#76529,#76530,#76531,#76532,
#76533,#76534,#76535,#76536,#76537,#76538,#76539,#76540,#76541,#76542,#76543,
#76544,#76545,#76546,#76547,#76548,#76549,#76550,#76551,#76552,#76553,#76554,
#76555,#76556,#76557,#76558,#76559,#76560,#76561,#76562,#76563,#76564,#76565,
#76566,#76567,#76568,#76569,#76570,#76571,#76572,#76573,#76574,#76575,#76576,
#76577,#76578,#76579,#76580,#76581,#76582,#76583,#76584,#76585,#76586,#76587,
#76588,#76589,#76590,#76591,#76592,#76593,#76594,#76595,#76596,#76597,#76598,
#76599,#76600,#76601,#76602,#76603,#76604,#76605,#76606,#76607,#76608,#76609,
#76610,#76611,#76612,#76613,#76614,#76615,#76616,#76617,#76618,#76619,#76620,
#76621,#76622,#76623,#76624,#76625,#76626,#76627,#76628,#76629,#76630,#76631,
#76632,#76633,#76634,#76635,#76636,#76637,#76638,#76639,#76640,#76641,#76642,
#76643,#76644,#76645,#76646,#76647,#76648,#76649,#76650,#76651,#76652,#76653,
#76654,#76655,#76656,#76657,#76658,#76659,#76660,#76661,#76662,#76663,#76664,
#76665,#76666,#76667,#76668,#76669,#76670,#76671,#76672,#76673,#76674,#76675,
#76676,#76677,#76678,#76679,#76680,#76681,#76682,#76683,#76684,#76685,#76686,
#76687,#76688,#76689,#76690,#76691,#76692,#76693,#76694,#76695,#76696,#76697,
#76698,#76699,#76700,#76701,#76702,#76703,#76704,#76705,#76706,#76707,#76708,
#76709,#76710,#76711,#76712,#76713,#76714,#76715,#76716,#76717,#76718),
 .UNSPECIFIED.,.F.,.F.)
B_SPLINE_CURVE_WITH_KNOTS((6,1,1,1,1,1,1,1,1,1,1,1,1,1,1,1,1,1,1,1,1,1,
1,1,1,1,1,1,1,1,1,1,1,1,1,1,1,1,1,1,1,1,1,1,1,1,1,1,1,1,1,1,1,1,1,1,1,1,
1,1,1,1,1,1,1,1,1,1,1,1,1,1,1,1,1,1,1,1,1,1,1,1,1,1,1,1,1,1,1,1,1,1,1,1,
1,1,1,1,1,1,1,1,1,1,1,1,1,1,1,1,1,1,1,1,1,1,1,1,1,1,1,1,1,1,1,1,1,1,1,1,
1,1,1,1,1,1,1,1,1,1,1,1,1,1,1,1,1,1,1,1,1,1,1,1,1,1,1,1,1,1,1,1,1,1,1,1,
1,1,1,1,1,1,1,1,1,1,1,1,1,1,1,1,1,1,1,1,1,1,1,6),(-0.9414298444315,-0.940000000000001,
-0.935000000000001,-0.930000000000001,-0.925000000000001,-0.920000000000001,
-0.915000000000001,-0.910000000000001,-0.905000000000001,-0.900000000000001,
-0.895000000000001,-0.890000000000001,-0.885000000000001,-0.880000000000001,
-0.875000000000001,-0.870000000000001,-0.865000000000001,-0.860000000000001,
-0.855000000000001,-0.850000000000001,-0.845000000000001,-0.840000000000001,
-0.835000000000001,-0.830000000000001,-0.825000000000001,-0.820000000000001,
-0.815000000000001,-0.810000000000001,-0.805000000000001,-0.800000000000001,
-0.795000000000001,-0.790000000000001,-0.785000000000001,-0.780000000000001,
-0.775000000000001,-0.770000000000001,-0.765000000000001,-0.760000000000001,
-0.755000000000001,-0.750000000000001,-0.745000000000001,-0.740000000000001,
-0.735000000000001,-0.730000000000001,-0.725000000000001,-0.720000000000001,
-0.715000000000001,-0.710000000000001,-0.705000000000001,-0.700000000000001,
-0.695000000000001,-0.690000000000001,-0.685,-0.68,-0.675,-0.67,-0.665,
-0.66,-0.655,-0.65,-0.645,-0.64,-0.635,-0.63,-0.625,-0.62,-0.615,-0.61,
-0.605,-0.6,-0.595,-0.59,-0.585,-0.58,-0.575,-0.57,-0.565,-0.56,-0.555,
-0.55,-0.545,-0.54,-0.535,-0.53,-0.525,-0.52,-0.515,-0.51,-0.505,-0.5,-0.495,
-0.49,-0.485,-0.48,-0.475,-0.47,-0.465,-0.46,-0.455,-0.45,-0.445,-0.44,
-0.435,-0.43,-0.425,-0.42,-0.415,-0.41,-0.405,-0.4,-0.395,-0.39,-0.385,
-0.38,-0.375,-0.37,-0.365,-0.36,-0.355,-0.35,-0.345,-0.34,-0.335,-0.33,
-0.325,-0.32,-0.315,-0.31,-0.305,-0.3,-0.295,-0.29,-0.285,-0.28,-0.275,
-0.27,-0.265,-0.26,-0.255,-0.25,-0.245,-0.24,-0.235,-0.23,-0.225,-0.22,
-0.215,-0.21,-0.205,-0.2,-0.195,-0.19,-0.185,-0.18,-0.175,-0.17,-0.165,
-0.16,-0.155,-0.15,-0.145,-0.14,-0.135,-0.13,-0.125,-0.12,-0.115,-0.11,
-0.105,-0.1,-0.095,-0.09,-0.085,-0.08,-0.075,-0.07,-0.065,-0.06,-0.055,
-0.05,-0.045,-0.04,-0.035,-0.03,-0.025,-0.02,-0.015,-0.01,-0.005,0.),
 .UNSPECIFIED.)
CURVE()
GEOMETRIC_REPRESENTATION_ITEM()
RATIONAL_B_SPLINE_CURVE((1.,1.,1.,1.,1.,1.,1.,1.,1.,1.,1.,1.,1.,1.,1.,1.,
1.,1.,1.,1.,1.,1.,1.,1.,1.,1.,1.,1.,1.,1.,1.,1.,1.,1.,1.,1.,1.,1.,1.,1.,
1.,1.,1.,1.,1.,1.,1.,1.,1.,1.,1.,1.,1.,1.,1.,1.,1.,1.,1.,1.,1.,1.,1.,1.,
1.,1.,1.,1.,1.,1.,1.,1.,1.,1.,1.,1.,1.,1.,1.,1.,1.,1.,1.,1.,1.,1.,1.,1.,
1.,1.,1.,1.,1.,1.,1.,1.,1.,1.,1.,1.,1.,1.,1.,1.,1.,1.,1.,1.,1.,1.,1.,1.,
1.,1.,1.,1.,1.,1.,1.,1.,1.,1.,1.,1.,1.,1.,1.,1.,1.,1.,1.,1.,1.,1.,1.,1.,
1.,1.,1.,1.,1.,1.,1.,1.,1.,1.,1.,1.,1.,1.,1.,1.,1.,1.,1.,1.,1.,1.,1.,1.,
1.,1.,1.,1.,1.,1.,1.,1.,1.,1.,1.,1.,1.,1.,1.,1.,1.,1.,1.,1.,1.,1.,1.,1.,
1.,1.,1.,1.,1.,1.,1.,1.,1.,1.))
REPRESENTATION_ITEM('')
);
#457=(
BOUNDED_CURVE()
B_SPLINE_CURVE(5,(#77225,#77226,#77227,#77228,#77229,#77230,#77231,#77232,
#77233,#77234,#77235,#77236,#77237,#77238,#77239,#77240,#77241,#77242,#77243,
#77244,#77245,#77246,#77247,#77248,#77249,#77250,#77251,#77252,#77253,#77254,
#77255,#77256,#77257,#77258,#77259,#77260,#77261,#77262,#77263,#77264,#77265,
#77266,#77267,#77268,#77269,#77270,#77271,#77272,#77273,#77274,#77275,#77276,
#77277,#77278,#77279,#77280,#77281,#77282,#77283,#77284,#77285,#77286,#77287,
#77288,#77289,#77290,#77291,#77292,#77293,#77294,#77295,#77296,#77297,#77298,
#77299,#77300,#77301,#77302,#77303,#77304,#77305,#77306,#77307,#77308,#77309,
#77310,#77311,#77312,#77313,#77314,#77315,#77316,#77317,#77318,#77319,#77320,
#77321,#77322,#77323,#77324,#77325,#77326,#77327,#77328,#77329,#77330,#77331,
#77332,#77333,#77334,#77335,#77336,#77337,#77338,#77339,#77340,#77341,#77342,
#77343,#77344,#77345,#77346,#77347,#77348,#77349,#77350,#77351,#77352,#77353,
#77354,#77355,#77356,#77357,#77358,#77359,#77360,#77361,#77362,#77363,#77364,
#77365,#77366,#77367,#77368,#77369,#77370,#77371,#77372,#77373,#77374,#77375,
#77376,#77377,#77378,#77379,#77380,#77381,#77382,#77383,#77384,#77385,#77386,
#77387,#77388,#77389,#77390,#77391,#77392,#77393,#77394,#77395,#77396,#77397,
#77398,#77399,#77400,#77401,#77402,#77403,#77404,#77405,#77406,#77407,#77408,
#77409,#77410,#77411,#77412,#77413,#77414,#77415,#77416,#77417,#77418),
 .UNSPECIFIED.,.F.,.F.)
B_SPLINE_CURVE_WITH_KNOTS((6,1,1,1,1,1,1,1,1,1,1,1,1,1,1,1,1,1,1,1,1,1,
1,1,1,1,1,1,1,1,1,1,1,1,1,1,1,1,1,1,1,1,1,1,1,1,1,1,1,1,1,1,1,1,1,1,1,1,
1,1,1,1,1,1,1,1,1,1,1,1,1,1,1,1,1,1,1,1,1,1,1,1,1,1,1,1,1,1,1,1,1,1,1,1,
1,1,1,1,1,1,1,1,1,1,1,1,1,1,1,1,1,1,1,1,1,1,1,1,1,1,1,1,1,1,1,1,1,1,1,1,
1,1,1,1,1,1,1,1,1,1,1,1,1,1,1,1,1,1,1,1,1,1,1,1,1,1,1,1,1,1,1,1,1,1,1,1,
1,1,1,1,1,1,1,1,1,1,1,1,1,1,1,1,1,1,1,1,1,1,1,6),(0.,0.005,0.01,0.015,0.02,
0.025,0.03,0.035,0.04,0.045,0.05,0.055,0.06,0.065,0.07,0.075,0.08,0.085,
0.09,0.095,0.1,0.105,0.11,0.115,0.12,0.125,0.13,0.135,0.14,0.145,0.15,0.155,
0.16,0.165,0.17,0.175,0.18,0.185,0.19,0.195,0.2,0.205,0.21,0.215,0.22,0.225,
0.23,0.235,0.24,0.245,0.25,0.255,0.26,0.265,0.27,0.275,0.28,0.285,0.29,
0.295,0.3,0.305,0.31,0.315,0.32,0.325,0.33,0.335,0.34,0.345,0.35,0.355,
0.36,0.365,0.37,0.375,0.38,0.385,0.39,0.395,0.4,0.405,0.41,0.415,0.42,0.425,
0.43,0.435,0.44,0.445,0.45,0.455,0.46,0.465,0.47,0.475,0.48,0.485,0.49,
0.495,0.5,0.505,0.51,0.515,0.52,0.525,0.53,0.535,0.54,0.545,0.55,0.555,
0.56,0.565,0.57,0.575,0.58,0.585,0.59,0.595,0.6,0.605,0.61,0.615,0.62,0.625,
0.63,0.635,0.64,0.645,0.65,0.655,0.66,0.665,0.67,0.675,0.68,0.685,0.690000000000001,
0.695000000000001,0.700000000000001,0.705000000000001,0.710000000000001,
0.715000000000001,0.720000000000001,0.725000000000001,0.730000000000001,
0.735000000000001,0.740000000000001,0.745000000000001,0.750000000000001,
0.755000000000001,0.760000000000001,0.765000000000001,0.770000000000001,
0.775000000000001,0.780000000000001,0.785000000000001,0.790000000000001,
0.795000000000001,0.800000000000001,0.805000000000001,0.810000000000001,
0.815000000000001,0.820000000000001,0.825000000000001,0.830000000000001,
0.835000000000001,0.840000000000001,0.845000000000001,0.850000000000001,
0.855000000000001,0.860000000000001,0.865000000000001,0.870000000000001,
0.875000000000001,0.880000000000001,0.885000000000001,0.890000000000001,
0.895000000000001,0.900000000000001,0.905000000000001,0.910000000000001,
0.915000000000001,0.920000000000001,0.925000000000001,0.930000000000001,
0.935000000000001,0.940000000000001,0.941429844431311),.UNSPECIFIED.)
CURVE()
GEOMETRIC_REPRESENTATION_ITEM()
RATIONAL_B_SPLINE_CURVE((1.,1.,1.,1.,1.,1.,1.,1.,1.,1.,1.,1.,1.,1.,1.,1.,
1.,1.,1.,1.,1.,1.,1.,1.,1.,1.,1.,1.,1.,1.,1.,1.,1.,1.,1.,1.,1.,1.,1.,1.,
1.,1.,1.,1.,1.,1.,1.,1.,1.,1.,1.,1.,1.,1.,1.,1.,1.,1.,1.,1.,1.,1.,1.,1.,
1.,1.,1.,1.,1.,1.,1.,1.,1.,1.,1.,1.,1.,1.,1.,1.,1.,1.,1.,1.,1.,1.,1.,1.,
1.,1.,1.,1.,1.,1.,1.,1.,1.,1.,1.,1.,1.,1.,1.,1.,1.,1.,1.,1.,1.,1.,1.,1.,
1.,1.,1.,1.,1.,1.,1.,1.,1.,1.,1.,1.,1.,1.,1.,1.,1.,1.,1.,1.,1.,1.,1.,1.,
1.,1.,1.,1.,1.,1.,1.,1.,1.,1.,1.,1.,1.,1.,1.,1.,1.,1.,1.,1.,1.,1.,1.,1.,
1.,1.,1.,1.,1.,1.,1.,1.,1.,1.,1.,1.,1.,1.,1.,1.,1.,1.,1.,1.,1.,1.,1.,1.,
1.,1.,1.,1.,1.,1.,1.,1.,1.,1.))
REPRESENTATION_ITEM('')
);
#458=(
BOUNDED_CURVE()
B_SPLINE_CURVE(5,(#77421,#77422,#77423,#77424,#77425,#77426,#77427,#77428,
#77429,#77430,#77431,#77432,#77433,#77434,#77435,#77436,#77437,#77438,#77439,
#77440,#77441,#77442,#77443,#77444,#77445,#77446,#77447,#77448,#77449,#77450,
#77451,#77452,#77453,#77454,#77455,#77456,#77457,#77458,#77459,#77460,#77461,
#77462,#77463,#77464,#77465,#77466,#77467,#77468,#77469,#77470,#77471,#77472,
#77473,#77474,#77475,#77476,#77477,#77478,#77479,#77480,#77481,#77482,#77483,
#77484,#77485,#77486,#77487,#77488,#77489,#77490,#77491,#77492,#77493,#77494,
#77495,#77496,#77497,#77498,#77499,#77500,#77501,#77502,#77503,#77504,#77505,
#77506,#77507,#77508,#77509,#77510,#77511,#77512,#77513,#77514,#77515,#77516,
#77517,#77518,#77519,#77520,#77521,#77522,#77523,#77524,#77525,#77526,#77527,
#77528,#77529,#77530,#77531,#77532,#77533,#77534,#77535,#77536,#77537,#77538,
#77539,#77540,#77541,#77542,#77543,#77544,#77545,#77546,#77547,#77548,#77549,
#77550,#77551,#77552,#77553,#77554,#77555,#77556,#77557,#77558,#77559,#77560,
#77561,#77562,#77563,#77564,#77565,#77566,#77567,#77568,#77569,#77570,#77571,
#77572,#77573,#77574,#77575,#77576,#77577,#77578,#77579,#77580,#77581,#77582,
#77583,#77584,#77585,#77586,#77587,#77588,#77589,#77590,#77591,#77592,#77593,
#77594,#77595,#77596,#77597,#77598,#77599,#77600,#77601,#77602,#77603,#77604,
#77605,#77606,#77607,#77608,#77609,#77610,#77611,#77612,#77613,#77614),
 .UNSPECIFIED.,.F.,.F.)
B_SPLINE_CURVE_WITH_KNOTS((6,1,1,1,1,1,1,1,1,1,1,1,1,1,1,1,1,1,1,1,1,1,
1,1,1,1,1,1,1,1,1,1,1,1,1,1,1,1,1,1,1,1,1,1,1,1,1,1,1,1,1,1,1,1,1,1,1,1,
1,1,1,1,1,1,1,1,1,1,1,1,1,1,1,1,1,1,1,1,1,1,1,1,1,1,1,1,1,1,1,1,1,1,1,1,
1,1,1,1,1,1,1,1,1,1,1,1,1,1,1,1,1,1,1,1,1,1,1,1,1,1,1,1,1,1,1,1,1,1,1,1,
1,1,1,1,1,1,1,1,1,1,1,1,1,1,1,1,1,1,1,1,1,1,1,1,1,1,1,1,1,1,1,1,1,1,1,1,
1,1,1,1,1,1,1,1,1,1,1,1,1,1,1,1,1,1,1,1,1,1,1,6),(-0.941429844431311,-0.940000000000001,
-0.935000000000001,-0.930000000000001,-0.925000000000001,-0.920000000000001,
-0.915000000000001,-0.910000000000001,-0.905000000000001,-0.900000000000001,
-0.895000000000001,-0.890000000000001,-0.885000000000001,-0.880000000000001,
-0.875000000000001,-0.870000000000001,-0.865000000000001,-0.860000000000001,
-0.855000000000001,-0.850000000000001,-0.845000000000001,-0.840000000000001,
-0.835000000000001,-0.830000000000001,-0.825000000000001,-0.820000000000001,
-0.815000000000001,-0.810000000000001,-0.805000000000001,-0.800000000000001,
-0.795000000000001,-0.790000000000001,-0.785000000000001,-0.780000000000001,
-0.775000000000001,-0.770000000000001,-0.765000000000001,-0.760000000000001,
-0.755000000000001,-0.750000000000001,-0.745000000000001,-0.740000000000001,
-0.735000000000001,-0.730000000000001,-0.725000000000001,-0.720000000000001,
-0.715000000000001,-0.710000000000001,-0.705000000000001,-0.700000000000001,
-0.695000000000001,-0.690000000000001,-0.685,-0.68,-0.675,-0.67,-0.665,
-0.66,-0.655,-0.65,-0.645,-0.64,-0.635,-0.63,-0.625,-0.62,-0.615,-0.61,
-0.605,-0.6,-0.595,-0.59,-0.585,-0.58,-0.575,-0.57,-0.565,-0.56,-0.555,
-0.55,-0.545,-0.54,-0.535,-0.53,-0.525,-0.52,-0.515,-0.51,-0.505,-0.5,-0.495,
-0.49,-0.485,-0.48,-0.475,-0.47,-0.465,-0.46,-0.455,-0.45,-0.445,-0.44,
-0.435,-0.43,-0.425,-0.42,-0.415,-0.41,-0.405,-0.4,-0.395,-0.39,-0.385,
-0.38,-0.375,-0.37,-0.365,-0.36,-0.355,-0.35,-0.345,-0.34,-0.335,-0.33,
-0.325,-0.32,-0.315,-0.31,-0.305,-0.3,-0.295,-0.29,-0.285,-0.28,-0.275,
-0.27,-0.265,-0.26,-0.255,-0.25,-0.245,-0.24,-0.235,-0.23,-0.225,-0.22,
-0.215,-0.21,-0.205,-0.2,-0.195,-0.19,-0.185,-0.18,-0.175,-0.17,-0.165,
-0.16,-0.155,-0.15,-0.145,-0.14,-0.135,-0.13,-0.125,-0.12,-0.115,-0.11,
-0.105,-0.1,-0.095,-0.09,-0.085,-0.08,-0.075,-0.07,-0.065,-0.06,-0.055,
-0.05,-0.045,-0.04,-0.035,-0.03,-0.025,-0.02,-0.015,-0.01,-0.005,0.),
 .UNSPECIFIED.)
CURVE()
GEOMETRIC_REPRESENTATION_ITEM()
RATIONAL_B_SPLINE_CURVE((1.,1.,1.,1.,1.,1.,1.,1.,1.,1.,1.,1.,1.,1.,1.,1.,
1.,1.,1.,1.,1.,1.,1.,1.,1.,1.,1.,1.,1.,1.,1.,1.,1.,1.,1.,1.,1.,1.,1.,1.,
1.,1.,1.,1.,1.,1.,1.,1.,1.,1.,1.,1.,1.,1.,1.,1.,1.,1.,1.,1.,1.,1.,1.,1.,
1.,1.,1.,1.,1.,1.,1.,1.,1.,1.,1.,1.,1.,1.,1.,1.,1.,1.,1.,1.,1.,1.,1.,1.,
1.,1.,1.,1.,1.,1.,1.,1.,1.,1.,1.,1.,1.,1.,1.,1.,1.,1.,1.,1.,1.,1.,1.,1.,
1.,1.,1.,1.,1.,1.,1.,1.,1.,1.,1.,1.,1.,1.,1.,1.,1.,1.,1.,1.,1.,1.,1.,1.,
1.,1.,1.,1.,1.,1.,1.,1.,1.,1.,1.,1.,1.,1.,1.,1.,1.,1.,1.,1.,1.,1.,1.,1.,
1.,1.,1.,1.,1.,1.,1.,1.,1.,1.,1.,1.,1.,1.,1.,1.,1.,1.,1.,1.,1.,1.,1.,1.,
1.,1.,1.,1.,1.,1.,1.,1.,1.,1.))
REPRESENTATION_ITEM('')
);
#459=(
BOUNDED_CURVE()
B_SPLINE_CURVE(5,(#78121,#78122,#78123,#78124,#78125,#78126,#78127,#78128,
#78129,#78130,#78131,#78132,#78133,#78134,#78135,#78136,#78137,#78138,#78139,
#78140,#78141,#78142,#78143,#78144,#78145,#78146,#78147,#78148,#78149,#78150,
#78151,#78152,#78153,#78154,#78155,#78156,#78157,#78158,#78159,#78160,#78161,
#78162,#78163,#78164,#78165,#78166,#78167,#78168,#78169,#78170,#78171,#78172,
#78173,#78174,#78175,#78176,#78177,#78178,#78179,#78180,#78181,#78182,#78183,
#78184,#78185,#78186,#78187,#78188,#78189,#78190,#78191,#78192,#78193,#78194,
#78195,#78196,#78197,#78198,#78199,#78200,#78201,#78202,#78203,#78204,#78205,
#78206,#78207,#78208,#78209,#78210,#78211,#78212,#78213,#78214,#78215,#78216,
#78217,#78218,#78219,#78220,#78221,#78222,#78223,#78224,#78225,#78226,#78227,
#78228,#78229,#78230,#78231,#78232,#78233,#78234,#78235,#78236,#78237,#78238,
#78239,#78240,#78241,#78242,#78243,#78244,#78245,#78246,#78247,#78248,#78249,
#78250,#78251,#78252,#78253,#78254,#78255,#78256,#78257,#78258,#78259,#78260,
#78261,#78262,#78263,#78264,#78265,#78266,#78267,#78268,#78269,#78270,#78271,
#78272,#78273,#78274,#78275,#78276,#78277,#78278,#78279,#78280,#78281,#78282,
#78283,#78284,#78285,#78286,#78287,#78288,#78289,#78290,#78291,#78292,#78293,
#78294,#78295,#78296,#78297,#78298,#78299,#78300,#78301,#78302,#78303,#78304,
#78305,#78306,#78307,#78308,#78309,#78310,#78311,#78312,#78313,#78314),
 .UNSPECIFIED.,.F.,.F.)
B_SPLINE_CURVE_WITH_KNOTS((6,1,1,1,1,1,1,1,1,1,1,1,1,1,1,1,1,1,1,1,1,1,
1,1,1,1,1,1,1,1,1,1,1,1,1,1,1,1,1,1,1,1,1,1,1,1,1,1,1,1,1,1,1,1,1,1,1,1,
1,1,1,1,1,1,1,1,1,1,1,1,1,1,1,1,1,1,1,1,1,1,1,1,1,1,1,1,1,1,1,1,1,1,1,1,
1,1,1,1,1,1,1,1,1,1,1,1,1,1,1,1,1,1,1,1,1,1,1,1,1,1,1,1,1,1,1,1,1,1,1,1,
1,1,1,1,1,1,1,1,1,1,1,1,1,1,1,1,1,1,1,1,1,1,1,1,1,1,1,1,1,1,1,1,1,1,1,1,
1,1,1,1,1,1,1,1,1,1,1,1,1,1,1,1,1,1,1,1,1,1,1,6),(0.,0.005,0.01,0.015,0.02,
0.025,0.03,0.035,0.04,0.045,0.05,0.055,0.06,0.065,0.07,0.075,0.08,0.085,
0.09,0.095,0.1,0.105,0.11,0.115,0.12,0.125,0.13,0.135,0.14,0.145,0.15,0.155,
0.16,0.165,0.17,0.175,0.18,0.185,0.19,0.195,0.2,0.205,0.21,0.215,0.22,0.225,
0.23,0.235,0.24,0.245,0.25,0.255,0.26,0.265,0.27,0.275,0.28,0.285,0.29,
0.295,0.3,0.305,0.31,0.315,0.32,0.325,0.33,0.335,0.34,0.345,0.35,0.355,
0.36,0.365,0.37,0.375,0.38,0.385,0.39,0.395,0.4,0.405,0.41,0.415,0.42,0.425,
0.43,0.435,0.44,0.445,0.45,0.455,0.46,0.465,0.47,0.475,0.48,0.485,0.49,
0.495,0.5,0.505,0.51,0.515,0.52,0.525,0.53,0.535,0.54,0.545,0.55,0.555,
0.56,0.565,0.57,0.575,0.58,0.585,0.59,0.595,0.6,0.605,0.61,0.615,0.62,0.625,
0.63,0.635,0.64,0.645,0.65,0.655,0.66,0.665,0.67,0.675,0.68,0.685,0.690000000000001,
0.695000000000001,0.700000000000001,0.705000000000001,0.710000000000001,
0.715000000000001,0.720000000000001,0.725000000000001,0.730000000000001,
0.735000000000001,0.740000000000001,0.745000000000001,0.750000000000001,
0.755000000000001,0.760000000000001,0.765000000000001,0.770000000000001,
0.775000000000001,0.780000000000001,0.785000000000001,0.790000000000001,
0.795000000000001,0.800000000000001,0.805000000000001,0.810000000000001,
0.815000000000001,0.820000000000001,0.825000000000001,0.830000000000001,
0.835000000000001,0.840000000000001,0.845000000000001,0.850000000000001,
0.855000000000001,0.860000000000001,0.865000000000001,0.870000000000001,
0.875000000000001,0.880000000000001,0.885000000000001,0.890000000000001,
0.895000000000001,0.900000000000001,0.905000000000001,0.910000000000001,
0.915000000000001,0.920000000000001,0.925000000000001,0.930000000000001,
0.935000000000001,0.940000000000001,0.94142984443127),.UNSPECIFIED.)
CURVE()
GEOMETRIC_REPRESENTATION_ITEM()
RATIONAL_B_SPLINE_CURVE((1.,1.,1.,1.,1.,1.,1.,1.,1.,1.,1.,1.,1.,1.,1.,1.,
1.,1.,1.,1.,1.,1.,1.,1.,1.,1.,1.,1.,1.,1.,1.,1.,1.,1.,1.,1.,1.,1.,1.,1.,
1.,1.,1.,1.,1.,1.,1.,1.,1.,1.,1.,1.,1.,1.,1.,1.,1.,1.,1.,1.,1.,1.,1.,1.,
1.,1.,1.,1.,1.,1.,1.,1.,1.,1.,1.,1.,1.,1.,1.,1.,1.,1.,1.,1.,1.,1.,1.,1.,
1.,1.,1.,1.,1.,1.,1.,1.,1.,1.,1.,1.,1.,1.,1.,1.,1.,1.,1.,1.,1.,1.,1.,1.,
1.,1.,1.,1.,1.,1.,1.,1.,1.,1.,1.,1.,1.,1.,1.,1.,1.,1.,1.,1.,1.,1.,1.,1.,
1.,1.,1.,1.,1.,1.,1.,1.,1.,1.,1.,1.,1.,1.,1.,1.,1.,1.,1.,1.,1.,1.,1.,1.,
1.,1.,1.,1.,1.,1.,1.,1.,1.,1.,1.,1.,1.,1.,1.,1.,1.,1.,1.,1.,1.,1.,1.,1.,
1.,1.,1.,1.,1.,1.,1.,1.,1.,1.))
REPRESENTATION_ITEM('')
);
#460=(
BOUNDED_CURVE()
B_SPLINE_CURVE(5,(#78317,#78318,#78319,#78320,#78321,#78322,#78323,#78324,
#78325,#78326,#78327,#78328,#78329,#78330,#78331,#78332,#78333,#78334,#78335,
#78336,#78337,#78338,#78339,#78340,#78341,#78342,#78343,#78344,#78345,#78346,
#78347,#78348,#78349,#78350,#78351,#78352,#78353,#78354,#78355,#78356,#78357,
#78358,#78359,#78360,#78361,#78362,#78363,#78364,#78365,#78366,#78367,#78368,
#78369,#78370,#78371,#78372,#78373,#78374,#78375,#78376,#78377,#78378,#78379,
#78380,#78381,#78382,#78383,#78384,#78385,#78386,#78387,#78388,#78389,#78390,
#78391,#78392,#78393,#78394,#78395,#78396,#78397,#78398,#78399,#78400,#78401,
#78402,#78403,#78404,#78405,#78406,#78407,#78408,#78409,#78410,#78411,#78412,
#78413,#78414,#78415,#78416,#78417,#78418,#78419,#78420,#78421,#78422,#78423,
#78424,#78425,#78426,#78427,#78428,#78429,#78430,#78431,#78432,#78433,#78434,
#78435,#78436,#78437,#78438,#78439,#78440,#78441,#78442,#78443,#78444,#78445,
#78446,#78447,#78448,#78449,#78450,#78451,#78452,#78453,#78454,#78455,#78456,
#78457,#78458,#78459,#78460,#78461,#78462,#78463,#78464,#78465,#78466,#78467,
#78468,#78469,#78470,#78471,#78472,#78473,#78474,#78475,#78476,#78477,#78478,
#78479,#78480,#78481,#78482,#78483,#78484,#78485,#78486,#78487,#78488,#78489,
#78490,#78491,#78492,#78493,#78494,#78495,#78496,#78497,#78498,#78499,#78500,
#78501,#78502,#78503,#78504,#78505,#78506,#78507,#78508,#78509,#78510),
 .UNSPECIFIED.,.F.,.F.)
B_SPLINE_CURVE_WITH_KNOTS((6,1,1,1,1,1,1,1,1,1,1,1,1,1,1,1,1,1,1,1,1,1,
1,1,1,1,1,1,1,1,1,1,1,1,1,1,1,1,1,1,1,1,1,1,1,1,1,1,1,1,1,1,1,1,1,1,1,1,
1,1,1,1,1,1,1,1,1,1,1,1,1,1,1,1,1,1,1,1,1,1,1,1,1,1,1,1,1,1,1,1,1,1,1,1,
1,1,1,1,1,1,1,1,1,1,1,1,1,1,1,1,1,1,1,1,1,1,1,1,1,1,1,1,1,1,1,1,1,1,1,1,
1,1,1,1,1,1,1,1,1,1,1,1,1,1,1,1,1,1,1,1,1,1,1,1,1,1,1,1,1,1,1,1,1,1,1,1,
1,1,1,1,1,1,1,1,1,1,1,1,1,1,1,1,1,1,1,1,1,1,1,6),(-0.941429844431257,-0.940000000000001,
-0.935000000000001,-0.930000000000001,-0.925000000000001,-0.920000000000001,
-0.915000000000001,-0.910000000000001,-0.905000000000001,-0.900000000000001,
-0.895000000000001,-0.890000000000001,-0.885000000000001,-0.880000000000001,
-0.875000000000001,-0.870000000000001,-0.865000000000001,-0.860000000000001,
-0.855000000000001,-0.850000000000001,-0.845000000000001,-0.840000000000001,
-0.835000000000001,-0.830000000000001,-0.825000000000001,-0.820000000000001,
-0.815000000000001,-0.810000000000001,-0.805000000000001,-0.800000000000001,
-0.795000000000001,-0.790000000000001,-0.785000000000001,-0.780000000000001,
-0.775000000000001,-0.770000000000001,-0.765000000000001,-0.760000000000001,
-0.755000000000001,-0.750000000000001,-0.745000000000001,-0.740000000000001,
-0.735000000000001,-0.730000000000001,-0.725000000000001,-0.720000000000001,
-0.715000000000001,-0.710000000000001,-0.705000000000001,-0.700000000000001,
-0.695000000000001,-0.690000000000001,-0.685,-0.68,-0.675,-0.67,-0.665,
-0.66,-0.655,-0.65,-0.645,-0.64,-0.635,-0.63,-0.625,-0.62,-0.615,-0.61,
-0.605,-0.6,-0.595,-0.59,-0.585,-0.58,-0.575,-0.57,-0.565,-0.56,-0.555,
-0.55,-0.545,-0.54,-0.535,-0.53,-0.525,-0.52,-0.515,-0.51,-0.505,-0.5,-0.495,
-0.49,-0.485,-0.48,-0.475,-0.47,-0.465,-0.46,-0.455,-0.45,-0.445,-0.44,
-0.435,-0.43,-0.425,-0.42,-0.415,-0.41,-0.405,-0.4,-0.395,-0.39,-0.385,
-0.38,-0.375,-0.37,-0.365,-0.36,-0.355,-0.35,-0.345,-0.34,-0.335,-0.33,
-0.325,-0.32,-0.315,-0.31,-0.305,-0.3,-0.295,-0.29,-0.285,-0.28,-0.275,
-0.27,-0.265,-0.26,-0.255,-0.25,-0.245,-0.24,-0.235,-0.23,-0.225,-0.22,
-0.215,-0.21,-0.205,-0.2,-0.195,-0.19,-0.185,-0.18,-0.175,-0.17,-0.165,
-0.16,-0.155,-0.15,-0.145,-0.14,-0.135,-0.13,-0.125,-0.12,-0.115,-0.11,
-0.105,-0.1,-0.095,-0.09,-0.085,-0.08,-0.075,-0.07,-0.065,-0.06,-0.055,
-0.05,-0.045,-0.04,-0.035,-0.03,-0.025,-0.02,-0.015,-0.01,-0.005,0.),
 .UNSPECIFIED.)
CURVE()
GEOMETRIC_REPRESENTATION_ITEM()
RATIONAL_B_SPLINE_CURVE((1.,1.,1.,1.,1.,1.,1.,1.,1.,1.,1.,1.,1.,1.,1.,1.,
1.,1.,1.,1.,1.,1.,1.,1.,1.,1.,1.,1.,1.,1.,1.,1.,1.,1.,1.,1.,1.,1.,1.,1.,
1.,1.,1.,1.,1.,1.,1.,1.,1.,1.,1.,1.,1.,1.,1.,1.,1.,1.,1.,1.,1.,1.,1.,1.,
1.,1.,1.,1.,1.,1.,1.,1.,1.,1.,1.,1.,1.,1.,1.,1.,1.,1.,1.,1.,1.,1.,1.,1.,
1.,1.,1.,1.,1.,1.,1.,1.,1.,1.,1.,1.,1.,1.,1.,1.,1.,1.,1.,1.,1.,1.,1.,1.,
1.,1.,1.,1.,1.,1.,1.,1.,1.,1.,1.,1.,1.,1.,1.,1.,1.,1.,1.,1.,1.,1.,1.,1.,
1.,1.,1.,1.,1.,1.,1.,1.,1.,1.,1.,1.,1.,1.,1.,1.,1.,1.,1.,1.,1.,1.,1.,1.,
1.,1.,1.,1.,1.,1.,1.,1.,1.,1.,1.,1.,1.,1.,1.,1.,1.,1.,1.,1.,1.,1.,1.,1.,
1.,1.,1.,1.,1.,1.,1.,1.,1.,1.))
REPRESENTATION_ITEM('')
);
#461=(
BOUNDED_CURVE()
B_SPLINE_CURVE(5,(#79017,#79018,#79019,#79020,#79021,#79022,#79023,#79024,
#79025,#79026,#79027,#79028,#79029,#79030,#79031,#79032,#79033,#79034,#79035,
#79036,#79037,#79038,#79039,#79040,#79041,#79042,#79043,#79044,#79045,#79046,
#79047,#79048,#79049,#79050,#79051,#79052,#79053,#79054,#79055,#79056,#79057,
#79058,#79059,#79060,#79061,#79062,#79063,#79064,#79065,#79066,#79067,#79068,
#79069,#79070,#79071,#79072,#79073,#79074,#79075,#79076,#79077,#79078,#79079,
#79080,#79081,#79082,#79083,#79084,#79085,#79086,#79087,#79088,#79089,#79090,
#79091,#79092,#79093,#79094,#79095,#79096,#79097,#79098,#79099,#79100,#79101,
#79102,#79103,#79104,#79105,#79106,#79107,#79108,#79109,#79110,#79111,#79112,
#79113,#79114,#79115,#79116,#79117,#79118,#79119,#79120,#79121,#79122,#79123,
#79124,#79125,#79126,#79127,#79128,#79129,#79130,#79131,#79132,#79133,#79134,
#79135,#79136,#79137,#79138,#79139,#79140,#79141,#79142,#79143,#79144,#79145,
#79146,#79147,#79148,#79149,#79150,#79151,#79152,#79153,#79154,#79155,#79156,
#79157,#79158,#79159,#79160,#79161,#79162,#79163,#79164,#79165,#79166,#79167,
#79168,#79169,#79170,#79171,#79172,#79173,#79174,#79175,#79176,#79177,#79178,
#79179,#79180,#79181,#79182,#79183,#79184,#79185,#79186,#79187,#79188,#79189,
#79190,#79191,#79192,#79193,#79194,#79195,#79196,#79197,#79198,#79199,#79200,
#79201,#79202,#79203,#79204,#79205,#79206,#79207,#79208,#79209,#79210),
 .UNSPECIFIED.,.F.,.F.)
B_SPLINE_CURVE_WITH_KNOTS((6,1,1,1,1,1,1,1,1,1,1,1,1,1,1,1,1,1,1,1,1,1,
1,1,1,1,1,1,1,1,1,1,1,1,1,1,1,1,1,1,1,1,1,1,1,1,1,1,1,1,1,1,1,1,1,1,1,1,
1,1,1,1,1,1,1,1,1,1,1,1,1,1,1,1,1,1,1,1,1,1,1,1,1,1,1,1,1,1,1,1,1,1,1,1,
1,1,1,1,1,1,1,1,1,1,1,1,1,1,1,1,1,1,1,1,1,1,1,1,1,1,1,1,1,1,1,1,1,1,1,1,
1,1,1,1,1,1,1,1,1,1,1,1,1,1,1,1,1,1,1,1,1,1,1,1,1,1,1,1,1,1,1,1,1,1,1,1,
1,1,1,1,1,1,1,1,1,1,1,1,1,1,1,1,1,1,1,1,1,1,1,6),(0.,0.005,0.01,0.015,0.02,
0.025,0.03,0.035,0.04,0.045,0.05,0.055,0.06,0.065,0.07,0.075,0.08,0.085,
0.09,0.095,0.1,0.105,0.11,0.115,0.12,0.125,0.13,0.135,0.14,0.145,0.15,0.155,
0.16,0.165,0.17,0.175,0.18,0.185,0.19,0.195,0.2,0.205,0.21,0.215,0.22,0.225,
0.23,0.235,0.24,0.245,0.25,0.255,0.26,0.265,0.27,0.275,0.28,0.285,0.29,
0.295,0.3,0.305,0.31,0.315,0.32,0.325,0.33,0.335,0.34,0.345,0.35,0.355,
0.36,0.365,0.37,0.375,0.38,0.385,0.39,0.395,0.4,0.405,0.41,0.415,0.42,0.425,
0.43,0.435,0.44,0.445,0.45,0.455,0.46,0.465,0.47,0.475,0.48,0.485,0.49,
0.495,0.5,0.505,0.51,0.515,0.52,0.525,0.53,0.535,0.54,0.545,0.55,0.555,
0.56,0.565,0.57,0.575,0.58,0.585,0.59,0.595,0.6,0.605,0.61,0.615,0.62,0.625,
0.63,0.635,0.64,0.645,0.65,0.655,0.66,0.665,0.67,0.675,0.68,0.685,0.690000000000001,
0.695000000000001,0.700000000000001,0.705000000000001,0.710000000000001,
0.715000000000001,0.720000000000001,0.725000000000001,0.730000000000001,
0.735000000000001,0.740000000000001,0.745000000000001,0.750000000000001,
0.755000000000001,0.760000000000001,0.765000000000001,0.770000000000001,
0.775000000000001,0.780000000000001,0.785000000000001,0.790000000000001,
0.795000000000001,0.800000000000001,0.805000000000001,0.810000000000001,
0.815000000000001,0.820000000000001,0.825000000000001,0.830000000000001,
0.835000000000001,0.840000000000001,0.845000000000001,0.850000000000001,
0.855000000000001,0.860000000000001,0.865000000000001,0.870000000000001,
0.875000000000001,0.880000000000001,0.885000000000001,0.890000000000001,
0.895000000000001,0.900000000000001,0.905000000000001,0.910000000000001,
0.915000000000001,0.920000000000001,0.925000000000001,0.930000000000001,
0.935000000000001,0.940000000000001,0.941429844431219),.UNSPECIFIED.)
CURVE()
GEOMETRIC_REPRESENTATION_ITEM()
RATIONAL_B_SPLINE_CURVE((1.,1.,1.,1.,1.,1.,1.,1.,1.,1.,1.,1.,1.,1.,1.,1.,
1.,1.,1.,1.,1.,1.,1.,1.,1.,1.,1.,1.,1.,1.,1.,1.,1.,1.,1.,1.,1.,1.,1.,1.,
1.,1.,1.,1.,1.,1.,1.,1.,1.,1.,1.,1.,1.,1.,1.,1.,1.,1.,1.,1.,1.,1.,1.,1.,
1.,1.,1.,1.,1.,1.,1.,1.,1.,1.,1.,1.,1.,1.,1.,1.,1.,1.,1.,1.,1.,1.,1.,1.,
1.,1.,1.,1.,1.,1.,1.,1.,1.,1.,1.,1.,1.,1.,1.,1.,1.,1.,1.,1.,1.,1.,1.,1.,
1.,1.,1.,1.,1.,1.,1.,1.,1.,1.,1.,1.,1.,1.,1.,1.,1.,1.,1.,1.,1.,1.,1.,1.,
1.,1.,1.,1.,1.,1.,1.,1.,1.,1.,1.,1.,1.,1.,1.,1.,1.,1.,1.,1.,1.,1.,1.,1.,
1.,1.,1.,1.,1.,1.,1.,1.,1.,1.,1.,1.,1.,1.,1.,1.,1.,1.,1.,1.,1.,1.,1.,1.,
1.,1.,1.,1.,1.,1.,1.,1.,1.,1.))
REPRESENTATION_ITEM('')
);
#462=(
BOUNDED_CURVE()
B_SPLINE_CURVE(5,(#79213,#79214,#79215,#79216,#79217,#79218,#79219,#79220,
#79221,#79222,#79223,#79224,#79225,#79226,#79227,#79228,#79229,#79230,#79231,
#79232,#79233,#79234,#79235,#79236,#79237,#79238,#79239,#79240,#79241,#79242,
#79243,#79244,#79245,#79246,#79247,#79248,#79249,#79250,#79251,#79252,#79253,
#79254,#79255,#79256,#79257,#79258,#79259,#79260,#79261,#79262,#79263,#79264,
#79265,#79266,#79267,#79268,#79269,#79270,#79271,#79272,#79273,#79274,#79275,
#79276,#79277,#79278,#79279,#79280,#79281,#79282,#79283,#79284,#79285,#79286,
#79287,#79288,#79289,#79290,#79291,#79292,#79293,#79294,#79295,#79296,#79297,
#79298,#79299,#79300,#79301,#79302,#79303,#79304,#79305,#79306,#79307,#79308,
#79309,#79310,#79311,#79312,#79313,#79314,#79315,#79316,#79317,#79318,#79319,
#79320,#79321,#79322,#79323,#79324,#79325,#79326,#79327,#79328,#79329,#79330,
#79331,#79332,#79333,#79334,#79335,#79336,#79337,#79338,#79339,#79340,#79341,
#79342,#79343,#79344,#79345,#79346,#79347,#79348,#79349,#79350,#79351,#79352,
#79353,#79354,#79355,#79356,#79357,#79358,#79359,#79360,#79361,#79362,#79363,
#79364,#79365,#79366,#79367,#79368,#79369,#79370,#79371,#79372,#79373,#79374,
#79375,#79376,#79377,#79378,#79379,#79380,#79381,#79382,#79383,#79384,#79385,
#79386,#79387,#79388,#79389,#79390,#79391,#79392,#79393,#79394,#79395,#79396,
#79397,#79398,#79399,#79400,#79401,#79402,#79403,#79404,#79405,#79406),
 .UNSPECIFIED.,.F.,.F.)
B_SPLINE_CURVE_WITH_KNOTS((6,1,1,1,1,1,1,1,1,1,1,1,1,1,1,1,1,1,1,1,1,1,
1,1,1,1,1,1,1,1,1,1,1,1,1,1,1,1,1,1,1,1,1,1,1,1,1,1,1,1,1,1,1,1,1,1,1,1,
1,1,1,1,1,1,1,1,1,1,1,1,1,1,1,1,1,1,1,1,1,1,1,1,1,1,1,1,1,1,1,1,1,1,1,1,
1,1,1,1,1,1,1,1,1,1,1,1,1,1,1,1,1,1,1,1,1,1,1,1,1,1,1,1,1,1,1,1,1,1,1,1,
1,1,1,1,1,1,1,1,1,1,1,1,1,1,1,1,1,1,1,1,1,1,1,1,1,1,1,1,1,1,1,1,1,1,1,1,
1,1,1,1,1,1,1,1,1,1,1,1,1,1,1,1,1,1,1,1,1,1,1,6),(-0.94142984443126,-0.940000000000001,
-0.935000000000001,-0.930000000000001,-0.925000000000001,-0.920000000000001,
-0.915000000000001,-0.910000000000001,-0.905000000000001,-0.900000000000001,
-0.895000000000001,-0.890000000000001,-0.885000000000001,-0.880000000000001,
-0.875000000000001,-0.870000000000001,-0.865000000000001,-0.860000000000001,
-0.855000000000001,-0.850000000000001,-0.845000000000001,-0.840000000000001,
-0.835000000000001,-0.830000000000001,-0.825000000000001,-0.820000000000001,
-0.815000000000001,-0.810000000000001,-0.805000000000001,-0.800000000000001,
-0.795000000000001,-0.790000000000001,-0.785000000000001,-0.780000000000001,
-0.775000000000001,-0.770000000000001,-0.765000000000001,-0.760000000000001,
-0.755000000000001,-0.750000000000001,-0.745000000000001,-0.740000000000001,
-0.735000000000001,-0.730000000000001,-0.725000000000001,-0.720000000000001,
-0.715000000000001,-0.710000000000001,-0.705000000000001,-0.700000000000001,
-0.695000000000001,-0.690000000000001,-0.685,-0.68,-0.675,-0.67,-0.665,
-0.66,-0.655,-0.65,-0.645,-0.64,-0.635,-0.63,-0.625,-0.62,-0.615,-0.61,
-0.605,-0.6,-0.595,-0.59,-0.585,-0.58,-0.575,-0.57,-0.565,-0.56,-0.555,
-0.55,-0.545,-0.54,-0.535,-0.53,-0.525,-0.52,-0.515,-0.51,-0.505,-0.5,-0.495,
-0.49,-0.485,-0.48,-0.475,-0.47,-0.465,-0.46,-0.455,-0.45,-0.445,-0.44,
-0.435,-0.43,-0.425,-0.42,-0.415,-0.41,-0.405,-0.4,-0.395,-0.39,-0.385,
-0.38,-0.375,-0.37,-0.365,-0.36,-0.355,-0.35,-0.345,-0.34,-0.335,-0.33,
-0.325,-0.32,-0.315,-0.31,-0.305,-0.3,-0.295,-0.29,-0.285,-0.28,-0.275,
-0.27,-0.265,-0.26,-0.255,-0.25,-0.245,-0.24,-0.235,-0.23,-0.225,-0.22,
-0.215,-0.21,-0.205,-0.2,-0.195,-0.19,-0.185,-0.18,-0.175,-0.17,-0.165,
-0.16,-0.155,-0.15,-0.145,-0.14,-0.135,-0.13,-0.125,-0.12,-0.115,-0.11,
-0.105,-0.1,-0.095,-0.09,-0.085,-0.08,-0.075,-0.07,-0.065,-0.06,-0.055,
-0.05,-0.045,-0.04,-0.035,-0.03,-0.025,-0.02,-0.015,-0.01,-0.005,0.),
 .UNSPECIFIED.)
CURVE()
GEOMETRIC_REPRESENTATION_ITEM()
RATIONAL_B_SPLINE_CURVE((1.,1.,1.,1.,1.,1.,1.,1.,1.,1.,1.,1.,1.,1.,1.,1.,
1.,1.,1.,1.,1.,1.,1.,1.,1.,1.,1.,1.,1.,1.,1.,1.,1.,1.,1.,1.,1.,1.,1.,1.,
1.,1.,1.,1.,1.,1.,1.,1.,1.,1.,1.,1.,1.,1.,1.,1.,1.,1.,1.,1.,1.,1.,1.,1.,
1.,1.,1.,1.,1.,1.,1.,1.,1.,1.,1.,1.,1.,1.,1.,1.,1.,1.,1.,1.,1.,1.,1.,1.,
1.,1.,1.,1.,1.,1.,1.,1.,1.,1.,1.,1.,1.,1.,1.,1.,1.,1.,1.,1.,1.,1.,1.,1.,
1.,1.,1.,1.,1.,1.,1.,1.,1.,1.,1.,1.,1.,1.,1.,1.,1.,1.,1.,1.,1.,1.,1.,1.,
1.,1.,1.,1.,1.,1.,1.,1.,1.,1.,1.,1.,1.,1.,1.,1.,1.,1.,1.,1.,1.,1.,1.,1.,
1.,1.,1.,1.,1.,1.,1.,1.,1.,1.,1.,1.,1.,1.,1.,1.,1.,1.,1.,1.,1.,1.,1.,1.,
1.,1.,1.,1.,1.,1.,1.,1.,1.,1.))
REPRESENTATION_ITEM('')
);
#463=(
BOUNDED_CURVE()
B_SPLINE_CURVE(5,(#79913,#79914,#79915,#79916,#79917,#79918,#79919,#79920,
#79921,#79922,#79923,#79924,#79925,#79926,#79927,#79928,#79929,#79930,#79931,
#79932,#79933,#79934,#79935,#79936,#79937,#79938,#79939,#79940,#79941,#79942,
#79943,#79944,#79945,#79946,#79947,#79948,#79949,#79950,#79951,#79952,#79953,
#79954,#79955,#79956,#79957,#79958,#79959,#79960,#79961,#79962,#79963,#79964,
#79965,#79966,#79967,#79968,#79969,#79970,#79971,#79972,#79973,#79974,#79975,
#79976,#79977,#79978,#79979,#79980,#79981,#79982,#79983,#79984,#79985,#79986,
#79987,#79988,#79989,#79990,#79991,#79992,#79993,#79994,#79995,#79996,#79997,
#79998,#79999,#80000,#80001,#80002,#80003,#80004,#80005,#80006,#80007,#80008,
#80009,#80010,#80011,#80012,#80013,#80014,#80015,#80016,#80017,#80018,#80019,
#80020,#80021,#80022,#80023,#80024,#80025,#80026,#80027,#80028,#80029,#80030,
#80031,#80032,#80033,#80034,#80035,#80036,#80037,#80038,#80039,#80040,#80041,
#80042,#80043,#80044,#80045,#80046,#80047,#80048,#80049,#80050,#80051,#80052,
#80053,#80054,#80055,#80056,#80057,#80058,#80059,#80060,#80061,#80062,#80063,
#80064,#80065,#80066,#80067,#80068,#80069,#80070,#80071,#80072,#80073,#80074,
#80075,#80076,#80077,#80078,#80079,#80080,#80081,#80082,#80083,#80084,#80085,
#80086,#80087,#80088,#80089,#80090,#80091,#80092,#80093,#80094,#80095,#80096,
#80097,#80098,#80099,#80100,#80101,#80102,#80103,#80104,#80105,#80106),
 .UNSPECIFIED.,.F.,.F.)
B_SPLINE_CURVE_WITH_KNOTS((6,1,1,1,1,1,1,1,1,1,1,1,1,1,1,1,1,1,1,1,1,1,
1,1,1,1,1,1,1,1,1,1,1,1,1,1,1,1,1,1,1,1,1,1,1,1,1,1,1,1,1,1,1,1,1,1,1,1,
1,1,1,1,1,1,1,1,1,1,1,1,1,1,1,1,1,1,1,1,1,1,1,1,1,1,1,1,1,1,1,1,1,1,1,1,
1,1,1,1,1,1,1,1,1,1,1,1,1,1,1,1,1,1,1,1,1,1,1,1,1,1,1,1,1,1,1,1,1,1,1,1,
1,1,1,1,1,1,1,1,1,1,1,1,1,1,1,1,1,1,1,1,1,1,1,1,1,1,1,1,1,1,1,1,1,1,1,1,
1,1,1,1,1,1,1,1,1,1,1,1,1,1,1,1,1,1,1,1,1,1,1,6),(0.,0.005,0.01,0.015,0.02,
0.025,0.03,0.035,0.04,0.045,0.05,0.055,0.06,0.065,0.07,0.075,0.08,0.085,
0.09,0.095,0.1,0.105,0.11,0.115,0.12,0.125,0.13,0.135,0.14,0.145,0.15,0.155,
0.16,0.165,0.17,0.175,0.18,0.185,0.19,0.195,0.2,0.205,0.21,0.215,0.22,0.225,
0.23,0.235,0.24,0.245,0.25,0.255,0.26,0.265,0.27,0.275,0.28,0.285,0.29,
0.295,0.3,0.305,0.31,0.315,0.32,0.325,0.33,0.335,0.34,0.345,0.35,0.355,
0.36,0.365,0.37,0.375,0.38,0.385,0.39,0.395,0.4,0.405,0.41,0.415,0.42,0.425,
0.43,0.435,0.44,0.445,0.45,0.455,0.46,0.465,0.47,0.475,0.48,0.485,0.49,
0.495,0.5,0.505,0.51,0.515,0.52,0.525,0.53,0.535,0.54,0.545,0.55,0.555,
0.56,0.565,0.57,0.575,0.58,0.585,0.59,0.595,0.6,0.605,0.61,0.615,0.62,0.625,
0.63,0.635,0.64,0.645,0.65,0.655,0.66,0.665,0.67,0.675,0.68,0.685,0.690000000000001,
0.695000000000001,0.700000000000001,0.705000000000001,0.710000000000001,
0.715000000000001,0.720000000000001,0.725000000000001,0.730000000000001,
0.735000000000001,0.740000000000001,0.745000000000001,0.750000000000001,
0.755000000000001,0.760000000000001,0.765000000000001,0.770000000000001,
0.775000000000001,0.780000000000001,0.785000000000001,0.790000000000001,
0.795000000000001,0.800000000000001,0.805000000000001,0.810000000000001,
0.815000000000001,0.820000000000001,0.825000000000001,0.830000000000001,
0.835000000000001,0.840000000000001,0.845000000000001,0.850000000000001,
0.855000000000001,0.860000000000001,0.865000000000001,0.870000000000001,
0.875000000000001,0.880000000000001,0.885000000000001,0.890000000000001,
0.895000000000001,0.900000000000001,0.905000000000001,0.910000000000001,
0.915000000000001,0.920000000000001,0.925000000000001,0.930000000000001,
0.935000000000001,0.940000000000001,0.941429844431402),.UNSPECIFIED.)
CURVE()
GEOMETRIC_REPRESENTATION_ITEM()
RATIONAL_B_SPLINE_CURVE((1.,1.,1.,1.,1.,1.,1.,1.,1.,1.,1.,1.,1.,1.,1.,1.,
1.,1.,1.,1.,1.,1.,1.,1.,1.,1.,1.,1.,1.,1.,1.,1.,1.,1.,1.,1.,1.,1.,1.,1.,
1.,1.,1.,1.,1.,1.,1.,1.,1.,1.,1.,1.,1.,1.,1.,1.,1.,1.,1.,1.,1.,1.,1.,1.,
1.,1.,1.,1.,1.,1.,1.,1.,1.,1.,1.,1.,1.,1.,1.,1.,1.,1.,1.,1.,1.,1.,1.,1.,
1.,1.,1.,1.,1.,1.,1.,1.,1.,1.,1.,1.,1.,1.,1.,1.,1.,1.,1.,1.,1.,1.,1.,1.,
1.,1.,1.,1.,1.,1.,1.,1.,1.,1.,1.,1.,1.,1.,1.,1.,1.,1.,1.,1.,1.,1.,1.,1.,
1.,1.,1.,1.,1.,1.,1.,1.,1.,1.,1.,1.,1.,1.,1.,1.,1.,1.,1.,1.,1.,1.,1.,1.,
1.,1.,1.,1.,1.,1.,1.,1.,1.,1.,1.,1.,1.,1.,1.,1.,1.,1.,1.,1.,1.,1.,1.,1.,
1.,1.,1.,1.,1.,1.,1.,1.,1.,1.))
REPRESENTATION_ITEM('')
);
#464=(
BOUNDED_CURVE()
B_SPLINE_CURVE(5,(#80109,#80110,#80111,#80112,#80113,#80114,#80115,#80116,
#80117,#80118,#80119,#80120,#80121,#80122,#80123,#80124,#80125,#80126,#80127,
#80128,#80129,#80130,#80131,#80132,#80133,#80134,#80135,#80136,#80137,#80138,
#80139,#80140,#80141,#80142,#80143,#80144,#80145,#80146,#80147,#80148,#80149,
#80150,#80151,#80152,#80153,#80154,#80155,#80156,#80157,#80158,#80159,#80160,
#80161,#80162,#80163,#80164,#80165,#80166,#80167,#80168,#80169,#80170,#80171,
#80172,#80173,#80174,#80175,#80176,#80177,#80178,#80179,#80180,#80181,#80182,
#80183,#80184,#80185,#80186,#80187,#80188,#80189,#80190,#80191,#80192,#80193,
#80194,#80195,#80196,#80197,#80198,#80199,#80200,#80201,#80202,#80203,#80204,
#80205,#80206,#80207,#80208,#80209,#80210,#80211,#80212,#80213,#80214,#80215,
#80216,#80217,#80218,#80219,#80220,#80221,#80222,#80223,#80224,#80225,#80226,
#80227,#80228,#80229,#80230,#80231,#80232,#80233,#80234,#80235,#80236,#80237,
#80238,#80239,#80240,#80241,#80242,#80243,#80244,#80245,#80246,#80247,#80248,
#80249,#80250,#80251,#80252,#80253,#80254,#80255,#80256,#80257,#80258,#80259,
#80260,#80261,#80262,#80263,#80264,#80265,#80266,#80267,#80268,#80269,#80270,
#80271,#80272,#80273,#80274,#80275,#80276,#80277,#80278,#80279,#80280,#80281,
#80282,#80283,#80284,#80285,#80286,#80287,#80288,#80289,#80290,#80291,#80292,
#80293,#80294,#80295,#80296,#80297,#80298,#80299,#80300,#80301,#80302),
 .UNSPECIFIED.,.F.,.F.)
B_SPLINE_CURVE_WITH_KNOTS((6,1,1,1,1,1,1,1,1,1,1,1,1,1,1,1,1,1,1,1,1,1,
1,1,1,1,1,1,1,1,1,1,1,1,1,1,1,1,1,1,1,1,1,1,1,1,1,1,1,1,1,1,1,1,1,1,1,1,
1,1,1,1,1,1,1,1,1,1,1,1,1,1,1,1,1,1,1,1,1,1,1,1,1,1,1,1,1,1,1,1,1,1,1,1,
1,1,1,1,1,1,1,1,1,1,1,1,1,1,1,1,1,1,1,1,1,1,1,1,1,1,1,1,1,1,1,1,1,1,1,1,
1,1,1,1,1,1,1,1,1,1,1,1,1,1,1,1,1,1,1,1,1,1,1,1,1,1,1,1,1,1,1,1,1,1,1,1,
1,1,1,1,1,1,1,1,1,1,1,1,1,1,1,1,1,1,1,1,1,1,1,6),(-0.941429844431404,-0.940000000000001,
-0.935000000000001,-0.930000000000001,-0.925000000000001,-0.920000000000001,
-0.915000000000001,-0.910000000000001,-0.905000000000001,-0.900000000000001,
-0.895000000000001,-0.890000000000001,-0.885000000000001,-0.880000000000001,
-0.875000000000001,-0.870000000000001,-0.865000000000001,-0.860000000000001,
-0.855000000000001,-0.850000000000001,-0.845000000000001,-0.840000000000001,
-0.835000000000001,-0.830000000000001,-0.825000000000001,-0.820000000000001,
-0.815000000000001,-0.810000000000001,-0.805000000000001,-0.800000000000001,
-0.795000000000001,-0.790000000000001,-0.785000000000001,-0.780000000000001,
-0.775000000000001,-0.770000000000001,-0.765000000000001,-0.760000000000001,
-0.755000000000001,-0.750000000000001,-0.745000000000001,-0.740000000000001,
-0.735000000000001,-0.730000000000001,-0.725000000000001,-0.720000000000001,
-0.715000000000001,-0.710000000000001,-0.705000000000001,-0.700000000000001,
-0.695000000000001,-0.690000000000001,-0.685,-0.68,-0.675,-0.67,-0.665,
-0.66,-0.655,-0.65,-0.645,-0.64,-0.635,-0.63,-0.625,-0.62,-0.615,-0.61,
-0.605,-0.6,-0.595,-0.59,-0.585,-0.58,-0.575,-0.57,-0.565,-0.56,-0.555,
-0.55,-0.545,-0.54,-0.535,-0.53,-0.525,-0.52,-0.515,-0.51,-0.505,-0.5,-0.495,
-0.49,-0.485,-0.48,-0.475,-0.47,-0.465,-0.46,-0.455,-0.45,-0.445,-0.44,
-0.435,-0.43,-0.425,-0.42,-0.415,-0.41,-0.405,-0.4,-0.395,-0.39,-0.385,
-0.38,-0.375,-0.37,-0.365,-0.36,-0.355,-0.35,-0.345,-0.34,-0.335,-0.33,
-0.325,-0.32,-0.315,-0.31,-0.305,-0.3,-0.295,-0.29,-0.285,-0.28,-0.275,
-0.27,-0.265,-0.26,-0.255,-0.25,-0.245,-0.24,-0.235,-0.23,-0.225,-0.22,
-0.215,-0.21,-0.205,-0.2,-0.195,-0.19,-0.185,-0.18,-0.175,-0.17,-0.165,
-0.16,-0.155,-0.15,-0.145,-0.14,-0.135,-0.13,-0.125,-0.12,-0.115,-0.11,
-0.105,-0.1,-0.095,-0.09,-0.085,-0.08,-0.075,-0.07,-0.065,-0.06,-0.055,
-0.05,-0.045,-0.04,-0.035,-0.03,-0.025,-0.02,-0.015,-0.01,-0.005,0.),
 .UNSPECIFIED.)
CURVE()
GEOMETRIC_REPRESENTATION_ITEM()
RATIONAL_B_SPLINE_CURVE((1.,1.,1.,1.,1.,1.,1.,1.,1.,1.,1.,1.,1.,1.,1.,1.,
1.,1.,1.,1.,1.,1.,1.,1.,1.,1.,1.,1.,1.,1.,1.,1.,1.,1.,1.,1.,1.,1.,1.,1.,
1.,1.,1.,1.,1.,1.,1.,1.,1.,1.,1.,1.,1.,1.,1.,1.,1.,1.,1.,1.,1.,1.,1.,1.,
1.,1.,1.,1.,1.,1.,1.,1.,1.,1.,1.,1.,1.,1.,1.,1.,1.,1.,1.,1.,1.,1.,1.,1.,
1.,1.,1.,1.,1.,1.,1.,1.,1.,1.,1.,1.,1.,1.,1.,1.,1.,1.,1.,1.,1.,1.,1.,1.,
1.,1.,1.,1.,1.,1.,1.,1.,1.,1.,1.,1.,1.,1.,1.,1.,1.,1.,1.,1.,1.,1.,1.,1.,
1.,1.,1.,1.,1.,1.,1.,1.,1.,1.,1.,1.,1.,1.,1.,1.,1.,1.,1.,1.,1.,1.,1.,1.,
1.,1.,1.,1.,1.,1.,1.,1.,1.,1.,1.,1.,1.,1.,1.,1.,1.,1.,1.,1.,1.,1.,1.,1.,
1.,1.,1.,1.,1.,1.,1.,1.,1.,1.))
REPRESENTATION_ITEM('')
);
#465=(
BOUNDED_CURVE()
B_SPLINE_CURVE(5,(#80809,#80810,#80811,#80812,#80813,#80814,#80815,#80816,
#80817,#80818,#80819,#80820,#80821,#80822,#80823,#80824,#80825,#80826,#80827,
#80828,#80829,#80830,#80831,#80832,#80833,#80834,#80835,#80836,#80837,#80838,
#80839,#80840,#80841,#80842,#80843,#80844,#80845,#80846,#80847,#80848,#80849,
#80850,#80851,#80852,#80853,#80854,#80855,#80856,#80857,#80858,#80859,#80860,
#80861,#80862,#80863,#80864,#80865,#80866,#80867,#80868,#80869,#80870,#80871,
#80872,#80873,#80874,#80875,#80876,#80877,#80878,#80879,#80880,#80881,#80882,
#80883,#80884,#80885,#80886,#80887,#80888,#80889,#80890,#80891,#80892,#80893,
#80894,#80895,#80896,#80897,#80898,#80899,#80900,#80901,#80902,#80903,#80904,
#80905,#80906,#80907,#80908,#80909,#80910,#80911,#80912,#80913,#80914,#80915,
#80916,#80917,#80918,#80919,#80920,#80921,#80922,#80923,#80924,#80925,#80926,
#80927,#80928,#80929,#80930,#80931,#80932,#80933,#80934,#80935,#80936,#80937,
#80938,#80939,#80940,#80941,#80942,#80943,#80944,#80945,#80946,#80947,#80948,
#80949,#80950,#80951,#80952,#80953,#80954,#80955,#80956,#80957,#80958,#80959,
#80960,#80961,#80962,#80963,#80964,#80965,#80966,#80967,#80968,#80969,#80970,
#80971,#80972,#80973,#80974,#80975,#80976,#80977,#80978,#80979,#80980,#80981,
#80982,#80983,#80984,#80985,#80986,#80987,#80988,#80989,#80990,#80991,#80992,
#80993,#80994,#80995,#80996,#80997,#80998,#80999,#81000,#81001,#81002),
 .UNSPECIFIED.,.F.,.F.)
B_SPLINE_CURVE_WITH_KNOTS((6,1,1,1,1,1,1,1,1,1,1,1,1,1,1,1,1,1,1,1,1,1,
1,1,1,1,1,1,1,1,1,1,1,1,1,1,1,1,1,1,1,1,1,1,1,1,1,1,1,1,1,1,1,1,1,1,1,1,
1,1,1,1,1,1,1,1,1,1,1,1,1,1,1,1,1,1,1,1,1,1,1,1,1,1,1,1,1,1,1,1,1,1,1,1,
1,1,1,1,1,1,1,1,1,1,1,1,1,1,1,1,1,1,1,1,1,1,1,1,1,1,1,1,1,1,1,1,1,1,1,1,
1,1,1,1,1,1,1,1,1,1,1,1,1,1,1,1,1,1,1,1,1,1,1,1,1,1,1,1,1,1,1,1,1,1,1,1,
1,1,1,1,1,1,1,1,1,1,1,1,1,1,1,1,1,1,1,1,1,1,1,6),(0.,0.005,0.01,0.015,0.02,
0.025,0.03,0.035,0.04,0.045,0.05,0.055,0.06,0.065,0.07,0.075,0.08,0.085,
0.09,0.095,0.1,0.105,0.11,0.115,0.12,0.125,0.13,0.135,0.14,0.145,0.15,0.155,
0.16,0.165,0.17,0.175,0.18,0.185,0.19,0.195,0.2,0.205,0.21,0.215,0.22,0.225,
0.23,0.235,0.24,0.245,0.25,0.255,0.26,0.265,0.27,0.275,0.28,0.285,0.29,
0.295,0.3,0.305,0.31,0.315,0.32,0.325,0.33,0.335,0.34,0.345,0.35,0.355,
0.36,0.365,0.37,0.375,0.38,0.385,0.39,0.395,0.4,0.405,0.41,0.415,0.42,0.425,
0.43,0.435,0.44,0.445,0.45,0.455,0.46,0.465,0.47,0.475,0.48,0.485,0.49,
0.495,0.5,0.505,0.51,0.515,0.52,0.525,0.53,0.535,0.54,0.545,0.55,0.555,
0.56,0.565,0.57,0.575,0.58,0.585,0.59,0.595,0.6,0.605,0.61,0.615,0.62,0.625,
0.63,0.635,0.64,0.645,0.65,0.655,0.66,0.665,0.67,0.675,0.68,0.685,0.690000000000001,
0.695000000000001,0.700000000000001,0.705000000000001,0.710000000000001,
0.715000000000001,0.720000000000001,0.725000000000001,0.730000000000001,
0.735000000000001,0.740000000000001,0.745000000000001,0.750000000000001,
0.755000000000001,0.760000000000001,0.765000000000001,0.770000000000001,
0.775000000000001,0.780000000000001,0.785000000000001,0.790000000000001,
0.795000000000001,0.800000000000001,0.805000000000001,0.810000000000001,
0.815000000000001,0.820000000000001,0.825000000000001,0.830000000000001,
0.835000000000001,0.840000000000001,0.845000000000001,0.850000000000001,
0.855000000000001,0.860000000000001,0.865000000000001,0.870000000000001,
0.875000000000001,0.880000000000001,0.885000000000001,0.890000000000001,
0.895000000000001,0.900000000000001,0.905000000000001,0.910000000000001,
0.915000000000001,0.920000000000001,0.925000000000001,0.930000000000001,
0.935000000000001,0.940000000000001,0.941429844431281),.UNSPECIFIED.)
CURVE()
GEOMETRIC_REPRESENTATION_ITEM()
RATIONAL_B_SPLINE_CURVE((1.,1.,1.,1.,1.,1.,1.,1.,1.,1.,1.,1.,1.,1.,1.,1.,
1.,1.,1.,1.,1.,1.,1.,1.,1.,1.,1.,1.,1.,1.,1.,1.,1.,1.,1.,1.,1.,1.,1.,1.,
1.,1.,1.,1.,1.,1.,1.,1.,1.,1.,1.,1.,1.,1.,1.,1.,1.,1.,1.,1.,1.,1.,1.,1.,
1.,1.,1.,1.,1.,1.,1.,1.,1.,1.,1.,1.,1.,1.,1.,1.,1.,1.,1.,1.,1.,1.,1.,1.,
1.,1.,1.,1.,1.,1.,1.,1.,1.,1.,1.,1.,1.,1.,1.,1.,1.,1.,1.,1.,1.,1.,1.,1.,
1.,1.,1.,1.,1.,1.,1.,1.,1.,1.,1.,1.,1.,1.,1.,1.,1.,1.,1.,1.,1.,1.,1.,1.,
1.,1.,1.,1.,1.,1.,1.,1.,1.,1.,1.,1.,1.,1.,1.,1.,1.,1.,1.,1.,1.,1.,1.,1.,
1.,1.,1.,1.,1.,1.,1.,1.,1.,1.,1.,1.,1.,1.,1.,1.,1.,1.,1.,1.,1.,1.,1.,1.,
1.,1.,1.,1.,1.,1.,1.,1.,1.,1.))
REPRESENTATION_ITEM('')
);
#466=(
BOUNDED_CURVE()
B_SPLINE_CURVE(5,(#81005,#81006,#81007,#81008,#81009,#81010,#81011,#81012,
#81013,#81014,#81015,#81016,#81017,#81018,#81019,#81020,#81021,#81022,#81023,
#81024,#81025,#81026,#81027,#81028,#81029,#81030,#81031,#81032,#81033,#81034,
#81035,#81036,#81037,#81038,#81039,#81040,#81041,#81042,#81043,#81044,#81045,
#81046,#81047,#81048,#81049,#81050,#81051,#81052,#81053,#81054,#81055,#81056,
#81057,#81058,#81059,#81060,#81061,#81062,#81063,#81064,#81065,#81066,#81067,
#81068,#81069,#81070,#81071,#81072,#81073,#81074,#81075,#81076,#81077,#81078,
#81079,#81080,#81081,#81082,#81083,#81084,#81085,#81086,#81087,#81088,#81089,
#81090,#81091,#81092,#81093,#81094,#81095,#81096,#81097,#81098,#81099,#81100,
#81101,#81102,#81103,#81104,#81105,#81106,#81107,#81108,#81109,#81110,#81111,
#81112,#81113,#81114,#81115,#81116,#81117,#81118,#81119,#81120,#81121,#81122,
#81123,#81124,#81125,#81126,#81127,#81128,#81129,#81130,#81131,#81132,#81133,
#81134,#81135,#81136,#81137,#81138,#81139,#81140,#81141,#81142,#81143,#81144,
#81145,#81146,#81147,#81148,#81149,#81150,#81151,#81152,#81153,#81154,#81155,
#81156,#81157,#81158,#81159,#81160,#81161,#81162,#81163,#81164,#81165,#81166,
#81167,#81168,#81169,#81170,#81171,#81172,#81173,#81174,#81175,#81176,#81177,
#81178,#81179,#81180,#81181,#81182,#81183,#81184,#81185,#81186,#81187,#81188,
#81189,#81190,#81191,#81192,#81193,#81194,#81195,#81196,#81197,#81198),
 .UNSPECIFIED.,.F.,.F.)
B_SPLINE_CURVE_WITH_KNOTS((6,1,1,1,1,1,1,1,1,1,1,1,1,1,1,1,1,1,1,1,1,1,
1,1,1,1,1,1,1,1,1,1,1,1,1,1,1,1,1,1,1,1,1,1,1,1,1,1,1,1,1,1,1,1,1,1,1,1,
1,1,1,1,1,1,1,1,1,1,1,1,1,1,1,1,1,1,1,1,1,1,1,1,1,1,1,1,1,1,1,1,1,1,1,1,
1,1,1,1,1,1,1,1,1,1,1,1,1,1,1,1,1,1,1,1,1,1,1,1,1,1,1,1,1,1,1,1,1,1,1,1,
1,1,1,1,1,1,1,1,1,1,1,1,1,1,1,1,1,1,1,1,1,1,1,1,1,1,1,1,1,1,1,1,1,1,1,1,
1,1,1,1,1,1,1,1,1,1,1,1,1,1,1,1,1,1,1,1,1,1,1,6),(-0.941429844431281,-0.940000000000001,
-0.935000000000001,-0.930000000000001,-0.925000000000001,-0.920000000000001,
-0.915000000000001,-0.910000000000001,-0.905000000000001,-0.900000000000001,
-0.895000000000001,-0.890000000000001,-0.885000000000001,-0.880000000000001,
-0.875000000000001,-0.870000000000001,-0.865000000000001,-0.860000000000001,
-0.855000000000001,-0.850000000000001,-0.845000000000001,-0.840000000000001,
-0.835000000000001,-0.830000000000001,-0.825000000000001,-0.820000000000001,
-0.815000000000001,-0.810000000000001,-0.805000000000001,-0.800000000000001,
-0.795000000000001,-0.790000000000001,-0.785000000000001,-0.780000000000001,
-0.775000000000001,-0.770000000000001,-0.765000000000001,-0.760000000000001,
-0.755000000000001,-0.750000000000001,-0.745000000000001,-0.740000000000001,
-0.735000000000001,-0.730000000000001,-0.725000000000001,-0.720000000000001,
-0.715000000000001,-0.710000000000001,-0.705000000000001,-0.700000000000001,
-0.695000000000001,-0.690000000000001,-0.685,-0.68,-0.675,-0.67,-0.665,
-0.66,-0.655,-0.65,-0.645,-0.64,-0.635,-0.63,-0.625,-0.62,-0.615,-0.61,
-0.605,-0.6,-0.595,-0.59,-0.585,-0.58,-0.575,-0.57,-0.565,-0.56,-0.555,
-0.55,-0.545,-0.54,-0.535,-0.53,-0.525,-0.52,-0.515,-0.51,-0.505,-0.5,-0.495,
-0.49,-0.485,-0.48,-0.475,-0.47,-0.465,-0.46,-0.455,-0.45,-0.445,-0.44,
-0.435,-0.43,-0.425,-0.42,-0.415,-0.41,-0.405,-0.4,-0.395,-0.39,-0.385,
-0.38,-0.375,-0.37,-0.365,-0.36,-0.355,-0.35,-0.345,-0.34,-0.335,-0.33,
-0.325,-0.32,-0.315,-0.31,-0.305,-0.3,-0.295,-0.29,-0.285,-0.28,-0.275,
-0.27,-0.265,-0.26,-0.255,-0.25,-0.245,-0.24,-0.235,-0.23,-0.225,-0.22,
-0.215,-0.21,-0.205,-0.2,-0.195,-0.19,-0.185,-0.18,-0.175,-0.17,-0.165,
-0.16,-0.155,-0.15,-0.145,-0.14,-0.135,-0.13,-0.125,-0.12,-0.115,-0.11,
-0.105,-0.1,-0.095,-0.09,-0.085,-0.08,-0.075,-0.07,-0.065,-0.06,-0.055,
-0.05,-0.045,-0.04,-0.035,-0.03,-0.025,-0.02,-0.015,-0.01,-0.005,0.),
 .UNSPECIFIED.)
CURVE()
GEOMETRIC_REPRESENTATION_ITEM()
RATIONAL_B_SPLINE_CURVE((1.,1.,1.,1.,1.,1.,1.,1.,1.,1.,1.,1.,1.,1.,1.,1.,
1.,1.,1.,1.,1.,1.,1.,1.,1.,1.,1.,1.,1.,1.,1.,1.,1.,1.,1.,1.,1.,1.,1.,1.,
1.,1.,1.,1.,1.,1.,1.,1.,1.,1.,1.,1.,1.,1.,1.,1.,1.,1.,1.,1.,1.,1.,1.,1.,
1.,1.,1.,1.,1.,1.,1.,1.,1.,1.,1.,1.,1.,1.,1.,1.,1.,1.,1.,1.,1.,1.,1.,1.,
1.,1.,1.,1.,1.,1.,1.,1.,1.,1.,1.,1.,1.,1.,1.,1.,1.,1.,1.,1.,1.,1.,1.,1.,
1.,1.,1.,1.,1.,1.,1.,1.,1.,1.,1.,1.,1.,1.,1.,1.,1.,1.,1.,1.,1.,1.,1.,1.,
1.,1.,1.,1.,1.,1.,1.,1.,1.,1.,1.,1.,1.,1.,1.,1.,1.,1.,1.,1.,1.,1.,1.,1.,
1.,1.,1.,1.,1.,1.,1.,1.,1.,1.,1.,1.,1.,1.,1.,1.,1.,1.,1.,1.,1.,1.,1.,1.,
1.,1.,1.,1.,1.,1.,1.,1.,1.,1.))
REPRESENTATION_ITEM('')
);
#467=(
BOUNDED_CURVE()
B_SPLINE_CURVE(5,(#81705,#81706,#81707,#81708,#81709,#81710,#81711,#81712,
#81713,#81714,#81715,#81716,#81717,#81718,#81719,#81720,#81721,#81722,#81723,
#81724,#81725,#81726,#81727,#81728,#81729,#81730,#81731,#81732,#81733,#81734,
#81735,#81736,#81737,#81738,#81739,#81740,#81741,#81742,#81743,#81744,#81745,
#81746,#81747,#81748,#81749,#81750,#81751,#81752,#81753,#81754,#81755,#81756,
#81757,#81758,#81759,#81760,#81761,#81762,#81763,#81764,#81765,#81766,#81767,
#81768,#81769,#81770,#81771,#81772,#81773,#81774,#81775,#81776,#81777,#81778,
#81779,#81780,#81781,#81782,#81783,#81784,#81785,#81786,#81787,#81788,#81789,
#81790,#81791,#81792,#81793,#81794,#81795,#81796,#81797,#81798,#81799,#81800,
#81801,#81802,#81803,#81804,#81805,#81806,#81807,#81808,#81809,#81810,#81811,
#81812,#81813,#81814,#81815,#81816,#81817,#81818,#81819,#81820,#81821,#81822,
#81823,#81824,#81825,#81826,#81827,#81828,#81829,#81830,#81831,#81832,#81833,
#81834,#81835,#81836,#81837,#81838,#81839,#81840,#81841,#81842,#81843,#81844,
#81845,#81846,#81847,#81848,#81849,#81850,#81851,#81852,#81853,#81854,#81855,
#81856,#81857,#81858,#81859,#81860,#81861,#81862,#81863,#81864,#81865,#81866,
#81867,#81868,#81869,#81870,#81871,#81872,#81873,#81874,#81875,#81876,#81877,
#81878,#81879,#81880,#81881,#81882,#81883,#81884,#81885,#81886,#81887,#81888,
#81889,#81890,#81891,#81892,#81893,#81894,#81895,#81896,#81897,#81898),
 .UNSPECIFIED.,.F.,.F.)
B_SPLINE_CURVE_WITH_KNOTS((6,1,1,1,1,1,1,1,1,1,1,1,1,1,1,1,1,1,1,1,1,1,
1,1,1,1,1,1,1,1,1,1,1,1,1,1,1,1,1,1,1,1,1,1,1,1,1,1,1,1,1,1,1,1,1,1,1,1,
1,1,1,1,1,1,1,1,1,1,1,1,1,1,1,1,1,1,1,1,1,1,1,1,1,1,1,1,1,1,1,1,1,1,1,1,
1,1,1,1,1,1,1,1,1,1,1,1,1,1,1,1,1,1,1,1,1,1,1,1,1,1,1,1,1,1,1,1,1,1,1,1,
1,1,1,1,1,1,1,1,1,1,1,1,1,1,1,1,1,1,1,1,1,1,1,1,1,1,1,1,1,1,1,1,1,1,1,1,
1,1,1,1,1,1,1,1,1,1,1,1,1,1,1,1,1,1,1,1,1,1,1,6),(0.,0.005,0.01,0.015,0.02,
0.025,0.03,0.035,0.04,0.045,0.05,0.055,0.06,0.065,0.07,0.075,0.08,0.085,
0.09,0.095,0.1,0.105,0.11,0.115,0.12,0.125,0.13,0.135,0.14,0.145,0.15,0.155,
0.16,0.165,0.17,0.175,0.18,0.185,0.19,0.195,0.2,0.205,0.21,0.215,0.22,0.225,
0.23,0.235,0.24,0.245,0.25,0.255,0.26,0.265,0.27,0.275,0.28,0.285,0.29,
0.295,0.3,0.305,0.31,0.315,0.32,0.325,0.33,0.335,0.34,0.345,0.35,0.355,
0.36,0.365,0.37,0.375,0.38,0.385,0.39,0.395,0.4,0.405,0.41,0.415,0.42,0.425,
0.43,0.435,0.44,0.445,0.45,0.455,0.46,0.465,0.47,0.475,0.48,0.485,0.49,
0.495,0.5,0.505,0.51,0.515,0.52,0.525,0.53,0.535,0.54,0.545,0.55,0.555,
0.56,0.565,0.57,0.575,0.58,0.585,0.59,0.595,0.6,0.605,0.61,0.615,0.62,0.625,
0.63,0.635,0.64,0.645,0.65,0.655,0.66,0.665,0.67,0.675,0.68,0.685,0.690000000000001,
0.695000000000001,0.700000000000001,0.705000000000001,0.710000000000001,
0.715000000000001,0.720000000000001,0.725000000000001,0.730000000000001,
0.735000000000001,0.740000000000001,0.745000000000001,0.750000000000001,
0.755000000000001,0.760000000000001,0.765000000000001,0.770000000000001,
0.775000000000001,0.780000000000001,0.785000000000001,0.790000000000001,
0.795000000000001,0.800000000000001,0.805000000000001,0.810000000000001,
0.815000000000001,0.820000000000001,0.825000000000001,0.830000000000001,
0.835000000000001,0.840000000000001,0.845000000000001,0.850000000000001,
0.855000000000001,0.860000000000001,0.865000000000001,0.870000000000001,
0.875000000000001,0.880000000000001,0.885000000000001,0.890000000000001,
0.895000000000001,0.900000000000001,0.905000000000001,0.910000000000001,
0.915000000000001,0.920000000000001,0.925000000000001,0.930000000000001,
0.935000000000001,0.940000000000001,0.941429844431456),.UNSPECIFIED.)
CURVE()
GEOMETRIC_REPRESENTATION_ITEM()
RATIONAL_B_SPLINE_CURVE((1.,1.,1.,1.,1.,1.,1.,1.,1.,1.,1.,1.,1.,1.,1.,1.,
1.,1.,1.,1.,1.,1.,1.,1.,1.,1.,1.,1.,1.,1.,1.,1.,1.,1.,1.,1.,1.,1.,1.,1.,
1.,1.,1.,1.,1.,1.,1.,1.,1.,1.,1.,1.,1.,1.,1.,1.,1.,1.,1.,1.,1.,1.,1.,1.,
1.,1.,1.,1.,1.,1.,1.,1.,1.,1.,1.,1.,1.,1.,1.,1.,1.,1.,1.,1.,1.,1.,1.,1.,
1.,1.,1.,1.,1.,1.,1.,1.,1.,1.,1.,1.,1.,1.,1.,1.,1.,1.,1.,1.,1.,1.,1.,1.,
1.,1.,1.,1.,1.,1.,1.,1.,1.,1.,1.,1.,1.,1.,1.,1.,1.,1.,1.,1.,1.,1.,1.,1.,
1.,1.,1.,1.,1.,1.,1.,1.,1.,1.,1.,1.,1.,1.,1.,1.,1.,1.,1.,1.,1.,1.,1.,1.,
1.,1.,1.,1.,1.,1.,1.,1.,1.,1.,1.,1.,1.,1.,1.,1.,1.,1.,1.,1.,1.,1.,1.,1.,
1.,1.,1.,1.,1.,1.,1.,1.,1.,1.))
REPRESENTATION_ITEM('')
);
#468=(
BOUNDED_CURVE()
B_SPLINE_CURVE(5,(#81901,#81902,#81903,#81904,#81905,#81906,#81907,#81908,
#81909,#81910,#81911,#81912,#81913,#81914,#81915,#81916,#81917,#81918,#81919,
#81920,#81921,#81922,#81923,#81924,#81925,#81926,#81927,#81928,#81929,#81930,
#81931,#81932,#81933,#81934,#81935,#81936,#81937,#81938,#81939,#81940,#81941,
#81942,#81943,#81944,#81945,#81946,#81947,#81948,#81949,#81950,#81951,#81952,
#81953,#81954,#81955,#81956,#81957,#81958,#81959,#81960,#81961,#81962,#81963,
#81964,#81965,#81966,#81967,#81968,#81969,#81970,#81971,#81972,#81973,#81974,
#81975,#81976,#81977,#81978,#81979,#81980,#81981,#81982,#81983,#81984,#81985,
#81986,#81987,#81988,#81989,#81990,#81991,#81992,#81993,#81994,#81995,#81996,
#81997,#81998,#81999,#82000,#82001,#82002,#82003,#82004,#82005,#82006,#82007,
#82008,#82009,#82010,#82011,#82012,#82013,#82014,#82015,#82016,#82017,#82018,
#82019,#82020,#82021,#82022,#82023,#82024,#82025,#82026,#82027,#82028,#82029,
#82030,#82031,#82032,#82033,#82034,#82035,#82036,#82037,#82038,#82039,#82040,
#82041,#82042,#82043,#82044,#82045,#82046,#82047,#82048,#82049,#82050,#82051,
#82052,#82053,#82054,#82055,#82056,#82057,#82058,#82059,#82060,#82061,#82062,
#82063,#82064,#82065,#82066,#82067,#82068,#82069,#82070,#82071,#82072,#82073,
#82074,#82075,#82076,#82077,#82078,#82079,#82080,#82081,#82082,#82083,#82084,
#82085,#82086,#82087,#82088,#82089,#82090,#82091,#82092,#82093,#82094),
 .UNSPECIFIED.,.F.,.F.)
B_SPLINE_CURVE_WITH_KNOTS((6,1,1,1,1,1,1,1,1,1,1,1,1,1,1,1,1,1,1,1,1,1,
1,1,1,1,1,1,1,1,1,1,1,1,1,1,1,1,1,1,1,1,1,1,1,1,1,1,1,1,1,1,1,1,1,1,1,1,
1,1,1,1,1,1,1,1,1,1,1,1,1,1,1,1,1,1,1,1,1,1,1,1,1,1,1,1,1,1,1,1,1,1,1,1,
1,1,1,1,1,1,1,1,1,1,1,1,1,1,1,1,1,1,1,1,1,1,1,1,1,1,1,1,1,1,1,1,1,1,1,1,
1,1,1,1,1,1,1,1,1,1,1,1,1,1,1,1,1,1,1,1,1,1,1,1,1,1,1,1,1,1,1,1,1,1,1,1,
1,1,1,1,1,1,1,1,1,1,1,1,1,1,1,1,1,1,1,1,1,1,1,6),(-0.941429844431454,-0.940000000000001,
-0.935000000000001,-0.930000000000001,-0.925000000000001,-0.920000000000001,
-0.915000000000001,-0.910000000000001,-0.905000000000001,-0.900000000000001,
-0.895000000000001,-0.890000000000001,-0.885000000000001,-0.880000000000001,
-0.875000000000001,-0.870000000000001,-0.865000000000001,-0.860000000000001,
-0.855000000000001,-0.850000000000001,-0.845000000000001,-0.840000000000001,
-0.835000000000001,-0.830000000000001,-0.825000000000001,-0.820000000000001,
-0.815000000000001,-0.810000000000001,-0.805000000000001,-0.800000000000001,
-0.795000000000001,-0.790000000000001,-0.785000000000001,-0.780000000000001,
-0.775000000000001,-0.770000000000001,-0.765000000000001,-0.760000000000001,
-0.755000000000001,-0.750000000000001,-0.745000000000001,-0.740000000000001,
-0.735000000000001,-0.730000000000001,-0.725000000000001,-0.720000000000001,
-0.715000000000001,-0.710000000000001,-0.705000000000001,-0.700000000000001,
-0.695000000000001,-0.690000000000001,-0.685,-0.68,-0.675,-0.67,-0.665,
-0.66,-0.655,-0.65,-0.645,-0.64,-0.635,-0.63,-0.625,-0.62,-0.615,-0.61,
-0.605,-0.6,-0.595,-0.59,-0.585,-0.58,-0.575,-0.57,-0.565,-0.56,-0.555,
-0.55,-0.545,-0.54,-0.535,-0.53,-0.525,-0.52,-0.515,-0.51,-0.505,-0.5,-0.495,
-0.49,-0.485,-0.48,-0.475,-0.47,-0.465,-0.46,-0.455,-0.45,-0.445,-0.44,
-0.435,-0.43,-0.425,-0.42,-0.415,-0.41,-0.405,-0.4,-0.395,-0.39,-0.385,
-0.38,-0.375,-0.37,-0.365,-0.36,-0.355,-0.35,-0.345,-0.34,-0.335,-0.33,
-0.325,-0.32,-0.315,-0.31,-0.305,-0.3,-0.295,-0.29,-0.285,-0.28,-0.275,
-0.27,-0.265,-0.26,-0.255,-0.25,-0.245,-0.24,-0.235,-0.23,-0.225,-0.22,
-0.215,-0.21,-0.205,-0.2,-0.195,-0.19,-0.185,-0.18,-0.175,-0.17,-0.165,
-0.16,-0.155,-0.15,-0.145,-0.14,-0.135,-0.13,-0.125,-0.12,-0.115,-0.11,
-0.105,-0.1,-0.095,-0.09,-0.085,-0.08,-0.075,-0.07,-0.065,-0.06,-0.055,
-0.05,-0.045,-0.04,-0.035,-0.03,-0.025,-0.02,-0.015,-0.01,-0.005,0.),
 .UNSPECIFIED.)
CURVE()
GEOMETRIC_REPRESENTATION_ITEM()
RATIONAL_B_SPLINE_CURVE((1.,1.,1.,1.,1.,1.,1.,1.,1.,1.,1.,1.,1.,1.,1.,1.,
1.,1.,1.,1.,1.,1.,1.,1.,1.,1.,1.,1.,1.,1.,1.,1.,1.,1.,1.,1.,1.,1.,1.,1.,
1.,1.,1.,1.,1.,1.,1.,1.,1.,1.,1.,1.,1.,1.,1.,1.,1.,1.,1.,1.,1.,1.,1.,1.,
1.,1.,1.,1.,1.,1.,1.,1.,1.,1.,1.,1.,1.,1.,1.,1.,1.,1.,1.,1.,1.,1.,1.,1.,
1.,1.,1.,1.,1.,1.,1.,1.,1.,1.,1.,1.,1.,1.,1.,1.,1.,1.,1.,1.,1.,1.,1.,1.,
1.,1.,1.,1.,1.,1.,1.,1.,1.,1.,1.,1.,1.,1.,1.,1.,1.,1.,1.,1.,1.,1.,1.,1.,
1.,1.,1.,1.,1.,1.,1.,1.,1.,1.,1.,1.,1.,1.,1.,1.,1.,1.,1.,1.,1.,1.,1.,1.,
1.,1.,1.,1.,1.,1.,1.,1.,1.,1.,1.,1.,1.,1.,1.,1.,1.,1.,1.,1.,1.,1.,1.,1.,
1.,1.,1.,1.,1.,1.,1.,1.,1.,1.))
REPRESENTATION_ITEM('')
);
#469=(
BOUNDED_CURVE()
B_SPLINE_CURVE(5,(#82601,#82602,#82603,#82604,#82605,#82606,#82607,#82608,
#82609,#82610,#82611,#82612,#82613,#82614,#82615,#82616,#82617,#82618,#82619,
#82620,#82621,#82622,#82623,#82624,#82625,#82626,#82627,#82628,#82629,#82630,
#82631,#82632,#82633,#82634,#82635,#82636,#82637,#82638,#82639,#82640,#82641,
#82642,#82643,#82644,#82645,#82646,#82647,#82648,#82649,#82650,#82651,#82652,
#82653,#82654,#82655,#82656,#82657,#82658,#82659,#82660,#82661,#82662,#82663,
#82664,#82665,#82666,#82667,#82668,#82669,#82670,#82671,#82672,#82673,#82674,
#82675,#82676,#82677,#82678,#82679,#82680,#82681,#82682,#82683,#82684,#82685,
#82686,#82687,#82688,#82689,#82690,#82691,#82692,#82693,#82694,#82695,#82696,
#82697,#82698,#82699,#82700,#82701,#82702,#82703,#82704,#82705,#82706,#82707,
#82708,#82709,#82710,#82711,#82712,#82713,#82714,#82715,#82716,#82717,#82718,
#82719,#82720,#82721,#82722,#82723,#82724,#82725,#82726,#82727,#82728,#82729,
#82730,#82731,#82732,#82733,#82734,#82735,#82736,#82737,#82738,#82739,#82740,
#82741,#82742,#82743,#82744,#82745,#82746,#82747,#82748,#82749,#82750,#82751,
#82752,#82753,#82754,#82755,#82756,#82757,#82758,#82759,#82760,#82761,#82762,
#82763,#82764,#82765,#82766,#82767,#82768,#82769,#82770,#82771,#82772,#82773,
#82774,#82775,#82776,#82777,#82778,#82779,#82780,#82781,#82782,#82783,#82784,
#82785,#82786,#82787,#82788,#82789,#82790,#82791,#82792,#82793,#82794),
 .UNSPECIFIED.,.F.,.F.)
B_SPLINE_CURVE_WITH_KNOTS((6,1,1,1,1,1,1,1,1,1,1,1,1,1,1,1,1,1,1,1,1,1,
1,1,1,1,1,1,1,1,1,1,1,1,1,1,1,1,1,1,1,1,1,1,1,1,1,1,1,1,1,1,1,1,1,1,1,1,
1,1,1,1,1,1,1,1,1,1,1,1,1,1,1,1,1,1,1,1,1,1,1,1,1,1,1,1,1,1,1,1,1,1,1,1,
1,1,1,1,1,1,1,1,1,1,1,1,1,1,1,1,1,1,1,1,1,1,1,1,1,1,1,1,1,1,1,1,1,1,1,1,
1,1,1,1,1,1,1,1,1,1,1,1,1,1,1,1,1,1,1,1,1,1,1,1,1,1,1,1,1,1,1,1,1,1,1,1,
1,1,1,1,1,1,1,1,1,1,1,1,1,1,1,1,1,1,1,1,1,1,1,6),(0.,0.005,0.01,0.015,0.02,
0.025,0.03,0.035,0.04,0.045,0.05,0.055,0.06,0.065,0.07,0.075,0.08,0.085,
0.09,0.095,0.1,0.105,0.11,0.115,0.12,0.125,0.13,0.135,0.14,0.145,0.15,0.155,
0.16,0.165,0.17,0.175,0.18,0.185,0.19,0.195,0.2,0.205,0.21,0.215,0.22,0.225,
0.23,0.235,0.24,0.245,0.25,0.255,0.26,0.265,0.27,0.275,0.28,0.285,0.29,
0.295,0.3,0.305,0.31,0.315,0.32,0.325,0.33,0.335,0.34,0.345,0.35,0.355,
0.36,0.365,0.37,0.375,0.38,0.385,0.39,0.395,0.4,0.405,0.41,0.415,0.42,0.425,
0.43,0.435,0.44,0.445,0.45,0.455,0.46,0.465,0.47,0.475,0.48,0.485,0.49,
0.495,0.5,0.505,0.51,0.515,0.52,0.525,0.53,0.535,0.54,0.545,0.55,0.555,
0.56,0.565,0.57,0.575,0.58,0.585,0.59,0.595,0.6,0.605,0.61,0.615,0.62,0.625,
0.63,0.635,0.64,0.645,0.65,0.655,0.66,0.665,0.67,0.675,0.68,0.685,0.690000000000001,
0.695000000000001,0.700000000000001,0.705000000000001,0.710000000000001,
0.715000000000001,0.720000000000001,0.725000000000001,0.730000000000001,
0.735000000000001,0.740000000000001,0.745000000000001,0.750000000000001,
0.755000000000001,0.760000000000001,0.765000000000001,0.770000000000001,
0.775000000000001,0.780000000000001,0.785000000000001,0.790000000000001,
0.795000000000001,0.800000000000001,0.805000000000001,0.810000000000001,
0.815000000000001,0.820000000000001,0.825000000000001,0.830000000000001,
0.835000000000001,0.840000000000001,0.845000000000001,0.850000000000001,
0.855000000000001,0.860000000000001,0.865000000000001,0.870000000000001,
0.875000000000001,0.880000000000001,0.885000000000001,0.890000000000001,
0.895000000000001,0.900000000000001,0.905000000000001,0.910000000000001,
0.915000000000001,0.920000000000001,0.925000000000001,0.930000000000001,
0.935000000000001,0.940000000000001,0.94142984443149),.UNSPECIFIED.)
CURVE()
GEOMETRIC_REPRESENTATION_ITEM()
RATIONAL_B_SPLINE_CURVE((1.,1.,1.,1.,1.,1.,1.,1.,1.,1.,1.,1.,1.,1.,1.,1.,
1.,1.,1.,1.,1.,1.,1.,1.,1.,1.,1.,1.,1.,1.,1.,1.,1.,1.,1.,1.,1.,1.,1.,1.,
1.,1.,1.,1.,1.,1.,1.,1.,1.,1.,1.,1.,1.,1.,1.,1.,1.,1.,1.,1.,1.,1.,1.,1.,
1.,1.,1.,1.,1.,1.,1.,1.,1.,1.,1.,1.,1.,1.,1.,1.,1.,1.,1.,1.,1.,1.,1.,1.,
1.,1.,1.,1.,1.,1.,1.,1.,1.,1.,1.,1.,1.,1.,1.,1.,1.,1.,1.,1.,1.,1.,1.,1.,
1.,1.,1.,1.,1.,1.,1.,1.,1.,1.,1.,1.,1.,1.,1.,1.,1.,1.,1.,1.,1.,1.,1.,1.,
1.,1.,1.,1.,1.,1.,1.,1.,1.,1.,1.,1.,1.,1.,1.,1.,1.,1.,1.,1.,1.,1.,1.,1.,
1.,1.,1.,1.,1.,1.,1.,1.,1.,1.,1.,1.,1.,1.,1.,1.,1.,1.,1.,1.,1.,1.,1.,1.,
1.,1.,1.,1.,1.,1.,1.,1.,1.,1.))
REPRESENTATION_ITEM('')
);
#470=(
BOUNDED_CURVE()
B_SPLINE_CURVE(5,(#82797,#82798,#82799,#82800,#82801,#82802,#82803,#82804,
#82805,#82806,#82807,#82808,#82809,#82810,#82811,#82812,#82813,#82814,#82815,
#82816,#82817,#82818,#82819,#82820,#82821,#82822,#82823,#82824,#82825,#82826,
#82827,#82828,#82829,#82830,#82831,#82832,#82833,#82834,#82835,#82836,#82837,
#82838,#82839,#82840,#82841,#82842,#82843,#82844,#82845,#82846,#82847,#82848,
#82849,#82850,#82851,#82852,#82853,#82854,#82855,#82856,#82857,#82858,#82859,
#82860,#82861,#82862,#82863,#82864,#82865,#82866,#82867,#82868,#82869,#82870,
#82871,#82872,#82873,#82874,#82875,#82876,#82877,#82878,#82879,#82880,#82881,
#82882,#82883,#82884,#82885,#82886,#82887,#82888,#82889,#82890,#82891,#82892,
#82893,#82894,#82895,#82896,#82897,#82898,#82899,#82900,#82901,#82902,#82903,
#82904,#82905,#82906,#82907,#82908,#82909,#82910,#82911,#82912,#82913,#82914,
#82915,#82916,#82917,#82918,#82919,#82920,#82921,#82922,#82923,#82924,#82925,
#82926,#82927,#82928,#82929,#82930,#82931,#82932,#82933,#82934,#82935,#82936,
#82937,#82938,#82939,#82940,#82941,#82942,#82943,#82944,#82945,#82946,#82947,
#82948,#82949,#82950,#82951,#82952,#82953,#82954,#82955,#82956,#82957,#82958,
#82959,#82960,#82961,#82962,#82963,#82964,#82965,#82966,#82967,#82968,#82969,
#82970,#82971,#82972,#82973,#82974,#82975,#82976,#82977,#82978,#82979,#82980,
#82981,#82982,#82983,#82984,#82985,#82986,#82987,#82988,#82989,#82990),
 .UNSPECIFIED.,.F.,.F.)
B_SPLINE_CURVE_WITH_KNOTS((6,1,1,1,1,1,1,1,1,1,1,1,1,1,1,1,1,1,1,1,1,1,
1,1,1,1,1,1,1,1,1,1,1,1,1,1,1,1,1,1,1,1,1,1,1,1,1,1,1,1,1,1,1,1,1,1,1,1,
1,1,1,1,1,1,1,1,1,1,1,1,1,1,1,1,1,1,1,1,1,1,1,1,1,1,1,1,1,1,1,1,1,1,1,1,
1,1,1,1,1,1,1,1,1,1,1,1,1,1,1,1,1,1,1,1,1,1,1,1,1,1,1,1,1,1,1,1,1,1,1,1,
1,1,1,1,1,1,1,1,1,1,1,1,1,1,1,1,1,1,1,1,1,1,1,1,1,1,1,1,1,1,1,1,1,1,1,1,
1,1,1,1,1,1,1,1,1,1,1,1,1,1,1,1,1,1,1,1,1,1,1,6),(-0.94142984443149,-0.940000000000001,
-0.935000000000001,-0.930000000000001,-0.925000000000001,-0.920000000000001,
-0.915000000000001,-0.910000000000001,-0.905000000000001,-0.900000000000001,
-0.895000000000001,-0.890000000000001,-0.885000000000001,-0.880000000000001,
-0.875000000000001,-0.870000000000001,-0.865000000000001,-0.860000000000001,
-0.855000000000001,-0.850000000000001,-0.845000000000001,-0.840000000000001,
-0.835000000000001,-0.830000000000001,-0.825000000000001,-0.820000000000001,
-0.815000000000001,-0.810000000000001,-0.805000000000001,-0.800000000000001,
-0.795000000000001,-0.790000000000001,-0.785000000000001,-0.780000000000001,
-0.775000000000001,-0.770000000000001,-0.765000000000001,-0.760000000000001,
-0.755000000000001,-0.750000000000001,-0.745000000000001,-0.740000000000001,
-0.735000000000001,-0.730000000000001,-0.725000000000001,-0.720000000000001,
-0.715000000000001,-0.710000000000001,-0.705000000000001,-0.700000000000001,
-0.695000000000001,-0.690000000000001,-0.685,-0.68,-0.675,-0.67,-0.665,
-0.66,-0.655,-0.65,-0.645,-0.64,-0.635,-0.63,-0.625,-0.62,-0.615,-0.61,
-0.605,-0.6,-0.595,-0.59,-0.585,-0.58,-0.575,-0.57,-0.565,-0.56,-0.555,
-0.55,-0.545,-0.54,-0.535,-0.53,-0.525,-0.52,-0.515,-0.51,-0.505,-0.5,-0.495,
-0.49,-0.485,-0.48,-0.475,-0.47,-0.465,-0.46,-0.455,-0.45,-0.445,-0.44,
-0.435,-0.43,-0.425,-0.42,-0.415,-0.41,-0.405,-0.4,-0.395,-0.39,-0.385,
-0.38,-0.375,-0.37,-0.365,-0.36,-0.355,-0.35,-0.345,-0.34,-0.335,-0.33,
-0.325,-0.32,-0.315,-0.31,-0.305,-0.3,-0.295,-0.29,-0.285,-0.28,-0.275,
-0.27,-0.265,-0.26,-0.255,-0.25,-0.245,-0.24,-0.235,-0.23,-0.225,-0.22,
-0.215,-0.21,-0.205,-0.2,-0.195,-0.19,-0.185,-0.18,-0.175,-0.17,-0.165,
-0.16,-0.155,-0.15,-0.145,-0.14,-0.135,-0.13,-0.125,-0.12,-0.115,-0.11,
-0.105,-0.1,-0.095,-0.09,-0.085,-0.08,-0.075,-0.07,-0.065,-0.06,-0.055,
-0.05,-0.045,-0.04,-0.035,-0.03,-0.025,-0.02,-0.015,-0.01,-0.005,0.),
 .UNSPECIFIED.)
CURVE()
GEOMETRIC_REPRESENTATION_ITEM()
RATIONAL_B_SPLINE_CURVE((1.,1.,1.,1.,1.,1.,1.,1.,1.,1.,1.,1.,1.,1.,1.,1.,
1.,1.,1.,1.,1.,1.,1.,1.,1.,1.,1.,1.,1.,1.,1.,1.,1.,1.,1.,1.,1.,1.,1.,1.,
1.,1.,1.,1.,1.,1.,1.,1.,1.,1.,1.,1.,1.,1.,1.,1.,1.,1.,1.,1.,1.,1.,1.,1.,
1.,1.,1.,1.,1.,1.,1.,1.,1.,1.,1.,1.,1.,1.,1.,1.,1.,1.,1.,1.,1.,1.,1.,1.,
1.,1.,1.,1.,1.,1.,1.,1.,1.,1.,1.,1.,1.,1.,1.,1.,1.,1.,1.,1.,1.,1.,1.,1.,
1.,1.,1.,1.,1.,1.,1.,1.,1.,1.,1.,1.,1.,1.,1.,1.,1.,1.,1.,1.,1.,1.,1.,1.,
1.,1.,1.,1.,1.,1.,1.,1.,1.,1.,1.,1.,1.,1.,1.,1.,1.,1.,1.,1.,1.,1.,1.,1.,
1.,1.,1.,1.,1.,1.,1.,1.,1.,1.,1.,1.,1.,1.,1.,1.,1.,1.,1.,1.,1.,1.,1.,1.,
1.,1.,1.,1.,1.,1.,1.,1.,1.,1.))
REPRESENTATION_ITEM('')
);
#471=(
BOUNDED_CURVE()
B_SPLINE_CURVE(5,(#83497,#83498,#83499,#83500,#83501,#83502,#83503,#83504,
#83505,#83506,#83507,#83508,#83509,#83510,#83511,#83512,#83513,#83514,#83515,
#83516,#83517,#83518,#83519,#83520,#83521,#83522,#83523,#83524,#83525,#83526,
#83527,#83528,#83529,#83530,#83531,#83532,#83533,#83534,#83535,#83536,#83537,
#83538,#83539,#83540,#83541,#83542,#83543,#83544,#83545,#83546,#83547,#83548,
#83549,#83550,#83551,#83552,#83553,#83554,#83555,#83556,#83557,#83558,#83559,
#83560,#83561,#83562,#83563,#83564,#83565,#83566,#83567,#83568,#83569,#83570,
#83571,#83572,#83573,#83574,#83575,#83576,#83577,#83578,#83579,#83580,#83581,
#83582,#83583,#83584,#83585,#83586,#83587,#83588,#83589,#83590,#83591,#83592,
#83593,#83594,#83595,#83596,#83597,#83598,#83599,#83600,#83601,#83602,#83603,
#83604,#83605,#83606,#83607,#83608,#83609,#83610,#83611,#83612,#83613,#83614,
#83615,#83616,#83617,#83618,#83619,#83620,#83621,#83622,#83623,#83624,#83625,
#83626,#83627,#83628,#83629,#83630,#83631,#83632,#83633,#83634,#83635,#83636,
#83637,#83638,#83639,#83640,#83641,#83642,#83643,#83644,#83645,#83646,#83647,
#83648,#83649,#83650,#83651,#83652,#83653,#83654,#83655,#83656,#83657,#83658,
#83659,#83660,#83661,#83662,#83663,#83664,#83665,#83666,#83667,#83668,#83669,
#83670,#83671,#83672,#83673,#83674,#83675,#83676,#83677,#83678,#83679,#83680,
#83681,#83682,#83683,#83684,#83685,#83686,#83687,#83688,#83689,#83690),
 .UNSPECIFIED.,.F.,.F.)
B_SPLINE_CURVE_WITH_KNOTS((6,1,1,1,1,1,1,1,1,1,1,1,1,1,1,1,1,1,1,1,1,1,
1,1,1,1,1,1,1,1,1,1,1,1,1,1,1,1,1,1,1,1,1,1,1,1,1,1,1,1,1,1,1,1,1,1,1,1,
1,1,1,1,1,1,1,1,1,1,1,1,1,1,1,1,1,1,1,1,1,1,1,1,1,1,1,1,1,1,1,1,1,1,1,1,
1,1,1,1,1,1,1,1,1,1,1,1,1,1,1,1,1,1,1,1,1,1,1,1,1,1,1,1,1,1,1,1,1,1,1,1,
1,1,1,1,1,1,1,1,1,1,1,1,1,1,1,1,1,1,1,1,1,1,1,1,1,1,1,1,1,1,1,1,1,1,1,1,
1,1,1,1,1,1,1,1,1,1,1,1,1,1,1,1,1,1,1,1,1,1,1,6),(0.,0.005,0.01,0.015,0.02,
0.025,0.03,0.035,0.04,0.045,0.05,0.055,0.06,0.065,0.07,0.075,0.08,0.085,
0.09,0.095,0.1,0.105,0.11,0.115,0.12,0.125,0.13,0.135,0.14,0.145,0.15,0.155,
0.16,0.165,0.17,0.175,0.18,0.185,0.19,0.195,0.2,0.205,0.21,0.215,0.22,0.225,
0.23,0.235,0.24,0.245,0.25,0.255,0.26,0.265,0.27,0.275,0.28,0.285,0.29,
0.295,0.3,0.305,0.31,0.315,0.32,0.325,0.33,0.335,0.34,0.345,0.35,0.355,
0.36,0.365,0.37,0.375,0.38,0.385,0.39,0.395,0.4,0.405,0.41,0.415,0.42,0.425,
0.43,0.435,0.44,0.445,0.45,0.455,0.46,0.465,0.47,0.475,0.48,0.485,0.49,
0.495,0.5,0.505,0.51,0.515,0.52,0.525,0.53,0.535,0.54,0.545,0.55,0.555,
0.56,0.565,0.57,0.575,0.58,0.585,0.59,0.595,0.6,0.605,0.61,0.615,0.62,0.625,
0.63,0.635,0.64,0.645,0.65,0.655,0.66,0.665,0.67,0.675,0.68,0.685,0.690000000000001,
0.695000000000001,0.700000000000001,0.705000000000001,0.710000000000001,
0.715000000000001,0.720000000000001,0.725000000000001,0.730000000000001,
0.735000000000001,0.740000000000001,0.745000000000001,0.750000000000001,
0.755000000000001,0.760000000000001,0.765000000000001,0.770000000000001,
0.775000000000001,0.780000000000001,0.785000000000001,0.790000000000001,
0.795000000000001,0.800000000000001,0.805000000000001,0.810000000000001,
0.815000000000001,0.820000000000001,0.825000000000001,0.830000000000001,
0.835000000000001,0.840000000000001,0.845000000000001,0.850000000000001,
0.855000000000001,0.860000000000001,0.865000000000001,0.870000000000001,
0.875000000000001,0.880000000000001,0.885000000000001,0.890000000000001,
0.895000000000001,0.900000000000001,0.905000000000001,0.910000000000001,
0.915000000000001,0.920000000000001,0.925000000000001,0.930000000000001,
0.935000000000001,0.940000000000001,0.941429844431321),.UNSPECIFIED.)
CURVE()
GEOMETRIC_REPRESENTATION_ITEM()
RATIONAL_B_SPLINE_CURVE((1.,1.,1.,1.,1.,1.,1.,1.,1.,1.,1.,1.,1.,1.,1.,1.,
1.,1.,1.,1.,1.,1.,1.,1.,1.,1.,1.,1.,1.,1.,1.,1.,1.,1.,1.,1.,1.,1.,1.,1.,
1.,1.,1.,1.,1.,1.,1.,1.,1.,1.,1.,1.,1.,1.,1.,1.,1.,1.,1.,1.,1.,1.,1.,1.,
1.,1.,1.,1.,1.,1.,1.,1.,1.,1.,1.,1.,1.,1.,1.,1.,1.,1.,1.,1.,1.,1.,1.,1.,
1.,1.,1.,1.,1.,1.,1.,1.,1.,1.,1.,1.,1.,1.,1.,1.,1.,1.,1.,1.,1.,1.,1.,1.,
1.,1.,1.,1.,1.,1.,1.,1.,1.,1.,1.,1.,1.,1.,1.,1.,1.,1.,1.,1.,1.,1.,1.,1.,
1.,1.,1.,1.,1.,1.,1.,1.,1.,1.,1.,1.,1.,1.,1.,1.,1.,1.,1.,1.,1.,1.,1.,1.,
1.,1.,1.,1.,1.,1.,1.,1.,1.,1.,1.,1.,1.,1.,1.,1.,1.,1.,1.,1.,1.,1.,1.,1.,
1.,1.,1.,1.,1.,1.,1.,1.,1.,1.))
REPRESENTATION_ITEM('')
);
#472=(
BOUNDED_CURVE()
B_SPLINE_CURVE(5,(#83693,#83694,#83695,#83696,#83697,#83698,#83699,#83700,
#83701,#83702,#83703,#83704,#83705,#83706,#83707,#83708,#83709,#83710,#83711,
#83712,#83713,#83714,#83715,#83716,#83717,#83718,#83719,#83720,#83721,#83722,
#83723,#83724,#83725,#83726,#83727,#83728,#83729,#83730,#83731,#83732,#83733,
#83734,#83735,#83736,#83737,#83738,#83739,#83740,#83741,#83742,#83743,#83744,
#83745,#83746,#83747,#83748,#83749,#83750,#83751,#83752,#83753,#83754,#83755,
#83756,#83757,#83758,#83759,#83760,#83761,#83762,#83763,#83764,#83765,#83766,
#83767,#83768,#83769,#83770,#83771,#83772,#83773,#83774,#83775,#83776,#83777,
#83778,#83779,#83780,#83781,#83782,#83783,#83784,#83785,#83786,#83787,#83788,
#83789,#83790,#83791,#83792,#83793,#83794,#83795,#83796,#83797,#83798,#83799,
#83800,#83801,#83802,#83803,#83804,#83805,#83806,#83807,#83808,#83809,#83810,
#83811,#83812,#83813,#83814,#83815,#83816,#83817,#83818,#83819,#83820,#83821,
#83822,#83823,#83824,#83825,#83826,#83827,#83828,#83829,#83830,#83831,#83832,
#83833,#83834,#83835,#83836,#83837,#83838,#83839,#83840,#83841,#83842,#83843,
#83844,#83845,#83846,#83847,#83848,#83849,#83850,#83851,#83852,#83853,#83854,
#83855,#83856,#83857,#83858,#83859,#83860,#83861,#83862,#83863,#83864,#83865,
#83866,#83867,#83868,#83869,#83870,#83871,#83872,#83873,#83874,#83875,#83876,
#83877,#83878,#83879,#83880,#83881,#83882,#83883,#83884,#83885,#83886),
 .UNSPECIFIED.,.F.,.F.)
B_SPLINE_CURVE_WITH_KNOTS((6,1,1,1,1,1,1,1,1,1,1,1,1,1,1,1,1,1,1,1,1,1,
1,1,1,1,1,1,1,1,1,1,1,1,1,1,1,1,1,1,1,1,1,1,1,1,1,1,1,1,1,1,1,1,1,1,1,1,
1,1,1,1,1,1,1,1,1,1,1,1,1,1,1,1,1,1,1,1,1,1,1,1,1,1,1,1,1,1,1,1,1,1,1,1,
1,1,1,1,1,1,1,1,1,1,1,1,1,1,1,1,1,1,1,1,1,1,1,1,1,1,1,1,1,1,1,1,1,1,1,1,
1,1,1,1,1,1,1,1,1,1,1,1,1,1,1,1,1,1,1,1,1,1,1,1,1,1,1,1,1,1,1,1,1,1,1,1,
1,1,1,1,1,1,1,1,1,1,1,1,1,1,1,1,1,1,1,1,1,1,1,6),(-0.94142984443133,-0.940000000000001,
-0.935000000000001,-0.930000000000001,-0.925000000000001,-0.920000000000001,
-0.915000000000001,-0.910000000000001,-0.905000000000001,-0.900000000000001,
-0.895000000000001,-0.890000000000001,-0.885000000000001,-0.880000000000001,
-0.875000000000001,-0.870000000000001,-0.865000000000001,-0.860000000000001,
-0.855000000000001,-0.850000000000001,-0.845000000000001,-0.840000000000001,
-0.835000000000001,-0.830000000000001,-0.825000000000001,-0.820000000000001,
-0.815000000000001,-0.810000000000001,-0.805000000000001,-0.800000000000001,
-0.795000000000001,-0.790000000000001,-0.785000000000001,-0.780000000000001,
-0.775000000000001,-0.770000000000001,-0.765000000000001,-0.760000000000001,
-0.755000000000001,-0.750000000000001,-0.745000000000001,-0.740000000000001,
-0.735000000000001,-0.730000000000001,-0.725000000000001,-0.720000000000001,
-0.715000000000001,-0.710000000000001,-0.705000000000001,-0.700000000000001,
-0.695000000000001,-0.690000000000001,-0.685,-0.68,-0.675,-0.67,-0.665,
-0.66,-0.655,-0.65,-0.645,-0.64,-0.635,-0.63,-0.625,-0.62,-0.615,-0.61,
-0.605,-0.6,-0.595,-0.59,-0.585,-0.58,-0.575,-0.57,-0.565,-0.56,-0.555,
-0.55,-0.545,-0.54,-0.535,-0.53,-0.525,-0.52,-0.515,-0.51,-0.505,-0.5,-0.495,
-0.49,-0.485,-0.48,-0.475,-0.47,-0.465,-0.46,-0.455,-0.45,-0.445,-0.44,
-0.435,-0.43,-0.425,-0.42,-0.415,-0.41,-0.405,-0.4,-0.395,-0.39,-0.385,
-0.38,-0.375,-0.37,-0.365,-0.36,-0.355,-0.35,-0.345,-0.34,-0.335,-0.33,
-0.325,-0.32,-0.315,-0.31,-0.305,-0.3,-0.295,-0.29,-0.285,-0.28,-0.275,
-0.27,-0.265,-0.26,-0.255,-0.25,-0.245,-0.24,-0.235,-0.23,-0.225,-0.22,
-0.215,-0.21,-0.205,-0.2,-0.195,-0.19,-0.185,-0.18,-0.175,-0.17,-0.165,
-0.16,-0.155,-0.15,-0.145,-0.14,-0.135,-0.13,-0.125,-0.12,-0.115,-0.11,
-0.105,-0.1,-0.095,-0.09,-0.085,-0.08,-0.075,-0.07,-0.065,-0.06,-0.055,
-0.05,-0.045,-0.04,-0.035,-0.03,-0.025,-0.02,-0.015,-0.01,-0.005,0.),
 .UNSPECIFIED.)
CURVE()
GEOMETRIC_REPRESENTATION_ITEM()
RATIONAL_B_SPLINE_CURVE((1.,1.,1.,1.,1.,1.,1.,1.,1.,1.,1.,1.,1.,1.,1.,1.,
1.,1.,1.,1.,1.,1.,1.,1.,1.,1.,1.,1.,1.,1.,1.,1.,1.,1.,1.,1.,1.,1.,1.,1.,
1.,1.,1.,1.,1.,1.,1.,1.,1.,1.,1.,1.,1.,1.,1.,1.,1.,1.,1.,1.,1.,1.,1.,1.,
1.,1.,1.,1.,1.,1.,1.,1.,1.,1.,1.,1.,1.,1.,1.,1.,1.,1.,1.,1.,1.,1.,1.,1.,
1.,1.,1.,1.,1.,1.,1.,1.,1.,1.,1.,1.,1.,1.,1.,1.,1.,1.,1.,1.,1.,1.,1.,1.,
1.,1.,1.,1.,1.,1.,1.,1.,1.,1.,1.,1.,1.,1.,1.,1.,1.,1.,1.,1.,1.,1.,1.,1.,
1.,1.,1.,1.,1.,1.,1.,1.,1.,1.,1.,1.,1.,1.,1.,1.,1.,1.,1.,1.,1.,1.,1.,1.,
1.,1.,1.,1.,1.,1.,1.,1.,1.,1.,1.,1.,1.,1.,1.,1.,1.,1.,1.,1.,1.,1.,1.,1.,
1.,1.,1.,1.,1.,1.,1.,1.,1.,1.))
REPRESENTATION_ITEM('')
);
#473=(
BOUNDED_CURVE()
B_SPLINE_CURVE(5,(#84393,#84394,#84395,#84396,#84397,#84398,#84399,#84400,
#84401,#84402,#84403,#84404,#84405,#84406,#84407,#84408,#84409,#84410,#84411,
#84412,#84413,#84414,#84415,#84416,#84417,#84418,#84419,#84420,#84421,#84422,
#84423,#84424,#84425,#84426,#84427,#84428,#84429,#84430,#84431,#84432,#84433,
#84434,#84435,#84436,#84437,#84438,#84439,#84440,#84441,#84442,#84443,#84444,
#84445,#84446,#84447,#84448,#84449,#84450,#84451,#84452,#84453,#84454,#84455,
#84456,#84457,#84458,#84459,#84460,#84461,#84462,#84463,#84464,#84465,#84466,
#84467,#84468,#84469,#84470,#84471,#84472,#84473,#84474,#84475,#84476,#84477,
#84478,#84479,#84480,#84481,#84482,#84483,#84484,#84485,#84486,#84487,#84488,
#84489,#84490,#84491,#84492,#84493,#84494,#84495,#84496,#84497,#84498,#84499,
#84500,#84501,#84502,#84503,#84504,#84505,#84506,#84507,#84508,#84509,#84510,
#84511,#84512,#84513,#84514,#84515,#84516,#84517,#84518,#84519,#84520,#84521,
#84522,#84523,#84524,#84525,#84526,#84527,#84528,#84529,#84530,#84531,#84532,
#84533,#84534,#84535,#84536,#84537,#84538,#84539,#84540,#84541,#84542,#84543,
#84544,#84545,#84546,#84547,#84548,#84549,#84550,#84551,#84552,#84553,#84554,
#84555,#84556,#84557,#84558,#84559,#84560,#84561,#84562,#84563,#84564,#84565,
#84566,#84567,#84568,#84569,#84570,#84571,#84572,#84573,#84574,#84575,#84576,
#84577,#84578,#84579,#84580,#84581,#84582,#84583,#84584,#84585,#84586),
 .UNSPECIFIED.,.F.,.F.)
B_SPLINE_CURVE_WITH_KNOTS((6,1,1,1,1,1,1,1,1,1,1,1,1,1,1,1,1,1,1,1,1,1,
1,1,1,1,1,1,1,1,1,1,1,1,1,1,1,1,1,1,1,1,1,1,1,1,1,1,1,1,1,1,1,1,1,1,1,1,
1,1,1,1,1,1,1,1,1,1,1,1,1,1,1,1,1,1,1,1,1,1,1,1,1,1,1,1,1,1,1,1,1,1,1,1,
1,1,1,1,1,1,1,1,1,1,1,1,1,1,1,1,1,1,1,1,1,1,1,1,1,1,1,1,1,1,1,1,1,1,1,1,
1,1,1,1,1,1,1,1,1,1,1,1,1,1,1,1,1,1,1,1,1,1,1,1,1,1,1,1,1,1,1,1,1,1,1,1,
1,1,1,1,1,1,1,1,1,1,1,1,1,1,1,1,1,1,1,1,1,1,1,6),(0.,0.005,0.01,0.015,0.02,
0.025,0.03,0.035,0.04,0.045,0.05,0.055,0.06,0.065,0.07,0.075,0.08,0.085,
0.09,0.095,0.1,0.105,0.11,0.115,0.12,0.125,0.13,0.135,0.14,0.145,0.15,0.155,
0.16,0.165,0.17,0.175,0.18,0.185,0.19,0.195,0.2,0.205,0.21,0.215,0.22,0.225,
0.23,0.235,0.24,0.245,0.25,0.255,0.26,0.265,0.27,0.275,0.28,0.285,0.29,
0.295,0.3,0.305,0.31,0.315,0.32,0.325,0.33,0.335,0.34,0.345,0.35,0.355,
0.36,0.365,0.37,0.375,0.38,0.385,0.39,0.395,0.4,0.405,0.41,0.415,0.42,0.425,
0.43,0.435,0.44,0.445,0.45,0.455,0.46,0.465,0.47,0.475,0.48,0.485,0.49,
0.495,0.5,0.505,0.51,0.515,0.52,0.525,0.53,0.535,0.54,0.545,0.55,0.555,
0.56,0.565,0.57,0.575,0.58,0.585,0.59,0.595,0.6,0.605,0.61,0.615,0.62,0.625,
0.63,0.635,0.64,0.645,0.65,0.655,0.66,0.665,0.67,0.675,0.68,0.685,0.690000000000001,
0.695000000000001,0.700000000000001,0.705000000000001,0.710000000000001,
0.715000000000001,0.720000000000001,0.725000000000001,0.730000000000001,
0.735000000000001,0.740000000000001,0.745000000000001,0.750000000000001,
0.755000000000001,0.760000000000001,0.765000000000001,0.770000000000001,
0.775000000000001,0.780000000000001,0.785000000000001,0.790000000000001,
0.795000000000001,0.800000000000001,0.805000000000001,0.810000000000001,
0.815000000000001,0.820000000000001,0.825000000000001,0.830000000000001,
0.835000000000001,0.840000000000001,0.845000000000001,0.850000000000001,
0.855000000000001,0.860000000000001,0.865000000000001,0.870000000000001,
0.875000000000001,0.880000000000001,0.885000000000001,0.890000000000001,
0.895000000000001,0.900000000000001,0.905000000000001,0.910000000000001,
0.915000000000001,0.920000000000001,0.925000000000001,0.930000000000001,
0.935000000000001,0.940000000000001,0.941429844431379),.UNSPECIFIED.)
CURVE()
GEOMETRIC_REPRESENTATION_ITEM()
RATIONAL_B_SPLINE_CURVE((1.,1.,1.,1.,1.,1.,1.,1.,1.,1.,1.,1.,1.,1.,1.,1.,
1.,1.,1.,1.,1.,1.,1.,1.,1.,1.,1.,1.,1.,1.,1.,1.,1.,1.,1.,1.,1.,1.,1.,1.,
1.,1.,1.,1.,1.,1.,1.,1.,1.,1.,1.,1.,1.,1.,1.,1.,1.,1.,1.,1.,1.,1.,1.,1.,
1.,1.,1.,1.,1.,1.,1.,1.,1.,1.,1.,1.,1.,1.,1.,1.,1.,1.,1.,1.,1.,1.,1.,1.,
1.,1.,1.,1.,1.,1.,1.,1.,1.,1.,1.,1.,1.,1.,1.,1.,1.,1.,1.,1.,1.,1.,1.,1.,
1.,1.,1.,1.,1.,1.,1.,1.,1.,1.,1.,1.,1.,1.,1.,1.,1.,1.,1.,1.,1.,1.,1.,1.,
1.,1.,1.,1.,1.,1.,1.,1.,1.,1.,1.,1.,1.,1.,1.,1.,1.,1.,1.,1.,1.,1.,1.,1.,
1.,1.,1.,1.,1.,1.,1.,1.,1.,1.,1.,1.,1.,1.,1.,1.,1.,1.,1.,1.,1.,1.,1.,1.,
1.,1.,1.,1.,1.,1.,1.,1.,1.,1.))
REPRESENTATION_ITEM('')
);
#474=(
BOUNDED_CURVE()
B_SPLINE_CURVE(5,(#84589,#84590,#84591,#84592,#84593,#84594,#84595,#84596,
#84597,#84598,#84599,#84600,#84601,#84602,#84603,#84604,#84605,#84606,#84607,
#84608,#84609,#84610,#84611,#84612,#84613,#84614,#84615,#84616,#84617,#84618,
#84619,#84620,#84621,#84622,#84623,#84624,#84625,#84626,#84627,#84628,#84629,
#84630,#84631,#84632,#84633,#84634,#84635,#84636,#84637,#84638,#84639,#84640,
#84641,#84642,#84643,#84644,#84645,#84646,#84647,#84648,#84649,#84650,#84651,
#84652,#84653,#84654,#84655,#84656,#84657,#84658,#84659,#84660,#84661,#84662,
#84663,#84664,#84665,#84666,#84667,#84668,#84669,#84670,#84671,#84672,#84673,
#84674,#84675,#84676,#84677,#84678,#84679,#84680,#84681,#84682,#84683,#84684,
#84685,#84686,#84687,#84688,#84689,#84690,#84691,#84692,#84693,#84694,#84695,
#84696,#84697,#84698,#84699,#84700,#84701,#84702,#84703,#84704,#84705,#84706,
#84707,#84708,#84709,#84710,#84711,#84712,#84713,#84714,#84715,#84716,#84717,
#84718,#84719,#84720,#84721,#84722,#84723,#84724,#84725,#84726,#84727,#84728,
#84729,#84730,#84731,#84732,#84733,#84734,#84735,#84736,#84737,#84738,#84739,
#84740,#84741,#84742,#84743,#84744,#84745,#84746,#84747,#84748,#84749,#84750,
#84751,#84752,#84753,#84754,#84755,#84756,#84757,#84758,#84759,#84760,#84761,
#84762,#84763,#84764,#84765,#84766,#84767,#84768,#84769,#84770,#84771,#84772,
#84773,#84774,#84775,#84776,#84777,#84778,#84779,#84780,#84781,#84782),
 .UNSPECIFIED.,.F.,.F.)
B_SPLINE_CURVE_WITH_KNOTS((6,1,1,1,1,1,1,1,1,1,1,1,1,1,1,1,1,1,1,1,1,1,
1,1,1,1,1,1,1,1,1,1,1,1,1,1,1,1,1,1,1,1,1,1,1,1,1,1,1,1,1,1,1,1,1,1,1,1,
1,1,1,1,1,1,1,1,1,1,1,1,1,1,1,1,1,1,1,1,1,1,1,1,1,1,1,1,1,1,1,1,1,1,1,1,
1,1,1,1,1,1,1,1,1,1,1,1,1,1,1,1,1,1,1,1,1,1,1,1,1,1,1,1,1,1,1,1,1,1,1,1,
1,1,1,1,1,1,1,1,1,1,1,1,1,1,1,1,1,1,1,1,1,1,1,1,1,1,1,1,1,1,1,1,1,1,1,1,
1,1,1,1,1,1,1,1,1,1,1,1,1,1,1,1,1,1,1,1,1,1,1,6),(-0.941429844431374,-0.940000000000001,
-0.935000000000001,-0.930000000000001,-0.925000000000001,-0.920000000000001,
-0.915000000000001,-0.910000000000001,-0.905000000000001,-0.900000000000001,
-0.895000000000001,-0.890000000000001,-0.885000000000001,-0.880000000000001,
-0.875000000000001,-0.870000000000001,-0.865000000000001,-0.860000000000001,
-0.855000000000001,-0.850000000000001,-0.845000000000001,-0.840000000000001,
-0.835000000000001,-0.830000000000001,-0.825000000000001,-0.820000000000001,
-0.815000000000001,-0.810000000000001,-0.805000000000001,-0.800000000000001,
-0.795000000000001,-0.790000000000001,-0.785000000000001,-0.780000000000001,
-0.775000000000001,-0.770000000000001,-0.765000000000001,-0.760000000000001,
-0.755000000000001,-0.750000000000001,-0.745000000000001,-0.740000000000001,
-0.735000000000001,-0.730000000000001,-0.725000000000001,-0.720000000000001,
-0.715000000000001,-0.710000000000001,-0.705000000000001,-0.700000000000001,
-0.695000000000001,-0.690000000000001,-0.685,-0.68,-0.675,-0.67,-0.665,
-0.66,-0.655,-0.65,-0.645,-0.64,-0.635,-0.63,-0.625,-0.62,-0.615,-0.61,
-0.605,-0.6,-0.595,-0.59,-0.585,-0.58,-0.575,-0.57,-0.565,-0.56,-0.555,
-0.55,-0.545,-0.54,-0.535,-0.53,-0.525,-0.52,-0.515,-0.51,-0.505,-0.5,-0.495,
-0.49,-0.485,-0.48,-0.475,-0.47,-0.465,-0.46,-0.455,-0.45,-0.445,-0.44,
-0.435,-0.43,-0.425,-0.42,-0.415,-0.41,-0.405,-0.4,-0.395,-0.39,-0.385,
-0.38,-0.375,-0.37,-0.365,-0.36,-0.355,-0.35,-0.345,-0.34,-0.335,-0.33,
-0.325,-0.32,-0.315,-0.31,-0.305,-0.3,-0.295,-0.29,-0.285,-0.28,-0.275,
-0.27,-0.265,-0.26,-0.255,-0.25,-0.245,-0.24,-0.235,-0.23,-0.225,-0.22,
-0.215,-0.21,-0.205,-0.2,-0.195,-0.19,-0.185,-0.18,-0.175,-0.17,-0.165,
-0.16,-0.155,-0.15,-0.145,-0.14,-0.135,-0.13,-0.125,-0.12,-0.115,-0.11,
-0.105,-0.1,-0.095,-0.09,-0.085,-0.08,-0.075,-0.07,-0.065,-0.06,-0.055,
-0.05,-0.045,-0.04,-0.035,-0.03,-0.025,-0.02,-0.015,-0.01,-0.005,0.),
 .UNSPECIFIED.)
CURVE()
GEOMETRIC_REPRESENTATION_ITEM()
RATIONAL_B_SPLINE_CURVE((1.,1.,1.,1.,1.,1.,1.,1.,1.,1.,1.,1.,1.,1.,1.,1.,
1.,1.,1.,1.,1.,1.,1.,1.,1.,1.,1.,1.,1.,1.,1.,1.,1.,1.,1.,1.,1.,1.,1.,1.,
1.,1.,1.,1.,1.,1.,1.,1.,1.,1.,1.,1.,1.,1.,1.,1.,1.,1.,1.,1.,1.,1.,1.,1.,
1.,1.,1.,1.,1.,1.,1.,1.,1.,1.,1.,1.,1.,1.,1.,1.,1.,1.,1.,1.,1.,1.,1.,1.,
1.,1.,1.,1.,1.,1.,1.,1.,1.,1.,1.,1.,1.,1.,1.,1.,1.,1.,1.,1.,1.,1.,1.,1.,
1.,1.,1.,1.,1.,1.,1.,1.,1.,1.,1.,1.,1.,1.,1.,1.,1.,1.,1.,1.,1.,1.,1.,1.,
1.,1.,1.,1.,1.,1.,1.,1.,1.,1.,1.,1.,1.,1.,1.,1.,1.,1.,1.,1.,1.,1.,1.,1.,
1.,1.,1.,1.,1.,1.,1.,1.,1.,1.,1.,1.,1.,1.,1.,1.,1.,1.,1.,1.,1.,1.,1.,1.,
1.,1.,1.,1.,1.,1.,1.,1.,1.,1.))
REPRESENTATION_ITEM('')
);
#475=(
BOUNDED_CURVE()
B_SPLINE_CURVE(5,(#85289,#85290,#85291,#85292,#85293,#85294,#85295,#85296,
#85297,#85298,#85299,#85300,#85301,#85302,#85303,#85304,#85305,#85306,#85307,
#85308,#85309,#85310,#85311,#85312,#85313,#85314,#85315,#85316,#85317,#85318,
#85319,#85320,#85321,#85322,#85323,#85324,#85325,#85326,#85327,#85328,#85329,
#85330,#85331,#85332,#85333,#85334,#85335,#85336,#85337,#85338,#85339,#85340,
#85341,#85342,#85343,#85344,#85345,#85346,#85347,#85348,#85349,#85350,#85351,
#85352,#85353,#85354,#85355,#85356,#85357,#85358,#85359,#85360,#85361,#85362,
#85363,#85364,#85365,#85366,#85367,#85368,#85369,#85370,#85371,#85372,#85373,
#85374,#85375,#85376,#85377,#85378,#85379,#85380,#85381,#85382,#85383,#85384,
#85385,#85386,#85387,#85388,#85389,#85390,#85391,#85392,#85393,#85394,#85395,
#85396,#85397,#85398,#85399,#85400,#85401,#85402,#85403,#85404,#85405,#85406,
#85407,#85408,#85409,#85410,#85411,#85412,#85413,#85414,#85415,#85416,#85417,
#85418,#85419,#85420,#85421,#85422,#85423,#85424,#85425,#85426,#85427,#85428,
#85429,#85430,#85431,#85432,#85433,#85434,#85435,#85436,#85437,#85438,#85439,
#85440,#85441,#85442,#85443,#85444,#85445,#85446,#85447,#85448,#85449,#85450,
#85451,#85452,#85453,#85454,#85455,#85456,#85457,#85458,#85459,#85460,#85461,
#85462,#85463,#85464,#85465,#85466,#85467,#85468,#85469,#85470,#85471,#85472,
#85473,#85474,#85475,#85476,#85477,#85478,#85479,#85480,#85481,#85482),
 .UNSPECIFIED.,.F.,.F.)
B_SPLINE_CURVE_WITH_KNOTS((6,1,1,1,1,1,1,1,1,1,1,1,1,1,1,1,1,1,1,1,1,1,
1,1,1,1,1,1,1,1,1,1,1,1,1,1,1,1,1,1,1,1,1,1,1,1,1,1,1,1,1,1,1,1,1,1,1,1,
1,1,1,1,1,1,1,1,1,1,1,1,1,1,1,1,1,1,1,1,1,1,1,1,1,1,1,1,1,1,1,1,1,1,1,1,
1,1,1,1,1,1,1,1,1,1,1,1,1,1,1,1,1,1,1,1,1,1,1,1,1,1,1,1,1,1,1,1,1,1,1,1,
1,1,1,1,1,1,1,1,1,1,1,1,1,1,1,1,1,1,1,1,1,1,1,1,1,1,1,1,1,1,1,1,1,1,1,1,
1,1,1,1,1,1,1,1,1,1,1,1,1,1,1,1,1,1,1,1,1,1,1,6),(0.,0.005,0.01,0.015,0.02,
0.025,0.03,0.035,0.04,0.045,0.05,0.055,0.06,0.065,0.07,0.075,0.08,0.085,
0.09,0.095,0.1,0.105,0.11,0.115,0.12,0.125,0.13,0.135,0.14,0.145,0.15,0.155,
0.16,0.165,0.17,0.175,0.18,0.185,0.19,0.195,0.2,0.205,0.21,0.215,0.22,0.225,
0.23,0.235,0.24,0.245,0.25,0.255,0.26,0.265,0.27,0.275,0.28,0.285,0.29,
0.295,0.3,0.305,0.31,0.315,0.32,0.325,0.33,0.335,0.34,0.345,0.35,0.355,
0.36,0.365,0.37,0.375,0.38,0.385,0.39,0.395,0.4,0.405,0.41,0.415,0.42,0.425,
0.43,0.435,0.44,0.445,0.45,0.455,0.46,0.465,0.47,0.475,0.48,0.485,0.49,
0.495,0.5,0.505,0.51,0.515,0.52,0.525,0.53,0.535,0.54,0.545,0.55,0.555,
0.56,0.565,0.57,0.575,0.58,0.585,0.59,0.595,0.6,0.605,0.61,0.615,0.62,0.625,
0.63,0.635,0.64,0.645,0.65,0.655,0.66,0.665,0.67,0.675,0.68,0.685,0.690000000000001,
0.695000000000001,0.700000000000001,0.705000000000001,0.710000000000001,
0.715000000000001,0.720000000000001,0.725000000000001,0.730000000000001,
0.735000000000001,0.740000000000001,0.745000000000001,0.750000000000001,
0.755000000000001,0.760000000000001,0.765000000000001,0.770000000000001,
0.775000000000001,0.780000000000001,0.785000000000001,0.790000000000001,
0.795000000000001,0.800000000000001,0.805000000000001,0.810000000000001,
0.815000000000001,0.820000000000001,0.825000000000001,0.830000000000001,
0.835000000000001,0.840000000000001,0.845000000000001,0.850000000000001,
0.855000000000001,0.860000000000001,0.865000000000001,0.870000000000001,
0.875000000000001,0.880000000000001,0.885000000000001,0.890000000000001,
0.895000000000001,0.900000000000001,0.905000000000001,0.910000000000001,
0.915000000000001,0.920000000000001,0.925000000000001,0.930000000000001,
0.935000000000001,0.940000000000001,0.94142984443142),.UNSPECIFIED.)
CURVE()
GEOMETRIC_REPRESENTATION_ITEM()
RATIONAL_B_SPLINE_CURVE((1.,1.,1.,1.,1.,1.,1.,1.,1.,1.,1.,1.,1.,1.,1.,1.,
1.,1.,1.,1.,1.,1.,1.,1.,1.,1.,1.,1.,1.,1.,1.,1.,1.,1.,1.,1.,1.,1.,1.,1.,
1.,1.,1.,1.,1.,1.,1.,1.,1.,1.,1.,1.,1.,1.,1.,1.,1.,1.,1.,1.,1.,1.,1.,1.,
1.,1.,1.,1.,1.,1.,1.,1.,1.,1.,1.,1.,1.,1.,1.,1.,1.,1.,1.,1.,1.,1.,1.,1.,
1.,1.,1.,1.,1.,1.,1.,1.,1.,1.,1.,1.,1.,1.,1.,1.,1.,1.,1.,1.,1.,1.,1.,1.,
1.,1.,1.,1.,1.,1.,1.,1.,1.,1.,1.,1.,1.,1.,1.,1.,1.,1.,1.,1.,1.,1.,1.,1.,
1.,1.,1.,1.,1.,1.,1.,1.,1.,1.,1.,1.,1.,1.,1.,1.,1.,1.,1.,1.,1.,1.,1.,1.,
1.,1.,1.,1.,1.,1.,1.,1.,1.,1.,1.,1.,1.,1.,1.,1.,1.,1.,1.,1.,1.,1.,1.,1.,
1.,1.,1.,1.,1.,1.,1.,1.,1.,1.))
REPRESENTATION_ITEM('')
);
#476=(
BOUNDED_CURVE()
B_SPLINE_CURVE(5,(#85485,#85486,#85487,#85488,#85489,#85490,#85491,#85492,
#85493,#85494,#85495,#85496,#85497,#85498,#85499,#85500,#85501,#85502,#85503,
#85504,#85505,#85506,#85507,#85508,#85509,#85510,#85511,#85512,#85513,#85514,
#85515,#85516,#85517,#85518,#85519,#85520,#85521,#85522,#85523,#85524,#85525,
#85526,#85527,#85528,#85529,#85530,#85531,#85532,#85533,#85534,#85535,#85536,
#85537,#85538,#85539,#85540,#85541,#85542,#85543,#85544,#85545,#85546,#85547,
#85548,#85549,#85550,#85551,#85552,#85553,#85554,#85555,#85556,#85557,#85558,
#85559,#85560,#85561,#85562,#85563,#85564,#85565,#85566,#85567,#85568,#85569,
#85570,#85571,#85572,#85573,#85574,#85575,#85576,#85577,#85578,#85579,#85580,
#85581,#85582,#85583,#85584,#85585,#85586,#85587,#85588,#85589,#85590,#85591,
#85592,#85593,#85594,#85595,#85596,#85597,#85598,#85599,#85600,#85601,#85602,
#85603,#85604,#85605,#85606,#85607,#85608,#85609,#85610,#85611,#85612,#85613,
#85614,#85615,#85616,#85617,#85618,#85619,#85620,#85621,#85622,#85623,#85624,
#85625,#85626,#85627,#85628,#85629,#85630,#85631,#85632,#85633,#85634,#85635,
#85636,#85637,#85638,#85639,#85640,#85641,#85642,#85643,#85644,#85645,#85646,
#85647,#85648,#85649,#85650,#85651,#85652,#85653,#85654,#85655,#85656,#85657,
#85658,#85659,#85660,#85661,#85662,#85663,#85664,#85665,#85666,#85667,#85668,
#85669,#85670,#85671,#85672,#85673,#85674,#85675,#85676,#85677,#85678),
 .UNSPECIFIED.,.F.,.F.)
B_SPLINE_CURVE_WITH_KNOTS((6,1,1,1,1,1,1,1,1,1,1,1,1,1,1,1,1,1,1,1,1,1,
1,1,1,1,1,1,1,1,1,1,1,1,1,1,1,1,1,1,1,1,1,1,1,1,1,1,1,1,1,1,1,1,1,1,1,1,
1,1,1,1,1,1,1,1,1,1,1,1,1,1,1,1,1,1,1,1,1,1,1,1,1,1,1,1,1,1,1,1,1,1,1,1,
1,1,1,1,1,1,1,1,1,1,1,1,1,1,1,1,1,1,1,1,1,1,1,1,1,1,1,1,1,1,1,1,1,1,1,1,
1,1,1,1,1,1,1,1,1,1,1,1,1,1,1,1,1,1,1,1,1,1,1,1,1,1,1,1,1,1,1,1,1,1,1,1,
1,1,1,1,1,1,1,1,1,1,1,1,1,1,1,1,1,1,1,1,1,1,1,6),(-0.94142984443141,-0.940000000000001,
-0.935000000000001,-0.930000000000001,-0.925000000000001,-0.920000000000001,
-0.915000000000001,-0.910000000000001,-0.905000000000001,-0.900000000000001,
-0.895000000000001,-0.890000000000001,-0.885000000000001,-0.880000000000001,
-0.875000000000001,-0.870000000000001,-0.865000000000001,-0.860000000000001,
-0.855000000000001,-0.850000000000001,-0.845000000000001,-0.840000000000001,
-0.835000000000001,-0.830000000000001,-0.825000000000001,-0.820000000000001,
-0.815000000000001,-0.810000000000001,-0.805000000000001,-0.800000000000001,
-0.795000000000001,-0.790000000000001,-0.785000000000001,-0.780000000000001,
-0.775000000000001,-0.770000000000001,-0.765000000000001,-0.760000000000001,
-0.755000000000001,-0.750000000000001,-0.745000000000001,-0.740000000000001,
-0.735000000000001,-0.730000000000001,-0.725000000000001,-0.720000000000001,
-0.715000000000001,-0.710000000000001,-0.705000000000001,-0.700000000000001,
-0.695000000000001,-0.690000000000001,-0.685,-0.68,-0.675,-0.67,-0.665,
-0.66,-0.655,-0.65,-0.645,-0.64,-0.635,-0.63,-0.625,-0.62,-0.615,-0.61,
-0.605,-0.6,-0.595,-0.59,-0.585,-0.58,-0.575,-0.57,-0.565,-0.56,-0.555,
-0.55,-0.545,-0.54,-0.535,-0.53,-0.525,-0.52,-0.515,-0.51,-0.505,-0.5,-0.495,
-0.49,-0.485,-0.48,-0.475,-0.47,-0.465,-0.46,-0.455,-0.45,-0.445,-0.44,
-0.435,-0.43,-0.425,-0.42,-0.415,-0.41,-0.405,-0.4,-0.395,-0.39,-0.385,
-0.38,-0.375,-0.37,-0.365,-0.36,-0.355,-0.35,-0.345,-0.34,-0.335,-0.33,
-0.325,-0.32,-0.315,-0.31,-0.305,-0.3,-0.295,-0.29,-0.285,-0.28,-0.275,
-0.27,-0.265,-0.26,-0.255,-0.25,-0.245,-0.24,-0.235,-0.23,-0.225,-0.22,
-0.215,-0.21,-0.205,-0.2,-0.195,-0.19,-0.185,-0.18,-0.175,-0.17,-0.165,
-0.16,-0.155,-0.15,-0.145,-0.14,-0.135,-0.13,-0.125,-0.12,-0.115,-0.11,
-0.105,-0.1,-0.095,-0.09,-0.085,-0.08,-0.075,-0.07,-0.065,-0.06,-0.055,
-0.05,-0.045,-0.04,-0.035,-0.03,-0.025,-0.02,-0.015,-0.01,-0.005,0.),
 .UNSPECIFIED.)
CURVE()
GEOMETRIC_REPRESENTATION_ITEM()
RATIONAL_B_SPLINE_CURVE((1.,1.,1.,1.,1.,1.,1.,1.,1.,1.,1.,1.,1.,1.,1.,1.,
1.,1.,1.,1.,1.,1.,1.,1.,1.,1.,1.,1.,1.,1.,1.,1.,1.,1.,1.,1.,1.,1.,1.,1.,
1.,1.,1.,1.,1.,1.,1.,1.,1.,1.,1.,1.,1.,1.,1.,1.,1.,1.,1.,1.,1.,1.,1.,1.,
1.,1.,1.,1.,1.,1.,1.,1.,1.,1.,1.,1.,1.,1.,1.,1.,1.,1.,1.,1.,1.,1.,1.,1.,
1.,1.,1.,1.,1.,1.,1.,1.,1.,1.,1.,1.,1.,1.,1.,1.,1.,1.,1.,1.,1.,1.,1.,1.,
1.,1.,1.,1.,1.,1.,1.,1.,1.,1.,1.,1.,1.,1.,1.,1.,1.,1.,1.,1.,1.,1.,1.,1.,
1.,1.,1.,1.,1.,1.,1.,1.,1.,1.,1.,1.,1.,1.,1.,1.,1.,1.,1.,1.,1.,1.,1.,1.,
1.,1.,1.,1.,1.,1.,1.,1.,1.,1.,1.,1.,1.,1.,1.,1.,1.,1.,1.,1.,1.,1.,1.,1.,
1.,1.,1.,1.,1.,1.,1.,1.,1.,1.))
REPRESENTATION_ITEM('')
);
#477=(
BOUNDED_CURVE()
B_SPLINE_CURVE(5,(#86185,#86186,#86187,#86188,#86189,#86190,#86191,#86192,
#86193,#86194,#86195,#86196,#86197,#86198,#86199,#86200,#86201,#86202,#86203,
#86204,#86205,#86206,#86207,#86208,#86209,#86210,#86211,#86212,#86213,#86214,
#86215,#86216,#86217,#86218,#86219,#86220,#86221,#86222,#86223,#86224,#86225,
#86226,#86227,#86228,#86229,#86230,#86231,#86232,#86233,#86234,#86235,#86236,
#86237,#86238,#86239,#86240,#86241,#86242,#86243,#86244,#86245,#86246,#86247,
#86248,#86249,#86250,#86251,#86252,#86253,#86254,#86255,#86256,#86257,#86258,
#86259,#86260,#86261,#86262,#86263,#86264,#86265,#86266,#86267,#86268,#86269,
#86270,#86271,#86272,#86273,#86274,#86275,#86276,#86277,#86278,#86279,#86280,
#86281,#86282,#86283,#86284,#86285,#86286,#86287,#86288,#86289,#86290,#86291,
#86292,#86293,#86294,#86295,#86296,#86297,#86298,#86299,#86300,#86301,#86302,
#86303,#86304,#86305,#86306,#86307,#86308,#86309,#86310,#86311,#86312,#86313,
#86314,#86315,#86316,#86317,#86318,#86319,#86320,#86321,#86322,#86323,#86324,
#86325,#86326,#86327,#86328,#86329,#86330,#86331,#86332,#86333,#86334,#86335,
#86336,#86337,#86338,#86339,#86340,#86341,#86342,#86343,#86344,#86345,#86346,
#86347,#86348,#86349,#86350,#86351,#86352,#86353,#86354,#86355,#86356,#86357,
#86358,#86359,#86360,#86361,#86362,#86363,#86364,#86365,#86366,#86367,#86368,
#86369,#86370,#86371,#86372,#86373,#86374,#86375,#86376,#86377,#86378),
 .UNSPECIFIED.,.F.,.F.)
B_SPLINE_CURVE_WITH_KNOTS((6,1,1,1,1,1,1,1,1,1,1,1,1,1,1,1,1,1,1,1,1,1,
1,1,1,1,1,1,1,1,1,1,1,1,1,1,1,1,1,1,1,1,1,1,1,1,1,1,1,1,1,1,1,1,1,1,1,1,
1,1,1,1,1,1,1,1,1,1,1,1,1,1,1,1,1,1,1,1,1,1,1,1,1,1,1,1,1,1,1,1,1,1,1,1,
1,1,1,1,1,1,1,1,1,1,1,1,1,1,1,1,1,1,1,1,1,1,1,1,1,1,1,1,1,1,1,1,1,1,1,1,
1,1,1,1,1,1,1,1,1,1,1,1,1,1,1,1,1,1,1,1,1,1,1,1,1,1,1,1,1,1,1,1,1,1,1,1,
1,1,1,1,1,1,1,1,1,1,1,1,1,1,1,1,1,1,1,1,1,1,1,6),(0.,0.005,0.01,0.015,0.02,
0.025,0.03,0.035,0.04,0.045,0.05,0.055,0.06,0.065,0.07,0.075,0.08,0.085,
0.09,0.095,0.1,0.105,0.11,0.115,0.12,0.125,0.13,0.135,0.14,0.145,0.15,0.155,
0.16,0.165,0.17,0.175,0.18,0.185,0.19,0.195,0.2,0.205,0.21,0.215,0.22,0.225,
0.23,0.235,0.24,0.245,0.25,0.255,0.26,0.265,0.27,0.275,0.28,0.285,0.29,
0.295,0.3,0.305,0.31,0.315,0.32,0.325,0.33,0.335,0.34,0.345,0.35,0.355,
0.36,0.365,0.37,0.375,0.38,0.385,0.39,0.395,0.4,0.405,0.41,0.415,0.42,0.425,
0.43,0.435,0.44,0.445,0.45,0.455,0.46,0.465,0.47,0.475,0.48,0.485,0.49,
0.495,0.5,0.505,0.51,0.515,0.52,0.525,0.53,0.535,0.54,0.545,0.55,0.555,
0.56,0.565,0.57,0.575,0.58,0.585,0.59,0.595,0.6,0.605,0.61,0.615,0.62,0.625,
0.63,0.635,0.64,0.645,0.65,0.655,0.66,0.665,0.67,0.675,0.68,0.685,0.690000000000001,
0.695000000000001,0.700000000000001,0.705000000000001,0.710000000000001,
0.715000000000001,0.720000000000001,0.725000000000001,0.730000000000001,
0.735000000000001,0.740000000000001,0.745000000000001,0.750000000000001,
0.755000000000001,0.760000000000001,0.765000000000001,0.770000000000001,
0.775000000000001,0.780000000000001,0.785000000000001,0.790000000000001,
0.795000000000001,0.800000000000001,0.805000000000001,0.810000000000001,
0.815000000000001,0.820000000000001,0.825000000000001,0.830000000000001,
0.835000000000001,0.840000000000001,0.845000000000001,0.850000000000001,
0.855000000000001,0.860000000000001,0.865000000000001,0.870000000000001,
0.875000000000001,0.880000000000001,0.885000000000001,0.890000000000001,
0.895000000000001,0.900000000000001,0.905000000000001,0.910000000000001,
0.915000000000001,0.920000000000001,0.925000000000001,0.930000000000001,
0.935000000000001,0.940000000000001,0.941429844431322),.UNSPECIFIED.)
CURVE()
GEOMETRIC_REPRESENTATION_ITEM()
RATIONAL_B_SPLINE_CURVE((1.,1.,1.,1.,1.,1.,1.,1.,1.,1.,1.,1.,1.,1.,1.,1.,
1.,1.,1.,1.,1.,1.,1.,1.,1.,1.,1.,1.,1.,1.,1.,1.,1.,1.,1.,1.,1.,1.,1.,1.,
1.,1.,1.,1.,1.,1.,1.,1.,1.,1.,1.,1.,1.,1.,1.,1.,1.,1.,1.,1.,1.,1.,1.,1.,
1.,1.,1.,1.,1.,1.,1.,1.,1.,1.,1.,1.,1.,1.,1.,1.,1.,1.,1.,1.,1.,1.,1.,1.,
1.,1.,1.,1.,1.,1.,1.,1.,1.,1.,1.,1.,1.,1.,1.,1.,1.,1.,1.,1.,1.,1.,1.,1.,
1.,1.,1.,1.,1.,1.,1.,1.,1.,1.,1.,1.,1.,1.,1.,1.,1.,1.,1.,1.,1.,1.,1.,1.,
1.,1.,1.,1.,1.,1.,1.,1.,1.,1.,1.,1.,1.,1.,1.,1.,1.,1.,1.,1.,1.,1.,1.,1.,
1.,1.,1.,1.,1.,1.,1.,1.,1.,1.,1.,1.,1.,1.,1.,1.,1.,1.,1.,1.,1.,1.,1.,1.,
1.,1.,1.,1.,1.,1.,1.,1.,1.,1.))
REPRESENTATION_ITEM('')
);
#478=(
BOUNDED_CURVE()
B_SPLINE_CURVE(5,(#86381,#86382,#86383,#86384,#86385,#86386,#86387,#86388,
#86389,#86390,#86391,#86392,#86393,#86394,#86395,#86396,#86397,#86398,#86399,
#86400,#86401,#86402,#86403,#86404,#86405,#86406,#86407,#86408,#86409,#86410,
#86411,#86412,#86413,#86414,#86415,#86416,#86417,#86418,#86419,#86420,#86421,
#86422,#86423,#86424,#86425,#86426,#86427,#86428,#86429,#86430,#86431,#86432,
#86433,#86434,#86435,#86436,#86437,#86438,#86439,#86440,#86441,#86442,#86443,
#86444,#86445,#86446,#86447,#86448,#86449,#86450,#86451,#86452,#86453,#86454,
#86455,#86456,#86457,#86458,#86459,#86460,#86461,#86462,#86463,#86464,#86465,
#86466,#86467,#86468,#86469,#86470,#86471,#86472,#86473,#86474,#86475,#86476,
#86477,#86478,#86479,#86480,#86481,#86482,#86483,#86484,#86485,#86486,#86487,
#86488,#86489,#86490,#86491,#86492,#86493,#86494,#86495,#86496,#86497,#86498,
#86499,#86500,#86501,#86502,#86503,#86504,#86505,#86506,#86507,#86508,#86509,
#86510,#86511,#86512,#86513,#86514,#86515,#86516,#86517,#86518,#86519,#86520,
#86521,#86522,#86523,#86524,#86525,#86526,#86527,#86528,#86529,#86530,#86531,
#86532,#86533,#86534,#86535,#86536,#86537,#86538,#86539,#86540,#86541,#86542,
#86543,#86544,#86545,#86546,#86547,#86548,#86549,#86550,#86551,#86552,#86553,
#86554,#86555,#86556,#86557,#86558,#86559,#86560,#86561,#86562,#86563,#86564,
#86565,#86566,#86567,#86568,#86569,#86570,#86571,#86572,#86573,#86574),
 .UNSPECIFIED.,.F.,.F.)
B_SPLINE_CURVE_WITH_KNOTS((6,1,1,1,1,1,1,1,1,1,1,1,1,1,1,1,1,1,1,1,1,1,
1,1,1,1,1,1,1,1,1,1,1,1,1,1,1,1,1,1,1,1,1,1,1,1,1,1,1,1,1,1,1,1,1,1,1,1,
1,1,1,1,1,1,1,1,1,1,1,1,1,1,1,1,1,1,1,1,1,1,1,1,1,1,1,1,1,1,1,1,1,1,1,1,
1,1,1,1,1,1,1,1,1,1,1,1,1,1,1,1,1,1,1,1,1,1,1,1,1,1,1,1,1,1,1,1,1,1,1,1,
1,1,1,1,1,1,1,1,1,1,1,1,1,1,1,1,1,1,1,1,1,1,1,1,1,1,1,1,1,1,1,1,1,1,1,1,
1,1,1,1,1,1,1,1,1,1,1,1,1,1,1,1,1,1,1,1,1,1,1,6),(-0.941429844431322,-0.940000000000001,
-0.935000000000001,-0.930000000000001,-0.925000000000001,-0.920000000000001,
-0.915000000000001,-0.910000000000001,-0.905000000000001,-0.900000000000001,
-0.895000000000001,-0.890000000000001,-0.885000000000001,-0.880000000000001,
-0.875000000000001,-0.870000000000001,-0.865000000000001,-0.860000000000001,
-0.855000000000001,-0.850000000000001,-0.845000000000001,-0.840000000000001,
-0.835000000000001,-0.830000000000001,-0.825000000000001,-0.820000000000001,
-0.815000000000001,-0.810000000000001,-0.805000000000001,-0.800000000000001,
-0.795000000000001,-0.790000000000001,-0.785000000000001,-0.780000000000001,
-0.775000000000001,-0.770000000000001,-0.765000000000001,-0.760000000000001,
-0.755000000000001,-0.750000000000001,-0.745000000000001,-0.740000000000001,
-0.735000000000001,-0.730000000000001,-0.725000000000001,-0.720000000000001,
-0.715000000000001,-0.710000000000001,-0.705000000000001,-0.700000000000001,
-0.695000000000001,-0.690000000000001,-0.685,-0.68,-0.675,-0.67,-0.665,
-0.66,-0.655,-0.65,-0.645,-0.64,-0.635,-0.63,-0.625,-0.62,-0.615,-0.61,
-0.605,-0.6,-0.595,-0.59,-0.585,-0.58,-0.575,-0.57,-0.565,-0.56,-0.555,
-0.55,-0.545,-0.54,-0.535,-0.53,-0.525,-0.52,-0.515,-0.51,-0.505,-0.5,-0.495,
-0.49,-0.485,-0.48,-0.475,-0.47,-0.465,-0.46,-0.455,-0.45,-0.445,-0.44,
-0.435,-0.43,-0.425,-0.42,-0.415,-0.41,-0.405,-0.4,-0.395,-0.39,-0.385,
-0.38,-0.375,-0.37,-0.365,-0.36,-0.355,-0.35,-0.345,-0.34,-0.335,-0.33,
-0.325,-0.32,-0.315,-0.31,-0.305,-0.3,-0.295,-0.29,-0.285,-0.28,-0.275,
-0.27,-0.265,-0.26,-0.255,-0.25,-0.245,-0.24,-0.235,-0.23,-0.225,-0.22,
-0.215,-0.21,-0.205,-0.2,-0.195,-0.19,-0.185,-0.18,-0.175,-0.17,-0.165,
-0.16,-0.155,-0.15,-0.145,-0.14,-0.135,-0.13,-0.125,-0.12,-0.115,-0.11,
-0.105,-0.1,-0.095,-0.09,-0.085,-0.08,-0.075,-0.07,-0.065,-0.06,-0.055,
-0.05,-0.045,-0.04,-0.035,-0.03,-0.025,-0.02,-0.015,-0.01,-0.005,0.),
 .UNSPECIFIED.)
CURVE()
GEOMETRIC_REPRESENTATION_ITEM()
RATIONAL_B_SPLINE_CURVE((1.,1.,1.,1.,1.,1.,1.,1.,1.,1.,1.,1.,1.,1.,1.,1.,
1.,1.,1.,1.,1.,1.,1.,1.,1.,1.,1.,1.,1.,1.,1.,1.,1.,1.,1.,1.,1.,1.,1.,1.,
1.,1.,1.,1.,1.,1.,1.,1.,1.,1.,1.,1.,1.,1.,1.,1.,1.,1.,1.,1.,1.,1.,1.,1.,
1.,1.,1.,1.,1.,1.,1.,1.,1.,1.,1.,1.,1.,1.,1.,1.,1.,1.,1.,1.,1.,1.,1.,1.,
1.,1.,1.,1.,1.,1.,1.,1.,1.,1.,1.,1.,1.,1.,1.,1.,1.,1.,1.,1.,1.,1.,1.,1.,
1.,1.,1.,1.,1.,1.,1.,1.,1.,1.,1.,1.,1.,1.,1.,1.,1.,1.,1.,1.,1.,1.,1.,1.,
1.,1.,1.,1.,1.,1.,1.,1.,1.,1.,1.,1.,1.,1.,1.,1.,1.,1.,1.,1.,1.,1.,1.,1.,
1.,1.,1.,1.,1.,1.,1.,1.,1.,1.,1.,1.,1.,1.,1.,1.,1.,1.,1.,1.,1.,1.,1.,1.,
1.,1.,1.,1.,1.,1.,1.,1.,1.,1.))
REPRESENTATION_ITEM('')
);
#479=(
BOUNDED_CURVE()
B_SPLINE_CURVE(5,(#87081,#87082,#87083,#87084,#87085,#87086,#87087,#87088,
#87089,#87090,#87091,#87092,#87093,#87094,#87095,#87096,#87097,#87098,#87099,
#87100,#87101,#87102,#87103,#87104,#87105,#87106,#87107,#87108,#87109,#87110,
#87111,#87112,#87113,#87114,#87115,#87116,#87117,#87118,#87119,#87120,#87121,
#87122,#87123,#87124,#87125,#87126,#87127,#87128,#87129,#87130,#87131,#87132,
#87133,#87134,#87135,#87136,#87137,#87138,#87139,#87140,#87141,#87142,#87143,
#87144,#87145,#87146,#87147,#87148,#87149,#87150,#87151,#87152,#87153,#87154,
#87155,#87156,#87157,#87158,#87159,#87160,#87161,#87162,#87163,#87164,#87165,
#87166,#87167,#87168,#87169,#87170,#87171,#87172,#87173,#87174,#87175,#87176,
#87177,#87178,#87179,#87180,#87181,#87182,#87183,#87184,#87185,#87186,#87187,
#87188,#87189,#87190,#87191,#87192,#87193,#87194,#87195,#87196,#87197,#87198,
#87199,#87200,#87201,#87202,#87203,#87204,#87205,#87206,#87207,#87208,#87209,
#87210,#87211,#87212,#87213,#87214,#87215,#87216,#87217,#87218,#87219,#87220,
#87221,#87222,#87223,#87224,#87225,#87226,#87227,#87228,#87229,#87230,#87231,
#87232,#87233,#87234,#87235,#87236,#87237,#87238,#87239,#87240,#87241,#87242,
#87243,#87244,#87245,#87246,#87247,#87248,#87249,#87250,#87251,#87252,#87253,
#87254,#87255,#87256,#87257,#87258,#87259,#87260,#87261,#87262,#87263,#87264,
#87265,#87266,#87267,#87268,#87269,#87270,#87271,#87272,#87273,#87274),
 .UNSPECIFIED.,.F.,.F.)
B_SPLINE_CURVE_WITH_KNOTS((6,1,1,1,1,1,1,1,1,1,1,1,1,1,1,1,1,1,1,1,1,1,
1,1,1,1,1,1,1,1,1,1,1,1,1,1,1,1,1,1,1,1,1,1,1,1,1,1,1,1,1,1,1,1,1,1,1,1,
1,1,1,1,1,1,1,1,1,1,1,1,1,1,1,1,1,1,1,1,1,1,1,1,1,1,1,1,1,1,1,1,1,1,1,1,
1,1,1,1,1,1,1,1,1,1,1,1,1,1,1,1,1,1,1,1,1,1,1,1,1,1,1,1,1,1,1,1,1,1,1,1,
1,1,1,1,1,1,1,1,1,1,1,1,1,1,1,1,1,1,1,1,1,1,1,1,1,1,1,1,1,1,1,1,1,1,1,1,
1,1,1,1,1,1,1,1,1,1,1,1,1,1,1,1,1,1,1,1,1,1,1,6),(0.,0.005,0.01,0.015,0.02,
0.025,0.03,0.035,0.04,0.045,0.05,0.055,0.06,0.065,0.07,0.075,0.08,0.085,
0.09,0.095,0.1,0.105,0.11,0.115,0.12,0.125,0.13,0.135,0.14,0.145,0.15,0.155,
0.16,0.165,0.17,0.175,0.18,0.185,0.19,0.195,0.2,0.205,0.21,0.215,0.22,0.225,
0.23,0.235,0.24,0.245,0.25,0.255,0.26,0.265,0.27,0.275,0.28,0.285,0.29,
0.295,0.3,0.305,0.31,0.315,0.32,0.325,0.33,0.335,0.34,0.345,0.35,0.355,
0.36,0.365,0.37,0.375,0.38,0.385,0.39,0.395,0.4,0.405,0.41,0.415,0.42,0.425,
0.43,0.435,0.44,0.445,0.45,0.455,0.46,0.465,0.47,0.475,0.48,0.485,0.49,
0.495,0.5,0.505,0.51,0.515,0.52,0.525,0.53,0.535,0.54,0.545,0.55,0.555,
0.56,0.565,0.57,0.575,0.58,0.585,0.59,0.595,0.6,0.605,0.61,0.615,0.62,0.625,
0.63,0.635,0.64,0.645,0.65,0.655,0.66,0.665,0.67,0.675,0.68,0.685,0.690000000000001,
0.695000000000001,0.700000000000001,0.705000000000001,0.710000000000001,
0.715000000000001,0.720000000000001,0.725000000000001,0.730000000000001,
0.735000000000001,0.740000000000001,0.745000000000001,0.750000000000001,
0.755000000000001,0.760000000000001,0.765000000000001,0.770000000000001,
0.775000000000001,0.780000000000001,0.785000000000001,0.790000000000001,
0.795000000000001,0.800000000000001,0.805000000000001,0.810000000000001,
0.815000000000001,0.820000000000001,0.825000000000001,0.830000000000001,
0.835000000000001,0.840000000000001,0.845000000000001,0.850000000000001,
0.855000000000001,0.860000000000001,0.865000000000001,0.870000000000001,
0.875000000000001,0.880000000000001,0.885000000000001,0.890000000000001,
0.895000000000001,0.900000000000001,0.905000000000001,0.910000000000001,
0.915000000000001,0.920000000000001,0.925000000000001,0.930000000000001,
0.935000000000001,0.940000000000001,0.941429844431316),.UNSPECIFIED.)
CURVE()
GEOMETRIC_REPRESENTATION_ITEM()
RATIONAL_B_SPLINE_CURVE((1.,1.,1.,1.,1.,1.,1.,1.,1.,1.,1.,1.,1.,1.,1.,1.,
1.,1.,1.,1.,1.,1.,1.,1.,1.,1.,1.,1.,1.,1.,1.,1.,1.,1.,1.,1.,1.,1.,1.,1.,
1.,1.,1.,1.,1.,1.,1.,1.,1.,1.,1.,1.,1.,1.,1.,1.,1.,1.,1.,1.,1.,1.,1.,1.,
1.,1.,1.,1.,1.,1.,1.,1.,1.,1.,1.,1.,1.,1.,1.,1.,1.,1.,1.,1.,1.,1.,1.,1.,
1.,1.,1.,1.,1.,1.,1.,1.,1.,1.,1.,1.,1.,1.,1.,1.,1.,1.,1.,1.,1.,1.,1.,1.,
1.,1.,1.,1.,1.,1.,1.,1.,1.,1.,1.,1.,1.,1.,1.,1.,1.,1.,1.,1.,1.,1.,1.,1.,
1.,1.,1.,1.,1.,1.,1.,1.,1.,1.,1.,1.,1.,1.,1.,1.,1.,1.,1.,1.,1.,1.,1.,1.,
1.,1.,1.,1.,1.,1.,1.,1.,1.,1.,1.,1.,1.,1.,1.,1.,1.,1.,1.,1.,1.,1.,1.,1.,
1.,1.,1.,1.,1.,1.,1.,1.,1.,1.))
REPRESENTATION_ITEM('')
);
#480=(
BOUNDED_CURVE()
B_SPLINE_CURVE(5,(#87277,#87278,#87279,#87280,#87281,#87282,#87283,#87284,
#87285,#87286,#87287,#87288,#87289,#87290,#87291,#87292,#87293,#87294,#87295,
#87296,#87297,#87298,#87299,#87300,#87301,#87302,#87303,#87304,#87305,#87306,
#87307,#87308,#87309,#87310,#87311,#87312,#87313,#87314,#87315,#87316,#87317,
#87318,#87319,#87320,#87321,#87322,#87323,#87324,#87325,#87326,#87327,#87328,
#87329,#87330,#87331,#87332,#87333,#87334,#87335,#87336,#87337,#87338,#87339,
#87340,#87341,#87342,#87343,#87344,#87345,#87346,#87347,#87348,#87349,#87350,
#87351,#87352,#87353,#87354,#87355,#87356,#87357,#87358,#87359,#87360,#87361,
#87362,#87363,#87364,#87365,#87366,#87367,#87368,#87369,#87370,#87371,#87372,
#87373,#87374,#87375,#87376,#87377,#87378,#87379,#87380,#87381,#87382,#87383,
#87384,#87385,#87386,#87387,#87388,#87389,#87390,#87391,#87392,#87393,#87394,
#87395,#87396,#87397,#87398,#87399,#87400,#87401,#87402,#87403,#87404,#87405,
#87406,#87407,#87408,#87409,#87410,#87411,#87412,#87413,#87414,#87415,#87416,
#87417,#87418,#87419,#87420,#87421,#87422,#87423,#87424,#87425,#87426,#87427,
#87428,#87429,#87430,#87431,#87432,#87433,#87434,#87435,#87436,#87437,#87438,
#87439,#87440,#87441,#87442,#87443,#87444,#87445,#87446,#87447,#87448,#87449,
#87450,#87451,#87452,#87453,#87454,#87455,#87456,#87457,#87458,#87459,#87460,
#87461,#87462,#87463,#87464,#87465,#87466,#87467,#87468,#87469,#87470),
 .UNSPECIFIED.,.F.,.F.)
B_SPLINE_CURVE_WITH_KNOTS((6,1,1,1,1,1,1,1,1,1,1,1,1,1,1,1,1,1,1,1,1,1,
1,1,1,1,1,1,1,1,1,1,1,1,1,1,1,1,1,1,1,1,1,1,1,1,1,1,1,1,1,1,1,1,1,1,1,1,
1,1,1,1,1,1,1,1,1,1,1,1,1,1,1,1,1,1,1,1,1,1,1,1,1,1,1,1,1,1,1,1,1,1,1,1,
1,1,1,1,1,1,1,1,1,1,1,1,1,1,1,1,1,1,1,1,1,1,1,1,1,1,1,1,1,1,1,1,1,1,1,1,
1,1,1,1,1,1,1,1,1,1,1,1,1,1,1,1,1,1,1,1,1,1,1,1,1,1,1,1,1,1,1,1,1,1,1,1,
1,1,1,1,1,1,1,1,1,1,1,1,1,1,1,1,1,1,1,1,1,1,1,6),(-0.941429844431316,-0.940000000000001,
-0.935000000000001,-0.930000000000001,-0.925000000000001,-0.920000000000001,
-0.915000000000001,-0.910000000000001,-0.905000000000001,-0.900000000000001,
-0.895000000000001,-0.890000000000001,-0.885000000000001,-0.880000000000001,
-0.875000000000001,-0.870000000000001,-0.865000000000001,-0.860000000000001,
-0.855000000000001,-0.850000000000001,-0.845000000000001,-0.840000000000001,
-0.835000000000001,-0.830000000000001,-0.825000000000001,-0.820000000000001,
-0.815000000000001,-0.810000000000001,-0.805000000000001,-0.800000000000001,
-0.795000000000001,-0.790000000000001,-0.785000000000001,-0.780000000000001,
-0.775000000000001,-0.770000000000001,-0.765000000000001,-0.760000000000001,
-0.755000000000001,-0.750000000000001,-0.745000000000001,-0.740000000000001,
-0.735000000000001,-0.730000000000001,-0.725000000000001,-0.720000000000001,
-0.715000000000001,-0.710000000000001,-0.705000000000001,-0.700000000000001,
-0.695000000000001,-0.690000000000001,-0.685,-0.68,-0.675,-0.67,-0.665,
-0.66,-0.655,-0.65,-0.645,-0.64,-0.635,-0.63,-0.625,-0.62,-0.615,-0.61,
-0.605,-0.6,-0.595,-0.59,-0.585,-0.58,-0.575,-0.57,-0.565,-0.56,-0.555,
-0.55,-0.545,-0.54,-0.535,-0.53,-0.525,-0.52,-0.515,-0.51,-0.505,-0.5,-0.495,
-0.49,-0.485,-0.48,-0.475,-0.47,-0.465,-0.46,-0.455,-0.45,-0.445,-0.44,
-0.435,-0.43,-0.425,-0.42,-0.415,-0.41,-0.405,-0.4,-0.395,-0.39,-0.385,
-0.38,-0.375,-0.37,-0.365,-0.36,-0.355,-0.35,-0.345,-0.34,-0.335,-0.33,
-0.325,-0.32,-0.315,-0.31,-0.305,-0.3,-0.295,-0.29,-0.285,-0.28,-0.275,
-0.27,-0.265,-0.26,-0.255,-0.25,-0.245,-0.24,-0.235,-0.23,-0.225,-0.22,
-0.215,-0.21,-0.205,-0.2,-0.195,-0.19,-0.185,-0.18,-0.175,-0.17,-0.165,
-0.16,-0.155,-0.15,-0.145,-0.14,-0.135,-0.13,-0.125,-0.12,-0.115,-0.11,
-0.105,-0.1,-0.095,-0.09,-0.085,-0.08,-0.075,-0.07,-0.065,-0.06,-0.055,
-0.05,-0.045,-0.04,-0.035,-0.03,-0.025,-0.02,-0.015,-0.01,-0.005,0.),
 .UNSPECIFIED.)
CURVE()
GEOMETRIC_REPRESENTATION_ITEM()
RATIONAL_B_SPLINE_CURVE((1.,1.,1.,1.,1.,1.,1.,1.,1.,1.,1.,1.,1.,1.,1.,1.,
1.,1.,1.,1.,1.,1.,1.,1.,1.,1.,1.,1.,1.,1.,1.,1.,1.,1.,1.,1.,1.,1.,1.,1.,
1.,1.,1.,1.,1.,1.,1.,1.,1.,1.,1.,1.,1.,1.,1.,1.,1.,1.,1.,1.,1.,1.,1.,1.,
1.,1.,1.,1.,1.,1.,1.,1.,1.,1.,1.,1.,1.,1.,1.,1.,1.,1.,1.,1.,1.,1.,1.,1.,
1.,1.,1.,1.,1.,1.,1.,1.,1.,1.,1.,1.,1.,1.,1.,1.,1.,1.,1.,1.,1.,1.,1.,1.,
1.,1.,1.,1.,1.,1.,1.,1.,1.,1.,1.,1.,1.,1.,1.,1.,1.,1.,1.,1.,1.,1.,1.,1.,
1.,1.,1.,1.,1.,1.,1.,1.,1.,1.,1.,1.,1.,1.,1.,1.,1.,1.,1.,1.,1.,1.,1.,1.,
1.,1.,1.,1.,1.,1.,1.,1.,1.,1.,1.,1.,1.,1.,1.,1.,1.,1.,1.,1.,1.,1.,1.,1.,
1.,1.,1.,1.,1.,1.,1.,1.,1.,1.))
REPRESENTATION_ITEM('')
);
#481=(
BOUNDED_CURVE()
B_SPLINE_CURVE(5,(#87977,#87978,#87979,#87980,#87981,#87982,#87983,#87984,
#87985,#87986,#87987,#87988,#87989,#87990,#87991,#87992,#87993,#87994,#87995,
#87996,#87997,#87998,#87999,#88000,#88001,#88002,#88003,#88004,#88005,#88006,
#88007,#88008,#88009,#88010,#88011,#88012,#88013,#88014,#88015,#88016,#88017,
#88018,#88019,#88020,#88021,#88022,#88023,#88024,#88025,#88026,#88027,#88028,
#88029,#88030,#88031,#88032,#88033,#88034,#88035,#88036,#88037,#88038,#88039,
#88040,#88041,#88042,#88043,#88044,#88045,#88046,#88047,#88048,#88049,#88050,
#88051,#88052,#88053,#88054,#88055,#88056,#88057,#88058,#88059,#88060,#88061,
#88062,#88063,#88064,#88065,#88066,#88067,#88068,#88069,#88070,#88071,#88072,
#88073,#88074,#88075,#88076,#88077,#88078,#88079,#88080,#88081,#88082,#88083,
#88084,#88085,#88086,#88087,#88088,#88089,#88090,#88091,#88092,#88093,#88094,
#88095,#88096,#88097,#88098,#88099,#88100,#88101,#88102,#88103,#88104,#88105,
#88106,#88107,#88108,#88109,#88110,#88111,#88112,#88113,#88114,#88115,#88116,
#88117,#88118,#88119,#88120,#88121,#88122,#88123,#88124,#88125,#88126,#88127,
#88128,#88129,#88130,#88131,#88132,#88133,#88134,#88135,#88136,#88137,#88138,
#88139,#88140,#88141,#88142,#88143,#88144,#88145,#88146,#88147,#88148,#88149,
#88150,#88151,#88152,#88153,#88154,#88155,#88156,#88157,#88158,#88159,#88160,
#88161,#88162,#88163,#88164,#88165,#88166,#88167,#88168,#88169,#88170),
 .UNSPECIFIED.,.F.,.F.)
B_SPLINE_CURVE_WITH_KNOTS((6,1,1,1,1,1,1,1,1,1,1,1,1,1,1,1,1,1,1,1,1,1,
1,1,1,1,1,1,1,1,1,1,1,1,1,1,1,1,1,1,1,1,1,1,1,1,1,1,1,1,1,1,1,1,1,1,1,1,
1,1,1,1,1,1,1,1,1,1,1,1,1,1,1,1,1,1,1,1,1,1,1,1,1,1,1,1,1,1,1,1,1,1,1,1,
1,1,1,1,1,1,1,1,1,1,1,1,1,1,1,1,1,1,1,1,1,1,1,1,1,1,1,1,1,1,1,1,1,1,1,1,
1,1,1,1,1,1,1,1,1,1,1,1,1,1,1,1,1,1,1,1,1,1,1,1,1,1,1,1,1,1,1,1,1,1,1,1,
1,1,1,1,1,1,1,1,1,1,1,1,1,1,1,1,1,1,1,1,1,1,1,6),(0.,0.005,0.01,0.015,0.02,
0.025,0.03,0.035,0.04,0.045,0.05,0.055,0.06,0.065,0.07,0.075,0.08,0.085,
0.09,0.095,0.1,0.105,0.11,0.115,0.12,0.125,0.13,0.135,0.14,0.145,0.15,0.155,
0.16,0.165,0.17,0.175,0.18,0.185,0.19,0.195,0.2,0.205,0.21,0.215,0.22,0.225,
0.23,0.235,0.24,0.245,0.25,0.255,0.26,0.265,0.27,0.275,0.28,0.285,0.29,
0.295,0.3,0.305,0.31,0.315,0.32,0.325,0.33,0.335,0.34,0.345,0.35,0.355,
0.36,0.365,0.37,0.375,0.38,0.385,0.39,0.395,0.4,0.405,0.41,0.415,0.42,0.425,
0.43,0.435,0.44,0.445,0.45,0.455,0.46,0.465,0.47,0.475,0.48,0.485,0.49,
0.495,0.5,0.505,0.51,0.515,0.52,0.525,0.53,0.535,0.54,0.545,0.55,0.555,
0.56,0.565,0.57,0.575,0.58,0.585,0.59,0.595,0.6,0.605,0.61,0.615,0.62,0.625,
0.63,0.635,0.64,0.645,0.65,0.655,0.66,0.665,0.67,0.675,0.68,0.685,0.690000000000001,
0.695000000000001,0.700000000000001,0.705000000000001,0.710000000000001,
0.715000000000001,0.720000000000001,0.725000000000001,0.730000000000001,
0.735000000000001,0.740000000000001,0.745000000000001,0.750000000000001,
0.755000000000001,0.760000000000001,0.765000000000001,0.770000000000001,
0.775000000000001,0.780000000000001,0.785000000000001,0.790000000000001,
0.795000000000001,0.800000000000001,0.805000000000001,0.810000000000001,
0.815000000000001,0.820000000000001,0.825000000000001,0.830000000000001,
0.835000000000001,0.840000000000001,0.845000000000001,0.850000000000001,
0.855000000000001,0.860000000000001,0.865000000000001,0.870000000000001,
0.875000000000001,0.880000000000001,0.885000000000001,0.890000000000001,
0.895000000000001,0.900000000000001,0.905000000000001,0.910000000000001,
0.915000000000001,0.920000000000001,0.925000000000001,0.930000000000001,
0.935000000000001,0.940000000000001,0.941429844431396),.UNSPECIFIED.)
CURVE()
GEOMETRIC_REPRESENTATION_ITEM()
RATIONAL_B_SPLINE_CURVE((1.,1.,1.,1.,1.,1.,1.,1.,1.,1.,1.,1.,1.,1.,1.,1.,
1.,1.,1.,1.,1.,1.,1.,1.,1.,1.,1.,1.,1.,1.,1.,1.,1.,1.,1.,1.,1.,1.,1.,1.,
1.,1.,1.,1.,1.,1.,1.,1.,1.,1.,1.,1.,1.,1.,1.,1.,1.,1.,1.,1.,1.,1.,1.,1.,
1.,1.,1.,1.,1.,1.,1.,1.,1.,1.,1.,1.,1.,1.,1.,1.,1.,1.,1.,1.,1.,1.,1.,1.,
1.,1.,1.,1.,1.,1.,1.,1.,1.,1.,1.,1.,1.,1.,1.,1.,1.,1.,1.,1.,1.,1.,1.,1.,
1.,1.,1.,1.,1.,1.,1.,1.,1.,1.,1.,1.,1.,1.,1.,1.,1.,1.,1.,1.,1.,1.,1.,1.,
1.,1.,1.,1.,1.,1.,1.,1.,1.,1.,1.,1.,1.,1.,1.,1.,1.,1.,1.,1.,1.,1.,1.,1.,
1.,1.,1.,1.,1.,1.,1.,1.,1.,1.,1.,1.,1.,1.,1.,1.,1.,1.,1.,1.,1.,1.,1.,1.,
1.,1.,1.,1.,1.,1.,1.,1.,1.,1.))
REPRESENTATION_ITEM('')
);
#482=(
BOUNDED_CURVE()
B_SPLINE_CURVE(5,(#88173,#88174,#88175,#88176,#88177,#88178,#88179,#88180,
#88181,#88182,#88183,#88184,#88185,#88186,#88187,#88188,#88189,#88190,#88191,
#88192,#88193,#88194,#88195,#88196,#88197,#88198,#88199,#88200,#88201,#88202,
#88203,#88204,#88205,#88206,#88207,#88208,#88209,#88210,#88211,#88212,#88213,
#88214,#88215,#88216,#88217,#88218,#88219,#88220,#88221,#88222,#88223,#88224,
#88225,#88226,#88227,#88228,#88229,#88230,#88231,#88232,#88233,#88234,#88235,
#88236,#88237,#88238,#88239,#88240,#88241,#88242,#88243,#88244,#88245,#88246,
#88247,#88248,#88249,#88250,#88251,#88252,#88253,#88254,#88255,#88256,#88257,
#88258,#88259,#88260,#88261,#88262,#88263,#88264,#88265,#88266,#88267,#88268,
#88269,#88270,#88271,#88272,#88273,#88274,#88275,#88276,#88277,#88278,#88279,
#88280,#88281,#88282,#88283,#88284,#88285,#88286,#88287,#88288,#88289,#88290,
#88291,#88292,#88293,#88294,#88295,#88296,#88297,#88298,#88299,#88300,#88301,
#88302,#88303,#88304,#88305,#88306,#88307,#88308,#88309,#88310,#88311,#88312,
#88313,#88314,#88315,#88316,#88317,#88318,#88319,#88320,#88321,#88322,#88323,
#88324,#88325,#88326,#88327,#88328,#88329,#88330,#88331,#88332,#88333,#88334,
#88335,#88336,#88337,#88338,#88339,#88340,#88341,#88342,#88343,#88344,#88345,
#88346,#88347,#88348,#88349,#88350,#88351,#88352,#88353,#88354,#88355,#88356,
#88357,#88358,#88359,#88360,#88361,#88362,#88363,#88364,#88365,#88366),
 .UNSPECIFIED.,.F.,.F.)
B_SPLINE_CURVE_WITH_KNOTS((6,1,1,1,1,1,1,1,1,1,1,1,1,1,1,1,1,1,1,1,1,1,
1,1,1,1,1,1,1,1,1,1,1,1,1,1,1,1,1,1,1,1,1,1,1,1,1,1,1,1,1,1,1,1,1,1,1,1,
1,1,1,1,1,1,1,1,1,1,1,1,1,1,1,1,1,1,1,1,1,1,1,1,1,1,1,1,1,1,1,1,1,1,1,1,
1,1,1,1,1,1,1,1,1,1,1,1,1,1,1,1,1,1,1,1,1,1,1,1,1,1,1,1,1,1,1,1,1,1,1,1,
1,1,1,1,1,1,1,1,1,1,1,1,1,1,1,1,1,1,1,1,1,1,1,1,1,1,1,1,1,1,1,1,1,1,1,1,
1,1,1,1,1,1,1,1,1,1,1,1,1,1,1,1,1,1,1,1,1,1,1,6),(-0.941429844431407,-0.940000000000001,
-0.935000000000001,-0.930000000000001,-0.925000000000001,-0.920000000000001,
-0.915000000000001,-0.910000000000001,-0.905000000000001,-0.900000000000001,
-0.895000000000001,-0.890000000000001,-0.885000000000001,-0.880000000000001,
-0.875000000000001,-0.870000000000001,-0.865000000000001,-0.860000000000001,
-0.855000000000001,-0.850000000000001,-0.845000000000001,-0.840000000000001,
-0.835000000000001,-0.830000000000001,-0.825000000000001,-0.820000000000001,
-0.815000000000001,-0.810000000000001,-0.805000000000001,-0.800000000000001,
-0.795000000000001,-0.790000000000001,-0.785000000000001,-0.780000000000001,
-0.775000000000001,-0.770000000000001,-0.765000000000001,-0.760000000000001,
-0.755000000000001,-0.750000000000001,-0.745000000000001,-0.740000000000001,
-0.735000000000001,-0.730000000000001,-0.725000000000001,-0.720000000000001,
-0.715000000000001,-0.710000000000001,-0.705000000000001,-0.700000000000001,
-0.695000000000001,-0.690000000000001,-0.685,-0.68,-0.675,-0.67,-0.665,
-0.66,-0.655,-0.65,-0.645,-0.64,-0.635,-0.63,-0.625,-0.62,-0.615,-0.61,
-0.605,-0.6,-0.595,-0.59,-0.585,-0.58,-0.575,-0.57,-0.565,-0.56,-0.555,
-0.55,-0.545,-0.54,-0.535,-0.53,-0.525,-0.52,-0.515,-0.51,-0.505,-0.5,-0.495,
-0.49,-0.485,-0.48,-0.475,-0.47,-0.465,-0.46,-0.455,-0.45,-0.445,-0.44,
-0.435,-0.43,-0.425,-0.42,-0.415,-0.41,-0.405,-0.4,-0.395,-0.39,-0.385,
-0.38,-0.375,-0.37,-0.365,-0.36,-0.355,-0.35,-0.345,-0.34,-0.335,-0.33,
-0.325,-0.32,-0.315,-0.31,-0.305,-0.3,-0.295,-0.29,-0.285,-0.28,-0.275,
-0.27,-0.265,-0.26,-0.255,-0.25,-0.245,-0.24,-0.235,-0.23,-0.225,-0.22,
-0.215,-0.21,-0.205,-0.2,-0.195,-0.19,-0.185,-0.18,-0.175,-0.17,-0.165,
-0.16,-0.155,-0.15,-0.145,-0.14,-0.135,-0.13,-0.125,-0.12,-0.115,-0.11,
-0.105,-0.1,-0.095,-0.09,-0.085,-0.08,-0.075,-0.07,-0.065,-0.06,-0.055,
-0.05,-0.045,-0.04,-0.035,-0.03,-0.025,-0.02,-0.015,-0.01,-0.005,0.),
 .UNSPECIFIED.)
CURVE()
GEOMETRIC_REPRESENTATION_ITEM()
RATIONAL_B_SPLINE_CURVE((1.,1.,1.,1.,1.,1.,1.,1.,1.,1.,1.,1.,1.,1.,1.,1.,
1.,1.,1.,1.,1.,1.,1.,1.,1.,1.,1.,1.,1.,1.,1.,1.,1.,1.,1.,1.,1.,1.,1.,1.,
1.,1.,1.,1.,1.,1.,1.,1.,1.,1.,1.,1.,1.,1.,1.,1.,1.,1.,1.,1.,1.,1.,1.,1.,
1.,1.,1.,1.,1.,1.,1.,1.,1.,1.,1.,1.,1.,1.,1.,1.,1.,1.,1.,1.,1.,1.,1.,1.,
1.,1.,1.,1.,1.,1.,1.,1.,1.,1.,1.,1.,1.,1.,1.,1.,1.,1.,1.,1.,1.,1.,1.,1.,
1.,1.,1.,1.,1.,1.,1.,1.,1.,1.,1.,1.,1.,1.,1.,1.,1.,1.,1.,1.,1.,1.,1.,1.,
1.,1.,1.,1.,1.,1.,1.,1.,1.,1.,1.,1.,1.,1.,1.,1.,1.,1.,1.,1.,1.,1.,1.,1.,
1.,1.,1.,1.,1.,1.,1.,1.,1.,1.,1.,1.,1.,1.,1.,1.,1.,1.,1.,1.,1.,1.,1.,1.,
1.,1.,1.,1.,1.,1.,1.,1.,1.,1.))
REPRESENTATION_ITEM('')
);
#483=(
BOUNDED_CURVE()
B_SPLINE_CURVE(5,(#88873,#88874,#88875,#88876,#88877,#88878,#88879,#88880,
#88881,#88882,#88883,#88884,#88885,#88886,#88887,#88888,#88889,#88890,#88891,
#88892,#88893,#88894,#88895,#88896,#88897,#88898,#88899,#88900,#88901,#88902,
#88903,#88904,#88905,#88906,#88907,#88908,#88909,#88910,#88911,#88912,#88913,
#88914,#88915,#88916,#88917,#88918,#88919,#88920,#88921,#88922,#88923,#88924,
#88925,#88926,#88927,#88928,#88929,#88930,#88931,#88932,#88933,#88934,#88935,
#88936,#88937,#88938,#88939,#88940,#88941,#88942,#88943,#88944,#88945,#88946,
#88947,#88948,#88949,#88950,#88951,#88952,#88953,#88954,#88955,#88956,#88957,
#88958,#88959,#88960,#88961,#88962,#88963,#88964,#88965,#88966,#88967,#88968,
#88969,#88970,#88971,#88972,#88973,#88974,#88975,#88976,#88977,#88978,#88979,
#88980,#88981,#88982,#88983,#88984,#88985,#88986,#88987,#88988,#88989,#88990,
#88991,#88992,#88993,#88994,#88995,#88996,#88997,#88998,#88999,#89000,#89001,
#89002,#89003,#89004,#89005,#89006,#89007,#89008,#89009,#89010,#89011,#89012,
#89013,#89014,#89015,#89016,#89017,#89018,#89019,#89020,#89021,#89022,#89023,
#89024,#89025,#89026,#89027,#89028,#89029,#89030,#89031,#89032,#89033,#89034,
#89035,#89036,#89037,#89038,#89039,#89040,#89041,#89042,#89043,#89044,#89045,
#89046,#89047,#89048,#89049,#89050,#89051,#89052,#89053,#89054,#89055,#89056,
#89057,#89058,#89059,#89060,#89061,#89062,#89063,#89064,#89065,#89066),
 .UNSPECIFIED.,.F.,.F.)
B_SPLINE_CURVE_WITH_KNOTS((6,1,1,1,1,1,1,1,1,1,1,1,1,1,1,1,1,1,1,1,1,1,
1,1,1,1,1,1,1,1,1,1,1,1,1,1,1,1,1,1,1,1,1,1,1,1,1,1,1,1,1,1,1,1,1,1,1,1,
1,1,1,1,1,1,1,1,1,1,1,1,1,1,1,1,1,1,1,1,1,1,1,1,1,1,1,1,1,1,1,1,1,1,1,1,
1,1,1,1,1,1,1,1,1,1,1,1,1,1,1,1,1,1,1,1,1,1,1,1,1,1,1,1,1,1,1,1,1,1,1,1,
1,1,1,1,1,1,1,1,1,1,1,1,1,1,1,1,1,1,1,1,1,1,1,1,1,1,1,1,1,1,1,1,1,1,1,1,
1,1,1,1,1,1,1,1,1,1,1,1,1,1,1,1,1,1,1,1,1,1,1,6),(0.,0.005,0.01,0.015,0.02,
0.025,0.03,0.035,0.04,0.045,0.05,0.055,0.06,0.065,0.07,0.075,0.08,0.085,
0.09,0.095,0.1,0.105,0.11,0.115,0.12,0.125,0.13,0.135,0.14,0.145,0.15,0.155,
0.16,0.165,0.17,0.175,0.18,0.185,0.19,0.195,0.2,0.205,0.21,0.215,0.22,0.225,
0.23,0.235,0.24,0.245,0.25,0.255,0.26,0.265,0.27,0.275,0.28,0.285,0.29,
0.295,0.3,0.305,0.31,0.315,0.32,0.325,0.33,0.335,0.34,0.345,0.35,0.355,
0.36,0.365,0.37,0.375,0.38,0.385,0.39,0.395,0.4,0.405,0.41,0.415,0.42,0.425,
0.43,0.435,0.44,0.445,0.45,0.455,0.46,0.465,0.47,0.475,0.48,0.485,0.49,
0.495,0.5,0.505,0.51,0.515,0.52,0.525,0.53,0.535,0.54,0.545,0.55,0.555,
0.56,0.565,0.57,0.575,0.58,0.585,0.59,0.595,0.6,0.605,0.61,0.615,0.62,0.625,
0.63,0.635,0.64,0.645,0.65,0.655,0.66,0.665,0.67,0.675,0.68,0.685,0.690000000000001,
0.695000000000001,0.700000000000001,0.705000000000001,0.710000000000001,
0.715000000000001,0.720000000000001,0.725000000000001,0.730000000000001,
0.735000000000001,0.740000000000001,0.745000000000001,0.750000000000001,
0.755000000000001,0.760000000000001,0.765000000000001,0.770000000000001,
0.775000000000001,0.780000000000001,0.785000000000001,0.790000000000001,
0.795000000000001,0.800000000000001,0.805000000000001,0.810000000000001,
0.815000000000001,0.820000000000001,0.825000000000001,0.830000000000001,
0.835000000000001,0.840000000000001,0.845000000000001,0.850000000000001,
0.855000000000001,0.860000000000001,0.865000000000001,0.870000000000001,
0.875000000000001,0.880000000000001,0.885000000000001,0.890000000000001,
0.895000000000001,0.900000000000001,0.905000000000001,0.910000000000001,
0.915000000000001,0.920000000000001,0.925000000000001,0.930000000000001,
0.935000000000001,0.940000000000001,0.941429844431366),.UNSPECIFIED.)
CURVE()
GEOMETRIC_REPRESENTATION_ITEM()
RATIONAL_B_SPLINE_CURVE((1.,1.,1.,1.,1.,1.,1.,1.,1.,1.,1.,1.,1.,1.,1.,1.,
1.,1.,1.,1.,1.,1.,1.,1.,1.,1.,1.,1.,1.,1.,1.,1.,1.,1.,1.,1.,1.,1.,1.,1.,
1.,1.,1.,1.,1.,1.,1.,1.,1.,1.,1.,1.,1.,1.,1.,1.,1.,1.,1.,1.,1.,1.,1.,1.,
1.,1.,1.,1.,1.,1.,1.,1.,1.,1.,1.,1.,1.,1.,1.,1.,1.,1.,1.,1.,1.,1.,1.,1.,
1.,1.,1.,1.,1.,1.,1.,1.,1.,1.,1.,1.,1.,1.,1.,1.,1.,1.,1.,1.,1.,1.,1.,1.,
1.,1.,1.,1.,1.,1.,1.,1.,1.,1.,1.,1.,1.,1.,1.,1.,1.,1.,1.,1.,1.,1.,1.,1.,
1.,1.,1.,1.,1.,1.,1.,1.,1.,1.,1.,1.,1.,1.,1.,1.,1.,1.,1.,1.,1.,1.,1.,1.,
1.,1.,1.,1.,1.,1.,1.,1.,1.,1.,1.,1.,1.,1.,1.,1.,1.,1.,1.,1.,1.,1.,1.,1.,
1.,1.,1.,1.,1.,1.,1.,1.,1.,1.))
REPRESENTATION_ITEM('')
);
#484=(
BOUNDED_CURVE()
B_SPLINE_CURVE(5,(#89069,#89070,#89071,#89072,#89073,#89074,#89075,#89076,
#89077,#89078,#89079,#89080,#89081,#89082,#89083,#89084,#89085,#89086,#89087,
#89088,#89089,#89090,#89091,#89092,#89093,#89094,#89095,#89096,#89097,#89098,
#89099,#89100,#89101,#89102,#89103,#89104,#89105,#89106,#89107,#89108,#89109,
#89110,#89111,#89112,#89113,#89114,#89115,#89116,#89117,#89118,#89119,#89120,
#89121,#89122,#89123,#89124,#89125,#89126,#89127,#89128,#89129,#89130,#89131,
#89132,#89133,#89134,#89135,#89136,#89137,#89138,#89139,#89140,#89141,#89142,
#89143,#89144,#89145,#89146,#89147,#89148,#89149,#89150,#89151,#89152,#89153,
#89154,#89155,#89156,#89157,#89158,#89159,#89160,#89161,#89162,#89163,#89164,
#89165,#89166,#89167,#89168,#89169,#89170,#89171,#89172,#89173,#89174,#89175,
#89176,#89177,#89178,#89179,#89180,#89181,#89182,#89183,#89184,#89185,#89186,
#89187,#89188,#89189,#89190,#89191,#89192,#89193,#89194,#89195,#89196,#89197,
#89198,#89199,#89200,#89201,#89202,#89203,#89204,#89205,#89206,#89207,#89208,
#89209,#89210,#89211,#89212,#89213,#89214,#89215,#89216,#89217,#89218,#89219,
#89220,#89221,#89222,#89223,#89224,#89225,#89226,#89227,#89228,#89229,#89230,
#89231,#89232,#89233,#89234,#89235,#89236,#89237,#89238,#89239,#89240,#89241,
#89242,#89243,#89244,#89245,#89246,#89247,#89248,#89249,#89250,#89251,#89252,
#89253,#89254,#89255,#89256,#89257,#89258,#89259,#89260,#89261,#89262),
 .UNSPECIFIED.,.F.,.F.)
B_SPLINE_CURVE_WITH_KNOTS((6,1,1,1,1,1,1,1,1,1,1,1,1,1,1,1,1,1,1,1,1,1,
1,1,1,1,1,1,1,1,1,1,1,1,1,1,1,1,1,1,1,1,1,1,1,1,1,1,1,1,1,1,1,1,1,1,1,1,
1,1,1,1,1,1,1,1,1,1,1,1,1,1,1,1,1,1,1,1,1,1,1,1,1,1,1,1,1,1,1,1,1,1,1,1,
1,1,1,1,1,1,1,1,1,1,1,1,1,1,1,1,1,1,1,1,1,1,1,1,1,1,1,1,1,1,1,1,1,1,1,1,
1,1,1,1,1,1,1,1,1,1,1,1,1,1,1,1,1,1,1,1,1,1,1,1,1,1,1,1,1,1,1,1,1,1,1,1,
1,1,1,1,1,1,1,1,1,1,1,1,1,1,1,1,1,1,1,1,1,1,1,6),(-0.941429844431363,-0.940000000000001,
-0.935000000000001,-0.930000000000001,-0.925000000000001,-0.920000000000001,
-0.915000000000001,-0.910000000000001,-0.905000000000001,-0.900000000000001,
-0.895000000000001,-0.890000000000001,-0.885000000000001,-0.880000000000001,
-0.875000000000001,-0.870000000000001,-0.865000000000001,-0.860000000000001,
-0.855000000000001,-0.850000000000001,-0.845000000000001,-0.840000000000001,
-0.835000000000001,-0.830000000000001,-0.825000000000001,-0.820000000000001,
-0.815000000000001,-0.810000000000001,-0.805000000000001,-0.800000000000001,
-0.795000000000001,-0.790000000000001,-0.785000000000001,-0.780000000000001,
-0.775000000000001,-0.770000000000001,-0.765000000000001,-0.760000000000001,
-0.755000000000001,-0.750000000000001,-0.745000000000001,-0.740000000000001,
-0.735000000000001,-0.730000000000001,-0.725000000000001,-0.720000000000001,
-0.715000000000001,-0.710000000000001,-0.705000000000001,-0.700000000000001,
-0.695000000000001,-0.690000000000001,-0.685,-0.68,-0.675,-0.67,-0.665,
-0.66,-0.655,-0.65,-0.645,-0.64,-0.635,-0.63,-0.625,-0.62,-0.615,-0.61,
-0.605,-0.6,-0.595,-0.59,-0.585,-0.58,-0.575,-0.57,-0.565,-0.56,-0.555,
-0.55,-0.545,-0.54,-0.535,-0.53,-0.525,-0.52,-0.515,-0.51,-0.505,-0.5,-0.495,
-0.49,-0.485,-0.48,-0.475,-0.47,-0.465,-0.46,-0.455,-0.45,-0.445,-0.44,
-0.435,-0.43,-0.425,-0.42,-0.415,-0.41,-0.405,-0.4,-0.395,-0.39,-0.385,
-0.38,-0.375,-0.37,-0.365,-0.36,-0.355,-0.35,-0.345,-0.34,-0.335,-0.33,
-0.325,-0.32,-0.315,-0.31,-0.305,-0.3,-0.295,-0.29,-0.285,-0.28,-0.275,
-0.27,-0.265,-0.26,-0.255,-0.25,-0.245,-0.24,-0.235,-0.23,-0.225,-0.22,
-0.215,-0.21,-0.205,-0.2,-0.195,-0.19,-0.185,-0.18,-0.175,-0.17,-0.165,
-0.16,-0.155,-0.15,-0.145,-0.14,-0.135,-0.13,-0.125,-0.12,-0.115,-0.11,
-0.105,-0.1,-0.095,-0.09,-0.085,-0.08,-0.075,-0.07,-0.065,-0.06,-0.055,
-0.05,-0.045,-0.04,-0.035,-0.03,-0.025,-0.02,-0.015,-0.01,-0.005,0.),
 .UNSPECIFIED.)
CURVE()
GEOMETRIC_REPRESENTATION_ITEM()
RATIONAL_B_SPLINE_CURVE((1.,1.,1.,1.,1.,1.,1.,1.,1.,1.,1.,1.,1.,1.,1.,1.,
1.,1.,1.,1.,1.,1.,1.,1.,1.,1.,1.,1.,1.,1.,1.,1.,1.,1.,1.,1.,1.,1.,1.,1.,
1.,1.,1.,1.,1.,1.,1.,1.,1.,1.,1.,1.,1.,1.,1.,1.,1.,1.,1.,1.,1.,1.,1.,1.,
1.,1.,1.,1.,1.,1.,1.,1.,1.,1.,1.,1.,1.,1.,1.,1.,1.,1.,1.,1.,1.,1.,1.,1.,
1.,1.,1.,1.,1.,1.,1.,1.,1.,1.,1.,1.,1.,1.,1.,1.,1.,1.,1.,1.,1.,1.,1.,1.,
1.,1.,1.,1.,1.,1.,1.,1.,1.,1.,1.,1.,1.,1.,1.,1.,1.,1.,1.,1.,1.,1.,1.,1.,
1.,1.,1.,1.,1.,1.,1.,1.,1.,1.,1.,1.,1.,1.,1.,1.,1.,1.,1.,1.,1.,1.,1.,1.,
1.,1.,1.,1.,1.,1.,1.,1.,1.,1.,1.,1.,1.,1.,1.,1.,1.,1.,1.,1.,1.,1.,1.,1.,
1.,1.,1.,1.,1.,1.,1.,1.,1.,1.))
REPRESENTATION_ITEM('')
);
#485=(
BOUNDED_CURVE()
B_SPLINE_CURVE(5,(#89769,#89770,#89771,#89772,#89773,#89774,#89775,#89776,
#89777,#89778,#89779,#89780,#89781,#89782,#89783,#89784,#89785,#89786,#89787,
#89788,#89789,#89790,#89791,#89792,#89793,#89794,#89795,#89796,#89797,#89798,
#89799,#89800,#89801,#89802,#89803,#89804,#89805,#89806,#89807,#89808,#89809,
#89810,#89811,#89812,#89813,#89814,#89815,#89816,#89817,#89818,#89819,#89820,
#89821,#89822,#89823,#89824,#89825,#89826,#89827,#89828,#89829,#89830,#89831,
#89832,#89833,#89834,#89835,#89836,#89837,#89838,#89839,#89840,#89841,#89842,
#89843,#89844,#89845,#89846,#89847,#89848,#89849,#89850,#89851,#89852,#89853,
#89854,#89855,#89856,#89857,#89858,#89859,#89860,#89861,#89862,#89863,#89864,
#89865,#89866,#89867,#89868,#89869,#89870,#89871,#89872,#89873,#89874,#89875,
#89876,#89877,#89878,#89879,#89880,#89881,#89882,#89883,#89884,#89885,#89886,
#89887,#89888,#89889,#89890,#89891,#89892,#89893,#89894,#89895,#89896,#89897,
#89898,#89899,#89900,#89901,#89902,#89903,#89904,#89905,#89906,#89907,#89908,
#89909,#89910,#89911,#89912,#89913,#89914,#89915,#89916,#89917,#89918,#89919,
#89920,#89921,#89922,#89923,#89924,#89925,#89926,#89927,#89928,#89929,#89930,
#89931,#89932,#89933,#89934,#89935,#89936,#89937,#89938,#89939,#89940,#89941,
#89942,#89943,#89944,#89945,#89946,#89947,#89948,#89949,#89950,#89951,#89952,
#89953,#89954,#89955,#89956,#89957,#89958,#89959,#89960,#89961,#89962),
 .UNSPECIFIED.,.F.,.F.)
B_SPLINE_CURVE_WITH_KNOTS((6,1,1,1,1,1,1,1,1,1,1,1,1,1,1,1,1,1,1,1,1,1,
1,1,1,1,1,1,1,1,1,1,1,1,1,1,1,1,1,1,1,1,1,1,1,1,1,1,1,1,1,1,1,1,1,1,1,1,
1,1,1,1,1,1,1,1,1,1,1,1,1,1,1,1,1,1,1,1,1,1,1,1,1,1,1,1,1,1,1,1,1,1,1,1,
1,1,1,1,1,1,1,1,1,1,1,1,1,1,1,1,1,1,1,1,1,1,1,1,1,1,1,1,1,1,1,1,1,1,1,1,
1,1,1,1,1,1,1,1,1,1,1,1,1,1,1,1,1,1,1,1,1,1,1,1,1,1,1,1,1,1,1,1,1,1,1,1,
1,1,1,1,1,1,1,1,1,1,1,1,1,1,1,1,1,1,1,1,1,1,1,6),(0.,0.005,0.01,0.015,0.02,
0.025,0.03,0.035,0.04,0.045,0.05,0.055,0.06,0.065,0.07,0.075,0.08,0.085,
0.09,0.095,0.1,0.105,0.11,0.115,0.12,0.125,0.13,0.135,0.14,0.145,0.15,0.155,
0.16,0.165,0.17,0.175,0.18,0.185,0.19,0.195,0.2,0.205,0.21,0.215,0.22,0.225,
0.23,0.235,0.24,0.245,0.25,0.255,0.26,0.265,0.27,0.275,0.28,0.285,0.29,
0.295,0.3,0.305,0.31,0.315,0.32,0.325,0.33,0.335,0.34,0.345,0.35,0.355,
0.36,0.365,0.37,0.375,0.38,0.385,0.39,0.395,0.4,0.405,0.41,0.415,0.42,0.425,
0.43,0.435,0.44,0.445,0.45,0.455,0.46,0.465,0.47,0.475,0.48,0.485,0.49,
0.495,0.5,0.505,0.51,0.515,0.52,0.525,0.53,0.535,0.54,0.545,0.55,0.555,
0.56,0.565,0.57,0.575,0.58,0.585,0.59,0.595,0.6,0.605,0.61,0.615,0.62,0.625,
0.63,0.635,0.64,0.645,0.65,0.655,0.66,0.665,0.67,0.675,0.68,0.685,0.690000000000001,
0.695000000000001,0.700000000000001,0.705000000000001,0.710000000000001,
0.715000000000001,0.720000000000001,0.725000000000001,0.730000000000001,
0.735000000000001,0.740000000000001,0.745000000000001,0.750000000000001,
0.755000000000001,0.760000000000001,0.765000000000001,0.770000000000001,
0.775000000000001,0.780000000000001,0.785000000000001,0.790000000000001,
0.795000000000001,0.800000000000001,0.805000000000001,0.810000000000001,
0.815000000000001,0.820000000000001,0.825000000000001,0.830000000000001,
0.835000000000001,0.840000000000001,0.845000000000001,0.850000000000001,
0.855000000000001,0.860000000000001,0.865000000000001,0.870000000000001,
0.875000000000001,0.880000000000001,0.885000000000001,0.890000000000001,
0.895000000000001,0.900000000000001,0.905000000000001,0.910000000000001,
0.915000000000001,0.920000000000001,0.925000000000001,0.930000000000001,
0.935000000000001,0.940000000000001,0.941429844431418),.UNSPECIFIED.)
CURVE()
GEOMETRIC_REPRESENTATION_ITEM()
RATIONAL_B_SPLINE_CURVE((1.,1.,1.,1.,1.,1.,1.,1.,1.,1.,1.,1.,1.,1.,1.,1.,
1.,1.,1.,1.,1.,1.,1.,1.,1.,1.,1.,1.,1.,1.,1.,1.,1.,1.,1.,1.,1.,1.,1.,1.,
1.,1.,1.,1.,1.,1.,1.,1.,1.,1.,1.,1.,1.,1.,1.,1.,1.,1.,1.,1.,1.,1.,1.,1.,
1.,1.,1.,1.,1.,1.,1.,1.,1.,1.,1.,1.,1.,1.,1.,1.,1.,1.,1.,1.,1.,1.,1.,1.,
1.,1.,1.,1.,1.,1.,1.,1.,1.,1.,1.,1.,1.,1.,1.,1.,1.,1.,1.,1.,1.,1.,1.,1.,
1.,1.,1.,1.,1.,1.,1.,1.,1.,1.,1.,1.,1.,1.,1.,1.,1.,1.,1.,1.,1.,1.,1.,1.,
1.,1.,1.,1.,1.,1.,1.,1.,1.,1.,1.,1.,1.,1.,1.,1.,1.,1.,1.,1.,1.,1.,1.,1.,
1.,1.,1.,1.,1.,1.,1.,1.,1.,1.,1.,1.,1.,1.,1.,1.,1.,1.,1.,1.,1.,1.,1.,1.,
1.,1.,1.,1.,1.,1.,1.,1.,1.,1.))
REPRESENTATION_ITEM('')
);
#486=(
BOUNDED_CURVE()
B_SPLINE_CURVE(5,(#89965,#89966,#89967,#89968,#89969,#89970,#89971,#89972,
#89973,#89974,#89975,#89976,#89977,#89978,#89979,#89980,#89981,#89982,#89983,
#89984,#89985,#89986,#89987,#89988,#89989,#89990,#89991,#89992,#89993,#89994,
#89995,#89996,#89997,#89998,#89999,#90000,#90001,#90002,#90003,#90004,#90005,
#90006,#90007,#90008,#90009,#90010,#90011,#90012,#90013,#90014,#90015,#90016,
#90017,#90018,#90019,#90020,#90021,#90022,#90023,#90024,#90025,#90026,#90027,
#90028,#90029,#90030,#90031,#90032,#90033,#90034,#90035,#90036,#90037,#90038,
#90039,#90040,#90041,#90042,#90043,#90044,#90045,#90046,#90047,#90048,#90049,
#90050,#90051,#90052,#90053,#90054,#90055,#90056,#90057,#90058,#90059,#90060,
#90061,#90062,#90063,#90064,#90065,#90066,#90067,#90068,#90069,#90070,#90071,
#90072,#90073,#90074,#90075,#90076,#90077,#90078,#90079,#90080,#90081,#90082,
#90083,#90084,#90085,#90086,#90087,#90088,#90089,#90090,#90091,#90092,#90093,
#90094,#90095,#90096,#90097,#90098,#90099,#90100,#90101,#90102,#90103,#90104,
#90105,#90106,#90107,#90108,#90109,#90110,#90111,#90112,#90113,#90114,#90115,
#90116,#90117,#90118,#90119,#90120,#90121,#90122,#90123,#90124,#90125,#90126,
#90127,#90128,#90129,#90130,#90131,#90132,#90133,#90134,#90135,#90136,#90137,
#90138,#90139,#90140,#90141,#90142,#90143,#90144,#90145,#90146,#90147,#90148,
#90149,#90150,#90151,#90152,#90153,#90154,#90155,#90156,#90157,#90158),
 .UNSPECIFIED.,.F.,.F.)
B_SPLINE_CURVE_WITH_KNOTS((6,1,1,1,1,1,1,1,1,1,1,1,1,1,1,1,1,1,1,1,1,1,
1,1,1,1,1,1,1,1,1,1,1,1,1,1,1,1,1,1,1,1,1,1,1,1,1,1,1,1,1,1,1,1,1,1,1,1,
1,1,1,1,1,1,1,1,1,1,1,1,1,1,1,1,1,1,1,1,1,1,1,1,1,1,1,1,1,1,1,1,1,1,1,1,
1,1,1,1,1,1,1,1,1,1,1,1,1,1,1,1,1,1,1,1,1,1,1,1,1,1,1,1,1,1,1,1,1,1,1,1,
1,1,1,1,1,1,1,1,1,1,1,1,1,1,1,1,1,1,1,1,1,1,1,1,1,1,1,1,1,1,1,1,1,1,1,1,
1,1,1,1,1,1,1,1,1,1,1,1,1,1,1,1,1,1,1,1,1,1,1,6),(-0.941429844431415,-0.940000000000001,
-0.935000000000001,-0.930000000000001,-0.925000000000001,-0.920000000000001,
-0.915000000000001,-0.910000000000001,-0.905000000000001,-0.900000000000001,
-0.895000000000001,-0.890000000000001,-0.885000000000001,-0.880000000000001,
-0.875000000000001,-0.870000000000001,-0.865000000000001,-0.860000000000001,
-0.855000000000001,-0.850000000000001,-0.845000000000001,-0.840000000000001,
-0.835000000000001,-0.830000000000001,-0.825000000000001,-0.820000000000001,
-0.815000000000001,-0.810000000000001,-0.805000000000001,-0.800000000000001,
-0.795000000000001,-0.790000000000001,-0.785000000000001,-0.780000000000001,
-0.775000000000001,-0.770000000000001,-0.765000000000001,-0.760000000000001,
-0.755000000000001,-0.750000000000001,-0.745000000000001,-0.740000000000001,
-0.735000000000001,-0.730000000000001,-0.725000000000001,-0.720000000000001,
-0.715000000000001,-0.710000000000001,-0.705000000000001,-0.700000000000001,
-0.695000000000001,-0.690000000000001,-0.685,-0.68,-0.675,-0.67,-0.665,
-0.66,-0.655,-0.65,-0.645,-0.64,-0.635,-0.63,-0.625,-0.62,-0.615,-0.61,
-0.605,-0.6,-0.595,-0.59,-0.585,-0.58,-0.575,-0.57,-0.565,-0.56,-0.555,
-0.55,-0.545,-0.54,-0.535,-0.53,-0.525,-0.52,-0.515,-0.51,-0.505,-0.5,-0.495,
-0.49,-0.485,-0.48,-0.475,-0.47,-0.465,-0.46,-0.455,-0.45,-0.445,-0.44,
-0.435,-0.43,-0.425,-0.42,-0.415,-0.41,-0.405,-0.4,-0.395,-0.39,-0.385,
-0.38,-0.375,-0.37,-0.365,-0.36,-0.355,-0.35,-0.345,-0.34,-0.335,-0.33,
-0.325,-0.32,-0.315,-0.31,-0.305,-0.3,-0.295,-0.29,-0.285,-0.28,-0.275,
-0.27,-0.265,-0.26,-0.255,-0.25,-0.245,-0.24,-0.235,-0.23,-0.225,-0.22,
-0.215,-0.21,-0.205,-0.2,-0.195,-0.19,-0.185,-0.18,-0.175,-0.17,-0.165,
-0.16,-0.155,-0.15,-0.145,-0.14,-0.135,-0.13,-0.125,-0.12,-0.115,-0.11,
-0.105,-0.1,-0.095,-0.09,-0.085,-0.08,-0.075,-0.07,-0.065,-0.06,-0.055,
-0.05,-0.045,-0.04,-0.035,-0.03,-0.025,-0.02,-0.015,-0.01,-0.005,0.),
 .UNSPECIFIED.)
CURVE()
GEOMETRIC_REPRESENTATION_ITEM()
RATIONAL_B_SPLINE_CURVE((1.,1.,1.,1.,1.,1.,1.,1.,1.,1.,1.,1.,1.,1.,1.,1.,
1.,1.,1.,1.,1.,1.,1.,1.,1.,1.,1.,1.,1.,1.,1.,1.,1.,1.,1.,1.,1.,1.,1.,1.,
1.,1.,1.,1.,1.,1.,1.,1.,1.,1.,1.,1.,1.,1.,1.,1.,1.,1.,1.,1.,1.,1.,1.,1.,
1.,1.,1.,1.,1.,1.,1.,1.,1.,1.,1.,1.,1.,1.,1.,1.,1.,1.,1.,1.,1.,1.,1.,1.,
1.,1.,1.,1.,1.,1.,1.,1.,1.,1.,1.,1.,1.,1.,1.,1.,1.,1.,1.,1.,1.,1.,1.,1.,
1.,1.,1.,1.,1.,1.,1.,1.,1.,1.,1.,1.,1.,1.,1.,1.,1.,1.,1.,1.,1.,1.,1.,1.,
1.,1.,1.,1.,1.,1.,1.,1.,1.,1.,1.,1.,1.,1.,1.,1.,1.,1.,1.,1.,1.,1.,1.,1.,
1.,1.,1.,1.,1.,1.,1.,1.,1.,1.,1.,1.,1.,1.,1.,1.,1.,1.,1.,1.,1.,1.,1.,1.,
1.,1.,1.,1.,1.,1.,1.,1.,1.,1.))
REPRESENTATION_ITEM('')
);
#487=(
BOUNDED_CURVE()
B_SPLINE_CURVE(5,(#90665,#90666,#90667,#90668,#90669,#90670,#90671,#90672,
#90673,#90674,#90675,#90676,#90677,#90678,#90679,#90680,#90681,#90682,#90683,
#90684,#90685,#90686,#90687,#90688,#90689,#90690,#90691,#90692,#90693,#90694,
#90695,#90696,#90697,#90698,#90699,#90700,#90701,#90702,#90703,#90704,#90705,
#90706,#90707,#90708,#90709,#90710,#90711,#90712,#90713,#90714,#90715,#90716,
#90717,#90718,#90719,#90720,#90721,#90722,#90723,#90724,#90725,#90726,#90727,
#90728,#90729,#90730,#90731,#90732,#90733,#90734,#90735,#90736,#90737,#90738,
#90739,#90740,#90741,#90742,#90743,#90744,#90745,#90746,#90747,#90748,#90749,
#90750,#90751,#90752,#90753,#90754,#90755,#90756,#90757,#90758,#90759,#90760,
#90761,#90762,#90763,#90764,#90765,#90766,#90767,#90768,#90769,#90770,#90771,
#90772,#90773,#90774,#90775,#90776,#90777,#90778,#90779,#90780,#90781,#90782,
#90783,#90784,#90785,#90786,#90787,#90788,#90789,#90790,#90791,#90792,#90793,
#90794,#90795,#90796,#90797,#90798,#90799,#90800,#90801,#90802,#90803,#90804,
#90805,#90806,#90807,#90808,#90809,#90810,#90811,#90812,#90813,#90814,#90815,
#90816,#90817,#90818,#90819,#90820,#90821,#90822,#90823,#90824,#90825,#90826,
#90827,#90828,#90829,#90830,#90831,#90832,#90833,#90834,#90835,#90836,#90837,
#90838,#90839,#90840,#90841,#90842,#90843,#90844,#90845,#90846,#90847,#90848,
#90849,#90850,#90851,#90852,#90853,#90854,#90855,#90856,#90857,#90858),
 .UNSPECIFIED.,.F.,.F.)
B_SPLINE_CURVE_WITH_KNOTS((6,1,1,1,1,1,1,1,1,1,1,1,1,1,1,1,1,1,1,1,1,1,
1,1,1,1,1,1,1,1,1,1,1,1,1,1,1,1,1,1,1,1,1,1,1,1,1,1,1,1,1,1,1,1,1,1,1,1,
1,1,1,1,1,1,1,1,1,1,1,1,1,1,1,1,1,1,1,1,1,1,1,1,1,1,1,1,1,1,1,1,1,1,1,1,
1,1,1,1,1,1,1,1,1,1,1,1,1,1,1,1,1,1,1,1,1,1,1,1,1,1,1,1,1,1,1,1,1,1,1,1,
1,1,1,1,1,1,1,1,1,1,1,1,1,1,1,1,1,1,1,1,1,1,1,1,1,1,1,1,1,1,1,1,1,1,1,1,
1,1,1,1,1,1,1,1,1,1,1,1,1,1,1,1,1,1,1,1,1,1,1,6),(0.,0.005,0.01,0.015,0.02,
0.025,0.03,0.035,0.04,0.045,0.05,0.055,0.06,0.065,0.07,0.075,0.08,0.085,
0.09,0.095,0.1,0.105,0.11,0.115,0.12,0.125,0.13,0.135,0.14,0.145,0.15,0.155,
0.16,0.165,0.17,0.175,0.18,0.185,0.19,0.195,0.2,0.205,0.21,0.215,0.22,0.225,
0.23,0.235,0.24,0.245,0.25,0.255,0.26,0.265,0.27,0.275,0.28,0.285,0.29,
0.295,0.3,0.305,0.31,0.315,0.32,0.325,0.33,0.335,0.34,0.345,0.35,0.355,
0.36,0.365,0.37,0.375,0.38,0.385,0.39,0.395,0.4,0.405,0.41,0.415,0.42,0.425,
0.43,0.435,0.44,0.445,0.45,0.455,0.46,0.465,0.47,0.475,0.48,0.485,0.49,
0.495,0.5,0.505,0.51,0.515,0.52,0.525,0.53,0.535,0.54,0.545,0.55,0.555,
0.56,0.565,0.57,0.575,0.58,0.585,0.59,0.595,0.6,0.605,0.61,0.615,0.62,0.625,
0.63,0.635,0.64,0.645,0.65,0.655,0.66,0.665,0.67,0.675,0.68,0.685,0.690000000000001,
0.695000000000001,0.700000000000001,0.705000000000001,0.710000000000001,
0.715000000000001,0.720000000000001,0.725000000000001,0.730000000000001,
0.735000000000001,0.740000000000001,0.745000000000001,0.750000000000001,
0.755000000000001,0.760000000000001,0.765000000000001,0.770000000000001,
0.775000000000001,0.780000000000001,0.785000000000001,0.790000000000001,
0.795000000000001,0.800000000000001,0.805000000000001,0.810000000000001,
0.815000000000001,0.820000000000001,0.825000000000001,0.830000000000001,
0.835000000000001,0.840000000000001,0.845000000000001,0.850000000000001,
0.855000000000001,0.860000000000001,0.865000000000001,0.870000000000001,
0.875000000000001,0.880000000000001,0.885000000000001,0.890000000000001,
0.895000000000001,0.900000000000001,0.905000000000001,0.910000000000001,
0.915000000000001,0.920000000000001,0.925000000000001,0.930000000000001,
0.935000000000001,0.940000000000001,0.941429844431454),.UNSPECIFIED.)
CURVE()
GEOMETRIC_REPRESENTATION_ITEM()
RATIONAL_B_SPLINE_CURVE((1.,1.,1.,1.,1.,1.,1.,1.,1.,1.,1.,1.,1.,1.,1.,1.,
1.,1.,1.,1.,1.,1.,1.,1.,1.,1.,1.,1.,1.,1.,1.,1.,1.,1.,1.,1.,1.,1.,1.,1.,
1.,1.,1.,1.,1.,1.,1.,1.,1.,1.,1.,1.,1.,1.,1.,1.,1.,1.,1.,1.,1.,1.,1.,1.,
1.,1.,1.,1.,1.,1.,1.,1.,1.,1.,1.,1.,1.,1.,1.,1.,1.,1.,1.,1.,1.,1.,1.,1.,
1.,1.,1.,1.,1.,1.,1.,1.,1.,1.,1.,1.,1.,1.,1.,1.,1.,1.,1.,1.,1.,1.,1.,1.,
1.,1.,1.,1.,1.,1.,1.,1.,1.,1.,1.,1.,1.,1.,1.,1.,1.,1.,1.,1.,1.,1.,1.,1.,
1.,1.,1.,1.,1.,1.,1.,1.,1.,1.,1.,1.,1.,1.,1.,1.,1.,1.,1.,1.,1.,1.,1.,1.,
1.,1.,1.,1.,1.,1.,1.,1.,1.,1.,1.,1.,1.,1.,1.,1.,1.,1.,1.,1.,1.,1.,1.,1.,
1.,1.,1.,1.,1.,1.,1.,1.,1.,1.))
REPRESENTATION_ITEM('')
);
#488=(
BOUNDED_CURVE()
B_SPLINE_CURVE(5,(#90861,#90862,#90863,#90864,#90865,#90866,#90867,#90868,
#90869,#90870,#90871,#90872,#90873,#90874,#90875,#90876,#90877,#90878,#90879,
#90880,#90881,#90882,#90883,#90884,#90885,#90886,#90887,#90888,#90889,#90890,
#90891,#90892,#90893,#90894,#90895,#90896,#90897,#90898,#90899,#90900,#90901,
#90902,#90903,#90904,#90905,#90906,#90907,#90908,#90909,#90910,#90911,#90912,
#90913,#90914,#90915,#90916,#90917,#90918,#90919,#90920,#90921,#90922,#90923,
#90924,#90925,#90926,#90927,#90928,#90929,#90930,#90931,#90932,#90933,#90934,
#90935,#90936,#90937,#90938,#90939,#90940,#90941,#90942,#90943,#90944,#90945,
#90946,#90947,#90948,#90949,#90950,#90951,#90952,#90953,#90954,#90955,#90956,
#90957,#90958,#90959,#90960,#90961,#90962,#90963,#90964,#90965,#90966,#90967,
#90968,#90969,#90970,#90971,#90972,#90973,#90974,#90975,#90976,#90977,#90978,
#90979,#90980,#90981,#90982,#90983,#90984,#90985,#90986,#90987,#90988,#90989,
#90990,#90991,#90992,#90993,#90994,#90995,#90996,#90997,#90998,#90999,#91000,
#91001,#91002,#91003,#91004,#91005,#91006,#91007,#91008,#91009,#91010,#91011,
#91012,#91013,#91014,#91015,#91016,#91017,#91018,#91019,#91020,#91021,#91022,
#91023,#91024,#91025,#91026,#91027,#91028,#91029,#91030,#91031,#91032,#91033,
#91034,#91035,#91036,#91037,#91038,#91039,#91040,#91041,#91042,#91043,#91044,
#91045,#91046,#91047,#91048,#91049,#91050,#91051,#91052,#91053,#91054),
 .UNSPECIFIED.,.F.,.F.)
B_SPLINE_CURVE_WITH_KNOTS((6,1,1,1,1,1,1,1,1,1,1,1,1,1,1,1,1,1,1,1,1,1,
1,1,1,1,1,1,1,1,1,1,1,1,1,1,1,1,1,1,1,1,1,1,1,1,1,1,1,1,1,1,1,1,1,1,1,1,
1,1,1,1,1,1,1,1,1,1,1,1,1,1,1,1,1,1,1,1,1,1,1,1,1,1,1,1,1,1,1,1,1,1,1,1,
1,1,1,1,1,1,1,1,1,1,1,1,1,1,1,1,1,1,1,1,1,1,1,1,1,1,1,1,1,1,1,1,1,1,1,1,
1,1,1,1,1,1,1,1,1,1,1,1,1,1,1,1,1,1,1,1,1,1,1,1,1,1,1,1,1,1,1,1,1,1,1,1,
1,1,1,1,1,1,1,1,1,1,1,1,1,1,1,1,1,1,1,1,1,1,1,6),(-0.941429844431448,-0.940000000000001,
-0.935000000000001,-0.930000000000001,-0.925000000000001,-0.920000000000001,
-0.915000000000001,-0.910000000000001,-0.905000000000001,-0.900000000000001,
-0.895000000000001,-0.890000000000001,-0.885000000000001,-0.880000000000001,
-0.875000000000001,-0.870000000000001,-0.865000000000001,-0.860000000000001,
-0.855000000000001,-0.850000000000001,-0.845000000000001,-0.840000000000001,
-0.835000000000001,-0.830000000000001,-0.825000000000001,-0.820000000000001,
-0.815000000000001,-0.810000000000001,-0.805000000000001,-0.800000000000001,
-0.795000000000001,-0.790000000000001,-0.785000000000001,-0.780000000000001,
-0.775000000000001,-0.770000000000001,-0.765000000000001,-0.760000000000001,
-0.755000000000001,-0.750000000000001,-0.745000000000001,-0.740000000000001,
-0.735000000000001,-0.730000000000001,-0.725000000000001,-0.720000000000001,
-0.715000000000001,-0.710000000000001,-0.705000000000001,-0.700000000000001,
-0.695000000000001,-0.690000000000001,-0.685,-0.68,-0.675,-0.67,-0.665,
-0.66,-0.655,-0.65,-0.645,-0.64,-0.635,-0.63,-0.625,-0.62,-0.615,-0.61,
-0.605,-0.6,-0.595,-0.59,-0.585,-0.58,-0.575,-0.57,-0.565,-0.56,-0.555,
-0.55,-0.545,-0.54,-0.535,-0.53,-0.525,-0.52,-0.515,-0.51,-0.505,-0.5,-0.495,
-0.49,-0.485,-0.48,-0.475,-0.47,-0.465,-0.46,-0.455,-0.45,-0.445,-0.44,
-0.435,-0.43,-0.425,-0.42,-0.415,-0.41,-0.405,-0.4,-0.395,-0.39,-0.385,
-0.38,-0.375,-0.37,-0.365,-0.36,-0.355,-0.35,-0.345,-0.34,-0.335,-0.33,
-0.325,-0.32,-0.315,-0.31,-0.305,-0.3,-0.295,-0.29,-0.285,-0.28,-0.275,
-0.27,-0.265,-0.26,-0.255,-0.25,-0.245,-0.24,-0.235,-0.23,-0.225,-0.22,
-0.215,-0.21,-0.205,-0.2,-0.195,-0.19,-0.185,-0.18,-0.175,-0.17,-0.165,
-0.16,-0.155,-0.15,-0.145,-0.14,-0.135,-0.13,-0.125,-0.12,-0.115,-0.11,
-0.105,-0.1,-0.095,-0.09,-0.085,-0.08,-0.075,-0.07,-0.065,-0.06,-0.055,
-0.05,-0.045,-0.04,-0.035,-0.03,-0.025,-0.02,-0.015,-0.01,-0.005,0.),
 .UNSPECIFIED.)
CURVE()
GEOMETRIC_REPRESENTATION_ITEM()
RATIONAL_B_SPLINE_CURVE((1.,1.,1.,1.,1.,1.,1.,1.,1.,1.,1.,1.,1.,1.,1.,1.,
1.,1.,1.,1.,1.,1.,1.,1.,1.,1.,1.,1.,1.,1.,1.,1.,1.,1.,1.,1.,1.,1.,1.,1.,
1.,1.,1.,1.,1.,1.,1.,1.,1.,1.,1.,1.,1.,1.,1.,1.,1.,1.,1.,1.,1.,1.,1.,1.,
1.,1.,1.,1.,1.,1.,1.,1.,1.,1.,1.,1.,1.,1.,1.,1.,1.,1.,1.,1.,1.,1.,1.,1.,
1.,1.,1.,1.,1.,1.,1.,1.,1.,1.,1.,1.,1.,1.,1.,1.,1.,1.,1.,1.,1.,1.,1.,1.,
1.,1.,1.,1.,1.,1.,1.,1.,1.,1.,1.,1.,1.,1.,1.,1.,1.,1.,1.,1.,1.,1.,1.,1.,
1.,1.,1.,1.,1.,1.,1.,1.,1.,1.,1.,1.,1.,1.,1.,1.,1.,1.,1.,1.,1.,1.,1.,1.,
1.,1.,1.,1.,1.,1.,1.,1.,1.,1.,1.,1.,1.,1.,1.,1.,1.,1.,1.,1.,1.,1.,1.,1.,
1.,1.,1.,1.,1.,1.,1.,1.,1.,1.))
REPRESENTATION_ITEM('')
);
#489=(
BOUNDED_CURVE()
B_SPLINE_CURVE(5,(#91561,#91562,#91563,#91564,#91565,#91566,#91567,#91568,
#91569,#91570,#91571,#91572,#91573,#91574,#91575,#91576,#91577,#91578,#91579,
#91580,#91581,#91582,#91583,#91584,#91585,#91586,#91587,#91588,#91589,#91590,
#91591,#91592,#91593,#91594,#91595,#91596,#91597,#91598,#91599,#91600,#91601,
#91602,#91603,#91604,#91605,#91606,#91607,#91608,#91609,#91610,#91611,#91612,
#91613,#91614,#91615,#91616,#91617,#91618,#91619,#91620,#91621,#91622,#91623,
#91624,#91625,#91626,#91627,#91628,#91629,#91630,#91631,#91632,#91633,#91634,
#91635,#91636,#91637,#91638,#91639,#91640,#91641,#91642,#91643,#91644,#91645,
#91646,#91647,#91648,#91649,#91650,#91651,#91652,#91653,#91654,#91655,#91656,
#91657,#91658,#91659,#91660,#91661,#91662,#91663,#91664,#91665,#91666,#91667,
#91668,#91669,#91670,#91671,#91672,#91673,#91674,#91675,#91676,#91677,#91678,
#91679,#91680,#91681,#91682,#91683,#91684,#91685,#91686,#91687,#91688,#91689,
#91690,#91691,#91692,#91693,#91694,#91695,#91696,#91697,#91698,#91699,#91700,
#91701,#91702,#91703,#91704,#91705,#91706,#91707,#91708,#91709,#91710,#91711,
#91712,#91713,#91714,#91715,#91716,#91717,#91718,#91719,#91720,#91721,#91722,
#91723,#91724,#91725,#91726,#91727,#91728,#91729,#91730,#91731,#91732,#91733,
#91734,#91735,#91736,#91737,#91738,#91739,#91740,#91741,#91742,#91743,#91744,
#91745,#91746,#91747,#91748,#91749,#91750,#91751,#91752,#91753,#91754),
 .UNSPECIFIED.,.F.,.F.)
B_SPLINE_CURVE_WITH_KNOTS((6,1,1,1,1,1,1,1,1,1,1,1,1,1,1,1,1,1,1,1,1,1,
1,1,1,1,1,1,1,1,1,1,1,1,1,1,1,1,1,1,1,1,1,1,1,1,1,1,1,1,1,1,1,1,1,1,1,1,
1,1,1,1,1,1,1,1,1,1,1,1,1,1,1,1,1,1,1,1,1,1,1,1,1,1,1,1,1,1,1,1,1,1,1,1,
1,1,1,1,1,1,1,1,1,1,1,1,1,1,1,1,1,1,1,1,1,1,1,1,1,1,1,1,1,1,1,1,1,1,1,1,
1,1,1,1,1,1,1,1,1,1,1,1,1,1,1,1,1,1,1,1,1,1,1,1,1,1,1,1,1,1,1,1,1,1,1,1,
1,1,1,1,1,1,1,1,1,1,1,1,1,1,1,1,1,1,1,1,1,1,1,6),(0.,0.005,0.01,0.015,0.02,
0.025,0.03,0.035,0.04,0.045,0.05,0.055,0.06,0.065,0.07,0.075,0.08,0.085,
0.09,0.095,0.1,0.105,0.11,0.115,0.12,0.125,0.13,0.135,0.14,0.145,0.15,0.155,
0.16,0.165,0.17,0.175,0.18,0.185,0.19,0.195,0.2,0.205,0.21,0.215,0.22,0.225,
0.23,0.235,0.24,0.245,0.25,0.255,0.26,0.265,0.27,0.275,0.28,0.285,0.29,
0.295,0.3,0.305,0.31,0.315,0.32,0.325,0.33,0.335,0.34,0.345,0.35,0.355,
0.36,0.365,0.37,0.375,0.38,0.385,0.39,0.395,0.4,0.405,0.41,0.415,0.42,0.425,
0.43,0.435,0.44,0.445,0.45,0.455,0.46,0.465,0.47,0.475,0.48,0.485,0.49,
0.495,0.5,0.505,0.51,0.515,0.52,0.525,0.53,0.535,0.54,0.545,0.55,0.555,
0.56,0.565,0.57,0.575,0.58,0.585,0.59,0.595,0.6,0.605,0.61,0.615,0.62,0.625,
0.63,0.635,0.64,0.645,0.65,0.655,0.66,0.665,0.67,0.675,0.68,0.685,0.690000000000001,
0.695000000000001,0.700000000000001,0.705000000000001,0.710000000000001,
0.715000000000001,0.720000000000001,0.725000000000001,0.730000000000001,
0.735000000000001,0.740000000000001,0.745000000000001,0.750000000000001,
0.755000000000001,0.760000000000001,0.765000000000001,0.770000000000001,
0.775000000000001,0.780000000000001,0.785000000000001,0.790000000000001,
0.795000000000001,0.800000000000001,0.805000000000001,0.810000000000001,
0.815000000000001,0.820000000000001,0.825000000000001,0.830000000000001,
0.835000000000001,0.840000000000001,0.845000000000001,0.850000000000001,
0.855000000000001,0.860000000000001,0.865000000000001,0.870000000000001,
0.875000000000001,0.880000000000001,0.885000000000001,0.890000000000001,
0.895000000000001,0.900000000000001,0.905000000000001,0.910000000000001,
0.915000000000001,0.920000000000001,0.925000000000001,0.930000000000001,
0.935000000000001,0.940000000000001,0.941429844431403),.UNSPECIFIED.)
CURVE()
GEOMETRIC_REPRESENTATION_ITEM()
RATIONAL_B_SPLINE_CURVE((1.,1.,1.,1.,1.,1.,1.,1.,1.,1.,1.,1.,1.,1.,1.,1.,
1.,1.,1.,1.,1.,1.,1.,1.,1.,1.,1.,1.,1.,1.,1.,1.,1.,1.,1.,1.,1.,1.,1.,1.,
1.,1.,1.,1.,1.,1.,1.,1.,1.,1.,1.,1.,1.,1.,1.,1.,1.,1.,1.,1.,1.,1.,1.,1.,
1.,1.,1.,1.,1.,1.,1.,1.,1.,1.,1.,1.,1.,1.,1.,1.,1.,1.,1.,1.,1.,1.,1.,1.,
1.,1.,1.,1.,1.,1.,1.,1.,1.,1.,1.,1.,1.,1.,1.,1.,1.,1.,1.,1.,1.,1.,1.,1.,
1.,1.,1.,1.,1.,1.,1.,1.,1.,1.,1.,1.,1.,1.,1.,1.,1.,1.,1.,1.,1.,1.,1.,1.,
1.,1.,1.,1.,1.,1.,1.,1.,1.,1.,1.,1.,1.,1.,1.,1.,1.,1.,1.,1.,1.,1.,1.,1.,
1.,1.,1.,1.,1.,1.,1.,1.,1.,1.,1.,1.,1.,1.,1.,1.,1.,1.,1.,1.,1.,1.,1.,1.,
1.,1.,1.,1.,1.,1.,1.,1.,1.,1.))
REPRESENTATION_ITEM('')
);
#490=(
BOUNDED_CURVE()
B_SPLINE_CURVE(5,(#91757,#91758,#91759,#91760,#91761,#91762,#91763,#91764,
#91765,#91766,#91767,#91768,#91769,#91770,#91771,#91772,#91773,#91774,#91775,
#91776,#91777,#91778,#91779,#91780,#91781,#91782,#91783,#91784,#91785,#91786,
#91787,#91788,#91789,#91790,#91791,#91792,#91793,#91794,#91795,#91796,#91797,
#91798,#91799,#91800,#91801,#91802,#91803,#91804,#91805,#91806,#91807,#91808,
#91809,#91810,#91811,#91812,#91813,#91814,#91815,#91816,#91817,#91818,#91819,
#91820,#91821,#91822,#91823,#91824,#91825,#91826,#91827,#91828,#91829,#91830,
#91831,#91832,#91833,#91834,#91835,#91836,#91837,#91838,#91839,#91840,#91841,
#91842,#91843,#91844,#91845,#91846,#91847,#91848,#91849,#91850,#91851,#91852,
#91853,#91854,#91855,#91856,#91857,#91858,#91859,#91860,#91861,#91862,#91863,
#91864,#91865,#91866,#91867,#91868,#91869,#91870,#91871,#91872,#91873,#91874,
#91875,#91876,#91877,#91878,#91879,#91880,#91881,#91882,#91883,#91884,#91885,
#91886,#91887,#91888,#91889,#91890,#91891,#91892,#91893,#91894,#91895,#91896,
#91897,#91898,#91899,#91900,#91901,#91902,#91903,#91904,#91905,#91906,#91907,
#91908,#91909,#91910,#91911,#91912,#91913,#91914,#91915,#91916,#91917,#91918,
#91919,#91920,#91921,#91922,#91923,#91924,#91925,#91926,#91927,#91928,#91929,
#91930,#91931,#91932,#91933,#91934,#91935,#91936,#91937,#91938,#91939,#91940,
#91941,#91942,#91943,#91944,#91945,#91946,#91947,#91948,#91949,#91950),
 .UNSPECIFIED.,.F.,.F.)
B_SPLINE_CURVE_WITH_KNOTS((6,1,1,1,1,1,1,1,1,1,1,1,1,1,1,1,1,1,1,1,1,1,
1,1,1,1,1,1,1,1,1,1,1,1,1,1,1,1,1,1,1,1,1,1,1,1,1,1,1,1,1,1,1,1,1,1,1,1,
1,1,1,1,1,1,1,1,1,1,1,1,1,1,1,1,1,1,1,1,1,1,1,1,1,1,1,1,1,1,1,1,1,1,1,1,
1,1,1,1,1,1,1,1,1,1,1,1,1,1,1,1,1,1,1,1,1,1,1,1,1,1,1,1,1,1,1,1,1,1,1,1,
1,1,1,1,1,1,1,1,1,1,1,1,1,1,1,1,1,1,1,1,1,1,1,1,1,1,1,1,1,1,1,1,1,1,1,1,
1,1,1,1,1,1,1,1,1,1,1,1,1,1,1,1,1,1,1,1,1,1,1,6),(-0.941429844431386,-0.940000000000001,
-0.935000000000001,-0.930000000000001,-0.925000000000001,-0.920000000000001,
-0.915000000000001,-0.910000000000001,-0.905000000000001,-0.900000000000001,
-0.895000000000001,-0.890000000000001,-0.885000000000001,-0.880000000000001,
-0.875000000000001,-0.870000000000001,-0.865000000000001,-0.860000000000001,
-0.855000000000001,-0.850000000000001,-0.845000000000001,-0.840000000000001,
-0.835000000000001,-0.830000000000001,-0.825000000000001,-0.820000000000001,
-0.815000000000001,-0.810000000000001,-0.805000000000001,-0.800000000000001,
-0.795000000000001,-0.790000000000001,-0.785000000000001,-0.780000000000001,
-0.775000000000001,-0.770000000000001,-0.765000000000001,-0.760000000000001,
-0.755000000000001,-0.750000000000001,-0.745000000000001,-0.740000000000001,
-0.735000000000001,-0.730000000000001,-0.725000000000001,-0.720000000000001,
-0.715000000000001,-0.710000000000001,-0.705000000000001,-0.700000000000001,
-0.695000000000001,-0.690000000000001,-0.685,-0.68,-0.675,-0.67,-0.665,
-0.66,-0.655,-0.65,-0.645,-0.64,-0.635,-0.63,-0.625,-0.62,-0.615,-0.61,
-0.605,-0.6,-0.595,-0.59,-0.585,-0.58,-0.575,-0.57,-0.565,-0.56,-0.555,
-0.55,-0.545,-0.54,-0.535,-0.53,-0.525,-0.52,-0.515,-0.51,-0.505,-0.5,-0.495,
-0.49,-0.485,-0.48,-0.475,-0.47,-0.465,-0.46,-0.455,-0.45,-0.445,-0.44,
-0.435,-0.43,-0.425,-0.42,-0.415,-0.41,-0.405,-0.4,-0.395,-0.39,-0.385,
-0.38,-0.375,-0.37,-0.365,-0.36,-0.355,-0.35,-0.345,-0.34,-0.335,-0.33,
-0.325,-0.32,-0.315,-0.31,-0.305,-0.3,-0.295,-0.29,-0.285,-0.28,-0.275,
-0.27,-0.265,-0.26,-0.255,-0.25,-0.245,-0.24,-0.235,-0.23,-0.225,-0.22,
-0.215,-0.21,-0.205,-0.2,-0.195,-0.19,-0.185,-0.18,-0.175,-0.17,-0.165,
-0.16,-0.155,-0.15,-0.145,-0.14,-0.135,-0.13,-0.125,-0.12,-0.115,-0.11,
-0.105,-0.1,-0.095,-0.09,-0.085,-0.08,-0.075,-0.07,-0.065,-0.06,-0.055,
-0.05,-0.045,-0.04,-0.035,-0.03,-0.025,-0.02,-0.015,-0.01,-0.005,0.),
 .UNSPECIFIED.)
CURVE()
GEOMETRIC_REPRESENTATION_ITEM()
RATIONAL_B_SPLINE_CURVE((1.,1.,1.,1.,1.,1.,1.,1.,1.,1.,1.,1.,1.,1.,1.,1.,
1.,1.,1.,1.,1.,1.,1.,1.,1.,1.,1.,1.,1.,1.,1.,1.,1.,1.,1.,1.,1.,1.,1.,1.,
1.,1.,1.,1.,1.,1.,1.,1.,1.,1.,1.,1.,1.,1.,1.,1.,1.,1.,1.,1.,1.,1.,1.,1.,
1.,1.,1.,1.,1.,1.,1.,1.,1.,1.,1.,1.,1.,1.,1.,1.,1.,1.,1.,1.,1.,1.,1.,1.,
1.,1.,1.,1.,1.,1.,1.,1.,1.,1.,1.,1.,1.,1.,1.,1.,1.,1.,1.,1.,1.,1.,1.,1.,
1.,1.,1.,1.,1.,1.,1.,1.,1.,1.,1.,1.,1.,1.,1.,1.,1.,1.,1.,1.,1.,1.,1.,1.,
1.,1.,1.,1.,1.,1.,1.,1.,1.,1.,1.,1.,1.,1.,1.,1.,1.,1.,1.,1.,1.,1.,1.,1.,
1.,1.,1.,1.,1.,1.,1.,1.,1.,1.,1.,1.,1.,1.,1.,1.,1.,1.,1.,1.,1.,1.,1.,1.,
1.,1.,1.,1.,1.,1.,1.,1.,1.,1.))
REPRESENTATION_ITEM('')
);
#491=(
BOUNDED_CURVE()
B_SPLINE_CURVE(5,(#92457,#92458,#92459,#92460,#92461,#92462,#92463,#92464,
#92465,#92466,#92467,#92468,#92469,#92470,#92471,#92472,#92473,#92474,#92475,
#92476,#92477,#92478,#92479,#92480,#92481,#92482,#92483,#92484,#92485,#92486,
#92487,#92488,#92489,#92490,#92491,#92492,#92493,#92494,#92495,#92496,#92497,
#92498,#92499,#92500,#92501,#92502,#92503,#92504,#92505,#92506,#92507,#92508,
#92509,#92510,#92511,#92512,#92513,#92514,#92515,#92516,#92517,#92518,#92519,
#92520,#92521,#92522,#92523,#92524,#92525,#92526,#92527,#92528,#92529,#92530,
#92531,#92532,#92533,#92534,#92535,#92536,#92537,#92538,#92539,#92540,#92541,
#92542,#92543,#92544,#92545,#92546,#92547,#92548,#92549,#92550,#92551,#92552,
#92553,#92554,#92555,#92556,#92557,#92558,#92559,#92560,#92561,#92562,#92563,
#92564,#92565,#92566,#92567,#92568,#92569,#92570,#92571,#92572,#92573,#92574,
#92575,#92576,#92577,#92578,#92579,#92580,#92581,#92582,#92583,#92584,#92585,
#92586,#92587,#92588,#92589,#92590,#92591,#92592,#92593,#92594,#92595,#92596,
#92597,#92598,#92599,#92600,#92601,#92602,#92603,#92604,#92605,#92606,#92607,
#92608,#92609,#92610,#92611,#92612,#92613,#92614,#92615,#92616,#92617,#92618,
#92619,#92620,#92621,#92622,#92623,#92624,#92625,#92626,#92627,#92628,#92629,
#92630,#92631,#92632,#92633,#92634,#92635,#92636,#92637,#92638,#92639,#92640,
#92641,#92642,#92643,#92644,#92645,#92646,#92647,#92648,#92649,#92650),
 .UNSPECIFIED.,.F.,.F.)
B_SPLINE_CURVE_WITH_KNOTS((6,1,1,1,1,1,1,1,1,1,1,1,1,1,1,1,1,1,1,1,1,1,
1,1,1,1,1,1,1,1,1,1,1,1,1,1,1,1,1,1,1,1,1,1,1,1,1,1,1,1,1,1,1,1,1,1,1,1,
1,1,1,1,1,1,1,1,1,1,1,1,1,1,1,1,1,1,1,1,1,1,1,1,1,1,1,1,1,1,1,1,1,1,1,1,
1,1,1,1,1,1,1,1,1,1,1,1,1,1,1,1,1,1,1,1,1,1,1,1,1,1,1,1,1,1,1,1,1,1,1,1,
1,1,1,1,1,1,1,1,1,1,1,1,1,1,1,1,1,1,1,1,1,1,1,1,1,1,1,1,1,1,1,1,1,1,1,1,
1,1,1,1,1,1,1,1,1,1,1,1,1,1,1,1,1,1,1,1,1,1,1,6),(0.,0.005,0.01,0.015,0.02,
0.025,0.03,0.035,0.04,0.045,0.05,0.055,0.06,0.065,0.07,0.075,0.08,0.085,
0.09,0.095,0.1,0.105,0.11,0.115,0.12,0.125,0.13,0.135,0.14,0.145,0.15,0.155,
0.16,0.165,0.17,0.175,0.18,0.185,0.19,0.195,0.2,0.205,0.21,0.215,0.22,0.225,
0.23,0.235,0.24,0.245,0.25,0.255,0.26,0.265,0.27,0.275,0.28,0.285,0.29,
0.295,0.3,0.305,0.31,0.315,0.32,0.325,0.33,0.335,0.34,0.345,0.35,0.355,
0.36,0.365,0.37,0.375,0.38,0.385,0.39,0.395,0.4,0.405,0.41,0.415,0.42,0.425,
0.43,0.435,0.44,0.445,0.45,0.455,0.46,0.465,0.47,0.475,0.48,0.485,0.49,
0.495,0.5,0.505,0.51,0.515,0.52,0.525,0.53,0.535,0.54,0.545,0.55,0.555,
0.56,0.565,0.57,0.575,0.58,0.585,0.59,0.595,0.6,0.605,0.61,0.615,0.62,0.625,
0.63,0.635,0.64,0.645,0.65,0.655,0.66,0.665,0.67,0.675,0.68,0.685,0.690000000000001,
0.695000000000001,0.700000000000001,0.705000000000001,0.710000000000001,
0.715000000000001,0.720000000000001,0.725000000000001,0.730000000000001,
0.735000000000001,0.740000000000001,0.745000000000001,0.750000000000001,
0.755000000000001,0.760000000000001,0.765000000000001,0.770000000000001,
0.775000000000001,0.780000000000001,0.785000000000001,0.790000000000001,
0.795000000000001,0.800000000000001,0.805000000000001,0.810000000000001,
0.815000000000001,0.820000000000001,0.825000000000001,0.830000000000001,
0.835000000000001,0.840000000000001,0.845000000000001,0.850000000000001,
0.855000000000001,0.860000000000001,0.865000000000001,0.870000000000001,
0.875000000000001,0.880000000000001,0.885000000000001,0.890000000000001,
0.895000000000001,0.900000000000001,0.905000000000001,0.910000000000001,
0.915000000000001,0.920000000000001,0.925000000000001,0.930000000000001,
0.935000000000001,0.940000000000001,0.941429844431541),.UNSPECIFIED.)
CURVE()
GEOMETRIC_REPRESENTATION_ITEM()
RATIONAL_B_SPLINE_CURVE((1.,1.,1.,1.,1.,1.,1.,1.,1.,1.,1.,1.,1.,1.,1.,1.,
1.,1.,1.,1.,1.,1.,1.,1.,1.,1.,1.,1.,1.,1.,1.,1.,1.,1.,1.,1.,1.,1.,1.,1.,
1.,1.,1.,1.,1.,1.,1.,1.,1.,1.,1.,1.,1.,1.,1.,1.,1.,1.,1.,1.,1.,1.,1.,1.,
1.,1.,1.,1.,1.,1.,1.,1.,1.,1.,1.,1.,1.,1.,1.,1.,1.,1.,1.,1.,1.,1.,1.,1.,
1.,1.,1.,1.,1.,1.,1.,1.,1.,1.,1.,1.,1.,1.,1.,1.,1.,1.,1.,1.,1.,1.,1.,1.,
1.,1.,1.,1.,1.,1.,1.,1.,1.,1.,1.,1.,1.,1.,1.,1.,1.,1.,1.,1.,1.,1.,1.,1.,
1.,1.,1.,1.,1.,1.,1.,1.,1.,1.,1.,1.,1.,1.,1.,1.,1.,1.,1.,1.,1.,1.,1.,1.,
1.,1.,1.,1.,1.,1.,1.,1.,1.,1.,1.,1.,1.,1.,1.,1.,1.,1.,1.,1.,1.,1.,1.,1.,
1.,1.,1.,1.,1.,1.,1.,1.,1.,1.))
REPRESENTATION_ITEM('')
);
#492=(
BOUNDED_CURVE()
B_SPLINE_CURVE(5,(#92653,#92654,#92655,#92656,#92657,#92658,#92659,#92660,
#92661,#92662,#92663,#92664,#92665,#92666,#92667,#92668,#92669,#92670,#92671,
#92672,#92673,#92674,#92675,#92676,#92677,#92678,#92679,#92680,#92681,#92682,
#92683,#92684,#92685,#92686,#92687,#92688,#92689,#92690,#92691,#92692,#92693,
#92694,#92695,#92696,#92697,#92698,#92699,#92700,#92701,#92702,#92703,#92704,
#92705,#92706,#92707,#92708,#92709,#92710,#92711,#92712,#92713,#92714,#92715,
#92716,#92717,#92718,#92719,#92720,#92721,#92722,#92723,#92724,#92725,#92726,
#92727,#92728,#92729,#92730,#92731,#92732,#92733,#92734,#92735,#92736,#92737,
#92738,#92739,#92740,#92741,#92742,#92743,#92744,#92745,#92746,#92747,#92748,
#92749,#92750,#92751,#92752,#92753,#92754,#92755,#92756,#92757,#92758,#92759,
#92760,#92761,#92762,#92763,#92764,#92765,#92766,#92767,#92768,#92769,#92770,
#92771,#92772,#92773,#92774,#92775,#92776,#92777,#92778,#92779,#92780,#92781,
#92782,#92783,#92784,#92785,#92786,#92787,#92788,#92789,#92790,#92791,#92792,
#92793,#92794,#92795,#92796,#92797,#92798,#92799,#92800,#92801,#92802,#92803,
#92804,#92805,#92806,#92807,#92808,#92809,#92810,#92811,#92812,#92813,#92814,
#92815,#92816,#92817,#92818,#92819,#92820,#92821,#92822,#92823,#92824,#92825,
#92826,#92827,#92828,#92829,#92830,#92831,#92832,#92833,#92834,#92835,#92836,
#92837,#92838,#92839,#92840,#92841,#92842,#92843,#92844,#92845,#92846),
 .UNSPECIFIED.,.F.,.F.)
B_SPLINE_CURVE_WITH_KNOTS((6,1,1,1,1,1,1,1,1,1,1,1,1,1,1,1,1,1,1,1,1,1,
1,1,1,1,1,1,1,1,1,1,1,1,1,1,1,1,1,1,1,1,1,1,1,1,1,1,1,1,1,1,1,1,1,1,1,1,
1,1,1,1,1,1,1,1,1,1,1,1,1,1,1,1,1,1,1,1,1,1,1,1,1,1,1,1,1,1,1,1,1,1,1,1,
1,1,1,1,1,1,1,1,1,1,1,1,1,1,1,1,1,1,1,1,1,1,1,1,1,1,1,1,1,1,1,1,1,1,1,1,
1,1,1,1,1,1,1,1,1,1,1,1,1,1,1,1,1,1,1,1,1,1,1,1,1,1,1,1,1,1,1,1,1,1,1,1,
1,1,1,1,1,1,1,1,1,1,1,1,1,1,1,1,1,1,1,1,1,1,1,6),(-0.941429844431541,-0.940000000000001,
-0.935000000000001,-0.930000000000001,-0.925000000000001,-0.920000000000001,
-0.915000000000001,-0.910000000000001,-0.905000000000001,-0.900000000000001,
-0.895000000000001,-0.890000000000001,-0.885000000000001,-0.880000000000001,
-0.875000000000001,-0.870000000000001,-0.865000000000001,-0.860000000000001,
-0.855000000000001,-0.850000000000001,-0.845000000000001,-0.840000000000001,
-0.835000000000001,-0.830000000000001,-0.825000000000001,-0.820000000000001,
-0.815000000000001,-0.810000000000001,-0.805000000000001,-0.800000000000001,
-0.795000000000001,-0.790000000000001,-0.785000000000001,-0.780000000000001,
-0.775000000000001,-0.770000000000001,-0.765000000000001,-0.760000000000001,
-0.755000000000001,-0.750000000000001,-0.745000000000001,-0.740000000000001,
-0.735000000000001,-0.730000000000001,-0.725000000000001,-0.720000000000001,
-0.715000000000001,-0.710000000000001,-0.705000000000001,-0.700000000000001,
-0.695000000000001,-0.690000000000001,-0.685,-0.68,-0.675,-0.67,-0.665,
-0.66,-0.655,-0.65,-0.645,-0.64,-0.635,-0.63,-0.625,-0.62,-0.615,-0.61,
-0.605,-0.6,-0.595,-0.59,-0.585,-0.58,-0.575,-0.57,-0.565,-0.56,-0.555,
-0.55,-0.545,-0.54,-0.535,-0.53,-0.525,-0.52,-0.515,-0.51,-0.505,-0.5,-0.495,
-0.49,-0.485,-0.48,-0.475,-0.47,-0.465,-0.46,-0.455,-0.45,-0.445,-0.44,
-0.435,-0.43,-0.425,-0.42,-0.415,-0.41,-0.405,-0.4,-0.395,-0.39,-0.385,
-0.38,-0.375,-0.37,-0.365,-0.36,-0.355,-0.35,-0.345,-0.34,-0.335,-0.33,
-0.325,-0.32,-0.315,-0.31,-0.305,-0.3,-0.295,-0.29,-0.285,-0.28,-0.275,
-0.27,-0.265,-0.26,-0.255,-0.25,-0.245,-0.24,-0.235,-0.23,-0.225,-0.22,
-0.215,-0.21,-0.205,-0.2,-0.195,-0.19,-0.185,-0.18,-0.175,-0.17,-0.165,
-0.16,-0.155,-0.15,-0.145,-0.14,-0.135,-0.13,-0.125,-0.12,-0.115,-0.11,
-0.105,-0.1,-0.095,-0.09,-0.085,-0.08,-0.075,-0.07,-0.065,-0.06,-0.055,
-0.05,-0.045,-0.04,-0.035,-0.03,-0.025,-0.02,-0.015,-0.01,-0.005,0.),
 .UNSPECIFIED.)
CURVE()
GEOMETRIC_REPRESENTATION_ITEM()
RATIONAL_B_SPLINE_CURVE((1.,1.,1.,1.,1.,1.,1.,1.,1.,1.,1.,1.,1.,1.,1.,1.,
1.,1.,1.,1.,1.,1.,1.,1.,1.,1.,1.,1.,1.,1.,1.,1.,1.,1.,1.,1.,1.,1.,1.,1.,
1.,1.,1.,1.,1.,1.,1.,1.,1.,1.,1.,1.,1.,1.,1.,1.,1.,1.,1.,1.,1.,1.,1.,1.,
1.,1.,1.,1.,1.,1.,1.,1.,1.,1.,1.,1.,1.,1.,1.,1.,1.,1.,1.,1.,1.,1.,1.,1.,
1.,1.,1.,1.,1.,1.,1.,1.,1.,1.,1.,1.,1.,1.,1.,1.,1.,1.,1.,1.,1.,1.,1.,1.,
1.,1.,1.,1.,1.,1.,1.,1.,1.,1.,1.,1.,1.,1.,1.,1.,1.,1.,1.,1.,1.,1.,1.,1.,
1.,1.,1.,1.,1.,1.,1.,1.,1.,1.,1.,1.,1.,1.,1.,1.,1.,1.,1.,1.,1.,1.,1.,1.,
1.,1.,1.,1.,1.,1.,1.,1.,1.,1.,1.,1.,1.,1.,1.,1.,1.,1.,1.,1.,1.,1.,1.,1.,
1.,1.,1.,1.,1.,1.,1.,1.,1.,1.))
REPRESENTATION_ITEM('')
);
#493=(
BOUNDED_CURVE()
B_SPLINE_CURVE(5,(#93353,#93354,#93355,#93356,#93357,#93358,#93359,#93360,
#93361,#93362,#93363,#93364,#93365,#93366,#93367,#93368,#93369,#93370,#93371,
#93372,#93373,#93374,#93375,#93376,#93377,#93378,#93379,#93380,#93381,#93382,
#93383,#93384,#93385,#93386,#93387,#93388,#93389,#93390,#93391,#93392,#93393,
#93394,#93395,#93396,#93397,#93398,#93399,#93400,#93401,#93402,#93403,#93404,
#93405,#93406,#93407,#93408,#93409,#93410,#93411,#93412,#93413,#93414,#93415,
#93416,#93417,#93418,#93419,#93420,#93421,#93422,#93423,#93424,#93425,#93426,
#93427,#93428,#93429,#93430,#93431,#93432,#93433,#93434,#93435,#93436,#93437,
#93438,#93439,#93440,#93441,#93442,#93443,#93444,#93445,#93446,#93447,#93448,
#93449,#93450,#93451,#93452,#93453,#93454,#93455,#93456,#93457,#93458,#93459,
#93460,#93461,#93462,#93463,#93464,#93465,#93466,#93467,#93468,#93469,#93470,
#93471,#93472,#93473,#93474,#93475,#93476,#93477,#93478,#93479,#93480,#93481,
#93482,#93483,#93484,#93485,#93486,#93487,#93488,#93489,#93490,#93491,#93492,
#93493,#93494,#93495,#93496,#93497,#93498,#93499,#93500,#93501,#93502,#93503,
#93504,#93505,#93506,#93507,#93508,#93509,#93510,#93511,#93512,#93513,#93514,
#93515,#93516,#93517,#93518,#93519,#93520,#93521,#93522,#93523,#93524,#93525,
#93526,#93527,#93528,#93529,#93530,#93531,#93532,#93533,#93534,#93535,#93536,
#93537,#93538,#93539,#93540,#93541,#93542,#93543,#93544,#93545,#93546),
 .UNSPECIFIED.,.F.,.F.)
B_SPLINE_CURVE_WITH_KNOTS((6,1,1,1,1,1,1,1,1,1,1,1,1,1,1,1,1,1,1,1,1,1,
1,1,1,1,1,1,1,1,1,1,1,1,1,1,1,1,1,1,1,1,1,1,1,1,1,1,1,1,1,1,1,1,1,1,1,1,
1,1,1,1,1,1,1,1,1,1,1,1,1,1,1,1,1,1,1,1,1,1,1,1,1,1,1,1,1,1,1,1,1,1,1,1,
1,1,1,1,1,1,1,1,1,1,1,1,1,1,1,1,1,1,1,1,1,1,1,1,1,1,1,1,1,1,1,1,1,1,1,1,
1,1,1,1,1,1,1,1,1,1,1,1,1,1,1,1,1,1,1,1,1,1,1,1,1,1,1,1,1,1,1,1,1,1,1,1,
1,1,1,1,1,1,1,1,1,1,1,1,1,1,1,1,1,1,1,1,1,1,1,6),(0.,0.005,0.01,0.015,0.02,
0.025,0.03,0.035,0.04,0.045,0.05,0.055,0.06,0.065,0.07,0.075,0.08,0.085,
0.09,0.095,0.1,0.105,0.11,0.115,0.12,0.125,0.13,0.135,0.14,0.145,0.15,0.155,
0.16,0.165,0.17,0.175,0.18,0.185,0.19,0.195,0.2,0.205,0.21,0.215,0.22,0.225,
0.23,0.235,0.24,0.245,0.25,0.255,0.26,0.265,0.27,0.275,0.28,0.285,0.29,
0.295,0.3,0.305,0.31,0.315,0.32,0.325,0.33,0.335,0.34,0.345,0.35,0.355,
0.36,0.365,0.37,0.375,0.38,0.385,0.39,0.395,0.4,0.405,0.41,0.415,0.42,0.425,
0.43,0.435,0.44,0.445,0.45,0.455,0.46,0.465,0.47,0.475,0.48,0.485,0.49,
0.495,0.5,0.505,0.51,0.515,0.52,0.525,0.53,0.535,0.54,0.545,0.55,0.555,
0.56,0.565,0.57,0.575,0.58,0.585,0.59,0.595,0.6,0.605,0.61,0.615,0.62,0.625,
0.63,0.635,0.64,0.645,0.65,0.655,0.66,0.665,0.67,0.675,0.68,0.685,0.690000000000001,
0.695000000000001,0.700000000000001,0.705000000000001,0.710000000000001,
0.715000000000001,0.720000000000001,0.725000000000001,0.730000000000001,
0.735000000000001,0.740000000000001,0.745000000000001,0.750000000000001,
0.755000000000001,0.760000000000001,0.765000000000001,0.770000000000001,
0.775000000000001,0.780000000000001,0.785000000000001,0.790000000000001,
0.795000000000001,0.800000000000001,0.805000000000001,0.810000000000001,
0.815000000000001,0.820000000000001,0.825000000000001,0.830000000000001,
0.835000000000001,0.840000000000001,0.845000000000001,0.850000000000001,
0.855000000000001,0.860000000000001,0.865000000000001,0.870000000000001,
0.875000000000001,0.880000000000001,0.885000000000001,0.890000000000001,
0.895000000000001,0.900000000000001,0.905000000000001,0.910000000000001,
0.915000000000001,0.920000000000001,0.925000000000001,0.930000000000001,
0.935000000000001,0.940000000000001,0.941429844431519),.UNSPECIFIED.)
CURVE()
GEOMETRIC_REPRESENTATION_ITEM()
RATIONAL_B_SPLINE_CURVE((1.,1.,1.,1.,1.,1.,1.,1.,1.,1.,1.,1.,1.,1.,1.,1.,
1.,1.,1.,1.,1.,1.,1.,1.,1.,1.,1.,1.,1.,1.,1.,1.,1.,1.,1.,1.,1.,1.,1.,1.,
1.,1.,1.,1.,1.,1.,1.,1.,1.,1.,1.,1.,1.,1.,1.,1.,1.,1.,1.,1.,1.,1.,1.,1.,
1.,1.,1.,1.,1.,1.,1.,1.,1.,1.,1.,1.,1.,1.,1.,1.,1.,1.,1.,1.,1.,1.,1.,1.,
1.,1.,1.,1.,1.,1.,1.,1.,1.,1.,1.,1.,1.,1.,1.,1.,1.,1.,1.,1.,1.,1.,1.,1.,
1.,1.,1.,1.,1.,1.,1.,1.,1.,1.,1.,1.,1.,1.,1.,1.,1.,1.,1.,1.,1.,1.,1.,1.,
1.,1.,1.,1.,1.,1.,1.,1.,1.,1.,1.,1.,1.,1.,1.,1.,1.,1.,1.,1.,1.,1.,1.,1.,
1.,1.,1.,1.,1.,1.,1.,1.,1.,1.,1.,1.,1.,1.,1.,1.,1.,1.,1.,1.,1.,1.,1.,1.,
1.,1.,1.,1.,1.,1.,1.,1.,1.,1.))
REPRESENTATION_ITEM('')
);
#494=(
BOUNDED_CURVE()
B_SPLINE_CURVE(5,(#93549,#93550,#93551,#93552,#93553,#93554,#93555,#93556,
#93557,#93558,#93559,#93560,#93561,#93562,#93563,#93564,#93565,#93566,#93567,
#93568,#93569,#93570,#93571,#93572,#93573,#93574,#93575,#93576,#93577,#93578,
#93579,#93580,#93581,#93582,#93583,#93584,#93585,#93586,#93587,#93588,#93589,
#93590,#93591,#93592,#93593,#93594,#93595,#93596,#93597,#93598,#93599,#93600,
#93601,#93602,#93603,#93604,#93605,#93606,#93607,#93608,#93609,#93610,#93611,
#93612,#93613,#93614,#93615,#93616,#93617,#93618,#93619,#93620,#93621,#93622,
#93623,#93624,#93625,#93626,#93627,#93628,#93629,#93630,#93631,#93632,#93633,
#93634,#93635,#93636,#93637,#93638,#93639,#93640,#93641,#93642,#93643,#93644,
#93645,#93646,#93647,#93648,#93649,#93650,#93651,#93652,#93653,#93654,#93655,
#93656,#93657,#93658,#93659,#93660,#93661,#93662,#93663,#93664,#93665,#93666,
#93667,#93668,#93669,#93670,#93671,#93672,#93673,#93674,#93675,#93676,#93677,
#93678,#93679,#93680,#93681,#93682,#93683,#93684,#93685,#93686,#93687,#93688,
#93689,#93690,#93691,#93692,#93693,#93694,#93695,#93696,#93697,#93698,#93699,
#93700,#93701,#93702,#93703,#93704,#93705,#93706,#93707,#93708,#93709,#93710,
#93711,#93712,#93713,#93714,#93715,#93716,#93717,#93718,#93719,#93720,#93721,
#93722,#93723,#93724,#93725,#93726,#93727,#93728,#93729,#93730,#93731,#93732,
#93733,#93734,#93735,#93736,#93737,#93738,#93739,#93740,#93741,#93742),
 .UNSPECIFIED.,.F.,.F.)
B_SPLINE_CURVE_WITH_KNOTS((6,1,1,1,1,1,1,1,1,1,1,1,1,1,1,1,1,1,1,1,1,1,
1,1,1,1,1,1,1,1,1,1,1,1,1,1,1,1,1,1,1,1,1,1,1,1,1,1,1,1,1,1,1,1,1,1,1,1,
1,1,1,1,1,1,1,1,1,1,1,1,1,1,1,1,1,1,1,1,1,1,1,1,1,1,1,1,1,1,1,1,1,1,1,1,
1,1,1,1,1,1,1,1,1,1,1,1,1,1,1,1,1,1,1,1,1,1,1,1,1,1,1,1,1,1,1,1,1,1,1,1,
1,1,1,1,1,1,1,1,1,1,1,1,1,1,1,1,1,1,1,1,1,1,1,1,1,1,1,1,1,1,1,1,1,1,1,1,
1,1,1,1,1,1,1,1,1,1,1,1,1,1,1,1,1,1,1,1,1,1,1,6),(-0.941429844431519,-0.940000000000001,
-0.935000000000001,-0.930000000000001,-0.925000000000001,-0.920000000000001,
-0.915000000000001,-0.910000000000001,-0.905000000000001,-0.900000000000001,
-0.895000000000001,-0.890000000000001,-0.885000000000001,-0.880000000000001,
-0.875000000000001,-0.870000000000001,-0.865000000000001,-0.860000000000001,
-0.855000000000001,-0.850000000000001,-0.845000000000001,-0.840000000000001,
-0.835000000000001,-0.830000000000001,-0.825000000000001,-0.820000000000001,
-0.815000000000001,-0.810000000000001,-0.805000000000001,-0.800000000000001,
-0.795000000000001,-0.790000000000001,-0.785000000000001,-0.780000000000001,
-0.775000000000001,-0.770000000000001,-0.765000000000001,-0.760000000000001,
-0.755000000000001,-0.750000000000001,-0.745000000000001,-0.740000000000001,
-0.735000000000001,-0.730000000000001,-0.725000000000001,-0.720000000000001,
-0.715000000000001,-0.710000000000001,-0.705000000000001,-0.700000000000001,
-0.695000000000001,-0.690000000000001,-0.685,-0.68,-0.675,-0.67,-0.665,
-0.66,-0.655,-0.65,-0.645,-0.64,-0.635,-0.63,-0.625,-0.62,-0.615,-0.61,
-0.605,-0.6,-0.595,-0.59,-0.585,-0.58,-0.575,-0.57,-0.565,-0.56,-0.555,
-0.55,-0.545,-0.54,-0.535,-0.53,-0.525,-0.52,-0.515,-0.51,-0.505,-0.5,-0.495,
-0.49,-0.485,-0.48,-0.475,-0.47,-0.465,-0.46,-0.455,-0.45,-0.445,-0.44,
-0.435,-0.43,-0.425,-0.42,-0.415,-0.41,-0.405,-0.4,-0.395,-0.39,-0.385,
-0.38,-0.375,-0.37,-0.365,-0.36,-0.355,-0.35,-0.345,-0.34,-0.335,-0.33,
-0.325,-0.32,-0.315,-0.31,-0.305,-0.3,-0.295,-0.29,-0.285,-0.28,-0.275,
-0.27,-0.265,-0.26,-0.255,-0.25,-0.245,-0.24,-0.235,-0.23,-0.225,-0.22,
-0.215,-0.21,-0.205,-0.2,-0.195,-0.19,-0.185,-0.18,-0.175,-0.17,-0.165,
-0.16,-0.155,-0.15,-0.145,-0.14,-0.135,-0.13,-0.125,-0.12,-0.115,-0.11,
-0.105,-0.1,-0.095,-0.09,-0.085,-0.08,-0.075,-0.07,-0.065,-0.06,-0.055,
-0.05,-0.045,-0.04,-0.035,-0.03,-0.025,-0.02,-0.015,-0.01,-0.005,0.),
 .UNSPECIFIED.)
CURVE()
GEOMETRIC_REPRESENTATION_ITEM()
RATIONAL_B_SPLINE_CURVE((1.,1.,1.,1.,1.,1.,1.,1.,1.,1.,1.,1.,1.,1.,1.,1.,
1.,1.,1.,1.,1.,1.,1.,1.,1.,1.,1.,1.,1.,1.,1.,1.,1.,1.,1.,1.,1.,1.,1.,1.,
1.,1.,1.,1.,1.,1.,1.,1.,1.,1.,1.,1.,1.,1.,1.,1.,1.,1.,1.,1.,1.,1.,1.,1.,
1.,1.,1.,1.,1.,1.,1.,1.,1.,1.,1.,1.,1.,1.,1.,1.,1.,1.,1.,1.,1.,1.,1.,1.,
1.,1.,1.,1.,1.,1.,1.,1.,1.,1.,1.,1.,1.,1.,1.,1.,1.,1.,1.,1.,1.,1.,1.,1.,
1.,1.,1.,1.,1.,1.,1.,1.,1.,1.,1.,1.,1.,1.,1.,1.,1.,1.,1.,1.,1.,1.,1.,1.,
1.,1.,1.,1.,1.,1.,1.,1.,1.,1.,1.,1.,1.,1.,1.,1.,1.,1.,1.,1.,1.,1.,1.,1.,
1.,1.,1.,1.,1.,1.,1.,1.,1.,1.,1.,1.,1.,1.,1.,1.,1.,1.,1.,1.,1.,1.,1.,1.,
1.,1.,1.,1.,1.,1.,1.,1.,1.,1.))
REPRESENTATION_ITEM('')
);
#495=(
BOUNDED_CURVE()
B_SPLINE_CURVE(5,(#94249,#94250,#94251,#94252,#94253,#94254,#94255,#94256,
#94257,#94258,#94259,#94260,#94261,#94262,#94263,#94264,#94265,#94266,#94267,
#94268,#94269,#94270,#94271,#94272,#94273,#94274,#94275,#94276,#94277,#94278,
#94279,#94280,#94281,#94282,#94283,#94284,#94285,#94286,#94287,#94288,#94289,
#94290,#94291,#94292,#94293,#94294,#94295,#94296,#94297,#94298,#94299,#94300,
#94301,#94302,#94303,#94304,#94305,#94306,#94307,#94308,#94309,#94310,#94311,
#94312,#94313,#94314,#94315,#94316,#94317,#94318,#94319,#94320,#94321,#94322,
#94323,#94324,#94325,#94326,#94327,#94328,#94329,#94330,#94331,#94332,#94333,
#94334,#94335,#94336,#94337,#94338,#94339,#94340,#94341,#94342,#94343,#94344,
#94345,#94346,#94347,#94348,#94349,#94350,#94351,#94352,#94353,#94354,#94355,
#94356,#94357,#94358,#94359,#94360,#94361,#94362,#94363,#94364,#94365,#94366,
#94367,#94368,#94369,#94370,#94371,#94372,#94373,#94374,#94375,#94376,#94377,
#94378,#94379,#94380,#94381,#94382,#94383,#94384,#94385,#94386,#94387,#94388,
#94389,#94390,#94391,#94392,#94393,#94394,#94395,#94396,#94397,#94398,#94399,
#94400,#94401,#94402,#94403,#94404,#94405,#94406,#94407,#94408,#94409,#94410,
#94411,#94412,#94413,#94414,#94415,#94416,#94417,#94418,#94419,#94420,#94421,
#94422,#94423,#94424,#94425,#94426,#94427,#94428,#94429,#94430,#94431,#94432,
#94433,#94434,#94435,#94436,#94437,#94438,#94439,#94440,#94441,#94442),
 .UNSPECIFIED.,.F.,.F.)
B_SPLINE_CURVE_WITH_KNOTS((6,1,1,1,1,1,1,1,1,1,1,1,1,1,1,1,1,1,1,1,1,1,
1,1,1,1,1,1,1,1,1,1,1,1,1,1,1,1,1,1,1,1,1,1,1,1,1,1,1,1,1,1,1,1,1,1,1,1,
1,1,1,1,1,1,1,1,1,1,1,1,1,1,1,1,1,1,1,1,1,1,1,1,1,1,1,1,1,1,1,1,1,1,1,1,
1,1,1,1,1,1,1,1,1,1,1,1,1,1,1,1,1,1,1,1,1,1,1,1,1,1,1,1,1,1,1,1,1,1,1,1,
1,1,1,1,1,1,1,1,1,1,1,1,1,1,1,1,1,1,1,1,1,1,1,1,1,1,1,1,1,1,1,1,1,1,1,1,
1,1,1,1,1,1,1,1,1,1,1,1,1,1,1,1,1,1,1,1,1,1,1,6),(0.,0.005,0.01,0.015,0.02,
0.025,0.03,0.035,0.04,0.045,0.05,0.055,0.06,0.065,0.07,0.075,0.08,0.085,
0.09,0.095,0.1,0.105,0.11,0.115,0.12,0.125,0.13,0.135,0.14,0.145,0.15,0.155,
0.16,0.165,0.17,0.175,0.18,0.185,0.19,0.195,0.2,0.205,0.21,0.215,0.22,0.225,
0.23,0.235,0.24,0.245,0.25,0.255,0.26,0.265,0.27,0.275,0.28,0.285,0.29,
0.295,0.3,0.305,0.31,0.315,0.32,0.325,0.33,0.335,0.34,0.345,0.35,0.355,
0.36,0.365,0.37,0.375,0.38,0.385,0.39,0.395,0.4,0.405,0.41,0.415,0.42,0.425,
0.43,0.435,0.44,0.445,0.45,0.455,0.46,0.465,0.47,0.475,0.48,0.485,0.49,
0.495,0.5,0.505,0.51,0.515,0.52,0.525,0.53,0.535,0.54,0.545,0.55,0.555,
0.56,0.565,0.57,0.575,0.58,0.585,0.59,0.595,0.6,0.605,0.61,0.615,0.62,0.625,
0.63,0.635,0.64,0.645,0.65,0.655,0.66,0.665,0.67,0.675,0.68,0.685,0.690000000000001,
0.695000000000001,0.700000000000001,0.705000000000001,0.710000000000001,
0.715000000000001,0.720000000000001,0.725000000000001,0.730000000000001,
0.735000000000001,0.740000000000001,0.745000000000001,0.750000000000001,
0.755000000000001,0.760000000000001,0.765000000000001,0.770000000000001,
0.775000000000001,0.780000000000001,0.785000000000001,0.790000000000001,
0.795000000000001,0.800000000000001,0.805000000000001,0.810000000000001,
0.815000000000001,0.820000000000001,0.825000000000001,0.830000000000001,
0.835000000000001,0.840000000000001,0.845000000000001,0.850000000000001,
0.855000000000001,0.860000000000001,0.865000000000001,0.870000000000001,
0.875000000000001,0.880000000000001,0.885000000000001,0.890000000000001,
0.895000000000001,0.900000000000001,0.905000000000001,0.910000000000001,
0.915000000000001,0.920000000000001,0.925000000000001,0.930000000000001,
0.935000000000001,0.940000000000001,0.94142984443127),.UNSPECIFIED.)
CURVE()
GEOMETRIC_REPRESENTATION_ITEM()
RATIONAL_B_SPLINE_CURVE((1.,1.,1.,1.,1.,1.,1.,1.,1.,1.,1.,1.,1.,1.,1.,1.,
1.,1.,1.,1.,1.,1.,1.,1.,1.,1.,1.,1.,1.,1.,1.,1.,1.,1.,1.,1.,1.,1.,1.,1.,
1.,1.,1.,1.,1.,1.,1.,1.,1.,1.,1.,1.,1.,1.,1.,1.,1.,1.,1.,1.,1.,1.,1.,1.,
1.,1.,1.,1.,1.,1.,1.,1.,1.,1.,1.,1.,1.,1.,1.,1.,1.,1.,1.,1.,1.,1.,1.,1.,
1.,1.,1.,1.,1.,1.,1.,1.,1.,1.,1.,1.,1.,1.,1.,1.,1.,1.,1.,1.,1.,1.,1.,1.,
1.,1.,1.,1.,1.,1.,1.,1.,1.,1.,1.,1.,1.,1.,1.,1.,1.,1.,1.,1.,1.,1.,1.,1.,
1.,1.,1.,1.,1.,1.,1.,1.,1.,1.,1.,1.,1.,1.,1.,1.,1.,1.,1.,1.,1.,1.,1.,1.,
1.,1.,1.,1.,1.,1.,1.,1.,1.,1.,1.,1.,1.,1.,1.,1.,1.,1.,1.,1.,1.,1.,1.,1.,
1.,1.,1.,1.,1.,1.,1.,1.,1.,1.))
REPRESENTATION_ITEM('')
);
#496=(
BOUNDED_CURVE()
B_SPLINE_CURVE(5,(#94445,#94446,#94447,#94448,#94449,#94450,#94451,#94452,
#94453,#94454,#94455,#94456,#94457,#94458,#94459,#94460,#94461,#94462,#94463,
#94464,#94465,#94466,#94467,#94468,#94469,#94470,#94471,#94472,#94473,#94474,
#94475,#94476,#94477,#94478,#94479,#94480,#94481,#94482,#94483,#94484,#94485,
#94486,#94487,#94488,#94489,#94490,#94491,#94492,#94493,#94494,#94495,#94496,
#94497,#94498,#94499,#94500,#94501,#94502,#94503,#94504,#94505,#94506,#94507,
#94508,#94509,#94510,#94511,#94512,#94513,#94514,#94515,#94516,#94517,#94518,
#94519,#94520,#94521,#94522,#94523,#94524,#94525,#94526,#94527,#94528,#94529,
#94530,#94531,#94532,#94533,#94534,#94535,#94536,#94537,#94538,#94539,#94540,
#94541,#94542,#94543,#94544,#94545,#94546,#94547,#94548,#94549,#94550,#94551,
#94552,#94553,#94554,#94555,#94556,#94557,#94558,#94559,#94560,#94561,#94562,
#94563,#94564,#94565,#94566,#94567,#94568,#94569,#94570,#94571,#94572,#94573,
#94574,#94575,#94576,#94577,#94578,#94579,#94580,#94581,#94582,#94583,#94584,
#94585,#94586,#94587,#94588,#94589,#94590,#94591,#94592,#94593,#94594,#94595,
#94596,#94597,#94598,#94599,#94600,#94601,#94602,#94603,#94604,#94605,#94606,
#94607,#94608,#94609,#94610,#94611,#94612,#94613,#94614,#94615,#94616,#94617,
#94618,#94619,#94620,#94621,#94622,#94623,#94624,#94625,#94626,#94627,#94628,
#94629,#94630,#94631,#94632,#94633,#94634,#94635,#94636,#94637,#94638),
 .UNSPECIFIED.,.F.,.F.)
B_SPLINE_CURVE_WITH_KNOTS((6,1,1,1,1,1,1,1,1,1,1,1,1,1,1,1,1,1,1,1,1,1,
1,1,1,1,1,1,1,1,1,1,1,1,1,1,1,1,1,1,1,1,1,1,1,1,1,1,1,1,1,1,1,1,1,1,1,1,
1,1,1,1,1,1,1,1,1,1,1,1,1,1,1,1,1,1,1,1,1,1,1,1,1,1,1,1,1,1,1,1,1,1,1,1,
1,1,1,1,1,1,1,1,1,1,1,1,1,1,1,1,1,1,1,1,1,1,1,1,1,1,1,1,1,1,1,1,1,1,1,1,
1,1,1,1,1,1,1,1,1,1,1,1,1,1,1,1,1,1,1,1,1,1,1,1,1,1,1,1,1,1,1,1,1,1,1,1,
1,1,1,1,1,1,1,1,1,1,1,1,1,1,1,1,1,1,1,1,1,1,1,6),(-0.941429844431257,-0.940000000000001,
-0.935000000000001,-0.930000000000001,-0.925000000000001,-0.920000000000001,
-0.915000000000001,-0.910000000000001,-0.905000000000001,-0.900000000000001,
-0.895000000000001,-0.890000000000001,-0.885000000000001,-0.880000000000001,
-0.875000000000001,-0.870000000000001,-0.865000000000001,-0.860000000000001,
-0.855000000000001,-0.850000000000001,-0.845000000000001,-0.840000000000001,
-0.835000000000001,-0.830000000000001,-0.825000000000001,-0.820000000000001,
-0.815000000000001,-0.810000000000001,-0.805000000000001,-0.800000000000001,
-0.795000000000001,-0.790000000000001,-0.785000000000001,-0.780000000000001,
-0.775000000000001,-0.770000000000001,-0.765000000000001,-0.760000000000001,
-0.755000000000001,-0.750000000000001,-0.745000000000001,-0.740000000000001,
-0.735000000000001,-0.730000000000001,-0.725000000000001,-0.720000000000001,
-0.715000000000001,-0.710000000000001,-0.705000000000001,-0.700000000000001,
-0.695000000000001,-0.690000000000001,-0.685,-0.68,-0.675,-0.67,-0.665,
-0.66,-0.655,-0.65,-0.645,-0.64,-0.635,-0.63,-0.625,-0.62,-0.615,-0.61,
-0.605,-0.6,-0.595,-0.59,-0.585,-0.58,-0.575,-0.57,-0.565,-0.56,-0.555,
-0.55,-0.545,-0.54,-0.535,-0.53,-0.525,-0.52,-0.515,-0.51,-0.505,-0.5,-0.495,
-0.49,-0.485,-0.48,-0.475,-0.47,-0.465,-0.46,-0.455,-0.45,-0.445,-0.44,
-0.435,-0.43,-0.425,-0.42,-0.415,-0.41,-0.405,-0.4,-0.395,-0.39,-0.385,
-0.38,-0.375,-0.37,-0.365,-0.36,-0.355,-0.35,-0.345,-0.34,-0.335,-0.33,
-0.325,-0.32,-0.315,-0.31,-0.305,-0.3,-0.295,-0.29,-0.285,-0.28,-0.275,
-0.27,-0.265,-0.26,-0.255,-0.25,-0.245,-0.24,-0.235,-0.23,-0.225,-0.22,
-0.215,-0.21,-0.205,-0.2,-0.195,-0.19,-0.185,-0.18,-0.175,-0.17,-0.165,
-0.16,-0.155,-0.15,-0.145,-0.14,-0.135,-0.13,-0.125,-0.12,-0.115,-0.11,
-0.105,-0.1,-0.095,-0.09,-0.085,-0.08,-0.075,-0.07,-0.065,-0.06,-0.055,
-0.05,-0.045,-0.04,-0.035,-0.03,-0.025,-0.02,-0.015,-0.01,-0.005,0.),
 .UNSPECIFIED.)
CURVE()
GEOMETRIC_REPRESENTATION_ITEM()
RATIONAL_B_SPLINE_CURVE((1.,1.,1.,1.,1.,1.,1.,1.,1.,1.,1.,1.,1.,1.,1.,1.,
1.,1.,1.,1.,1.,1.,1.,1.,1.,1.,1.,1.,1.,1.,1.,1.,1.,1.,1.,1.,1.,1.,1.,1.,
1.,1.,1.,1.,1.,1.,1.,1.,1.,1.,1.,1.,1.,1.,1.,1.,1.,1.,1.,1.,1.,1.,1.,1.,
1.,1.,1.,1.,1.,1.,1.,1.,1.,1.,1.,1.,1.,1.,1.,1.,1.,1.,1.,1.,1.,1.,1.,1.,
1.,1.,1.,1.,1.,1.,1.,1.,1.,1.,1.,1.,1.,1.,1.,1.,1.,1.,1.,1.,1.,1.,1.,1.,
1.,1.,1.,1.,1.,1.,1.,1.,1.,1.,1.,1.,1.,1.,1.,1.,1.,1.,1.,1.,1.,1.,1.,1.,
1.,1.,1.,1.,1.,1.,1.,1.,1.,1.,1.,1.,1.,1.,1.,1.,1.,1.,1.,1.,1.,1.,1.,1.,
1.,1.,1.,1.,1.,1.,1.,1.,1.,1.,1.,1.,1.,1.,1.,1.,1.,1.,1.,1.,1.,1.,1.,1.,
1.,1.,1.,1.,1.,1.,1.,1.,1.,1.))
REPRESENTATION_ITEM('')
);
#497=(
BOUNDED_CURVE()
B_SPLINE_CURVE(5,(#95145,#95146,#95147,#95148,#95149,#95150,#95151,#95152,
#95153,#95154,#95155,#95156,#95157,#95158,#95159,#95160,#95161,#95162,#95163,
#95164,#95165,#95166,#95167,#95168,#95169,#95170,#95171,#95172,#95173,#95174,
#95175,#95176,#95177,#95178,#95179,#95180,#95181,#95182,#95183,#95184,#95185,
#95186,#95187,#95188,#95189,#95190,#95191,#95192,#95193,#95194,#95195,#95196,
#95197,#95198,#95199,#95200,#95201,#95202,#95203,#95204,#95205,#95206,#95207,
#95208,#95209,#95210,#95211,#95212,#95213,#95214,#95215,#95216,#95217,#95218,
#95219,#95220,#95221,#95222,#95223,#95224,#95225,#95226,#95227,#95228,#95229,
#95230,#95231,#95232,#95233,#95234,#95235,#95236,#95237,#95238,#95239,#95240,
#95241,#95242,#95243,#95244,#95245,#95246,#95247,#95248,#95249,#95250,#95251,
#95252,#95253,#95254,#95255,#95256,#95257,#95258,#95259,#95260,#95261,#95262,
#95263,#95264,#95265,#95266,#95267,#95268,#95269,#95270,#95271,#95272,#95273,
#95274,#95275,#95276,#95277,#95278,#95279,#95280,#95281,#95282,#95283,#95284,
#95285,#95286,#95287,#95288,#95289,#95290,#95291,#95292,#95293,#95294,#95295,
#95296,#95297,#95298,#95299,#95300,#95301,#95302,#95303,#95304,#95305,#95306,
#95307,#95308,#95309,#95310,#95311,#95312,#95313,#95314,#95315,#95316,#95317,
#95318,#95319,#95320,#95321,#95322,#95323,#95324,#95325,#95326,#95327,#95328,
#95329,#95330,#95331,#95332,#95333,#95334,#95335,#95336,#95337,#95338),
 .UNSPECIFIED.,.F.,.F.)
B_SPLINE_CURVE_WITH_KNOTS((6,1,1,1,1,1,1,1,1,1,1,1,1,1,1,1,1,1,1,1,1,1,
1,1,1,1,1,1,1,1,1,1,1,1,1,1,1,1,1,1,1,1,1,1,1,1,1,1,1,1,1,1,1,1,1,1,1,1,
1,1,1,1,1,1,1,1,1,1,1,1,1,1,1,1,1,1,1,1,1,1,1,1,1,1,1,1,1,1,1,1,1,1,1,1,
1,1,1,1,1,1,1,1,1,1,1,1,1,1,1,1,1,1,1,1,1,1,1,1,1,1,1,1,1,1,1,1,1,1,1,1,
1,1,1,1,1,1,1,1,1,1,1,1,1,1,1,1,1,1,1,1,1,1,1,1,1,1,1,1,1,1,1,1,1,1,1,1,
1,1,1,1,1,1,1,1,1,1,1,1,1,1,1,1,1,1,1,1,1,1,1,6),(0.,0.005,0.01,0.015,0.02,
0.025,0.03,0.035,0.04,0.045,0.05,0.055,0.06,0.065,0.07,0.075,0.08,0.085,
0.09,0.095,0.1,0.105,0.11,0.115,0.12,0.125,0.13,0.135,0.14,0.145,0.15,0.155,
0.16,0.165,0.17,0.175,0.18,0.185,0.19,0.195,0.2,0.205,0.21,0.215,0.22,0.225,
0.23,0.235,0.24,0.245,0.25,0.255,0.26,0.265,0.27,0.275,0.28,0.285,0.29,
0.295,0.3,0.305,0.31,0.315,0.32,0.325,0.33,0.335,0.34,0.345,0.35,0.355,
0.36,0.365,0.37,0.375,0.38,0.385,0.39,0.395,0.4,0.405,0.41,0.415,0.42,0.425,
0.43,0.435,0.44,0.445,0.45,0.455,0.46,0.465,0.47,0.475,0.48,0.485,0.49,
0.495,0.5,0.505,0.51,0.515,0.52,0.525,0.53,0.535,0.54,0.545,0.55,0.555,
0.56,0.565,0.57,0.575,0.58,0.585,0.59,0.595,0.6,0.605,0.61,0.615,0.62,0.625,
0.63,0.635,0.64,0.645,0.65,0.655,0.66,0.665,0.67,0.675,0.68,0.685,0.690000000000001,
0.695000000000001,0.700000000000001,0.705000000000001,0.710000000000001,
0.715000000000001,0.720000000000001,0.725000000000001,0.730000000000001,
0.735000000000001,0.740000000000001,0.745000000000001,0.750000000000001,
0.755000000000001,0.760000000000001,0.765000000000001,0.770000000000001,
0.775000000000001,0.780000000000001,0.785000000000001,0.790000000000001,
0.795000000000001,0.800000000000001,0.805000000000001,0.810000000000001,
0.815000000000001,0.820000000000001,0.825000000000001,0.830000000000001,
0.835000000000001,0.840000000000001,0.845000000000001,0.850000000000001,
0.855000000000001,0.860000000000001,0.865000000000001,0.870000000000001,
0.875000000000001,0.880000000000001,0.885000000000001,0.890000000000001,
0.895000000000001,0.900000000000001,0.905000000000001,0.910000000000001,
0.915000000000001,0.920000000000001,0.925000000000001,0.930000000000001,
0.935000000000001,0.940000000000001,0.9414298444314),.UNSPECIFIED.)
CURVE()
GEOMETRIC_REPRESENTATION_ITEM()
RATIONAL_B_SPLINE_CURVE((1.,1.,1.,1.,1.,1.,1.,1.,1.,1.,1.,1.,1.,1.,1.,1.,
1.,1.,1.,1.,1.,1.,1.,1.,1.,1.,1.,1.,1.,1.,1.,1.,1.,1.,1.,1.,1.,1.,1.,1.,
1.,1.,1.,1.,1.,1.,1.,1.,1.,1.,1.,1.,1.,1.,1.,1.,1.,1.,1.,1.,1.,1.,1.,1.,
1.,1.,1.,1.,1.,1.,1.,1.,1.,1.,1.,1.,1.,1.,1.,1.,1.,1.,1.,1.,1.,1.,1.,1.,
1.,1.,1.,1.,1.,1.,1.,1.,1.,1.,1.,1.,1.,1.,1.,1.,1.,1.,1.,1.,1.,1.,1.,1.,
1.,1.,1.,1.,1.,1.,1.,1.,1.,1.,1.,1.,1.,1.,1.,1.,1.,1.,1.,1.,1.,1.,1.,1.,
1.,1.,1.,1.,1.,1.,1.,1.,1.,1.,1.,1.,1.,1.,1.,1.,1.,1.,1.,1.,1.,1.,1.,1.,
1.,1.,1.,1.,1.,1.,1.,1.,1.,1.,1.,1.,1.,1.,1.,1.,1.,1.,1.,1.,1.,1.,1.,1.,
1.,1.,1.,1.,1.,1.,1.,1.,1.,1.))
REPRESENTATION_ITEM('')
);
#498=(
BOUNDED_CURVE()
B_SPLINE_CURVE(5,(#95341,#95342,#95343,#95344,#95345,#95346,#95347,#95348,
#95349,#95350,#95351,#95352,#95353,#95354,#95355,#95356,#95357,#95358,#95359,
#95360,#95361,#95362,#95363,#95364,#95365,#95366,#95367,#95368,#95369,#95370,
#95371,#95372,#95373,#95374,#95375,#95376,#95377,#95378,#95379,#95380,#95381,
#95382,#95383,#95384,#95385,#95386,#95387,#95388,#95389,#95390,#95391,#95392,
#95393,#95394,#95395,#95396,#95397,#95398,#95399,#95400,#95401,#95402,#95403,
#95404,#95405,#95406,#95407,#95408,#95409,#95410,#95411,#95412,#95413,#95414,
#95415,#95416,#95417,#95418,#95419,#95420,#95421,#95422,#95423,#95424,#95425,
#95426,#95427,#95428,#95429,#95430,#95431,#95432,#95433,#95434,#95435,#95436,
#95437,#95438,#95439,#95440,#95441,#95442,#95443,#95444,#95445,#95446,#95447,
#95448,#95449,#95450,#95451,#95452,#95453,#95454,#95455,#95456,#95457,#95458,
#95459,#95460,#95461,#95462,#95463,#95464,#95465,#95466,#95467,#95468,#95469,
#95470,#95471,#95472,#95473,#95474,#95475,#95476,#95477,#95478,#95479,#95480,
#95481,#95482,#95483,#95484,#95485,#95486,#95487,#95488,#95489,#95490,#95491,
#95492,#95493,#95494,#95495,#95496,#95497,#95498,#95499,#95500,#95501,#95502,
#95503,#95504,#95505,#95506,#95507,#95508,#95509,#95510,#95511,#95512,#95513,
#95514,#95515,#95516,#95517,#95518,#95519,#95520,#95521,#95522,#95523,#95524,
#95525,#95526,#95527,#95528,#95529,#95530,#95531,#95532,#95533,#95534),
 .UNSPECIFIED.,.F.,.F.)
B_SPLINE_CURVE_WITH_KNOTS((6,1,1,1,1,1,1,1,1,1,1,1,1,1,1,1,1,1,1,1,1,1,
1,1,1,1,1,1,1,1,1,1,1,1,1,1,1,1,1,1,1,1,1,1,1,1,1,1,1,1,1,1,1,1,1,1,1,1,
1,1,1,1,1,1,1,1,1,1,1,1,1,1,1,1,1,1,1,1,1,1,1,1,1,1,1,1,1,1,1,1,1,1,1,1,
1,1,1,1,1,1,1,1,1,1,1,1,1,1,1,1,1,1,1,1,1,1,1,1,1,1,1,1,1,1,1,1,1,1,1,1,
1,1,1,1,1,1,1,1,1,1,1,1,1,1,1,1,1,1,1,1,1,1,1,1,1,1,1,1,1,1,1,1,1,1,1,1,
1,1,1,1,1,1,1,1,1,1,1,1,1,1,1,1,1,1,1,1,1,1,1,6),(-0.941429844431388,-0.940000000000001,
-0.935000000000001,-0.930000000000001,-0.925000000000001,-0.920000000000001,
-0.915000000000001,-0.910000000000001,-0.905000000000001,-0.900000000000001,
-0.895000000000001,-0.890000000000001,-0.885000000000001,-0.880000000000001,
-0.875000000000001,-0.870000000000001,-0.865000000000001,-0.860000000000001,
-0.855000000000001,-0.850000000000001,-0.845000000000001,-0.840000000000001,
-0.835000000000001,-0.830000000000001,-0.825000000000001,-0.820000000000001,
-0.815000000000001,-0.810000000000001,-0.805000000000001,-0.800000000000001,
-0.795000000000001,-0.790000000000001,-0.785000000000001,-0.780000000000001,
-0.775000000000001,-0.770000000000001,-0.765000000000001,-0.760000000000001,
-0.755000000000001,-0.750000000000001,-0.745000000000001,-0.740000000000001,
-0.735000000000001,-0.730000000000001,-0.725000000000001,-0.720000000000001,
-0.715000000000001,-0.710000000000001,-0.705000000000001,-0.700000000000001,
-0.695000000000001,-0.690000000000001,-0.685,-0.68,-0.675,-0.67,-0.665,
-0.66,-0.655,-0.65,-0.645,-0.64,-0.635,-0.63,-0.625,-0.62,-0.615,-0.61,
-0.605,-0.6,-0.595,-0.59,-0.585,-0.58,-0.575,-0.57,-0.565,-0.56,-0.555,
-0.55,-0.545,-0.54,-0.535,-0.53,-0.525,-0.52,-0.515,-0.51,-0.505,-0.5,-0.495,
-0.49,-0.485,-0.48,-0.475,-0.47,-0.465,-0.46,-0.455,-0.45,-0.445,-0.44,
-0.435,-0.43,-0.425,-0.42,-0.415,-0.41,-0.405,-0.4,-0.395,-0.39,-0.385,
-0.38,-0.375,-0.37,-0.365,-0.36,-0.355,-0.35,-0.345,-0.34,-0.335,-0.33,
-0.325,-0.32,-0.315,-0.31,-0.305,-0.3,-0.295,-0.29,-0.285,-0.28,-0.275,
-0.27,-0.265,-0.26,-0.255,-0.25,-0.245,-0.24,-0.235,-0.23,-0.225,-0.22,
-0.215,-0.21,-0.205,-0.2,-0.195,-0.19,-0.185,-0.18,-0.175,-0.17,-0.165,
-0.16,-0.155,-0.15,-0.145,-0.14,-0.135,-0.13,-0.125,-0.12,-0.115,-0.11,
-0.105,-0.1,-0.095,-0.09,-0.085,-0.08,-0.075,-0.07,-0.065,-0.06,-0.055,
-0.05,-0.045,-0.04,-0.035,-0.03,-0.025,-0.02,-0.015,-0.01,-0.005,0.),
 .UNSPECIFIED.)
CURVE()
GEOMETRIC_REPRESENTATION_ITEM()
RATIONAL_B_SPLINE_CURVE((1.,1.,1.,1.,1.,1.,1.,1.,1.,1.,1.,1.,1.,1.,1.,1.,
1.,1.,1.,1.,1.,1.,1.,1.,1.,1.,1.,1.,1.,1.,1.,1.,1.,1.,1.,1.,1.,1.,1.,1.,
1.,1.,1.,1.,1.,1.,1.,1.,1.,1.,1.,1.,1.,1.,1.,1.,1.,1.,1.,1.,1.,1.,1.,1.,
1.,1.,1.,1.,1.,1.,1.,1.,1.,1.,1.,1.,1.,1.,1.,1.,1.,1.,1.,1.,1.,1.,1.,1.,
1.,1.,1.,1.,1.,1.,1.,1.,1.,1.,1.,1.,1.,1.,1.,1.,1.,1.,1.,1.,1.,1.,1.,1.,
1.,1.,1.,1.,1.,1.,1.,1.,1.,1.,1.,1.,1.,1.,1.,1.,1.,1.,1.,1.,1.,1.,1.,1.,
1.,1.,1.,1.,1.,1.,1.,1.,1.,1.,1.,1.,1.,1.,1.,1.,1.,1.,1.,1.,1.,1.,1.,1.,
1.,1.,1.,1.,1.,1.,1.,1.,1.,1.,1.,1.,1.,1.,1.,1.,1.,1.,1.,1.,1.,1.,1.,1.,
1.,1.,1.,1.,1.,1.,1.,1.,1.,1.))
REPRESENTATION_ITEM('')
);
#499=(
BOUNDED_CURVE()
B_SPLINE_CURVE(5,(#96041,#96042,#96043,#96044,#96045,#96046,#96047,#96048,
#96049,#96050,#96051,#96052,#96053,#96054,#96055,#96056,#96057,#96058,#96059,
#96060,#96061,#96062,#96063,#96064,#96065,#96066,#96067,#96068,#96069,#96070,
#96071,#96072,#96073,#96074,#96075,#96076,#96077,#96078,#96079,#96080,#96081,
#96082,#96083,#96084,#96085,#96086,#96087,#96088,#96089,#96090,#96091,#96092,
#96093,#96094,#96095,#96096,#96097,#96098,#96099,#96100,#96101,#96102,#96103,
#96104,#96105,#96106,#96107,#96108,#96109,#96110,#96111,#96112,#96113,#96114,
#96115,#96116,#96117,#96118,#96119,#96120,#96121,#96122,#96123,#96124,#96125,
#96126,#96127,#96128,#96129,#96130,#96131,#96132,#96133,#96134,#96135,#96136,
#96137,#96138,#96139,#96140,#96141,#96142,#96143,#96144,#96145,#96146,#96147,
#96148,#96149,#96150,#96151,#96152,#96153,#96154,#96155,#96156,#96157,#96158,
#96159,#96160,#96161,#96162,#96163,#96164,#96165,#96166,#96167,#96168,#96169,
#96170,#96171,#96172,#96173,#96174,#96175,#96176,#96177,#96178,#96179,#96180,
#96181,#96182,#96183,#96184,#96185,#96186,#96187,#96188,#96189,#96190,#96191,
#96192,#96193,#96194,#96195,#96196,#96197,#96198,#96199,#96200,#96201,#96202,
#96203,#96204,#96205,#96206,#96207,#96208,#96209,#96210,#96211,#96212,#96213,
#96214,#96215,#96216,#96217,#96218,#96219,#96220,#96221,#96222,#96223,#96224,
#96225,#96226,#96227,#96228,#96229,#96230,#96231,#96232,#96233,#96234),
 .UNSPECIFIED.,.F.,.F.)
B_SPLINE_CURVE_WITH_KNOTS((6,1,1,1,1,1,1,1,1,1,1,1,1,1,1,1,1,1,1,1,1,1,
1,1,1,1,1,1,1,1,1,1,1,1,1,1,1,1,1,1,1,1,1,1,1,1,1,1,1,1,1,1,1,1,1,1,1,1,
1,1,1,1,1,1,1,1,1,1,1,1,1,1,1,1,1,1,1,1,1,1,1,1,1,1,1,1,1,1,1,1,1,1,1,1,
1,1,1,1,1,1,1,1,1,1,1,1,1,1,1,1,1,1,1,1,1,1,1,1,1,1,1,1,1,1,1,1,1,1,1,1,
1,1,1,1,1,1,1,1,1,1,1,1,1,1,1,1,1,1,1,1,1,1,1,1,1,1,1,1,1,1,1,1,1,1,1,1,
1,1,1,1,1,1,1,1,1,1,1,1,1,1,1,1,1,1,1,1,1,1,1,6),(0.,0.005,0.01,0.015,0.02,
0.025,0.03,0.035,0.04,0.045,0.05,0.055,0.06,0.065,0.07,0.075,0.08,0.085,
0.09,0.095,0.1,0.105,0.11,0.115,0.12,0.125,0.13,0.135,0.14,0.145,0.15,0.155,
0.16,0.165,0.17,0.175,0.18,0.185,0.19,0.195,0.2,0.205,0.21,0.215,0.22,0.225,
0.23,0.235,0.24,0.245,0.25,0.255,0.26,0.265,0.27,0.275,0.28,0.285,0.29,
0.295,0.3,0.305,0.31,0.315,0.32,0.325,0.33,0.335,0.34,0.345,0.35,0.355,
0.36,0.365,0.37,0.375,0.38,0.385,0.39,0.395,0.4,0.405,0.41,0.415,0.42,0.425,
0.43,0.435,0.44,0.445,0.45,0.455,0.46,0.465,0.47,0.475,0.48,0.485,0.49,
0.495,0.5,0.505,0.51,0.515,0.52,0.525,0.53,0.535,0.54,0.545,0.55,0.555,
0.56,0.565,0.57,0.575,0.58,0.585,0.59,0.595,0.6,0.605,0.61,0.615,0.62,0.625,
0.63,0.635,0.64,0.645,0.65,0.655,0.66,0.665,0.67,0.675,0.68,0.685,0.690000000000001,
0.695000000000001,0.700000000000001,0.705000000000001,0.710000000000001,
0.715000000000001,0.720000000000001,0.725000000000001,0.730000000000001,
0.735000000000001,0.740000000000001,0.745000000000001,0.750000000000001,
0.755000000000001,0.760000000000001,0.765000000000001,0.770000000000001,
0.775000000000001,0.780000000000001,0.785000000000001,0.790000000000001,
0.795000000000001,0.800000000000001,0.805000000000001,0.810000000000001,
0.815000000000001,0.820000000000001,0.825000000000001,0.830000000000001,
0.835000000000001,0.840000000000001,0.845000000000001,0.850000000000001,
0.855000000000001,0.860000000000001,0.865000000000001,0.870000000000001,
0.875000000000001,0.880000000000001,0.885000000000001,0.890000000000001,
0.895000000000001,0.900000000000001,0.905000000000001,0.910000000000001,
0.915000000000001,0.920000000000001,0.925000000000001,0.930000000000001,
0.935000000000001,0.940000000000001,0.941429844431407),.UNSPECIFIED.)
CURVE()
GEOMETRIC_REPRESENTATION_ITEM()
RATIONAL_B_SPLINE_CURVE((1.,1.,1.,1.,1.,1.,1.,1.,1.,1.,1.,1.,1.,1.,1.,1.,
1.,1.,1.,1.,1.,1.,1.,1.,1.,1.,1.,1.,1.,1.,1.,1.,1.,1.,1.,1.,1.,1.,1.,1.,
1.,1.,1.,1.,1.,1.,1.,1.,1.,1.,1.,1.,1.,1.,1.,1.,1.,1.,1.,1.,1.,1.,1.,1.,
1.,1.,1.,1.,1.,1.,1.,1.,1.,1.,1.,1.,1.,1.,1.,1.,1.,1.,1.,1.,1.,1.,1.,1.,
1.,1.,1.,1.,1.,1.,1.,1.,1.,1.,1.,1.,1.,1.,1.,1.,1.,1.,1.,1.,1.,1.,1.,1.,
1.,1.,1.,1.,1.,1.,1.,1.,1.,1.,1.,1.,1.,1.,1.,1.,1.,1.,1.,1.,1.,1.,1.,1.,
1.,1.,1.,1.,1.,1.,1.,1.,1.,1.,1.,1.,1.,1.,1.,1.,1.,1.,1.,1.,1.,1.,1.,1.,
1.,1.,1.,1.,1.,1.,1.,1.,1.,1.,1.,1.,1.,1.,1.,1.,1.,1.,1.,1.,1.,1.,1.,1.,
1.,1.,1.,1.,1.,1.,1.,1.,1.,1.))
REPRESENTATION_ITEM('')
);
#500=(
BOUNDED_CURVE()
B_SPLINE_CURVE(5,(#96237,#96238,#96239,#96240,#96241,#96242,#96243,#96244,
#96245,#96246,#96247,#96248,#96249,#96250,#96251,#96252,#96253,#96254,#96255,
#96256,#96257,#96258,#96259,#96260,#96261,#96262,#96263,#96264,#96265,#96266,
#96267,#96268,#96269,#96270,#96271,#96272,#96273,#96274,#96275,#96276,#96277,
#96278,#96279,#96280,#96281,#96282,#96283,#96284,#96285,#96286,#96287,#96288,
#96289,#96290,#96291,#96292,#96293,#96294,#96295,#96296,#96297,#96298,#96299,
#96300,#96301,#96302,#96303,#96304,#96305,#96306,#96307,#96308,#96309,#96310,
#96311,#96312,#96313,#96314,#96315,#96316,#96317,#96318,#96319,#96320,#96321,
#96322,#96323,#96324,#96325,#96326,#96327,#96328,#96329,#96330,#96331,#96332,
#96333,#96334,#96335,#96336,#96337,#96338,#96339,#96340,#96341,#96342,#96343,
#96344,#96345,#96346,#96347,#96348,#96349,#96350,#96351,#96352,#96353,#96354,
#96355,#96356,#96357,#96358,#96359,#96360,#96361,#96362,#96363,#96364,#96365,
#96366,#96367,#96368,#96369,#96370,#96371,#96372,#96373,#96374,#96375,#96376,
#96377,#96378,#96379,#96380,#96381,#96382,#96383,#96384,#96385,#96386,#96387,
#96388,#96389,#96390,#96391,#96392,#96393,#96394,#96395,#96396,#96397,#96398,
#96399,#96400,#96401,#96402,#96403,#96404,#96405,#96406,#96407,#96408,#96409,
#96410,#96411,#96412,#96413,#96414,#96415,#96416,#96417,#96418,#96419,#96420,
#96421,#96422,#96423,#96424,#96425,#96426,#96427,#96428,#96429,#96430),
 .UNSPECIFIED.,.F.,.F.)
B_SPLINE_CURVE_WITH_KNOTS((6,1,1,1,1,1,1,1,1,1,1,1,1,1,1,1,1,1,1,1,1,1,
1,1,1,1,1,1,1,1,1,1,1,1,1,1,1,1,1,1,1,1,1,1,1,1,1,1,1,1,1,1,1,1,1,1,1,1,
1,1,1,1,1,1,1,1,1,1,1,1,1,1,1,1,1,1,1,1,1,1,1,1,1,1,1,1,1,1,1,1,1,1,1,1,
1,1,1,1,1,1,1,1,1,1,1,1,1,1,1,1,1,1,1,1,1,1,1,1,1,1,1,1,1,1,1,1,1,1,1,1,
1,1,1,1,1,1,1,1,1,1,1,1,1,1,1,1,1,1,1,1,1,1,1,1,1,1,1,1,1,1,1,1,1,1,1,1,
1,1,1,1,1,1,1,1,1,1,1,1,1,1,1,1,1,1,1,1,1,1,1,6),(-0.941429844431431,-0.940000000000001,
-0.935000000000001,-0.930000000000001,-0.925000000000001,-0.920000000000001,
-0.915000000000001,-0.910000000000001,-0.905000000000001,-0.900000000000001,
-0.895000000000001,-0.890000000000001,-0.885000000000001,-0.880000000000001,
-0.875000000000001,-0.870000000000001,-0.865000000000001,-0.860000000000001,
-0.855000000000001,-0.850000000000001,-0.845000000000001,-0.840000000000001,
-0.835000000000001,-0.830000000000001,-0.825000000000001,-0.820000000000001,
-0.815000000000001,-0.810000000000001,-0.805000000000001,-0.800000000000001,
-0.795000000000001,-0.790000000000001,-0.785000000000001,-0.780000000000001,
-0.775000000000001,-0.770000000000001,-0.765000000000001,-0.760000000000001,
-0.755000000000001,-0.750000000000001,-0.745000000000001,-0.740000000000001,
-0.735000000000001,-0.730000000000001,-0.725000000000001,-0.720000000000001,
-0.715000000000001,-0.710000000000001,-0.705000000000001,-0.700000000000001,
-0.695000000000001,-0.690000000000001,-0.685,-0.68,-0.675,-0.67,-0.665,
-0.66,-0.655,-0.65,-0.645,-0.64,-0.635,-0.63,-0.625,-0.62,-0.615,-0.61,
-0.605,-0.6,-0.595,-0.59,-0.585,-0.58,-0.575,-0.57,-0.565,-0.56,-0.555,
-0.55,-0.545,-0.54,-0.535,-0.53,-0.525,-0.52,-0.515,-0.51,-0.505,-0.5,-0.495,
-0.49,-0.485,-0.48,-0.475,-0.47,-0.465,-0.46,-0.455,-0.45,-0.445,-0.44,
-0.435,-0.43,-0.425,-0.42,-0.415,-0.41,-0.405,-0.4,-0.395,-0.39,-0.385,
-0.38,-0.375,-0.37,-0.365,-0.36,-0.355,-0.35,-0.345,-0.34,-0.335,-0.33,
-0.325,-0.32,-0.315,-0.31,-0.305,-0.3,-0.295,-0.29,-0.285,-0.28,-0.275,
-0.27,-0.265,-0.26,-0.255,-0.25,-0.245,-0.24,-0.235,-0.23,-0.225,-0.22,
-0.215,-0.21,-0.205,-0.2,-0.195,-0.19,-0.185,-0.18,-0.175,-0.17,-0.165,
-0.16,-0.155,-0.15,-0.145,-0.14,-0.135,-0.13,-0.125,-0.12,-0.115,-0.11,
-0.105,-0.1,-0.095,-0.09,-0.085,-0.08,-0.075,-0.07,-0.065,-0.06,-0.055,
-0.05,-0.045,-0.04,-0.035,-0.03,-0.025,-0.02,-0.015,-0.01,-0.005,0.),
 .UNSPECIFIED.)
CURVE()
GEOMETRIC_REPRESENTATION_ITEM()
RATIONAL_B_SPLINE_CURVE((1.,1.,1.,1.,1.,1.,1.,1.,1.,1.,1.,1.,1.,1.,1.,1.,
1.,1.,1.,1.,1.,1.,1.,1.,1.,1.,1.,1.,1.,1.,1.,1.,1.,1.,1.,1.,1.,1.,1.,1.,
1.,1.,1.,1.,1.,1.,1.,1.,1.,1.,1.,1.,1.,1.,1.,1.,1.,1.,1.,1.,1.,1.,1.,1.,
1.,1.,1.,1.,1.,1.,1.,1.,1.,1.,1.,1.,1.,1.,1.,1.,1.,1.,1.,1.,1.,1.,1.,1.,
1.,1.,1.,1.,1.,1.,1.,1.,1.,1.,1.,1.,1.,1.,1.,1.,1.,1.,1.,1.,1.,1.,1.,1.,
1.,1.,1.,1.,1.,1.,1.,1.,1.,1.,1.,1.,1.,1.,1.,1.,1.,1.,1.,1.,1.,1.,1.,1.,
1.,1.,1.,1.,1.,1.,1.,1.,1.,1.,1.,1.,1.,1.,1.,1.,1.,1.,1.,1.,1.,1.,1.,1.,
1.,1.,1.,1.,1.,1.,1.,1.,1.,1.,1.,1.,1.,1.,1.,1.,1.,1.,1.,1.,1.,1.,1.,1.,
1.,1.,1.,1.,1.,1.,1.,1.,1.,1.))
REPRESENTATION_ITEM('')
);
#501=(
BOUNDED_CURVE()
B_SPLINE_CURVE(5,(#96937,#96938,#96939,#96940,#96941,#96942,#96943,#96944,
#96945,#96946,#96947,#96948,#96949,#96950,#96951,#96952,#96953,#96954,#96955,
#96956,#96957,#96958,#96959,#96960,#96961,#96962,#96963,#96964,#96965,#96966,
#96967,#96968,#96969,#96970,#96971,#96972,#96973,#96974,#96975,#96976,#96977,
#96978,#96979,#96980,#96981,#96982,#96983,#96984,#96985,#96986,#96987,#96988,
#96989,#96990,#96991,#96992,#96993,#96994,#96995,#96996,#96997,#96998,#96999,
#97000,#97001,#97002,#97003,#97004,#97005,#97006,#97007,#97008,#97009,#97010,
#97011,#97012,#97013,#97014,#97015,#97016,#97017,#97018,#97019,#97020,#97021,
#97022,#97023,#97024,#97025,#97026,#97027,#97028,#97029,#97030,#97031,#97032,
#97033,#97034,#97035,#97036,#97037,#97038,#97039,#97040,#97041,#97042,#97043,
#97044,#97045,#97046,#97047,#97048,#97049,#97050,#97051,#97052,#97053,#97054,
#97055,#97056,#97057,#97058,#97059,#97060,#97061,#97062,#97063,#97064,#97065,
#97066,#97067,#97068,#97069,#97070,#97071,#97072,#97073,#97074,#97075,#97076,
#97077,#97078,#97079,#97080,#97081,#97082,#97083,#97084,#97085,#97086,#97087,
#97088,#97089,#97090,#97091,#97092,#97093,#97094,#97095,#97096,#97097,#97098,
#97099,#97100,#97101,#97102,#97103,#97104,#97105,#97106,#97107,#97108,#97109,
#97110,#97111,#97112,#97113,#97114,#97115,#97116,#97117,#97118,#97119,#97120,
#97121,#97122,#97123,#97124,#97125,#97126,#97127,#97128,#97129,#97130),
 .UNSPECIFIED.,.F.,.F.)
B_SPLINE_CURVE_WITH_KNOTS((6,1,1,1,1,1,1,1,1,1,1,1,1,1,1,1,1,1,1,1,1,1,
1,1,1,1,1,1,1,1,1,1,1,1,1,1,1,1,1,1,1,1,1,1,1,1,1,1,1,1,1,1,1,1,1,1,1,1,
1,1,1,1,1,1,1,1,1,1,1,1,1,1,1,1,1,1,1,1,1,1,1,1,1,1,1,1,1,1,1,1,1,1,1,1,
1,1,1,1,1,1,1,1,1,1,1,1,1,1,1,1,1,1,1,1,1,1,1,1,1,1,1,1,1,1,1,1,1,1,1,1,
1,1,1,1,1,1,1,1,1,1,1,1,1,1,1,1,1,1,1,1,1,1,1,1,1,1,1,1,1,1,1,1,1,1,1,1,
1,1,1,1,1,1,1,1,1,1,1,1,1,1,1,1,1,1,1,1,1,1,1,6),(0.,0.005,0.01,0.015,0.02,
0.025,0.03,0.035,0.04,0.045,0.05,0.055,0.06,0.065,0.07,0.075,0.08,0.085,
0.09,0.095,0.1,0.105,0.11,0.115,0.12,0.125,0.13,0.135,0.14,0.145,0.15,0.155,
0.16,0.165,0.17,0.175,0.18,0.185,0.19,0.195,0.2,0.205,0.21,0.215,0.22,0.225,
0.23,0.235,0.24,0.245,0.25,0.255,0.26,0.265,0.27,0.275,0.28,0.285,0.29,
0.295,0.3,0.305,0.31,0.315,0.32,0.325,0.33,0.335,0.34,0.345,0.35,0.355,
0.36,0.365,0.37,0.375,0.38,0.385,0.39,0.395,0.4,0.405,0.41,0.415,0.42,0.425,
0.43,0.435,0.44,0.445,0.45,0.455,0.46,0.465,0.47,0.475,0.48,0.485,0.49,
0.495,0.5,0.505,0.51,0.515,0.52,0.525,0.53,0.535,0.54,0.545,0.55,0.555,
0.56,0.565,0.57,0.575,0.58,0.585,0.59,0.595,0.6,0.605,0.61,0.615,0.62,0.625,
0.63,0.635,0.64,0.645,0.65,0.655,0.66,0.665,0.67,0.675,0.68,0.685,0.690000000000001,
0.695000000000001,0.700000000000001,0.705000000000001,0.710000000000001,
0.715000000000001,0.720000000000001,0.725000000000001,0.730000000000001,
0.735000000000001,0.740000000000001,0.745000000000001,0.750000000000001,
0.755000000000001,0.760000000000001,0.765000000000001,0.770000000000001,
0.775000000000001,0.780000000000001,0.785000000000001,0.790000000000001,
0.795000000000001,0.800000000000001,0.805000000000001,0.810000000000001,
0.815000000000001,0.820000000000001,0.825000000000001,0.830000000000001,
0.835000000000001,0.840000000000001,0.845000000000001,0.850000000000001,
0.855000000000001,0.860000000000001,0.865000000000001,0.870000000000001,
0.875000000000001,0.880000000000001,0.885000000000001,0.890000000000001,
0.895000000000001,0.900000000000001,0.905000000000001,0.910000000000001,
0.915000000000001,0.920000000000001,0.925000000000001,0.930000000000001,
0.935000000000001,0.940000000000001,0.941429844431522),.UNSPECIFIED.)
CURVE()
GEOMETRIC_REPRESENTATION_ITEM()
RATIONAL_B_SPLINE_CURVE((1.,1.,1.,1.,1.,1.,1.,1.,1.,1.,1.,1.,1.,1.,1.,1.,
1.,1.,1.,1.,1.,1.,1.,1.,1.,1.,1.,1.,1.,1.,1.,1.,1.,1.,1.,1.,1.,1.,1.,1.,
1.,1.,1.,1.,1.,1.,1.,1.,1.,1.,1.,1.,1.,1.,1.,1.,1.,1.,1.,1.,1.,1.,1.,1.,
1.,1.,1.,1.,1.,1.,1.,1.,1.,1.,1.,1.,1.,1.,1.,1.,1.,1.,1.,1.,1.,1.,1.,1.,
1.,1.,1.,1.,1.,1.,1.,1.,1.,1.,1.,1.,1.,1.,1.,1.,1.,1.,1.,1.,1.,1.,1.,1.,
1.,1.,1.,1.,1.,1.,1.,1.,1.,1.,1.,1.,1.,1.,1.,1.,1.,1.,1.,1.,1.,1.,1.,1.,
1.,1.,1.,1.,1.,1.,1.,1.,1.,1.,1.,1.,1.,1.,1.,1.,1.,1.,1.,1.,1.,1.,1.,1.,
1.,1.,1.,1.,1.,1.,1.,1.,1.,1.,1.,1.,1.,1.,1.,1.,1.,1.,1.,1.,1.,1.,1.,1.,
1.,1.,1.,1.,1.,1.,1.,1.,1.,1.))
REPRESENTATION_ITEM('')
);
#502=(
BOUNDED_CURVE()
B_SPLINE_CURVE(5,(#97133,#97134,#97135,#97136,#97137,#97138,#97139,#97140,
#97141,#97142,#97143,#97144,#97145,#97146,#97147,#97148,#97149,#97150,#97151,
#97152,#97153,#97154,#97155,#97156,#97157,#97158,#97159,#97160,#97161,#97162,
#97163,#97164,#97165,#97166,#97167,#97168,#97169,#97170,#97171,#97172,#97173,
#97174,#97175,#97176,#97177,#97178,#97179,#97180,#97181,#97182,#97183,#97184,
#97185,#97186,#97187,#97188,#97189,#97190,#97191,#97192,#97193,#97194,#97195,
#97196,#97197,#97198,#97199,#97200,#97201,#97202,#97203,#97204,#97205,#97206,
#97207,#97208,#97209,#97210,#97211,#97212,#97213,#97214,#97215,#97216,#97217,
#97218,#97219,#97220,#97221,#97222,#97223,#97224,#97225,#97226,#97227,#97228,
#97229,#97230,#97231,#97232,#97233,#97234,#97235,#97236,#97237,#97238,#97239,
#97240,#97241,#97242,#97243,#97244,#97245,#97246,#97247,#97248,#97249,#97250,
#97251,#97252,#97253,#97254,#97255,#97256,#97257,#97258,#97259,#97260,#97261,
#97262,#97263,#97264,#97265,#97266,#97267,#97268,#97269,#97270,#97271,#97272,
#97273,#97274,#97275,#97276,#97277,#97278,#97279,#97280,#97281,#97282,#97283,
#97284,#97285,#97286,#97287,#97288,#97289,#97290,#97291,#97292,#97293,#97294,
#97295,#97296,#97297,#97298,#97299,#97300,#97301,#97302,#97303,#97304,#97305,
#97306,#97307,#97308,#97309,#97310,#97311,#97312,#97313,#97314,#97315,#97316,
#97317,#97318,#97319,#97320,#97321,#97322,#97323,#97324,#97325,#97326),
 .UNSPECIFIED.,.F.,.F.)
B_SPLINE_CURVE_WITH_KNOTS((6,1,1,1,1,1,1,1,1,1,1,1,1,1,1,1,1,1,1,1,1,1,
1,1,1,1,1,1,1,1,1,1,1,1,1,1,1,1,1,1,1,1,1,1,1,1,1,1,1,1,1,1,1,1,1,1,1,1,
1,1,1,1,1,1,1,1,1,1,1,1,1,1,1,1,1,1,1,1,1,1,1,1,1,1,1,1,1,1,1,1,1,1,1,1,
1,1,1,1,1,1,1,1,1,1,1,1,1,1,1,1,1,1,1,1,1,1,1,1,1,1,1,1,1,1,1,1,1,1,1,1,
1,1,1,1,1,1,1,1,1,1,1,1,1,1,1,1,1,1,1,1,1,1,1,1,1,1,1,1,1,1,1,1,1,1,1,1,
1,1,1,1,1,1,1,1,1,1,1,1,1,1,1,1,1,1,1,1,1,1,1,6),(-0.941429844431529,-0.940000000000001,
-0.935000000000001,-0.930000000000001,-0.925000000000001,-0.920000000000001,
-0.915000000000001,-0.910000000000001,-0.905000000000001,-0.900000000000001,
-0.895000000000001,-0.890000000000001,-0.885000000000001,-0.880000000000001,
-0.875000000000001,-0.870000000000001,-0.865000000000001,-0.860000000000001,
-0.855000000000001,-0.850000000000001,-0.845000000000001,-0.840000000000001,
-0.835000000000001,-0.830000000000001,-0.825000000000001,-0.820000000000001,
-0.815000000000001,-0.810000000000001,-0.805000000000001,-0.800000000000001,
-0.795000000000001,-0.790000000000001,-0.785000000000001,-0.780000000000001,
-0.775000000000001,-0.770000000000001,-0.765000000000001,-0.760000000000001,
-0.755000000000001,-0.750000000000001,-0.745000000000001,-0.740000000000001,
-0.735000000000001,-0.730000000000001,-0.725000000000001,-0.720000000000001,
-0.715000000000001,-0.710000000000001,-0.705000000000001,-0.700000000000001,
-0.695000000000001,-0.690000000000001,-0.685,-0.68,-0.675,-0.67,-0.665,
-0.66,-0.655,-0.65,-0.645,-0.64,-0.635,-0.63,-0.625,-0.62,-0.615,-0.61,
-0.605,-0.6,-0.595,-0.59,-0.585,-0.58,-0.575,-0.57,-0.565,-0.56,-0.555,
-0.55,-0.545,-0.54,-0.535,-0.53,-0.525,-0.52,-0.515,-0.51,-0.505,-0.5,-0.495,
-0.49,-0.485,-0.48,-0.475,-0.47,-0.465,-0.46,-0.455,-0.45,-0.445,-0.44,
-0.435,-0.43,-0.425,-0.42,-0.415,-0.41,-0.405,-0.4,-0.395,-0.39,-0.385,
-0.38,-0.375,-0.37,-0.365,-0.36,-0.355,-0.35,-0.345,-0.34,-0.335,-0.33,
-0.325,-0.32,-0.315,-0.31,-0.305,-0.3,-0.295,-0.29,-0.285,-0.28,-0.275,
-0.27,-0.265,-0.26,-0.255,-0.25,-0.245,-0.24,-0.235,-0.23,-0.225,-0.22,
-0.215,-0.21,-0.205,-0.2,-0.195,-0.19,-0.185,-0.18,-0.175,-0.17,-0.165,
-0.16,-0.155,-0.15,-0.145,-0.14,-0.135,-0.13,-0.125,-0.12,-0.115,-0.11,
-0.105,-0.1,-0.095,-0.09,-0.085,-0.08,-0.075,-0.07,-0.065,-0.06,-0.055,
-0.05,-0.045,-0.04,-0.035,-0.03,-0.025,-0.02,-0.015,-0.01,-0.005,0.),
 .UNSPECIFIED.)
CURVE()
GEOMETRIC_REPRESENTATION_ITEM()
RATIONAL_B_SPLINE_CURVE((1.,1.,1.,1.,1.,1.,1.,1.,1.,1.,1.,1.,1.,1.,1.,1.,
1.,1.,1.,1.,1.,1.,1.,1.,1.,1.,1.,1.,1.,1.,1.,1.,1.,1.,1.,1.,1.,1.,1.,1.,
1.,1.,1.,1.,1.,1.,1.,1.,1.,1.,1.,1.,1.,1.,1.,1.,1.,1.,1.,1.,1.,1.,1.,1.,
1.,1.,1.,1.,1.,1.,1.,1.,1.,1.,1.,1.,1.,1.,1.,1.,1.,1.,1.,1.,1.,1.,1.,1.,
1.,1.,1.,1.,1.,1.,1.,1.,1.,1.,1.,1.,1.,1.,1.,1.,1.,1.,1.,1.,1.,1.,1.,1.,
1.,1.,1.,1.,1.,1.,1.,1.,1.,1.,1.,1.,1.,1.,1.,1.,1.,1.,1.,1.,1.,1.,1.,1.,
1.,1.,1.,1.,1.,1.,1.,1.,1.,1.,1.,1.,1.,1.,1.,1.,1.,1.,1.,1.,1.,1.,1.,1.,
1.,1.,1.,1.,1.,1.,1.,1.,1.,1.,1.,1.,1.,1.,1.,1.,1.,1.,1.,1.,1.,1.,1.,1.,
1.,1.,1.,1.,1.,1.,1.,1.,1.,1.))
REPRESENTATION_ITEM('')
);
#503=(
BOUNDED_CURVE()
B_SPLINE_CURVE(5,(#97833,#97834,#97835,#97836,#97837,#97838,#97839,#97840,
#97841,#97842,#97843,#97844,#97845,#97846,#97847,#97848,#97849,#97850,#97851,
#97852,#97853,#97854,#97855,#97856,#97857,#97858,#97859,#97860,#97861,#97862,
#97863,#97864,#97865,#97866,#97867,#97868,#97869,#97870,#97871,#97872,#97873,
#97874,#97875,#97876,#97877,#97878,#97879,#97880,#97881,#97882,#97883,#97884,
#97885,#97886,#97887,#97888,#97889,#97890,#97891,#97892,#97893,#97894,#97895,
#97896,#97897,#97898,#97899,#97900,#97901,#97902,#97903,#97904,#97905,#97906,
#97907,#97908,#97909,#97910,#97911,#97912,#97913,#97914,#97915,#97916,#97917,
#97918,#97919,#97920,#97921,#97922,#97923,#97924,#97925,#97926,#97927,#97928,
#97929,#97930,#97931,#97932,#97933,#97934,#97935,#97936,#97937,#97938,#97939,
#97940,#97941,#97942,#97943,#97944,#97945,#97946,#97947,#97948,#97949,#97950,
#97951,#97952,#97953,#97954,#97955,#97956,#97957,#97958,#97959,#97960,#97961,
#97962,#97963,#97964,#97965,#97966,#97967,#97968,#97969,#97970,#97971,#97972,
#97973,#97974,#97975,#97976,#97977,#97978,#97979,#97980,#97981,#97982,#97983,
#97984,#97985,#97986,#97987,#97988,#97989,#97990,#97991,#97992,#97993,#97994,
#97995,#97996,#97997,#97998,#97999,#98000,#98001,#98002,#98003,#98004,#98005,
#98006,#98007,#98008,#98009,#98010,#98011,#98012,#98013,#98014,#98015,#98016,
#98017,#98018,#98019,#98020,#98021,#98022,#98023,#98024,#98025,#98026),
 .UNSPECIFIED.,.F.,.F.)
B_SPLINE_CURVE_WITH_KNOTS((6,1,1,1,1,1,1,1,1,1,1,1,1,1,1,1,1,1,1,1,1,1,
1,1,1,1,1,1,1,1,1,1,1,1,1,1,1,1,1,1,1,1,1,1,1,1,1,1,1,1,1,1,1,1,1,1,1,1,
1,1,1,1,1,1,1,1,1,1,1,1,1,1,1,1,1,1,1,1,1,1,1,1,1,1,1,1,1,1,1,1,1,1,1,1,
1,1,1,1,1,1,1,1,1,1,1,1,1,1,1,1,1,1,1,1,1,1,1,1,1,1,1,1,1,1,1,1,1,1,1,1,
1,1,1,1,1,1,1,1,1,1,1,1,1,1,1,1,1,1,1,1,1,1,1,1,1,1,1,1,1,1,1,1,1,1,1,1,
1,1,1,1,1,1,1,1,1,1,1,1,1,1,1,1,1,1,1,1,1,1,1,6),(0.,0.005,0.01,0.015,0.02,
0.025,0.03,0.035,0.04,0.045,0.05,0.055,0.06,0.065,0.07,0.075,0.08,0.085,
0.09,0.095,0.1,0.105,0.11,0.115,0.12,0.125,0.13,0.135,0.14,0.145,0.15,0.155,
0.16,0.165,0.17,0.175,0.18,0.185,0.19,0.195,0.2,0.205,0.21,0.215,0.22,0.225,
0.23,0.235,0.24,0.245,0.25,0.255,0.26,0.265,0.27,0.275,0.28,0.285,0.29,
0.295,0.3,0.305,0.31,0.315,0.32,0.325,0.33,0.335,0.34,0.345,0.35,0.355,
0.36,0.365,0.37,0.375,0.38,0.385,0.39,0.395,0.4,0.405,0.41,0.415,0.42,0.425,
0.43,0.435,0.44,0.445,0.45,0.455,0.46,0.465,0.47,0.475,0.48,0.485,0.49,
0.495,0.5,0.505,0.51,0.515,0.52,0.525,0.53,0.535,0.54,0.545,0.55,0.555,
0.56,0.565,0.57,0.575,0.58,0.585,0.59,0.595,0.6,0.605,0.61,0.615,0.62,0.625,
0.63,0.635,0.64,0.645,0.65,0.655,0.66,0.665,0.67,0.675,0.68,0.685,0.690000000000001,
0.695000000000001,0.700000000000001,0.705000000000001,0.710000000000001,
0.715000000000001,0.720000000000001,0.725000000000001,0.730000000000001,
0.735000000000001,0.740000000000001,0.745000000000001,0.750000000000001,
0.755000000000001,0.760000000000001,0.765000000000001,0.770000000000001,
0.775000000000001,0.780000000000001,0.785000000000001,0.790000000000001,
0.795000000000001,0.800000000000001,0.805000000000001,0.810000000000001,
0.815000000000001,0.820000000000001,0.825000000000001,0.830000000000001,
0.835000000000001,0.840000000000001,0.845000000000001,0.850000000000001,
0.855000000000001,0.860000000000001,0.865000000000001,0.870000000000001,
0.875000000000001,0.880000000000001,0.885000000000001,0.890000000000001,
0.895000000000001,0.900000000000001,0.905000000000001,0.910000000000001,
0.915000000000001,0.920000000000001,0.925000000000001,0.930000000000001,
0.935000000000001,0.940000000000001,0.941429844431384),.UNSPECIFIED.)
CURVE()
GEOMETRIC_REPRESENTATION_ITEM()
RATIONAL_B_SPLINE_CURVE((1.,1.,1.,1.,1.,1.,1.,1.,1.,1.,1.,1.,1.,1.,1.,1.,
1.,1.,1.,1.,1.,1.,1.,1.,1.,1.,1.,1.,1.,1.,1.,1.,1.,1.,1.,1.,1.,1.,1.,1.,
1.,1.,1.,1.,1.,1.,1.,1.,1.,1.,1.,1.,1.,1.,1.,1.,1.,1.,1.,1.,1.,1.,1.,1.,
1.,1.,1.,1.,1.,1.,1.,1.,1.,1.,1.,1.,1.,1.,1.,1.,1.,1.,1.,1.,1.,1.,1.,1.,
1.,1.,1.,1.,1.,1.,1.,1.,1.,1.,1.,1.,1.,1.,1.,1.,1.,1.,1.,1.,1.,1.,1.,1.,
1.,1.,1.,1.,1.,1.,1.,1.,1.,1.,1.,1.,1.,1.,1.,1.,1.,1.,1.,1.,1.,1.,1.,1.,
1.,1.,1.,1.,1.,1.,1.,1.,1.,1.,1.,1.,1.,1.,1.,1.,1.,1.,1.,1.,1.,1.,1.,1.,
1.,1.,1.,1.,1.,1.,1.,1.,1.,1.,1.,1.,1.,1.,1.,1.,1.,1.,1.,1.,1.,1.,1.,1.,
1.,1.,1.,1.,1.,1.,1.,1.,1.,1.))
REPRESENTATION_ITEM('')
);
#504=(
BOUNDED_CURVE()
B_SPLINE_CURVE(5,(#98029,#98030,#98031,#98032,#98033,#98034,#98035,#98036,
#98037,#98038,#98039,#98040,#98041,#98042,#98043,#98044,#98045,#98046,#98047,
#98048,#98049,#98050,#98051,#98052,#98053,#98054,#98055,#98056,#98057,#98058,
#98059,#98060,#98061,#98062,#98063,#98064,#98065,#98066,#98067,#98068,#98069,
#98070,#98071,#98072,#98073,#98074,#98075,#98076,#98077,#98078,#98079,#98080,
#98081,#98082,#98083,#98084,#98085,#98086,#98087,#98088,#98089,#98090,#98091,
#98092,#98093,#98094,#98095,#98096,#98097,#98098,#98099,#98100,#98101,#98102,
#98103,#98104,#98105,#98106,#98107,#98108,#98109,#98110,#98111,#98112,#98113,
#98114,#98115,#98116,#98117,#98118,#98119,#98120,#98121,#98122,#98123,#98124,
#98125,#98126,#98127,#98128,#98129,#98130,#98131,#98132,#98133,#98134,#98135,
#98136,#98137,#98138,#98139,#98140,#98141,#98142,#98143,#98144,#98145,#98146,
#98147,#98148,#98149,#98150,#98151,#98152,#98153,#98154,#98155,#98156,#98157,
#98158,#98159,#98160,#98161,#98162,#98163,#98164,#98165,#98166,#98167,#98168,
#98169,#98170,#98171,#98172,#98173,#98174,#98175,#98176,#98177,#98178,#98179,
#98180,#98181,#98182,#98183,#98184,#98185,#98186,#98187,#98188,#98189,#98190,
#98191,#98192,#98193,#98194,#98195,#98196,#98197,#98198,#98199,#98200,#98201,
#98202,#98203,#98204,#98205,#98206,#98207,#98208,#98209,#98210,#98211,#98212,
#98213,#98214,#98215,#98216,#98217,#98218,#98219,#98220,#98221,#98222),
 .UNSPECIFIED.,.F.,.F.)
B_SPLINE_CURVE_WITH_KNOTS((6,1,1,1,1,1,1,1,1,1,1,1,1,1,1,1,1,1,1,1,1,1,
1,1,1,1,1,1,1,1,1,1,1,1,1,1,1,1,1,1,1,1,1,1,1,1,1,1,1,1,1,1,1,1,1,1,1,1,
1,1,1,1,1,1,1,1,1,1,1,1,1,1,1,1,1,1,1,1,1,1,1,1,1,1,1,1,1,1,1,1,1,1,1,1,
1,1,1,1,1,1,1,1,1,1,1,1,1,1,1,1,1,1,1,1,1,1,1,1,1,1,1,1,1,1,1,1,1,1,1,1,
1,1,1,1,1,1,1,1,1,1,1,1,1,1,1,1,1,1,1,1,1,1,1,1,1,1,1,1,1,1,1,1,1,1,1,1,
1,1,1,1,1,1,1,1,1,1,1,1,1,1,1,1,1,1,1,1,1,1,1,6),(-0.941429844431385,-0.940000000000001,
-0.935000000000001,-0.930000000000001,-0.925000000000001,-0.920000000000001,
-0.915000000000001,-0.910000000000001,-0.905000000000001,-0.900000000000001,
-0.895000000000001,-0.890000000000001,-0.885000000000001,-0.880000000000001,
-0.875000000000001,-0.870000000000001,-0.865000000000001,-0.860000000000001,
-0.855000000000001,-0.850000000000001,-0.845000000000001,-0.840000000000001,
-0.835000000000001,-0.830000000000001,-0.825000000000001,-0.820000000000001,
-0.815000000000001,-0.810000000000001,-0.805000000000001,-0.800000000000001,
-0.795000000000001,-0.790000000000001,-0.785000000000001,-0.780000000000001,
-0.775000000000001,-0.770000000000001,-0.765000000000001,-0.760000000000001,
-0.755000000000001,-0.750000000000001,-0.745000000000001,-0.740000000000001,
-0.735000000000001,-0.730000000000001,-0.725000000000001,-0.720000000000001,
-0.715000000000001,-0.710000000000001,-0.705000000000001,-0.700000000000001,
-0.695000000000001,-0.690000000000001,-0.685,-0.68,-0.675,-0.67,-0.665,
-0.66,-0.655,-0.65,-0.645,-0.64,-0.635,-0.63,-0.625,-0.62,-0.615,-0.61,
-0.605,-0.6,-0.595,-0.59,-0.585,-0.58,-0.575,-0.57,-0.565,-0.56,-0.555,
-0.55,-0.545,-0.54,-0.535,-0.53,-0.525,-0.52,-0.515,-0.51,-0.505,-0.5,-0.495,
-0.49,-0.485,-0.48,-0.475,-0.47,-0.465,-0.46,-0.455,-0.45,-0.445,-0.44,
-0.435,-0.43,-0.425,-0.42,-0.415,-0.41,-0.405,-0.4,-0.395,-0.39,-0.385,
-0.38,-0.375,-0.37,-0.365,-0.36,-0.355,-0.35,-0.345,-0.34,-0.335,-0.33,
-0.325,-0.32,-0.315,-0.31,-0.305,-0.3,-0.295,-0.29,-0.285,-0.28,-0.275,
-0.27,-0.265,-0.26,-0.255,-0.25,-0.245,-0.24,-0.235,-0.23,-0.225,-0.22,
-0.215,-0.21,-0.205,-0.2,-0.195,-0.19,-0.185,-0.18,-0.175,-0.17,-0.165,
-0.16,-0.155,-0.15,-0.145,-0.14,-0.135,-0.13,-0.125,-0.12,-0.115,-0.11,
-0.105,-0.1,-0.095,-0.09,-0.085,-0.08,-0.075,-0.07,-0.065,-0.06,-0.055,
-0.05,-0.045,-0.04,-0.035,-0.03,-0.025,-0.02,-0.015,-0.01,-0.005,0.),
 .UNSPECIFIED.)
CURVE()
GEOMETRIC_REPRESENTATION_ITEM()
RATIONAL_B_SPLINE_CURVE((1.,1.,1.,1.,1.,1.,1.,1.,1.,1.,1.,1.,1.,1.,1.,1.,
1.,1.,1.,1.,1.,1.,1.,1.,1.,1.,1.,1.,1.,1.,1.,1.,1.,1.,1.,1.,1.,1.,1.,1.,
1.,1.,1.,1.,1.,1.,1.,1.,1.,1.,1.,1.,1.,1.,1.,1.,1.,1.,1.,1.,1.,1.,1.,1.,
1.,1.,1.,1.,1.,1.,1.,1.,1.,1.,1.,1.,1.,1.,1.,1.,1.,1.,1.,1.,1.,1.,1.,1.,
1.,1.,1.,1.,1.,1.,1.,1.,1.,1.,1.,1.,1.,1.,1.,1.,1.,1.,1.,1.,1.,1.,1.,1.,
1.,1.,1.,1.,1.,1.,1.,1.,1.,1.,1.,1.,1.,1.,1.,1.,1.,1.,1.,1.,1.,1.,1.,1.,
1.,1.,1.,1.,1.,1.,1.,1.,1.,1.,1.,1.,1.,1.,1.,1.,1.,1.,1.,1.,1.,1.,1.,1.,
1.,1.,1.,1.,1.,1.,1.,1.,1.,1.,1.,1.,1.,1.,1.,1.,1.,1.,1.,1.,1.,1.,1.,1.,
1.,1.,1.,1.,1.,1.,1.,1.,1.,1.))
REPRESENTATION_ITEM('')
);
#505=(
BOUNDED_CURVE()
B_SPLINE_CURVE(5,(#98729,#98730,#98731,#98732,#98733,#98734,#98735,#98736,
#98737,#98738,#98739,#98740,#98741,#98742,#98743,#98744,#98745,#98746,#98747,
#98748,#98749,#98750,#98751,#98752,#98753,#98754,#98755,#98756,#98757,#98758,
#98759,#98760,#98761,#98762,#98763,#98764,#98765,#98766,#98767,#98768,#98769,
#98770,#98771,#98772,#98773,#98774,#98775,#98776,#98777,#98778,#98779,#98780,
#98781,#98782,#98783,#98784,#98785,#98786,#98787,#98788,#98789,#98790,#98791,
#98792,#98793,#98794,#98795,#98796,#98797,#98798,#98799,#98800,#98801,#98802,
#98803,#98804,#98805,#98806,#98807,#98808,#98809,#98810,#98811,#98812,#98813,
#98814,#98815,#98816,#98817,#98818,#98819,#98820,#98821,#98822,#98823,#98824,
#98825,#98826,#98827,#98828,#98829,#98830,#98831,#98832,#98833,#98834,#98835,
#98836,#98837,#98838,#98839,#98840,#98841,#98842,#98843,#98844,#98845,#98846,
#98847,#98848,#98849,#98850,#98851,#98852,#98853,#98854,#98855,#98856,#98857,
#98858,#98859,#98860,#98861,#98862,#98863,#98864,#98865,#98866,#98867,#98868,
#98869,#98870,#98871,#98872,#98873,#98874,#98875,#98876,#98877,#98878,#98879,
#98880,#98881,#98882,#98883,#98884,#98885,#98886,#98887,#98888,#98889,#98890,
#98891,#98892,#98893,#98894,#98895,#98896,#98897,#98898,#98899,#98900,#98901,
#98902,#98903,#98904,#98905,#98906,#98907,#98908,#98909,#98910,#98911,#98912,
#98913,#98914,#98915,#98916,#98917,#98918,#98919,#98920,#98921,#98922),
 .UNSPECIFIED.,.F.,.F.)
B_SPLINE_CURVE_WITH_KNOTS((6,1,1,1,1,1,1,1,1,1,1,1,1,1,1,1,1,1,1,1,1,1,
1,1,1,1,1,1,1,1,1,1,1,1,1,1,1,1,1,1,1,1,1,1,1,1,1,1,1,1,1,1,1,1,1,1,1,1,
1,1,1,1,1,1,1,1,1,1,1,1,1,1,1,1,1,1,1,1,1,1,1,1,1,1,1,1,1,1,1,1,1,1,1,1,
1,1,1,1,1,1,1,1,1,1,1,1,1,1,1,1,1,1,1,1,1,1,1,1,1,1,1,1,1,1,1,1,1,1,1,1,
1,1,1,1,1,1,1,1,1,1,1,1,1,1,1,1,1,1,1,1,1,1,1,1,1,1,1,1,1,1,1,1,1,1,1,1,
1,1,1,1,1,1,1,1,1,1,1,1,1,1,1,1,1,1,1,1,1,1,1,6),(0.,0.005,0.01,0.015,0.02,
0.025,0.03,0.035,0.04,0.045,0.05,0.055,0.06,0.065,0.07,0.075,0.08,0.085,
0.09,0.095,0.1,0.105,0.11,0.115,0.12,0.125,0.13,0.135,0.14,0.145,0.15,0.155,
0.16,0.165,0.17,0.175,0.18,0.185,0.19,0.195,0.2,0.205,0.21,0.215,0.22,0.225,
0.23,0.235,0.24,0.245,0.25,0.255,0.26,0.265,0.27,0.275,0.28,0.285,0.29,
0.295,0.3,0.305,0.31,0.315,0.32,0.325,0.33,0.335,0.34,0.345,0.35,0.355,
0.36,0.365,0.37,0.375,0.38,0.385,0.39,0.395,0.4,0.405,0.41,0.415,0.42,0.425,
0.43,0.435,0.44,0.445,0.45,0.455,0.46,0.465,0.47,0.475,0.48,0.485,0.49,
0.495,0.5,0.505,0.51,0.515,0.52,0.525,0.53,0.535,0.54,0.545,0.55,0.555,
0.56,0.565,0.57,0.575,0.58,0.585,0.59,0.595,0.6,0.605,0.61,0.615,0.62,0.625,
0.63,0.635,0.64,0.645,0.65,0.655,0.66,0.665,0.67,0.675,0.68,0.685,0.690000000000001,
0.695000000000001,0.700000000000001,0.705000000000001,0.710000000000001,
0.715000000000001,0.720000000000001,0.725000000000001,0.730000000000001,
0.735000000000001,0.740000000000001,0.745000000000001,0.750000000000001,
0.755000000000001,0.760000000000001,0.765000000000001,0.770000000000001,
0.775000000000001,0.780000000000001,0.785000000000001,0.790000000000001,
0.795000000000001,0.800000000000001,0.805000000000001,0.810000000000001,
0.815000000000001,0.820000000000001,0.825000000000001,0.830000000000001,
0.835000000000001,0.840000000000001,0.845000000000001,0.850000000000001,
0.855000000000001,0.860000000000001,0.865000000000001,0.870000000000001,
0.875000000000001,0.880000000000001,0.885000000000001,0.890000000000001,
0.895000000000001,0.900000000000001,0.905000000000001,0.910000000000001,
0.915000000000001,0.920000000000001,0.925000000000001,0.930000000000001,
0.935000000000001,0.940000000000001,0.941429844431381),.UNSPECIFIED.)
CURVE()
GEOMETRIC_REPRESENTATION_ITEM()
RATIONAL_B_SPLINE_CURVE((1.,1.,1.,1.,1.,1.,1.,1.,1.,1.,1.,1.,1.,1.,1.,1.,
1.,1.,1.,1.,1.,1.,1.,1.,1.,1.,1.,1.,1.,1.,1.,1.,1.,1.,1.,1.,1.,1.,1.,1.,
1.,1.,1.,1.,1.,1.,1.,1.,1.,1.,1.,1.,1.,1.,1.,1.,1.,1.,1.,1.,1.,1.,1.,1.,
1.,1.,1.,1.,1.,1.,1.,1.,1.,1.,1.,1.,1.,1.,1.,1.,1.,1.,1.,1.,1.,1.,1.,1.,
1.,1.,1.,1.,1.,1.,1.,1.,1.,1.,1.,1.,1.,1.,1.,1.,1.,1.,1.,1.,1.,1.,1.,1.,
1.,1.,1.,1.,1.,1.,1.,1.,1.,1.,1.,1.,1.,1.,1.,1.,1.,1.,1.,1.,1.,1.,1.,1.,
1.,1.,1.,1.,1.,1.,1.,1.,1.,1.,1.,1.,1.,1.,1.,1.,1.,1.,1.,1.,1.,1.,1.,1.,
1.,1.,1.,1.,1.,1.,1.,1.,1.,1.,1.,1.,1.,1.,1.,1.,1.,1.,1.,1.,1.,1.,1.,1.,
1.,1.,1.,1.,1.,1.,1.,1.,1.,1.))
REPRESENTATION_ITEM('')
);
#506=(
BOUNDED_CURVE()
B_SPLINE_CURVE(5,(#98925,#98926,#98927,#98928,#98929,#98930,#98931,#98932,
#98933,#98934,#98935,#98936,#98937,#98938,#98939,#98940,#98941,#98942,#98943,
#98944,#98945,#98946,#98947,#98948,#98949,#98950,#98951,#98952,#98953,#98954,
#98955,#98956,#98957,#98958,#98959,#98960,#98961,#98962,#98963,#98964,#98965,
#98966,#98967,#98968,#98969,#98970,#98971,#98972,#98973,#98974,#98975,#98976,
#98977,#98978,#98979,#98980,#98981,#98982,#98983,#98984,#98985,#98986,#98987,
#98988,#98989,#98990,#98991,#98992,#98993,#98994,#98995,#98996,#98997,#98998,
#98999,#99000,#99001,#99002,#99003,#99004,#99005,#99006,#99007,#99008,#99009,
#99010,#99011,#99012,#99013,#99014,#99015,#99016,#99017,#99018,#99019,#99020,
#99021,#99022,#99023,#99024,#99025,#99026,#99027,#99028,#99029,#99030,#99031,
#99032,#99033,#99034,#99035,#99036,#99037,#99038,#99039,#99040,#99041,#99042,
#99043,#99044,#99045,#99046,#99047,#99048,#99049,#99050,#99051,#99052,#99053,
#99054,#99055,#99056,#99057,#99058,#99059,#99060,#99061,#99062,#99063,#99064,
#99065,#99066,#99067,#99068,#99069,#99070,#99071,#99072,#99073,#99074,#99075,
#99076,#99077,#99078,#99079,#99080,#99081,#99082,#99083,#99084,#99085,#99086,
#99087,#99088,#99089,#99090,#99091,#99092,#99093,#99094,#99095,#99096,#99097,
#99098,#99099,#99100,#99101,#99102,#99103,#99104,#99105,#99106,#99107,#99108,
#99109,#99110,#99111,#99112,#99113,#99114,#99115,#99116,#99117,#99118),
 .UNSPECIFIED.,.F.,.F.)
B_SPLINE_CURVE_WITH_KNOTS((6,1,1,1,1,1,1,1,1,1,1,1,1,1,1,1,1,1,1,1,1,1,
1,1,1,1,1,1,1,1,1,1,1,1,1,1,1,1,1,1,1,1,1,1,1,1,1,1,1,1,1,1,1,1,1,1,1,1,
1,1,1,1,1,1,1,1,1,1,1,1,1,1,1,1,1,1,1,1,1,1,1,1,1,1,1,1,1,1,1,1,1,1,1,1,
1,1,1,1,1,1,1,1,1,1,1,1,1,1,1,1,1,1,1,1,1,1,1,1,1,1,1,1,1,1,1,1,1,1,1,1,
1,1,1,1,1,1,1,1,1,1,1,1,1,1,1,1,1,1,1,1,1,1,1,1,1,1,1,1,1,1,1,1,1,1,1,1,
1,1,1,1,1,1,1,1,1,1,1,1,1,1,1,1,1,1,1,1,1,1,1,6),(-0.941429844431409,-0.940000000000001,
-0.935000000000001,-0.930000000000001,-0.925000000000001,-0.920000000000001,
-0.915000000000001,-0.910000000000001,-0.905000000000001,-0.900000000000001,
-0.895000000000001,-0.890000000000001,-0.885000000000001,-0.880000000000001,
-0.875000000000001,-0.870000000000001,-0.865000000000001,-0.860000000000001,
-0.855000000000001,-0.850000000000001,-0.845000000000001,-0.840000000000001,
-0.835000000000001,-0.830000000000001,-0.825000000000001,-0.820000000000001,
-0.815000000000001,-0.810000000000001,-0.805000000000001,-0.800000000000001,
-0.795000000000001,-0.790000000000001,-0.785000000000001,-0.780000000000001,
-0.775000000000001,-0.770000000000001,-0.765000000000001,-0.760000000000001,
-0.755000000000001,-0.750000000000001,-0.745000000000001,-0.740000000000001,
-0.735000000000001,-0.730000000000001,-0.725000000000001,-0.720000000000001,
-0.715000000000001,-0.710000000000001,-0.705000000000001,-0.700000000000001,
-0.695000000000001,-0.690000000000001,-0.685,-0.68,-0.675,-0.67,-0.665,
-0.66,-0.655,-0.65,-0.645,-0.64,-0.635,-0.63,-0.625,-0.62,-0.615,-0.61,
-0.605,-0.6,-0.595,-0.59,-0.585,-0.58,-0.575,-0.57,-0.565,-0.56,-0.555,
-0.55,-0.545,-0.54,-0.535,-0.53,-0.525,-0.52,-0.515,-0.51,-0.505,-0.5,-0.495,
-0.49,-0.485,-0.48,-0.475,-0.47,-0.465,-0.46,-0.455,-0.45,-0.445,-0.44,
-0.435,-0.43,-0.425,-0.42,-0.415,-0.41,-0.405,-0.4,-0.395,-0.39,-0.385,
-0.38,-0.375,-0.37,-0.365,-0.36,-0.355,-0.35,-0.345,-0.34,-0.335,-0.33,
-0.325,-0.32,-0.315,-0.31,-0.305,-0.3,-0.295,-0.29,-0.285,-0.28,-0.275,
-0.27,-0.265,-0.26,-0.255,-0.25,-0.245,-0.24,-0.235,-0.23,-0.225,-0.22,
-0.215,-0.21,-0.205,-0.2,-0.195,-0.19,-0.185,-0.18,-0.175,-0.17,-0.165,
-0.16,-0.155,-0.15,-0.145,-0.14,-0.135,-0.13,-0.125,-0.12,-0.115,-0.11,
-0.105,-0.1,-0.095,-0.09,-0.085,-0.08,-0.075,-0.07,-0.065,-0.06,-0.055,
-0.05,-0.045,-0.04,-0.035,-0.03,-0.025,-0.02,-0.015,-0.01,-0.005,0.),
 .UNSPECIFIED.)
CURVE()
GEOMETRIC_REPRESENTATION_ITEM()
RATIONAL_B_SPLINE_CURVE((1.,1.,1.,1.,1.,1.,1.,1.,1.,1.,1.,1.,1.,1.,1.,1.,
1.,1.,1.,1.,1.,1.,1.,1.,1.,1.,1.,1.,1.,1.,1.,1.,1.,1.,1.,1.,1.,1.,1.,1.,
1.,1.,1.,1.,1.,1.,1.,1.,1.,1.,1.,1.,1.,1.,1.,1.,1.,1.,1.,1.,1.,1.,1.,1.,
1.,1.,1.,1.,1.,1.,1.,1.,1.,1.,1.,1.,1.,1.,1.,1.,1.,1.,1.,1.,1.,1.,1.,1.,
1.,1.,1.,1.,1.,1.,1.,1.,1.,1.,1.,1.,1.,1.,1.,1.,1.,1.,1.,1.,1.,1.,1.,1.,
1.,1.,1.,1.,1.,1.,1.,1.,1.,1.,1.,1.,1.,1.,1.,1.,1.,1.,1.,1.,1.,1.,1.,1.,
1.,1.,1.,1.,1.,1.,1.,1.,1.,1.,1.,1.,1.,1.,1.,1.,1.,1.,1.,1.,1.,1.,1.,1.,
1.,1.,1.,1.,1.,1.,1.,1.,1.,1.,1.,1.,1.,1.,1.,1.,1.,1.,1.,1.,1.,1.,1.,1.,
1.,1.,1.,1.,1.,1.,1.,1.,1.,1.))
REPRESENTATION_ITEM('')
);
#507=(
BOUNDED_CURVE()
B_SPLINE_CURVE(5,(#99625,#99626,#99627,#99628,#99629,#99630,#99631,#99632,
#99633,#99634,#99635,#99636,#99637,#99638,#99639,#99640,#99641,#99642,#99643,
#99644,#99645,#99646,#99647,#99648,#99649,#99650,#99651,#99652,#99653,#99654,
#99655,#99656,#99657,#99658,#99659,#99660,#99661,#99662,#99663,#99664,#99665,
#99666,#99667,#99668,#99669,#99670,#99671,#99672,#99673,#99674,#99675,#99676,
#99677,#99678,#99679,#99680,#99681,#99682,#99683,#99684,#99685,#99686,#99687,
#99688,#99689,#99690,#99691,#99692,#99693,#99694,#99695,#99696,#99697,#99698,
#99699,#99700,#99701,#99702,#99703,#99704,#99705,#99706,#99707,#99708,#99709,
#99710,#99711,#99712,#99713,#99714,#99715,#99716,#99717,#99718,#99719,#99720,
#99721,#99722,#99723,#99724,#99725,#99726,#99727,#99728,#99729,#99730,#99731,
#99732,#99733,#99734,#99735,#99736,#99737,#99738,#99739,#99740,#99741,#99742,
#99743,#99744,#99745,#99746,#99747,#99748,#99749,#99750,#99751,#99752,#99753,
#99754,#99755,#99756,#99757,#99758,#99759,#99760,#99761,#99762,#99763,#99764,
#99765,#99766,#99767,#99768,#99769,#99770,#99771,#99772,#99773,#99774,#99775,
#99776,#99777,#99778,#99779,#99780,#99781,#99782,#99783,#99784,#99785,#99786,
#99787,#99788,#99789,#99790,#99791,#99792,#99793,#99794,#99795,#99796,#99797,
#99798,#99799,#99800,#99801,#99802,#99803,#99804,#99805,#99806,#99807,#99808,
#99809,#99810,#99811,#99812,#99813,#99814,#99815,#99816,#99817,#99818),
 .UNSPECIFIED.,.F.,.F.)
B_SPLINE_CURVE_WITH_KNOTS((6,1,1,1,1,1,1,1,1,1,1,1,1,1,1,1,1,1,1,1,1,1,
1,1,1,1,1,1,1,1,1,1,1,1,1,1,1,1,1,1,1,1,1,1,1,1,1,1,1,1,1,1,1,1,1,1,1,1,
1,1,1,1,1,1,1,1,1,1,1,1,1,1,1,1,1,1,1,1,1,1,1,1,1,1,1,1,1,1,1,1,1,1,1,1,
1,1,1,1,1,1,1,1,1,1,1,1,1,1,1,1,1,1,1,1,1,1,1,1,1,1,1,1,1,1,1,1,1,1,1,1,
1,1,1,1,1,1,1,1,1,1,1,1,1,1,1,1,1,1,1,1,1,1,1,1,1,1,1,1,1,1,1,1,1,1,1,1,
1,1,1,1,1,1,1,1,1,1,1,1,1,1,1,1,1,1,1,1,1,1,1,6),(0.,0.005,0.01,0.015,0.02,
0.025,0.03,0.035,0.04,0.045,0.05,0.055,0.06,0.065,0.07,0.075,0.08,0.085,
0.09,0.095,0.1,0.105,0.11,0.115,0.12,0.125,0.13,0.135,0.14,0.145,0.15,0.155,
0.16,0.165,0.17,0.175,0.18,0.185,0.19,0.195,0.2,0.205,0.21,0.215,0.22,0.225,
0.23,0.235,0.24,0.245,0.25,0.255,0.26,0.265,0.27,0.275,0.28,0.285,0.29,
0.295,0.3,0.305,0.31,0.315,0.32,0.325,0.33,0.335,0.34,0.345,0.35,0.355,
0.36,0.365,0.37,0.375,0.38,0.385,0.39,0.395,0.4,0.405,0.41,0.415,0.42,0.425,
0.43,0.435,0.44,0.445,0.45,0.455,0.46,0.465,0.47,0.475,0.48,0.485,0.49,
0.495,0.5,0.505,0.51,0.515,0.52,0.525,0.53,0.535,0.54,0.545,0.55,0.555,
0.56,0.565,0.57,0.575,0.58,0.585,0.59,0.595,0.6,0.605,0.61,0.615,0.62,0.625,
0.63,0.635,0.64,0.645,0.65,0.655,0.66,0.665,0.67,0.675,0.68,0.685,0.690000000000001,
0.695000000000001,0.700000000000001,0.705000000000001,0.710000000000001,
0.715000000000001,0.720000000000001,0.725000000000001,0.730000000000001,
0.735000000000001,0.740000000000001,0.745000000000001,0.750000000000001,
0.755000000000001,0.760000000000001,0.765000000000001,0.770000000000001,
0.775000000000001,0.780000000000001,0.785000000000001,0.790000000000001,
0.795000000000001,0.800000000000001,0.805000000000001,0.810000000000001,
0.815000000000001,0.820000000000001,0.825000000000001,0.830000000000001,
0.835000000000001,0.840000000000001,0.845000000000001,0.850000000000001,
0.855000000000001,0.860000000000001,0.865000000000001,0.870000000000001,
0.875000000000001,0.880000000000001,0.885000000000001,0.890000000000001,
0.895000000000001,0.900000000000001,0.905000000000001,0.910000000000001,
0.915000000000001,0.920000000000001,0.925000000000001,0.930000000000001,
0.935000000000001,0.940000000000001,0.941429844431327),.UNSPECIFIED.)
CURVE()
GEOMETRIC_REPRESENTATION_ITEM()
RATIONAL_B_SPLINE_CURVE((1.,1.,1.,1.,1.,1.,1.,1.,1.,1.,1.,1.,1.,1.,1.,1.,
1.,1.,1.,1.,1.,1.,1.,1.,1.,1.,1.,1.,1.,1.,1.,1.,1.,1.,1.,1.,1.,1.,1.,1.,
1.,1.,1.,1.,1.,1.,1.,1.,1.,1.,1.,1.,1.,1.,1.,1.,1.,1.,1.,1.,1.,1.,1.,1.,
1.,1.,1.,1.,1.,1.,1.,1.,1.,1.,1.,1.,1.,1.,1.,1.,1.,1.,1.,1.,1.,1.,1.,1.,
1.,1.,1.,1.,1.,1.,1.,1.,1.,1.,1.,1.,1.,1.,1.,1.,1.,1.,1.,1.,1.,1.,1.,1.,
1.,1.,1.,1.,1.,1.,1.,1.,1.,1.,1.,1.,1.,1.,1.,1.,1.,1.,1.,1.,1.,1.,1.,1.,
1.,1.,1.,1.,1.,1.,1.,1.,1.,1.,1.,1.,1.,1.,1.,1.,1.,1.,1.,1.,1.,1.,1.,1.,
1.,1.,1.,1.,1.,1.,1.,1.,1.,1.,1.,1.,1.,1.,1.,1.,1.,1.,1.,1.,1.,1.,1.,1.,
1.,1.,1.,1.,1.,1.,1.,1.,1.,1.))
REPRESENTATION_ITEM('')
);
#508=(
BOUNDED_CURVE()
B_SPLINE_CURVE(5,(#99821,#99822,#99823,#99824,#99825,#99826,#99827,#99828,
#99829,#99830,#99831,#99832,#99833,#99834,#99835,#99836,#99837,#99838,#99839,
#99840,#99841,#99842,#99843,#99844,#99845,#99846,#99847,#99848,#99849,#99850,
#99851,#99852,#99853,#99854,#99855,#99856,#99857,#99858,#99859,#99860,#99861,
#99862,#99863,#99864,#99865,#99866,#99867,#99868,#99869,#99870,#99871,#99872,
#99873,#99874,#99875,#99876,#99877,#99878,#99879,#99880,#99881,#99882,#99883,
#99884,#99885,#99886,#99887,#99888,#99889,#99890,#99891,#99892,#99893,#99894,
#99895,#99896,#99897,#99898,#99899,#99900,#99901,#99902,#99903,#99904,#99905,
#99906,#99907,#99908,#99909,#99910,#99911,#99912,#99913,#99914,#99915,#99916,
#99917,#99918,#99919,#99920,#99921,#99922,#99923,#99924,#99925,#99926,#99927,
#99928,#99929,#99930,#99931,#99932,#99933,#99934,#99935,#99936,#99937,#99938,
#99939,#99940,#99941,#99942,#99943,#99944,#99945,#99946,#99947,#99948,#99949,
#99950,#99951,#99952,#99953,#99954,#99955,#99956,#99957,#99958,#99959,#99960,
#99961,#99962,#99963,#99964,#99965,#99966,#99967,#99968,#99969,#99970,#99971,
#99972,#99973,#99974,#99975,#99976,#99977,#99978,#99979,#99980,#99981,#99982,
#99983,#99984,#99985,#99986,#99987,#99988,#99989,#99990,#99991,#99992,#99993,
#99994,#99995,#99996,#99997,#99998,#99999,#100000,#100001,#100002,#100003,
#100004,#100005,#100006,#100007,#100008,#100009,#100010,#100011,#100012,
#100013,#100014),.UNSPECIFIED.,.F.,.F.)
B_SPLINE_CURVE_WITH_KNOTS((6,1,1,1,1,1,1,1,1,1,1,1,1,1,1,1,1,1,1,1,1,1,
1,1,1,1,1,1,1,1,1,1,1,1,1,1,1,1,1,1,1,1,1,1,1,1,1,1,1,1,1,1,1,1,1,1,1,1,
1,1,1,1,1,1,1,1,1,1,1,1,1,1,1,1,1,1,1,1,1,1,1,1,1,1,1,1,1,1,1,1,1,1,1,1,
1,1,1,1,1,1,1,1,1,1,1,1,1,1,1,1,1,1,1,1,1,1,1,1,1,1,1,1,1,1,1,1,1,1,1,1,
1,1,1,1,1,1,1,1,1,1,1,1,1,1,1,1,1,1,1,1,1,1,1,1,1,1,1,1,1,1,1,1,1,1,1,1,
1,1,1,1,1,1,1,1,1,1,1,1,1,1,1,1,1,1,1,1,1,1,1,6),(-0.941429844431327,-0.940000000000001,
-0.935000000000001,-0.930000000000001,-0.925000000000001,-0.920000000000001,
-0.915000000000001,-0.910000000000001,-0.905000000000001,-0.900000000000001,
-0.895000000000001,-0.890000000000001,-0.885000000000001,-0.880000000000001,
-0.875000000000001,-0.870000000000001,-0.865000000000001,-0.860000000000001,
-0.855000000000001,-0.850000000000001,-0.845000000000001,-0.840000000000001,
-0.835000000000001,-0.830000000000001,-0.825000000000001,-0.820000000000001,
-0.815000000000001,-0.810000000000001,-0.805000000000001,-0.800000000000001,
-0.795000000000001,-0.790000000000001,-0.785000000000001,-0.780000000000001,
-0.775000000000001,-0.770000000000001,-0.765000000000001,-0.760000000000001,
-0.755000000000001,-0.750000000000001,-0.745000000000001,-0.740000000000001,
-0.735000000000001,-0.730000000000001,-0.725000000000001,-0.720000000000001,
-0.715000000000001,-0.710000000000001,-0.705000000000001,-0.700000000000001,
-0.695000000000001,-0.690000000000001,-0.685,-0.68,-0.675,-0.67,-0.665,
-0.66,-0.655,-0.65,-0.645,-0.64,-0.635,-0.63,-0.625,-0.62,-0.615,-0.61,
-0.605,-0.6,-0.595,-0.59,-0.585,-0.58,-0.575,-0.57,-0.565,-0.56,-0.555,
-0.55,-0.545,-0.54,-0.535,-0.53,-0.525,-0.52,-0.515,-0.51,-0.505,-0.5,-0.495,
-0.49,-0.485,-0.48,-0.475,-0.47,-0.465,-0.46,-0.455,-0.45,-0.445,-0.44,
-0.435,-0.43,-0.425,-0.42,-0.415,-0.41,-0.405,-0.4,-0.395,-0.39,-0.385,
-0.38,-0.375,-0.37,-0.365,-0.36,-0.355,-0.35,-0.345,-0.34,-0.335,-0.33,
-0.325,-0.32,-0.315,-0.31,-0.305,-0.3,-0.295,-0.29,-0.285,-0.28,-0.275,
-0.27,-0.265,-0.26,-0.255,-0.25,-0.245,-0.24,-0.235,-0.23,-0.225,-0.22,
-0.215,-0.21,-0.205,-0.2,-0.195,-0.19,-0.185,-0.18,-0.175,-0.17,-0.165,
-0.16,-0.155,-0.15,-0.145,-0.14,-0.135,-0.13,-0.125,-0.12,-0.115,-0.11,
-0.105,-0.1,-0.095,-0.09,-0.085,-0.08,-0.075,-0.07,-0.065,-0.06,-0.055,
-0.05,-0.045,-0.04,-0.035,-0.03,-0.025,-0.02,-0.015,-0.01,-0.005,0.),
 .UNSPECIFIED.)
CURVE()
GEOMETRIC_REPRESENTATION_ITEM()
RATIONAL_B_SPLINE_CURVE((1.,1.,1.,1.,1.,1.,1.,1.,1.,1.,1.,1.,1.,1.,1.,1.,
1.,1.,1.,1.,1.,1.,1.,1.,1.,1.,1.,1.,1.,1.,1.,1.,1.,1.,1.,1.,1.,1.,1.,1.,
1.,1.,1.,1.,1.,1.,1.,1.,1.,1.,1.,1.,1.,1.,1.,1.,1.,1.,1.,1.,1.,1.,1.,1.,
1.,1.,1.,1.,1.,1.,1.,1.,1.,1.,1.,1.,1.,1.,1.,1.,1.,1.,1.,1.,1.,1.,1.,1.,
1.,1.,1.,1.,1.,1.,1.,1.,1.,1.,1.,1.,1.,1.,1.,1.,1.,1.,1.,1.,1.,1.,1.,1.,
1.,1.,1.,1.,1.,1.,1.,1.,1.,1.,1.,1.,1.,1.,1.,1.,1.,1.,1.,1.,1.,1.,1.,1.,
1.,1.,1.,1.,1.,1.,1.,1.,1.,1.,1.,1.,1.,1.,1.,1.,1.,1.,1.,1.,1.,1.,1.,1.,
1.,1.,1.,1.,1.,1.,1.,1.,1.,1.,1.,1.,1.,1.,1.,1.,1.,1.,1.,1.,1.,1.,1.,1.,
1.,1.,1.,1.,1.,1.,1.,1.,1.,1.))
REPRESENTATION_ITEM('')
);
#509=(
BOUNDED_CURVE()
B_SPLINE_CURVE(5,(#100521,#100522,#100523,#100524,#100525,#100526,#100527,
#100528,#100529,#100530,#100531,#100532,#100533,#100534,#100535,#100536,
#100537,#100538,#100539,#100540,#100541,#100542,#100543,#100544,#100545,
#100546,#100547,#100548,#100549,#100550,#100551,#100552,#100553,#100554,
#100555,#100556,#100557,#100558,#100559,#100560,#100561,#100562,#100563,
#100564,#100565,#100566,#100567,#100568,#100569,#100570,#100571,#100572,
#100573,#100574,#100575,#100576,#100577,#100578,#100579,#100580,#100581,
#100582,#100583,#100584,#100585,#100586,#100587,#100588,#100589,#100590,
#100591,#100592,#100593,#100594,#100595,#100596,#100597,#100598,#100599,
#100600,#100601,#100602,#100603,#100604,#100605,#100606,#100607,#100608,
#100609,#100610,#100611,#100612,#100613,#100614,#100615,#100616,#100617,
#100618,#100619,#100620,#100621,#100622,#100623,#100624,#100625,#100626,
#100627,#100628,#100629,#100630,#100631,#100632,#100633,#100634,#100635,
#100636,#100637,#100638,#100639,#100640,#100641,#100642,#100643,#100644,
#100645,#100646,#100647,#100648,#100649,#100650,#100651,#100652,#100653,
#100654,#100655,#100656,#100657,#100658,#100659,#100660,#100661,#100662,
#100663,#100664,#100665,#100666,#100667,#100668,#100669,#100670,#100671,
#100672,#100673,#100674,#100675,#100676,#100677,#100678,#100679,#100680,
#100681,#100682,#100683,#100684,#100685,#100686,#100687,#100688,#100689,
#100690,#100691,#100692,#100693,#100694,#100695,#100696,#100697,#100698,
#100699,#100700,#100701,#100702,#100703,#100704,#100705,#100706,#100707,
#100708,#100709,#100710,#100711,#100712,#100713,#100714),.UNSPECIFIED.,
 .F.,.F.)
B_SPLINE_CURVE_WITH_KNOTS((6,1,1,1,1,1,1,1,1,1,1,1,1,1,1,1,1,1,1,1,1,1,
1,1,1,1,1,1,1,1,1,1,1,1,1,1,1,1,1,1,1,1,1,1,1,1,1,1,1,1,1,1,1,1,1,1,1,1,
1,1,1,1,1,1,1,1,1,1,1,1,1,1,1,1,1,1,1,1,1,1,1,1,1,1,1,1,1,1,1,1,1,1,1,1,
1,1,1,1,1,1,1,1,1,1,1,1,1,1,1,1,1,1,1,1,1,1,1,1,1,1,1,1,1,1,1,1,1,1,1,1,
1,1,1,1,1,1,1,1,1,1,1,1,1,1,1,1,1,1,1,1,1,1,1,1,1,1,1,1,1,1,1,1,1,1,1,1,
1,1,1,1,1,1,1,1,1,1,1,1,1,1,1,1,1,1,1,1,1,1,1,6),(0.,0.005,0.01,0.015,0.02,
0.025,0.03,0.035,0.04,0.045,0.05,0.055,0.06,0.065,0.07,0.075,0.08,0.085,
0.09,0.095,0.1,0.105,0.11,0.115,0.12,0.125,0.13,0.135,0.14,0.145,0.15,0.155,
0.16,0.165,0.17,0.175,0.18,0.185,0.19,0.195,0.2,0.205,0.21,0.215,0.22,0.225,
0.23,0.235,0.24,0.245,0.25,0.255,0.26,0.265,0.27,0.275,0.28,0.285,0.29,
0.295,0.3,0.305,0.31,0.315,0.32,0.325,0.33,0.335,0.34,0.345,0.35,0.355,
0.36,0.365,0.37,0.375,0.38,0.385,0.39,0.395,0.4,0.405,0.41,0.415,0.42,0.425,
0.43,0.435,0.44,0.445,0.45,0.455,0.46,0.465,0.47,0.475,0.48,0.485,0.49,
0.495,0.5,0.505,0.51,0.515,0.52,0.525,0.53,0.535,0.54,0.545,0.55,0.555,
0.56,0.565,0.57,0.575,0.58,0.585,0.59,0.595,0.6,0.605,0.61,0.615,0.62,0.625,
0.63,0.635,0.64,0.645,0.65,0.655,0.66,0.665,0.67,0.675,0.68,0.685,0.690000000000001,
0.695000000000001,0.700000000000001,0.705000000000001,0.710000000000001,
0.715000000000001,0.720000000000001,0.725000000000001,0.730000000000001,
0.735000000000001,0.740000000000001,0.745000000000001,0.750000000000001,
0.755000000000001,0.760000000000001,0.765000000000001,0.770000000000001,
0.775000000000001,0.780000000000001,0.785000000000001,0.790000000000001,
0.795000000000001,0.800000000000001,0.805000000000001,0.810000000000001,
0.815000000000001,0.820000000000001,0.825000000000001,0.830000000000001,
0.835000000000001,0.840000000000001,0.845000000000001,0.850000000000001,
0.855000000000001,0.860000000000001,0.865000000000001,0.870000000000001,
0.875000000000001,0.880000000000001,0.885000000000001,0.890000000000001,
0.895000000000001,0.900000000000001,0.905000000000001,0.910000000000001,
0.915000000000001,0.920000000000001,0.925000000000001,0.930000000000001,
0.935000000000001,0.940000000000001,0.94142984443144),.UNSPECIFIED.)
CURVE()
GEOMETRIC_REPRESENTATION_ITEM()
RATIONAL_B_SPLINE_CURVE((1.,1.,1.,1.,1.,1.,1.,1.,1.,1.,1.,1.,1.,1.,1.,1.,
1.,1.,1.,1.,1.,1.,1.,1.,1.,1.,1.,1.,1.,1.,1.,1.,1.,1.,1.,1.,1.,1.,1.,1.,
1.,1.,1.,1.,1.,1.,1.,1.,1.,1.,1.,1.,1.,1.,1.,1.,1.,1.,1.,1.,1.,1.,1.,1.,
1.,1.,1.,1.,1.,1.,1.,1.,1.,1.,1.,1.,1.,1.,1.,1.,1.,1.,1.,1.,1.,1.,1.,1.,
1.,1.,1.,1.,1.,1.,1.,1.,1.,1.,1.,1.,1.,1.,1.,1.,1.,1.,1.,1.,1.,1.,1.,1.,
1.,1.,1.,1.,1.,1.,1.,1.,1.,1.,1.,1.,1.,1.,1.,1.,1.,1.,1.,1.,1.,1.,1.,1.,
1.,1.,1.,1.,1.,1.,1.,1.,1.,1.,1.,1.,1.,1.,1.,1.,1.,1.,1.,1.,1.,1.,1.,1.,
1.,1.,1.,1.,1.,1.,1.,1.,1.,1.,1.,1.,1.,1.,1.,1.,1.,1.,1.,1.,1.,1.,1.,1.,
1.,1.,1.,1.,1.,1.,1.,1.,1.,1.))
REPRESENTATION_ITEM('')
);
#510=(
BOUNDED_CURVE()
B_SPLINE_CURVE(5,(#100717,#100718,#100719,#100720,#100721,#100722,#100723,
#100724,#100725,#100726,#100727,#100728,#100729,#100730,#100731,#100732,
#100733,#100734,#100735,#100736,#100737,#100738,#100739,#100740,#100741,
#100742,#100743,#100744,#100745,#100746,#100747,#100748,#100749,#100750,
#100751,#100752,#100753,#100754,#100755,#100756,#100757,#100758,#100759,
#100760,#100761,#100762,#100763,#100764,#100765,#100766,#100767,#100768,
#100769,#100770,#100771,#100772,#100773,#100774,#100775,#100776,#100777,
#100778,#100779,#100780,#100781,#100782,#100783,#100784,#100785,#100786,
#100787,#100788,#100789,#100790,#100791,#100792,#100793,#100794,#100795,
#100796,#100797,#100798,#100799,#100800,#100801,#100802,#100803,#100804,
#100805,#100806,#100807,#100808,#100809,#100810,#100811,#100812,#100813,
#100814,#100815,#100816,#100817,#100818,#100819,#100820,#100821,#100822,
#100823,#100824,#100825,#100826,#100827,#100828,#100829,#100830,#100831,
#100832,#100833,#100834,#100835,#100836,#100837,#100838,#100839,#100840,
#100841,#100842,#100843,#100844,#100845,#100846,#100847,#100848,#100849,
#100850,#100851,#100852,#100853,#100854,#100855,#100856,#100857,#100858,
#100859,#100860,#100861,#100862,#100863,#100864,#100865,#100866,#100867,
#100868,#100869,#100870,#100871,#100872,#100873,#100874,#100875,#100876,
#100877,#100878,#100879,#100880,#100881,#100882,#100883,#100884,#100885,
#100886,#100887,#100888,#100889,#100890,#100891,#100892,#100893,#100894,
#100895,#100896,#100897,#100898,#100899,#100900,#100901,#100902,#100903,
#100904,#100905,#100906,#100907,#100908,#100909,#100910),.UNSPECIFIED.,
 .F.,.F.)
B_SPLINE_CURVE_WITH_KNOTS((6,1,1,1,1,1,1,1,1,1,1,1,1,1,1,1,1,1,1,1,1,1,
1,1,1,1,1,1,1,1,1,1,1,1,1,1,1,1,1,1,1,1,1,1,1,1,1,1,1,1,1,1,1,1,1,1,1,1,
1,1,1,1,1,1,1,1,1,1,1,1,1,1,1,1,1,1,1,1,1,1,1,1,1,1,1,1,1,1,1,1,1,1,1,1,
1,1,1,1,1,1,1,1,1,1,1,1,1,1,1,1,1,1,1,1,1,1,1,1,1,1,1,1,1,1,1,1,1,1,1,1,
1,1,1,1,1,1,1,1,1,1,1,1,1,1,1,1,1,1,1,1,1,1,1,1,1,1,1,1,1,1,1,1,1,1,1,1,
1,1,1,1,1,1,1,1,1,1,1,1,1,1,1,1,1,1,1,1,1,1,1,6),(-0.941429844431447,-0.940000000000001,
-0.935000000000001,-0.930000000000001,-0.925000000000001,-0.920000000000001,
-0.915000000000001,-0.910000000000001,-0.905000000000001,-0.900000000000001,
-0.895000000000001,-0.890000000000001,-0.885000000000001,-0.880000000000001,
-0.875000000000001,-0.870000000000001,-0.865000000000001,-0.860000000000001,
-0.855000000000001,-0.850000000000001,-0.845000000000001,-0.840000000000001,
-0.835000000000001,-0.830000000000001,-0.825000000000001,-0.820000000000001,
-0.815000000000001,-0.810000000000001,-0.805000000000001,-0.800000000000001,
-0.795000000000001,-0.790000000000001,-0.785000000000001,-0.780000000000001,
-0.775000000000001,-0.770000000000001,-0.765000000000001,-0.760000000000001,
-0.755000000000001,-0.750000000000001,-0.745000000000001,-0.740000000000001,
-0.735000000000001,-0.730000000000001,-0.725000000000001,-0.720000000000001,
-0.715000000000001,-0.710000000000001,-0.705000000000001,-0.700000000000001,
-0.695000000000001,-0.690000000000001,-0.685,-0.68,-0.675,-0.67,-0.665,
-0.66,-0.655,-0.65,-0.645,-0.64,-0.635,-0.63,-0.625,-0.62,-0.615,-0.61,
-0.605,-0.6,-0.595,-0.59,-0.585,-0.58,-0.575,-0.57,-0.565,-0.56,-0.555,
-0.55,-0.545,-0.54,-0.535,-0.53,-0.525,-0.52,-0.515,-0.51,-0.505,-0.5,-0.495,
-0.49,-0.485,-0.48,-0.475,-0.47,-0.465,-0.46,-0.455,-0.45,-0.445,-0.44,
-0.435,-0.43,-0.425,-0.42,-0.415,-0.41,-0.405,-0.4,-0.395,-0.39,-0.385,
-0.38,-0.375,-0.37,-0.365,-0.36,-0.355,-0.35,-0.345,-0.34,-0.335,-0.33,
-0.325,-0.32,-0.315,-0.31,-0.305,-0.3,-0.295,-0.29,-0.285,-0.28,-0.275,
-0.27,-0.265,-0.26,-0.255,-0.25,-0.245,-0.24,-0.235,-0.23,-0.225,-0.22,
-0.215,-0.21,-0.205,-0.2,-0.195,-0.19,-0.185,-0.18,-0.175,-0.17,-0.165,
-0.16,-0.155,-0.15,-0.145,-0.14,-0.135,-0.13,-0.125,-0.12,-0.115,-0.11,
-0.105,-0.1,-0.095,-0.09,-0.085,-0.08,-0.075,-0.07,-0.065,-0.06,-0.055,
-0.05,-0.045,-0.04,-0.035,-0.03,-0.025,-0.02,-0.015,-0.01,-0.005,0.),
 .UNSPECIFIED.)
CURVE()
GEOMETRIC_REPRESENTATION_ITEM()
RATIONAL_B_SPLINE_CURVE((1.,1.,1.,1.,1.,1.,1.,1.,1.,1.,1.,1.,1.,1.,1.,1.,
1.,1.,1.,1.,1.,1.,1.,1.,1.,1.,1.,1.,1.,1.,1.,1.,1.,1.,1.,1.,1.,1.,1.,1.,
1.,1.,1.,1.,1.,1.,1.,1.,1.,1.,1.,1.,1.,1.,1.,1.,1.,1.,1.,1.,1.,1.,1.,1.,
1.,1.,1.,1.,1.,1.,1.,1.,1.,1.,1.,1.,1.,1.,1.,1.,1.,1.,1.,1.,1.,1.,1.,1.,
1.,1.,1.,1.,1.,1.,1.,1.,1.,1.,1.,1.,1.,1.,1.,1.,1.,1.,1.,1.,1.,1.,1.,1.,
1.,1.,1.,1.,1.,1.,1.,1.,1.,1.,1.,1.,1.,1.,1.,1.,1.,1.,1.,1.,1.,1.,1.,1.,
1.,1.,1.,1.,1.,1.,1.,1.,1.,1.,1.,1.,1.,1.,1.,1.,1.,1.,1.,1.,1.,1.,1.,1.,
1.,1.,1.,1.,1.,1.,1.,1.,1.,1.,1.,1.,1.,1.,1.,1.,1.,1.,1.,1.,1.,1.,1.,1.,
1.,1.,1.,1.,1.,1.,1.,1.,1.,1.))
REPRESENTATION_ITEM('')
);
#511=(
BOUNDED_CURVE()
B_SPLINE_CURVE(5,(#101417,#101418,#101419,#101420,#101421,#101422,#101423,
#101424,#101425,#101426,#101427,#101428,#101429,#101430,#101431,#101432,
#101433,#101434,#101435,#101436,#101437,#101438,#101439,#101440,#101441,
#101442,#101443,#101444,#101445,#101446,#101447,#101448,#101449,#101450,
#101451,#101452,#101453,#101454,#101455,#101456,#101457,#101458,#101459,
#101460,#101461,#101462,#101463,#101464,#101465,#101466,#101467,#101468,
#101469,#101470,#101471,#101472,#101473,#101474,#101475,#101476,#101477,
#101478,#101479,#101480,#101481,#101482,#101483,#101484,#101485,#101486,
#101487,#101488,#101489,#101490,#101491,#101492,#101493,#101494,#101495,
#101496,#101497,#101498,#101499,#101500,#101501,#101502,#101503,#101504,
#101505,#101506,#101507,#101508,#101509,#101510,#101511,#101512,#101513,
#101514,#101515,#101516,#101517,#101518,#101519,#101520,#101521,#101522,
#101523,#101524,#101525,#101526,#101527,#101528,#101529,#101530,#101531,
#101532,#101533,#101534,#101535,#101536,#101537,#101538,#101539,#101540,
#101541,#101542,#101543,#101544,#101545,#101546,#101547,#101548,#101549,
#101550,#101551,#101552,#101553,#101554,#101555,#101556,#101557,#101558,
#101559,#101560,#101561,#101562,#101563,#101564,#101565,#101566,#101567,
#101568,#101569,#101570,#101571,#101572,#101573,#101574,#101575,#101576,
#101577,#101578,#101579,#101580,#101581,#101582,#101583,#101584,#101585,
#101586,#101587,#101588,#101589,#101590,#101591,#101592,#101593,#101594,
#101595,#101596,#101597,#101598,#101599,#101600,#101601,#101602,#101603,
#101604,#101605,#101606,#101607,#101608,#101609,#101610),.UNSPECIFIED.,
 .F.,.F.)
B_SPLINE_CURVE_WITH_KNOTS((6,1,1,1,1,1,1,1,1,1,1,1,1,1,1,1,1,1,1,1,1,1,
1,1,1,1,1,1,1,1,1,1,1,1,1,1,1,1,1,1,1,1,1,1,1,1,1,1,1,1,1,1,1,1,1,1,1,1,
1,1,1,1,1,1,1,1,1,1,1,1,1,1,1,1,1,1,1,1,1,1,1,1,1,1,1,1,1,1,1,1,1,1,1,1,
1,1,1,1,1,1,1,1,1,1,1,1,1,1,1,1,1,1,1,1,1,1,1,1,1,1,1,1,1,1,1,1,1,1,1,1,
1,1,1,1,1,1,1,1,1,1,1,1,1,1,1,1,1,1,1,1,1,1,1,1,1,1,1,1,1,1,1,1,1,1,1,1,
1,1,1,1,1,1,1,1,1,1,1,1,1,1,1,1,1,1,1,1,1,1,1,6),(0.,0.005,0.01,0.015,0.02,
0.025,0.03,0.035,0.04,0.045,0.05,0.055,0.06,0.065,0.07,0.075,0.08,0.085,
0.09,0.095,0.1,0.105,0.11,0.115,0.12,0.125,0.13,0.135,0.14,0.145,0.15,0.155,
0.16,0.165,0.17,0.175,0.18,0.185,0.19,0.195,0.2,0.205,0.21,0.215,0.22,0.225,
0.23,0.235,0.24,0.245,0.25,0.255,0.26,0.265,0.27,0.275,0.28,0.285,0.29,
0.295,0.3,0.305,0.31,0.315,0.32,0.325,0.33,0.335,0.34,0.345,0.35,0.355,
0.36,0.365,0.37,0.375,0.38,0.385,0.39,0.395,0.4,0.405,0.41,0.415,0.42,0.425,
0.43,0.435,0.44,0.445,0.45,0.455,0.46,0.465,0.47,0.475,0.48,0.485,0.49,
0.495,0.5,0.505,0.51,0.515,0.52,0.525,0.53,0.535,0.54,0.545,0.55,0.555,
0.56,0.565,0.57,0.575,0.58,0.585,0.59,0.595,0.6,0.605,0.61,0.615,0.62,0.625,
0.63,0.635,0.64,0.645,0.65,0.655,0.66,0.665,0.67,0.675,0.68,0.685,0.690000000000001,
0.695000000000001,0.700000000000001,0.705000000000001,0.710000000000001,
0.715000000000001,0.720000000000001,0.725000000000001,0.730000000000001,
0.735000000000001,0.740000000000001,0.745000000000001,0.750000000000001,
0.755000000000001,0.760000000000001,0.765000000000001,0.770000000000001,
0.775000000000001,0.780000000000001,0.785000000000001,0.790000000000001,
0.795000000000001,0.800000000000001,0.805000000000001,0.810000000000001,
0.815000000000001,0.820000000000001,0.825000000000001,0.830000000000001,
0.835000000000001,0.840000000000001,0.845000000000001,0.850000000000001,
0.855000000000001,0.860000000000001,0.865000000000001,0.870000000000001,
0.875000000000001,0.880000000000001,0.885000000000001,0.890000000000001,
0.895000000000001,0.900000000000001,0.905000000000001,0.910000000000001,
0.915000000000001,0.920000000000001,0.925000000000001,0.930000000000001,
0.935000000000001,0.940000000000001,0.94142984443143),.UNSPECIFIED.)
CURVE()
GEOMETRIC_REPRESENTATION_ITEM()
RATIONAL_B_SPLINE_CURVE((1.,1.,1.,1.,1.,1.,1.,1.,1.,1.,1.,1.,1.,1.,1.,1.,
1.,1.,1.,1.,1.,1.,1.,1.,1.,1.,1.,1.,1.,1.,1.,1.,1.,1.,1.,1.,1.,1.,1.,1.,
1.,1.,1.,1.,1.,1.,1.,1.,1.,1.,1.,1.,1.,1.,1.,1.,1.,1.,1.,1.,1.,1.,1.,1.,
1.,1.,1.,1.,1.,1.,1.,1.,1.,1.,1.,1.,1.,1.,1.,1.,1.,1.,1.,1.,1.,1.,1.,1.,
1.,1.,1.,1.,1.,1.,1.,1.,1.,1.,1.,1.,1.,1.,1.,1.,1.,1.,1.,1.,1.,1.,1.,1.,
1.,1.,1.,1.,1.,1.,1.,1.,1.,1.,1.,1.,1.,1.,1.,1.,1.,1.,1.,1.,1.,1.,1.,1.,
1.,1.,1.,1.,1.,1.,1.,1.,1.,1.,1.,1.,1.,1.,1.,1.,1.,1.,1.,1.,1.,1.,1.,1.,
1.,1.,1.,1.,1.,1.,1.,1.,1.,1.,1.,1.,1.,1.,1.,1.,1.,1.,1.,1.,1.,1.,1.,1.,
1.,1.,1.,1.,1.,1.,1.,1.,1.,1.))
REPRESENTATION_ITEM('')
);
#512=(
BOUNDED_CURVE()
B_SPLINE_CURVE(5,(#101613,#101614,#101615,#101616,#101617,#101618,#101619,
#101620,#101621,#101622,#101623,#101624,#101625,#101626,#101627,#101628,
#101629,#101630,#101631,#101632,#101633,#101634,#101635,#101636,#101637,
#101638,#101639,#101640,#101641,#101642,#101643,#101644,#101645,#101646,
#101647,#101648,#101649,#101650,#101651,#101652,#101653,#101654,#101655,
#101656,#101657,#101658,#101659,#101660,#101661,#101662,#101663,#101664,
#101665,#101666,#101667,#101668,#101669,#101670,#101671,#101672,#101673,
#101674,#101675,#101676,#101677,#101678,#101679,#101680,#101681,#101682,
#101683,#101684,#101685,#101686,#101687,#101688,#101689,#101690,#101691,
#101692,#101693,#101694,#101695,#101696,#101697,#101698,#101699,#101700,
#101701,#101702,#101703,#101704,#101705,#101706,#101707,#101708,#101709,
#101710,#101711,#101712,#101713,#101714,#101715,#101716,#101717,#101718,
#101719,#101720,#101721,#101722,#101723,#101724,#101725,#101726,#101727,
#101728,#101729,#101730,#101731,#101732,#101733,#101734,#101735,#101736,
#101737,#101738,#101739,#101740,#101741,#101742,#101743,#101744,#101745,
#101746,#101747,#101748,#101749,#101750,#101751,#101752,#101753,#101754,
#101755,#101756,#101757,#101758,#101759,#101760,#101761,#101762,#101763,
#101764,#101765,#101766,#101767,#101768,#101769,#101770,#101771,#101772,
#101773,#101774,#101775,#101776,#101777,#101778,#101779,#101780,#101781,
#101782,#101783,#101784,#101785,#101786,#101787,#101788,#101789,#101790,
#101791,#101792,#101793,#101794,#101795,#101796,#101797,#101798,#101799,
#101800,#101801,#101802,#101803,#101804,#101805,#101806),.UNSPECIFIED.,
 .F.,.F.)
B_SPLINE_CURVE_WITH_KNOTS((6,1,1,1,1,1,1,1,1,1,1,1,1,1,1,1,1,1,1,1,1,1,
1,1,1,1,1,1,1,1,1,1,1,1,1,1,1,1,1,1,1,1,1,1,1,1,1,1,1,1,1,1,1,1,1,1,1,1,
1,1,1,1,1,1,1,1,1,1,1,1,1,1,1,1,1,1,1,1,1,1,1,1,1,1,1,1,1,1,1,1,1,1,1,1,
1,1,1,1,1,1,1,1,1,1,1,1,1,1,1,1,1,1,1,1,1,1,1,1,1,1,1,1,1,1,1,1,1,1,1,1,
1,1,1,1,1,1,1,1,1,1,1,1,1,1,1,1,1,1,1,1,1,1,1,1,1,1,1,1,1,1,1,1,1,1,1,1,
1,1,1,1,1,1,1,1,1,1,1,1,1,1,1,1,1,1,1,1,1,1,1,6),(-0.94142984443143,-0.940000000000001,
-0.935000000000001,-0.930000000000001,-0.925000000000001,-0.920000000000001,
-0.915000000000001,-0.910000000000001,-0.905000000000001,-0.900000000000001,
-0.895000000000001,-0.890000000000001,-0.885000000000001,-0.880000000000001,
-0.875000000000001,-0.870000000000001,-0.865000000000001,-0.860000000000001,
-0.855000000000001,-0.850000000000001,-0.845000000000001,-0.840000000000001,
-0.835000000000001,-0.830000000000001,-0.825000000000001,-0.820000000000001,
-0.815000000000001,-0.810000000000001,-0.805000000000001,-0.800000000000001,
-0.795000000000001,-0.790000000000001,-0.785000000000001,-0.780000000000001,
-0.775000000000001,-0.770000000000001,-0.765000000000001,-0.760000000000001,
-0.755000000000001,-0.750000000000001,-0.745000000000001,-0.740000000000001,
-0.735000000000001,-0.730000000000001,-0.725000000000001,-0.720000000000001,
-0.715000000000001,-0.710000000000001,-0.705000000000001,-0.700000000000001,
-0.695000000000001,-0.690000000000001,-0.685,-0.68,-0.675,-0.67,-0.665,
-0.66,-0.655,-0.65,-0.645,-0.64,-0.635,-0.63,-0.625,-0.62,-0.615,-0.61,
-0.605,-0.6,-0.595,-0.59,-0.585,-0.58,-0.575,-0.57,-0.565,-0.56,-0.555,
-0.55,-0.545,-0.54,-0.535,-0.53,-0.525,-0.52,-0.515,-0.51,-0.505,-0.5,-0.495,
-0.49,-0.485,-0.48,-0.475,-0.47,-0.465,-0.46,-0.455,-0.45,-0.445,-0.44,
-0.435,-0.43,-0.425,-0.42,-0.415,-0.41,-0.405,-0.4,-0.395,-0.39,-0.385,
-0.38,-0.375,-0.37,-0.365,-0.36,-0.355,-0.35,-0.345,-0.34,-0.335,-0.33,
-0.325,-0.32,-0.315,-0.31,-0.305,-0.3,-0.295,-0.29,-0.285,-0.28,-0.275,
-0.27,-0.265,-0.26,-0.255,-0.25,-0.245,-0.24,-0.235,-0.23,-0.225,-0.22,
-0.215,-0.21,-0.205,-0.2,-0.195,-0.19,-0.185,-0.18,-0.175,-0.17,-0.165,
-0.16,-0.155,-0.15,-0.145,-0.14,-0.135,-0.13,-0.125,-0.12,-0.115,-0.11,
-0.105,-0.1,-0.095,-0.09,-0.085,-0.08,-0.075,-0.07,-0.065,-0.06,-0.055,
-0.05,-0.045,-0.04,-0.035,-0.03,-0.025,-0.02,-0.015,-0.01,-0.005,0.),
 .UNSPECIFIED.)
CURVE()
GEOMETRIC_REPRESENTATION_ITEM()
RATIONAL_B_SPLINE_CURVE((1.,1.,1.,1.,1.,1.,1.,1.,1.,1.,1.,1.,1.,1.,1.,1.,
1.,1.,1.,1.,1.,1.,1.,1.,1.,1.,1.,1.,1.,1.,1.,1.,1.,1.,1.,1.,1.,1.,1.,1.,
1.,1.,1.,1.,1.,1.,1.,1.,1.,1.,1.,1.,1.,1.,1.,1.,1.,1.,1.,1.,1.,1.,1.,1.,
1.,1.,1.,1.,1.,1.,1.,1.,1.,1.,1.,1.,1.,1.,1.,1.,1.,1.,1.,1.,1.,1.,1.,1.,
1.,1.,1.,1.,1.,1.,1.,1.,1.,1.,1.,1.,1.,1.,1.,1.,1.,1.,1.,1.,1.,1.,1.,1.,
1.,1.,1.,1.,1.,1.,1.,1.,1.,1.,1.,1.,1.,1.,1.,1.,1.,1.,1.,1.,1.,1.,1.,1.,
1.,1.,1.,1.,1.,1.,1.,1.,1.,1.,1.,1.,1.,1.,1.,1.,1.,1.,1.,1.,1.,1.,1.,1.,
1.,1.,1.,1.,1.,1.,1.,1.,1.,1.,1.,1.,1.,1.,1.,1.,1.,1.,1.,1.,1.,1.,1.,1.,
1.,1.,1.,1.,1.,1.,1.,1.,1.,1.))
REPRESENTATION_ITEM('')
);
#513=(
BOUNDED_CURVE()
B_SPLINE_CURVE(5,(#102313,#102314,#102315,#102316,#102317,#102318,#102319,
#102320,#102321,#102322,#102323,#102324,#102325,#102326,#102327,#102328,
#102329,#102330,#102331,#102332,#102333,#102334,#102335,#102336,#102337,
#102338,#102339,#102340,#102341,#102342,#102343,#102344,#102345,#102346,
#102347,#102348,#102349,#102350,#102351,#102352,#102353,#102354,#102355,
#102356,#102357,#102358,#102359,#102360,#102361,#102362,#102363,#102364,
#102365,#102366,#102367,#102368,#102369,#102370,#102371,#102372,#102373,
#102374,#102375,#102376,#102377,#102378,#102379,#102380,#102381,#102382,
#102383,#102384,#102385,#102386,#102387,#102388,#102389,#102390,#102391,
#102392,#102393,#102394,#102395,#102396,#102397,#102398,#102399,#102400,
#102401,#102402,#102403,#102404,#102405,#102406,#102407,#102408,#102409,
#102410,#102411,#102412,#102413,#102414,#102415,#102416,#102417,#102418,
#102419,#102420,#102421,#102422,#102423,#102424,#102425,#102426,#102427,
#102428,#102429,#102430,#102431,#102432,#102433,#102434,#102435,#102436,
#102437,#102438,#102439,#102440,#102441,#102442,#102443,#102444,#102445,
#102446,#102447,#102448,#102449,#102450,#102451,#102452,#102453,#102454,
#102455,#102456,#102457,#102458,#102459,#102460,#102461,#102462,#102463,
#102464,#102465,#102466,#102467,#102468,#102469,#102470,#102471,#102472,
#102473,#102474,#102475,#102476,#102477,#102478,#102479,#102480,#102481,
#102482,#102483,#102484,#102485,#102486,#102487,#102488,#102489,#102490,
#102491,#102492,#102493,#102494,#102495,#102496,#102497,#102498,#102499,
#102500,#102501,#102502,#102503,#102504,#102505,#102506),.UNSPECIFIED.,
 .F.,.F.)
B_SPLINE_CURVE_WITH_KNOTS((6,1,1,1,1,1,1,1,1,1,1,1,1,1,1,1,1,1,1,1,1,1,
1,1,1,1,1,1,1,1,1,1,1,1,1,1,1,1,1,1,1,1,1,1,1,1,1,1,1,1,1,1,1,1,1,1,1,1,
1,1,1,1,1,1,1,1,1,1,1,1,1,1,1,1,1,1,1,1,1,1,1,1,1,1,1,1,1,1,1,1,1,1,1,1,
1,1,1,1,1,1,1,1,1,1,1,1,1,1,1,1,1,1,1,1,1,1,1,1,1,1,1,1,1,1,1,1,1,1,1,1,
1,1,1,1,1,1,1,1,1,1,1,1,1,1,1,1,1,1,1,1,1,1,1,1,1,1,1,1,1,1,1,1,1,1,1,1,
1,1,1,1,1,1,1,1,1,1,1,1,1,1,1,1,1,1,1,1,1,1,1,6),(0.,0.005,0.01,0.015,0.02,
0.025,0.03,0.035,0.04,0.045,0.05,0.055,0.06,0.065,0.07,0.075,0.08,0.085,
0.09,0.095,0.1,0.105,0.11,0.115,0.12,0.125,0.13,0.135,0.14,0.145,0.15,0.155,
0.16,0.165,0.17,0.175,0.18,0.185,0.19,0.195,0.2,0.205,0.21,0.215,0.22,0.225,
0.23,0.235,0.24,0.245,0.25,0.255,0.26,0.265,0.27,0.275,0.28,0.285,0.29,
0.295,0.3,0.305,0.31,0.315,0.32,0.325,0.33,0.335,0.34,0.345,0.35,0.355,
0.36,0.365,0.37,0.375,0.38,0.385,0.39,0.395,0.4,0.405,0.41,0.415,0.42,0.425,
0.43,0.435,0.44,0.445,0.45,0.455,0.46,0.465,0.47,0.475,0.48,0.485,0.49,
0.495,0.5,0.505,0.51,0.515,0.52,0.525,0.53,0.535,0.54,0.545,0.55,0.555,
0.56,0.565,0.57,0.575,0.58,0.585,0.59,0.595,0.6,0.605,0.61,0.615,0.62,0.625,
0.63,0.635,0.64,0.645,0.65,0.655,0.66,0.665,0.67,0.675,0.68,0.685,0.690000000000001,
0.695000000000001,0.700000000000001,0.705000000000001,0.710000000000001,
0.715000000000001,0.720000000000001,0.725000000000001,0.730000000000001,
0.735000000000001,0.740000000000001,0.745000000000001,0.750000000000001,
0.755000000000001,0.760000000000001,0.765000000000001,0.770000000000001,
0.775000000000001,0.780000000000001,0.785000000000001,0.790000000000001,
0.795000000000001,0.800000000000001,0.805000000000001,0.810000000000001,
0.815000000000001,0.820000000000001,0.825000000000001,0.830000000000001,
0.835000000000001,0.840000000000001,0.845000000000001,0.850000000000001,
0.855000000000001,0.860000000000001,0.865000000000001,0.870000000000001,
0.875000000000001,0.880000000000001,0.885000000000001,0.890000000000001,
0.895000000000001,0.900000000000001,0.905000000000001,0.910000000000001,
0.915000000000001,0.920000000000001,0.925000000000001,0.930000000000001,
0.935000000000001,0.940000000000001,0.941429844431364),.UNSPECIFIED.)
CURVE()
GEOMETRIC_REPRESENTATION_ITEM()
RATIONAL_B_SPLINE_CURVE((1.,1.,1.,1.,1.,1.,1.,1.,1.,1.,1.,1.,1.,1.,1.,1.,
1.,1.,1.,1.,1.,1.,1.,1.,1.,1.,1.,1.,1.,1.,1.,1.,1.,1.,1.,1.,1.,1.,1.,1.,
1.,1.,1.,1.,1.,1.,1.,1.,1.,1.,1.,1.,1.,1.,1.,1.,1.,1.,1.,1.,1.,1.,1.,1.,
1.,1.,1.,1.,1.,1.,1.,1.,1.,1.,1.,1.,1.,1.,1.,1.,1.,1.,1.,1.,1.,1.,1.,1.,
1.,1.,1.,1.,1.,1.,1.,1.,1.,1.,1.,1.,1.,1.,1.,1.,1.,1.,1.,1.,1.,1.,1.,1.,
1.,1.,1.,1.,1.,1.,1.,1.,1.,1.,1.,1.,1.,1.,1.,1.,1.,1.,1.,1.,1.,1.,1.,1.,
1.,1.,1.,1.,1.,1.,1.,1.,1.,1.,1.,1.,1.,1.,1.,1.,1.,1.,1.,1.,1.,1.,1.,1.,
1.,1.,1.,1.,1.,1.,1.,1.,1.,1.,1.,1.,1.,1.,1.,1.,1.,1.,1.,1.,1.,1.,1.,1.,
1.,1.,1.,1.,1.,1.,1.,1.,1.,1.))
REPRESENTATION_ITEM('')
);
#514=(
BOUNDED_CURVE()
B_SPLINE_CURVE(5,(#102509,#102510,#102511,#102512,#102513,#102514,#102515,
#102516,#102517,#102518,#102519,#102520,#102521,#102522,#102523,#102524,
#102525,#102526,#102527,#102528,#102529,#102530,#102531,#102532,#102533,
#102534,#102535,#102536,#102537,#102538,#102539,#102540,#102541,#102542,
#102543,#102544,#102545,#102546,#102547,#102548,#102549,#102550,#102551,
#102552,#102553,#102554,#102555,#102556,#102557,#102558,#102559,#102560,
#102561,#102562,#102563,#102564,#102565,#102566,#102567,#102568,#102569,
#102570,#102571,#102572,#102573,#102574,#102575,#102576,#102577,#102578,
#102579,#102580,#102581,#102582,#102583,#102584,#102585,#102586,#102587,
#102588,#102589,#102590,#102591,#102592,#102593,#102594,#102595,#102596,
#102597,#102598,#102599,#102600,#102601,#102602,#102603,#102604,#102605,
#102606,#102607,#102608,#102609,#102610,#102611,#102612,#102613,#102614,
#102615,#102616,#102617,#102618,#102619,#102620,#102621,#102622,#102623,
#102624,#102625,#102626,#102627,#102628,#102629,#102630,#102631,#102632,
#102633,#102634,#102635,#102636,#102637,#102638,#102639,#102640,#102641,
#102642,#102643,#102644,#102645,#102646,#102647,#102648,#102649,#102650,
#102651,#102652,#102653,#102654,#102655,#102656,#102657,#102658,#102659,
#102660,#102661,#102662,#102663,#102664,#102665,#102666,#102667,#102668,
#102669,#102670,#102671,#102672,#102673,#102674,#102675,#102676,#102677,
#102678,#102679,#102680,#102681,#102682,#102683,#102684,#102685,#102686,
#102687,#102688,#102689,#102690,#102691,#102692,#102693,#102694,#102695,
#102696,#102697,#102698,#102699,#102700,#102701,#102702),.UNSPECIFIED.,
 .F.,.F.)
B_SPLINE_CURVE_WITH_KNOTS((6,1,1,1,1,1,1,1,1,1,1,1,1,1,1,1,1,1,1,1,1,1,
1,1,1,1,1,1,1,1,1,1,1,1,1,1,1,1,1,1,1,1,1,1,1,1,1,1,1,1,1,1,1,1,1,1,1,1,
1,1,1,1,1,1,1,1,1,1,1,1,1,1,1,1,1,1,1,1,1,1,1,1,1,1,1,1,1,1,1,1,1,1,1,1,
1,1,1,1,1,1,1,1,1,1,1,1,1,1,1,1,1,1,1,1,1,1,1,1,1,1,1,1,1,1,1,1,1,1,1,1,
1,1,1,1,1,1,1,1,1,1,1,1,1,1,1,1,1,1,1,1,1,1,1,1,1,1,1,1,1,1,1,1,1,1,1,1,
1,1,1,1,1,1,1,1,1,1,1,1,1,1,1,1,1,1,1,1,1,1,1,6),(-0.941429844431374,-0.940000000000001,
-0.935000000000001,-0.930000000000001,-0.925000000000001,-0.920000000000001,
-0.915000000000001,-0.910000000000001,-0.905000000000001,-0.900000000000001,
-0.895000000000001,-0.890000000000001,-0.885000000000001,-0.880000000000001,
-0.875000000000001,-0.870000000000001,-0.865000000000001,-0.860000000000001,
-0.855000000000001,-0.850000000000001,-0.845000000000001,-0.840000000000001,
-0.835000000000001,-0.830000000000001,-0.825000000000001,-0.820000000000001,
-0.815000000000001,-0.810000000000001,-0.805000000000001,-0.800000000000001,
-0.795000000000001,-0.790000000000001,-0.785000000000001,-0.780000000000001,
-0.775000000000001,-0.770000000000001,-0.765000000000001,-0.760000000000001,
-0.755000000000001,-0.750000000000001,-0.745000000000001,-0.740000000000001,
-0.735000000000001,-0.730000000000001,-0.725000000000001,-0.720000000000001,
-0.715000000000001,-0.710000000000001,-0.705000000000001,-0.700000000000001,
-0.695000000000001,-0.690000000000001,-0.685,-0.68,-0.675,-0.67,-0.665,
-0.66,-0.655,-0.65,-0.645,-0.64,-0.635,-0.63,-0.625,-0.62,-0.615,-0.61,
-0.605,-0.6,-0.595,-0.59,-0.585,-0.58,-0.575,-0.57,-0.565,-0.56,-0.555,
-0.55,-0.545,-0.54,-0.535,-0.53,-0.525,-0.52,-0.515,-0.51,-0.505,-0.5,-0.495,
-0.49,-0.485,-0.48,-0.475,-0.47,-0.465,-0.46,-0.455,-0.45,-0.445,-0.44,
-0.435,-0.43,-0.425,-0.42,-0.415,-0.41,-0.405,-0.4,-0.395,-0.39,-0.385,
-0.38,-0.375,-0.37,-0.365,-0.36,-0.355,-0.35,-0.345,-0.34,-0.335,-0.33,
-0.325,-0.32,-0.315,-0.31,-0.305,-0.3,-0.295,-0.29,-0.285,-0.28,-0.275,
-0.27,-0.265,-0.26,-0.255,-0.25,-0.245,-0.24,-0.235,-0.23,-0.225,-0.22,
-0.215,-0.21,-0.205,-0.2,-0.195,-0.19,-0.185,-0.18,-0.175,-0.17,-0.165,
-0.16,-0.155,-0.15,-0.145,-0.14,-0.135,-0.13,-0.125,-0.12,-0.115,-0.11,
-0.105,-0.1,-0.095,-0.09,-0.085,-0.08,-0.075,-0.07,-0.065,-0.06,-0.055,
-0.05,-0.045,-0.04,-0.035,-0.03,-0.025,-0.02,-0.015,-0.01,-0.005,0.),
 .UNSPECIFIED.)
CURVE()
GEOMETRIC_REPRESENTATION_ITEM()
RATIONAL_B_SPLINE_CURVE((1.,1.,1.,1.,1.,1.,1.,1.,1.,1.,1.,1.,1.,1.,1.,1.,
1.,1.,1.,1.,1.,1.,1.,1.,1.,1.,1.,1.,1.,1.,1.,1.,1.,1.,1.,1.,1.,1.,1.,1.,
1.,1.,1.,1.,1.,1.,1.,1.,1.,1.,1.,1.,1.,1.,1.,1.,1.,1.,1.,1.,1.,1.,1.,1.,
1.,1.,1.,1.,1.,1.,1.,1.,1.,1.,1.,1.,1.,1.,1.,1.,1.,1.,1.,1.,1.,1.,1.,1.,
1.,1.,1.,1.,1.,1.,1.,1.,1.,1.,1.,1.,1.,1.,1.,1.,1.,1.,1.,1.,1.,1.,1.,1.,
1.,1.,1.,1.,1.,1.,1.,1.,1.,1.,1.,1.,1.,1.,1.,1.,1.,1.,1.,1.,1.,1.,1.,1.,
1.,1.,1.,1.,1.,1.,1.,1.,1.,1.,1.,1.,1.,1.,1.,1.,1.,1.,1.,1.,1.,1.,1.,1.,
1.,1.,1.,1.,1.,1.,1.,1.,1.,1.,1.,1.,1.,1.,1.,1.,1.,1.,1.,1.,1.,1.,1.,1.,
1.,1.,1.,1.,1.,1.,1.,1.,1.,1.))
REPRESENTATION_ITEM('')
);
#515=(
BOUNDED_CURVE()
B_SPLINE_CURVE(5,(#103209,#103210,#103211,#103212,#103213,#103214,#103215,
#103216,#103217,#103218,#103219,#103220,#103221,#103222,#103223,#103224,
#103225,#103226,#103227,#103228,#103229,#103230,#103231,#103232,#103233,
#103234,#103235,#103236,#103237,#103238,#103239,#103240,#103241,#103242,
#103243,#103244,#103245,#103246,#103247,#103248,#103249,#103250,#103251,
#103252,#103253,#103254,#103255,#103256,#103257,#103258,#103259,#103260,
#103261,#103262,#103263,#103264,#103265,#103266,#103267,#103268,#103269,
#103270,#103271,#103272,#103273,#103274,#103275,#103276,#103277,#103278,
#103279,#103280,#103281,#103282,#103283,#103284,#103285,#103286,#103287,
#103288,#103289,#103290,#103291,#103292,#103293,#103294,#103295,#103296,
#103297,#103298,#103299,#103300,#103301,#103302,#103303,#103304,#103305,
#103306,#103307,#103308,#103309,#103310,#103311,#103312,#103313,#103314,
#103315,#103316,#103317,#103318,#103319,#103320,#103321,#103322,#103323,
#103324,#103325,#103326,#103327,#103328,#103329,#103330,#103331,#103332,
#103333,#103334,#103335,#103336,#103337,#103338,#103339,#103340,#103341,
#103342,#103343,#103344,#103345,#103346,#103347,#103348,#103349,#103350,
#103351,#103352,#103353,#103354,#103355,#103356,#103357,#103358,#103359,
#103360,#103361,#103362,#103363,#103364,#103365,#103366,#103367,#103368,
#103369,#103370,#103371,#103372,#103373,#103374,#103375,#103376,#103377,
#103378,#103379,#103380,#103381,#103382,#103383,#103384,#103385,#103386,
#103387,#103388,#103389,#103390,#103391,#103392,#103393,#103394,#103395,
#103396,#103397,#103398,#103399,#103400,#103401,#103402),.UNSPECIFIED.,
 .F.,.F.)
B_SPLINE_CURVE_WITH_KNOTS((6,1,1,1,1,1,1,1,1,1,1,1,1,1,1,1,1,1,1,1,1,1,
1,1,1,1,1,1,1,1,1,1,1,1,1,1,1,1,1,1,1,1,1,1,1,1,1,1,1,1,1,1,1,1,1,1,1,1,
1,1,1,1,1,1,1,1,1,1,1,1,1,1,1,1,1,1,1,1,1,1,1,1,1,1,1,1,1,1,1,1,1,1,1,1,
1,1,1,1,1,1,1,1,1,1,1,1,1,1,1,1,1,1,1,1,1,1,1,1,1,1,1,1,1,1,1,1,1,1,1,1,
1,1,1,1,1,1,1,1,1,1,1,1,1,1,1,1,1,1,1,1,1,1,1,1,1,1,1,1,1,1,1,1,1,1,1,1,
1,1,1,1,1,1,1,1,1,1,1,1,1,1,1,1,1,1,1,1,1,1,1,6),(0.,0.005,0.01,0.015,0.02,
0.025,0.03,0.035,0.04,0.045,0.05,0.055,0.06,0.065,0.07,0.075,0.08,0.085,
0.09,0.095,0.1,0.105,0.11,0.115,0.12,0.125,0.13,0.135,0.14,0.145,0.15,0.155,
0.16,0.165,0.17,0.175,0.18,0.185,0.19,0.195,0.2,0.205,0.21,0.215,0.22,0.225,
0.23,0.235,0.24,0.245,0.25,0.255,0.26,0.265,0.27,0.275,0.28,0.285,0.29,
0.295,0.3,0.305,0.31,0.315,0.32,0.325,0.33,0.335,0.34,0.345,0.35,0.355,
0.36,0.365,0.37,0.375,0.38,0.385,0.39,0.395,0.4,0.405,0.41,0.415,0.42,0.425,
0.43,0.435,0.44,0.445,0.45,0.455,0.46,0.465,0.47,0.475,0.48,0.485,0.49,
0.495,0.5,0.505,0.51,0.515,0.52,0.525,0.53,0.535,0.54,0.545,0.55,0.555,
0.56,0.565,0.57,0.575,0.58,0.585,0.59,0.595,0.6,0.605,0.61,0.615,0.62,0.625,
0.63,0.635,0.64,0.645,0.65,0.655,0.66,0.665,0.67,0.675,0.68,0.685,0.690000000000001,
0.695000000000001,0.700000000000001,0.705000000000001,0.710000000000001,
0.715000000000001,0.720000000000001,0.725000000000001,0.730000000000001,
0.735000000000001,0.740000000000001,0.745000000000001,0.750000000000001,
0.755000000000001,0.760000000000001,0.765000000000001,0.770000000000001,
0.775000000000001,0.780000000000001,0.785000000000001,0.790000000000001,
0.795000000000001,0.800000000000001,0.805000000000001,0.810000000000001,
0.815000000000001,0.820000000000001,0.825000000000001,0.830000000000001,
0.835000000000001,0.840000000000001,0.845000000000001,0.850000000000001,
0.855000000000001,0.860000000000001,0.865000000000001,0.870000000000001,
0.875000000000001,0.880000000000001,0.885000000000001,0.890000000000001,
0.895000000000001,0.900000000000001,0.905000000000001,0.910000000000001,
0.915000000000001,0.920000000000001,0.925000000000001,0.930000000000001,
0.935000000000001,0.940000000000001,0.94142984443135),.UNSPECIFIED.)
CURVE()
GEOMETRIC_REPRESENTATION_ITEM()
RATIONAL_B_SPLINE_CURVE((1.,1.,1.,1.,1.,1.,1.,1.,1.,1.,1.,1.,1.,1.,1.,1.,
1.,1.,1.,1.,1.,1.,1.,1.,1.,1.,1.,1.,1.,1.,1.,1.,1.,1.,1.,1.,1.,1.,1.,1.,
1.,1.,1.,1.,1.,1.,1.,1.,1.,1.,1.,1.,1.,1.,1.,1.,1.,1.,1.,1.,1.,1.,1.,1.,
1.,1.,1.,1.,1.,1.,1.,1.,1.,1.,1.,1.,1.,1.,1.,1.,1.,1.,1.,1.,1.,1.,1.,1.,
1.,1.,1.,1.,1.,1.,1.,1.,1.,1.,1.,1.,1.,1.,1.,1.,1.,1.,1.,1.,1.,1.,1.,1.,
1.,1.,1.,1.,1.,1.,1.,1.,1.,1.,1.,1.,1.,1.,1.,1.,1.,1.,1.,1.,1.,1.,1.,1.,
1.,1.,1.,1.,1.,1.,1.,1.,1.,1.,1.,1.,1.,1.,1.,1.,1.,1.,1.,1.,1.,1.,1.,1.,
1.,1.,1.,1.,1.,1.,1.,1.,1.,1.,1.,1.,1.,1.,1.,1.,1.,1.,1.,1.,1.,1.,1.,1.,
1.,1.,1.,1.,1.,1.,1.,1.,1.,1.))
REPRESENTATION_ITEM('')
);
#516=(
BOUNDED_CURVE()
B_SPLINE_CURVE(5,(#103405,#103406,#103407,#103408,#103409,#103410,#103411,
#103412,#103413,#103414,#103415,#103416,#103417,#103418,#103419,#103420,
#103421,#103422,#103423,#103424,#103425,#103426,#103427,#103428,#103429,
#103430,#103431,#103432,#103433,#103434,#103435,#103436,#103437,#103438,
#103439,#103440,#103441,#103442,#103443,#103444,#103445,#103446,#103447,
#103448,#103449,#103450,#103451,#103452,#103453,#103454,#103455,#103456,
#103457,#103458,#103459,#103460,#103461,#103462,#103463,#103464,#103465,
#103466,#103467,#103468,#103469,#103470,#103471,#103472,#103473,#103474,
#103475,#103476,#103477,#103478,#103479,#103480,#103481,#103482,#103483,
#103484,#103485,#103486,#103487,#103488,#103489,#103490,#103491,#103492,
#103493,#103494,#103495,#103496,#103497,#103498,#103499,#103500,#103501,
#103502,#103503,#103504,#103505,#103506,#103507,#103508,#103509,#103510,
#103511,#103512,#103513,#103514,#103515,#103516,#103517,#103518,#103519,
#103520,#103521,#103522,#103523,#103524,#103525,#103526,#103527,#103528,
#103529,#103530,#103531,#103532,#103533,#103534,#103535,#103536,#103537,
#103538,#103539,#103540,#103541,#103542,#103543,#103544,#103545,#103546,
#103547,#103548,#103549,#103550,#103551,#103552,#103553,#103554,#103555,
#103556,#103557,#103558,#103559,#103560,#103561,#103562,#103563,#103564,
#103565,#103566,#103567,#103568,#103569,#103570,#103571,#103572,#103573,
#103574,#103575,#103576,#103577,#103578,#103579,#103580,#103581,#103582,
#103583,#103584,#103585,#103586,#103587,#103588,#103589,#103590,#103591,
#103592,#103593,#103594,#103595,#103596,#103597,#103598),.UNSPECIFIED.,
 .F.,.F.)
B_SPLINE_CURVE_WITH_KNOTS((6,1,1,1,1,1,1,1,1,1,1,1,1,1,1,1,1,1,1,1,1,1,
1,1,1,1,1,1,1,1,1,1,1,1,1,1,1,1,1,1,1,1,1,1,1,1,1,1,1,1,1,1,1,1,1,1,1,1,
1,1,1,1,1,1,1,1,1,1,1,1,1,1,1,1,1,1,1,1,1,1,1,1,1,1,1,1,1,1,1,1,1,1,1,1,
1,1,1,1,1,1,1,1,1,1,1,1,1,1,1,1,1,1,1,1,1,1,1,1,1,1,1,1,1,1,1,1,1,1,1,1,
1,1,1,1,1,1,1,1,1,1,1,1,1,1,1,1,1,1,1,1,1,1,1,1,1,1,1,1,1,1,1,1,1,1,1,1,
1,1,1,1,1,1,1,1,1,1,1,1,1,1,1,1,1,1,1,1,1,1,1,6),(-0.94142984443135,-0.940000000000001,
-0.935000000000001,-0.930000000000001,-0.925000000000001,-0.920000000000001,
-0.915000000000001,-0.910000000000001,-0.905000000000001,-0.900000000000001,
-0.895000000000001,-0.890000000000001,-0.885000000000001,-0.880000000000001,
-0.875000000000001,-0.870000000000001,-0.865000000000001,-0.860000000000001,
-0.855000000000001,-0.850000000000001,-0.845000000000001,-0.840000000000001,
-0.835000000000001,-0.830000000000001,-0.825000000000001,-0.820000000000001,
-0.815000000000001,-0.810000000000001,-0.805000000000001,-0.800000000000001,
-0.795000000000001,-0.790000000000001,-0.785000000000001,-0.780000000000001,
-0.775000000000001,-0.770000000000001,-0.765000000000001,-0.760000000000001,
-0.755000000000001,-0.750000000000001,-0.745000000000001,-0.740000000000001,
-0.735000000000001,-0.730000000000001,-0.725000000000001,-0.720000000000001,
-0.715000000000001,-0.710000000000001,-0.705000000000001,-0.700000000000001,
-0.695000000000001,-0.690000000000001,-0.685,-0.68,-0.675,-0.67,-0.665,
-0.66,-0.655,-0.65,-0.645,-0.64,-0.635,-0.63,-0.625,-0.62,-0.615,-0.61,
-0.605,-0.6,-0.595,-0.59,-0.585,-0.58,-0.575,-0.57,-0.565,-0.56,-0.555,
-0.55,-0.545,-0.54,-0.535,-0.53,-0.525,-0.52,-0.515,-0.51,-0.505,-0.5,-0.495,
-0.49,-0.485,-0.48,-0.475,-0.47,-0.465,-0.46,-0.455,-0.45,-0.445,-0.44,
-0.435,-0.43,-0.425,-0.42,-0.415,-0.41,-0.405,-0.4,-0.395,-0.39,-0.385,
-0.38,-0.375,-0.37,-0.365,-0.36,-0.355,-0.35,-0.345,-0.34,-0.335,-0.33,
-0.325,-0.32,-0.315,-0.31,-0.305,-0.3,-0.295,-0.29,-0.285,-0.28,-0.275,
-0.27,-0.265,-0.26,-0.255,-0.25,-0.245,-0.24,-0.235,-0.23,-0.225,-0.22,
-0.215,-0.21,-0.205,-0.2,-0.195,-0.19,-0.185,-0.18,-0.175,-0.17,-0.165,
-0.16,-0.155,-0.15,-0.145,-0.14,-0.135,-0.13,-0.125,-0.12,-0.115,-0.11,
-0.105,-0.1,-0.095,-0.09,-0.085,-0.08,-0.075,-0.07,-0.065,-0.06,-0.055,
-0.05,-0.045,-0.04,-0.035,-0.03,-0.025,-0.02,-0.015,-0.01,-0.005,0.),
 .UNSPECIFIED.)
CURVE()
GEOMETRIC_REPRESENTATION_ITEM()
RATIONAL_B_SPLINE_CURVE((1.,1.,1.,1.,1.,1.,1.,1.,1.,1.,1.,1.,1.,1.,1.,1.,
1.,1.,1.,1.,1.,1.,1.,1.,1.,1.,1.,1.,1.,1.,1.,1.,1.,1.,1.,1.,1.,1.,1.,1.,
1.,1.,1.,1.,1.,1.,1.,1.,1.,1.,1.,1.,1.,1.,1.,1.,1.,1.,1.,1.,1.,1.,1.,1.,
1.,1.,1.,1.,1.,1.,1.,1.,1.,1.,1.,1.,1.,1.,1.,1.,1.,1.,1.,1.,1.,1.,1.,1.,
1.,1.,1.,1.,1.,1.,1.,1.,1.,1.,1.,1.,1.,1.,1.,1.,1.,1.,1.,1.,1.,1.,1.,1.,
1.,1.,1.,1.,1.,1.,1.,1.,1.,1.,1.,1.,1.,1.,1.,1.,1.,1.,1.,1.,1.,1.,1.,1.,
1.,1.,1.,1.,1.,1.,1.,1.,1.,1.,1.,1.,1.,1.,1.,1.,1.,1.,1.,1.,1.,1.,1.,1.,
1.,1.,1.,1.,1.,1.,1.,1.,1.,1.,1.,1.,1.,1.,1.,1.,1.,1.,1.,1.,1.,1.,1.,1.,
1.,1.,1.,1.,1.,1.,1.,1.,1.,1.))
REPRESENTATION_ITEM('')
);
#517=(
BOUNDED_CURVE()
B_SPLINE_CURVE(5,(#104105,#104106,#104107,#104108,#104109,#104110,#104111,
#104112,#104113,#104114,#104115,#104116,#104117,#104118,#104119,#104120,
#104121,#104122,#104123,#104124,#104125,#104126,#104127,#104128,#104129,
#104130,#104131,#104132,#104133,#104134,#104135,#104136,#104137,#104138,
#104139,#104140,#104141,#104142,#104143,#104144,#104145,#104146,#104147,
#104148,#104149,#104150,#104151,#104152,#104153,#104154,#104155,#104156,
#104157,#104158,#104159,#104160,#104161,#104162,#104163,#104164,#104165,
#104166,#104167,#104168,#104169,#104170,#104171,#104172,#104173,#104174,
#104175,#104176,#104177,#104178,#104179,#104180,#104181,#104182,#104183,
#104184,#104185,#104186,#104187,#104188,#104189,#104190,#104191,#104192,
#104193,#104194,#104195,#104196,#104197,#104198,#104199,#104200,#104201,
#104202,#104203,#104204,#104205,#104206,#104207,#104208,#104209,#104210,
#104211,#104212,#104213,#104214,#104215,#104216,#104217,#104218,#104219,
#104220,#104221,#104222,#104223,#104224,#104225,#104226,#104227,#104228,
#104229,#104230,#104231,#104232,#104233,#104234,#104235,#104236,#104237,
#104238,#104239,#104240,#104241,#104242,#104243,#104244,#104245,#104246,
#104247,#104248,#104249,#104250,#104251,#104252,#104253,#104254,#104255,
#104256,#104257,#104258,#104259,#104260,#104261,#104262,#104263,#104264,
#104265,#104266,#104267,#104268,#104269,#104270,#104271,#104272,#104273,
#104274,#104275,#104276,#104277,#104278,#104279,#104280,#104281,#104282,
#104283,#104284,#104285,#104286,#104287,#104288,#104289,#104290,#104291,
#104292,#104293,#104294,#104295,#104296,#104297,#104298),.UNSPECIFIED.,
 .F.,.F.)
B_SPLINE_CURVE_WITH_KNOTS((6,1,1,1,1,1,1,1,1,1,1,1,1,1,1,1,1,1,1,1,1,1,
1,1,1,1,1,1,1,1,1,1,1,1,1,1,1,1,1,1,1,1,1,1,1,1,1,1,1,1,1,1,1,1,1,1,1,1,
1,1,1,1,1,1,1,1,1,1,1,1,1,1,1,1,1,1,1,1,1,1,1,1,1,1,1,1,1,1,1,1,1,1,1,1,
1,1,1,1,1,1,1,1,1,1,1,1,1,1,1,1,1,1,1,1,1,1,1,1,1,1,1,1,1,1,1,1,1,1,1,1,
1,1,1,1,1,1,1,1,1,1,1,1,1,1,1,1,1,1,1,1,1,1,1,1,1,1,1,1,1,1,1,1,1,1,1,1,
1,1,1,1,1,1,1,1,1,1,1,1,1,1,1,1,1,1,1,1,1,1,1,6),(0.,0.005,0.01,0.015,0.02,
0.025,0.03,0.035,0.04,0.045,0.05,0.055,0.06,0.065,0.07,0.075,0.08,0.085,
0.09,0.095,0.1,0.105,0.11,0.115,0.12,0.125,0.13,0.135,0.14,0.145,0.15,0.155,
0.16,0.165,0.17,0.175,0.18,0.185,0.19,0.195,0.2,0.205,0.21,0.215,0.22,0.225,
0.23,0.235,0.24,0.245,0.25,0.255,0.26,0.265,0.27,0.275,0.28,0.285,0.29,
0.295,0.3,0.305,0.31,0.315,0.32,0.325,0.33,0.335,0.34,0.345,0.35,0.355,
0.36,0.365,0.37,0.375,0.38,0.385,0.39,0.395,0.4,0.405,0.41,0.415,0.42,0.425,
0.43,0.435,0.44,0.445,0.45,0.455,0.46,0.465,0.47,0.475,0.48,0.485,0.49,
0.495,0.5,0.505,0.51,0.515,0.52,0.525,0.53,0.535,0.54,0.545,0.55,0.555,
0.56,0.565,0.57,0.575,0.58,0.585,0.59,0.595,0.6,0.605,0.61,0.615,0.62,0.625,
0.63,0.635,0.64,0.645,0.65,0.655,0.66,0.665,0.67,0.675,0.68,0.685,0.690000000000001,
0.695000000000001,0.700000000000001,0.705000000000001,0.710000000000001,
0.715000000000001,0.720000000000001,0.725000000000001,0.730000000000001,
0.735000000000001,0.740000000000001,0.745000000000001,0.750000000000001,
0.755000000000001,0.760000000000001,0.765000000000001,0.770000000000001,
0.775000000000001,0.780000000000001,0.785000000000001,0.790000000000001,
0.795000000000001,0.800000000000001,0.805000000000001,0.810000000000001,
0.815000000000001,0.820000000000001,0.825000000000001,0.830000000000001,
0.835000000000001,0.840000000000001,0.845000000000001,0.850000000000001,
0.855000000000001,0.860000000000001,0.865000000000001,0.870000000000001,
0.875000000000001,0.880000000000001,0.885000000000001,0.890000000000001,
0.895000000000001,0.900000000000001,0.905000000000001,0.910000000000001,
0.915000000000001,0.920000000000001,0.925000000000001,0.930000000000001,
0.935000000000001,0.940000000000001,0.941429844431347),.UNSPECIFIED.)
CURVE()
GEOMETRIC_REPRESENTATION_ITEM()
RATIONAL_B_SPLINE_CURVE((1.,1.,1.,1.,1.,1.,1.,1.,1.,1.,1.,1.,1.,1.,1.,1.,
1.,1.,1.,1.,1.,1.,1.,1.,1.,1.,1.,1.,1.,1.,1.,1.,1.,1.,1.,1.,1.,1.,1.,1.,
1.,1.,1.,1.,1.,1.,1.,1.,1.,1.,1.,1.,1.,1.,1.,1.,1.,1.,1.,1.,1.,1.,1.,1.,
1.,1.,1.,1.,1.,1.,1.,1.,1.,1.,1.,1.,1.,1.,1.,1.,1.,1.,1.,1.,1.,1.,1.,1.,
1.,1.,1.,1.,1.,1.,1.,1.,1.,1.,1.,1.,1.,1.,1.,1.,1.,1.,1.,1.,1.,1.,1.,1.,
1.,1.,1.,1.,1.,1.,1.,1.,1.,1.,1.,1.,1.,1.,1.,1.,1.,1.,1.,1.,1.,1.,1.,1.,
1.,1.,1.,1.,1.,1.,1.,1.,1.,1.,1.,1.,1.,1.,1.,1.,1.,1.,1.,1.,1.,1.,1.,1.,
1.,1.,1.,1.,1.,1.,1.,1.,1.,1.,1.,1.,1.,1.,1.,1.,1.,1.,1.,1.,1.,1.,1.,1.,
1.,1.,1.,1.,1.,1.,1.,1.,1.,1.))
REPRESENTATION_ITEM('')
);
#518=(
BOUNDED_CURVE()
B_SPLINE_CURVE(5,(#104301,#104302,#104303,#104304,#104305,#104306,#104307,
#104308,#104309,#104310,#104311,#104312,#104313,#104314,#104315,#104316,
#104317,#104318,#104319,#104320,#104321,#104322,#104323,#104324,#104325,
#104326,#104327,#104328,#104329,#104330,#104331,#104332,#104333,#104334,
#104335,#104336,#104337,#104338,#104339,#104340,#104341,#104342,#104343,
#104344,#104345,#104346,#104347,#104348,#104349,#104350,#104351,#104352,
#104353,#104354,#104355,#104356,#104357,#104358,#104359,#104360,#104361,
#104362,#104363,#104364,#104365,#104366,#104367,#104368,#104369,#104370,
#104371,#104372,#104373,#104374,#104375,#104376,#104377,#104378,#104379,
#104380,#104381,#104382,#104383,#104384,#104385,#104386,#104387,#104388,
#104389,#104390,#104391,#104392,#104393,#104394,#104395,#104396,#104397,
#104398,#104399,#104400,#104401,#104402,#104403,#104404,#104405,#104406,
#104407,#104408,#104409,#104410,#104411,#104412,#104413,#104414,#104415,
#104416,#104417,#104418,#104419,#104420,#104421,#104422,#104423,#104424,
#104425,#104426,#104427,#104428,#104429,#104430,#104431,#104432,#104433,
#104434,#104435,#104436,#104437,#104438,#104439,#104440,#104441,#104442,
#104443,#104444,#104445,#104446,#104447,#104448,#104449,#104450,#104451,
#104452,#104453,#104454,#104455,#104456,#104457,#104458,#104459,#104460,
#104461,#104462,#104463,#104464,#104465,#104466,#104467,#104468,#104469,
#104470,#104471,#104472,#104473,#104474,#104475,#104476,#104477,#104478,
#104479,#104480,#104481,#104482,#104483,#104484,#104485,#104486,#104487,
#104488,#104489,#104490,#104491,#104492,#104493,#104494),.UNSPECIFIED.,
 .F.,.F.)
B_SPLINE_CURVE_WITH_KNOTS((6,1,1,1,1,1,1,1,1,1,1,1,1,1,1,1,1,1,1,1,1,1,
1,1,1,1,1,1,1,1,1,1,1,1,1,1,1,1,1,1,1,1,1,1,1,1,1,1,1,1,1,1,1,1,1,1,1,1,
1,1,1,1,1,1,1,1,1,1,1,1,1,1,1,1,1,1,1,1,1,1,1,1,1,1,1,1,1,1,1,1,1,1,1,1,
1,1,1,1,1,1,1,1,1,1,1,1,1,1,1,1,1,1,1,1,1,1,1,1,1,1,1,1,1,1,1,1,1,1,1,1,
1,1,1,1,1,1,1,1,1,1,1,1,1,1,1,1,1,1,1,1,1,1,1,1,1,1,1,1,1,1,1,1,1,1,1,1,
1,1,1,1,1,1,1,1,1,1,1,1,1,1,1,1,1,1,1,1,1,1,1,6),(-0.941429844431341,-0.940000000000001,
-0.935000000000001,-0.930000000000001,-0.925000000000001,-0.920000000000001,
-0.915000000000001,-0.910000000000001,-0.905000000000001,-0.900000000000001,
-0.895000000000001,-0.890000000000001,-0.885000000000001,-0.880000000000001,
-0.875000000000001,-0.870000000000001,-0.865000000000001,-0.860000000000001,
-0.855000000000001,-0.850000000000001,-0.845000000000001,-0.840000000000001,
-0.835000000000001,-0.830000000000001,-0.825000000000001,-0.820000000000001,
-0.815000000000001,-0.810000000000001,-0.805000000000001,-0.800000000000001,
-0.795000000000001,-0.790000000000001,-0.785000000000001,-0.780000000000001,
-0.775000000000001,-0.770000000000001,-0.765000000000001,-0.760000000000001,
-0.755000000000001,-0.750000000000001,-0.745000000000001,-0.740000000000001,
-0.735000000000001,-0.730000000000001,-0.725000000000001,-0.720000000000001,
-0.715000000000001,-0.710000000000001,-0.705000000000001,-0.700000000000001,
-0.695000000000001,-0.690000000000001,-0.685,-0.68,-0.675,-0.67,-0.665,
-0.66,-0.655,-0.65,-0.645,-0.64,-0.635,-0.63,-0.625,-0.62,-0.615,-0.61,
-0.605,-0.6,-0.595,-0.59,-0.585,-0.58,-0.575,-0.57,-0.565,-0.56,-0.555,
-0.55,-0.545,-0.54,-0.535,-0.53,-0.525,-0.52,-0.515,-0.51,-0.505,-0.5,-0.495,
-0.49,-0.485,-0.48,-0.475,-0.47,-0.465,-0.46,-0.455,-0.45,-0.445,-0.44,
-0.435,-0.43,-0.425,-0.42,-0.415,-0.41,-0.405,-0.4,-0.395,-0.39,-0.385,
-0.38,-0.375,-0.37,-0.365,-0.36,-0.355,-0.35,-0.345,-0.34,-0.335,-0.33,
-0.325,-0.32,-0.315,-0.31,-0.305,-0.3,-0.295,-0.29,-0.285,-0.28,-0.275,
-0.27,-0.265,-0.26,-0.255,-0.25,-0.245,-0.24,-0.235,-0.23,-0.225,-0.22,
-0.215,-0.21,-0.205,-0.2,-0.195,-0.19,-0.185,-0.18,-0.175,-0.17,-0.165,
-0.16,-0.155,-0.15,-0.145,-0.14,-0.135,-0.13,-0.125,-0.12,-0.115,-0.11,
-0.105,-0.1,-0.095,-0.09,-0.085,-0.08,-0.075,-0.07,-0.065,-0.06,-0.055,
-0.05,-0.045,-0.04,-0.035,-0.03,-0.025,-0.02,-0.015,-0.01,-0.005,0.),
 .UNSPECIFIED.)
CURVE()
GEOMETRIC_REPRESENTATION_ITEM()
RATIONAL_B_SPLINE_CURVE((1.,1.,1.,1.,1.,1.,1.,1.,1.,1.,1.,1.,1.,1.,1.,1.,
1.,1.,1.,1.,1.,1.,1.,1.,1.,1.,1.,1.,1.,1.,1.,1.,1.,1.,1.,1.,1.,1.,1.,1.,
1.,1.,1.,1.,1.,1.,1.,1.,1.,1.,1.,1.,1.,1.,1.,1.,1.,1.,1.,1.,1.,1.,1.,1.,
1.,1.,1.,1.,1.,1.,1.,1.,1.,1.,1.,1.,1.,1.,1.,1.,1.,1.,1.,1.,1.,1.,1.,1.,
1.,1.,1.,1.,1.,1.,1.,1.,1.,1.,1.,1.,1.,1.,1.,1.,1.,1.,1.,1.,1.,1.,1.,1.,
1.,1.,1.,1.,1.,1.,1.,1.,1.,1.,1.,1.,1.,1.,1.,1.,1.,1.,1.,1.,1.,1.,1.,1.,
1.,1.,1.,1.,1.,1.,1.,1.,1.,1.,1.,1.,1.,1.,1.,1.,1.,1.,1.,1.,1.,1.,1.,1.,
1.,1.,1.,1.,1.,1.,1.,1.,1.,1.,1.,1.,1.,1.,1.,1.,1.,1.,1.,1.,1.,1.,1.,1.,
1.,1.,1.,1.,1.,1.,1.,1.,1.,1.))
REPRESENTATION_ITEM('')
);
#519=(
BOUNDED_CURVE()
B_SPLINE_CURVE(5,(#105001,#105002,#105003,#105004,#105005,#105006,#105007,
#105008,#105009,#105010,#105011,#105012,#105013,#105014,#105015,#105016,
#105017,#105018,#105019,#105020,#105021,#105022,#105023,#105024,#105025,
#105026,#105027,#105028,#105029,#105030,#105031,#105032,#105033,#105034,
#105035,#105036,#105037,#105038,#105039,#105040,#105041,#105042,#105043,
#105044,#105045,#105046,#105047,#105048,#105049,#105050,#105051,#105052,
#105053,#105054,#105055,#105056,#105057,#105058,#105059,#105060,#105061,
#105062,#105063,#105064,#105065,#105066,#105067,#105068,#105069,#105070,
#105071,#105072,#105073,#105074,#105075,#105076,#105077,#105078,#105079,
#105080,#105081,#105082,#105083,#105084,#105085,#105086,#105087,#105088,
#105089,#105090,#105091,#105092,#105093,#105094,#105095,#105096,#105097,
#105098,#105099,#105100,#105101,#105102,#105103,#105104,#105105,#105106,
#105107,#105108,#105109,#105110,#105111,#105112,#105113,#105114,#105115,
#105116,#105117,#105118,#105119,#105120,#105121,#105122,#105123,#105124,
#105125,#105126,#105127,#105128,#105129,#105130,#105131,#105132,#105133,
#105134,#105135,#105136,#105137,#105138,#105139,#105140,#105141,#105142,
#105143,#105144,#105145,#105146,#105147,#105148,#105149,#105150,#105151,
#105152,#105153,#105154,#105155,#105156,#105157,#105158,#105159,#105160,
#105161,#105162,#105163,#105164,#105165,#105166,#105167,#105168,#105169,
#105170,#105171,#105172,#105173,#105174,#105175,#105176,#105177,#105178,
#105179,#105180,#105181,#105182,#105183,#105184,#105185,#105186,#105187,
#105188,#105189,#105190,#105191,#105192,#105193,#105194),.UNSPECIFIED.,
 .F.,.F.)
B_SPLINE_CURVE_WITH_KNOTS((6,1,1,1,1,1,1,1,1,1,1,1,1,1,1,1,1,1,1,1,1,1,
1,1,1,1,1,1,1,1,1,1,1,1,1,1,1,1,1,1,1,1,1,1,1,1,1,1,1,1,1,1,1,1,1,1,1,1,
1,1,1,1,1,1,1,1,1,1,1,1,1,1,1,1,1,1,1,1,1,1,1,1,1,1,1,1,1,1,1,1,1,1,1,1,
1,1,1,1,1,1,1,1,1,1,1,1,1,1,1,1,1,1,1,1,1,1,1,1,1,1,1,1,1,1,1,1,1,1,1,1,
1,1,1,1,1,1,1,1,1,1,1,1,1,1,1,1,1,1,1,1,1,1,1,1,1,1,1,1,1,1,1,1,1,1,1,1,
1,1,1,1,1,1,1,1,1,1,1,1,1,1,1,1,1,1,1,1,1,1,1,6),(0.,0.005,0.01,0.015,0.02,
0.025,0.03,0.035,0.04,0.045,0.05,0.055,0.06,0.065,0.07,0.075,0.08,0.085,
0.09,0.095,0.1,0.105,0.11,0.115,0.12,0.125,0.13,0.135,0.14,0.145,0.15,0.155,
0.16,0.165,0.17,0.175,0.18,0.185,0.19,0.195,0.2,0.205,0.21,0.215,0.22,0.225,
0.23,0.235,0.24,0.245,0.25,0.255,0.26,0.265,0.27,0.275,0.28,0.285,0.29,
0.295,0.3,0.305,0.31,0.315,0.32,0.325,0.33,0.335,0.34,0.345,0.35,0.355,
0.36,0.365,0.37,0.375,0.38,0.385,0.39,0.395,0.4,0.405,0.41,0.415,0.42,0.425,
0.43,0.435,0.44,0.445,0.45,0.455,0.46,0.465,0.47,0.475,0.48,0.485,0.49,
0.495,0.5,0.505,0.51,0.515,0.52,0.525,0.53,0.535,0.54,0.545,0.55,0.555,
0.56,0.565,0.57,0.575,0.58,0.585,0.59,0.595,0.6,0.605,0.61,0.615,0.62,0.625,
0.63,0.635,0.64,0.645,0.65,0.655,0.66,0.665,0.67,0.675,0.68,0.685,0.690000000000001,
0.695000000000001,0.700000000000001,0.705000000000001,0.710000000000001,
0.715000000000001,0.720000000000001,0.725000000000001,0.730000000000001,
0.735000000000001,0.740000000000001,0.745000000000001,0.750000000000001,
0.755000000000001,0.760000000000001,0.765000000000001,0.770000000000001,
0.775000000000001,0.780000000000001,0.785000000000001,0.790000000000001,
0.795000000000001,0.800000000000001,0.805000000000001,0.810000000000001,
0.815000000000001,0.820000000000001,0.825000000000001,0.830000000000001,
0.835000000000001,0.840000000000001,0.845000000000001,0.850000000000001,
0.855000000000001,0.860000000000001,0.865000000000001,0.870000000000001,
0.875000000000001,0.880000000000001,0.885000000000001,0.890000000000001,
0.895000000000001,0.900000000000001,0.905000000000001,0.910000000000001,
0.915000000000001,0.920000000000001,0.925000000000001,0.930000000000001,
0.935000000000001,0.940000000000001,0.941429844431379),.UNSPECIFIED.)
CURVE()
GEOMETRIC_REPRESENTATION_ITEM()
RATIONAL_B_SPLINE_CURVE((1.,1.,1.,1.,1.,1.,1.,1.,1.,1.,1.,1.,1.,1.,1.,1.,
1.,1.,1.,1.,1.,1.,1.,1.,1.,1.,1.,1.,1.,1.,1.,1.,1.,1.,1.,1.,1.,1.,1.,1.,
1.,1.,1.,1.,1.,1.,1.,1.,1.,1.,1.,1.,1.,1.,1.,1.,1.,1.,1.,1.,1.,1.,1.,1.,
1.,1.,1.,1.,1.,1.,1.,1.,1.,1.,1.,1.,1.,1.,1.,1.,1.,1.,1.,1.,1.,1.,1.,1.,
1.,1.,1.,1.,1.,1.,1.,1.,1.,1.,1.,1.,1.,1.,1.,1.,1.,1.,1.,1.,1.,1.,1.,1.,
1.,1.,1.,1.,1.,1.,1.,1.,1.,1.,1.,1.,1.,1.,1.,1.,1.,1.,1.,1.,1.,1.,1.,1.,
1.,1.,1.,1.,1.,1.,1.,1.,1.,1.,1.,1.,1.,1.,1.,1.,1.,1.,1.,1.,1.,1.,1.,1.,
1.,1.,1.,1.,1.,1.,1.,1.,1.,1.,1.,1.,1.,1.,1.,1.,1.,1.,1.,1.,1.,1.,1.,1.,
1.,1.,1.,1.,1.,1.,1.,1.,1.,1.))
REPRESENTATION_ITEM('')
);
#520=(
BOUNDED_CURVE()
B_SPLINE_CURVE(5,(#105197,#105198,#105199,#105200,#105201,#105202,#105203,
#105204,#105205,#105206,#105207,#105208,#105209,#105210,#105211,#105212,
#105213,#105214,#105215,#105216,#105217,#105218,#105219,#105220,#105221,
#105222,#105223,#105224,#105225,#105226,#105227,#105228,#105229,#105230,
#105231,#105232,#105233,#105234,#105235,#105236,#105237,#105238,#105239,
#105240,#105241,#105242,#105243,#105244,#105245,#105246,#105247,#105248,
#105249,#105250,#105251,#105252,#105253,#105254,#105255,#105256,#105257,
#105258,#105259,#105260,#105261,#105262,#105263,#105264,#105265,#105266,
#105267,#105268,#105269,#105270,#105271,#105272,#105273,#105274,#105275,
#105276,#105277,#105278,#105279,#105280,#105281,#105282,#105283,#105284,
#105285,#105286,#105287,#105288,#105289,#105290,#105291,#105292,#105293,
#105294,#105295,#105296,#105297,#105298,#105299,#105300,#105301,#105302,
#105303,#105304,#105305,#105306,#105307,#105308,#105309,#105310,#105311,
#105312,#105313,#105314,#105315,#105316,#105317,#105318,#105319,#105320,
#105321,#105322,#105323,#105324,#105325,#105326,#105327,#105328,#105329,
#105330,#105331,#105332,#105333,#105334,#105335,#105336,#105337,#105338,
#105339,#105340,#105341,#105342,#105343,#105344,#105345,#105346,#105347,
#105348,#105349,#105350,#105351,#105352,#105353,#105354,#105355,#105356,
#105357,#105358,#105359,#105360,#105361,#105362,#105363,#105364,#105365,
#105366,#105367,#105368,#105369,#105370,#105371,#105372,#105373,#105374,
#105375,#105376,#105377,#105378,#105379,#105380,#105381,#105382,#105383,
#105384,#105385,#105386,#105387,#105388,#105389,#105390),.UNSPECIFIED.,
 .F.,.F.)
B_SPLINE_CURVE_WITH_KNOTS((6,1,1,1,1,1,1,1,1,1,1,1,1,1,1,1,1,1,1,1,1,1,
1,1,1,1,1,1,1,1,1,1,1,1,1,1,1,1,1,1,1,1,1,1,1,1,1,1,1,1,1,1,1,1,1,1,1,1,
1,1,1,1,1,1,1,1,1,1,1,1,1,1,1,1,1,1,1,1,1,1,1,1,1,1,1,1,1,1,1,1,1,1,1,1,
1,1,1,1,1,1,1,1,1,1,1,1,1,1,1,1,1,1,1,1,1,1,1,1,1,1,1,1,1,1,1,1,1,1,1,1,
1,1,1,1,1,1,1,1,1,1,1,1,1,1,1,1,1,1,1,1,1,1,1,1,1,1,1,1,1,1,1,1,1,1,1,1,
1,1,1,1,1,1,1,1,1,1,1,1,1,1,1,1,1,1,1,1,1,1,1,6),(-0.941429844431382,-0.940000000000001,
-0.935000000000001,-0.930000000000001,-0.925000000000001,-0.920000000000001,
-0.915000000000001,-0.910000000000001,-0.905000000000001,-0.900000000000001,
-0.895000000000001,-0.890000000000001,-0.885000000000001,-0.880000000000001,
-0.875000000000001,-0.870000000000001,-0.865000000000001,-0.860000000000001,
-0.855000000000001,-0.850000000000001,-0.845000000000001,-0.840000000000001,
-0.835000000000001,-0.830000000000001,-0.825000000000001,-0.820000000000001,
-0.815000000000001,-0.810000000000001,-0.805000000000001,-0.800000000000001,
-0.795000000000001,-0.790000000000001,-0.785000000000001,-0.780000000000001,
-0.775000000000001,-0.770000000000001,-0.765000000000001,-0.760000000000001,
-0.755000000000001,-0.750000000000001,-0.745000000000001,-0.740000000000001,
-0.735000000000001,-0.730000000000001,-0.725000000000001,-0.720000000000001,
-0.715000000000001,-0.710000000000001,-0.705000000000001,-0.700000000000001,
-0.695000000000001,-0.690000000000001,-0.685,-0.68,-0.675,-0.67,-0.665,
-0.66,-0.655,-0.65,-0.645,-0.64,-0.635,-0.63,-0.625,-0.62,-0.615,-0.61,
-0.605,-0.6,-0.595,-0.59,-0.585,-0.58,-0.575,-0.57,-0.565,-0.56,-0.555,
-0.55,-0.545,-0.54,-0.535,-0.53,-0.525,-0.52,-0.515,-0.51,-0.505,-0.5,-0.495,
-0.49,-0.485,-0.48,-0.475,-0.47,-0.465,-0.46,-0.455,-0.45,-0.445,-0.44,
-0.435,-0.43,-0.425,-0.42,-0.415,-0.41,-0.405,-0.4,-0.395,-0.39,-0.385,
-0.38,-0.375,-0.37,-0.365,-0.36,-0.355,-0.35,-0.345,-0.34,-0.335,-0.33,
-0.325,-0.32,-0.315,-0.31,-0.305,-0.3,-0.295,-0.29,-0.285,-0.28,-0.275,
-0.27,-0.265,-0.26,-0.255,-0.25,-0.245,-0.24,-0.235,-0.23,-0.225,-0.22,
-0.215,-0.21,-0.205,-0.2,-0.195,-0.19,-0.185,-0.18,-0.175,-0.17,-0.165,
-0.16,-0.155,-0.15,-0.145,-0.14,-0.135,-0.13,-0.125,-0.12,-0.115,-0.11,
-0.105,-0.1,-0.095,-0.09,-0.085,-0.08,-0.075,-0.07,-0.065,-0.06,-0.055,
-0.05,-0.045,-0.04,-0.035,-0.03,-0.025,-0.02,-0.015,-0.01,-0.005,0.),
 .UNSPECIFIED.)
CURVE()
GEOMETRIC_REPRESENTATION_ITEM()
RATIONAL_B_SPLINE_CURVE((1.,1.,1.,1.,1.,1.,1.,1.,1.,1.,1.,1.,1.,1.,1.,1.,
1.,1.,1.,1.,1.,1.,1.,1.,1.,1.,1.,1.,1.,1.,1.,1.,1.,1.,1.,1.,1.,1.,1.,1.,
1.,1.,1.,1.,1.,1.,1.,1.,1.,1.,1.,1.,1.,1.,1.,1.,1.,1.,1.,1.,1.,1.,1.,1.,
1.,1.,1.,1.,1.,1.,1.,1.,1.,1.,1.,1.,1.,1.,1.,1.,1.,1.,1.,1.,1.,1.,1.,1.,
1.,1.,1.,1.,1.,1.,1.,1.,1.,1.,1.,1.,1.,1.,1.,1.,1.,1.,1.,1.,1.,1.,1.,1.,
1.,1.,1.,1.,1.,1.,1.,1.,1.,1.,1.,1.,1.,1.,1.,1.,1.,1.,1.,1.,1.,1.,1.,1.,
1.,1.,1.,1.,1.,1.,1.,1.,1.,1.,1.,1.,1.,1.,1.,1.,1.,1.,1.,1.,1.,1.,1.,1.,
1.,1.,1.,1.,1.,1.,1.,1.,1.,1.,1.,1.,1.,1.,1.,1.,1.,1.,1.,1.,1.,1.,1.,1.,
1.,1.,1.,1.,1.,1.,1.,1.,1.,1.))
REPRESENTATION_ITEM('')
);
#521=(
BOUNDED_CURVE()
B_SPLINE_CURVE(5,(#105897,#105898,#105899,#105900,#105901,#105902,#105903,
#105904,#105905,#105906,#105907,#105908,#105909,#105910,#105911,#105912,
#105913,#105914,#105915,#105916,#105917,#105918,#105919,#105920,#105921,
#105922,#105923,#105924,#105925,#105926,#105927,#105928,#105929,#105930,
#105931,#105932,#105933,#105934,#105935,#105936,#105937,#105938,#105939,
#105940,#105941,#105942,#105943,#105944,#105945,#105946,#105947,#105948,
#105949,#105950,#105951,#105952,#105953,#105954,#105955,#105956,#105957,
#105958,#105959,#105960,#105961,#105962,#105963,#105964,#105965,#105966,
#105967,#105968,#105969,#105970,#105971,#105972,#105973,#105974,#105975,
#105976,#105977,#105978,#105979,#105980,#105981,#105982,#105983,#105984,
#105985,#105986,#105987,#105988,#105989,#105990,#105991,#105992,#105993,
#105994,#105995,#105996,#105997,#105998,#105999,#106000,#106001,#106002,
#106003,#106004,#106005,#106006,#106007,#106008,#106009,#106010,#106011,
#106012,#106013,#106014,#106015,#106016,#106017,#106018,#106019,#106020,
#106021,#106022,#106023,#106024,#106025,#106026,#106027,#106028,#106029,
#106030,#106031,#106032,#106033,#106034,#106035,#106036,#106037,#106038,
#106039,#106040,#106041,#106042,#106043,#106044,#106045,#106046,#106047,
#106048,#106049,#106050,#106051,#106052,#106053,#106054,#106055,#106056,
#106057,#106058,#106059,#106060,#106061,#106062,#106063,#106064,#106065,
#106066,#106067,#106068,#106069,#106070,#106071,#106072,#106073,#106074,
#106075,#106076,#106077,#106078,#106079,#106080,#106081,#106082,#106083,
#106084,#106085,#106086,#106087,#106088,#106089,#106090),.UNSPECIFIED.,
 .F.,.F.)
B_SPLINE_CURVE_WITH_KNOTS((6,1,1,1,1,1,1,1,1,1,1,1,1,1,1,1,1,1,1,1,1,1,
1,1,1,1,1,1,1,1,1,1,1,1,1,1,1,1,1,1,1,1,1,1,1,1,1,1,1,1,1,1,1,1,1,1,1,1,
1,1,1,1,1,1,1,1,1,1,1,1,1,1,1,1,1,1,1,1,1,1,1,1,1,1,1,1,1,1,1,1,1,1,1,1,
1,1,1,1,1,1,1,1,1,1,1,1,1,1,1,1,1,1,1,1,1,1,1,1,1,1,1,1,1,1,1,1,1,1,1,1,
1,1,1,1,1,1,1,1,1,1,1,1,1,1,1,1,1,1,1,1,1,1,1,1,1,1,1,1,1,1,1,1,1,1,1,1,
1,1,1,1,1,1,1,1,1,1,1,1,1,1,1,1,1,1,1,1,1,1,1,6),(0.,0.005,0.01,0.015,0.02,
0.025,0.03,0.035,0.04,0.045,0.05,0.055,0.06,0.065,0.07,0.075,0.08,0.085,
0.09,0.095,0.1,0.105,0.11,0.115,0.12,0.125,0.13,0.135,0.14,0.145,0.15,0.155,
0.16,0.165,0.17,0.175,0.18,0.185,0.19,0.195,0.2,0.205,0.21,0.215,0.22,0.225,
0.23,0.235,0.24,0.245,0.25,0.255,0.26,0.265,0.27,0.275,0.28,0.285,0.29,
0.295,0.3,0.305,0.31,0.315,0.32,0.325,0.33,0.335,0.34,0.345,0.35,0.355,
0.36,0.365,0.37,0.375,0.38,0.385,0.39,0.395,0.4,0.405,0.41,0.415,0.42,0.425,
0.43,0.435,0.44,0.445,0.45,0.455,0.46,0.465,0.47,0.475,0.48,0.485,0.49,
0.495,0.5,0.505,0.51,0.515,0.52,0.525,0.53,0.535,0.54,0.545,0.55,0.555,
0.56,0.565,0.57,0.575,0.58,0.585,0.59,0.595,0.6,0.605,0.61,0.615,0.62,0.625,
0.63,0.635,0.64,0.645,0.65,0.655,0.66,0.665,0.67,0.675,0.68,0.685,0.690000000000001,
0.695000000000001,0.700000000000001,0.705000000000001,0.710000000000001,
0.715000000000001,0.720000000000001,0.725000000000001,0.730000000000001,
0.735000000000001,0.740000000000001,0.745000000000001,0.750000000000001,
0.755000000000001,0.760000000000001,0.765000000000001,0.770000000000001,
0.775000000000001,0.780000000000001,0.785000000000001,0.790000000000001,
0.795000000000001,0.800000000000001,0.805000000000001,0.810000000000001,
0.815000000000001,0.820000000000001,0.825000000000001,0.830000000000001,
0.835000000000001,0.840000000000001,0.845000000000001,0.850000000000001,
0.855000000000001,0.860000000000001,0.865000000000001,0.870000000000001,
0.875000000000001,0.880000000000001,0.885000000000001,0.890000000000001,
0.895000000000001,0.900000000000001,0.905000000000001,0.910000000000001,
0.915000000000001,0.920000000000001,0.925000000000001,0.930000000000001,
0.935000000000001,0.940000000000001,0.941429844431321),.UNSPECIFIED.)
CURVE()
GEOMETRIC_REPRESENTATION_ITEM()
RATIONAL_B_SPLINE_CURVE((1.,1.,1.,1.,1.,1.,1.,1.,1.,1.,1.,1.,1.,1.,1.,1.,
1.,1.,1.,1.,1.,1.,1.,1.,1.,1.,1.,1.,1.,1.,1.,1.,1.,1.,1.,1.,1.,1.,1.,1.,
1.,1.,1.,1.,1.,1.,1.,1.,1.,1.,1.,1.,1.,1.,1.,1.,1.,1.,1.,1.,1.,1.,1.,1.,
1.,1.,1.,1.,1.,1.,1.,1.,1.,1.,1.,1.,1.,1.,1.,1.,1.,1.,1.,1.,1.,1.,1.,1.,
1.,1.,1.,1.,1.,1.,1.,1.,1.,1.,1.,1.,1.,1.,1.,1.,1.,1.,1.,1.,1.,1.,1.,1.,
1.,1.,1.,1.,1.,1.,1.,1.,1.,1.,1.,1.,1.,1.,1.,1.,1.,1.,1.,1.,1.,1.,1.,1.,
1.,1.,1.,1.,1.,1.,1.,1.,1.,1.,1.,1.,1.,1.,1.,1.,1.,1.,1.,1.,1.,1.,1.,1.,
1.,1.,1.,1.,1.,1.,1.,1.,1.,1.,1.,1.,1.,1.,1.,1.,1.,1.,1.,1.,1.,1.,1.,1.,
1.,1.,1.,1.,1.,1.,1.,1.,1.,1.))
REPRESENTATION_ITEM('')
);
#522=(
BOUNDED_CURVE()
B_SPLINE_CURVE(5,(#106093,#106094,#106095,#106096,#106097,#106098,#106099,
#106100,#106101,#106102,#106103,#106104,#106105,#106106,#106107,#106108,
#106109,#106110,#106111,#106112,#106113,#106114,#106115,#106116,#106117,
#106118,#106119,#106120,#106121,#106122,#106123,#106124,#106125,#106126,
#106127,#106128,#106129,#106130,#106131,#106132,#106133,#106134,#106135,
#106136,#106137,#106138,#106139,#106140,#106141,#106142,#106143,#106144,
#106145,#106146,#106147,#106148,#106149,#106150,#106151,#106152,#106153,
#106154,#106155,#106156,#106157,#106158,#106159,#106160,#106161,#106162,
#106163,#106164,#106165,#106166,#106167,#106168,#106169,#106170,#106171,
#106172,#106173,#106174,#106175,#106176,#106177,#106178,#106179,#106180,
#106181,#106182,#106183,#106184,#106185,#106186,#106187,#106188,#106189,
#106190,#106191,#106192,#106193,#106194,#106195,#106196,#106197,#106198,
#106199,#106200,#106201,#106202,#106203,#106204,#106205,#106206,#106207,
#106208,#106209,#106210,#106211,#106212,#106213,#106214,#106215,#106216,
#106217,#106218,#106219,#106220,#106221,#106222,#106223,#106224,#106225,
#106226,#106227,#106228,#106229,#106230,#106231,#106232,#106233,#106234,
#106235,#106236,#106237,#106238,#106239,#106240,#106241,#106242,#106243,
#106244,#106245,#106246,#106247,#106248,#106249,#106250,#106251,#106252,
#106253,#106254,#106255,#106256,#106257,#106258,#106259,#106260,#106261,
#106262,#106263,#106264,#106265,#106266,#106267,#106268,#106269,#106270,
#106271,#106272,#106273,#106274,#106275,#106276,#106277,#106278,#106279,
#106280,#106281,#106282,#106283,#106284,#106285,#106286),.UNSPECIFIED.,
 .F.,.F.)
B_SPLINE_CURVE_WITH_KNOTS((6,1,1,1,1,1,1,1,1,1,1,1,1,1,1,1,1,1,1,1,1,1,
1,1,1,1,1,1,1,1,1,1,1,1,1,1,1,1,1,1,1,1,1,1,1,1,1,1,1,1,1,1,1,1,1,1,1,1,
1,1,1,1,1,1,1,1,1,1,1,1,1,1,1,1,1,1,1,1,1,1,1,1,1,1,1,1,1,1,1,1,1,1,1,1,
1,1,1,1,1,1,1,1,1,1,1,1,1,1,1,1,1,1,1,1,1,1,1,1,1,1,1,1,1,1,1,1,1,1,1,1,
1,1,1,1,1,1,1,1,1,1,1,1,1,1,1,1,1,1,1,1,1,1,1,1,1,1,1,1,1,1,1,1,1,1,1,1,
1,1,1,1,1,1,1,1,1,1,1,1,1,1,1,1,1,1,1,1,1,1,1,6),(-0.941429844431305,-0.940000000000001,
-0.935000000000001,-0.930000000000001,-0.925000000000001,-0.920000000000001,
-0.915000000000001,-0.910000000000001,-0.905000000000001,-0.900000000000001,
-0.895000000000001,-0.890000000000001,-0.885000000000001,-0.880000000000001,
-0.875000000000001,-0.870000000000001,-0.865000000000001,-0.860000000000001,
-0.855000000000001,-0.850000000000001,-0.845000000000001,-0.840000000000001,
-0.835000000000001,-0.830000000000001,-0.825000000000001,-0.820000000000001,
-0.815000000000001,-0.810000000000001,-0.805000000000001,-0.800000000000001,
-0.795000000000001,-0.790000000000001,-0.785000000000001,-0.780000000000001,
-0.775000000000001,-0.770000000000001,-0.765000000000001,-0.760000000000001,
-0.755000000000001,-0.750000000000001,-0.745000000000001,-0.740000000000001,
-0.735000000000001,-0.730000000000001,-0.725000000000001,-0.720000000000001,
-0.715000000000001,-0.710000000000001,-0.705000000000001,-0.700000000000001,
-0.695000000000001,-0.690000000000001,-0.685,-0.68,-0.675,-0.67,-0.665,
-0.66,-0.655,-0.65,-0.645,-0.64,-0.635,-0.63,-0.625,-0.62,-0.615,-0.61,
-0.605,-0.6,-0.595,-0.59,-0.585,-0.58,-0.575,-0.57,-0.565,-0.56,-0.555,
-0.55,-0.545,-0.54,-0.535,-0.53,-0.525,-0.52,-0.515,-0.51,-0.505,-0.5,-0.495,
-0.49,-0.485,-0.48,-0.475,-0.47,-0.465,-0.46,-0.455,-0.45,-0.445,-0.44,
-0.435,-0.43,-0.425,-0.42,-0.415,-0.41,-0.405,-0.4,-0.395,-0.39,-0.385,
-0.38,-0.375,-0.37,-0.365,-0.36,-0.355,-0.35,-0.345,-0.34,-0.335,-0.33,
-0.325,-0.32,-0.315,-0.31,-0.305,-0.3,-0.295,-0.29,-0.285,-0.28,-0.275,
-0.27,-0.265,-0.26,-0.255,-0.25,-0.245,-0.24,-0.235,-0.23,-0.225,-0.22,
-0.215,-0.21,-0.205,-0.2,-0.195,-0.19,-0.185,-0.18,-0.175,-0.17,-0.165,
-0.16,-0.155,-0.15,-0.145,-0.14,-0.135,-0.13,-0.125,-0.12,-0.115,-0.11,
-0.105,-0.1,-0.095,-0.09,-0.085,-0.08,-0.075,-0.07,-0.065,-0.06,-0.055,
-0.05,-0.045,-0.04,-0.035,-0.03,-0.025,-0.02,-0.015,-0.01,-0.005,0.),
 .UNSPECIFIED.)
CURVE()
GEOMETRIC_REPRESENTATION_ITEM()
RATIONAL_B_SPLINE_CURVE((1.,1.,1.,1.,1.,1.,1.,1.,1.,1.,1.,1.,1.,1.,1.,1.,
1.,1.,1.,1.,1.,1.,1.,1.,1.,1.,1.,1.,1.,1.,1.,1.,1.,1.,1.,1.,1.,1.,1.,1.,
1.,1.,1.,1.,1.,1.,1.,1.,1.,1.,1.,1.,1.,1.,1.,1.,1.,1.,1.,1.,1.,1.,1.,1.,
1.,1.,1.,1.,1.,1.,1.,1.,1.,1.,1.,1.,1.,1.,1.,1.,1.,1.,1.,1.,1.,1.,1.,1.,
1.,1.,1.,1.,1.,1.,1.,1.,1.,1.,1.,1.,1.,1.,1.,1.,1.,1.,1.,1.,1.,1.,1.,1.,
1.,1.,1.,1.,1.,1.,1.,1.,1.,1.,1.,1.,1.,1.,1.,1.,1.,1.,1.,1.,1.,1.,1.,1.,
1.,1.,1.,1.,1.,1.,1.,1.,1.,1.,1.,1.,1.,1.,1.,1.,1.,1.,1.,1.,1.,1.,1.,1.,
1.,1.,1.,1.,1.,1.,1.,1.,1.,1.,1.,1.,1.,1.,1.,1.,1.,1.,1.,1.,1.,1.,1.,1.,
1.,1.,1.,1.,1.,1.,1.,1.,1.,1.))
REPRESENTATION_ITEM('')
);
#523=(
BOUNDED_CURVE()
B_SPLINE_CURVE(5,(#106793,#106794,#106795,#106796,#106797,#106798,#106799,
#106800,#106801,#106802,#106803,#106804,#106805,#106806,#106807,#106808,
#106809,#106810,#106811,#106812,#106813,#106814,#106815,#106816,#106817,
#106818,#106819,#106820,#106821,#106822,#106823,#106824,#106825,#106826,
#106827,#106828,#106829,#106830,#106831,#106832,#106833,#106834,#106835,
#106836,#106837,#106838,#106839,#106840,#106841,#106842,#106843,#106844,
#106845,#106846,#106847,#106848,#106849,#106850,#106851,#106852,#106853,
#106854,#106855,#106856,#106857,#106858,#106859,#106860,#106861,#106862,
#106863,#106864,#106865,#106866,#106867,#106868,#106869,#106870,#106871,
#106872,#106873,#106874,#106875,#106876,#106877,#106878,#106879,#106880,
#106881,#106882,#106883,#106884,#106885,#106886,#106887,#106888,#106889,
#106890,#106891,#106892,#106893,#106894,#106895,#106896,#106897,#106898,
#106899,#106900,#106901,#106902,#106903,#106904,#106905,#106906,#106907,
#106908,#106909,#106910,#106911,#106912,#106913,#106914,#106915,#106916,
#106917,#106918,#106919,#106920,#106921,#106922,#106923,#106924,#106925,
#106926,#106927,#106928,#106929,#106930,#106931,#106932,#106933,#106934,
#106935,#106936,#106937,#106938,#106939,#106940,#106941,#106942,#106943,
#106944,#106945,#106946,#106947,#106948,#106949,#106950,#106951,#106952,
#106953,#106954,#106955,#106956,#106957,#106958,#106959,#106960,#106961,
#106962,#106963,#106964,#106965,#106966,#106967,#106968,#106969,#106970,
#106971,#106972,#106973,#106974,#106975,#106976,#106977,#106978,#106979,
#106980,#106981,#106982,#106983,#106984,#106985,#106986),.UNSPECIFIED.,
 .F.,.F.)
B_SPLINE_CURVE_WITH_KNOTS((6,1,1,1,1,1,1,1,1,1,1,1,1,1,1,1,1,1,1,1,1,1,
1,1,1,1,1,1,1,1,1,1,1,1,1,1,1,1,1,1,1,1,1,1,1,1,1,1,1,1,1,1,1,1,1,1,1,1,
1,1,1,1,1,1,1,1,1,1,1,1,1,1,1,1,1,1,1,1,1,1,1,1,1,1,1,1,1,1,1,1,1,1,1,1,
1,1,1,1,1,1,1,1,1,1,1,1,1,1,1,1,1,1,1,1,1,1,1,1,1,1,1,1,1,1,1,1,1,1,1,1,
1,1,1,1,1,1,1,1,1,1,1,1,1,1,1,1,1,1,1,1,1,1,1,1,1,1,1,1,1,1,1,1,1,1,1,1,
1,1,1,1,1,1,1,1,1,1,1,1,1,1,1,1,1,1,1,1,1,1,1,6),(0.,0.005,0.01,0.015,0.02,
0.025,0.03,0.035,0.04,0.045,0.05,0.055,0.06,0.065,0.07,0.075,0.08,0.085,
0.09,0.095,0.1,0.105,0.11,0.115,0.12,0.125,0.13,0.135,0.14,0.145,0.15,0.155,
0.16,0.165,0.17,0.175,0.18,0.185,0.19,0.195,0.2,0.205,0.21,0.215,0.22,0.225,
0.23,0.235,0.24,0.245,0.25,0.255,0.26,0.265,0.27,0.275,0.28,0.285,0.29,
0.295,0.3,0.305,0.31,0.315,0.32,0.325,0.33,0.335,0.34,0.345,0.35,0.355,
0.36,0.365,0.37,0.375,0.38,0.385,0.39,0.395,0.4,0.405,0.41,0.415,0.42,0.425,
0.43,0.435,0.44,0.445,0.45,0.455,0.46,0.465,0.47,0.475,0.48,0.485,0.49,
0.495,0.5,0.505,0.51,0.515,0.52,0.525,0.53,0.535,0.54,0.545,0.55,0.555,
0.56,0.565,0.57,0.575,0.58,0.585,0.59,0.595,0.6,0.605,0.61,0.615,0.62,0.625,
0.63,0.635,0.64,0.645,0.65,0.655,0.66,0.665,0.67,0.675,0.68,0.685,0.690000000000001,
0.695000000000001,0.700000000000001,0.705000000000001,0.710000000000001,
0.715000000000001,0.720000000000001,0.725000000000001,0.730000000000001,
0.735000000000001,0.740000000000001,0.745000000000001,0.750000000000001,
0.755000000000001,0.760000000000001,0.765000000000001,0.770000000000001,
0.775000000000001,0.780000000000001,0.785000000000001,0.790000000000001,
0.795000000000001,0.800000000000001,0.805000000000001,0.810000000000001,
0.815000000000001,0.820000000000001,0.825000000000001,0.830000000000001,
0.835000000000001,0.840000000000001,0.845000000000001,0.850000000000001,
0.855000000000001,0.860000000000001,0.865000000000001,0.870000000000001,
0.875000000000001,0.880000000000001,0.885000000000001,0.890000000000001,
0.895000000000001,0.900000000000001,0.905000000000001,0.910000000000001,
0.915000000000001,0.920000000000001,0.925000000000001,0.930000000000001,
0.935000000000001,0.940000000000001,0.941429844431252),.UNSPECIFIED.)
CURVE()
GEOMETRIC_REPRESENTATION_ITEM()
RATIONAL_B_SPLINE_CURVE((1.,1.,1.,1.,1.,1.,1.,1.,1.,1.,1.,1.,1.,1.,1.,1.,
1.,1.,1.,1.,1.,1.,1.,1.,1.,1.,1.,1.,1.,1.,1.,1.,1.,1.,1.,1.,1.,1.,1.,1.,
1.,1.,1.,1.,1.,1.,1.,1.,1.,1.,1.,1.,1.,1.,1.,1.,1.,1.,1.,1.,1.,1.,1.,1.,
1.,1.,1.,1.,1.,1.,1.,1.,1.,1.,1.,1.,1.,1.,1.,1.,1.,1.,1.,1.,1.,1.,1.,1.,
1.,1.,1.,1.,1.,1.,1.,1.,1.,1.,1.,1.,1.,1.,1.,1.,1.,1.,1.,1.,1.,1.,1.,1.,
1.,1.,1.,1.,1.,1.,1.,1.,1.,1.,1.,1.,1.,1.,1.,1.,1.,1.,1.,1.,1.,1.,1.,1.,
1.,1.,1.,1.,1.,1.,1.,1.,1.,1.,1.,1.,1.,1.,1.,1.,1.,1.,1.,1.,1.,1.,1.,1.,
1.,1.,1.,1.,1.,1.,1.,1.,1.,1.,1.,1.,1.,1.,1.,1.,1.,1.,1.,1.,1.,1.,1.,1.,
1.,1.,1.,1.,1.,1.,1.,1.,1.,1.))
REPRESENTATION_ITEM('')
);
#524=(
BOUNDED_CURVE()
B_SPLINE_CURVE(5,(#106989,#106990,#106991,#106992,#106993,#106994,#106995,
#106996,#106997,#106998,#106999,#107000,#107001,#107002,#107003,#107004,
#107005,#107006,#107007,#107008,#107009,#107010,#107011,#107012,#107013,
#107014,#107015,#107016,#107017,#107018,#107019,#107020,#107021,#107022,
#107023,#107024,#107025,#107026,#107027,#107028,#107029,#107030,#107031,
#107032,#107033,#107034,#107035,#107036,#107037,#107038,#107039,#107040,
#107041,#107042,#107043,#107044,#107045,#107046,#107047,#107048,#107049,
#107050,#107051,#107052,#107053,#107054,#107055,#107056,#107057,#107058,
#107059,#107060,#107061,#107062,#107063,#107064,#107065,#107066,#107067,
#107068,#107069,#107070,#107071,#107072,#107073,#107074,#107075,#107076,
#107077,#107078,#107079,#107080,#107081,#107082,#107083,#107084,#107085,
#107086,#107087,#107088,#107089,#107090,#107091,#107092,#107093,#107094,
#107095,#107096,#107097,#107098,#107099,#107100,#107101,#107102,#107103,
#107104,#107105,#107106,#107107,#107108,#107109,#107110,#107111,#107112,
#107113,#107114,#107115,#107116,#107117,#107118,#107119,#107120,#107121,
#107122,#107123,#107124,#107125,#107126,#107127,#107128,#107129,#107130,
#107131,#107132,#107133,#107134,#107135,#107136,#107137,#107138,#107139,
#107140,#107141,#107142,#107143,#107144,#107145,#107146,#107147,#107148,
#107149,#107150,#107151,#107152,#107153,#107154,#107155,#107156,#107157,
#107158,#107159,#107160,#107161,#107162,#107163,#107164,#107165,#107166,
#107167,#107168,#107169,#107170,#107171,#107172,#107173,#107174,#107175,
#107176,#107177,#107178,#107179,#107180,#107181,#107182),.UNSPECIFIED.,
 .F.,.F.)
B_SPLINE_CURVE_WITH_KNOTS((6,1,1,1,1,1,1,1,1,1,1,1,1,1,1,1,1,1,1,1,1,1,
1,1,1,1,1,1,1,1,1,1,1,1,1,1,1,1,1,1,1,1,1,1,1,1,1,1,1,1,1,1,1,1,1,1,1,1,
1,1,1,1,1,1,1,1,1,1,1,1,1,1,1,1,1,1,1,1,1,1,1,1,1,1,1,1,1,1,1,1,1,1,1,1,
1,1,1,1,1,1,1,1,1,1,1,1,1,1,1,1,1,1,1,1,1,1,1,1,1,1,1,1,1,1,1,1,1,1,1,1,
1,1,1,1,1,1,1,1,1,1,1,1,1,1,1,1,1,1,1,1,1,1,1,1,1,1,1,1,1,1,1,1,1,1,1,1,
1,1,1,1,1,1,1,1,1,1,1,1,1,1,1,1,1,1,1,1,1,1,1,6),(-0.94142984443125,-0.940000000000001,
-0.935000000000001,-0.930000000000001,-0.925000000000001,-0.920000000000001,
-0.915000000000001,-0.910000000000001,-0.905000000000001,-0.900000000000001,
-0.895000000000001,-0.890000000000001,-0.885000000000001,-0.880000000000001,
-0.875000000000001,-0.870000000000001,-0.865000000000001,-0.860000000000001,
-0.855000000000001,-0.850000000000001,-0.845000000000001,-0.840000000000001,
-0.835000000000001,-0.830000000000001,-0.825000000000001,-0.820000000000001,
-0.815000000000001,-0.810000000000001,-0.805000000000001,-0.800000000000001,
-0.795000000000001,-0.790000000000001,-0.785000000000001,-0.780000000000001,
-0.775000000000001,-0.770000000000001,-0.765000000000001,-0.760000000000001,
-0.755000000000001,-0.750000000000001,-0.745000000000001,-0.740000000000001,
-0.735000000000001,-0.730000000000001,-0.725000000000001,-0.720000000000001,
-0.715000000000001,-0.710000000000001,-0.705000000000001,-0.700000000000001,
-0.695000000000001,-0.690000000000001,-0.685,-0.68,-0.675,-0.67,-0.665,
-0.66,-0.655,-0.65,-0.645,-0.64,-0.635,-0.63,-0.625,-0.62,-0.615,-0.61,
-0.605,-0.6,-0.595,-0.59,-0.585,-0.58,-0.575,-0.57,-0.565,-0.56,-0.555,
-0.55,-0.545,-0.54,-0.535,-0.53,-0.525,-0.52,-0.515,-0.51,-0.505,-0.5,-0.495,
-0.49,-0.485,-0.48,-0.475,-0.47,-0.465,-0.46,-0.455,-0.45,-0.445,-0.44,
-0.435,-0.43,-0.425,-0.42,-0.415,-0.41,-0.405,-0.4,-0.395,-0.39,-0.385,
-0.38,-0.375,-0.37,-0.365,-0.36,-0.355,-0.35,-0.345,-0.34,-0.335,-0.33,
-0.325,-0.32,-0.315,-0.31,-0.305,-0.3,-0.295,-0.29,-0.285,-0.28,-0.275,
-0.27,-0.265,-0.26,-0.255,-0.25,-0.245,-0.24,-0.235,-0.23,-0.225,-0.22,
-0.215,-0.21,-0.205,-0.2,-0.195,-0.19,-0.185,-0.18,-0.175,-0.17,-0.165,
-0.16,-0.155,-0.15,-0.145,-0.14,-0.135,-0.13,-0.125,-0.12,-0.115,-0.11,
-0.105,-0.1,-0.095,-0.09,-0.085,-0.08,-0.075,-0.07,-0.065,-0.06,-0.055,
-0.05,-0.045,-0.04,-0.035,-0.03,-0.025,-0.02,-0.015,-0.01,-0.005,0.),
 .UNSPECIFIED.)
CURVE()
GEOMETRIC_REPRESENTATION_ITEM()
RATIONAL_B_SPLINE_CURVE((1.,1.,1.,1.,1.,1.,1.,1.,1.,1.,1.,1.,1.,1.,1.,1.,
1.,1.,1.,1.,1.,1.,1.,1.,1.,1.,1.,1.,1.,1.,1.,1.,1.,1.,1.,1.,1.,1.,1.,1.,
1.,1.,1.,1.,1.,1.,1.,1.,1.,1.,1.,1.,1.,1.,1.,1.,1.,1.,1.,1.,1.,1.,1.,1.,
1.,1.,1.,1.,1.,1.,1.,1.,1.,1.,1.,1.,1.,1.,1.,1.,1.,1.,1.,1.,1.,1.,1.,1.,
1.,1.,1.,1.,1.,1.,1.,1.,1.,1.,1.,1.,1.,1.,1.,1.,1.,1.,1.,1.,1.,1.,1.,1.,
1.,1.,1.,1.,1.,1.,1.,1.,1.,1.,1.,1.,1.,1.,1.,1.,1.,1.,1.,1.,1.,1.,1.,1.,
1.,1.,1.,1.,1.,1.,1.,1.,1.,1.,1.,1.,1.,1.,1.,1.,1.,1.,1.,1.,1.,1.,1.,1.,
1.,1.,1.,1.,1.,1.,1.,1.,1.,1.,1.,1.,1.,1.,1.,1.,1.,1.,1.,1.,1.,1.,1.,1.,
1.,1.,1.,1.,1.,1.,1.,1.,1.,1.))
REPRESENTATION_ITEM('')
);
#525=(
BOUNDED_CURVE()
B_SPLINE_CURVE(5,(#107689,#107690,#107691,#107692,#107693,#107694,#107695,
#107696,#107697,#107698,#107699,#107700,#107701,#107702,#107703,#107704,
#107705,#107706,#107707,#107708,#107709,#107710,#107711,#107712,#107713,
#107714,#107715,#107716,#107717,#107718,#107719,#107720,#107721,#107722,
#107723,#107724,#107725,#107726,#107727,#107728,#107729,#107730,#107731,
#107732,#107733,#107734,#107735,#107736,#107737,#107738,#107739,#107740,
#107741,#107742,#107743,#107744,#107745,#107746,#107747,#107748,#107749,
#107750,#107751,#107752,#107753,#107754,#107755,#107756,#107757,#107758,
#107759,#107760,#107761,#107762,#107763,#107764,#107765,#107766,#107767,
#107768,#107769,#107770,#107771,#107772,#107773,#107774,#107775,#107776,
#107777,#107778,#107779,#107780,#107781,#107782,#107783,#107784,#107785,
#107786,#107787,#107788,#107789,#107790,#107791,#107792,#107793,#107794,
#107795,#107796,#107797,#107798,#107799,#107800,#107801,#107802,#107803,
#107804,#107805,#107806,#107807,#107808,#107809,#107810,#107811,#107812,
#107813,#107814,#107815,#107816,#107817,#107818,#107819,#107820,#107821,
#107822,#107823,#107824,#107825,#107826,#107827,#107828,#107829,#107830,
#107831,#107832,#107833,#107834,#107835,#107836,#107837,#107838,#107839,
#107840,#107841,#107842,#107843,#107844,#107845,#107846,#107847,#107848,
#107849,#107850,#107851,#107852,#107853,#107854,#107855,#107856,#107857,
#107858,#107859,#107860,#107861,#107862,#107863,#107864,#107865,#107866,
#107867,#107868,#107869,#107870,#107871,#107872,#107873,#107874,#107875,
#107876,#107877,#107878,#107879,#107880,#107881,#107882),.UNSPECIFIED.,
 .F.,.F.)
B_SPLINE_CURVE_WITH_KNOTS((6,1,1,1,1,1,1,1,1,1,1,1,1,1,1,1,1,1,1,1,1,1,
1,1,1,1,1,1,1,1,1,1,1,1,1,1,1,1,1,1,1,1,1,1,1,1,1,1,1,1,1,1,1,1,1,1,1,1,
1,1,1,1,1,1,1,1,1,1,1,1,1,1,1,1,1,1,1,1,1,1,1,1,1,1,1,1,1,1,1,1,1,1,1,1,
1,1,1,1,1,1,1,1,1,1,1,1,1,1,1,1,1,1,1,1,1,1,1,1,1,1,1,1,1,1,1,1,1,1,1,1,
1,1,1,1,1,1,1,1,1,1,1,1,1,1,1,1,1,1,1,1,1,1,1,1,1,1,1,1,1,1,1,1,1,1,1,1,
1,1,1,1,1,1,1,1,1,1,1,1,1,1,1,1,1,1,1,1,1,1,1,6),(0.,0.005,0.01,0.015,0.02,
0.025,0.03,0.035,0.04,0.045,0.05,0.055,0.06,0.065,0.07,0.075,0.08,0.085,
0.09,0.095,0.1,0.105,0.11,0.115,0.12,0.125,0.13,0.135,0.14,0.145,0.15,0.155,
0.16,0.165,0.17,0.175,0.18,0.185,0.19,0.195,0.2,0.205,0.21,0.215,0.22,0.225,
0.23,0.235,0.24,0.245,0.25,0.255,0.26,0.265,0.27,0.275,0.28,0.285,0.29,
0.295,0.3,0.305,0.31,0.315,0.32,0.325,0.33,0.335,0.34,0.345,0.35,0.355,
0.36,0.365,0.37,0.375,0.38,0.385,0.39,0.395,0.4,0.405,0.41,0.415,0.42,0.425,
0.43,0.435,0.44,0.445,0.45,0.455,0.46,0.465,0.47,0.475,0.48,0.485,0.49,
0.495,0.5,0.505,0.51,0.515,0.52,0.525,0.53,0.535,0.54,0.545,0.55,0.555,
0.56,0.565,0.57,0.575,0.58,0.585,0.59,0.595,0.6,0.605,0.61,0.615,0.62,0.625,
0.63,0.635,0.64,0.645,0.65,0.655,0.66,0.665,0.67,0.675,0.68,0.685,0.690000000000001,
0.695000000000001,0.700000000000001,0.705000000000001,0.710000000000001,
0.715000000000001,0.720000000000001,0.725000000000001,0.730000000000001,
0.735000000000001,0.740000000000001,0.745000000000001,0.750000000000001,
0.755000000000001,0.760000000000001,0.765000000000001,0.770000000000001,
0.775000000000001,0.780000000000001,0.785000000000001,0.790000000000001,
0.795000000000001,0.800000000000001,0.805000000000001,0.810000000000001,
0.815000000000001,0.820000000000001,0.825000000000001,0.830000000000001,
0.835000000000001,0.840000000000001,0.845000000000001,0.850000000000001,
0.855000000000001,0.860000000000001,0.865000000000001,0.870000000000001,
0.875000000000001,0.880000000000001,0.885000000000001,0.890000000000001,
0.895000000000001,0.900000000000001,0.905000000000001,0.910000000000001,
0.915000000000001,0.920000000000001,0.925000000000001,0.930000000000001,
0.935000000000001,0.940000000000001,0.941429844431358),.UNSPECIFIED.)
CURVE()
GEOMETRIC_REPRESENTATION_ITEM()
RATIONAL_B_SPLINE_CURVE((1.,1.,1.,1.,1.,1.,1.,1.,1.,1.,1.,1.,1.,1.,1.,1.,
1.,1.,1.,1.,1.,1.,1.,1.,1.,1.,1.,1.,1.,1.,1.,1.,1.,1.,1.,1.,1.,1.,1.,1.,
1.,1.,1.,1.,1.,1.,1.,1.,1.,1.,1.,1.,1.,1.,1.,1.,1.,1.,1.,1.,1.,1.,1.,1.,
1.,1.,1.,1.,1.,1.,1.,1.,1.,1.,1.,1.,1.,1.,1.,1.,1.,1.,1.,1.,1.,1.,1.,1.,
1.,1.,1.,1.,1.,1.,1.,1.,1.,1.,1.,1.,1.,1.,1.,1.,1.,1.,1.,1.,1.,1.,1.,1.,
1.,1.,1.,1.,1.,1.,1.,1.,1.,1.,1.,1.,1.,1.,1.,1.,1.,1.,1.,1.,1.,1.,1.,1.,
1.,1.,1.,1.,1.,1.,1.,1.,1.,1.,1.,1.,1.,1.,1.,1.,1.,1.,1.,1.,1.,1.,1.,1.,
1.,1.,1.,1.,1.,1.,1.,1.,1.,1.,1.,1.,1.,1.,1.,1.,1.,1.,1.,1.,1.,1.,1.,1.,
1.,1.,1.,1.,1.,1.,1.,1.,1.,1.))
REPRESENTATION_ITEM('')
);
#526=(
BOUNDED_CURVE()
B_SPLINE_CURVE(5,(#107885,#107886,#107887,#107888,#107889,#107890,#107891,
#107892,#107893,#107894,#107895,#107896,#107897,#107898,#107899,#107900,
#107901,#107902,#107903,#107904,#107905,#107906,#107907,#107908,#107909,
#107910,#107911,#107912,#107913,#107914,#107915,#107916,#107917,#107918,
#107919,#107920,#107921,#107922,#107923,#107924,#107925,#107926,#107927,
#107928,#107929,#107930,#107931,#107932,#107933,#107934,#107935,#107936,
#107937,#107938,#107939,#107940,#107941,#107942,#107943,#107944,#107945,
#107946,#107947,#107948,#107949,#107950,#107951,#107952,#107953,#107954,
#107955,#107956,#107957,#107958,#107959,#107960,#107961,#107962,#107963,
#107964,#107965,#107966,#107967,#107968,#107969,#107970,#107971,#107972,
#107973,#107974,#107975,#107976,#107977,#107978,#107979,#107980,#107981,
#107982,#107983,#107984,#107985,#107986,#107987,#107988,#107989,#107990,
#107991,#107992,#107993,#107994,#107995,#107996,#107997,#107998,#107999,
#108000,#108001,#108002,#108003,#108004,#108005,#108006,#108007,#108008,
#108009,#108010,#108011,#108012,#108013,#108014,#108015,#108016,#108017,
#108018,#108019,#108020,#108021,#108022,#108023,#108024,#108025,#108026,
#108027,#108028,#108029,#108030,#108031,#108032,#108033,#108034,#108035,
#108036,#108037,#108038,#108039,#108040,#108041,#108042,#108043,#108044,
#108045,#108046,#108047,#108048,#108049,#108050,#108051,#108052,#108053,
#108054,#108055,#108056,#108057,#108058,#108059,#108060,#108061,#108062,
#108063,#108064,#108065,#108066,#108067,#108068,#108069,#108070,#108071,
#108072,#108073,#108074,#108075,#108076,#108077,#108078),.UNSPECIFIED.,
 .F.,.F.)
B_SPLINE_CURVE_WITH_KNOTS((6,1,1,1,1,1,1,1,1,1,1,1,1,1,1,1,1,1,1,1,1,1,
1,1,1,1,1,1,1,1,1,1,1,1,1,1,1,1,1,1,1,1,1,1,1,1,1,1,1,1,1,1,1,1,1,1,1,1,
1,1,1,1,1,1,1,1,1,1,1,1,1,1,1,1,1,1,1,1,1,1,1,1,1,1,1,1,1,1,1,1,1,1,1,1,
1,1,1,1,1,1,1,1,1,1,1,1,1,1,1,1,1,1,1,1,1,1,1,1,1,1,1,1,1,1,1,1,1,1,1,1,
1,1,1,1,1,1,1,1,1,1,1,1,1,1,1,1,1,1,1,1,1,1,1,1,1,1,1,1,1,1,1,1,1,1,1,1,
1,1,1,1,1,1,1,1,1,1,1,1,1,1,1,1,1,1,1,1,1,1,1,6),(-0.941429844431381,-0.940000000000001,
-0.935000000000001,-0.930000000000001,-0.925000000000001,-0.920000000000001,
-0.915000000000001,-0.910000000000001,-0.905000000000001,-0.900000000000001,
-0.895000000000001,-0.890000000000001,-0.885000000000001,-0.880000000000001,
-0.875000000000001,-0.870000000000001,-0.865000000000001,-0.860000000000001,
-0.855000000000001,-0.850000000000001,-0.845000000000001,-0.840000000000001,
-0.835000000000001,-0.830000000000001,-0.825000000000001,-0.820000000000001,
-0.815000000000001,-0.810000000000001,-0.805000000000001,-0.800000000000001,
-0.795000000000001,-0.790000000000001,-0.785000000000001,-0.780000000000001,
-0.775000000000001,-0.770000000000001,-0.765000000000001,-0.760000000000001,
-0.755000000000001,-0.750000000000001,-0.745000000000001,-0.740000000000001,
-0.735000000000001,-0.730000000000001,-0.725000000000001,-0.720000000000001,
-0.715000000000001,-0.710000000000001,-0.705000000000001,-0.700000000000001,
-0.695000000000001,-0.690000000000001,-0.685,-0.68,-0.675,-0.67,-0.665,
-0.66,-0.655,-0.65,-0.645,-0.64,-0.635,-0.63,-0.625,-0.62,-0.615,-0.61,
-0.605,-0.6,-0.595,-0.59,-0.585,-0.58,-0.575,-0.57,-0.565,-0.56,-0.555,
-0.55,-0.545,-0.54,-0.535,-0.53,-0.525,-0.52,-0.515,-0.51,-0.505,-0.5,-0.495,
-0.49,-0.485,-0.48,-0.475,-0.47,-0.465,-0.46,-0.455,-0.45,-0.445,-0.44,
-0.435,-0.43,-0.425,-0.42,-0.415,-0.41,-0.405,-0.4,-0.395,-0.39,-0.385,
-0.38,-0.375,-0.37,-0.365,-0.36,-0.355,-0.35,-0.345,-0.34,-0.335,-0.33,
-0.325,-0.32,-0.315,-0.31,-0.305,-0.3,-0.295,-0.29,-0.285,-0.28,-0.275,
-0.27,-0.265,-0.26,-0.255,-0.25,-0.245,-0.24,-0.235,-0.23,-0.225,-0.22,
-0.215,-0.21,-0.205,-0.2,-0.195,-0.19,-0.185,-0.18,-0.175,-0.17,-0.165,
-0.16,-0.155,-0.15,-0.145,-0.14,-0.135,-0.13,-0.125,-0.12,-0.115,-0.11,
-0.105,-0.1,-0.095,-0.09,-0.085,-0.08,-0.075,-0.07,-0.065,-0.06,-0.055,
-0.05,-0.045,-0.04,-0.035,-0.03,-0.025,-0.02,-0.015,-0.01,-0.005,0.),
 .UNSPECIFIED.)
CURVE()
GEOMETRIC_REPRESENTATION_ITEM()
RATIONAL_B_SPLINE_CURVE((1.,1.,1.,1.,1.,1.,1.,1.,1.,1.,1.,1.,1.,1.,1.,1.,
1.,1.,1.,1.,1.,1.,1.,1.,1.,1.,1.,1.,1.,1.,1.,1.,1.,1.,1.,1.,1.,1.,1.,1.,
1.,1.,1.,1.,1.,1.,1.,1.,1.,1.,1.,1.,1.,1.,1.,1.,1.,1.,1.,1.,1.,1.,1.,1.,
1.,1.,1.,1.,1.,1.,1.,1.,1.,1.,1.,1.,1.,1.,1.,1.,1.,1.,1.,1.,1.,1.,1.,1.,
1.,1.,1.,1.,1.,1.,1.,1.,1.,1.,1.,1.,1.,1.,1.,1.,1.,1.,1.,1.,1.,1.,1.,1.,
1.,1.,1.,1.,1.,1.,1.,1.,1.,1.,1.,1.,1.,1.,1.,1.,1.,1.,1.,1.,1.,1.,1.,1.,
1.,1.,1.,1.,1.,1.,1.,1.,1.,1.,1.,1.,1.,1.,1.,1.,1.,1.,1.,1.,1.,1.,1.,1.,
1.,1.,1.,1.,1.,1.,1.,1.,1.,1.,1.,1.,1.,1.,1.,1.,1.,1.,1.,1.,1.,1.,1.,1.,
1.,1.,1.,1.,1.,1.,1.,1.,1.,1.))
REPRESENTATION_ITEM('')
);
#527=(
BOUNDED_CURVE()
B_SPLINE_CURVE(5,(#108585,#108586,#108587,#108588,#108589,#108590,#108591,
#108592,#108593,#108594,#108595,#108596,#108597,#108598,#108599,#108600,
#108601,#108602,#108603,#108604,#108605,#108606,#108607,#108608,#108609,
#108610,#108611,#108612,#108613,#108614,#108615,#108616,#108617,#108618,
#108619,#108620,#108621,#108622,#108623,#108624,#108625,#108626,#108627,
#108628,#108629,#108630,#108631,#108632,#108633,#108634,#108635,#108636,
#108637,#108638,#108639,#108640,#108641,#108642,#108643,#108644,#108645,
#108646,#108647,#108648,#108649,#108650,#108651,#108652,#108653,#108654,
#108655,#108656,#108657,#108658,#108659,#108660,#108661,#108662,#108663,
#108664,#108665,#108666,#108667,#108668,#108669,#108670,#108671,#108672,
#108673,#108674,#108675,#108676,#108677,#108678,#108679,#108680,#108681,
#108682,#108683,#108684,#108685,#108686,#108687,#108688,#108689,#108690,
#108691,#108692,#108693,#108694,#108695,#108696,#108697,#108698,#108699,
#108700,#108701,#108702,#108703,#108704,#108705,#108706,#108707,#108708,
#108709,#108710,#108711,#108712,#108713,#108714,#108715,#108716,#108717,
#108718,#108719,#108720,#108721,#108722,#108723,#108724,#108725,#108726,
#108727,#108728,#108729,#108730,#108731,#108732,#108733,#108734,#108735,
#108736,#108737,#108738,#108739,#108740,#108741,#108742,#108743,#108744,
#108745,#108746,#108747,#108748,#108749,#108750,#108751,#108752,#108753,
#108754,#108755,#108756,#108757,#108758,#108759,#108760,#108761,#108762,
#108763,#108764,#108765,#108766,#108767,#108768,#108769,#108770,#108771,
#108772,#108773,#108774,#108775,#108776,#108777,#108778),.UNSPECIFIED.,
 .F.,.F.)
B_SPLINE_CURVE_WITH_KNOTS((6,1,1,1,1,1,1,1,1,1,1,1,1,1,1,1,1,1,1,1,1,1,
1,1,1,1,1,1,1,1,1,1,1,1,1,1,1,1,1,1,1,1,1,1,1,1,1,1,1,1,1,1,1,1,1,1,1,1,
1,1,1,1,1,1,1,1,1,1,1,1,1,1,1,1,1,1,1,1,1,1,1,1,1,1,1,1,1,1,1,1,1,1,1,1,
1,1,1,1,1,1,1,1,1,1,1,1,1,1,1,1,1,1,1,1,1,1,1,1,1,1,1,1,1,1,1,1,1,1,1,1,
1,1,1,1,1,1,1,1,1,1,1,1,1,1,1,1,1,1,1,1,1,1,1,1,1,1,1,1,1,1,1,1,1,1,1,1,
1,1,1,1,1,1,1,1,1,1,1,1,1,1,1,1,1,1,1,1,1,1,1,6),(0.,0.005,0.01,0.015,0.02,
0.025,0.03,0.035,0.04,0.045,0.05,0.055,0.06,0.065,0.07,0.075,0.08,0.085,
0.09,0.095,0.1,0.105,0.11,0.115,0.12,0.125,0.13,0.135,0.14,0.145,0.15,0.155,
0.16,0.165,0.17,0.175,0.18,0.185,0.19,0.195,0.2,0.205,0.21,0.215,0.22,0.225,
0.23,0.235,0.24,0.245,0.25,0.255,0.26,0.265,0.27,0.275,0.28,0.285,0.29,
0.295,0.3,0.305,0.31,0.315,0.32,0.325,0.33,0.335,0.34,0.345,0.35,0.355,
0.36,0.365,0.37,0.375,0.38,0.385,0.39,0.395,0.4,0.405,0.41,0.415,0.42,0.425,
0.43,0.435,0.44,0.445,0.45,0.455,0.46,0.465,0.47,0.475,0.48,0.485,0.49,
0.495,0.5,0.505,0.51,0.515,0.52,0.525,0.53,0.535,0.54,0.545,0.55,0.555,
0.56,0.565,0.57,0.575,0.58,0.585,0.59,0.595,0.6,0.605,0.61,0.615,0.62,0.625,
0.63,0.635,0.64,0.645,0.65,0.655,0.66,0.665,0.67,0.675,0.68,0.685,0.690000000000001,
0.695000000000001,0.700000000000001,0.705000000000001,0.710000000000001,
0.715000000000001,0.720000000000001,0.725000000000001,0.730000000000001,
0.735000000000001,0.740000000000001,0.745000000000001,0.750000000000001,
0.755000000000001,0.760000000000001,0.765000000000001,0.770000000000001,
0.775000000000001,0.780000000000001,0.785000000000001,0.790000000000001,
0.795000000000001,0.800000000000001,0.805000000000001,0.810000000000001,
0.815000000000001,0.820000000000001,0.825000000000001,0.830000000000001,
0.835000000000001,0.840000000000001,0.845000000000001,0.850000000000001,
0.855000000000001,0.860000000000001,0.865000000000001,0.870000000000001,
0.875000000000001,0.880000000000001,0.885000000000001,0.890000000000001,
0.895000000000001,0.900000000000001,0.905000000000001,0.910000000000001,
0.915000000000001,0.920000000000001,0.925000000000001,0.930000000000001,
0.935000000000001,0.940000000000001,0.941429844431541),.UNSPECIFIED.)
CURVE()
GEOMETRIC_REPRESENTATION_ITEM()
RATIONAL_B_SPLINE_CURVE((1.,1.,1.,1.,1.,1.,1.,1.,1.,1.,1.,1.,1.,1.,1.,1.,
1.,1.,1.,1.,1.,1.,1.,1.,1.,1.,1.,1.,1.,1.,1.,1.,1.,1.,1.,1.,1.,1.,1.,1.,
1.,1.,1.,1.,1.,1.,1.,1.,1.,1.,1.,1.,1.,1.,1.,1.,1.,1.,1.,1.,1.,1.,1.,1.,
1.,1.,1.,1.,1.,1.,1.,1.,1.,1.,1.,1.,1.,1.,1.,1.,1.,1.,1.,1.,1.,1.,1.,1.,
1.,1.,1.,1.,1.,1.,1.,1.,1.,1.,1.,1.,1.,1.,1.,1.,1.,1.,1.,1.,1.,1.,1.,1.,
1.,1.,1.,1.,1.,1.,1.,1.,1.,1.,1.,1.,1.,1.,1.,1.,1.,1.,1.,1.,1.,1.,1.,1.,
1.,1.,1.,1.,1.,1.,1.,1.,1.,1.,1.,1.,1.,1.,1.,1.,1.,1.,1.,1.,1.,1.,1.,1.,
1.,1.,1.,1.,1.,1.,1.,1.,1.,1.,1.,1.,1.,1.,1.,1.,1.,1.,1.,1.,1.,1.,1.,1.,
1.,1.,1.,1.,1.,1.,1.,1.,1.,1.))
REPRESENTATION_ITEM('')
);
#528=(
BOUNDED_CURVE()
B_SPLINE_CURVE(5,(#108781,#108782,#108783,#108784,#108785,#108786,#108787,
#108788,#108789,#108790,#108791,#108792,#108793,#108794,#108795,#108796,
#108797,#108798,#108799,#108800,#108801,#108802,#108803,#108804,#108805,
#108806,#108807,#108808,#108809,#108810,#108811,#108812,#108813,#108814,
#108815,#108816,#108817,#108818,#108819,#108820,#108821,#108822,#108823,
#108824,#108825,#108826,#108827,#108828,#108829,#108830,#108831,#108832,
#108833,#108834,#108835,#108836,#108837,#108838,#108839,#108840,#108841,
#108842,#108843,#108844,#108845,#108846,#108847,#108848,#108849,#108850,
#108851,#108852,#108853,#108854,#108855,#108856,#108857,#108858,#108859,
#108860,#108861,#108862,#108863,#108864,#108865,#108866,#108867,#108868,
#108869,#108870,#108871,#108872,#108873,#108874,#108875,#108876,#108877,
#108878,#108879,#108880,#108881,#108882,#108883,#108884,#108885,#108886,
#108887,#108888,#108889,#108890,#108891,#108892,#108893,#108894,#108895,
#108896,#108897,#108898,#108899,#108900,#108901,#108902,#108903,#108904,
#108905,#108906,#108907,#108908,#108909,#108910,#108911,#108912,#108913,
#108914,#108915,#108916,#108917,#108918,#108919,#108920,#108921,#108922,
#108923,#108924,#108925,#108926,#108927,#108928,#108929,#108930,#108931,
#108932,#108933,#108934,#108935,#108936,#108937,#108938,#108939,#108940,
#108941,#108942,#108943,#108944,#108945,#108946,#108947,#108948,#108949,
#108950,#108951,#108952,#108953,#108954,#108955,#108956,#108957,#108958,
#108959,#108960,#108961,#108962,#108963,#108964,#108965,#108966,#108967,
#108968,#108969,#108970,#108971,#108972,#108973,#108974),.UNSPECIFIED.,
 .F.,.F.)
B_SPLINE_CURVE_WITH_KNOTS((6,1,1,1,1,1,1,1,1,1,1,1,1,1,1,1,1,1,1,1,1,1,
1,1,1,1,1,1,1,1,1,1,1,1,1,1,1,1,1,1,1,1,1,1,1,1,1,1,1,1,1,1,1,1,1,1,1,1,
1,1,1,1,1,1,1,1,1,1,1,1,1,1,1,1,1,1,1,1,1,1,1,1,1,1,1,1,1,1,1,1,1,1,1,1,
1,1,1,1,1,1,1,1,1,1,1,1,1,1,1,1,1,1,1,1,1,1,1,1,1,1,1,1,1,1,1,1,1,1,1,1,
1,1,1,1,1,1,1,1,1,1,1,1,1,1,1,1,1,1,1,1,1,1,1,1,1,1,1,1,1,1,1,1,1,1,1,1,
1,1,1,1,1,1,1,1,1,1,1,1,1,1,1,1,1,1,1,1,1,1,1,6),(-0.941429844431541,-0.940000000000001,
-0.935000000000001,-0.930000000000001,-0.925000000000001,-0.920000000000001,
-0.915000000000001,-0.910000000000001,-0.905000000000001,-0.900000000000001,
-0.895000000000001,-0.890000000000001,-0.885000000000001,-0.880000000000001,
-0.875000000000001,-0.870000000000001,-0.865000000000001,-0.860000000000001,
-0.855000000000001,-0.850000000000001,-0.845000000000001,-0.840000000000001,
-0.835000000000001,-0.830000000000001,-0.825000000000001,-0.820000000000001,
-0.815000000000001,-0.810000000000001,-0.805000000000001,-0.800000000000001,
-0.795000000000001,-0.790000000000001,-0.785000000000001,-0.780000000000001,
-0.775000000000001,-0.770000000000001,-0.765000000000001,-0.760000000000001,
-0.755000000000001,-0.750000000000001,-0.745000000000001,-0.740000000000001,
-0.735000000000001,-0.730000000000001,-0.725000000000001,-0.720000000000001,
-0.715000000000001,-0.710000000000001,-0.705000000000001,-0.700000000000001,
-0.695000000000001,-0.690000000000001,-0.685,-0.68,-0.675,-0.67,-0.665,
-0.66,-0.655,-0.65,-0.645,-0.64,-0.635,-0.63,-0.625,-0.62,-0.615,-0.61,
-0.605,-0.6,-0.595,-0.59,-0.585,-0.58,-0.575,-0.57,-0.565,-0.56,-0.555,
-0.55,-0.545,-0.54,-0.535,-0.53,-0.525,-0.52,-0.515,-0.51,-0.505,-0.5,-0.495,
-0.49,-0.485,-0.48,-0.475,-0.47,-0.465,-0.46,-0.455,-0.45,-0.445,-0.44,
-0.435,-0.43,-0.425,-0.42,-0.415,-0.41,-0.405,-0.4,-0.395,-0.39,-0.385,
-0.38,-0.375,-0.37,-0.365,-0.36,-0.355,-0.35,-0.345,-0.34,-0.335,-0.33,
-0.325,-0.32,-0.315,-0.31,-0.305,-0.3,-0.295,-0.29,-0.285,-0.28,-0.275,
-0.27,-0.265,-0.26,-0.255,-0.25,-0.245,-0.24,-0.235,-0.23,-0.225,-0.22,
-0.215,-0.21,-0.205,-0.2,-0.195,-0.19,-0.185,-0.18,-0.175,-0.17,-0.165,
-0.16,-0.155,-0.15,-0.145,-0.14,-0.135,-0.13,-0.125,-0.12,-0.115,-0.11,
-0.105,-0.1,-0.095,-0.09,-0.085,-0.08,-0.075,-0.07,-0.065,-0.06,-0.055,
-0.05,-0.045,-0.04,-0.035,-0.03,-0.025,-0.02,-0.015,-0.01,-0.005,0.),
 .UNSPECIFIED.)
CURVE()
GEOMETRIC_REPRESENTATION_ITEM()
RATIONAL_B_SPLINE_CURVE((1.,1.,1.,1.,1.,1.,1.,1.,1.,1.,1.,1.,1.,1.,1.,1.,
1.,1.,1.,1.,1.,1.,1.,1.,1.,1.,1.,1.,1.,1.,1.,1.,1.,1.,1.,1.,1.,1.,1.,1.,
1.,1.,1.,1.,1.,1.,1.,1.,1.,1.,1.,1.,1.,1.,1.,1.,1.,1.,1.,1.,1.,1.,1.,1.,
1.,1.,1.,1.,1.,1.,1.,1.,1.,1.,1.,1.,1.,1.,1.,1.,1.,1.,1.,1.,1.,1.,1.,1.,
1.,1.,1.,1.,1.,1.,1.,1.,1.,1.,1.,1.,1.,1.,1.,1.,1.,1.,1.,1.,1.,1.,1.,1.,
1.,1.,1.,1.,1.,1.,1.,1.,1.,1.,1.,1.,1.,1.,1.,1.,1.,1.,1.,1.,1.,1.,1.,1.,
1.,1.,1.,1.,1.,1.,1.,1.,1.,1.,1.,1.,1.,1.,1.,1.,1.,1.,1.,1.,1.,1.,1.,1.,
1.,1.,1.,1.,1.,1.,1.,1.,1.,1.,1.,1.,1.,1.,1.,1.,1.,1.,1.,1.,1.,1.,1.,1.,
1.,1.,1.,1.,1.,1.,1.,1.,1.,1.))
REPRESENTATION_ITEM('')
);
#529=(
BOUNDED_CURVE()
B_SPLINE_CURVE(5,(#109481,#109482,#109483,#109484,#109485,#109486,#109487,
#109488,#109489,#109490,#109491,#109492,#109493,#109494,#109495,#109496,
#109497,#109498,#109499,#109500,#109501,#109502,#109503,#109504,#109505,
#109506,#109507,#109508,#109509,#109510,#109511,#109512,#109513,#109514,
#109515,#109516,#109517,#109518,#109519,#109520,#109521,#109522,#109523,
#109524,#109525,#109526,#109527,#109528,#109529,#109530,#109531,#109532,
#109533,#109534,#109535,#109536,#109537,#109538,#109539,#109540,#109541,
#109542,#109543,#109544,#109545,#109546,#109547,#109548,#109549,#109550,
#109551,#109552,#109553,#109554,#109555,#109556,#109557,#109558,#109559,
#109560,#109561,#109562,#109563,#109564,#109565,#109566,#109567,#109568,
#109569,#109570,#109571,#109572,#109573,#109574,#109575,#109576,#109577,
#109578,#109579,#109580,#109581,#109582,#109583,#109584,#109585,#109586,
#109587,#109588,#109589,#109590,#109591,#109592,#109593,#109594,#109595,
#109596,#109597,#109598,#109599,#109600,#109601,#109602,#109603,#109604,
#109605,#109606,#109607,#109608,#109609,#109610,#109611,#109612,#109613,
#109614,#109615,#109616,#109617,#109618,#109619,#109620,#109621,#109622,
#109623,#109624,#109625,#109626,#109627,#109628,#109629,#109630,#109631,
#109632,#109633,#109634,#109635,#109636,#109637,#109638,#109639,#109640,
#109641,#109642,#109643,#109644,#109645,#109646,#109647,#109648,#109649,
#109650,#109651,#109652,#109653,#109654,#109655,#109656,#109657,#109658,
#109659,#109660,#109661,#109662,#109663,#109664,#109665,#109666,#109667,
#109668,#109669,#109670,#109671,#109672,#109673,#109674),.UNSPECIFIED.,
 .F.,.F.)
B_SPLINE_CURVE_WITH_KNOTS((6,1,1,1,1,1,1,1,1,1,1,1,1,1,1,1,1,1,1,1,1,1,
1,1,1,1,1,1,1,1,1,1,1,1,1,1,1,1,1,1,1,1,1,1,1,1,1,1,1,1,1,1,1,1,1,1,1,1,
1,1,1,1,1,1,1,1,1,1,1,1,1,1,1,1,1,1,1,1,1,1,1,1,1,1,1,1,1,1,1,1,1,1,1,1,
1,1,1,1,1,1,1,1,1,1,1,1,1,1,1,1,1,1,1,1,1,1,1,1,1,1,1,1,1,1,1,1,1,1,1,1,
1,1,1,1,1,1,1,1,1,1,1,1,1,1,1,1,1,1,1,1,1,1,1,1,1,1,1,1,1,1,1,1,1,1,1,1,
1,1,1,1,1,1,1,1,1,1,1,1,1,1,1,1,1,1,1,1,1,1,1,6),(0.,0.005,0.01,0.015,0.02,
0.025,0.03,0.035,0.04,0.045,0.05,0.055,0.06,0.065,0.07,0.075,0.08,0.085,
0.09,0.095,0.1,0.105,0.11,0.115,0.12,0.125,0.13,0.135,0.14,0.145,0.15,0.155,
0.16,0.165,0.17,0.175,0.18,0.185,0.19,0.195,0.2,0.205,0.21,0.215,0.22,0.225,
0.23,0.235,0.24,0.245,0.25,0.255,0.26,0.265,0.27,0.275,0.28,0.285,0.29,
0.295,0.3,0.305,0.31,0.315,0.32,0.325,0.33,0.335,0.34,0.345,0.35,0.355,
0.36,0.365,0.37,0.375,0.38,0.385,0.39,0.395,0.4,0.405,0.41,0.415,0.42,0.425,
0.43,0.435,0.44,0.445,0.45,0.455,0.46,0.465,0.47,0.475,0.48,0.485,0.49,
0.495,0.5,0.505,0.51,0.515,0.52,0.525,0.53,0.535,0.54,0.545,0.55,0.555,
0.56,0.565,0.57,0.575,0.58,0.585,0.59,0.595,0.6,0.605,0.61,0.615,0.62,0.625,
0.63,0.635,0.64,0.645,0.65,0.655,0.66,0.665,0.67,0.675,0.68,0.685,0.690000000000001,
0.695000000000001,0.700000000000001,0.705000000000001,0.710000000000001,
0.715000000000001,0.720000000000001,0.725000000000001,0.730000000000001,
0.735000000000001,0.740000000000001,0.745000000000001,0.750000000000001,
0.755000000000001,0.760000000000001,0.765000000000001,0.770000000000001,
0.775000000000001,0.780000000000001,0.785000000000001,0.790000000000001,
0.795000000000001,0.800000000000001,0.805000000000001,0.810000000000001,
0.815000000000001,0.820000000000001,0.825000000000001,0.830000000000001,
0.835000000000001,0.840000000000001,0.845000000000001,0.850000000000001,
0.855000000000001,0.860000000000001,0.865000000000001,0.870000000000001,
0.875000000000001,0.880000000000001,0.885000000000001,0.890000000000001,
0.895000000000001,0.900000000000001,0.905000000000001,0.910000000000001,
0.915000000000001,0.920000000000001,0.925000000000001,0.930000000000001,
0.935000000000001,0.940000000000001,0.941429844431311),.UNSPECIFIED.)
CURVE()
GEOMETRIC_REPRESENTATION_ITEM()
RATIONAL_B_SPLINE_CURVE((1.,1.,1.,1.,1.,1.,1.,1.,1.,1.,1.,1.,1.,1.,1.,1.,
1.,1.,1.,1.,1.,1.,1.,1.,1.,1.,1.,1.,1.,1.,1.,1.,1.,1.,1.,1.,1.,1.,1.,1.,
1.,1.,1.,1.,1.,1.,1.,1.,1.,1.,1.,1.,1.,1.,1.,1.,1.,1.,1.,1.,1.,1.,1.,1.,
1.,1.,1.,1.,1.,1.,1.,1.,1.,1.,1.,1.,1.,1.,1.,1.,1.,1.,1.,1.,1.,1.,1.,1.,
1.,1.,1.,1.,1.,1.,1.,1.,1.,1.,1.,1.,1.,1.,1.,1.,1.,1.,1.,1.,1.,1.,1.,1.,
1.,1.,1.,1.,1.,1.,1.,1.,1.,1.,1.,1.,1.,1.,1.,1.,1.,1.,1.,1.,1.,1.,1.,1.,
1.,1.,1.,1.,1.,1.,1.,1.,1.,1.,1.,1.,1.,1.,1.,1.,1.,1.,1.,1.,1.,1.,1.,1.,
1.,1.,1.,1.,1.,1.,1.,1.,1.,1.,1.,1.,1.,1.,1.,1.,1.,1.,1.,1.,1.,1.,1.,1.,
1.,1.,1.,1.,1.,1.,1.,1.,1.,1.))
REPRESENTATION_ITEM('')
);
#530=(
BOUNDED_CURVE()
B_SPLINE_CURVE(5,(#109677,#109678,#109679,#109680,#109681,#109682,#109683,
#109684,#109685,#109686,#109687,#109688,#109689,#109690,#109691,#109692,
#109693,#109694,#109695,#109696,#109697,#109698,#109699,#109700,#109701,
#109702,#109703,#109704,#109705,#109706,#109707,#109708,#109709,#109710,
#109711,#109712,#109713,#109714,#109715,#109716,#109717,#109718,#109719,
#109720,#109721,#109722,#109723,#109724,#109725,#109726,#109727,#109728,
#109729,#109730,#109731,#109732,#109733,#109734,#109735,#109736,#109737,
#109738,#109739,#109740,#109741,#109742,#109743,#109744,#109745,#109746,
#109747,#109748,#109749,#109750,#109751,#109752,#109753,#109754,#109755,
#109756,#109757,#109758,#109759,#109760,#109761,#109762,#109763,#109764,
#109765,#109766,#109767,#109768,#109769,#109770,#109771,#109772,#109773,
#109774,#109775,#109776,#109777,#109778,#109779,#109780,#109781,#109782,
#109783,#109784,#109785,#109786,#109787,#109788,#109789,#109790,#109791,
#109792,#109793,#109794,#109795,#109796,#109797,#109798,#109799,#109800,
#109801,#109802,#109803,#109804,#109805,#109806,#109807,#109808,#109809,
#109810,#109811,#109812,#109813,#109814,#109815,#109816,#109817,#109818,
#109819,#109820,#109821,#109822,#109823,#109824,#109825,#109826,#109827,
#109828,#109829,#109830,#109831,#109832,#109833,#109834,#109835,#109836,
#109837,#109838,#109839,#109840,#109841,#109842,#109843,#109844,#109845,
#109846,#109847,#109848,#109849,#109850,#109851,#109852,#109853,#109854,
#109855,#109856,#109857,#109858,#109859,#109860,#109861,#109862,#109863,
#109864,#109865,#109866,#109867,#109868,#109869,#109870),.UNSPECIFIED.,
 .F.,.F.)
B_SPLINE_CURVE_WITH_KNOTS((6,1,1,1,1,1,1,1,1,1,1,1,1,1,1,1,1,1,1,1,1,1,
1,1,1,1,1,1,1,1,1,1,1,1,1,1,1,1,1,1,1,1,1,1,1,1,1,1,1,1,1,1,1,1,1,1,1,1,
1,1,1,1,1,1,1,1,1,1,1,1,1,1,1,1,1,1,1,1,1,1,1,1,1,1,1,1,1,1,1,1,1,1,1,1,
1,1,1,1,1,1,1,1,1,1,1,1,1,1,1,1,1,1,1,1,1,1,1,1,1,1,1,1,1,1,1,1,1,1,1,1,
1,1,1,1,1,1,1,1,1,1,1,1,1,1,1,1,1,1,1,1,1,1,1,1,1,1,1,1,1,1,1,1,1,1,1,1,
1,1,1,1,1,1,1,1,1,1,1,1,1,1,1,1,1,1,1,1,1,1,1,6),(-0.941429844431311,-0.940000000000001,
-0.935000000000001,-0.930000000000001,-0.925000000000001,-0.920000000000001,
-0.915000000000001,-0.910000000000001,-0.905000000000001,-0.900000000000001,
-0.895000000000001,-0.890000000000001,-0.885000000000001,-0.880000000000001,
-0.875000000000001,-0.870000000000001,-0.865000000000001,-0.860000000000001,
-0.855000000000001,-0.850000000000001,-0.845000000000001,-0.840000000000001,
-0.835000000000001,-0.830000000000001,-0.825000000000001,-0.820000000000001,
-0.815000000000001,-0.810000000000001,-0.805000000000001,-0.800000000000001,
-0.795000000000001,-0.790000000000001,-0.785000000000001,-0.780000000000001,
-0.775000000000001,-0.770000000000001,-0.765000000000001,-0.760000000000001,
-0.755000000000001,-0.750000000000001,-0.745000000000001,-0.740000000000001,
-0.735000000000001,-0.730000000000001,-0.725000000000001,-0.720000000000001,
-0.715000000000001,-0.710000000000001,-0.705000000000001,-0.700000000000001,
-0.695000000000001,-0.690000000000001,-0.685,-0.68,-0.675,-0.67,-0.665,
-0.66,-0.655,-0.65,-0.645,-0.64,-0.635,-0.63,-0.625,-0.62,-0.615,-0.61,
-0.605,-0.6,-0.595,-0.59,-0.585,-0.58,-0.575,-0.57,-0.565,-0.56,-0.555,
-0.55,-0.545,-0.54,-0.535,-0.53,-0.525,-0.52,-0.515,-0.51,-0.505,-0.5,-0.495,
-0.49,-0.485,-0.48,-0.475,-0.47,-0.465,-0.46,-0.455,-0.45,-0.445,-0.44,
-0.435,-0.43,-0.425,-0.42,-0.415,-0.41,-0.405,-0.4,-0.395,-0.39,-0.385,
-0.38,-0.375,-0.37,-0.365,-0.36,-0.355,-0.35,-0.345,-0.34,-0.335,-0.33,
-0.325,-0.32,-0.315,-0.31,-0.305,-0.3,-0.295,-0.29,-0.285,-0.28,-0.275,
-0.27,-0.265,-0.26,-0.255,-0.25,-0.245,-0.24,-0.235,-0.23,-0.225,-0.22,
-0.215,-0.21,-0.205,-0.2,-0.195,-0.19,-0.185,-0.18,-0.175,-0.17,-0.165,
-0.16,-0.155,-0.15,-0.145,-0.14,-0.135,-0.13,-0.125,-0.12,-0.115,-0.11,
-0.105,-0.1,-0.095,-0.09,-0.085,-0.08,-0.075,-0.07,-0.065,-0.06,-0.055,
-0.05,-0.045,-0.04,-0.035,-0.03,-0.025,-0.02,-0.015,-0.01,-0.005,0.),
 .UNSPECIFIED.)
CURVE()
GEOMETRIC_REPRESENTATION_ITEM()
RATIONAL_B_SPLINE_CURVE((1.,1.,1.,1.,1.,1.,1.,1.,1.,1.,1.,1.,1.,1.,1.,1.,
1.,1.,1.,1.,1.,1.,1.,1.,1.,1.,1.,1.,1.,1.,1.,1.,1.,1.,1.,1.,1.,1.,1.,1.,
1.,1.,1.,1.,1.,1.,1.,1.,1.,1.,1.,1.,1.,1.,1.,1.,1.,1.,1.,1.,1.,1.,1.,1.,
1.,1.,1.,1.,1.,1.,1.,1.,1.,1.,1.,1.,1.,1.,1.,1.,1.,1.,1.,1.,1.,1.,1.,1.,
1.,1.,1.,1.,1.,1.,1.,1.,1.,1.,1.,1.,1.,1.,1.,1.,1.,1.,1.,1.,1.,1.,1.,1.,
1.,1.,1.,1.,1.,1.,1.,1.,1.,1.,1.,1.,1.,1.,1.,1.,1.,1.,1.,1.,1.,1.,1.,1.,
1.,1.,1.,1.,1.,1.,1.,1.,1.,1.,1.,1.,1.,1.,1.,1.,1.,1.,1.,1.,1.,1.,1.,1.,
1.,1.,1.,1.,1.,1.,1.,1.,1.,1.,1.,1.,1.,1.,1.,1.,1.,1.,1.,1.,1.,1.,1.,1.,
1.,1.,1.,1.,1.,1.,1.,1.,1.,1.))
REPRESENTATION_ITEM('')
);
#531=(
BOUNDED_CURVE()
B_SPLINE_CURVE(5,(#110377,#110378,#110379,#110380,#110381,#110382,#110383,
#110384,#110385,#110386,#110387,#110388,#110389,#110390,#110391,#110392,
#110393,#110394,#110395,#110396,#110397,#110398,#110399,#110400,#110401,
#110402,#110403,#110404,#110405,#110406,#110407,#110408,#110409,#110410,
#110411,#110412,#110413,#110414,#110415,#110416,#110417,#110418,#110419,
#110420,#110421,#110422,#110423,#110424,#110425,#110426,#110427,#110428,
#110429,#110430,#110431,#110432,#110433,#110434,#110435,#110436,#110437,
#110438,#110439,#110440,#110441,#110442,#110443,#110444,#110445,#110446,
#110447,#110448,#110449,#110450,#110451,#110452,#110453,#110454,#110455,
#110456,#110457,#110458,#110459,#110460,#110461,#110462,#110463,#110464,
#110465,#110466,#110467,#110468,#110469,#110470,#110471,#110472,#110473,
#110474,#110475,#110476,#110477,#110478,#110479,#110480,#110481,#110482,
#110483,#110484,#110485,#110486,#110487,#110488,#110489,#110490,#110491,
#110492,#110493,#110494,#110495,#110496,#110497,#110498,#110499,#110500,
#110501,#110502,#110503,#110504,#110505,#110506,#110507,#110508,#110509,
#110510,#110511,#110512,#110513,#110514,#110515,#110516,#110517,#110518,
#110519,#110520,#110521,#110522,#110523,#110524,#110525,#110526,#110527,
#110528,#110529,#110530,#110531,#110532,#110533,#110534,#110535,#110536,
#110537,#110538,#110539,#110540,#110541,#110542,#110543,#110544,#110545,
#110546,#110547,#110548,#110549,#110550,#110551,#110552,#110553,#110554,
#110555,#110556,#110557,#110558,#110559,#110560,#110561,#110562,#110563,
#110564,#110565,#110566,#110567,#110568,#110569,#110570),.UNSPECIFIED.,
 .F.,.F.)
B_SPLINE_CURVE_WITH_KNOTS((6,1,1,1,1,1,1,1,1,1,1,1,1,1,1,1,1,1,1,1,1,1,
1,1,1,1,1,1,1,1,1,1,1,1,1,1,1,1,1,1,1,1,1,1,1,1,1,1,1,1,1,1,1,1,1,1,1,1,
1,1,1,1,1,1,1,1,1,1,1,1,1,1,1,1,1,1,1,1,1,1,1,1,1,1,1,1,1,1,1,1,1,1,1,1,
1,1,1,1,1,1,1,1,1,1,1,1,1,1,1,1,1,1,1,1,1,1,1,1,1,1,1,1,1,1,1,1,1,1,1,1,
1,1,1,1,1,1,1,1,1,1,1,1,1,1,1,1,1,1,1,1,1,1,1,1,1,1,1,1,1,1,1,1,1,1,1,1,
1,1,1,1,1,1,1,1,1,1,1,1,1,1,1,1,1,1,1,1,1,1,1,6),(0.,0.005,0.01,0.015,0.02,
0.025,0.03,0.035,0.04,0.045,0.05,0.055,0.06,0.065,0.07,0.075,0.08,0.085,
0.09,0.095,0.1,0.105,0.11,0.115,0.12,0.125,0.13,0.135,0.14,0.145,0.15,0.155,
0.16,0.165,0.17,0.175,0.18,0.185,0.19,0.195,0.2,0.205,0.21,0.215,0.22,0.225,
0.23,0.235,0.24,0.245,0.25,0.255,0.26,0.265,0.27,0.275,0.28,0.285,0.29,
0.295,0.3,0.305,0.31,0.315,0.32,0.325,0.33,0.335,0.34,0.345,0.35,0.355,
0.36,0.365,0.37,0.375,0.38,0.385,0.39,0.395,0.4,0.405,0.41,0.415,0.42,0.425,
0.43,0.435,0.44,0.445,0.45,0.455,0.46,0.465,0.47,0.475,0.48,0.485,0.49,
0.495,0.5,0.505,0.51,0.515,0.52,0.525,0.53,0.535,0.54,0.545,0.55,0.555,
0.56,0.565,0.57,0.575,0.58,0.585,0.59,0.595,0.6,0.605,0.61,0.615,0.62,0.625,
0.63,0.635,0.64,0.645,0.65,0.655,0.66,0.665,0.67,0.675,0.68,0.685,0.690000000000001,
0.695000000000001,0.700000000000001,0.705000000000001,0.710000000000001,
0.715000000000001,0.720000000000001,0.725000000000001,0.730000000000001,
0.735000000000001,0.740000000000001,0.745000000000001,0.750000000000001,
0.755000000000001,0.760000000000001,0.765000000000001,0.770000000000001,
0.775000000000001,0.780000000000001,0.785000000000001,0.790000000000001,
0.795000000000001,0.800000000000001,0.805000000000001,0.810000000000001,
0.815000000000001,0.820000000000001,0.825000000000001,0.830000000000001,
0.835000000000001,0.840000000000001,0.845000000000001,0.850000000000001,
0.855000000000001,0.860000000000001,0.865000000000001,0.870000000000001,
0.875000000000001,0.880000000000001,0.885000000000001,0.890000000000001,
0.895000000000001,0.900000000000001,0.905000000000001,0.910000000000001,
0.915000000000001,0.920000000000001,0.925000000000001,0.930000000000001,
0.935000000000001,0.940000000000001,0.941429844431297),.UNSPECIFIED.)
CURVE()
GEOMETRIC_REPRESENTATION_ITEM()
RATIONAL_B_SPLINE_CURVE((1.,1.,1.,1.,1.,1.,1.,1.,1.,1.,1.,1.,1.,1.,1.,1.,
1.,1.,1.,1.,1.,1.,1.,1.,1.,1.,1.,1.,1.,1.,1.,1.,1.,1.,1.,1.,1.,1.,1.,1.,
1.,1.,1.,1.,1.,1.,1.,1.,1.,1.,1.,1.,1.,1.,1.,1.,1.,1.,1.,1.,1.,1.,1.,1.,
1.,1.,1.,1.,1.,1.,1.,1.,1.,1.,1.,1.,1.,1.,1.,1.,1.,1.,1.,1.,1.,1.,1.,1.,
1.,1.,1.,1.,1.,1.,1.,1.,1.,1.,1.,1.,1.,1.,1.,1.,1.,1.,1.,1.,1.,1.,1.,1.,
1.,1.,1.,1.,1.,1.,1.,1.,1.,1.,1.,1.,1.,1.,1.,1.,1.,1.,1.,1.,1.,1.,1.,1.,
1.,1.,1.,1.,1.,1.,1.,1.,1.,1.,1.,1.,1.,1.,1.,1.,1.,1.,1.,1.,1.,1.,1.,1.,
1.,1.,1.,1.,1.,1.,1.,1.,1.,1.,1.,1.,1.,1.,1.,1.,1.,1.,1.,1.,1.,1.,1.,1.,
1.,1.,1.,1.,1.,1.,1.,1.,1.,1.))
REPRESENTATION_ITEM('')
);
#532=(
BOUNDED_CURVE()
B_SPLINE_CURVE(5,(#110573,#110574,#110575,#110576,#110577,#110578,#110579,
#110580,#110581,#110582,#110583,#110584,#110585,#110586,#110587,#110588,
#110589,#110590,#110591,#110592,#110593,#110594,#110595,#110596,#110597,
#110598,#110599,#110600,#110601,#110602,#110603,#110604,#110605,#110606,
#110607,#110608,#110609,#110610,#110611,#110612,#110613,#110614,#110615,
#110616,#110617,#110618,#110619,#110620,#110621,#110622,#110623,#110624,
#110625,#110626,#110627,#110628,#110629,#110630,#110631,#110632,#110633,
#110634,#110635,#110636,#110637,#110638,#110639,#110640,#110641,#110642,
#110643,#110644,#110645,#110646,#110647,#110648,#110649,#110650,#110651,
#110652,#110653,#110654,#110655,#110656,#110657,#110658,#110659,#110660,
#110661,#110662,#110663,#110664,#110665,#110666,#110667,#110668,#110669,
#110670,#110671,#110672,#110673,#110674,#110675,#110676,#110677,#110678,
#110679,#110680,#110681,#110682,#110683,#110684,#110685,#110686,#110687,
#110688,#110689,#110690,#110691,#110692,#110693,#110694,#110695,#110696,
#110697,#110698,#110699,#110700,#110701,#110702,#110703,#110704,#110705,
#110706,#110707,#110708,#110709,#110710,#110711,#110712,#110713,#110714,
#110715,#110716,#110717,#110718,#110719,#110720,#110721,#110722,#110723,
#110724,#110725,#110726,#110727,#110728,#110729,#110730,#110731,#110732,
#110733,#110734,#110735,#110736,#110737,#110738,#110739,#110740,#110741,
#110742,#110743,#110744,#110745,#110746,#110747,#110748,#110749,#110750,
#110751,#110752,#110753,#110754,#110755,#110756,#110757,#110758,#110759,
#110760,#110761,#110762,#110763,#110764,#110765,#110766),.UNSPECIFIED.,
 .F.,.F.)
B_SPLINE_CURVE_WITH_KNOTS((6,1,1,1,1,1,1,1,1,1,1,1,1,1,1,1,1,1,1,1,1,1,
1,1,1,1,1,1,1,1,1,1,1,1,1,1,1,1,1,1,1,1,1,1,1,1,1,1,1,1,1,1,1,1,1,1,1,1,
1,1,1,1,1,1,1,1,1,1,1,1,1,1,1,1,1,1,1,1,1,1,1,1,1,1,1,1,1,1,1,1,1,1,1,1,
1,1,1,1,1,1,1,1,1,1,1,1,1,1,1,1,1,1,1,1,1,1,1,1,1,1,1,1,1,1,1,1,1,1,1,1,
1,1,1,1,1,1,1,1,1,1,1,1,1,1,1,1,1,1,1,1,1,1,1,1,1,1,1,1,1,1,1,1,1,1,1,1,
1,1,1,1,1,1,1,1,1,1,1,1,1,1,1,1,1,1,1,1,1,1,1,6),(-0.941429844431289,-0.940000000000001,
-0.935000000000001,-0.930000000000001,-0.925000000000001,-0.920000000000001,
-0.915000000000001,-0.910000000000001,-0.905000000000001,-0.900000000000001,
-0.895000000000001,-0.890000000000001,-0.885000000000001,-0.880000000000001,
-0.875000000000001,-0.870000000000001,-0.865000000000001,-0.860000000000001,
-0.855000000000001,-0.850000000000001,-0.845000000000001,-0.840000000000001,
-0.835000000000001,-0.830000000000001,-0.825000000000001,-0.820000000000001,
-0.815000000000001,-0.810000000000001,-0.805000000000001,-0.800000000000001,
-0.795000000000001,-0.790000000000001,-0.785000000000001,-0.780000000000001,
-0.775000000000001,-0.770000000000001,-0.765000000000001,-0.760000000000001,
-0.755000000000001,-0.750000000000001,-0.745000000000001,-0.740000000000001,
-0.735000000000001,-0.730000000000001,-0.725000000000001,-0.720000000000001,
-0.715000000000001,-0.710000000000001,-0.705000000000001,-0.700000000000001,
-0.695000000000001,-0.690000000000001,-0.685,-0.68,-0.675,-0.67,-0.665,
-0.66,-0.655,-0.65,-0.645,-0.64,-0.635,-0.63,-0.625,-0.62,-0.615,-0.61,
-0.605,-0.6,-0.595,-0.59,-0.585,-0.58,-0.575,-0.57,-0.565,-0.56,-0.555,
-0.55,-0.545,-0.54,-0.535,-0.53,-0.525,-0.52,-0.515,-0.51,-0.505,-0.5,-0.495,
-0.49,-0.485,-0.48,-0.475,-0.47,-0.465,-0.46,-0.455,-0.45,-0.445,-0.44,
-0.435,-0.43,-0.425,-0.42,-0.415,-0.41,-0.405,-0.4,-0.395,-0.39,-0.385,
-0.38,-0.375,-0.37,-0.365,-0.36,-0.355,-0.35,-0.345,-0.34,-0.335,-0.33,
-0.325,-0.32,-0.315,-0.31,-0.305,-0.3,-0.295,-0.29,-0.285,-0.28,-0.275,
-0.27,-0.265,-0.26,-0.255,-0.25,-0.245,-0.24,-0.235,-0.23,-0.225,-0.22,
-0.215,-0.21,-0.205,-0.2,-0.195,-0.19,-0.185,-0.18,-0.175,-0.17,-0.165,
-0.16,-0.155,-0.15,-0.145,-0.14,-0.135,-0.13,-0.125,-0.12,-0.115,-0.11,
-0.105,-0.1,-0.095,-0.09,-0.085,-0.08,-0.075,-0.07,-0.065,-0.06,-0.055,
-0.05,-0.045,-0.04,-0.035,-0.03,-0.025,-0.02,-0.015,-0.01,-0.005,0.),
 .UNSPECIFIED.)
CURVE()
GEOMETRIC_REPRESENTATION_ITEM()
RATIONAL_B_SPLINE_CURVE((1.,1.,1.,1.,1.,1.,1.,1.,1.,1.,1.,1.,1.,1.,1.,1.,
1.,1.,1.,1.,1.,1.,1.,1.,1.,1.,1.,1.,1.,1.,1.,1.,1.,1.,1.,1.,1.,1.,1.,1.,
1.,1.,1.,1.,1.,1.,1.,1.,1.,1.,1.,1.,1.,1.,1.,1.,1.,1.,1.,1.,1.,1.,1.,1.,
1.,1.,1.,1.,1.,1.,1.,1.,1.,1.,1.,1.,1.,1.,1.,1.,1.,1.,1.,1.,1.,1.,1.,1.,
1.,1.,1.,1.,1.,1.,1.,1.,1.,1.,1.,1.,1.,1.,1.,1.,1.,1.,1.,1.,1.,1.,1.,1.,
1.,1.,1.,1.,1.,1.,1.,1.,1.,1.,1.,1.,1.,1.,1.,1.,1.,1.,1.,1.,1.,1.,1.,1.,
1.,1.,1.,1.,1.,1.,1.,1.,1.,1.,1.,1.,1.,1.,1.,1.,1.,1.,1.,1.,1.,1.,1.,1.,
1.,1.,1.,1.,1.,1.,1.,1.,1.,1.,1.,1.,1.,1.,1.,1.,1.,1.,1.,1.,1.,1.,1.,1.,
1.,1.,1.,1.,1.,1.,1.,1.,1.,1.))
REPRESENTATION_ITEM('')
);
#533=(
BOUNDED_CURVE()
B_SPLINE_CURVE(5,(#111273,#111274,#111275,#111276,#111277,#111278,#111279,
#111280,#111281,#111282,#111283,#111284,#111285,#111286,#111287,#111288,
#111289,#111290,#111291,#111292,#111293,#111294,#111295,#111296,#111297,
#111298,#111299,#111300,#111301,#111302,#111303,#111304,#111305,#111306,
#111307,#111308,#111309,#111310,#111311,#111312,#111313,#111314,#111315,
#111316,#111317,#111318,#111319,#111320,#111321,#111322,#111323,#111324,
#111325,#111326,#111327,#111328,#111329,#111330,#111331,#111332,#111333,
#111334,#111335,#111336,#111337,#111338,#111339,#111340,#111341,#111342,
#111343,#111344,#111345,#111346,#111347,#111348,#111349,#111350,#111351,
#111352,#111353,#111354,#111355,#111356,#111357,#111358,#111359,#111360,
#111361,#111362,#111363,#111364,#111365,#111366,#111367,#111368,#111369,
#111370,#111371,#111372,#111373,#111374,#111375,#111376,#111377,#111378,
#111379,#111380,#111381,#111382,#111383,#111384,#111385,#111386,#111387,
#111388,#111389,#111390,#111391,#111392,#111393,#111394,#111395,#111396,
#111397,#111398,#111399,#111400,#111401,#111402,#111403,#111404,#111405,
#111406,#111407,#111408,#111409,#111410,#111411,#111412,#111413,#111414,
#111415,#111416,#111417,#111418,#111419,#111420,#111421,#111422,#111423,
#111424,#111425,#111426,#111427,#111428,#111429,#111430,#111431,#111432,
#111433,#111434,#111435,#111436,#111437,#111438,#111439,#111440,#111441,
#111442,#111443,#111444,#111445,#111446,#111447,#111448,#111449,#111450,
#111451,#111452,#111453,#111454,#111455,#111456,#111457,#111458,#111459,
#111460,#111461,#111462,#111463,#111464,#111465,#111466),.UNSPECIFIED.,
 .F.,.F.)
B_SPLINE_CURVE_WITH_KNOTS((6,1,1,1,1,1,1,1,1,1,1,1,1,1,1,1,1,1,1,1,1,1,
1,1,1,1,1,1,1,1,1,1,1,1,1,1,1,1,1,1,1,1,1,1,1,1,1,1,1,1,1,1,1,1,1,1,1,1,
1,1,1,1,1,1,1,1,1,1,1,1,1,1,1,1,1,1,1,1,1,1,1,1,1,1,1,1,1,1,1,1,1,1,1,1,
1,1,1,1,1,1,1,1,1,1,1,1,1,1,1,1,1,1,1,1,1,1,1,1,1,1,1,1,1,1,1,1,1,1,1,1,
1,1,1,1,1,1,1,1,1,1,1,1,1,1,1,1,1,1,1,1,1,1,1,1,1,1,1,1,1,1,1,1,1,1,1,1,
1,1,1,1,1,1,1,1,1,1,1,1,1,1,1,1,1,1,1,1,1,1,1,6),(0.,0.005,0.01,0.015,0.02,
0.025,0.03,0.035,0.04,0.045,0.05,0.055,0.06,0.065,0.07,0.075,0.08,0.085,
0.09,0.095,0.1,0.105,0.11,0.115,0.12,0.125,0.13,0.135,0.14,0.145,0.15,0.155,
0.16,0.165,0.17,0.175,0.18,0.185,0.19,0.195,0.2,0.205,0.21,0.215,0.22,0.225,
0.23,0.235,0.24,0.245,0.25,0.255,0.26,0.265,0.27,0.275,0.28,0.285,0.29,
0.295,0.3,0.305,0.31,0.315,0.32,0.325,0.33,0.335,0.34,0.345,0.35,0.355,
0.36,0.365,0.37,0.375,0.38,0.385,0.39,0.395,0.4,0.405,0.41,0.415,0.42,0.425,
0.43,0.435,0.44,0.445,0.45,0.455,0.46,0.465,0.47,0.475,0.48,0.485,0.49,
0.495,0.5,0.505,0.51,0.515,0.52,0.525,0.53,0.535,0.54,0.545,0.55,0.555,
0.56,0.565,0.57,0.575,0.58,0.585,0.59,0.595,0.6,0.605,0.61,0.615,0.62,0.625,
0.63,0.635,0.64,0.645,0.65,0.655,0.66,0.665,0.67,0.675,0.68,0.685,0.690000000000001,
0.695000000000001,0.700000000000001,0.705000000000001,0.710000000000001,
0.715000000000001,0.720000000000001,0.725000000000001,0.730000000000001,
0.735000000000001,0.740000000000001,0.745000000000001,0.750000000000001,
0.755000000000001,0.760000000000001,0.765000000000001,0.770000000000001,
0.775000000000001,0.780000000000001,0.785000000000001,0.790000000000001,
0.795000000000001,0.800000000000001,0.805000000000001,0.810000000000001,
0.815000000000001,0.820000000000001,0.825000000000001,0.830000000000001,
0.835000000000001,0.840000000000001,0.845000000000001,0.850000000000001,
0.855000000000001,0.860000000000001,0.865000000000001,0.870000000000001,
0.875000000000001,0.880000000000001,0.885000000000001,0.890000000000001,
0.895000000000001,0.900000000000001,0.905000000000001,0.910000000000001,
0.915000000000001,0.920000000000001,0.925000000000001,0.930000000000001,
0.935000000000001,0.940000000000001,0.941429844431415),.UNSPECIFIED.)
CURVE()
GEOMETRIC_REPRESENTATION_ITEM()
RATIONAL_B_SPLINE_CURVE((1.,1.,1.,1.,1.,1.,1.,1.,1.,1.,1.,1.,1.,1.,1.,1.,
1.,1.,1.,1.,1.,1.,1.,1.,1.,1.,1.,1.,1.,1.,1.,1.,1.,1.,1.,1.,1.,1.,1.,1.,
1.,1.,1.,1.,1.,1.,1.,1.,1.,1.,1.,1.,1.,1.,1.,1.,1.,1.,1.,1.,1.,1.,1.,1.,
1.,1.,1.,1.,1.,1.,1.,1.,1.,1.,1.,1.,1.,1.,1.,1.,1.,1.,1.,1.,1.,1.,1.,1.,
1.,1.,1.,1.,1.,1.,1.,1.,1.,1.,1.,1.,1.,1.,1.,1.,1.,1.,1.,1.,1.,1.,1.,1.,
1.,1.,1.,1.,1.,1.,1.,1.,1.,1.,1.,1.,1.,1.,1.,1.,1.,1.,1.,1.,1.,1.,1.,1.,
1.,1.,1.,1.,1.,1.,1.,1.,1.,1.,1.,1.,1.,1.,1.,1.,1.,1.,1.,1.,1.,1.,1.,1.,
1.,1.,1.,1.,1.,1.,1.,1.,1.,1.,1.,1.,1.,1.,1.,1.,1.,1.,1.,1.,1.,1.,1.,1.,
1.,1.,1.,1.,1.,1.,1.,1.,1.,1.))
REPRESENTATION_ITEM('')
);
#534=(
BOUNDED_CURVE()
B_SPLINE_CURVE(5,(#111469,#111470,#111471,#111472,#111473,#111474,#111475,
#111476,#111477,#111478,#111479,#111480,#111481,#111482,#111483,#111484,
#111485,#111486,#111487,#111488,#111489,#111490,#111491,#111492,#111493,
#111494,#111495,#111496,#111497,#111498,#111499,#111500,#111501,#111502,
#111503,#111504,#111505,#111506,#111507,#111508,#111509,#111510,#111511,
#111512,#111513,#111514,#111515,#111516,#111517,#111518,#111519,#111520,
#111521,#111522,#111523,#111524,#111525,#111526,#111527,#111528,#111529,
#111530,#111531,#111532,#111533,#111534,#111535,#111536,#111537,#111538,
#111539,#111540,#111541,#111542,#111543,#111544,#111545,#111546,#111547,
#111548,#111549,#111550,#111551,#111552,#111553,#111554,#111555,#111556,
#111557,#111558,#111559,#111560,#111561,#111562,#111563,#111564,#111565,
#111566,#111567,#111568,#111569,#111570,#111571,#111572,#111573,#111574,
#111575,#111576,#111577,#111578,#111579,#111580,#111581,#111582,#111583,
#111584,#111585,#111586,#111587,#111588,#111589,#111590,#111591,#111592,
#111593,#111594,#111595,#111596,#111597,#111598,#111599,#111600,#111601,
#111602,#111603,#111604,#111605,#111606,#111607,#111608,#111609,#111610,
#111611,#111612,#111613,#111614,#111615,#111616,#111617,#111618,#111619,
#111620,#111621,#111622,#111623,#111624,#111625,#111626,#111627,#111628,
#111629,#111630,#111631,#111632,#111633,#111634,#111635,#111636,#111637,
#111638,#111639,#111640,#111641,#111642,#111643,#111644,#111645,#111646,
#111647,#111648,#111649,#111650,#111651,#111652,#111653,#111654,#111655,
#111656,#111657,#111658,#111659,#111660,#111661,#111662),.UNSPECIFIED.,
 .F.,.F.)
B_SPLINE_CURVE_WITH_KNOTS((6,1,1,1,1,1,1,1,1,1,1,1,1,1,1,1,1,1,1,1,1,1,
1,1,1,1,1,1,1,1,1,1,1,1,1,1,1,1,1,1,1,1,1,1,1,1,1,1,1,1,1,1,1,1,1,1,1,1,
1,1,1,1,1,1,1,1,1,1,1,1,1,1,1,1,1,1,1,1,1,1,1,1,1,1,1,1,1,1,1,1,1,1,1,1,
1,1,1,1,1,1,1,1,1,1,1,1,1,1,1,1,1,1,1,1,1,1,1,1,1,1,1,1,1,1,1,1,1,1,1,1,
1,1,1,1,1,1,1,1,1,1,1,1,1,1,1,1,1,1,1,1,1,1,1,1,1,1,1,1,1,1,1,1,1,1,1,1,
1,1,1,1,1,1,1,1,1,1,1,1,1,1,1,1,1,1,1,1,1,1,1,6),(-0.941429844431415,-0.940000000000001,
-0.935000000000001,-0.930000000000001,-0.925000000000001,-0.920000000000001,
-0.915000000000001,-0.910000000000001,-0.905000000000001,-0.900000000000001,
-0.895000000000001,-0.890000000000001,-0.885000000000001,-0.880000000000001,
-0.875000000000001,-0.870000000000001,-0.865000000000001,-0.860000000000001,
-0.855000000000001,-0.850000000000001,-0.845000000000001,-0.840000000000001,
-0.835000000000001,-0.830000000000001,-0.825000000000001,-0.820000000000001,
-0.815000000000001,-0.810000000000001,-0.805000000000001,-0.800000000000001,
-0.795000000000001,-0.790000000000001,-0.785000000000001,-0.780000000000001,
-0.775000000000001,-0.770000000000001,-0.765000000000001,-0.760000000000001,
-0.755000000000001,-0.750000000000001,-0.745000000000001,-0.740000000000001,
-0.735000000000001,-0.730000000000001,-0.725000000000001,-0.720000000000001,
-0.715000000000001,-0.710000000000001,-0.705000000000001,-0.700000000000001,
-0.695000000000001,-0.690000000000001,-0.685,-0.68,-0.675,-0.67,-0.665,
-0.66,-0.655,-0.65,-0.645,-0.64,-0.635,-0.63,-0.625,-0.62,-0.615,-0.61,
-0.605,-0.6,-0.595,-0.59,-0.585,-0.58,-0.575,-0.57,-0.565,-0.56,-0.555,
-0.55,-0.545,-0.54,-0.535,-0.53,-0.525,-0.52,-0.515,-0.51,-0.505,-0.5,-0.495,
-0.49,-0.485,-0.48,-0.475,-0.47,-0.465,-0.46,-0.455,-0.45,-0.445,-0.44,
-0.435,-0.43,-0.425,-0.42,-0.415,-0.41,-0.405,-0.4,-0.395,-0.39,-0.385,
-0.38,-0.375,-0.37,-0.365,-0.36,-0.355,-0.35,-0.345,-0.34,-0.335,-0.33,
-0.325,-0.32,-0.315,-0.31,-0.305,-0.3,-0.295,-0.29,-0.285,-0.28,-0.275,
-0.27,-0.265,-0.26,-0.255,-0.25,-0.245,-0.24,-0.235,-0.23,-0.225,-0.22,
-0.215,-0.21,-0.205,-0.2,-0.195,-0.19,-0.185,-0.18,-0.175,-0.17,-0.165,
-0.16,-0.155,-0.15,-0.145,-0.14,-0.135,-0.13,-0.125,-0.12,-0.115,-0.11,
-0.105,-0.1,-0.095,-0.09,-0.085,-0.08,-0.075,-0.07,-0.065,-0.06,-0.055,
-0.05,-0.045,-0.04,-0.035,-0.03,-0.025,-0.02,-0.015,-0.01,-0.005,0.),
 .UNSPECIFIED.)
CURVE()
GEOMETRIC_REPRESENTATION_ITEM()
RATIONAL_B_SPLINE_CURVE((1.,1.,1.,1.,1.,1.,1.,1.,1.,1.,1.,1.,1.,1.,1.,1.,
1.,1.,1.,1.,1.,1.,1.,1.,1.,1.,1.,1.,1.,1.,1.,1.,1.,1.,1.,1.,1.,1.,1.,1.,
1.,1.,1.,1.,1.,1.,1.,1.,1.,1.,1.,1.,1.,1.,1.,1.,1.,1.,1.,1.,1.,1.,1.,1.,
1.,1.,1.,1.,1.,1.,1.,1.,1.,1.,1.,1.,1.,1.,1.,1.,1.,1.,1.,1.,1.,1.,1.,1.,
1.,1.,1.,1.,1.,1.,1.,1.,1.,1.,1.,1.,1.,1.,1.,1.,1.,1.,1.,1.,1.,1.,1.,1.,
1.,1.,1.,1.,1.,1.,1.,1.,1.,1.,1.,1.,1.,1.,1.,1.,1.,1.,1.,1.,1.,1.,1.,1.,
1.,1.,1.,1.,1.,1.,1.,1.,1.,1.,1.,1.,1.,1.,1.,1.,1.,1.,1.,1.,1.,1.,1.,1.,
1.,1.,1.,1.,1.,1.,1.,1.,1.,1.,1.,1.,1.,1.,1.,1.,1.,1.,1.,1.,1.,1.,1.,1.,
1.,1.,1.,1.,1.,1.,1.,1.,1.,1.))
REPRESENTATION_ITEM('')
);
#535=(
BOUNDED_CURVE()
B_SPLINE_CURVE(5,(#112169,#112170,#112171,#112172,#112173,#112174,#112175,
#112176,#112177,#112178,#112179,#112180,#112181,#112182,#112183,#112184,
#112185,#112186,#112187,#112188,#112189,#112190,#112191,#112192,#112193,
#112194,#112195,#112196,#112197,#112198,#112199,#112200,#112201,#112202,
#112203,#112204,#112205,#112206,#112207,#112208,#112209,#112210,#112211,
#112212,#112213,#112214,#112215,#112216,#112217,#112218,#112219,#112220,
#112221,#112222,#112223,#112224,#112225,#112226,#112227,#112228,#112229,
#112230,#112231,#112232,#112233,#112234,#112235,#112236,#112237,#112238,
#112239,#112240,#112241,#112242,#112243,#112244,#112245,#112246,#112247,
#112248,#112249,#112250,#112251,#112252,#112253,#112254,#112255,#112256,
#112257,#112258,#112259,#112260,#112261,#112262,#112263,#112264,#112265,
#112266,#112267,#112268,#112269,#112270,#112271,#112272,#112273,#112274,
#112275,#112276,#112277,#112278,#112279,#112280,#112281,#112282,#112283,
#112284,#112285,#112286,#112287,#112288,#112289,#112290,#112291,#112292,
#112293,#112294,#112295,#112296,#112297,#112298,#112299,#112300,#112301,
#112302,#112303,#112304,#112305,#112306,#112307,#112308,#112309,#112310,
#112311,#112312,#112313,#112314,#112315,#112316,#112317,#112318,#112319,
#112320,#112321,#112322,#112323,#112324,#112325,#112326,#112327,#112328,
#112329,#112330,#112331,#112332,#112333,#112334,#112335,#112336,#112337,
#112338,#112339,#112340,#112341,#112342,#112343,#112344,#112345,#112346,
#112347,#112348,#112349,#112350,#112351,#112352,#112353,#112354,#112355,
#112356,#112357,#112358,#112359,#112360,#112361,#112362),.UNSPECIFIED.,
 .F.,.F.)
B_SPLINE_CURVE_WITH_KNOTS((6,1,1,1,1,1,1,1,1,1,1,1,1,1,1,1,1,1,1,1,1,1,
1,1,1,1,1,1,1,1,1,1,1,1,1,1,1,1,1,1,1,1,1,1,1,1,1,1,1,1,1,1,1,1,1,1,1,1,
1,1,1,1,1,1,1,1,1,1,1,1,1,1,1,1,1,1,1,1,1,1,1,1,1,1,1,1,1,1,1,1,1,1,1,1,
1,1,1,1,1,1,1,1,1,1,1,1,1,1,1,1,1,1,1,1,1,1,1,1,1,1,1,1,1,1,1,1,1,1,1,1,
1,1,1,1,1,1,1,1,1,1,1,1,1,1,1,1,1,1,1,1,1,1,1,1,1,1,1,1,1,1,1,1,1,1,1,1,
1,1,1,1,1,1,1,1,1,1,1,1,1,1,1,1,1,1,1,1,1,1,1,6),(0.,0.005,0.01,0.015,0.02,
0.025,0.03,0.035,0.04,0.045,0.05,0.055,0.06,0.065,0.07,0.075,0.08,0.085,
0.09,0.095,0.1,0.105,0.11,0.115,0.12,0.125,0.13,0.135,0.14,0.145,0.15,0.155,
0.16,0.165,0.17,0.175,0.18,0.185,0.19,0.195,0.2,0.205,0.21,0.215,0.22,0.225,
0.23,0.235,0.24,0.245,0.25,0.255,0.26,0.265,0.27,0.275,0.28,0.285,0.29,
0.295,0.3,0.305,0.31,0.315,0.32,0.325,0.33,0.335,0.34,0.345,0.35,0.355,
0.36,0.365,0.37,0.375,0.38,0.385,0.39,0.395,0.4,0.405,0.41,0.415,0.42,0.425,
0.43,0.435,0.44,0.445,0.45,0.455,0.46,0.465,0.47,0.475,0.48,0.485,0.49,
0.495,0.5,0.505,0.51,0.515,0.52,0.525,0.53,0.535,0.54,0.545,0.55,0.555,
0.56,0.565,0.57,0.575,0.58,0.585,0.59,0.595,0.6,0.605,0.61,0.615,0.62,0.625,
0.63,0.635,0.64,0.645,0.65,0.655,0.66,0.665,0.67,0.675,0.68,0.685,0.690000000000001,
0.695000000000001,0.700000000000001,0.705000000000001,0.710000000000001,
0.715000000000001,0.720000000000001,0.725000000000001,0.730000000000001,
0.735000000000001,0.740000000000001,0.745000000000001,0.750000000000001,
0.755000000000001,0.760000000000001,0.765000000000001,0.770000000000001,
0.775000000000001,0.780000000000001,0.785000000000001,0.790000000000001,
0.795000000000001,0.800000000000001,0.805000000000001,0.810000000000001,
0.815000000000001,0.820000000000001,0.825000000000001,0.830000000000001,
0.835000000000001,0.840000000000001,0.845000000000001,0.850000000000001,
0.855000000000001,0.860000000000001,0.865000000000001,0.870000000000001,
0.875000000000001,0.880000000000001,0.885000000000001,0.890000000000001,
0.895000000000001,0.900000000000001,0.905000000000001,0.910000000000001,
0.915000000000001,0.920000000000001,0.925000000000001,0.930000000000001,
0.935000000000001,0.940000000000001,0.941429844431445),.UNSPECIFIED.)
CURVE()
GEOMETRIC_REPRESENTATION_ITEM()
RATIONAL_B_SPLINE_CURVE((1.,1.,1.,1.,1.,1.,1.,1.,1.,1.,1.,1.,1.,1.,1.,1.,
1.,1.,1.,1.,1.,1.,1.,1.,1.,1.,1.,1.,1.,1.,1.,1.,1.,1.,1.,1.,1.,1.,1.,1.,
1.,1.,1.,1.,1.,1.,1.,1.,1.,1.,1.,1.,1.,1.,1.,1.,1.,1.,1.,1.,1.,1.,1.,1.,
1.,1.,1.,1.,1.,1.,1.,1.,1.,1.,1.,1.,1.,1.,1.,1.,1.,1.,1.,1.,1.,1.,1.,1.,
1.,1.,1.,1.,1.,1.,1.,1.,1.,1.,1.,1.,1.,1.,1.,1.,1.,1.,1.,1.,1.,1.,1.,1.,
1.,1.,1.,1.,1.,1.,1.,1.,1.,1.,1.,1.,1.,1.,1.,1.,1.,1.,1.,1.,1.,1.,1.,1.,
1.,1.,1.,1.,1.,1.,1.,1.,1.,1.,1.,1.,1.,1.,1.,1.,1.,1.,1.,1.,1.,1.,1.,1.,
1.,1.,1.,1.,1.,1.,1.,1.,1.,1.,1.,1.,1.,1.,1.,1.,1.,1.,1.,1.,1.,1.,1.,1.,
1.,1.,1.,1.,1.,1.,1.,1.,1.,1.))
REPRESENTATION_ITEM('')
);
#536=(
BOUNDED_CURVE()
B_SPLINE_CURVE(5,(#112365,#112366,#112367,#112368,#112369,#112370,#112371,
#112372,#112373,#112374,#112375,#112376,#112377,#112378,#112379,#112380,
#112381,#112382,#112383,#112384,#112385,#112386,#112387,#112388,#112389,
#112390,#112391,#112392,#112393,#112394,#112395,#112396,#112397,#112398,
#112399,#112400,#112401,#112402,#112403,#112404,#112405,#112406,#112407,
#112408,#112409,#112410,#112411,#112412,#112413,#112414,#112415,#112416,
#112417,#112418,#112419,#112420,#112421,#112422,#112423,#112424,#112425,
#112426,#112427,#112428,#112429,#112430,#112431,#112432,#112433,#112434,
#112435,#112436,#112437,#112438,#112439,#112440,#112441,#112442,#112443,
#112444,#112445,#112446,#112447,#112448,#112449,#112450,#112451,#112452,
#112453,#112454,#112455,#112456,#112457,#112458,#112459,#112460,#112461,
#112462,#112463,#112464,#112465,#112466,#112467,#112468,#112469,#112470,
#112471,#112472,#112473,#112474,#112475,#112476,#112477,#112478,#112479,
#112480,#112481,#112482,#112483,#112484,#112485,#112486,#112487,#112488,
#112489,#112490,#112491,#112492,#112493,#112494,#112495,#112496,#112497,
#112498,#112499,#112500,#112501,#112502,#112503,#112504,#112505,#112506,
#112507,#112508,#112509,#112510,#112511,#112512,#112513,#112514,#112515,
#112516,#112517,#112518,#112519,#112520,#112521,#112522,#112523,#112524,
#112525,#112526,#112527,#112528,#112529,#112530,#112531,#112532,#112533,
#112534,#112535,#112536,#112537,#112538,#112539,#112540,#112541,#112542,
#112543,#112544,#112545,#112546,#112547,#112548,#112549,#112550,#112551,
#112552,#112553,#112554,#112555,#112556,#112557,#112558),.UNSPECIFIED.,
 .F.,.F.)
B_SPLINE_CURVE_WITH_KNOTS((6,1,1,1,1,1,1,1,1,1,1,1,1,1,1,1,1,1,1,1,1,1,
1,1,1,1,1,1,1,1,1,1,1,1,1,1,1,1,1,1,1,1,1,1,1,1,1,1,1,1,1,1,1,1,1,1,1,1,
1,1,1,1,1,1,1,1,1,1,1,1,1,1,1,1,1,1,1,1,1,1,1,1,1,1,1,1,1,1,1,1,1,1,1,1,
1,1,1,1,1,1,1,1,1,1,1,1,1,1,1,1,1,1,1,1,1,1,1,1,1,1,1,1,1,1,1,1,1,1,1,1,
1,1,1,1,1,1,1,1,1,1,1,1,1,1,1,1,1,1,1,1,1,1,1,1,1,1,1,1,1,1,1,1,1,1,1,1,
1,1,1,1,1,1,1,1,1,1,1,1,1,1,1,1,1,1,1,1,1,1,1,6),(-0.941429844431472,-0.940000000000001,
-0.935000000000001,-0.930000000000001,-0.925000000000001,-0.920000000000001,
-0.915000000000001,-0.910000000000001,-0.905000000000001,-0.900000000000001,
-0.895000000000001,-0.890000000000001,-0.885000000000001,-0.880000000000001,
-0.875000000000001,-0.870000000000001,-0.865000000000001,-0.860000000000001,
-0.855000000000001,-0.850000000000001,-0.845000000000001,-0.840000000000001,
-0.835000000000001,-0.830000000000001,-0.825000000000001,-0.820000000000001,
-0.815000000000001,-0.810000000000001,-0.805000000000001,-0.800000000000001,
-0.795000000000001,-0.790000000000001,-0.785000000000001,-0.780000000000001,
-0.775000000000001,-0.770000000000001,-0.765000000000001,-0.760000000000001,
-0.755000000000001,-0.750000000000001,-0.745000000000001,-0.740000000000001,
-0.735000000000001,-0.730000000000001,-0.725000000000001,-0.720000000000001,
-0.715000000000001,-0.710000000000001,-0.705000000000001,-0.700000000000001,
-0.695000000000001,-0.690000000000001,-0.685,-0.68,-0.675,-0.67,-0.665,
-0.66,-0.655,-0.65,-0.645,-0.64,-0.635,-0.63,-0.625,-0.62,-0.615,-0.61,
-0.605,-0.6,-0.595,-0.59,-0.585,-0.58,-0.575,-0.57,-0.565,-0.56,-0.555,
-0.55,-0.545,-0.54,-0.535,-0.53,-0.525,-0.52,-0.515,-0.51,-0.505,-0.5,-0.495,
-0.49,-0.485,-0.48,-0.475,-0.47,-0.465,-0.46,-0.455,-0.45,-0.445,-0.44,
-0.435,-0.43,-0.425,-0.42,-0.415,-0.41,-0.405,-0.4,-0.395,-0.39,-0.385,
-0.38,-0.375,-0.37,-0.365,-0.36,-0.355,-0.35,-0.345,-0.34,-0.335,-0.33,
-0.325,-0.32,-0.315,-0.31,-0.305,-0.3,-0.295,-0.29,-0.285,-0.28,-0.275,
-0.27,-0.265,-0.26,-0.255,-0.25,-0.245,-0.24,-0.235,-0.23,-0.225,-0.22,
-0.215,-0.21,-0.205,-0.2,-0.195,-0.19,-0.185,-0.18,-0.175,-0.17,-0.165,
-0.16,-0.155,-0.15,-0.145,-0.14,-0.135,-0.13,-0.125,-0.12,-0.115,-0.11,
-0.105,-0.1,-0.095,-0.09,-0.085,-0.08,-0.075,-0.07,-0.065,-0.06,-0.055,
-0.05,-0.045,-0.04,-0.035,-0.03,-0.025,-0.02,-0.015,-0.01,-0.005,0.),
 .UNSPECIFIED.)
CURVE()
GEOMETRIC_REPRESENTATION_ITEM()
RATIONAL_B_SPLINE_CURVE((1.,1.,1.,1.,1.,1.,1.,1.,1.,1.,1.,1.,1.,1.,1.,1.,
1.,1.,1.,1.,1.,1.,1.,1.,1.,1.,1.,1.,1.,1.,1.,1.,1.,1.,1.,1.,1.,1.,1.,1.,
1.,1.,1.,1.,1.,1.,1.,1.,1.,1.,1.,1.,1.,1.,1.,1.,1.,1.,1.,1.,1.,1.,1.,1.,
1.,1.,1.,1.,1.,1.,1.,1.,1.,1.,1.,1.,1.,1.,1.,1.,1.,1.,1.,1.,1.,1.,1.,1.,
1.,1.,1.,1.,1.,1.,1.,1.,1.,1.,1.,1.,1.,1.,1.,1.,1.,1.,1.,1.,1.,1.,1.,1.,
1.,1.,1.,1.,1.,1.,1.,1.,1.,1.,1.,1.,1.,1.,1.,1.,1.,1.,1.,1.,1.,1.,1.,1.,
1.,1.,1.,1.,1.,1.,1.,1.,1.,1.,1.,1.,1.,1.,1.,1.,1.,1.,1.,1.,1.,1.,1.,1.,
1.,1.,1.,1.,1.,1.,1.,1.,1.,1.,1.,1.,1.,1.,1.,1.,1.,1.,1.,1.,1.,1.,1.,1.,
1.,1.,1.,1.,1.,1.,1.,1.,1.,1.))
REPRESENTATION_ITEM('')
);
#537=(
BOUNDED_CURVE()
B_SPLINE_CURVE(5,(#113065,#113066,#113067,#113068,#113069,#113070,#113071,
#113072,#113073,#113074,#113075,#113076,#113077,#113078,#113079,#113080,
#113081,#113082,#113083,#113084,#113085,#113086,#113087,#113088,#113089,
#113090,#113091,#113092,#113093,#113094,#113095,#113096,#113097,#113098,
#113099,#113100,#113101,#113102,#113103,#113104,#113105,#113106,#113107,
#113108,#113109,#113110,#113111,#113112,#113113,#113114,#113115,#113116,
#113117,#113118,#113119,#113120,#113121,#113122,#113123,#113124,#113125,
#113126,#113127,#113128,#113129,#113130,#113131,#113132,#113133,#113134,
#113135,#113136,#113137,#113138,#113139,#113140,#113141,#113142,#113143,
#113144,#113145,#113146,#113147,#113148,#113149,#113150,#113151,#113152,
#113153,#113154,#113155,#113156,#113157,#113158,#113159,#113160,#113161,
#113162,#113163,#113164,#113165,#113166,#113167,#113168,#113169,#113170,
#113171,#113172,#113173,#113174,#113175,#113176,#113177,#113178,#113179,
#113180,#113181,#113182,#113183,#113184,#113185,#113186,#113187,#113188,
#113189,#113190,#113191,#113192,#113193,#113194,#113195,#113196,#113197,
#113198,#113199,#113200,#113201,#113202,#113203,#113204,#113205,#113206,
#113207,#113208,#113209,#113210,#113211,#113212,#113213,#113214,#113215,
#113216,#113217,#113218,#113219,#113220,#113221,#113222,#113223,#113224,
#113225,#113226,#113227,#113228,#113229,#113230,#113231,#113232,#113233,
#113234,#113235,#113236,#113237,#113238,#113239,#113240,#113241,#113242,
#113243,#113244,#113245,#113246,#113247,#113248,#113249,#113250,#113251,
#113252,#113253,#113254,#113255,#113256,#113257,#113258),.UNSPECIFIED.,
 .F.,.F.)
B_SPLINE_CURVE_WITH_KNOTS((6,1,1,1,1,1,1,1,1,1,1,1,1,1,1,1,1,1,1,1,1,1,
1,1,1,1,1,1,1,1,1,1,1,1,1,1,1,1,1,1,1,1,1,1,1,1,1,1,1,1,1,1,1,1,1,1,1,1,
1,1,1,1,1,1,1,1,1,1,1,1,1,1,1,1,1,1,1,1,1,1,1,1,1,1,1,1,1,1,1,1,1,1,1,1,
1,1,1,1,1,1,1,1,1,1,1,1,1,1,1,1,1,1,1,1,1,1,1,1,1,1,1,1,1,1,1,1,1,1,1,1,
1,1,1,1,1,1,1,1,1,1,1,1,1,1,1,1,1,1,1,1,1,1,1,1,1,1,1,1,1,1,1,1,1,1,1,1,
1,1,1,1,1,1,1,1,1,1,1,1,1,1,1,1,1,1,1,1,1,1,1,6),(0.,0.005,0.01,0.015,0.02,
0.025,0.03,0.035,0.04,0.045,0.05,0.055,0.06,0.065,0.07,0.075,0.08,0.085,
0.09,0.095,0.1,0.105,0.11,0.115,0.12,0.125,0.13,0.135,0.14,0.145,0.15,0.155,
0.16,0.165,0.17,0.175,0.18,0.185,0.19,0.195,0.2,0.205,0.21,0.215,0.22,0.225,
0.23,0.235,0.24,0.245,0.25,0.255,0.26,0.265,0.27,0.275,0.28,0.285,0.29,
0.295,0.3,0.305,0.31,0.315,0.32,0.325,0.33,0.335,0.34,0.345,0.35,0.355,
0.36,0.365,0.37,0.375,0.38,0.385,0.39,0.395,0.4,0.405,0.41,0.415,0.42,0.425,
0.43,0.435,0.44,0.445,0.45,0.455,0.46,0.465,0.47,0.475,0.48,0.485,0.49,
0.495,0.5,0.505,0.51,0.515,0.52,0.525,0.53,0.535,0.54,0.545,0.55,0.555,
0.56,0.565,0.57,0.575,0.58,0.585,0.59,0.595,0.6,0.605,0.61,0.615,0.62,0.625,
0.63,0.635,0.64,0.645,0.65,0.655,0.66,0.665,0.67,0.675,0.68,0.685,0.690000000000001,
0.695000000000001,0.700000000000001,0.705000000000001,0.710000000000001,
0.715000000000001,0.720000000000001,0.725000000000001,0.730000000000001,
0.735000000000001,0.740000000000001,0.745000000000001,0.750000000000001,
0.755000000000001,0.760000000000001,0.765000000000001,0.770000000000001,
0.775000000000001,0.780000000000001,0.785000000000001,0.790000000000001,
0.795000000000001,0.800000000000001,0.805000000000001,0.810000000000001,
0.815000000000001,0.820000000000001,0.825000000000001,0.830000000000001,
0.835000000000001,0.840000000000001,0.845000000000001,0.850000000000001,
0.855000000000001,0.860000000000001,0.865000000000001,0.870000000000001,
0.875000000000001,0.880000000000001,0.885000000000001,0.890000000000001,
0.895000000000001,0.900000000000001,0.905000000000001,0.910000000000001,
0.915000000000001,0.920000000000001,0.925000000000001,0.930000000000001,
0.935000000000001,0.940000000000001,0.941429844431522),.UNSPECIFIED.)
CURVE()
GEOMETRIC_REPRESENTATION_ITEM()
RATIONAL_B_SPLINE_CURVE((1.,1.,1.,1.,1.,1.,1.,1.,1.,1.,1.,1.,1.,1.,1.,1.,
1.,1.,1.,1.,1.,1.,1.,1.,1.,1.,1.,1.,1.,1.,1.,1.,1.,1.,1.,1.,1.,1.,1.,1.,
1.,1.,1.,1.,1.,1.,1.,1.,1.,1.,1.,1.,1.,1.,1.,1.,1.,1.,1.,1.,1.,1.,1.,1.,
1.,1.,1.,1.,1.,1.,1.,1.,1.,1.,1.,1.,1.,1.,1.,1.,1.,1.,1.,1.,1.,1.,1.,1.,
1.,1.,1.,1.,1.,1.,1.,1.,1.,1.,1.,1.,1.,1.,1.,1.,1.,1.,1.,1.,1.,1.,1.,1.,
1.,1.,1.,1.,1.,1.,1.,1.,1.,1.,1.,1.,1.,1.,1.,1.,1.,1.,1.,1.,1.,1.,1.,1.,
1.,1.,1.,1.,1.,1.,1.,1.,1.,1.,1.,1.,1.,1.,1.,1.,1.,1.,1.,1.,1.,1.,1.,1.,
1.,1.,1.,1.,1.,1.,1.,1.,1.,1.,1.,1.,1.,1.,1.,1.,1.,1.,1.,1.,1.,1.,1.,1.,
1.,1.,1.,1.,1.,1.,1.,1.,1.,1.))
REPRESENTATION_ITEM('')
);
#538=(
BOUNDED_CURVE()
B_SPLINE_CURVE(5,(#113261,#113262,#113263,#113264,#113265,#113266,#113267,
#113268,#113269,#113270,#113271,#113272,#113273,#113274,#113275,#113276,
#113277,#113278,#113279,#113280,#113281,#113282,#113283,#113284,#113285,
#113286,#113287,#113288,#113289,#113290,#113291,#113292,#113293,#113294,
#113295,#113296,#113297,#113298,#113299,#113300,#113301,#113302,#113303,
#113304,#113305,#113306,#113307,#113308,#113309,#113310,#113311,#113312,
#113313,#113314,#113315,#113316,#113317,#113318,#113319,#113320,#113321,
#113322,#113323,#113324,#113325,#113326,#113327,#113328,#113329,#113330,
#113331,#113332,#113333,#113334,#113335,#113336,#113337,#113338,#113339,
#113340,#113341,#113342,#113343,#113344,#113345,#113346,#113347,#113348,
#113349,#113350,#113351,#113352,#113353,#113354,#113355,#113356,#113357,
#113358,#113359,#113360,#113361,#113362,#113363,#113364,#113365,#113366,
#113367,#113368,#113369,#113370,#113371,#113372,#113373,#113374,#113375,
#113376,#113377,#113378,#113379,#113380,#113381,#113382,#113383,#113384,
#113385,#113386,#113387,#113388,#113389,#113390,#113391,#113392,#113393,
#113394,#113395,#113396,#113397,#113398,#113399,#113400,#113401,#113402,
#113403,#113404,#113405,#113406,#113407,#113408,#113409,#113410,#113411,
#113412,#113413,#113414,#113415,#113416,#113417,#113418,#113419,#113420,
#113421,#113422,#113423,#113424,#113425,#113426,#113427,#113428,#113429,
#113430,#113431,#113432,#113433,#113434,#113435,#113436,#113437,#113438,
#113439,#113440,#113441,#113442,#113443,#113444,#113445,#113446,#113447,
#113448,#113449,#113450,#113451,#113452,#113453,#113454),.UNSPECIFIED.,
 .F.,.F.)
B_SPLINE_CURVE_WITH_KNOTS((6,1,1,1,1,1,1,1,1,1,1,1,1,1,1,1,1,1,1,1,1,1,
1,1,1,1,1,1,1,1,1,1,1,1,1,1,1,1,1,1,1,1,1,1,1,1,1,1,1,1,1,1,1,1,1,1,1,1,
1,1,1,1,1,1,1,1,1,1,1,1,1,1,1,1,1,1,1,1,1,1,1,1,1,1,1,1,1,1,1,1,1,1,1,1,
1,1,1,1,1,1,1,1,1,1,1,1,1,1,1,1,1,1,1,1,1,1,1,1,1,1,1,1,1,1,1,1,1,1,1,1,
1,1,1,1,1,1,1,1,1,1,1,1,1,1,1,1,1,1,1,1,1,1,1,1,1,1,1,1,1,1,1,1,1,1,1,1,
1,1,1,1,1,1,1,1,1,1,1,1,1,1,1,1,1,1,1,1,1,1,1,6),(-0.941429844431529,-0.940000000000001,
-0.935000000000001,-0.930000000000001,-0.925000000000001,-0.920000000000001,
-0.915000000000001,-0.910000000000001,-0.905000000000001,-0.900000000000001,
-0.895000000000001,-0.890000000000001,-0.885000000000001,-0.880000000000001,
-0.875000000000001,-0.870000000000001,-0.865000000000001,-0.860000000000001,
-0.855000000000001,-0.850000000000001,-0.845000000000001,-0.840000000000001,
-0.835000000000001,-0.830000000000001,-0.825000000000001,-0.820000000000001,
-0.815000000000001,-0.810000000000001,-0.805000000000001,-0.800000000000001,
-0.795000000000001,-0.790000000000001,-0.785000000000001,-0.780000000000001,
-0.775000000000001,-0.770000000000001,-0.765000000000001,-0.760000000000001,
-0.755000000000001,-0.750000000000001,-0.745000000000001,-0.740000000000001,
-0.735000000000001,-0.730000000000001,-0.725000000000001,-0.720000000000001,
-0.715000000000001,-0.710000000000001,-0.705000000000001,-0.700000000000001,
-0.695000000000001,-0.690000000000001,-0.685,-0.68,-0.675,-0.67,-0.665,
-0.66,-0.655,-0.65,-0.645,-0.64,-0.635,-0.63,-0.625,-0.62,-0.615,-0.61,
-0.605,-0.6,-0.595,-0.59,-0.585,-0.58,-0.575,-0.57,-0.565,-0.56,-0.555,
-0.55,-0.545,-0.54,-0.535,-0.53,-0.525,-0.52,-0.515,-0.51,-0.505,-0.5,-0.495,
-0.49,-0.485,-0.48,-0.475,-0.47,-0.465,-0.46,-0.455,-0.45,-0.445,-0.44,
-0.435,-0.43,-0.425,-0.42,-0.415,-0.41,-0.405,-0.4,-0.395,-0.39,-0.385,
-0.38,-0.375,-0.37,-0.365,-0.36,-0.355,-0.35,-0.345,-0.34,-0.335,-0.33,
-0.325,-0.32,-0.315,-0.31,-0.305,-0.3,-0.295,-0.29,-0.285,-0.28,-0.275,
-0.27,-0.265,-0.26,-0.255,-0.25,-0.245,-0.24,-0.235,-0.23,-0.225,-0.22,
-0.215,-0.21,-0.205,-0.2,-0.195,-0.19,-0.185,-0.18,-0.175,-0.17,-0.165,
-0.16,-0.155,-0.15,-0.145,-0.14,-0.135,-0.13,-0.125,-0.12,-0.115,-0.11,
-0.105,-0.1,-0.095,-0.09,-0.085,-0.08,-0.075,-0.07,-0.065,-0.06,-0.055,
-0.05,-0.045,-0.04,-0.035,-0.03,-0.025,-0.02,-0.015,-0.01,-0.005,0.),
 .UNSPECIFIED.)
CURVE()
GEOMETRIC_REPRESENTATION_ITEM()
RATIONAL_B_SPLINE_CURVE((1.,1.,1.,1.,1.,1.,1.,1.,1.,1.,1.,1.,1.,1.,1.,1.,
1.,1.,1.,1.,1.,1.,1.,1.,1.,1.,1.,1.,1.,1.,1.,1.,1.,1.,1.,1.,1.,1.,1.,1.,
1.,1.,1.,1.,1.,1.,1.,1.,1.,1.,1.,1.,1.,1.,1.,1.,1.,1.,1.,1.,1.,1.,1.,1.,
1.,1.,1.,1.,1.,1.,1.,1.,1.,1.,1.,1.,1.,1.,1.,1.,1.,1.,1.,1.,1.,1.,1.,1.,
1.,1.,1.,1.,1.,1.,1.,1.,1.,1.,1.,1.,1.,1.,1.,1.,1.,1.,1.,1.,1.,1.,1.,1.,
1.,1.,1.,1.,1.,1.,1.,1.,1.,1.,1.,1.,1.,1.,1.,1.,1.,1.,1.,1.,1.,1.,1.,1.,
1.,1.,1.,1.,1.,1.,1.,1.,1.,1.,1.,1.,1.,1.,1.,1.,1.,1.,1.,1.,1.,1.,1.,1.,
1.,1.,1.,1.,1.,1.,1.,1.,1.,1.,1.,1.,1.,1.,1.,1.,1.,1.,1.,1.,1.,1.,1.,1.,
1.,1.,1.,1.,1.,1.,1.,1.,1.,1.))
REPRESENTATION_ITEM('')
);
#539=(
BOUNDED_CURVE()
B_SPLINE_CURVE(5,(#113961,#113962,#113963,#113964,#113965,#113966,#113967,
#113968,#113969,#113970,#113971,#113972,#113973,#113974,#113975,#113976,
#113977,#113978,#113979,#113980,#113981,#113982,#113983,#113984,#113985,
#113986,#113987,#113988,#113989,#113990,#113991,#113992,#113993,#113994,
#113995,#113996,#113997,#113998,#113999,#114000,#114001,#114002,#114003,
#114004,#114005,#114006,#114007,#114008,#114009,#114010,#114011,#114012,
#114013,#114014,#114015,#114016,#114017,#114018,#114019,#114020,#114021,
#114022,#114023,#114024,#114025,#114026,#114027,#114028,#114029,#114030,
#114031,#114032,#114033,#114034,#114035,#114036,#114037,#114038,#114039,
#114040,#114041,#114042,#114043,#114044,#114045,#114046,#114047,#114048,
#114049,#114050,#114051,#114052,#114053,#114054,#114055,#114056,#114057,
#114058,#114059,#114060,#114061,#114062,#114063,#114064,#114065,#114066,
#114067,#114068,#114069,#114070,#114071,#114072,#114073,#114074,#114075,
#114076,#114077,#114078,#114079,#114080,#114081,#114082,#114083,#114084,
#114085,#114086,#114087,#114088,#114089,#114090,#114091,#114092,#114093,
#114094,#114095,#114096,#114097,#114098,#114099,#114100,#114101,#114102,
#114103,#114104,#114105,#114106,#114107,#114108,#114109,#114110,#114111,
#114112,#114113,#114114,#114115,#114116,#114117,#114118,#114119,#114120,
#114121,#114122,#114123,#114124,#114125,#114126,#114127,#114128,#114129,
#114130,#114131,#114132,#114133,#114134,#114135,#114136,#114137,#114138,
#114139,#114140,#114141,#114142,#114143,#114144,#114145,#114146,#114147,
#114148,#114149,#114150,#114151,#114152,#114153,#114154),.UNSPECIFIED.,
 .F.,.F.)
B_SPLINE_CURVE_WITH_KNOTS((6,1,1,1,1,1,1,1,1,1,1,1,1,1,1,1,1,1,1,1,1,1,
1,1,1,1,1,1,1,1,1,1,1,1,1,1,1,1,1,1,1,1,1,1,1,1,1,1,1,1,1,1,1,1,1,1,1,1,
1,1,1,1,1,1,1,1,1,1,1,1,1,1,1,1,1,1,1,1,1,1,1,1,1,1,1,1,1,1,1,1,1,1,1,1,
1,1,1,1,1,1,1,1,1,1,1,1,1,1,1,1,1,1,1,1,1,1,1,1,1,1,1,1,1,1,1,1,1,1,1,1,
1,1,1,1,1,1,1,1,1,1,1,1,1,1,1,1,1,1,1,1,1,1,1,1,1,1,1,1,1,1,1,1,1,1,1,1,
1,1,1,1,1,1,1,1,1,1,1,1,1,1,1,1,1,1,1,1,1,1,1,6),(0.,0.005,0.01,0.015,0.02,
0.025,0.03,0.035,0.04,0.045,0.05,0.055,0.06,0.065,0.07,0.075,0.08,0.085,
0.09,0.095,0.1,0.105,0.11,0.115,0.12,0.125,0.13,0.135,0.14,0.145,0.15,0.155,
0.16,0.165,0.17,0.175,0.18,0.185,0.19,0.195,0.2,0.205,0.21,0.215,0.22,0.225,
0.23,0.235,0.24,0.245,0.25,0.255,0.26,0.265,0.27,0.275,0.28,0.285,0.29,
0.295,0.3,0.305,0.31,0.315,0.32,0.325,0.33,0.335,0.34,0.345,0.35,0.355,
0.36,0.365,0.37,0.375,0.38,0.385,0.39,0.395,0.4,0.405,0.41,0.415,0.42,0.425,
0.43,0.435,0.44,0.445,0.45,0.455,0.46,0.465,0.47,0.475,0.48,0.485,0.49,
0.495,0.5,0.505,0.51,0.515,0.52,0.525,0.53,0.535,0.54,0.545,0.55,0.555,
0.56,0.565,0.57,0.575,0.58,0.585,0.59,0.595,0.6,0.605,0.61,0.615,0.62,0.625,
0.63,0.635,0.64,0.645,0.65,0.655,0.66,0.665,0.67,0.675,0.68,0.685,0.690000000000001,
0.695000000000001,0.700000000000001,0.705000000000001,0.710000000000001,
0.715000000000001,0.720000000000001,0.725000000000001,0.730000000000001,
0.735000000000001,0.740000000000001,0.745000000000001,0.750000000000001,
0.755000000000001,0.760000000000001,0.765000000000001,0.770000000000001,
0.775000000000001,0.780000000000001,0.785000000000001,0.790000000000001,
0.795000000000001,0.800000000000001,0.805000000000001,0.810000000000001,
0.815000000000001,0.820000000000001,0.825000000000001,0.830000000000001,
0.835000000000001,0.840000000000001,0.845000000000001,0.850000000000001,
0.855000000000001,0.860000000000001,0.865000000000001,0.870000000000001,
0.875000000000001,0.880000000000001,0.885000000000001,0.890000000000001,
0.895000000000001,0.900000000000001,0.905000000000001,0.910000000000001,
0.915000000000001,0.920000000000001,0.925000000000001,0.930000000000001,
0.935000000000001,0.940000000000001,0.941429844431397),.UNSPECIFIED.)
CURVE()
GEOMETRIC_REPRESENTATION_ITEM()
RATIONAL_B_SPLINE_CURVE((1.,1.,1.,1.,1.,1.,1.,1.,1.,1.,1.,1.,1.,1.,1.,1.,
1.,1.,1.,1.,1.,1.,1.,1.,1.,1.,1.,1.,1.,1.,1.,1.,1.,1.,1.,1.,1.,1.,1.,1.,
1.,1.,1.,1.,1.,1.,1.,1.,1.,1.,1.,1.,1.,1.,1.,1.,1.,1.,1.,1.,1.,1.,1.,1.,
1.,1.,1.,1.,1.,1.,1.,1.,1.,1.,1.,1.,1.,1.,1.,1.,1.,1.,1.,1.,1.,1.,1.,1.,
1.,1.,1.,1.,1.,1.,1.,1.,1.,1.,1.,1.,1.,1.,1.,1.,1.,1.,1.,1.,1.,1.,1.,1.,
1.,1.,1.,1.,1.,1.,1.,1.,1.,1.,1.,1.,1.,1.,1.,1.,1.,1.,1.,1.,1.,1.,1.,1.,
1.,1.,1.,1.,1.,1.,1.,1.,1.,1.,1.,1.,1.,1.,1.,1.,1.,1.,1.,1.,1.,1.,1.,1.,
1.,1.,1.,1.,1.,1.,1.,1.,1.,1.,1.,1.,1.,1.,1.,1.,1.,1.,1.,1.,1.,1.,1.,1.,
1.,1.,1.,1.,1.,1.,1.,1.,1.,1.))
REPRESENTATION_ITEM('')
);
#540=(
BOUNDED_CURVE()
B_SPLINE_CURVE(5,(#114157,#114158,#114159,#114160,#114161,#114162,#114163,
#114164,#114165,#114166,#114167,#114168,#114169,#114170,#114171,#114172,
#114173,#114174,#114175,#114176,#114177,#114178,#114179,#114180,#114181,
#114182,#114183,#114184,#114185,#114186,#114187,#114188,#114189,#114190,
#114191,#114192,#114193,#114194,#114195,#114196,#114197,#114198,#114199,
#114200,#114201,#114202,#114203,#114204,#114205,#114206,#114207,#114208,
#114209,#114210,#114211,#114212,#114213,#114214,#114215,#114216,#114217,
#114218,#114219,#114220,#114221,#114222,#114223,#114224,#114225,#114226,
#114227,#114228,#114229,#114230,#114231,#114232,#114233,#114234,#114235,
#114236,#114237,#114238,#114239,#114240,#114241,#114242,#114243,#114244,
#114245,#114246,#114247,#114248,#114249,#114250,#114251,#114252,#114253,
#114254,#114255,#114256,#114257,#114258,#114259,#114260,#114261,#114262,
#114263,#114264,#114265,#114266,#114267,#114268,#114269,#114270,#114271,
#114272,#114273,#114274,#114275,#114276,#114277,#114278,#114279,#114280,
#114281,#114282,#114283,#114284,#114285,#114286,#114287,#114288,#114289,
#114290,#114291,#114292,#114293,#114294,#114295,#114296,#114297,#114298,
#114299,#114300,#114301,#114302,#114303,#114304,#114305,#114306,#114307,
#114308,#114309,#114310,#114311,#114312,#114313,#114314,#114315,#114316,
#114317,#114318,#114319,#114320,#114321,#114322,#114323,#114324,#114325,
#114326,#114327,#114328,#114329,#114330,#114331,#114332,#114333,#114334,
#114335,#114336,#114337,#114338,#114339,#114340,#114341,#114342,#114343,
#114344,#114345,#114346,#114347,#114348,#114349,#114350),.UNSPECIFIED.,
 .F.,.F.)
B_SPLINE_CURVE_WITH_KNOTS((6,1,1,1,1,1,1,1,1,1,1,1,1,1,1,1,1,1,1,1,1,1,
1,1,1,1,1,1,1,1,1,1,1,1,1,1,1,1,1,1,1,1,1,1,1,1,1,1,1,1,1,1,1,1,1,1,1,1,
1,1,1,1,1,1,1,1,1,1,1,1,1,1,1,1,1,1,1,1,1,1,1,1,1,1,1,1,1,1,1,1,1,1,1,1,
1,1,1,1,1,1,1,1,1,1,1,1,1,1,1,1,1,1,1,1,1,1,1,1,1,1,1,1,1,1,1,1,1,1,1,1,
1,1,1,1,1,1,1,1,1,1,1,1,1,1,1,1,1,1,1,1,1,1,1,1,1,1,1,1,1,1,1,1,1,1,1,1,
1,1,1,1,1,1,1,1,1,1,1,1,1,1,1,1,1,1,1,1,1,1,1,6),(-0.941429844431401,-0.940000000000001,
-0.935000000000001,-0.930000000000001,-0.925000000000001,-0.920000000000001,
-0.915000000000001,-0.910000000000001,-0.905000000000001,-0.900000000000001,
-0.895000000000001,-0.890000000000001,-0.885000000000001,-0.880000000000001,
-0.875000000000001,-0.870000000000001,-0.865000000000001,-0.860000000000001,
-0.855000000000001,-0.850000000000001,-0.845000000000001,-0.840000000000001,
-0.835000000000001,-0.830000000000001,-0.825000000000001,-0.820000000000001,
-0.815000000000001,-0.810000000000001,-0.805000000000001,-0.800000000000001,
-0.795000000000001,-0.790000000000001,-0.785000000000001,-0.780000000000001,
-0.775000000000001,-0.770000000000001,-0.765000000000001,-0.760000000000001,
-0.755000000000001,-0.750000000000001,-0.745000000000001,-0.740000000000001,
-0.735000000000001,-0.730000000000001,-0.725000000000001,-0.720000000000001,
-0.715000000000001,-0.710000000000001,-0.705000000000001,-0.700000000000001,
-0.695000000000001,-0.690000000000001,-0.685,-0.68,-0.675,-0.67,-0.665,
-0.66,-0.655,-0.65,-0.645,-0.64,-0.635,-0.63,-0.625,-0.62,-0.615,-0.61,
-0.605,-0.6,-0.595,-0.59,-0.585,-0.58,-0.575,-0.57,-0.565,-0.56,-0.555,
-0.55,-0.545,-0.54,-0.535,-0.53,-0.525,-0.52,-0.515,-0.51,-0.505,-0.5,-0.495,
-0.49,-0.485,-0.48,-0.475,-0.47,-0.465,-0.46,-0.455,-0.45,-0.445,-0.44,
-0.435,-0.43,-0.425,-0.42,-0.415,-0.41,-0.405,-0.4,-0.395,-0.39,-0.385,
-0.38,-0.375,-0.37,-0.365,-0.36,-0.355,-0.35,-0.345,-0.34,-0.335,-0.33,
-0.325,-0.32,-0.315,-0.31,-0.305,-0.3,-0.295,-0.29,-0.285,-0.28,-0.275,
-0.27,-0.265,-0.26,-0.255,-0.25,-0.245,-0.24,-0.235,-0.23,-0.225,-0.22,
-0.215,-0.21,-0.205,-0.2,-0.195,-0.19,-0.185,-0.18,-0.175,-0.17,-0.165,
-0.16,-0.155,-0.15,-0.145,-0.14,-0.135,-0.13,-0.125,-0.12,-0.115,-0.11,
-0.105,-0.1,-0.095,-0.09,-0.085,-0.08,-0.075,-0.07,-0.065,-0.06,-0.055,
-0.05,-0.045,-0.04,-0.035,-0.03,-0.025,-0.02,-0.015,-0.01,-0.005,0.),
 .UNSPECIFIED.)
CURVE()
GEOMETRIC_REPRESENTATION_ITEM()
RATIONAL_B_SPLINE_CURVE((1.,1.,1.,1.,1.,1.,1.,1.,1.,1.,1.,1.,1.,1.,1.,1.,
1.,1.,1.,1.,1.,1.,1.,1.,1.,1.,1.,1.,1.,1.,1.,1.,1.,1.,1.,1.,1.,1.,1.,1.,
1.,1.,1.,1.,1.,1.,1.,1.,1.,1.,1.,1.,1.,1.,1.,1.,1.,1.,1.,1.,1.,1.,1.,1.,
1.,1.,1.,1.,1.,1.,1.,1.,1.,1.,1.,1.,1.,1.,1.,1.,1.,1.,1.,1.,1.,1.,1.,1.,
1.,1.,1.,1.,1.,1.,1.,1.,1.,1.,1.,1.,1.,1.,1.,1.,1.,1.,1.,1.,1.,1.,1.,1.,
1.,1.,1.,1.,1.,1.,1.,1.,1.,1.,1.,1.,1.,1.,1.,1.,1.,1.,1.,1.,1.,1.,1.,1.,
1.,1.,1.,1.,1.,1.,1.,1.,1.,1.,1.,1.,1.,1.,1.,1.,1.,1.,1.,1.,1.,1.,1.,1.,
1.,1.,1.,1.,1.,1.,1.,1.,1.,1.,1.,1.,1.,1.,1.,1.,1.,1.,1.,1.,1.,1.,1.,1.,
1.,1.,1.,1.,1.,1.,1.,1.,1.,1.))
REPRESENTATION_ITEM('')
);
#541=(
BOUNDED_CURVE()
B_SPLINE_CURVE(5,(#114857,#114858,#114859,#114860,#114861,#114862,#114863,
#114864,#114865,#114866,#114867,#114868,#114869,#114870,#114871,#114872,
#114873,#114874,#114875,#114876,#114877,#114878,#114879,#114880,#114881,
#114882,#114883,#114884,#114885,#114886,#114887,#114888,#114889,#114890,
#114891,#114892,#114893,#114894,#114895,#114896,#114897,#114898,#114899,
#114900,#114901,#114902,#114903,#114904,#114905,#114906,#114907,#114908,
#114909,#114910,#114911,#114912,#114913,#114914,#114915,#114916,#114917,
#114918,#114919,#114920,#114921,#114922,#114923,#114924,#114925,#114926,
#114927,#114928,#114929,#114930,#114931,#114932,#114933,#114934,#114935,
#114936,#114937,#114938,#114939,#114940,#114941,#114942,#114943,#114944,
#114945,#114946,#114947,#114948,#114949,#114950,#114951,#114952,#114953,
#114954,#114955,#114956,#114957,#114958,#114959,#114960,#114961,#114962,
#114963,#114964,#114965,#114966,#114967,#114968,#114969,#114970,#114971,
#114972,#114973,#114974,#114975,#114976,#114977,#114978,#114979,#114980,
#114981,#114982,#114983,#114984,#114985,#114986,#114987,#114988,#114989,
#114990,#114991,#114992,#114993,#114994,#114995,#114996,#114997,#114998,
#114999,#115000,#115001,#115002,#115003,#115004,#115005,#115006,#115007,
#115008,#115009,#115010,#115011,#115012,#115013,#115014,#115015,#115016,
#115017,#115018,#115019,#115020,#115021,#115022,#115023,#115024,#115025,
#115026,#115027,#115028,#115029,#115030,#115031,#115032,#115033,#115034,
#115035,#115036,#115037,#115038,#115039,#115040,#115041,#115042,#115043,
#115044,#115045,#115046,#115047,#115048,#115049,#115050),.UNSPECIFIED.,
 .F.,.F.)
B_SPLINE_CURVE_WITH_KNOTS((6,1,1,1,1,1,1,1,1,1,1,1,1,1,1,1,1,1,1,1,1,1,
1,1,1,1,1,1,1,1,1,1,1,1,1,1,1,1,1,1,1,1,1,1,1,1,1,1,1,1,1,1,1,1,1,1,1,1,
1,1,1,1,1,1,1,1,1,1,1,1,1,1,1,1,1,1,1,1,1,1,1,1,1,1,1,1,1,1,1,1,1,1,1,1,
1,1,1,1,1,1,1,1,1,1,1,1,1,1,1,1,1,1,1,1,1,1,1,1,1,1,1,1,1,1,1,1,1,1,1,1,
1,1,1,1,1,1,1,1,1,1,1,1,1,1,1,1,1,1,1,1,1,1,1,1,1,1,1,1,1,1,1,1,1,1,1,1,
1,1,1,1,1,1,1,1,1,1,1,1,1,1,1,1,1,1,1,1,1,1,1,6),(0.,0.005,0.01,0.015,0.02,
0.025,0.03,0.035,0.04,0.045,0.05,0.055,0.06,0.065,0.07,0.075,0.08,0.085,
0.09,0.095,0.1,0.105,0.11,0.115,0.12,0.125,0.13,0.135,0.14,0.145,0.15,0.155,
0.16,0.165,0.17,0.175,0.18,0.185,0.19,0.195,0.2,0.205,0.21,0.215,0.22,0.225,
0.23,0.235,0.24,0.245,0.25,0.255,0.26,0.265,0.27,0.275,0.28,0.285,0.29,
0.295,0.3,0.305,0.31,0.315,0.32,0.325,0.33,0.335,0.34,0.345,0.35,0.355,
0.36,0.365,0.37,0.375,0.38,0.385,0.39,0.395,0.4,0.405,0.41,0.415,0.42,0.425,
0.43,0.435,0.44,0.445,0.45,0.455,0.46,0.465,0.47,0.475,0.48,0.485,0.49,
0.495,0.5,0.505,0.51,0.515,0.52,0.525,0.53,0.535,0.54,0.545,0.55,0.555,
0.56,0.565,0.57,0.575,0.58,0.585,0.59,0.595,0.6,0.605,0.61,0.615,0.62,0.625,
0.63,0.635,0.64,0.645,0.65,0.655,0.66,0.665,0.67,0.675,0.68,0.685,0.690000000000001,
0.695000000000001,0.700000000000001,0.705000000000001,0.710000000000001,
0.715000000000001,0.720000000000001,0.725000000000001,0.730000000000001,
0.735000000000001,0.740000000000001,0.745000000000001,0.750000000000001,
0.755000000000001,0.760000000000001,0.765000000000001,0.770000000000001,
0.775000000000001,0.780000000000001,0.785000000000001,0.790000000000001,
0.795000000000001,0.800000000000001,0.805000000000001,0.810000000000001,
0.815000000000001,0.820000000000001,0.825000000000001,0.830000000000001,
0.835000000000001,0.840000000000001,0.845000000000001,0.850000000000001,
0.855000000000001,0.860000000000001,0.865000000000001,0.870000000000001,
0.875000000000001,0.880000000000001,0.885000000000001,0.890000000000001,
0.895000000000001,0.900000000000001,0.905000000000001,0.910000000000001,
0.915000000000001,0.920000000000001,0.925000000000001,0.930000000000001,
0.935000000000001,0.940000000000001,0.94142984443138),.UNSPECIFIED.)
CURVE()
GEOMETRIC_REPRESENTATION_ITEM()
RATIONAL_B_SPLINE_CURVE((1.,1.,1.,1.,1.,1.,1.,1.,1.,1.,1.,1.,1.,1.,1.,1.,
1.,1.,1.,1.,1.,1.,1.,1.,1.,1.,1.,1.,1.,1.,1.,1.,1.,1.,1.,1.,1.,1.,1.,1.,
1.,1.,1.,1.,1.,1.,1.,1.,1.,1.,1.,1.,1.,1.,1.,1.,1.,1.,1.,1.,1.,1.,1.,1.,
1.,1.,1.,1.,1.,1.,1.,1.,1.,1.,1.,1.,1.,1.,1.,1.,1.,1.,1.,1.,1.,1.,1.,1.,
1.,1.,1.,1.,1.,1.,1.,1.,1.,1.,1.,1.,1.,1.,1.,1.,1.,1.,1.,1.,1.,1.,1.,1.,
1.,1.,1.,1.,1.,1.,1.,1.,1.,1.,1.,1.,1.,1.,1.,1.,1.,1.,1.,1.,1.,1.,1.,1.,
1.,1.,1.,1.,1.,1.,1.,1.,1.,1.,1.,1.,1.,1.,1.,1.,1.,1.,1.,1.,1.,1.,1.,1.,
1.,1.,1.,1.,1.,1.,1.,1.,1.,1.,1.,1.,1.,1.,1.,1.,1.,1.,1.,1.,1.,1.,1.,1.,
1.,1.,1.,1.,1.,1.,1.,1.,1.,1.))
REPRESENTATION_ITEM('')
);
#542=(
BOUNDED_CURVE()
B_SPLINE_CURVE(5,(#115053,#115054,#115055,#115056,#115057,#115058,#115059,
#115060,#115061,#115062,#115063,#115064,#115065,#115066,#115067,#115068,
#115069,#115070,#115071,#115072,#115073,#115074,#115075,#115076,#115077,
#115078,#115079,#115080,#115081,#115082,#115083,#115084,#115085,#115086,
#115087,#115088,#115089,#115090,#115091,#115092,#115093,#115094,#115095,
#115096,#115097,#115098,#115099,#115100,#115101,#115102,#115103,#115104,
#115105,#115106,#115107,#115108,#115109,#115110,#115111,#115112,#115113,
#115114,#115115,#115116,#115117,#115118,#115119,#115120,#115121,#115122,
#115123,#115124,#115125,#115126,#115127,#115128,#115129,#115130,#115131,
#115132,#115133,#115134,#115135,#115136,#115137,#115138,#115139,#115140,
#115141,#115142,#115143,#115144,#115145,#115146,#115147,#115148,#115149,
#115150,#115151,#115152,#115153,#115154,#115155,#115156,#115157,#115158,
#115159,#115160,#115161,#115162,#115163,#115164,#115165,#115166,#115167,
#115168,#115169,#115170,#115171,#115172,#115173,#115174,#115175,#115176,
#115177,#115178,#115179,#115180,#115181,#115182,#115183,#115184,#115185,
#115186,#115187,#115188,#115189,#115190,#115191,#115192,#115193,#115194,
#115195,#115196,#115197,#115198,#115199,#115200,#115201,#115202,#115203,
#115204,#115205,#115206,#115207,#115208,#115209,#115210,#115211,#115212,
#115213,#115214,#115215,#115216,#115217,#115218,#115219,#115220,#115221,
#115222,#115223,#115224,#115225,#115226,#115227,#115228,#115229,#115230,
#115231,#115232,#115233,#115234,#115235,#115236,#115237,#115238,#115239,
#115240,#115241,#115242,#115243,#115244,#115245,#115246),.UNSPECIFIED.,
 .F.,.F.)
B_SPLINE_CURVE_WITH_KNOTS((6,1,1,1,1,1,1,1,1,1,1,1,1,1,1,1,1,1,1,1,1,1,
1,1,1,1,1,1,1,1,1,1,1,1,1,1,1,1,1,1,1,1,1,1,1,1,1,1,1,1,1,1,1,1,1,1,1,1,
1,1,1,1,1,1,1,1,1,1,1,1,1,1,1,1,1,1,1,1,1,1,1,1,1,1,1,1,1,1,1,1,1,1,1,1,
1,1,1,1,1,1,1,1,1,1,1,1,1,1,1,1,1,1,1,1,1,1,1,1,1,1,1,1,1,1,1,1,1,1,1,1,
1,1,1,1,1,1,1,1,1,1,1,1,1,1,1,1,1,1,1,1,1,1,1,1,1,1,1,1,1,1,1,1,1,1,1,1,
1,1,1,1,1,1,1,1,1,1,1,1,1,1,1,1,1,1,1,1,1,1,1,6),(-0.941429844431381,-0.940000000000001,
-0.935000000000001,-0.930000000000001,-0.925000000000001,-0.920000000000001,
-0.915000000000001,-0.910000000000001,-0.905000000000001,-0.900000000000001,
-0.895000000000001,-0.890000000000001,-0.885000000000001,-0.880000000000001,
-0.875000000000001,-0.870000000000001,-0.865000000000001,-0.860000000000001,
-0.855000000000001,-0.850000000000001,-0.845000000000001,-0.840000000000001,
-0.835000000000001,-0.830000000000001,-0.825000000000001,-0.820000000000001,
-0.815000000000001,-0.810000000000001,-0.805000000000001,-0.800000000000001,
-0.795000000000001,-0.790000000000001,-0.785000000000001,-0.780000000000001,
-0.775000000000001,-0.770000000000001,-0.765000000000001,-0.760000000000001,
-0.755000000000001,-0.750000000000001,-0.745000000000001,-0.740000000000001,
-0.735000000000001,-0.730000000000001,-0.725000000000001,-0.720000000000001,
-0.715000000000001,-0.710000000000001,-0.705000000000001,-0.700000000000001,
-0.695000000000001,-0.690000000000001,-0.685,-0.68,-0.675,-0.67,-0.665,
-0.66,-0.655,-0.65,-0.645,-0.64,-0.635,-0.63,-0.625,-0.62,-0.615,-0.61,
-0.605,-0.6,-0.595,-0.59,-0.585,-0.58,-0.575,-0.57,-0.565,-0.56,-0.555,
-0.55,-0.545,-0.54,-0.535,-0.53,-0.525,-0.52,-0.515,-0.51,-0.505,-0.5,-0.495,
-0.49,-0.485,-0.48,-0.475,-0.47,-0.465,-0.46,-0.455,-0.45,-0.445,-0.44,
-0.435,-0.43,-0.425,-0.42,-0.415,-0.41,-0.405,-0.4,-0.395,-0.39,-0.385,
-0.38,-0.375,-0.37,-0.365,-0.36,-0.355,-0.35,-0.345,-0.34,-0.335,-0.33,
-0.325,-0.32,-0.315,-0.31,-0.305,-0.3,-0.295,-0.29,-0.285,-0.28,-0.275,
-0.27,-0.265,-0.26,-0.255,-0.25,-0.245,-0.24,-0.235,-0.23,-0.225,-0.22,
-0.215,-0.21,-0.205,-0.2,-0.195,-0.19,-0.185,-0.18,-0.175,-0.17,-0.165,
-0.16,-0.155,-0.15,-0.145,-0.14,-0.135,-0.13,-0.125,-0.12,-0.115,-0.11,
-0.105,-0.1,-0.095,-0.09,-0.085,-0.08,-0.075,-0.07,-0.065,-0.06,-0.055,
-0.05,-0.045,-0.04,-0.035,-0.03,-0.025,-0.02,-0.015,-0.01,-0.005,0.),
 .UNSPECIFIED.)
CURVE()
GEOMETRIC_REPRESENTATION_ITEM()
RATIONAL_B_SPLINE_CURVE((1.,1.,1.,1.,1.,1.,1.,1.,1.,1.,1.,1.,1.,1.,1.,1.,
1.,1.,1.,1.,1.,1.,1.,1.,1.,1.,1.,1.,1.,1.,1.,1.,1.,1.,1.,1.,1.,1.,1.,1.,
1.,1.,1.,1.,1.,1.,1.,1.,1.,1.,1.,1.,1.,1.,1.,1.,1.,1.,1.,1.,1.,1.,1.,1.,
1.,1.,1.,1.,1.,1.,1.,1.,1.,1.,1.,1.,1.,1.,1.,1.,1.,1.,1.,1.,1.,1.,1.,1.,
1.,1.,1.,1.,1.,1.,1.,1.,1.,1.,1.,1.,1.,1.,1.,1.,1.,1.,1.,1.,1.,1.,1.,1.,
1.,1.,1.,1.,1.,1.,1.,1.,1.,1.,1.,1.,1.,1.,1.,1.,1.,1.,1.,1.,1.,1.,1.,1.,
1.,1.,1.,1.,1.,1.,1.,1.,1.,1.,1.,1.,1.,1.,1.,1.,1.,1.,1.,1.,1.,1.,1.,1.,
1.,1.,1.,1.,1.,1.,1.,1.,1.,1.,1.,1.,1.,1.,1.,1.,1.,1.,1.,1.,1.,1.,1.,1.,
1.,1.,1.,1.,1.,1.,1.,1.,1.,1.))
REPRESENTATION_ITEM('')
);
#543=(
BOUNDED_CURVE()
B_SPLINE_CURVE(5,(#115753,#115754,#115755,#115756,#115757,#115758,#115759,
#115760,#115761,#115762,#115763,#115764,#115765,#115766,#115767,#115768,
#115769,#115770,#115771,#115772,#115773,#115774,#115775,#115776,#115777,
#115778,#115779,#115780,#115781,#115782,#115783,#115784,#115785,#115786,
#115787,#115788,#115789,#115790,#115791,#115792,#115793,#115794,#115795,
#115796,#115797,#115798,#115799,#115800,#115801,#115802,#115803,#115804,
#115805,#115806,#115807,#115808,#115809,#115810,#115811,#115812,#115813,
#115814,#115815,#115816,#115817,#115818,#115819,#115820,#115821,#115822,
#115823,#115824,#115825,#115826,#115827,#115828,#115829,#115830,#115831,
#115832,#115833,#115834,#115835,#115836,#115837,#115838,#115839,#115840,
#115841,#115842,#115843,#115844,#115845,#115846,#115847,#115848,#115849,
#115850,#115851,#115852,#115853,#115854,#115855,#115856,#115857,#115858,
#115859,#115860,#115861,#115862,#115863,#115864,#115865,#115866,#115867,
#115868,#115869,#115870,#115871,#115872,#115873,#115874,#115875,#115876,
#115877,#115878,#115879,#115880,#115881,#115882,#115883,#115884,#115885,
#115886,#115887,#115888,#115889,#115890,#115891,#115892,#115893,#115894,
#115895,#115896,#115897,#115898,#115899,#115900,#115901,#115902,#115903,
#115904,#115905,#115906,#115907,#115908,#115909,#115910,#115911,#115912,
#115913,#115914,#115915,#115916,#115917,#115918,#115919,#115920,#115921,
#115922,#115923,#115924,#115925,#115926,#115927,#115928,#115929,#115930,
#115931,#115932,#115933,#115934,#115935,#115936,#115937,#115938,#115939,
#115940,#115941,#115942,#115943,#115944,#115945,#115946),.UNSPECIFIED.,
 .F.,.F.)
B_SPLINE_CURVE_WITH_KNOTS((6,1,1,1,1,1,1,1,1,1,1,1,1,1,1,1,1,1,1,1,1,1,
1,1,1,1,1,1,1,1,1,1,1,1,1,1,1,1,1,1,1,1,1,1,1,1,1,1,1,1,1,1,1,1,1,1,1,1,
1,1,1,1,1,1,1,1,1,1,1,1,1,1,1,1,1,1,1,1,1,1,1,1,1,1,1,1,1,1,1,1,1,1,1,1,
1,1,1,1,1,1,1,1,1,1,1,1,1,1,1,1,1,1,1,1,1,1,1,1,1,1,1,1,1,1,1,1,1,1,1,1,
1,1,1,1,1,1,1,1,1,1,1,1,1,1,1,1,1,1,1,1,1,1,1,1,1,1,1,1,1,1,1,1,1,1,1,1,
1,1,1,1,1,1,1,1,1,1,1,1,1,1,1,1,1,1,1,1,1,1,1,6),(0.,0.005,0.01,0.015,0.02,
0.025,0.03,0.035,0.04,0.045,0.05,0.055,0.06,0.065,0.07,0.075,0.08,0.085,
0.09,0.095,0.1,0.105,0.11,0.115,0.12,0.125,0.13,0.135,0.14,0.145,0.15,0.155,
0.16,0.165,0.17,0.175,0.18,0.185,0.19,0.195,0.2,0.205,0.21,0.215,0.22,0.225,
0.23,0.235,0.24,0.245,0.25,0.255,0.26,0.265,0.27,0.275,0.28,0.285,0.29,
0.295,0.3,0.305,0.31,0.315,0.32,0.325,0.33,0.335,0.34,0.345,0.35,0.355,
0.36,0.365,0.37,0.375,0.38,0.385,0.39,0.395,0.4,0.405,0.41,0.415,0.42,0.425,
0.43,0.435,0.44,0.445,0.45,0.455,0.46,0.465,0.47,0.475,0.48,0.485,0.49,
0.495,0.5,0.505,0.51,0.515,0.52,0.525,0.53,0.535,0.54,0.545,0.55,0.555,
0.56,0.565,0.57,0.575,0.58,0.585,0.59,0.595,0.6,0.605,0.61,0.615,0.62,0.625,
0.63,0.635,0.64,0.645,0.65,0.655,0.66,0.665,0.67,0.675,0.68,0.685,0.690000000000001,
0.695000000000001,0.700000000000001,0.705000000000001,0.710000000000001,
0.715000000000001,0.720000000000001,0.725000000000001,0.730000000000001,
0.735000000000001,0.740000000000001,0.745000000000001,0.750000000000001,
0.755000000000001,0.760000000000001,0.765000000000001,0.770000000000001,
0.775000000000001,0.780000000000001,0.785000000000001,0.790000000000001,
0.795000000000001,0.800000000000001,0.805000000000001,0.810000000000001,
0.815000000000001,0.820000000000001,0.825000000000001,0.830000000000001,
0.835000000000001,0.840000000000001,0.845000000000001,0.850000000000001,
0.855000000000001,0.860000000000001,0.865000000000001,0.870000000000001,
0.875000000000001,0.880000000000001,0.885000000000001,0.890000000000001,
0.895000000000001,0.900000000000001,0.905000000000001,0.910000000000001,
0.915000000000001,0.920000000000001,0.925000000000001,0.930000000000001,
0.935000000000001,0.940000000000001,0.941429844431474),.UNSPECIFIED.)
CURVE()
GEOMETRIC_REPRESENTATION_ITEM()
RATIONAL_B_SPLINE_CURVE((1.,1.,1.,1.,1.,1.,1.,1.,1.,1.,1.,1.,1.,1.,1.,1.,
1.,1.,1.,1.,1.,1.,1.,1.,1.,1.,1.,1.,1.,1.,1.,1.,1.,1.,1.,1.,1.,1.,1.,1.,
1.,1.,1.,1.,1.,1.,1.,1.,1.,1.,1.,1.,1.,1.,1.,1.,1.,1.,1.,1.,1.,1.,1.,1.,
1.,1.,1.,1.,1.,1.,1.,1.,1.,1.,1.,1.,1.,1.,1.,1.,1.,1.,1.,1.,1.,1.,1.,1.,
1.,1.,1.,1.,1.,1.,1.,1.,1.,1.,1.,1.,1.,1.,1.,1.,1.,1.,1.,1.,1.,1.,1.,1.,
1.,1.,1.,1.,1.,1.,1.,1.,1.,1.,1.,1.,1.,1.,1.,1.,1.,1.,1.,1.,1.,1.,1.,1.,
1.,1.,1.,1.,1.,1.,1.,1.,1.,1.,1.,1.,1.,1.,1.,1.,1.,1.,1.,1.,1.,1.,1.,1.,
1.,1.,1.,1.,1.,1.,1.,1.,1.,1.,1.,1.,1.,1.,1.,1.,1.,1.,1.,1.,1.,1.,1.,1.,
1.,1.,1.,1.,1.,1.,1.,1.,1.,1.))
REPRESENTATION_ITEM('')
);
#544=(
BOUNDED_CURVE()
B_SPLINE_CURVE(5,(#115949,#115950,#115951,#115952,#115953,#115954,#115955,
#115956,#115957,#115958,#115959,#115960,#115961,#115962,#115963,#115964,
#115965,#115966,#115967,#115968,#115969,#115970,#115971,#115972,#115973,
#115974,#115975,#115976,#115977,#115978,#115979,#115980,#115981,#115982,
#115983,#115984,#115985,#115986,#115987,#115988,#115989,#115990,#115991,
#115992,#115993,#115994,#115995,#115996,#115997,#115998,#115999,#116000,
#116001,#116002,#116003,#116004,#116005,#116006,#116007,#116008,#116009,
#116010,#116011,#116012,#116013,#116014,#116015,#116016,#116017,#116018,
#116019,#116020,#116021,#116022,#116023,#116024,#116025,#116026,#116027,
#116028,#116029,#116030,#116031,#116032,#116033,#116034,#116035,#116036,
#116037,#116038,#116039,#116040,#116041,#116042,#116043,#116044,#116045,
#116046,#116047,#116048,#116049,#116050,#116051,#116052,#116053,#116054,
#116055,#116056,#116057,#116058,#116059,#116060,#116061,#116062,#116063,
#116064,#116065,#116066,#116067,#116068,#116069,#116070,#116071,#116072,
#116073,#116074,#116075,#116076,#116077,#116078,#116079,#116080,#116081,
#116082,#116083,#116084,#116085,#116086,#116087,#116088,#116089,#116090,
#116091,#116092,#116093,#116094,#116095,#116096,#116097,#116098,#116099,
#116100,#116101,#116102,#116103,#116104,#116105,#116106,#116107,#116108,
#116109,#116110,#116111,#116112,#116113,#116114,#116115,#116116,#116117,
#116118,#116119,#116120,#116121,#116122,#116123,#116124,#116125,#116126,
#116127,#116128,#116129,#116130,#116131,#116132,#116133,#116134,#116135,
#116136,#116137,#116138,#116139,#116140,#116141,#116142),.UNSPECIFIED.,
 .F.,.F.)
B_SPLINE_CURVE_WITH_KNOTS((6,1,1,1,1,1,1,1,1,1,1,1,1,1,1,1,1,1,1,1,1,1,
1,1,1,1,1,1,1,1,1,1,1,1,1,1,1,1,1,1,1,1,1,1,1,1,1,1,1,1,1,1,1,1,1,1,1,1,
1,1,1,1,1,1,1,1,1,1,1,1,1,1,1,1,1,1,1,1,1,1,1,1,1,1,1,1,1,1,1,1,1,1,1,1,
1,1,1,1,1,1,1,1,1,1,1,1,1,1,1,1,1,1,1,1,1,1,1,1,1,1,1,1,1,1,1,1,1,1,1,1,
1,1,1,1,1,1,1,1,1,1,1,1,1,1,1,1,1,1,1,1,1,1,1,1,1,1,1,1,1,1,1,1,1,1,1,1,
1,1,1,1,1,1,1,1,1,1,1,1,1,1,1,1,1,1,1,1,1,1,1,6),(-0.941429844431504,-0.940000000000001,
-0.935000000000001,-0.930000000000001,-0.925000000000001,-0.920000000000001,
-0.915000000000001,-0.910000000000001,-0.905000000000001,-0.900000000000001,
-0.895000000000001,-0.890000000000001,-0.885000000000001,-0.880000000000001,
-0.875000000000001,-0.870000000000001,-0.865000000000001,-0.860000000000001,
-0.855000000000001,-0.850000000000001,-0.845000000000001,-0.840000000000001,
-0.835000000000001,-0.830000000000001,-0.825000000000001,-0.820000000000001,
-0.815000000000001,-0.810000000000001,-0.805000000000001,-0.800000000000001,
-0.795000000000001,-0.790000000000001,-0.785000000000001,-0.780000000000001,
-0.775000000000001,-0.770000000000001,-0.765000000000001,-0.760000000000001,
-0.755000000000001,-0.750000000000001,-0.745000000000001,-0.740000000000001,
-0.735000000000001,-0.730000000000001,-0.725000000000001,-0.720000000000001,
-0.715000000000001,-0.710000000000001,-0.705000000000001,-0.700000000000001,
-0.695000000000001,-0.690000000000001,-0.685,-0.68,-0.675,-0.67,-0.665,
-0.66,-0.655,-0.65,-0.645,-0.64,-0.635,-0.63,-0.625,-0.62,-0.615,-0.61,
-0.605,-0.6,-0.595,-0.59,-0.585,-0.58,-0.575,-0.57,-0.565,-0.56,-0.555,
-0.55,-0.545,-0.54,-0.535,-0.53,-0.525,-0.52,-0.515,-0.51,-0.505,-0.5,-0.495,
-0.49,-0.485,-0.48,-0.475,-0.47,-0.465,-0.46,-0.455,-0.45,-0.445,-0.44,
-0.435,-0.43,-0.425,-0.42,-0.415,-0.41,-0.405,-0.4,-0.395,-0.39,-0.385,
-0.38,-0.375,-0.37,-0.365,-0.36,-0.355,-0.35,-0.345,-0.34,-0.335,-0.33,
-0.325,-0.32,-0.315,-0.31,-0.305,-0.3,-0.295,-0.29,-0.285,-0.28,-0.275,
-0.27,-0.265,-0.26,-0.255,-0.25,-0.245,-0.24,-0.235,-0.23,-0.225,-0.22,
-0.215,-0.21,-0.205,-0.2,-0.195,-0.19,-0.185,-0.18,-0.175,-0.17,-0.165,
-0.16,-0.155,-0.15,-0.145,-0.14,-0.135,-0.13,-0.125,-0.12,-0.115,-0.11,
-0.105,-0.1,-0.095,-0.09,-0.085,-0.08,-0.075,-0.07,-0.065,-0.06,-0.055,
-0.05,-0.045,-0.04,-0.035,-0.03,-0.025,-0.02,-0.015,-0.01,-0.005,0.),
 .UNSPECIFIED.)
CURVE()
GEOMETRIC_REPRESENTATION_ITEM()
RATIONAL_B_SPLINE_CURVE((1.,1.,1.,1.,1.,1.,1.,1.,1.,1.,1.,1.,1.,1.,1.,1.,
1.,1.,1.,1.,1.,1.,1.,1.,1.,1.,1.,1.,1.,1.,1.,1.,1.,1.,1.,1.,1.,1.,1.,1.,
1.,1.,1.,1.,1.,1.,1.,1.,1.,1.,1.,1.,1.,1.,1.,1.,1.,1.,1.,1.,1.,1.,1.,1.,
1.,1.,1.,1.,1.,1.,1.,1.,1.,1.,1.,1.,1.,1.,1.,1.,1.,1.,1.,1.,1.,1.,1.,1.,
1.,1.,1.,1.,1.,1.,1.,1.,1.,1.,1.,1.,1.,1.,1.,1.,1.,1.,1.,1.,1.,1.,1.,1.,
1.,1.,1.,1.,1.,1.,1.,1.,1.,1.,1.,1.,1.,1.,1.,1.,1.,1.,1.,1.,1.,1.,1.,1.,
1.,1.,1.,1.,1.,1.,1.,1.,1.,1.,1.,1.,1.,1.,1.,1.,1.,1.,1.,1.,1.,1.,1.,1.,
1.,1.,1.,1.,1.,1.,1.,1.,1.,1.,1.,1.,1.,1.,1.,1.,1.,1.,1.,1.,1.,1.,1.,1.,
1.,1.,1.,1.,1.,1.,1.,1.,1.,1.))
REPRESENTATION_ITEM('')
);
#545=(
BOUNDED_CURVE()
B_SPLINE_CURVE(5,(#116603,#116604,#116605,#116606,#116607,#116608,#116609,
#116610,#116611,#116612,#116613,#116614,#116615,#116616,#116617,#116618,
#116619,#116620,#116621,#116622,#116623,#116624,#116625,#116626,#116627,
#116628,#116629,#116630,#116631,#116632,#116633,#116634,#116635,#116636,
#116637,#116638,#116639,#116640,#116641,#116642,#116643,#116644,#116645,
#116646,#116647,#116648,#116649,#116650,#116651,#116652,#116653,#116654,
#116655,#116656,#116657,#116658,#116659,#116660,#116661,#116662,#116663,
#116664,#116665,#116666,#116667,#116668,#116669,#116670,#116671,#116672,
#116673,#116674,#116675,#116676,#116677,#116678,#116679,#116680,#116681,
#116682,#116683,#116684,#116685,#116686,#116687,#116688,#116689,#116690,
#116691,#116692,#116693,#116694,#116695,#116696,#116697,#116698,#116699,
#116700,#116701,#116702,#116703,#116704,#116705,#116706,#116707,#116708,
#116709,#116710,#116711,#116712,#116713,#116714,#116715,#116716,#116717,
#116718,#116719,#116720,#116721,#116722,#116723,#116724,#116725,#116726,
#116727,#116728,#116729,#116730,#116731,#116732,#116733,#116734,#116735,
#116736,#116737,#116738,#116739,#116740,#116741,#116742,#116743,#116744,
#116745,#116746,#116747,#116748,#116749,#116750,#116751,#116752,#116753,
#116754,#116755,#116756,#116757,#116758,#116759,#116760,#116761,#116762,
#116763,#116764,#116765,#116766,#116767,#116768,#116769,#116770,#116771,
#116772,#116773,#116774,#116775,#116776,#116777,#116778,#116779,#116780,
#116781,#116782,#116783,#116784,#116785,#116786,#116787,#116788,#116789,
#116790,#116791,#116792,#116793,#116794,#116795,#116796),.UNSPECIFIED.,
 .F.,.F.)
B_SPLINE_CURVE_WITH_KNOTS((6,1,1,1,1,1,1,1,1,1,1,1,1,1,1,1,1,1,1,1,1,1,
1,1,1,1,1,1,1,1,1,1,1,1,1,1,1,1,1,1,1,1,1,1,1,1,1,1,1,1,1,1,1,1,1,1,1,1,
1,1,1,1,1,1,1,1,1,1,1,1,1,1,1,1,1,1,1,1,1,1,1,1,1,1,1,1,1,1,1,1,1,1,1,1,
1,1,1,1,1,1,1,1,1,1,1,1,1,1,1,1,1,1,1,1,1,1,1,1,1,1,1,1,1,1,1,1,1,1,1,1,
1,1,1,1,1,1,1,1,1,1,1,1,1,1,1,1,1,1,1,1,1,1,1,1,1,1,1,1,1,1,1,1,1,1,1,1,
1,1,1,1,1,1,1,1,1,1,1,1,1,1,1,1,1,1,1,1,1,1,1,6),(0.,0.005,0.01,0.015,0.02,
0.025,0.03,0.035,0.04,0.045,0.05,0.055,0.06,0.065,0.07,0.075,0.08,0.085,
0.09,0.095,0.1,0.105,0.11,0.115,0.12,0.125,0.13,0.135,0.14,0.145,0.15,0.155,
0.16,0.165,0.17,0.175,0.18,0.185,0.19,0.195,0.2,0.205,0.21,0.215,0.22,0.225,
0.23,0.235,0.24,0.245,0.25,0.255,0.26,0.265,0.27,0.275,0.28,0.285,0.29,
0.295,0.3,0.305,0.31,0.315,0.32,0.325,0.33,0.335,0.34,0.345,0.35,0.355,
0.36,0.365,0.37,0.375,0.38,0.385,0.39,0.395,0.4,0.405,0.41,0.415,0.42,0.425,
0.43,0.435,0.44,0.445,0.45,0.455,0.46,0.465,0.47,0.475,0.48,0.485,0.49,
0.495,0.5,0.505,0.51,0.515,0.52,0.525,0.53,0.535,0.54,0.545,0.55,0.555,
0.56,0.565,0.57,0.575,0.58,0.585,0.59,0.595,0.6,0.605,0.61,0.615,0.62,0.625,
0.63,0.635,0.64,0.645,0.65,0.655,0.66,0.665,0.67,0.675,0.68,0.685,0.690000000000001,
0.695000000000001,0.700000000000001,0.705000000000001,0.710000000000001,
0.715000000000001,0.720000000000001,0.725000000000001,0.730000000000001,
0.735000000000001,0.740000000000001,0.745000000000001,0.750000000000001,
0.755000000000001,0.760000000000001,0.765000000000001,0.770000000000001,
0.775000000000001,0.780000000000001,0.785000000000001,0.790000000000001,
0.795000000000001,0.800000000000001,0.805000000000001,0.810000000000001,
0.815000000000001,0.820000000000001,0.825000000000001,0.830000000000001,
0.835000000000001,0.840000000000001,0.845000000000001,0.850000000000001,
0.855000000000001,0.860000000000001,0.865000000000001,0.870000000000001,
0.875000000000001,0.880000000000001,0.885000000000001,0.890000000000001,
0.895000000000001,0.900000000000001,0.905000000000001,0.910000000000001,
0.915000000000001,0.920000000000001,0.925000000000001,0.930000000000001,
0.935000000000001,0.940000000000001,0.941429844438054),.UNSPECIFIED.)
CURVE()
GEOMETRIC_REPRESENTATION_ITEM()
RATIONAL_B_SPLINE_CURVE((1.,1.,1.,1.,1.,1.,1.,1.,1.,1.,1.,1.,1.,1.,1.,1.,
1.,1.,1.,1.,1.,1.,1.,1.,1.,1.,1.,1.,1.,1.,1.,1.,1.,1.,1.,1.,1.,1.,1.,1.,
1.,1.,1.,1.,1.,1.,1.,1.,1.,1.,1.,1.,1.,1.,1.,1.,1.,1.,1.,1.,1.,1.,1.,1.,
1.,1.,1.,1.,1.,1.,1.,1.,1.,1.,1.,1.,1.,1.,1.,1.,1.,1.,1.,1.,1.,1.,1.,1.,
1.,1.,1.,1.,1.,1.,1.,1.,1.,1.,1.,1.,1.,1.,1.,1.,1.,1.,1.,1.,1.,1.,1.,1.,
1.,1.,1.,1.,1.,1.,1.,1.,1.,1.,1.,1.,1.,1.,1.,1.,1.,1.,1.,1.,1.,1.,1.,1.,
1.,1.,1.,1.,1.,1.,1.,1.,1.,1.,1.,1.,1.,1.,1.,1.,1.,1.,1.,1.,1.,1.,1.,1.,
1.,1.,1.,1.,1.,1.,1.,1.,1.,1.,1.,1.,1.,1.,1.,1.,1.,1.,1.,1.,1.,1.,1.,1.,
1.,1.,1.,1.,1.,1.,1.,1.,1.,1.))
REPRESENTATION_ITEM('')
);
#546=(
BOUNDED_CURVE()
B_SPLINE_CURVE(5,(#116799,#116800,#116801,#116802,#116803,#116804,#116805,
#116806,#116807,#116808,#116809,#116810,#116811,#116812,#116813,#116814,
#116815,#116816,#116817,#116818,#116819,#116820,#116821,#116822,#116823,
#116824,#116825,#116826,#116827,#116828,#116829,#116830,#116831,#116832,
#116833,#116834,#116835,#116836,#116837,#116838,#116839,#116840,#116841,
#116842,#116843,#116844,#116845,#116846,#116847,#116848,#116849,#116850,
#116851,#116852,#116853,#116854,#116855,#116856,#116857,#116858,#116859,
#116860,#116861,#116862,#116863,#116864,#116865,#116866,#116867,#116868,
#116869,#116870,#116871,#116872,#116873,#116874,#116875,#116876,#116877,
#116878,#116879,#116880,#116881,#116882,#116883,#116884,#116885,#116886,
#116887,#116888,#116889,#116890,#116891,#116892,#116893,#116894,#116895,
#116896,#116897,#116898,#116899,#116900,#116901,#116902,#116903,#116904,
#116905,#116906,#116907,#116908,#116909,#116910,#116911,#116912,#116913,
#116914,#116915,#116916,#116917,#116918,#116919,#116920,#116921,#116922,
#116923,#116924,#116925,#116926,#116927,#116928,#116929,#116930,#116931,
#116932,#116933,#116934,#116935,#116936,#116937,#116938,#116939,#116940,
#116941,#116942,#116943,#116944,#116945,#116946,#116947,#116948,#116949,
#116950,#116951,#116952,#116953,#116954,#116955,#116956,#116957,#116958,
#116959,#116960,#116961,#116962,#116963,#116964,#116965,#116966,#116967,
#116968,#116969,#116970,#116971,#116972,#116973,#116974,#116975,#116976,
#116977,#116978,#116979,#116980,#116981,#116982,#116983,#116984,#116985,
#116986,#116987,#116988,#116989,#116990,#116991,#116992),.UNSPECIFIED.,
 .F.,.F.)
B_SPLINE_CURVE_WITH_KNOTS((6,1,1,1,1,1,1,1,1,1,1,1,1,1,1,1,1,1,1,1,1,1,
1,1,1,1,1,1,1,1,1,1,1,1,1,1,1,1,1,1,1,1,1,1,1,1,1,1,1,1,1,1,1,1,1,1,1,1,
1,1,1,1,1,1,1,1,1,1,1,1,1,1,1,1,1,1,1,1,1,1,1,1,1,1,1,1,1,1,1,1,1,1,1,1,
1,1,1,1,1,1,1,1,1,1,1,1,1,1,1,1,1,1,1,1,1,1,1,1,1,1,1,1,1,1,1,1,1,1,1,1,
1,1,1,1,1,1,1,1,1,1,1,1,1,1,1,1,1,1,1,1,1,1,1,1,1,1,1,1,1,1,1,1,1,1,1,1,
1,1,1,1,1,1,1,1,1,1,1,1,1,1,1,1,1,1,1,1,1,1,1,6),(-0.941429844438061,-0.940000000000001,
-0.935000000000001,-0.930000000000001,-0.925000000000001,-0.920000000000001,
-0.915000000000001,-0.910000000000001,-0.905000000000001,-0.900000000000001,
-0.895000000000001,-0.890000000000001,-0.885000000000001,-0.880000000000001,
-0.875000000000001,-0.870000000000001,-0.865000000000001,-0.860000000000001,
-0.855000000000001,-0.850000000000001,-0.845000000000001,-0.840000000000001,
-0.835000000000001,-0.830000000000001,-0.825000000000001,-0.820000000000001,
-0.815000000000001,-0.810000000000001,-0.805000000000001,-0.800000000000001,
-0.795000000000001,-0.790000000000001,-0.785000000000001,-0.780000000000001,
-0.775000000000001,-0.770000000000001,-0.765000000000001,-0.760000000000001,
-0.755000000000001,-0.750000000000001,-0.745000000000001,-0.740000000000001,
-0.735000000000001,-0.730000000000001,-0.725000000000001,-0.720000000000001,
-0.715000000000001,-0.710000000000001,-0.705000000000001,-0.700000000000001,
-0.695000000000001,-0.690000000000001,-0.685,-0.68,-0.675,-0.67,-0.665,
-0.66,-0.655,-0.65,-0.645,-0.64,-0.635,-0.63,-0.625,-0.62,-0.615,-0.61,
-0.605,-0.6,-0.595,-0.59,-0.585,-0.58,-0.575,-0.57,-0.565,-0.56,-0.555,
-0.55,-0.545,-0.54,-0.535,-0.53,-0.525,-0.52,-0.515,-0.51,-0.505,-0.5,-0.495,
-0.49,-0.485,-0.48,-0.475,-0.47,-0.465,-0.46,-0.455,-0.45,-0.445,-0.44,
-0.435,-0.43,-0.425,-0.42,-0.415,-0.41,-0.405,-0.4,-0.395,-0.39,-0.385,
-0.38,-0.375,-0.37,-0.365,-0.36,-0.355,-0.35,-0.345,-0.34,-0.335,-0.33,
-0.325,-0.32,-0.315,-0.31,-0.305,-0.3,-0.295,-0.29,-0.285,-0.28,-0.275,
-0.27,-0.265,-0.26,-0.255,-0.25,-0.245,-0.24,-0.235,-0.23,-0.225,-0.22,
-0.215,-0.21,-0.205,-0.2,-0.195,-0.19,-0.185,-0.18,-0.175,-0.17,-0.165,
-0.16,-0.155,-0.15,-0.145,-0.14,-0.135,-0.13,-0.125,-0.12,-0.115,-0.11,
-0.105,-0.1,-0.095,-0.09,-0.085,-0.08,-0.075,-0.07,-0.065,-0.06,-0.055,
-0.05,-0.045,-0.04,-0.035,-0.03,-0.025,-0.02,-0.015,-0.01,-0.005,0.),
 .UNSPECIFIED.)
CURVE()
GEOMETRIC_REPRESENTATION_ITEM()
RATIONAL_B_SPLINE_CURVE((1.,1.,1.,1.,1.,1.,1.,1.,1.,1.,1.,1.,1.,1.,1.,1.,
1.,1.,1.,1.,1.,1.,1.,1.,1.,1.,1.,1.,1.,1.,1.,1.,1.,1.,1.,1.,1.,1.,1.,1.,
1.,1.,1.,1.,1.,1.,1.,1.,1.,1.,1.,1.,1.,1.,1.,1.,1.,1.,1.,1.,1.,1.,1.,1.,
1.,1.,1.,1.,1.,1.,1.,1.,1.,1.,1.,1.,1.,1.,1.,1.,1.,1.,1.,1.,1.,1.,1.,1.,
1.,1.,1.,1.,1.,1.,1.,1.,1.,1.,1.,1.,1.,1.,1.,1.,1.,1.,1.,1.,1.,1.,1.,1.,
1.,1.,1.,1.,1.,1.,1.,1.,1.,1.,1.,1.,1.,1.,1.,1.,1.,1.,1.,1.,1.,1.,1.,1.,
1.,1.,1.,1.,1.,1.,1.,1.,1.,1.,1.,1.,1.,1.,1.,1.,1.,1.,1.,1.,1.,1.,1.,1.,
1.,1.,1.,1.,1.,1.,1.,1.,1.,1.,1.,1.,1.,1.,1.,1.,1.,1.,1.,1.,1.,1.,1.,1.,
1.,1.,1.,1.,1.,1.,1.,1.,1.,1.))
REPRESENTATION_ITEM('')
);
#547=(
BOUNDED_CURVE()
B_SPLINE_CURVE(5,(#117404,#117405,#117406,#117407,#117408,#117409,#117410,
#117411,#117412,#117413,#117414,#117415,#117416,#117417,#117418,#117419,
#117420,#117421,#117422,#117423,#117424,#117425,#117426,#117427,#117428,
#117429,#117430,#117431,#117432,#117433,#117434,#117435,#117436,#117437,
#117438,#117439,#117440,#117441,#117442,#117443,#117444,#117445,#117446,
#117447,#117448,#117449,#117450,#117451,#117452,#117453,#117454,#117455,
#117456,#117457,#117458,#117459,#117460,#117461,#117462,#117463,#117464,
#117465,#117466,#117467,#117468,#117469,#117470,#117471,#117472,#117473,
#117474,#117475,#117476,#117477,#117478,#117479,#117480,#117481,#117482,
#117483,#117484,#117485,#117486,#117487,#117488,#117489,#117490,#117491,
#117492,#117493,#117494,#117495,#117496,#117497,#117498,#117499,#117500,
#117501,#117502,#117503,#117504,#117505,#117506,#117507,#117508,#117509,
#117510,#117511,#117512,#117513,#117514,#117515,#117516,#117517,#117518,
#117519,#117520,#117521,#117522,#117523,#117524,#117525,#117526,#117527,
#117528,#117529,#117530,#117531,#117532,#117533,#117534,#117535,#117536,
#117537,#117538,#117539,#117540,#117541,#117542,#117543,#117544,#117545,
#117546,#117547,#117548,#117549,#117550,#117551,#117552,#117553,#117554,
#117555,#117556,#117557,#117558,#117559,#117560,#117561,#117562,#117563,
#117564,#117565,#117566,#117567,#117568,#117569,#117570,#117571,#117572,
#117573,#117574,#117575,#117576,#117577,#117578,#117579,#117580,#117581,
#117582,#117583,#117584,#117585,#117586,#117587,#117588,#117589,#117590,
#117591,#117592,#117593,#117594,#117595,#117596,#117597),.UNSPECIFIED.,
 .F.,.F.)
B_SPLINE_CURVE_WITH_KNOTS((6,1,1,1,1,1,1,1,1,1,1,1,1,1,1,1,1,1,1,1,1,1,
1,1,1,1,1,1,1,1,1,1,1,1,1,1,1,1,1,1,1,1,1,1,1,1,1,1,1,1,1,1,1,1,1,1,1,1,
1,1,1,1,1,1,1,1,1,1,1,1,1,1,1,1,1,1,1,1,1,1,1,1,1,1,1,1,1,1,1,1,1,1,1,1,
1,1,1,1,1,1,1,1,1,1,1,1,1,1,1,1,1,1,1,1,1,1,1,1,1,1,1,1,1,1,1,1,1,1,1,1,
1,1,1,1,1,1,1,1,1,1,1,1,1,1,1,1,1,1,1,1,1,1,1,1,1,1,1,1,1,1,1,1,1,1,1,1,
1,1,1,1,1,1,1,1,1,1,1,1,1,1,1,1,1,1,1,1,1,1,1,6),(0.,0.005,0.01,0.015,0.02,
0.025,0.03,0.035,0.04,0.045,0.05,0.055,0.06,0.065,0.07,0.075,0.08,0.085,
0.09,0.095,0.1,0.105,0.11,0.115,0.12,0.125,0.13,0.135,0.14,0.145,0.15,0.155,
0.16,0.165,0.17,0.175,0.18,0.185,0.19,0.195,0.2,0.205,0.21,0.215,0.22,0.225,
0.23,0.235,0.24,0.245,0.25,0.255,0.26,0.265,0.27,0.275,0.28,0.285,0.29,
0.295,0.3,0.305,0.31,0.315,0.32,0.325,0.33,0.335,0.34,0.345,0.35,0.355,
0.36,0.365,0.37,0.375,0.38,0.385,0.39,0.395,0.4,0.405,0.41,0.415,0.42,0.425,
0.43,0.435,0.44,0.445,0.45,0.455,0.46,0.465,0.47,0.475,0.48,0.485,0.49,
0.495,0.5,0.505,0.51,0.515,0.52,0.525,0.53,0.535,0.54,0.545,0.55,0.555,
0.56,0.565,0.57,0.575,0.58,0.585,0.59,0.595,0.6,0.605,0.61,0.615,0.62,0.625,
0.63,0.635,0.64,0.645,0.65,0.655,0.66,0.665,0.67,0.675,0.68,0.685,0.690000000000001,
0.695000000000001,0.700000000000001,0.705000000000001,0.710000000000001,
0.715000000000001,0.720000000000001,0.725000000000001,0.730000000000001,
0.735000000000001,0.740000000000001,0.745000000000001,0.750000000000001,
0.755000000000001,0.760000000000001,0.765000000000001,0.770000000000001,
0.775000000000001,0.780000000000001,0.785000000000001,0.790000000000001,
0.795000000000001,0.800000000000001,0.805000000000001,0.810000000000001,
0.815000000000001,0.820000000000001,0.825000000000001,0.830000000000001,
0.835000000000001,0.840000000000001,0.845000000000001,0.850000000000001,
0.855000000000001,0.860000000000001,0.865000000000001,0.870000000000001,
0.875000000000001,0.880000000000001,0.885000000000001,0.890000000000001,
0.895000000000001,0.900000000000001,0.905000000000001,0.910000000000001,
0.915000000000001,0.920000000000001,0.925000000000001,0.930000000000001,
0.935000000000001,0.940000000000001,0.9414298444381),.UNSPECIFIED.)
CURVE()
GEOMETRIC_REPRESENTATION_ITEM()
RATIONAL_B_SPLINE_CURVE((1.,1.,1.,1.,1.,1.,1.,1.,1.,1.,1.,1.,1.,1.,1.,1.,
1.,1.,1.,1.,1.,1.,1.,1.,1.,1.,1.,1.,1.,1.,1.,1.,1.,1.,1.,1.,1.,1.,1.,1.,
1.,1.,1.,1.,1.,1.,1.,1.,1.,1.,1.,1.,1.,1.,1.,1.,1.,1.,1.,1.,1.,1.,1.,1.,
1.,1.,1.,1.,1.,1.,1.,1.,1.,1.,1.,1.,1.,1.,1.,1.,1.,1.,1.,1.,1.,1.,1.,1.,
1.,1.,1.,1.,1.,1.,1.,1.,1.,1.,1.,1.,1.,1.,1.,1.,1.,1.,1.,1.,1.,1.,1.,1.,
1.,1.,1.,1.,1.,1.,1.,1.,1.,1.,1.,1.,1.,1.,1.,1.,1.,1.,1.,1.,1.,1.,1.,1.,
1.,1.,1.,1.,1.,1.,1.,1.,1.,1.,1.,1.,1.,1.,1.,1.,1.,1.,1.,1.,1.,1.,1.,1.,
1.,1.,1.,1.,1.,1.,1.,1.,1.,1.,1.,1.,1.,1.,1.,1.,1.,1.,1.,1.,1.,1.,1.,1.,
1.,1.,1.,1.,1.,1.,1.,1.,1.,1.))
REPRESENTATION_ITEM('')
);
#548=(
BOUNDED_CURVE()
B_SPLINE_CURVE(5,(#117600,#117601,#117602,#117603,#117604,#117605,#117606,
#117607,#117608,#117609,#117610,#117611,#117612,#117613,#117614,#117615,
#117616,#117617,#117618,#117619,#117620,#117621,#117622,#117623,#117624,
#117625,#117626,#117627,#117628,#117629,#117630,#117631,#117632,#117633,
#117634,#117635,#117636,#117637,#117638,#117639,#117640,#117641,#117642,
#117643,#117644,#117645,#117646,#117647,#117648,#117649,#117650,#117651,
#117652,#117653,#117654,#117655,#117656,#117657,#117658,#117659,#117660,
#117661,#117662,#117663,#117664,#117665,#117666,#117667,#117668,#117669,
#117670,#117671,#117672,#117673,#117674,#117675,#117676,#117677,#117678,
#117679,#117680,#117681,#117682,#117683,#117684,#117685,#117686,#117687,
#117688,#117689,#117690,#117691,#117692,#117693,#117694,#117695,#117696,
#117697,#117698,#117699,#117700,#117701,#117702,#117703,#117704,#117705,
#117706,#117707,#117708,#117709,#117710,#117711,#117712,#117713,#117714,
#117715,#117716,#117717,#117718,#117719,#117720,#117721,#117722,#117723,
#117724,#117725,#117726,#117727,#117728,#117729,#117730,#117731,#117732,
#117733,#117734,#117735,#117736,#117737,#117738,#117739,#117740,#117741,
#117742,#117743,#117744,#117745,#117746,#117747,#117748,#117749,#117750,
#117751,#117752,#117753,#117754,#117755,#117756,#117757,#117758,#117759,
#117760,#117761,#117762,#117763,#117764,#117765,#117766,#117767,#117768,
#117769,#117770,#117771,#117772,#117773,#117774,#117775,#117776,#117777,
#117778,#117779,#117780,#117781,#117782,#117783,#117784,#117785,#117786,
#117787,#117788,#117789,#117790,#117791,#117792,#117793),.UNSPECIFIED.,
 .F.,.F.)
B_SPLINE_CURVE_WITH_KNOTS((6,1,1,1,1,1,1,1,1,1,1,1,1,1,1,1,1,1,1,1,1,1,
1,1,1,1,1,1,1,1,1,1,1,1,1,1,1,1,1,1,1,1,1,1,1,1,1,1,1,1,1,1,1,1,1,1,1,1,
1,1,1,1,1,1,1,1,1,1,1,1,1,1,1,1,1,1,1,1,1,1,1,1,1,1,1,1,1,1,1,1,1,1,1,1,
1,1,1,1,1,1,1,1,1,1,1,1,1,1,1,1,1,1,1,1,1,1,1,1,1,1,1,1,1,1,1,1,1,1,1,1,
1,1,1,1,1,1,1,1,1,1,1,1,1,1,1,1,1,1,1,1,1,1,1,1,1,1,1,1,1,1,1,1,1,1,1,1,
1,1,1,1,1,1,1,1,1,1,1,1,1,1,1,1,1,1,1,1,1,1,1,6),(-0.941429844438093,-0.940000000000001,
-0.935000000000001,-0.930000000000001,-0.925000000000001,-0.920000000000001,
-0.915000000000001,-0.910000000000001,-0.905000000000001,-0.900000000000001,
-0.895000000000001,-0.890000000000001,-0.885000000000001,-0.880000000000001,
-0.875000000000001,-0.870000000000001,-0.865000000000001,-0.860000000000001,
-0.855000000000001,-0.850000000000001,-0.845000000000001,-0.840000000000001,
-0.835000000000001,-0.830000000000001,-0.825000000000001,-0.820000000000001,
-0.815000000000001,-0.810000000000001,-0.805000000000001,-0.800000000000001,
-0.795000000000001,-0.790000000000001,-0.785000000000001,-0.780000000000001,
-0.775000000000001,-0.770000000000001,-0.765000000000001,-0.760000000000001,
-0.755000000000001,-0.750000000000001,-0.745000000000001,-0.740000000000001,
-0.735000000000001,-0.730000000000001,-0.725000000000001,-0.720000000000001,
-0.715000000000001,-0.710000000000001,-0.705000000000001,-0.700000000000001,
-0.695000000000001,-0.690000000000001,-0.685,-0.68,-0.675,-0.67,-0.665,
-0.66,-0.655,-0.65,-0.645,-0.64,-0.635,-0.63,-0.625,-0.62,-0.615,-0.61,
-0.605,-0.6,-0.595,-0.59,-0.585,-0.58,-0.575,-0.57,-0.565,-0.56,-0.555,
-0.55,-0.545,-0.54,-0.535,-0.53,-0.525,-0.52,-0.515,-0.51,-0.505,-0.5,-0.495,
-0.49,-0.485,-0.48,-0.475,-0.47,-0.465,-0.46,-0.455,-0.45,-0.445,-0.44,
-0.435,-0.43,-0.425,-0.42,-0.415,-0.41,-0.405,-0.4,-0.395,-0.39,-0.385,
-0.38,-0.375,-0.37,-0.365,-0.36,-0.355,-0.35,-0.345,-0.34,-0.335,-0.33,
-0.325,-0.32,-0.315,-0.31,-0.305,-0.3,-0.295,-0.29,-0.285,-0.28,-0.275,
-0.27,-0.265,-0.26,-0.255,-0.25,-0.245,-0.24,-0.235,-0.23,-0.225,-0.22,
-0.215,-0.21,-0.205,-0.2,-0.195,-0.19,-0.185,-0.18,-0.175,-0.17,-0.165,
-0.16,-0.155,-0.15,-0.145,-0.14,-0.135,-0.13,-0.125,-0.12,-0.115,-0.11,
-0.105,-0.1,-0.095,-0.09,-0.085,-0.08,-0.075,-0.07,-0.065,-0.06,-0.055,
-0.05,-0.045,-0.04,-0.035,-0.03,-0.025,-0.02,-0.015,-0.01,-0.005,0.),
 .UNSPECIFIED.)
CURVE()
GEOMETRIC_REPRESENTATION_ITEM()
RATIONAL_B_SPLINE_CURVE((1.,1.,1.,1.,1.,1.,1.,1.,1.,1.,1.,1.,1.,1.,1.,1.,
1.,1.,1.,1.,1.,1.,1.,1.,1.,1.,1.,1.,1.,1.,1.,1.,1.,1.,1.,1.,1.,1.,1.,1.,
1.,1.,1.,1.,1.,1.,1.,1.,1.,1.,1.,1.,1.,1.,1.,1.,1.,1.,1.,1.,1.,1.,1.,1.,
1.,1.,1.,1.,1.,1.,1.,1.,1.,1.,1.,1.,1.,1.,1.,1.,1.,1.,1.,1.,1.,1.,1.,1.,
1.,1.,1.,1.,1.,1.,1.,1.,1.,1.,1.,1.,1.,1.,1.,1.,1.,1.,1.,1.,1.,1.,1.,1.,
1.,1.,1.,1.,1.,1.,1.,1.,1.,1.,1.,1.,1.,1.,1.,1.,1.,1.,1.,1.,1.,1.,1.,1.,
1.,1.,1.,1.,1.,1.,1.,1.,1.,1.,1.,1.,1.,1.,1.,1.,1.,1.,1.,1.,1.,1.,1.,1.,
1.,1.,1.,1.,1.,1.,1.,1.,1.,1.,1.,1.,1.,1.,1.,1.,1.,1.,1.,1.,1.,1.,1.,1.,
1.,1.,1.,1.,1.,1.,1.,1.,1.,1.))
REPRESENTATION_ITEM('')
);
#549=(
BOUNDED_CURVE()
B_SPLINE_CURVE(5,(#118205,#118206,#118207,#118208,#118209,#118210,#118211,
#118212,#118213,#118214,#118215,#118216,#118217,#118218,#118219,#118220,
#118221,#118222,#118223,#118224,#118225,#118226,#118227,#118228,#118229,
#118230,#118231,#118232,#118233,#118234,#118235,#118236,#118237,#118238,
#118239,#118240,#118241,#118242,#118243,#118244,#118245,#118246,#118247,
#118248,#118249,#118250,#118251,#118252,#118253,#118254,#118255,#118256,
#118257,#118258,#118259,#118260,#118261,#118262,#118263,#118264,#118265,
#118266,#118267,#118268,#118269,#118270,#118271,#118272,#118273,#118274,
#118275,#118276,#118277,#118278,#118279,#118280,#118281,#118282,#118283,
#118284,#118285,#118286,#118287,#118288,#118289,#118290,#118291,#118292,
#118293,#118294,#118295,#118296,#118297,#118298,#118299,#118300,#118301,
#118302,#118303,#118304,#118305,#118306,#118307,#118308,#118309,#118310,
#118311,#118312,#118313,#118314,#118315,#118316,#118317,#118318,#118319,
#118320,#118321,#118322,#118323,#118324,#118325,#118326,#118327,#118328,
#118329,#118330,#118331,#118332,#118333,#118334,#118335,#118336,#118337,
#118338,#118339,#118340,#118341,#118342,#118343,#118344,#118345,#118346,
#118347,#118348,#118349,#118350,#118351,#118352,#118353,#118354,#118355,
#118356,#118357,#118358,#118359,#118360,#118361,#118362,#118363,#118364,
#118365,#118366,#118367,#118368,#118369,#118370,#118371,#118372,#118373,
#118374,#118375,#118376,#118377,#118378,#118379,#118380,#118381,#118382,
#118383,#118384,#118385,#118386,#118387,#118388,#118389,#118390,#118391,
#118392,#118393,#118394,#118395,#118396,#118397,#118398),.UNSPECIFIED.,
 .F.,.F.)
B_SPLINE_CURVE_WITH_KNOTS((6,1,1,1,1,1,1,1,1,1,1,1,1,1,1,1,1,1,1,1,1,1,
1,1,1,1,1,1,1,1,1,1,1,1,1,1,1,1,1,1,1,1,1,1,1,1,1,1,1,1,1,1,1,1,1,1,1,1,
1,1,1,1,1,1,1,1,1,1,1,1,1,1,1,1,1,1,1,1,1,1,1,1,1,1,1,1,1,1,1,1,1,1,1,1,
1,1,1,1,1,1,1,1,1,1,1,1,1,1,1,1,1,1,1,1,1,1,1,1,1,1,1,1,1,1,1,1,1,1,1,1,
1,1,1,1,1,1,1,1,1,1,1,1,1,1,1,1,1,1,1,1,1,1,1,1,1,1,1,1,1,1,1,1,1,1,1,1,
1,1,1,1,1,1,1,1,1,1,1,1,1,1,1,1,1,1,1,1,1,1,1,6),(0.,0.005,0.01,0.015,0.02,
0.025,0.03,0.035,0.04,0.045,0.05,0.055,0.06,0.065,0.07,0.075,0.08,0.085,
0.09,0.095,0.1,0.105,0.11,0.115,0.12,0.125,0.13,0.135,0.14,0.145,0.15,0.155,
0.16,0.165,0.17,0.175,0.18,0.185,0.19,0.195,0.2,0.205,0.21,0.215,0.22,0.225,
0.23,0.235,0.24,0.245,0.25,0.255,0.26,0.265,0.27,0.275,0.28,0.285,0.29,
0.295,0.3,0.305,0.31,0.315,0.32,0.325,0.33,0.335,0.34,0.345,0.35,0.355,
0.36,0.365,0.37,0.375,0.38,0.385,0.39,0.395,0.4,0.405,0.41,0.415,0.42,0.425,
0.43,0.435,0.44,0.445,0.45,0.455,0.46,0.465,0.47,0.475,0.48,0.485,0.49,
0.495,0.5,0.505,0.51,0.515,0.52,0.525,0.53,0.535,0.54,0.545,0.55,0.555,
0.56,0.565,0.57,0.575,0.58,0.585,0.59,0.595,0.6,0.605,0.61,0.615,0.62,0.625,
0.63,0.635,0.64,0.645,0.65,0.655,0.66,0.665,0.67,0.675,0.68,0.685,0.690000000000001,
0.695000000000001,0.700000000000001,0.705000000000001,0.710000000000001,
0.715000000000001,0.720000000000001,0.725000000000001,0.730000000000001,
0.735000000000001,0.740000000000001,0.745000000000001,0.750000000000001,
0.755000000000001,0.760000000000001,0.765000000000001,0.770000000000001,
0.775000000000001,0.780000000000001,0.785000000000001,0.790000000000001,
0.795000000000001,0.800000000000001,0.805000000000001,0.810000000000001,
0.815000000000001,0.820000000000001,0.825000000000001,0.830000000000001,
0.835000000000001,0.840000000000001,0.845000000000001,0.850000000000001,
0.855000000000001,0.860000000000001,0.865000000000001,0.870000000000001,
0.875000000000001,0.880000000000001,0.885000000000001,0.890000000000001,
0.895000000000001,0.900000000000001,0.905000000000001,0.910000000000001,
0.915000000000001,0.920000000000001,0.925000000000001,0.930000000000001,
0.935000000000001,0.940000000000001,0.941429844438101),.UNSPECIFIED.)
CURVE()
GEOMETRIC_REPRESENTATION_ITEM()
RATIONAL_B_SPLINE_CURVE((1.,1.,1.,1.,1.,1.,1.,1.,1.,1.,1.,1.,1.,1.,1.,1.,
1.,1.,1.,1.,1.,1.,1.,1.,1.,1.,1.,1.,1.,1.,1.,1.,1.,1.,1.,1.,1.,1.,1.,1.,
1.,1.,1.,1.,1.,1.,1.,1.,1.,1.,1.,1.,1.,1.,1.,1.,1.,1.,1.,1.,1.,1.,1.,1.,
1.,1.,1.,1.,1.,1.,1.,1.,1.,1.,1.,1.,1.,1.,1.,1.,1.,1.,1.,1.,1.,1.,1.,1.,
1.,1.,1.,1.,1.,1.,1.,1.,1.,1.,1.,1.,1.,1.,1.,1.,1.,1.,1.,1.,1.,1.,1.,1.,
1.,1.,1.,1.,1.,1.,1.,1.,1.,1.,1.,1.,1.,1.,1.,1.,1.,1.,1.,1.,1.,1.,1.,1.,
1.,1.,1.,1.,1.,1.,1.,1.,1.,1.,1.,1.,1.,1.,1.,1.,1.,1.,1.,1.,1.,1.,1.,1.,
1.,1.,1.,1.,1.,1.,1.,1.,1.,1.,1.,1.,1.,1.,1.,1.,1.,1.,1.,1.,1.,1.,1.,1.,
1.,1.,1.,1.,1.,1.,1.,1.,1.,1.))
REPRESENTATION_ITEM('')
);
#550=(
BOUNDED_CURVE()
B_SPLINE_CURVE(5,(#118401,#118402,#118403,#118404,#118405,#118406,#118407,
#118408,#118409,#118410,#118411,#118412,#118413,#118414,#118415,#118416,
#118417,#118418,#118419,#118420,#118421,#118422,#118423,#118424,#118425,
#118426,#118427,#118428,#118429,#118430,#118431,#118432,#118433,#118434,
#118435,#118436,#118437,#118438,#118439,#118440,#118441,#118442,#118443,
#118444,#118445,#118446,#118447,#118448,#118449,#118450,#118451,#118452,
#118453,#118454,#118455,#118456,#118457,#118458,#118459,#118460,#118461,
#118462,#118463,#118464,#118465,#118466,#118467,#118468,#118469,#118470,
#118471,#118472,#118473,#118474,#118475,#118476,#118477,#118478,#118479,
#118480,#118481,#118482,#118483,#118484,#118485,#118486,#118487,#118488,
#118489,#118490,#118491,#118492,#118493,#118494,#118495,#118496,#118497,
#118498,#118499,#118500,#118501,#118502,#118503,#118504,#118505,#118506,
#118507,#118508,#118509,#118510,#118511,#118512,#118513,#118514,#118515,
#118516,#118517,#118518,#118519,#118520,#118521,#118522,#118523,#118524,
#118525,#118526,#118527,#118528,#118529,#118530,#118531,#118532,#118533,
#118534,#118535,#118536,#118537,#118538,#118539,#118540,#118541,#118542,
#118543,#118544,#118545,#118546,#118547,#118548,#118549,#118550,#118551,
#118552,#118553,#118554,#118555,#118556,#118557,#118558,#118559,#118560,
#118561,#118562,#118563,#118564,#118565,#118566,#118567,#118568,#118569,
#118570,#118571,#118572,#118573,#118574,#118575,#118576,#118577,#118578,
#118579,#118580,#118581,#118582,#118583,#118584,#118585,#118586,#118587,
#118588,#118589,#118590,#118591,#118592,#118593,#118594),.UNSPECIFIED.,
 .F.,.F.)
B_SPLINE_CURVE_WITH_KNOTS((6,1,1,1,1,1,1,1,1,1,1,1,1,1,1,1,1,1,1,1,1,1,
1,1,1,1,1,1,1,1,1,1,1,1,1,1,1,1,1,1,1,1,1,1,1,1,1,1,1,1,1,1,1,1,1,1,1,1,
1,1,1,1,1,1,1,1,1,1,1,1,1,1,1,1,1,1,1,1,1,1,1,1,1,1,1,1,1,1,1,1,1,1,1,1,
1,1,1,1,1,1,1,1,1,1,1,1,1,1,1,1,1,1,1,1,1,1,1,1,1,1,1,1,1,1,1,1,1,1,1,1,
1,1,1,1,1,1,1,1,1,1,1,1,1,1,1,1,1,1,1,1,1,1,1,1,1,1,1,1,1,1,1,1,1,1,1,1,
1,1,1,1,1,1,1,1,1,1,1,1,1,1,1,1,1,1,1,1,1,1,1,6),(-0.941429844438086,-0.940000000000001,
-0.935000000000001,-0.930000000000001,-0.925000000000001,-0.920000000000001,
-0.915000000000001,-0.910000000000001,-0.905000000000001,-0.900000000000001,
-0.895000000000001,-0.890000000000001,-0.885000000000001,-0.880000000000001,
-0.875000000000001,-0.870000000000001,-0.865000000000001,-0.860000000000001,
-0.855000000000001,-0.850000000000001,-0.845000000000001,-0.840000000000001,
-0.835000000000001,-0.830000000000001,-0.825000000000001,-0.820000000000001,
-0.815000000000001,-0.810000000000001,-0.805000000000001,-0.800000000000001,
-0.795000000000001,-0.790000000000001,-0.785000000000001,-0.780000000000001,
-0.775000000000001,-0.770000000000001,-0.765000000000001,-0.760000000000001,
-0.755000000000001,-0.750000000000001,-0.745000000000001,-0.740000000000001,
-0.735000000000001,-0.730000000000001,-0.725000000000001,-0.720000000000001,
-0.715000000000001,-0.710000000000001,-0.705000000000001,-0.700000000000001,
-0.695000000000001,-0.690000000000001,-0.685,-0.68,-0.675,-0.67,-0.665,
-0.66,-0.655,-0.65,-0.645,-0.64,-0.635,-0.63,-0.625,-0.62,-0.615,-0.61,
-0.605,-0.6,-0.595,-0.59,-0.585,-0.58,-0.575,-0.57,-0.565,-0.56,-0.555,
-0.55,-0.545,-0.54,-0.535,-0.53,-0.525,-0.52,-0.515,-0.51,-0.505,-0.5,-0.495,
-0.49,-0.485,-0.48,-0.475,-0.47,-0.465,-0.46,-0.455,-0.45,-0.445,-0.44,
-0.435,-0.43,-0.425,-0.42,-0.415,-0.41,-0.405,-0.4,-0.395,-0.39,-0.385,
-0.38,-0.375,-0.37,-0.365,-0.36,-0.355,-0.35,-0.345,-0.34,-0.335,-0.33,
-0.325,-0.32,-0.315,-0.31,-0.305,-0.3,-0.295,-0.29,-0.285,-0.28,-0.275,
-0.27,-0.265,-0.26,-0.255,-0.25,-0.245,-0.24,-0.235,-0.23,-0.225,-0.22,
-0.215,-0.21,-0.205,-0.2,-0.195,-0.19,-0.185,-0.18,-0.175,-0.17,-0.165,
-0.16,-0.155,-0.15,-0.145,-0.14,-0.135,-0.13,-0.125,-0.12,-0.115,-0.11,
-0.105,-0.1,-0.095,-0.09,-0.085,-0.08,-0.075,-0.07,-0.065,-0.06,-0.055,
-0.05,-0.045,-0.04,-0.035,-0.03,-0.025,-0.02,-0.015,-0.01,-0.005,0.),
 .UNSPECIFIED.)
CURVE()
GEOMETRIC_REPRESENTATION_ITEM()
RATIONAL_B_SPLINE_CURVE((1.,1.,1.,1.,1.,1.,1.,1.,1.,1.,1.,1.,1.,1.,1.,1.,
1.,1.,1.,1.,1.,1.,1.,1.,1.,1.,1.,1.,1.,1.,1.,1.,1.,1.,1.,1.,1.,1.,1.,1.,
1.,1.,1.,1.,1.,1.,1.,1.,1.,1.,1.,1.,1.,1.,1.,1.,1.,1.,1.,1.,1.,1.,1.,1.,
1.,1.,1.,1.,1.,1.,1.,1.,1.,1.,1.,1.,1.,1.,1.,1.,1.,1.,1.,1.,1.,1.,1.,1.,
1.,1.,1.,1.,1.,1.,1.,1.,1.,1.,1.,1.,1.,1.,1.,1.,1.,1.,1.,1.,1.,1.,1.,1.,
1.,1.,1.,1.,1.,1.,1.,1.,1.,1.,1.,1.,1.,1.,1.,1.,1.,1.,1.,1.,1.,1.,1.,1.,
1.,1.,1.,1.,1.,1.,1.,1.,1.,1.,1.,1.,1.,1.,1.,1.,1.,1.,1.,1.,1.,1.,1.,1.,
1.,1.,1.,1.,1.,1.,1.,1.,1.,1.,1.,1.,1.,1.,1.,1.,1.,1.,1.,1.,1.,1.,1.,1.,
1.,1.,1.,1.,1.,1.,1.,1.,1.,1.))
REPRESENTATION_ITEM('')
);
#551=(
BOUNDED_CURVE()
B_SPLINE_CURVE(5,(#119006,#119007,#119008,#119009,#119010,#119011,#119012,
#119013,#119014,#119015,#119016,#119017,#119018,#119019,#119020,#119021,
#119022,#119023,#119024,#119025,#119026,#119027,#119028,#119029,#119030,
#119031,#119032,#119033,#119034,#119035,#119036,#119037,#119038,#119039,
#119040,#119041,#119042,#119043,#119044,#119045,#119046,#119047,#119048,
#119049,#119050,#119051,#119052,#119053,#119054,#119055,#119056,#119057,
#119058,#119059,#119060,#119061,#119062,#119063,#119064,#119065,#119066,
#119067,#119068,#119069,#119070,#119071,#119072,#119073,#119074,#119075,
#119076,#119077,#119078,#119079,#119080,#119081,#119082,#119083,#119084,
#119085,#119086,#119087,#119088,#119089,#119090,#119091,#119092,#119093,
#119094,#119095,#119096,#119097,#119098,#119099,#119100,#119101,#119102,
#119103,#119104,#119105,#119106,#119107,#119108,#119109,#119110,#119111,
#119112,#119113,#119114,#119115,#119116,#119117,#119118,#119119,#119120,
#119121,#119122,#119123,#119124,#119125,#119126,#119127,#119128,#119129,
#119130,#119131,#119132,#119133,#119134,#119135,#119136,#119137,#119138,
#119139,#119140,#119141,#119142,#119143,#119144,#119145,#119146,#119147,
#119148,#119149,#119150,#119151,#119152,#119153,#119154,#119155,#119156,
#119157,#119158,#119159,#119160,#119161,#119162,#119163,#119164,#119165,
#119166,#119167,#119168,#119169,#119170,#119171,#119172,#119173,#119174,
#119175,#119176,#119177,#119178,#119179,#119180,#119181,#119182,#119183,
#119184,#119185,#119186,#119187,#119188,#119189,#119190,#119191,#119192,
#119193,#119194,#119195,#119196,#119197,#119198,#119199),.UNSPECIFIED.,
 .F.,.F.)
B_SPLINE_CURVE_WITH_KNOTS((6,1,1,1,1,1,1,1,1,1,1,1,1,1,1,1,1,1,1,1,1,1,
1,1,1,1,1,1,1,1,1,1,1,1,1,1,1,1,1,1,1,1,1,1,1,1,1,1,1,1,1,1,1,1,1,1,1,1,
1,1,1,1,1,1,1,1,1,1,1,1,1,1,1,1,1,1,1,1,1,1,1,1,1,1,1,1,1,1,1,1,1,1,1,1,
1,1,1,1,1,1,1,1,1,1,1,1,1,1,1,1,1,1,1,1,1,1,1,1,1,1,1,1,1,1,1,1,1,1,1,1,
1,1,1,1,1,1,1,1,1,1,1,1,1,1,1,1,1,1,1,1,1,1,1,1,1,1,1,1,1,1,1,1,1,1,1,1,
1,1,1,1,1,1,1,1,1,1,1,1,1,1,1,1,1,1,1,1,1,1,1,6),(0.,0.005,0.01,0.015,0.02,
0.025,0.03,0.035,0.04,0.045,0.05,0.055,0.06,0.065,0.07,0.075,0.08,0.085,
0.09,0.095,0.1,0.105,0.11,0.115,0.12,0.125,0.13,0.135,0.14,0.145,0.15,0.155,
0.16,0.165,0.17,0.175,0.18,0.185,0.19,0.195,0.2,0.205,0.21,0.215,0.22,0.225,
0.23,0.235,0.24,0.245,0.25,0.255,0.26,0.265,0.27,0.275,0.28,0.285,0.29,
0.295,0.3,0.305,0.31,0.315,0.32,0.325,0.33,0.335,0.34,0.345,0.35,0.355,
0.36,0.365,0.37,0.375,0.38,0.385,0.39,0.395,0.4,0.405,0.41,0.415,0.42,0.425,
0.43,0.435,0.44,0.445,0.45,0.455,0.46,0.465,0.47,0.475,0.48,0.485,0.49,
0.495,0.5,0.505,0.51,0.515,0.52,0.525,0.53,0.535,0.54,0.545,0.55,0.555,
0.56,0.565,0.57,0.575,0.58,0.585,0.59,0.595,0.6,0.605,0.61,0.615,0.62,0.625,
0.63,0.635,0.64,0.645,0.65,0.655,0.66,0.665,0.67,0.675,0.68,0.685,0.690000000000001,
0.695000000000001,0.700000000000001,0.705000000000001,0.710000000000001,
0.715000000000001,0.720000000000001,0.725000000000001,0.730000000000001,
0.735000000000001,0.740000000000001,0.745000000000001,0.750000000000001,
0.755000000000001,0.760000000000001,0.765000000000001,0.770000000000001,
0.775000000000001,0.780000000000001,0.785000000000001,0.790000000000001,
0.795000000000001,0.800000000000001,0.805000000000001,0.810000000000001,
0.815000000000001,0.820000000000001,0.825000000000001,0.830000000000001,
0.835000000000001,0.840000000000001,0.845000000000001,0.850000000000001,
0.855000000000001,0.860000000000001,0.865000000000001,0.870000000000001,
0.875000000000001,0.880000000000001,0.885000000000001,0.890000000000001,
0.895000000000001,0.900000000000001,0.905000000000001,0.910000000000001,
0.915000000000001,0.920000000000001,0.925000000000001,0.930000000000001,
0.935000000000001,0.940000000000001,0.941429844438003),.UNSPECIFIED.)
CURVE()
GEOMETRIC_REPRESENTATION_ITEM()
RATIONAL_B_SPLINE_CURVE((1.,1.,1.,1.,1.,1.,1.,1.,1.,1.,1.,1.,1.,1.,1.,1.,
1.,1.,1.,1.,1.,1.,1.,1.,1.,1.,1.,1.,1.,1.,1.,1.,1.,1.,1.,1.,1.,1.,1.,1.,
1.,1.,1.,1.,1.,1.,1.,1.,1.,1.,1.,1.,1.,1.,1.,1.,1.,1.,1.,1.,1.,1.,1.,1.,
1.,1.,1.,1.,1.,1.,1.,1.,1.,1.,1.,1.,1.,1.,1.,1.,1.,1.,1.,1.,1.,1.,1.,1.,
1.,1.,1.,1.,1.,1.,1.,1.,1.,1.,1.,1.,1.,1.,1.,1.,1.,1.,1.,1.,1.,1.,1.,1.,
1.,1.,1.,1.,1.,1.,1.,1.,1.,1.,1.,1.,1.,1.,1.,1.,1.,1.,1.,1.,1.,1.,1.,1.,
1.,1.,1.,1.,1.,1.,1.,1.,1.,1.,1.,1.,1.,1.,1.,1.,1.,1.,1.,1.,1.,1.,1.,1.,
1.,1.,1.,1.,1.,1.,1.,1.,1.,1.,1.,1.,1.,1.,1.,1.,1.,1.,1.,1.,1.,1.,1.,1.,
1.,1.,1.,1.,1.,1.,1.,1.,1.,1.))
REPRESENTATION_ITEM('')
);
#552=(
BOUNDED_CURVE()
B_SPLINE_CURVE(5,(#119202,#119203,#119204,#119205,#119206,#119207,#119208,
#119209,#119210,#119211,#119212,#119213,#119214,#119215,#119216,#119217,
#119218,#119219,#119220,#119221,#119222,#119223,#119224,#119225,#119226,
#119227,#119228,#119229,#119230,#119231,#119232,#119233,#119234,#119235,
#119236,#119237,#119238,#119239,#119240,#119241,#119242,#119243,#119244,
#119245,#119246,#119247,#119248,#119249,#119250,#119251,#119252,#119253,
#119254,#119255,#119256,#119257,#119258,#119259,#119260,#119261,#119262,
#119263,#119264,#119265,#119266,#119267,#119268,#119269,#119270,#119271,
#119272,#119273,#119274,#119275,#119276,#119277,#119278,#119279,#119280,
#119281,#119282,#119283,#119284,#119285,#119286,#119287,#119288,#119289,
#119290,#119291,#119292,#119293,#119294,#119295,#119296,#119297,#119298,
#119299,#119300,#119301,#119302,#119303,#119304,#119305,#119306,#119307,
#119308,#119309,#119310,#119311,#119312,#119313,#119314,#119315,#119316,
#119317,#119318,#119319,#119320,#119321,#119322,#119323,#119324,#119325,
#119326,#119327,#119328,#119329,#119330,#119331,#119332,#119333,#119334,
#119335,#119336,#119337,#119338,#119339,#119340,#119341,#119342,#119343,
#119344,#119345,#119346,#119347,#119348,#119349,#119350,#119351,#119352,
#119353,#119354,#119355,#119356,#119357,#119358,#119359,#119360,#119361,
#119362,#119363,#119364,#119365,#119366,#119367,#119368,#119369,#119370,
#119371,#119372,#119373,#119374,#119375,#119376,#119377,#119378,#119379,
#119380,#119381,#119382,#119383,#119384,#119385,#119386,#119387,#119388,
#119389,#119390,#119391,#119392,#119393,#119394,#119395),.UNSPECIFIED.,
 .F.,.F.)
B_SPLINE_CURVE_WITH_KNOTS((6,1,1,1,1,1,1,1,1,1,1,1,1,1,1,1,1,1,1,1,1,1,
1,1,1,1,1,1,1,1,1,1,1,1,1,1,1,1,1,1,1,1,1,1,1,1,1,1,1,1,1,1,1,1,1,1,1,1,
1,1,1,1,1,1,1,1,1,1,1,1,1,1,1,1,1,1,1,1,1,1,1,1,1,1,1,1,1,1,1,1,1,1,1,1,
1,1,1,1,1,1,1,1,1,1,1,1,1,1,1,1,1,1,1,1,1,1,1,1,1,1,1,1,1,1,1,1,1,1,1,1,
1,1,1,1,1,1,1,1,1,1,1,1,1,1,1,1,1,1,1,1,1,1,1,1,1,1,1,1,1,1,1,1,1,1,1,1,
1,1,1,1,1,1,1,1,1,1,1,1,1,1,1,1,1,1,1,1,1,1,1,6),(-0.941429844438003,-0.940000000000001,
-0.935000000000001,-0.930000000000001,-0.925000000000001,-0.920000000000001,
-0.915000000000001,-0.910000000000001,-0.905000000000001,-0.900000000000001,
-0.895000000000001,-0.890000000000001,-0.885000000000001,-0.880000000000001,
-0.875000000000001,-0.870000000000001,-0.865000000000001,-0.860000000000001,
-0.855000000000001,-0.850000000000001,-0.845000000000001,-0.840000000000001,
-0.835000000000001,-0.830000000000001,-0.825000000000001,-0.820000000000001,
-0.815000000000001,-0.810000000000001,-0.805000000000001,-0.800000000000001,
-0.795000000000001,-0.790000000000001,-0.785000000000001,-0.780000000000001,
-0.775000000000001,-0.770000000000001,-0.765000000000001,-0.760000000000001,
-0.755000000000001,-0.750000000000001,-0.745000000000001,-0.740000000000001,
-0.735000000000001,-0.730000000000001,-0.725000000000001,-0.720000000000001,
-0.715000000000001,-0.710000000000001,-0.705000000000001,-0.700000000000001,
-0.695000000000001,-0.690000000000001,-0.685,-0.68,-0.675,-0.67,-0.665,
-0.66,-0.655,-0.65,-0.645,-0.64,-0.635,-0.63,-0.625,-0.62,-0.615,-0.61,
-0.605,-0.6,-0.595,-0.59,-0.585,-0.58,-0.575,-0.57,-0.565,-0.56,-0.555,
-0.55,-0.545,-0.54,-0.535,-0.53,-0.525,-0.52,-0.515,-0.51,-0.505,-0.5,-0.495,
-0.49,-0.485,-0.48,-0.475,-0.47,-0.465,-0.46,-0.455,-0.45,-0.445,-0.44,
-0.435,-0.43,-0.425,-0.42,-0.415,-0.41,-0.405,-0.4,-0.395,-0.39,-0.385,
-0.38,-0.375,-0.37,-0.365,-0.36,-0.355,-0.35,-0.345,-0.34,-0.335,-0.33,
-0.325,-0.32,-0.315,-0.31,-0.305,-0.3,-0.295,-0.29,-0.285,-0.28,-0.275,
-0.27,-0.265,-0.26,-0.255,-0.25,-0.245,-0.24,-0.235,-0.23,-0.225,-0.22,
-0.215,-0.21,-0.205,-0.2,-0.195,-0.19,-0.185,-0.18,-0.175,-0.17,-0.165,
-0.16,-0.155,-0.15,-0.145,-0.14,-0.135,-0.13,-0.125,-0.12,-0.115,-0.11,
-0.105,-0.1,-0.095,-0.09,-0.085,-0.08,-0.075,-0.07,-0.065,-0.06,-0.055,
-0.05,-0.045,-0.04,-0.035,-0.03,-0.025,-0.02,-0.015,-0.01,-0.005,0.),
 .UNSPECIFIED.)
CURVE()
GEOMETRIC_REPRESENTATION_ITEM()
RATIONAL_B_SPLINE_CURVE((1.,1.,1.,1.,1.,1.,1.,1.,1.,1.,1.,1.,1.,1.,1.,1.,
1.,1.,1.,1.,1.,1.,1.,1.,1.,1.,1.,1.,1.,1.,1.,1.,1.,1.,1.,1.,1.,1.,1.,1.,
1.,1.,1.,1.,1.,1.,1.,1.,1.,1.,1.,1.,1.,1.,1.,1.,1.,1.,1.,1.,1.,1.,1.,1.,
1.,1.,1.,1.,1.,1.,1.,1.,1.,1.,1.,1.,1.,1.,1.,1.,1.,1.,1.,1.,1.,1.,1.,1.,
1.,1.,1.,1.,1.,1.,1.,1.,1.,1.,1.,1.,1.,1.,1.,1.,1.,1.,1.,1.,1.,1.,1.,1.,
1.,1.,1.,1.,1.,1.,1.,1.,1.,1.,1.,1.,1.,1.,1.,1.,1.,1.,1.,1.,1.,1.,1.,1.,
1.,1.,1.,1.,1.,1.,1.,1.,1.,1.,1.,1.,1.,1.,1.,1.,1.,1.,1.,1.,1.,1.,1.,1.,
1.,1.,1.,1.,1.,1.,1.,1.,1.,1.,1.,1.,1.,1.,1.,1.,1.,1.,1.,1.,1.,1.,1.,1.,
1.,1.,1.,1.,1.,1.,1.,1.,1.,1.))
REPRESENTATION_ITEM('')
);
#553=(
BOUNDED_CURVE()
B_SPLINE_CURVE(5,(#119807,#119808,#119809,#119810,#119811,#119812,#119813,
#119814,#119815,#119816,#119817,#119818,#119819,#119820,#119821,#119822,
#119823,#119824,#119825,#119826,#119827,#119828,#119829,#119830,#119831,
#119832,#119833,#119834,#119835,#119836,#119837,#119838,#119839,#119840,
#119841,#119842,#119843,#119844,#119845,#119846,#119847,#119848,#119849,
#119850,#119851,#119852,#119853,#119854,#119855,#119856,#119857,#119858,
#119859,#119860,#119861,#119862,#119863,#119864,#119865,#119866,#119867,
#119868,#119869,#119870,#119871,#119872,#119873,#119874,#119875,#119876,
#119877,#119878,#119879,#119880,#119881,#119882,#119883,#119884,#119885,
#119886,#119887,#119888,#119889,#119890,#119891,#119892,#119893,#119894,
#119895,#119896,#119897,#119898,#119899,#119900,#119901,#119902,#119903,
#119904,#119905,#119906,#119907,#119908,#119909,#119910,#119911,#119912,
#119913,#119914,#119915,#119916,#119917,#119918,#119919,#119920,#119921,
#119922,#119923,#119924,#119925,#119926,#119927,#119928,#119929,#119930,
#119931,#119932,#119933,#119934,#119935,#119936,#119937,#119938,#119939,
#119940,#119941,#119942,#119943,#119944,#119945,#119946,#119947,#119948,
#119949,#119950,#119951,#119952,#119953,#119954,#119955,#119956,#119957,
#119958,#119959,#119960,#119961,#119962,#119963,#119964,#119965,#119966,
#119967,#119968,#119969,#119970,#119971,#119972,#119973,#119974,#119975,
#119976,#119977,#119978,#119979,#119980,#119981,#119982,#119983,#119984,
#119985,#119986,#119987,#119988,#119989,#119990,#119991,#119992,#119993,
#119994,#119995,#119996,#119997,#119998,#119999,#120000),.UNSPECIFIED.,
 .F.,.F.)
B_SPLINE_CURVE_WITH_KNOTS((6,1,1,1,1,1,1,1,1,1,1,1,1,1,1,1,1,1,1,1,1,1,
1,1,1,1,1,1,1,1,1,1,1,1,1,1,1,1,1,1,1,1,1,1,1,1,1,1,1,1,1,1,1,1,1,1,1,1,
1,1,1,1,1,1,1,1,1,1,1,1,1,1,1,1,1,1,1,1,1,1,1,1,1,1,1,1,1,1,1,1,1,1,1,1,
1,1,1,1,1,1,1,1,1,1,1,1,1,1,1,1,1,1,1,1,1,1,1,1,1,1,1,1,1,1,1,1,1,1,1,1,
1,1,1,1,1,1,1,1,1,1,1,1,1,1,1,1,1,1,1,1,1,1,1,1,1,1,1,1,1,1,1,1,1,1,1,1,
1,1,1,1,1,1,1,1,1,1,1,1,1,1,1,1,1,1,1,1,1,1,1,6),(0.,0.005,0.01,0.015,0.02,
0.025,0.03,0.035,0.04,0.045,0.05,0.055,0.06,0.065,0.07,0.075,0.08,0.085,
0.09,0.095,0.1,0.105,0.11,0.115,0.12,0.125,0.13,0.135,0.14,0.145,0.15,0.155,
0.16,0.165,0.17,0.175,0.18,0.185,0.19,0.195,0.2,0.205,0.21,0.215,0.22,0.225,
0.23,0.235,0.24,0.245,0.25,0.255,0.26,0.265,0.27,0.275,0.28,0.285,0.29,
0.295,0.3,0.305,0.31,0.315,0.32,0.325,0.33,0.335,0.34,0.345,0.35,0.355,
0.36,0.365,0.37,0.375,0.38,0.385,0.39,0.395,0.4,0.405,0.41,0.415,0.42,0.425,
0.43,0.435,0.44,0.445,0.45,0.455,0.46,0.465,0.47,0.475,0.48,0.485,0.49,
0.495,0.5,0.505,0.51,0.515,0.52,0.525,0.53,0.535,0.54,0.545,0.55,0.555,
0.56,0.565,0.57,0.575,0.58,0.585,0.59,0.595,0.6,0.605,0.61,0.615,0.62,0.625,
0.63,0.635,0.64,0.645,0.65,0.655,0.66,0.665,0.67,0.675,0.68,0.685,0.690000000000001,
0.695000000000001,0.700000000000001,0.705000000000001,0.710000000000001,
0.715000000000001,0.720000000000001,0.725000000000001,0.730000000000001,
0.735000000000001,0.740000000000001,0.745000000000001,0.750000000000001,
0.755000000000001,0.760000000000001,0.765000000000001,0.770000000000001,
0.775000000000001,0.780000000000001,0.785000000000001,0.790000000000001,
0.795000000000001,0.800000000000001,0.805000000000001,0.810000000000001,
0.815000000000001,0.820000000000001,0.825000000000001,0.830000000000001,
0.835000000000001,0.840000000000001,0.845000000000001,0.850000000000001,
0.855000000000001,0.860000000000001,0.865000000000001,0.870000000000001,
0.875000000000001,0.880000000000001,0.885000000000001,0.890000000000001,
0.895000000000001,0.900000000000001,0.905000000000001,0.910000000000001,
0.915000000000001,0.920000000000001,0.925000000000001,0.930000000000001,
0.935000000000001,0.940000000000001,0.941429844437941),.UNSPECIFIED.)
CURVE()
GEOMETRIC_REPRESENTATION_ITEM()
RATIONAL_B_SPLINE_CURVE((1.,1.,1.,1.,1.,1.,1.,1.,1.,1.,1.,1.,1.,1.,1.,1.,
1.,1.,1.,1.,1.,1.,1.,1.,1.,1.,1.,1.,1.,1.,1.,1.,1.,1.,1.,1.,1.,1.,1.,1.,
1.,1.,1.,1.,1.,1.,1.,1.,1.,1.,1.,1.,1.,1.,1.,1.,1.,1.,1.,1.,1.,1.,1.,1.,
1.,1.,1.,1.,1.,1.,1.,1.,1.,1.,1.,1.,1.,1.,1.,1.,1.,1.,1.,1.,1.,1.,1.,1.,
1.,1.,1.,1.,1.,1.,1.,1.,1.,1.,1.,1.,1.,1.,1.,1.,1.,1.,1.,1.,1.,1.,1.,1.,
1.,1.,1.,1.,1.,1.,1.,1.,1.,1.,1.,1.,1.,1.,1.,1.,1.,1.,1.,1.,1.,1.,1.,1.,
1.,1.,1.,1.,1.,1.,1.,1.,1.,1.,1.,1.,1.,1.,1.,1.,1.,1.,1.,1.,1.,1.,1.,1.,
1.,1.,1.,1.,1.,1.,1.,1.,1.,1.,1.,1.,1.,1.,1.,1.,1.,1.,1.,1.,1.,1.,1.,1.,
1.,1.,1.,1.,1.,1.,1.,1.,1.,1.))
REPRESENTATION_ITEM('')
);
#554=(
BOUNDED_CURVE()
B_SPLINE_CURVE(5,(#120003,#120004,#120005,#120006,#120007,#120008,#120009,
#120010,#120011,#120012,#120013,#120014,#120015,#120016,#120017,#120018,
#120019,#120020,#120021,#120022,#120023,#120024,#120025,#120026,#120027,
#120028,#120029,#120030,#120031,#120032,#120033,#120034,#120035,#120036,
#120037,#120038,#120039,#120040,#120041,#120042,#120043,#120044,#120045,
#120046,#120047,#120048,#120049,#120050,#120051,#120052,#120053,#120054,
#120055,#120056,#120057,#120058,#120059,#120060,#120061,#120062,#120063,
#120064,#120065,#120066,#120067,#120068,#120069,#120070,#120071,#120072,
#120073,#120074,#120075,#120076,#120077,#120078,#120079,#120080,#120081,
#120082,#120083,#120084,#120085,#120086,#120087,#120088,#120089,#120090,
#120091,#120092,#120093,#120094,#120095,#120096,#120097,#120098,#120099,
#120100,#120101,#120102,#120103,#120104,#120105,#120106,#120107,#120108,
#120109,#120110,#120111,#120112,#120113,#120114,#120115,#120116,#120117,
#120118,#120119,#120120,#120121,#120122,#120123,#120124,#120125,#120126,
#120127,#120128,#120129,#120130,#120131,#120132,#120133,#120134,#120135,
#120136,#120137,#120138,#120139,#120140,#120141,#120142,#120143,#120144,
#120145,#120146,#120147,#120148,#120149,#120150,#120151,#120152,#120153,
#120154,#120155,#120156,#120157,#120158,#120159,#120160,#120161,#120162,
#120163,#120164,#120165,#120166,#120167,#120168,#120169,#120170,#120171,
#120172,#120173,#120174,#120175,#120176,#120177,#120178,#120179,#120180,
#120181,#120182,#120183,#120184,#120185,#120186,#120187,#120188,#120189,
#120190,#120191,#120192,#120193,#120194,#120195,#120196),.UNSPECIFIED.,
 .F.,.F.)
B_SPLINE_CURVE_WITH_KNOTS((6,1,1,1,1,1,1,1,1,1,1,1,1,1,1,1,1,1,1,1,1,1,
1,1,1,1,1,1,1,1,1,1,1,1,1,1,1,1,1,1,1,1,1,1,1,1,1,1,1,1,1,1,1,1,1,1,1,1,
1,1,1,1,1,1,1,1,1,1,1,1,1,1,1,1,1,1,1,1,1,1,1,1,1,1,1,1,1,1,1,1,1,1,1,1,
1,1,1,1,1,1,1,1,1,1,1,1,1,1,1,1,1,1,1,1,1,1,1,1,1,1,1,1,1,1,1,1,1,1,1,1,
1,1,1,1,1,1,1,1,1,1,1,1,1,1,1,1,1,1,1,1,1,1,1,1,1,1,1,1,1,1,1,1,1,1,1,1,
1,1,1,1,1,1,1,1,1,1,1,1,1,1,1,1,1,1,1,1,1,1,1,6),(-0.941429844437942,-0.940000000000001,
-0.935000000000001,-0.930000000000001,-0.925000000000001,-0.920000000000001,
-0.915000000000001,-0.910000000000001,-0.905000000000001,-0.900000000000001,
-0.895000000000001,-0.890000000000001,-0.885000000000001,-0.880000000000001,
-0.875000000000001,-0.870000000000001,-0.865000000000001,-0.860000000000001,
-0.855000000000001,-0.850000000000001,-0.845000000000001,-0.840000000000001,
-0.835000000000001,-0.830000000000001,-0.825000000000001,-0.820000000000001,
-0.815000000000001,-0.810000000000001,-0.805000000000001,-0.800000000000001,
-0.795000000000001,-0.790000000000001,-0.785000000000001,-0.780000000000001,
-0.775000000000001,-0.770000000000001,-0.765000000000001,-0.760000000000001,
-0.755000000000001,-0.750000000000001,-0.745000000000001,-0.740000000000001,
-0.735000000000001,-0.730000000000001,-0.725000000000001,-0.720000000000001,
-0.715000000000001,-0.710000000000001,-0.705000000000001,-0.700000000000001,
-0.695000000000001,-0.690000000000001,-0.685,-0.68,-0.675,-0.67,-0.665,
-0.66,-0.655,-0.65,-0.645,-0.64,-0.635,-0.63,-0.625,-0.62,-0.615,-0.61,
-0.605,-0.6,-0.595,-0.59,-0.585,-0.58,-0.575,-0.57,-0.565,-0.56,-0.555,
-0.55,-0.545,-0.54,-0.535,-0.53,-0.525,-0.52,-0.515,-0.51,-0.505,-0.5,-0.495,
-0.49,-0.485,-0.48,-0.475,-0.47,-0.465,-0.46,-0.455,-0.45,-0.445,-0.44,
-0.435,-0.43,-0.425,-0.42,-0.415,-0.41,-0.405,-0.4,-0.395,-0.39,-0.385,
-0.38,-0.375,-0.37,-0.365,-0.36,-0.355,-0.35,-0.345,-0.34,-0.335,-0.33,
-0.325,-0.32,-0.315,-0.31,-0.305,-0.3,-0.295,-0.29,-0.285,-0.28,-0.275,
-0.27,-0.265,-0.26,-0.255,-0.25,-0.245,-0.24,-0.235,-0.23,-0.225,-0.22,
-0.215,-0.21,-0.205,-0.2,-0.195,-0.19,-0.185,-0.18,-0.175,-0.17,-0.165,
-0.16,-0.155,-0.15,-0.145,-0.14,-0.135,-0.13,-0.125,-0.12,-0.115,-0.11,
-0.105,-0.1,-0.095,-0.09,-0.085,-0.08,-0.075,-0.07,-0.065,-0.06,-0.055,
-0.05,-0.045,-0.04,-0.035,-0.03,-0.025,-0.02,-0.015,-0.01,-0.005,0.),
 .UNSPECIFIED.)
CURVE()
GEOMETRIC_REPRESENTATION_ITEM()
RATIONAL_B_SPLINE_CURVE((1.,1.,1.,1.,1.,1.,1.,1.,1.,1.,1.,1.,1.,1.,1.,1.,
1.,1.,1.,1.,1.,1.,1.,1.,1.,1.,1.,1.,1.,1.,1.,1.,1.,1.,1.,1.,1.,1.,1.,1.,
1.,1.,1.,1.,1.,1.,1.,1.,1.,1.,1.,1.,1.,1.,1.,1.,1.,1.,1.,1.,1.,1.,1.,1.,
1.,1.,1.,1.,1.,1.,1.,1.,1.,1.,1.,1.,1.,1.,1.,1.,1.,1.,1.,1.,1.,1.,1.,1.,
1.,1.,1.,1.,1.,1.,1.,1.,1.,1.,1.,1.,1.,1.,1.,1.,1.,1.,1.,1.,1.,1.,1.,1.,
1.,1.,1.,1.,1.,1.,1.,1.,1.,1.,1.,1.,1.,1.,1.,1.,1.,1.,1.,1.,1.,1.,1.,1.,
1.,1.,1.,1.,1.,1.,1.,1.,1.,1.,1.,1.,1.,1.,1.,1.,1.,1.,1.,1.,1.,1.,1.,1.,
1.,1.,1.,1.,1.,1.,1.,1.,1.,1.,1.,1.,1.,1.,1.,1.,1.,1.,1.,1.,1.,1.,1.,1.,
1.,1.,1.,1.,1.,1.,1.,1.,1.,1.))
REPRESENTATION_ITEM('')
);
#555=(
BOUNDED_CURVE()
B_SPLINE_CURVE(5,(#120608,#120609,#120610,#120611,#120612,#120613,#120614,
#120615,#120616,#120617,#120618,#120619,#120620,#120621,#120622,#120623,
#120624,#120625,#120626,#120627,#120628,#120629,#120630,#120631,#120632,
#120633,#120634,#120635,#120636,#120637,#120638,#120639,#120640,#120641,
#120642,#120643,#120644,#120645,#120646,#120647,#120648,#120649,#120650,
#120651,#120652,#120653,#120654,#120655,#120656,#120657,#120658,#120659,
#120660,#120661,#120662,#120663,#120664,#120665,#120666,#120667,#120668,
#120669,#120670,#120671,#120672,#120673,#120674,#120675,#120676,#120677,
#120678,#120679,#120680,#120681,#120682,#120683,#120684,#120685,#120686,
#120687,#120688,#120689,#120690,#120691,#120692,#120693,#120694,#120695,
#120696,#120697,#120698,#120699,#120700,#120701,#120702,#120703,#120704,
#120705,#120706,#120707,#120708,#120709,#120710,#120711,#120712,#120713,
#120714,#120715,#120716,#120717,#120718,#120719,#120720,#120721,#120722,
#120723,#120724,#120725,#120726,#120727,#120728,#120729,#120730,#120731,
#120732,#120733,#120734,#120735,#120736,#120737,#120738,#120739,#120740,
#120741,#120742,#120743,#120744,#120745,#120746,#120747,#120748,#120749,
#120750,#120751,#120752,#120753,#120754,#120755,#120756,#120757,#120758,
#120759,#120760,#120761,#120762,#120763,#120764,#120765,#120766,#120767,
#120768,#120769,#120770,#120771,#120772,#120773,#120774,#120775,#120776,
#120777,#120778,#120779,#120780,#120781,#120782,#120783,#120784,#120785,
#120786,#120787,#120788,#120789,#120790,#120791,#120792,#120793,#120794,
#120795,#120796,#120797,#120798,#120799,#120800,#120801),.UNSPECIFIED.,
 .F.,.F.)
B_SPLINE_CURVE_WITH_KNOTS((6,1,1,1,1,1,1,1,1,1,1,1,1,1,1,1,1,1,1,1,1,1,
1,1,1,1,1,1,1,1,1,1,1,1,1,1,1,1,1,1,1,1,1,1,1,1,1,1,1,1,1,1,1,1,1,1,1,1,
1,1,1,1,1,1,1,1,1,1,1,1,1,1,1,1,1,1,1,1,1,1,1,1,1,1,1,1,1,1,1,1,1,1,1,1,
1,1,1,1,1,1,1,1,1,1,1,1,1,1,1,1,1,1,1,1,1,1,1,1,1,1,1,1,1,1,1,1,1,1,1,1,
1,1,1,1,1,1,1,1,1,1,1,1,1,1,1,1,1,1,1,1,1,1,1,1,1,1,1,1,1,1,1,1,1,1,1,1,
1,1,1,1,1,1,1,1,1,1,1,1,1,1,1,1,1,1,1,1,1,1,1,6),(0.,0.005,0.01,0.015,0.02,
0.025,0.03,0.035,0.04,0.045,0.05,0.055,0.06,0.065,0.07,0.075,0.08,0.085,
0.09,0.095,0.1,0.105,0.11,0.115,0.12,0.125,0.13,0.135,0.14,0.145,0.15,0.155,
0.16,0.165,0.17,0.175,0.18,0.185,0.19,0.195,0.2,0.205,0.21,0.215,0.22,0.225,
0.23,0.235,0.24,0.245,0.25,0.255,0.26,0.265,0.27,0.275,0.28,0.285,0.29,
0.295,0.3,0.305,0.31,0.315,0.32,0.325,0.33,0.335,0.34,0.345,0.35,0.355,
0.36,0.365,0.37,0.375,0.38,0.385,0.39,0.395,0.4,0.405,0.41,0.415,0.42,0.425,
0.43,0.435,0.44,0.445,0.45,0.455,0.46,0.465,0.47,0.475,0.48,0.485,0.49,
0.495,0.5,0.505,0.51,0.515,0.52,0.525,0.53,0.535,0.54,0.545,0.55,0.555,
0.56,0.565,0.57,0.575,0.58,0.585,0.59,0.595,0.6,0.605,0.61,0.615,0.62,0.625,
0.63,0.635,0.64,0.645,0.65,0.655,0.66,0.665,0.67,0.675,0.68,0.685,0.690000000000001,
0.695000000000001,0.700000000000001,0.705000000000001,0.710000000000001,
0.715000000000001,0.720000000000001,0.725000000000001,0.730000000000001,
0.735000000000001,0.740000000000001,0.745000000000001,0.750000000000001,
0.755000000000001,0.760000000000001,0.765000000000001,0.770000000000001,
0.775000000000001,0.780000000000001,0.785000000000001,0.790000000000001,
0.795000000000001,0.800000000000001,0.805000000000001,0.810000000000001,
0.815000000000001,0.820000000000001,0.825000000000001,0.830000000000001,
0.835000000000001,0.840000000000001,0.845000000000001,0.850000000000001,
0.855000000000001,0.860000000000001,0.865000000000001,0.870000000000001,
0.875000000000001,0.880000000000001,0.885000000000001,0.890000000000001,
0.895000000000001,0.900000000000001,0.905000000000001,0.910000000000001,
0.915000000000001,0.920000000000001,0.925000000000001,0.930000000000001,
0.935000000000001,0.940000000000001,0.941429844438099),.UNSPECIFIED.)
CURVE()
GEOMETRIC_REPRESENTATION_ITEM()
RATIONAL_B_SPLINE_CURVE((1.,1.,1.,1.,1.,1.,1.,1.,1.,1.,1.,1.,1.,1.,1.,1.,
1.,1.,1.,1.,1.,1.,1.,1.,1.,1.,1.,1.,1.,1.,1.,1.,1.,1.,1.,1.,1.,1.,1.,1.,
1.,1.,1.,1.,1.,1.,1.,1.,1.,1.,1.,1.,1.,1.,1.,1.,1.,1.,1.,1.,1.,1.,1.,1.,
1.,1.,1.,1.,1.,1.,1.,1.,1.,1.,1.,1.,1.,1.,1.,1.,1.,1.,1.,1.,1.,1.,1.,1.,
1.,1.,1.,1.,1.,1.,1.,1.,1.,1.,1.,1.,1.,1.,1.,1.,1.,1.,1.,1.,1.,1.,1.,1.,
1.,1.,1.,1.,1.,1.,1.,1.,1.,1.,1.,1.,1.,1.,1.,1.,1.,1.,1.,1.,1.,1.,1.,1.,
1.,1.,1.,1.,1.,1.,1.,1.,1.,1.,1.,1.,1.,1.,1.,1.,1.,1.,1.,1.,1.,1.,1.,1.,
1.,1.,1.,1.,1.,1.,1.,1.,1.,1.,1.,1.,1.,1.,1.,1.,1.,1.,1.,1.,1.,1.,1.,1.,
1.,1.,1.,1.,1.,1.,1.,1.,1.,1.))
REPRESENTATION_ITEM('')
);
#556=(
BOUNDED_CURVE()
B_SPLINE_CURVE(5,(#120804,#120805,#120806,#120807,#120808,#120809,#120810,
#120811,#120812,#120813,#120814,#120815,#120816,#120817,#120818,#120819,
#120820,#120821,#120822,#120823,#120824,#120825,#120826,#120827,#120828,
#120829,#120830,#120831,#120832,#120833,#120834,#120835,#120836,#120837,
#120838,#120839,#120840,#120841,#120842,#120843,#120844,#120845,#120846,
#120847,#120848,#120849,#120850,#120851,#120852,#120853,#120854,#120855,
#120856,#120857,#120858,#120859,#120860,#120861,#120862,#120863,#120864,
#120865,#120866,#120867,#120868,#120869,#120870,#120871,#120872,#120873,
#120874,#120875,#120876,#120877,#120878,#120879,#120880,#120881,#120882,
#120883,#120884,#120885,#120886,#120887,#120888,#120889,#120890,#120891,
#120892,#120893,#120894,#120895,#120896,#120897,#120898,#120899,#120900,
#120901,#120902,#120903,#120904,#120905,#120906,#120907,#120908,#120909,
#120910,#120911,#120912,#120913,#120914,#120915,#120916,#120917,#120918,
#120919,#120920,#120921,#120922,#120923,#120924,#120925,#120926,#120927,
#120928,#120929,#120930,#120931,#120932,#120933,#120934,#120935,#120936,
#120937,#120938,#120939,#120940,#120941,#120942,#120943,#120944,#120945,
#120946,#120947,#120948,#120949,#120950,#120951,#120952,#120953,#120954,
#120955,#120956,#120957,#120958,#120959,#120960,#120961,#120962,#120963,
#120964,#120965,#120966,#120967,#120968,#120969,#120970,#120971,#120972,
#120973,#120974,#120975,#120976,#120977,#120978,#120979,#120980,#120981,
#120982,#120983,#120984,#120985,#120986,#120987,#120988,#120989,#120990,
#120991,#120992,#120993,#120994,#120995,#120996,#120997),.UNSPECIFIED.,
 .F.,.F.)
B_SPLINE_CURVE_WITH_KNOTS((6,1,1,1,1,1,1,1,1,1,1,1,1,1,1,1,1,1,1,1,1,1,
1,1,1,1,1,1,1,1,1,1,1,1,1,1,1,1,1,1,1,1,1,1,1,1,1,1,1,1,1,1,1,1,1,1,1,1,
1,1,1,1,1,1,1,1,1,1,1,1,1,1,1,1,1,1,1,1,1,1,1,1,1,1,1,1,1,1,1,1,1,1,1,1,
1,1,1,1,1,1,1,1,1,1,1,1,1,1,1,1,1,1,1,1,1,1,1,1,1,1,1,1,1,1,1,1,1,1,1,1,
1,1,1,1,1,1,1,1,1,1,1,1,1,1,1,1,1,1,1,1,1,1,1,1,1,1,1,1,1,1,1,1,1,1,1,1,
1,1,1,1,1,1,1,1,1,1,1,1,1,1,1,1,1,1,1,1,1,1,1,6),(-0.941429844438094,-0.940000000000001,
-0.935000000000001,-0.930000000000001,-0.925000000000001,-0.920000000000001,
-0.915000000000001,-0.910000000000001,-0.905000000000001,-0.900000000000001,
-0.895000000000001,-0.890000000000001,-0.885000000000001,-0.880000000000001,
-0.875000000000001,-0.870000000000001,-0.865000000000001,-0.860000000000001,
-0.855000000000001,-0.850000000000001,-0.845000000000001,-0.840000000000001,
-0.835000000000001,-0.830000000000001,-0.825000000000001,-0.820000000000001,
-0.815000000000001,-0.810000000000001,-0.805000000000001,-0.800000000000001,
-0.795000000000001,-0.790000000000001,-0.785000000000001,-0.780000000000001,
-0.775000000000001,-0.770000000000001,-0.765000000000001,-0.760000000000001,
-0.755000000000001,-0.750000000000001,-0.745000000000001,-0.740000000000001,
-0.735000000000001,-0.730000000000001,-0.725000000000001,-0.720000000000001,
-0.715000000000001,-0.710000000000001,-0.705000000000001,-0.700000000000001,
-0.695000000000001,-0.690000000000001,-0.685,-0.68,-0.675,-0.67,-0.665,
-0.66,-0.655,-0.65,-0.645,-0.64,-0.635,-0.63,-0.625,-0.62,-0.615,-0.61,
-0.605,-0.6,-0.595,-0.59,-0.585,-0.58,-0.575,-0.57,-0.565,-0.56,-0.555,
-0.55,-0.545,-0.54,-0.535,-0.53,-0.525,-0.52,-0.515,-0.51,-0.505,-0.5,-0.495,
-0.49,-0.485,-0.48,-0.475,-0.47,-0.465,-0.46,-0.455,-0.45,-0.445,-0.44,
-0.435,-0.43,-0.425,-0.42,-0.415,-0.41,-0.405,-0.4,-0.395,-0.39,-0.385,
-0.38,-0.375,-0.37,-0.365,-0.36,-0.355,-0.35,-0.345,-0.34,-0.335,-0.33,
-0.325,-0.32,-0.315,-0.31,-0.305,-0.3,-0.295,-0.29,-0.285,-0.28,-0.275,
-0.27,-0.265,-0.26,-0.255,-0.25,-0.245,-0.24,-0.235,-0.23,-0.225,-0.22,
-0.215,-0.21,-0.205,-0.2,-0.195,-0.19,-0.185,-0.18,-0.175,-0.17,-0.165,
-0.16,-0.155,-0.15,-0.145,-0.14,-0.135,-0.13,-0.125,-0.12,-0.115,-0.11,
-0.105,-0.1,-0.095,-0.09,-0.085,-0.08,-0.075,-0.07,-0.065,-0.06,-0.055,
-0.05,-0.045,-0.04,-0.035,-0.03,-0.025,-0.02,-0.015,-0.01,-0.005,0.),
 .UNSPECIFIED.)
CURVE()
GEOMETRIC_REPRESENTATION_ITEM()
RATIONAL_B_SPLINE_CURVE((1.,1.,1.,1.,1.,1.,1.,1.,1.,1.,1.,1.,1.,1.,1.,1.,
1.,1.,1.,1.,1.,1.,1.,1.,1.,1.,1.,1.,1.,1.,1.,1.,1.,1.,1.,1.,1.,1.,1.,1.,
1.,1.,1.,1.,1.,1.,1.,1.,1.,1.,1.,1.,1.,1.,1.,1.,1.,1.,1.,1.,1.,1.,1.,1.,
1.,1.,1.,1.,1.,1.,1.,1.,1.,1.,1.,1.,1.,1.,1.,1.,1.,1.,1.,1.,1.,1.,1.,1.,
1.,1.,1.,1.,1.,1.,1.,1.,1.,1.,1.,1.,1.,1.,1.,1.,1.,1.,1.,1.,1.,1.,1.,1.,
1.,1.,1.,1.,1.,1.,1.,1.,1.,1.,1.,1.,1.,1.,1.,1.,1.,1.,1.,1.,1.,1.,1.,1.,
1.,1.,1.,1.,1.,1.,1.,1.,1.,1.,1.,1.,1.,1.,1.,1.,1.,1.,1.,1.,1.,1.,1.,1.,
1.,1.,1.,1.,1.,1.,1.,1.,1.,1.,1.,1.,1.,1.,1.,1.,1.,1.,1.,1.,1.,1.,1.,1.,
1.,1.,1.,1.,1.,1.,1.,1.,1.,1.))
REPRESENTATION_ITEM('')
);
#557=(
BOUNDED_CURVE()
B_SPLINE_CURVE(5,(#121409,#121410,#121411,#121412,#121413,#121414,#121415,
#121416,#121417,#121418,#121419,#121420,#121421,#121422,#121423,#121424,
#121425,#121426,#121427,#121428,#121429,#121430,#121431,#121432,#121433,
#121434,#121435,#121436,#121437,#121438,#121439,#121440,#121441,#121442,
#121443,#121444,#121445,#121446,#121447,#121448,#121449,#121450,#121451,
#121452,#121453,#121454,#121455,#121456,#121457,#121458,#121459,#121460,
#121461,#121462,#121463,#121464,#121465,#121466,#121467,#121468,#121469,
#121470,#121471,#121472,#121473,#121474,#121475,#121476,#121477,#121478,
#121479,#121480,#121481,#121482,#121483,#121484,#121485,#121486,#121487,
#121488,#121489,#121490,#121491,#121492,#121493,#121494,#121495,#121496,
#121497,#121498,#121499,#121500,#121501,#121502,#121503,#121504,#121505,
#121506,#121507,#121508,#121509,#121510,#121511,#121512,#121513,#121514,
#121515,#121516,#121517,#121518,#121519,#121520,#121521,#121522,#121523,
#121524,#121525,#121526,#121527,#121528,#121529,#121530,#121531,#121532,
#121533,#121534,#121535,#121536,#121537,#121538,#121539,#121540,#121541,
#121542,#121543,#121544,#121545,#121546,#121547,#121548,#121549,#121550,
#121551,#121552,#121553,#121554,#121555,#121556,#121557,#121558,#121559,
#121560,#121561,#121562,#121563,#121564,#121565,#121566,#121567,#121568,
#121569,#121570,#121571,#121572,#121573,#121574,#121575,#121576,#121577,
#121578,#121579,#121580,#121581,#121582,#121583,#121584,#121585,#121586,
#121587,#121588,#121589,#121590,#121591,#121592,#121593,#121594,#121595,
#121596,#121597,#121598,#121599,#121600,#121601,#121602),.UNSPECIFIED.,
 .F.,.F.)
B_SPLINE_CURVE_WITH_KNOTS((6,1,1,1,1,1,1,1,1,1,1,1,1,1,1,1,1,1,1,1,1,1,
1,1,1,1,1,1,1,1,1,1,1,1,1,1,1,1,1,1,1,1,1,1,1,1,1,1,1,1,1,1,1,1,1,1,1,1,
1,1,1,1,1,1,1,1,1,1,1,1,1,1,1,1,1,1,1,1,1,1,1,1,1,1,1,1,1,1,1,1,1,1,1,1,
1,1,1,1,1,1,1,1,1,1,1,1,1,1,1,1,1,1,1,1,1,1,1,1,1,1,1,1,1,1,1,1,1,1,1,1,
1,1,1,1,1,1,1,1,1,1,1,1,1,1,1,1,1,1,1,1,1,1,1,1,1,1,1,1,1,1,1,1,1,1,1,1,
1,1,1,1,1,1,1,1,1,1,1,1,1,1,1,1,1,1,1,1,1,1,1,6),(0.,0.005,0.01,0.015,0.02,
0.025,0.03,0.035,0.04,0.045,0.05,0.055,0.06,0.065,0.07,0.075,0.08,0.085,
0.09,0.095,0.1,0.105,0.11,0.115,0.12,0.125,0.13,0.135,0.14,0.145,0.15,0.155,
0.16,0.165,0.17,0.175,0.18,0.185,0.19,0.195,0.2,0.205,0.21,0.215,0.22,0.225,
0.23,0.235,0.24,0.245,0.25,0.255,0.26,0.265,0.27,0.275,0.28,0.285,0.29,
0.295,0.3,0.305,0.31,0.315,0.32,0.325,0.33,0.335,0.34,0.345,0.35,0.355,
0.36,0.365,0.37,0.375,0.38,0.385,0.39,0.395,0.4,0.405,0.41,0.415,0.42,0.425,
0.43,0.435,0.44,0.445,0.45,0.455,0.46,0.465,0.47,0.475,0.48,0.485,0.49,
0.495,0.5,0.505,0.51,0.515,0.52,0.525,0.53,0.535,0.54,0.545,0.55,0.555,
0.56,0.565,0.57,0.575,0.58,0.585,0.59,0.595,0.6,0.605,0.61,0.615,0.62,0.625,
0.63,0.635,0.64,0.645,0.65,0.655,0.66,0.665,0.67,0.675,0.68,0.685,0.690000000000001,
0.695000000000001,0.700000000000001,0.705000000000001,0.710000000000001,
0.715000000000001,0.720000000000001,0.725000000000001,0.730000000000001,
0.735000000000001,0.740000000000001,0.745000000000001,0.750000000000001,
0.755000000000001,0.760000000000001,0.765000000000001,0.770000000000001,
0.775000000000001,0.780000000000001,0.785000000000001,0.790000000000001,
0.795000000000001,0.800000000000001,0.805000000000001,0.810000000000001,
0.815000000000001,0.820000000000001,0.825000000000001,0.830000000000001,
0.835000000000001,0.840000000000001,0.845000000000001,0.850000000000001,
0.855000000000001,0.860000000000001,0.865000000000001,0.870000000000001,
0.875000000000001,0.880000000000001,0.885000000000001,0.890000000000001,
0.895000000000001,0.900000000000001,0.905000000000001,0.910000000000001,
0.915000000000001,0.920000000000001,0.925000000000001,0.930000000000001,
0.935000000000001,0.940000000000001,0.941429844437999),.UNSPECIFIED.)
CURVE()
GEOMETRIC_REPRESENTATION_ITEM()
RATIONAL_B_SPLINE_CURVE((1.,1.,1.,1.,1.,1.,1.,1.,1.,1.,1.,1.,1.,1.,1.,1.,
1.,1.,1.,1.,1.,1.,1.,1.,1.,1.,1.,1.,1.,1.,1.,1.,1.,1.,1.,1.,1.,1.,1.,1.,
1.,1.,1.,1.,1.,1.,1.,1.,1.,1.,1.,1.,1.,1.,1.,1.,1.,1.,1.,1.,1.,1.,1.,1.,
1.,1.,1.,1.,1.,1.,1.,1.,1.,1.,1.,1.,1.,1.,1.,1.,1.,1.,1.,1.,1.,1.,1.,1.,
1.,1.,1.,1.,1.,1.,1.,1.,1.,1.,1.,1.,1.,1.,1.,1.,1.,1.,1.,1.,1.,1.,1.,1.,
1.,1.,1.,1.,1.,1.,1.,1.,1.,1.,1.,1.,1.,1.,1.,1.,1.,1.,1.,1.,1.,1.,1.,1.,
1.,1.,1.,1.,1.,1.,1.,1.,1.,1.,1.,1.,1.,1.,1.,1.,1.,1.,1.,1.,1.,1.,1.,1.,
1.,1.,1.,1.,1.,1.,1.,1.,1.,1.,1.,1.,1.,1.,1.,1.,1.,1.,1.,1.,1.,1.,1.,1.,
1.,1.,1.,1.,1.,1.,1.,1.,1.,1.))
REPRESENTATION_ITEM('')
);
#558=(
BOUNDED_CURVE()
B_SPLINE_CURVE(5,(#121605,#121606,#121607,#121608,#121609,#121610,#121611,
#121612,#121613,#121614,#121615,#121616,#121617,#121618,#121619,#121620,
#121621,#121622,#121623,#121624,#121625,#121626,#121627,#121628,#121629,
#121630,#121631,#121632,#121633,#121634,#121635,#121636,#121637,#121638,
#121639,#121640,#121641,#121642,#121643,#121644,#121645,#121646,#121647,
#121648,#121649,#121650,#121651,#121652,#121653,#121654,#121655,#121656,
#121657,#121658,#121659,#121660,#121661,#121662,#121663,#121664,#121665,
#121666,#121667,#121668,#121669,#121670,#121671,#121672,#121673,#121674,
#121675,#121676,#121677,#121678,#121679,#121680,#121681,#121682,#121683,
#121684,#121685,#121686,#121687,#121688,#121689,#121690,#121691,#121692,
#121693,#121694,#121695,#121696,#121697,#121698,#121699,#121700,#121701,
#121702,#121703,#121704,#121705,#121706,#121707,#121708,#121709,#121710,
#121711,#121712,#121713,#121714,#121715,#121716,#121717,#121718,#121719,
#121720,#121721,#121722,#121723,#121724,#121725,#121726,#121727,#121728,
#121729,#121730,#121731,#121732,#121733,#121734,#121735,#121736,#121737,
#121738,#121739,#121740,#121741,#121742,#121743,#121744,#121745,#121746,
#121747,#121748,#121749,#121750,#121751,#121752,#121753,#121754,#121755,
#121756,#121757,#121758,#121759,#121760,#121761,#121762,#121763,#121764,
#121765,#121766,#121767,#121768,#121769,#121770,#121771,#121772,#121773,
#121774,#121775,#121776,#121777,#121778,#121779,#121780,#121781,#121782,
#121783,#121784,#121785,#121786,#121787,#121788,#121789,#121790,#121791,
#121792,#121793,#121794,#121795,#121796,#121797,#121798),.UNSPECIFIED.,
 .F.,.F.)
B_SPLINE_CURVE_WITH_KNOTS((6,1,1,1,1,1,1,1,1,1,1,1,1,1,1,1,1,1,1,1,1,1,
1,1,1,1,1,1,1,1,1,1,1,1,1,1,1,1,1,1,1,1,1,1,1,1,1,1,1,1,1,1,1,1,1,1,1,1,
1,1,1,1,1,1,1,1,1,1,1,1,1,1,1,1,1,1,1,1,1,1,1,1,1,1,1,1,1,1,1,1,1,1,1,1,
1,1,1,1,1,1,1,1,1,1,1,1,1,1,1,1,1,1,1,1,1,1,1,1,1,1,1,1,1,1,1,1,1,1,1,1,
1,1,1,1,1,1,1,1,1,1,1,1,1,1,1,1,1,1,1,1,1,1,1,1,1,1,1,1,1,1,1,1,1,1,1,1,
1,1,1,1,1,1,1,1,1,1,1,1,1,1,1,1,1,1,1,1,1,1,1,6),(-0.941429844438006,-0.940000000000001,
-0.935000000000001,-0.930000000000001,-0.925000000000001,-0.920000000000001,
-0.915000000000001,-0.910000000000001,-0.905000000000001,-0.900000000000001,
-0.895000000000001,-0.890000000000001,-0.885000000000001,-0.880000000000001,
-0.875000000000001,-0.870000000000001,-0.865000000000001,-0.860000000000001,
-0.855000000000001,-0.850000000000001,-0.845000000000001,-0.840000000000001,
-0.835000000000001,-0.830000000000001,-0.825000000000001,-0.820000000000001,
-0.815000000000001,-0.810000000000001,-0.805000000000001,-0.800000000000001,
-0.795000000000001,-0.790000000000001,-0.785000000000001,-0.780000000000001,
-0.775000000000001,-0.770000000000001,-0.765000000000001,-0.760000000000001,
-0.755000000000001,-0.750000000000001,-0.745000000000001,-0.740000000000001,
-0.735000000000001,-0.730000000000001,-0.725000000000001,-0.720000000000001,
-0.715000000000001,-0.710000000000001,-0.705000000000001,-0.700000000000001,
-0.695000000000001,-0.690000000000001,-0.685,-0.68,-0.675,-0.67,-0.665,
-0.66,-0.655,-0.65,-0.645,-0.64,-0.635,-0.63,-0.625,-0.62,-0.615,-0.61,
-0.605,-0.6,-0.595,-0.59,-0.585,-0.58,-0.575,-0.57,-0.565,-0.56,-0.555,
-0.55,-0.545,-0.54,-0.535,-0.53,-0.525,-0.52,-0.515,-0.51,-0.505,-0.5,-0.495,
-0.49,-0.485,-0.48,-0.475,-0.47,-0.465,-0.46,-0.455,-0.45,-0.445,-0.44,
-0.435,-0.43,-0.425,-0.42,-0.415,-0.41,-0.405,-0.4,-0.395,-0.39,-0.385,
-0.38,-0.375,-0.37,-0.365,-0.36,-0.355,-0.35,-0.345,-0.34,-0.335,-0.33,
-0.325,-0.32,-0.315,-0.31,-0.305,-0.3,-0.295,-0.29,-0.285,-0.28,-0.275,
-0.27,-0.265,-0.26,-0.255,-0.25,-0.245,-0.24,-0.235,-0.23,-0.225,-0.22,
-0.215,-0.21,-0.205,-0.2,-0.195,-0.19,-0.185,-0.18,-0.175,-0.17,-0.165,
-0.16,-0.155,-0.15,-0.145,-0.14,-0.135,-0.13,-0.125,-0.12,-0.115,-0.11,
-0.105,-0.1,-0.095,-0.09,-0.085,-0.08,-0.075,-0.07,-0.065,-0.06,-0.055,
-0.05,-0.045,-0.04,-0.035,-0.03,-0.025,-0.02,-0.015,-0.01,-0.005,0.),
 .UNSPECIFIED.)
CURVE()
GEOMETRIC_REPRESENTATION_ITEM()
RATIONAL_B_SPLINE_CURVE((1.,1.,1.,1.,1.,1.,1.,1.,1.,1.,1.,1.,1.,1.,1.,1.,
1.,1.,1.,1.,1.,1.,1.,1.,1.,1.,1.,1.,1.,1.,1.,1.,1.,1.,1.,1.,1.,1.,1.,1.,
1.,1.,1.,1.,1.,1.,1.,1.,1.,1.,1.,1.,1.,1.,1.,1.,1.,1.,1.,1.,1.,1.,1.,1.,
1.,1.,1.,1.,1.,1.,1.,1.,1.,1.,1.,1.,1.,1.,1.,1.,1.,1.,1.,1.,1.,1.,1.,1.,
1.,1.,1.,1.,1.,1.,1.,1.,1.,1.,1.,1.,1.,1.,1.,1.,1.,1.,1.,1.,1.,1.,1.,1.,
1.,1.,1.,1.,1.,1.,1.,1.,1.,1.,1.,1.,1.,1.,1.,1.,1.,1.,1.,1.,1.,1.,1.,1.,
1.,1.,1.,1.,1.,1.,1.,1.,1.,1.,1.,1.,1.,1.,1.,1.,1.,1.,1.,1.,1.,1.,1.,1.,
1.,1.,1.,1.,1.,1.,1.,1.,1.,1.,1.,1.,1.,1.,1.,1.,1.,1.,1.,1.,1.,1.,1.,1.,
1.,1.,1.,1.,1.,1.,1.,1.,1.,1.))
REPRESENTATION_ITEM('')
);
#559=(
BOUNDED_CURVE()
B_SPLINE_CURVE(5,(#122210,#122211,#122212,#122213,#122214,#122215,#122216,
#122217,#122218,#122219,#122220,#122221,#122222,#122223,#122224,#122225,
#122226,#122227,#122228,#122229,#122230,#122231,#122232,#122233,#122234,
#122235,#122236,#122237,#122238,#122239,#122240,#122241,#122242,#122243,
#122244,#122245,#122246,#122247,#122248,#122249,#122250,#122251,#122252,
#122253,#122254,#122255,#122256,#122257,#122258,#122259,#122260,#122261,
#122262,#122263,#122264,#122265,#122266,#122267,#122268,#122269,#122270,
#122271,#122272,#122273,#122274,#122275,#122276,#122277,#122278,#122279,
#122280,#122281,#122282,#122283,#122284,#122285,#122286,#122287,#122288,
#122289,#122290,#122291,#122292,#122293,#122294,#122295,#122296,#122297,
#122298,#122299,#122300,#122301,#122302,#122303,#122304,#122305,#122306,
#122307,#122308,#122309,#122310,#122311,#122312,#122313,#122314,#122315,
#122316,#122317,#122318,#122319,#122320,#122321,#122322,#122323,#122324,
#122325,#122326,#122327,#122328,#122329,#122330,#122331,#122332,#122333,
#122334,#122335,#122336,#122337,#122338,#122339,#122340,#122341,#122342,
#122343,#122344,#122345,#122346,#122347,#122348,#122349,#122350,#122351,
#122352,#122353,#122354,#122355,#122356,#122357,#122358,#122359,#122360,
#122361,#122362,#122363,#122364,#122365,#122366,#122367,#122368,#122369,
#122370,#122371,#122372,#122373,#122374,#122375,#122376,#122377,#122378,
#122379,#122380,#122381,#122382,#122383,#122384,#122385,#122386,#122387,
#122388,#122389,#122390,#122391,#122392,#122393,#122394,#122395,#122396,
#122397,#122398,#122399,#122400,#122401,#122402,#122403),.UNSPECIFIED.,
 .F.,.F.)
B_SPLINE_CURVE_WITH_KNOTS((6,1,1,1,1,1,1,1,1,1,1,1,1,1,1,1,1,1,1,1,1,1,
1,1,1,1,1,1,1,1,1,1,1,1,1,1,1,1,1,1,1,1,1,1,1,1,1,1,1,1,1,1,1,1,1,1,1,1,
1,1,1,1,1,1,1,1,1,1,1,1,1,1,1,1,1,1,1,1,1,1,1,1,1,1,1,1,1,1,1,1,1,1,1,1,
1,1,1,1,1,1,1,1,1,1,1,1,1,1,1,1,1,1,1,1,1,1,1,1,1,1,1,1,1,1,1,1,1,1,1,1,
1,1,1,1,1,1,1,1,1,1,1,1,1,1,1,1,1,1,1,1,1,1,1,1,1,1,1,1,1,1,1,1,1,1,1,1,
1,1,1,1,1,1,1,1,1,1,1,1,1,1,1,1,1,1,1,1,1,1,1,6),(0.,0.005,0.01,0.015,0.02,
0.025,0.03,0.035,0.04,0.045,0.05,0.055,0.06,0.065,0.07,0.075,0.08,0.085,
0.09,0.095,0.1,0.105,0.11,0.115,0.12,0.125,0.13,0.135,0.14,0.145,0.15,0.155,
0.16,0.165,0.17,0.175,0.18,0.185,0.19,0.195,0.2,0.205,0.21,0.215,0.22,0.225,
0.23,0.235,0.24,0.245,0.25,0.255,0.26,0.265,0.27,0.275,0.28,0.285,0.29,
0.295,0.3,0.305,0.31,0.315,0.32,0.325,0.33,0.335,0.34,0.345,0.35,0.355,
0.36,0.365,0.37,0.375,0.38,0.385,0.39,0.395,0.4,0.405,0.41,0.415,0.42,0.425,
0.43,0.435,0.44,0.445,0.45,0.455,0.46,0.465,0.47,0.475,0.48,0.485,0.49,
0.495,0.5,0.505,0.51,0.515,0.52,0.525,0.53,0.535,0.54,0.545,0.55,0.555,
0.56,0.565,0.57,0.575,0.58,0.585,0.59,0.595,0.6,0.605,0.61,0.615,0.62,0.625,
0.63,0.635,0.64,0.645,0.65,0.655,0.66,0.665,0.67,0.675,0.68,0.685,0.690000000000001,
0.695000000000001,0.700000000000001,0.705000000000001,0.710000000000001,
0.715000000000001,0.720000000000001,0.725000000000001,0.730000000000001,
0.735000000000001,0.740000000000001,0.745000000000001,0.750000000000001,
0.755000000000001,0.760000000000001,0.765000000000001,0.770000000000001,
0.775000000000001,0.780000000000001,0.785000000000001,0.790000000000001,
0.795000000000001,0.800000000000001,0.805000000000001,0.810000000000001,
0.815000000000001,0.820000000000001,0.825000000000001,0.830000000000001,
0.835000000000001,0.840000000000001,0.845000000000001,0.850000000000001,
0.855000000000001,0.860000000000001,0.865000000000001,0.870000000000001,
0.875000000000001,0.880000000000001,0.885000000000001,0.890000000000001,
0.895000000000001,0.900000000000001,0.905000000000001,0.910000000000001,
0.915000000000001,0.920000000000001,0.925000000000001,0.930000000000001,
0.935000000000001,0.940000000000001,0.94142984443805),.UNSPECIFIED.)
CURVE()
GEOMETRIC_REPRESENTATION_ITEM()
RATIONAL_B_SPLINE_CURVE((1.,1.,1.,1.,1.,1.,1.,1.,1.,1.,1.,1.,1.,1.,1.,1.,
1.,1.,1.,1.,1.,1.,1.,1.,1.,1.,1.,1.,1.,1.,1.,1.,1.,1.,1.,1.,1.,1.,1.,1.,
1.,1.,1.,1.,1.,1.,1.,1.,1.,1.,1.,1.,1.,1.,1.,1.,1.,1.,1.,1.,1.,1.,1.,1.,
1.,1.,1.,1.,1.,1.,1.,1.,1.,1.,1.,1.,1.,1.,1.,1.,1.,1.,1.,1.,1.,1.,1.,1.,
1.,1.,1.,1.,1.,1.,1.,1.,1.,1.,1.,1.,1.,1.,1.,1.,1.,1.,1.,1.,1.,1.,1.,1.,
1.,1.,1.,1.,1.,1.,1.,1.,1.,1.,1.,1.,1.,1.,1.,1.,1.,1.,1.,1.,1.,1.,1.,1.,
1.,1.,1.,1.,1.,1.,1.,1.,1.,1.,1.,1.,1.,1.,1.,1.,1.,1.,1.,1.,1.,1.,1.,1.,
1.,1.,1.,1.,1.,1.,1.,1.,1.,1.,1.,1.,1.,1.,1.,1.,1.,1.,1.,1.,1.,1.,1.,1.,
1.,1.,1.,1.,1.,1.,1.,1.,1.,1.))
REPRESENTATION_ITEM('')
);
#560=(
BOUNDED_CURVE()
B_SPLINE_CURVE(5,(#122406,#122407,#122408,#122409,#122410,#122411,#122412,
#122413,#122414,#122415,#122416,#122417,#122418,#122419,#122420,#122421,
#122422,#122423,#122424,#122425,#122426,#122427,#122428,#122429,#122430,
#122431,#122432,#122433,#122434,#122435,#122436,#122437,#122438,#122439,
#122440,#122441,#122442,#122443,#122444,#122445,#122446,#122447,#122448,
#122449,#122450,#122451,#122452,#122453,#122454,#122455,#122456,#122457,
#122458,#122459,#122460,#122461,#122462,#122463,#122464,#122465,#122466,
#122467,#122468,#122469,#122470,#122471,#122472,#122473,#122474,#122475,
#122476,#122477,#122478,#122479,#122480,#122481,#122482,#122483,#122484,
#122485,#122486,#122487,#122488,#122489,#122490,#122491,#122492,#122493,
#122494,#122495,#122496,#122497,#122498,#122499,#122500,#122501,#122502,
#122503,#122504,#122505,#122506,#122507,#122508,#122509,#122510,#122511,
#122512,#122513,#122514,#122515,#122516,#122517,#122518,#122519,#122520,
#122521,#122522,#122523,#122524,#122525,#122526,#122527,#122528,#122529,
#122530,#122531,#122532,#122533,#122534,#122535,#122536,#122537,#122538,
#122539,#122540,#122541,#122542,#122543,#122544,#122545,#122546,#122547,
#122548,#122549,#122550,#122551,#122552,#122553,#122554,#122555,#122556,
#122557,#122558,#122559,#122560,#122561,#122562,#122563,#122564,#122565,
#122566,#122567,#122568,#122569,#122570,#122571,#122572,#122573,#122574,
#122575,#122576,#122577,#122578,#122579,#122580,#122581,#122582,#122583,
#122584,#122585,#122586,#122587,#122588,#122589,#122590,#122591,#122592,
#122593,#122594,#122595,#122596,#122597,#122598,#122599),.UNSPECIFIED.,
 .F.,.F.)
B_SPLINE_CURVE_WITH_KNOTS((6,1,1,1,1,1,1,1,1,1,1,1,1,1,1,1,1,1,1,1,1,1,
1,1,1,1,1,1,1,1,1,1,1,1,1,1,1,1,1,1,1,1,1,1,1,1,1,1,1,1,1,1,1,1,1,1,1,1,
1,1,1,1,1,1,1,1,1,1,1,1,1,1,1,1,1,1,1,1,1,1,1,1,1,1,1,1,1,1,1,1,1,1,1,1,
1,1,1,1,1,1,1,1,1,1,1,1,1,1,1,1,1,1,1,1,1,1,1,1,1,1,1,1,1,1,1,1,1,1,1,1,
1,1,1,1,1,1,1,1,1,1,1,1,1,1,1,1,1,1,1,1,1,1,1,1,1,1,1,1,1,1,1,1,1,1,1,1,
1,1,1,1,1,1,1,1,1,1,1,1,1,1,1,1,1,1,1,1,1,1,1,6),(-0.941429844438018,-0.940000000000001,
-0.935000000000001,-0.930000000000001,-0.925000000000001,-0.920000000000001,
-0.915000000000001,-0.910000000000001,-0.905000000000001,-0.900000000000001,
-0.895000000000001,-0.890000000000001,-0.885000000000001,-0.880000000000001,
-0.875000000000001,-0.870000000000001,-0.865000000000001,-0.860000000000001,
-0.855000000000001,-0.850000000000001,-0.845000000000001,-0.840000000000001,
-0.835000000000001,-0.830000000000001,-0.825000000000001,-0.820000000000001,
-0.815000000000001,-0.810000000000001,-0.805000000000001,-0.800000000000001,
-0.795000000000001,-0.790000000000001,-0.785000000000001,-0.780000000000001,
-0.775000000000001,-0.770000000000001,-0.765000000000001,-0.760000000000001,
-0.755000000000001,-0.750000000000001,-0.745000000000001,-0.740000000000001,
-0.735000000000001,-0.730000000000001,-0.725000000000001,-0.720000000000001,
-0.715000000000001,-0.710000000000001,-0.705000000000001,-0.700000000000001,
-0.695000000000001,-0.690000000000001,-0.685,-0.68,-0.675,-0.67,-0.665,
-0.66,-0.655,-0.65,-0.645,-0.64,-0.635,-0.63,-0.625,-0.62,-0.615,-0.61,
-0.605,-0.6,-0.595,-0.59,-0.585,-0.58,-0.575,-0.57,-0.565,-0.56,-0.555,
-0.55,-0.545,-0.54,-0.535,-0.53,-0.525,-0.52,-0.515,-0.51,-0.505,-0.5,-0.495,
-0.49,-0.485,-0.48,-0.475,-0.47,-0.465,-0.46,-0.455,-0.45,-0.445,-0.44,
-0.435,-0.43,-0.425,-0.42,-0.415,-0.41,-0.405,-0.4,-0.395,-0.39,-0.385,
-0.38,-0.375,-0.37,-0.365,-0.36,-0.355,-0.35,-0.345,-0.34,-0.335,-0.33,
-0.325,-0.32,-0.315,-0.31,-0.305,-0.3,-0.295,-0.29,-0.285,-0.28,-0.275,
-0.27,-0.265,-0.26,-0.255,-0.25,-0.245,-0.24,-0.235,-0.23,-0.225,-0.22,
-0.215,-0.21,-0.205,-0.2,-0.195,-0.19,-0.185,-0.18,-0.175,-0.17,-0.165,
-0.16,-0.155,-0.15,-0.145,-0.14,-0.135,-0.13,-0.125,-0.12,-0.115,-0.11,
-0.105,-0.1,-0.095,-0.09,-0.085,-0.08,-0.075,-0.07,-0.065,-0.06,-0.055,
-0.05,-0.045,-0.04,-0.035,-0.03,-0.025,-0.02,-0.015,-0.01,-0.005,0.),
 .UNSPECIFIED.)
CURVE()
GEOMETRIC_REPRESENTATION_ITEM()
RATIONAL_B_SPLINE_CURVE((1.,1.,1.,1.,1.,1.,1.,1.,1.,1.,1.,1.,1.,1.,1.,1.,
1.,1.,1.,1.,1.,1.,1.,1.,1.,1.,1.,1.,1.,1.,1.,1.,1.,1.,1.,1.,1.,1.,1.,1.,
1.,1.,1.,1.,1.,1.,1.,1.,1.,1.,1.,1.,1.,1.,1.,1.,1.,1.,1.,1.,1.,1.,1.,1.,
1.,1.,1.,1.,1.,1.,1.,1.,1.,1.,1.,1.,1.,1.,1.,1.,1.,1.,1.,1.,1.,1.,1.,1.,
1.,1.,1.,1.,1.,1.,1.,1.,1.,1.,1.,1.,1.,1.,1.,1.,1.,1.,1.,1.,1.,1.,1.,1.,
1.,1.,1.,1.,1.,1.,1.,1.,1.,1.,1.,1.,1.,1.,1.,1.,1.,1.,1.,1.,1.,1.,1.,1.,
1.,1.,1.,1.,1.,1.,1.,1.,1.,1.,1.,1.,1.,1.,1.,1.,1.,1.,1.,1.,1.,1.,1.,1.,
1.,1.,1.,1.,1.,1.,1.,1.,1.,1.,1.,1.,1.,1.,1.,1.,1.,1.,1.,1.,1.,1.,1.,1.,
1.,1.,1.,1.,1.,1.,1.,1.,1.,1.))
REPRESENTATION_ITEM('')
);
#561=(
BOUNDED_CURVE()
B_SPLINE_CURVE(5,(#123011,#123012,#123013,#123014,#123015,#123016,#123017,
#123018,#123019,#123020,#123021,#123022,#123023,#123024,#123025,#123026,
#123027,#123028,#123029,#123030,#123031,#123032,#123033,#123034,#123035,
#123036,#123037,#123038,#123039,#123040,#123041,#123042,#123043,#123044,
#123045,#123046,#123047,#123048,#123049,#123050,#123051,#123052,#123053,
#123054,#123055,#123056,#123057,#123058,#123059,#123060,#123061,#123062,
#123063,#123064,#123065,#123066,#123067,#123068,#123069,#123070,#123071,
#123072,#123073,#123074,#123075,#123076,#123077,#123078,#123079,#123080,
#123081,#123082,#123083,#123084,#123085,#123086,#123087,#123088,#123089,
#123090,#123091,#123092,#123093,#123094,#123095,#123096,#123097,#123098,
#123099,#123100,#123101,#123102,#123103,#123104,#123105,#123106,#123107,
#123108,#123109,#123110,#123111,#123112,#123113,#123114,#123115,#123116,
#123117,#123118,#123119,#123120,#123121,#123122,#123123,#123124,#123125,
#123126,#123127,#123128,#123129,#123130,#123131,#123132,#123133,#123134,
#123135,#123136,#123137,#123138,#123139,#123140,#123141,#123142,#123143,
#123144,#123145,#123146,#123147,#123148,#123149,#123150,#123151,#123152,
#123153,#123154,#123155,#123156,#123157,#123158,#123159,#123160,#123161,
#123162,#123163,#123164,#123165,#123166,#123167,#123168,#123169,#123170,
#123171,#123172,#123173,#123174,#123175,#123176,#123177,#123178,#123179,
#123180,#123181,#123182,#123183,#123184,#123185,#123186,#123187,#123188,
#123189,#123190,#123191,#123192,#123193,#123194,#123195,#123196,#123197,
#123198,#123199,#123200,#123201,#123202,#123203,#123204),.UNSPECIFIED.,
 .F.,.F.)
B_SPLINE_CURVE_WITH_KNOTS((6,1,1,1,1,1,1,1,1,1,1,1,1,1,1,1,1,1,1,1,1,1,
1,1,1,1,1,1,1,1,1,1,1,1,1,1,1,1,1,1,1,1,1,1,1,1,1,1,1,1,1,1,1,1,1,1,1,1,
1,1,1,1,1,1,1,1,1,1,1,1,1,1,1,1,1,1,1,1,1,1,1,1,1,1,1,1,1,1,1,1,1,1,1,1,
1,1,1,1,1,1,1,1,1,1,1,1,1,1,1,1,1,1,1,1,1,1,1,1,1,1,1,1,1,1,1,1,1,1,1,1,
1,1,1,1,1,1,1,1,1,1,1,1,1,1,1,1,1,1,1,1,1,1,1,1,1,1,1,1,1,1,1,1,1,1,1,1,
1,1,1,1,1,1,1,1,1,1,1,1,1,1,1,1,1,1,1,1,1,1,1,6),(0.,0.005,0.01,0.015,0.02,
0.025,0.03,0.035,0.04,0.045,0.05,0.055,0.06,0.065,0.07,0.075,0.08,0.085,
0.09,0.095,0.1,0.105,0.11,0.115,0.12,0.125,0.13,0.135,0.14,0.145,0.15,0.155,
0.16,0.165,0.17,0.175,0.18,0.185,0.19,0.195,0.2,0.205,0.21,0.215,0.22,0.225,
0.23,0.235,0.24,0.245,0.25,0.255,0.26,0.265,0.27,0.275,0.28,0.285,0.29,
0.295,0.3,0.305,0.31,0.315,0.32,0.325,0.33,0.335,0.34,0.345,0.35,0.355,
0.36,0.365,0.37,0.375,0.38,0.385,0.39,0.395,0.4,0.405,0.41,0.415,0.42,0.425,
0.43,0.435,0.44,0.445,0.45,0.455,0.46,0.465,0.47,0.475,0.48,0.485,0.49,
0.495,0.5,0.505,0.51,0.515,0.52,0.525,0.53,0.535,0.54,0.545,0.55,0.555,
0.56,0.565,0.57,0.575,0.58,0.585,0.59,0.595,0.6,0.605,0.61,0.615,0.62,0.625,
0.63,0.635,0.64,0.645,0.65,0.655,0.66,0.665,0.67,0.675,0.68,0.685,0.690000000000001,
0.695000000000001,0.700000000000001,0.705000000000001,0.710000000000001,
0.715000000000001,0.720000000000001,0.725000000000001,0.730000000000001,
0.735000000000001,0.740000000000001,0.745000000000001,0.750000000000001,
0.755000000000001,0.760000000000001,0.765000000000001,0.770000000000001,
0.775000000000001,0.780000000000001,0.785000000000001,0.790000000000001,
0.795000000000001,0.800000000000001,0.805000000000001,0.810000000000001,
0.815000000000001,0.820000000000001,0.825000000000001,0.830000000000001,
0.835000000000001,0.840000000000001,0.845000000000001,0.850000000000001,
0.855000000000001,0.860000000000001,0.865000000000001,0.870000000000001,
0.875000000000001,0.880000000000001,0.885000000000001,0.890000000000001,
0.895000000000001,0.900000000000001,0.905000000000001,0.910000000000001,
0.915000000000001,0.920000000000001,0.925000000000001,0.930000000000001,
0.935000000000001,0.940000000000001,0.941429844438072),.UNSPECIFIED.)
CURVE()
GEOMETRIC_REPRESENTATION_ITEM()
RATIONAL_B_SPLINE_CURVE((1.,1.,1.,1.,1.,1.,1.,1.,1.,1.,1.,1.,1.,1.,1.,1.,
1.,1.,1.,1.,1.,1.,1.,1.,1.,1.,1.,1.,1.,1.,1.,1.,1.,1.,1.,1.,1.,1.,1.,1.,
1.,1.,1.,1.,1.,1.,1.,1.,1.,1.,1.,1.,1.,1.,1.,1.,1.,1.,1.,1.,1.,1.,1.,1.,
1.,1.,1.,1.,1.,1.,1.,1.,1.,1.,1.,1.,1.,1.,1.,1.,1.,1.,1.,1.,1.,1.,1.,1.,
1.,1.,1.,1.,1.,1.,1.,1.,1.,1.,1.,1.,1.,1.,1.,1.,1.,1.,1.,1.,1.,1.,1.,1.,
1.,1.,1.,1.,1.,1.,1.,1.,1.,1.,1.,1.,1.,1.,1.,1.,1.,1.,1.,1.,1.,1.,1.,1.,
1.,1.,1.,1.,1.,1.,1.,1.,1.,1.,1.,1.,1.,1.,1.,1.,1.,1.,1.,1.,1.,1.,1.,1.,
1.,1.,1.,1.,1.,1.,1.,1.,1.,1.,1.,1.,1.,1.,1.,1.,1.,1.,1.,1.,1.,1.,1.,1.,
1.,1.,1.,1.,1.,1.,1.,1.,1.,1.))
REPRESENTATION_ITEM('')
);
#562=(
BOUNDED_CURVE()
B_SPLINE_CURVE(5,(#123207,#123208,#123209,#123210,#123211,#123212,#123213,
#123214,#123215,#123216,#123217,#123218,#123219,#123220,#123221,#123222,
#123223,#123224,#123225,#123226,#123227,#123228,#123229,#123230,#123231,
#123232,#123233,#123234,#123235,#123236,#123237,#123238,#123239,#123240,
#123241,#123242,#123243,#123244,#123245,#123246,#123247,#123248,#123249,
#123250,#123251,#123252,#123253,#123254,#123255,#123256,#123257,#123258,
#123259,#123260,#123261,#123262,#123263,#123264,#123265,#123266,#123267,
#123268,#123269,#123270,#123271,#123272,#123273,#123274,#123275,#123276,
#123277,#123278,#123279,#123280,#123281,#123282,#123283,#123284,#123285,
#123286,#123287,#123288,#123289,#123290,#123291,#123292,#123293,#123294,
#123295,#123296,#123297,#123298,#123299,#123300,#123301,#123302,#123303,
#123304,#123305,#123306,#123307,#123308,#123309,#123310,#123311,#123312,
#123313,#123314,#123315,#123316,#123317,#123318,#123319,#123320,#123321,
#123322,#123323,#123324,#123325,#123326,#123327,#123328,#123329,#123330,
#123331,#123332,#123333,#123334,#123335,#123336,#123337,#123338,#123339,
#123340,#123341,#123342,#123343,#123344,#123345,#123346,#123347,#123348,
#123349,#123350,#123351,#123352,#123353,#123354,#123355,#123356,#123357,
#123358,#123359,#123360,#123361,#123362,#123363,#123364,#123365,#123366,
#123367,#123368,#123369,#123370,#123371,#123372,#123373,#123374,#123375,
#123376,#123377,#123378,#123379,#123380,#123381,#123382,#123383,#123384,
#123385,#123386,#123387,#123388,#123389,#123390,#123391,#123392,#123393,
#123394,#123395,#123396,#123397,#123398,#123399,#123400),.UNSPECIFIED.,
 .F.,.F.)
B_SPLINE_CURVE_WITH_KNOTS((6,1,1,1,1,1,1,1,1,1,1,1,1,1,1,1,1,1,1,1,1,1,
1,1,1,1,1,1,1,1,1,1,1,1,1,1,1,1,1,1,1,1,1,1,1,1,1,1,1,1,1,1,1,1,1,1,1,1,
1,1,1,1,1,1,1,1,1,1,1,1,1,1,1,1,1,1,1,1,1,1,1,1,1,1,1,1,1,1,1,1,1,1,1,1,
1,1,1,1,1,1,1,1,1,1,1,1,1,1,1,1,1,1,1,1,1,1,1,1,1,1,1,1,1,1,1,1,1,1,1,1,
1,1,1,1,1,1,1,1,1,1,1,1,1,1,1,1,1,1,1,1,1,1,1,1,1,1,1,1,1,1,1,1,1,1,1,1,
1,1,1,1,1,1,1,1,1,1,1,1,1,1,1,1,1,1,1,1,1,1,1,6),(-0.941429844438072,-0.940000000000001,
-0.935000000000001,-0.930000000000001,-0.925000000000001,-0.920000000000001,
-0.915000000000001,-0.910000000000001,-0.905000000000001,-0.900000000000001,
-0.895000000000001,-0.890000000000001,-0.885000000000001,-0.880000000000001,
-0.875000000000001,-0.870000000000001,-0.865000000000001,-0.860000000000001,
-0.855000000000001,-0.850000000000001,-0.845000000000001,-0.840000000000001,
-0.835000000000001,-0.830000000000001,-0.825000000000001,-0.820000000000001,
-0.815000000000001,-0.810000000000001,-0.805000000000001,-0.800000000000001,
-0.795000000000001,-0.790000000000001,-0.785000000000001,-0.780000000000001,
-0.775000000000001,-0.770000000000001,-0.765000000000001,-0.760000000000001,
-0.755000000000001,-0.750000000000001,-0.745000000000001,-0.740000000000001,
-0.735000000000001,-0.730000000000001,-0.725000000000001,-0.720000000000001,
-0.715000000000001,-0.710000000000001,-0.705000000000001,-0.700000000000001,
-0.695000000000001,-0.690000000000001,-0.685,-0.68,-0.675,-0.67,-0.665,
-0.66,-0.655,-0.65,-0.645,-0.64,-0.635,-0.63,-0.625,-0.62,-0.615,-0.61,
-0.605,-0.6,-0.595,-0.59,-0.585,-0.58,-0.575,-0.57,-0.565,-0.56,-0.555,
-0.55,-0.545,-0.54,-0.535,-0.53,-0.525,-0.52,-0.515,-0.51,-0.505,-0.5,-0.495,
-0.49,-0.485,-0.48,-0.475,-0.47,-0.465,-0.46,-0.455,-0.45,-0.445,-0.44,
-0.435,-0.43,-0.425,-0.42,-0.415,-0.41,-0.405,-0.4,-0.395,-0.39,-0.385,
-0.38,-0.375,-0.37,-0.365,-0.36,-0.355,-0.35,-0.345,-0.34,-0.335,-0.33,
-0.325,-0.32,-0.315,-0.31,-0.305,-0.3,-0.295,-0.29,-0.285,-0.28,-0.275,
-0.27,-0.265,-0.26,-0.255,-0.25,-0.245,-0.24,-0.235,-0.23,-0.225,-0.22,
-0.215,-0.21,-0.205,-0.2,-0.195,-0.19,-0.185,-0.18,-0.175,-0.17,-0.165,
-0.16,-0.155,-0.15,-0.145,-0.14,-0.135,-0.13,-0.125,-0.12,-0.115,-0.11,
-0.105,-0.1,-0.095,-0.09,-0.085,-0.08,-0.075,-0.07,-0.065,-0.06,-0.055,
-0.05,-0.045,-0.04,-0.035,-0.03,-0.025,-0.02,-0.015,-0.01,-0.005,0.),
 .UNSPECIFIED.)
CURVE()
GEOMETRIC_REPRESENTATION_ITEM()
RATIONAL_B_SPLINE_CURVE((1.,1.,1.,1.,1.,1.,1.,1.,1.,1.,1.,1.,1.,1.,1.,1.,
1.,1.,1.,1.,1.,1.,1.,1.,1.,1.,1.,1.,1.,1.,1.,1.,1.,1.,1.,1.,1.,1.,1.,1.,
1.,1.,1.,1.,1.,1.,1.,1.,1.,1.,1.,1.,1.,1.,1.,1.,1.,1.,1.,1.,1.,1.,1.,1.,
1.,1.,1.,1.,1.,1.,1.,1.,1.,1.,1.,1.,1.,1.,1.,1.,1.,1.,1.,1.,1.,1.,1.,1.,
1.,1.,1.,1.,1.,1.,1.,1.,1.,1.,1.,1.,1.,1.,1.,1.,1.,1.,1.,1.,1.,1.,1.,1.,
1.,1.,1.,1.,1.,1.,1.,1.,1.,1.,1.,1.,1.,1.,1.,1.,1.,1.,1.,1.,1.,1.,1.,1.,
1.,1.,1.,1.,1.,1.,1.,1.,1.,1.,1.,1.,1.,1.,1.,1.,1.,1.,1.,1.,1.,1.,1.,1.,
1.,1.,1.,1.,1.,1.,1.,1.,1.,1.,1.,1.,1.,1.,1.,1.,1.,1.,1.,1.,1.,1.,1.,1.,
1.,1.,1.,1.,1.,1.,1.,1.,1.,1.))
REPRESENTATION_ITEM('')
);
#563=(
BOUNDED_CURVE()
B_SPLINE_CURVE(5,(#123812,#123813,#123814,#123815,#123816,#123817,#123818,
#123819,#123820,#123821,#123822,#123823,#123824,#123825,#123826,#123827,
#123828,#123829,#123830,#123831,#123832,#123833,#123834,#123835,#123836,
#123837,#123838,#123839,#123840,#123841,#123842,#123843,#123844,#123845,
#123846,#123847,#123848,#123849,#123850,#123851,#123852,#123853,#123854,
#123855,#123856,#123857,#123858,#123859,#123860,#123861,#123862,#123863,
#123864,#123865,#123866,#123867,#123868,#123869,#123870,#123871,#123872,
#123873,#123874,#123875,#123876,#123877,#123878,#123879,#123880,#123881,
#123882,#123883,#123884,#123885,#123886,#123887,#123888,#123889,#123890,
#123891,#123892,#123893,#123894,#123895,#123896,#123897,#123898,#123899,
#123900,#123901,#123902,#123903,#123904,#123905,#123906,#123907,#123908,
#123909,#123910,#123911,#123912,#123913,#123914,#123915,#123916,#123917,
#123918,#123919,#123920,#123921,#123922,#123923,#123924,#123925,#123926,
#123927,#123928,#123929,#123930,#123931,#123932,#123933,#123934,#123935,
#123936,#123937,#123938,#123939,#123940,#123941,#123942,#123943,#123944,
#123945,#123946,#123947,#123948,#123949,#123950,#123951,#123952,#123953,
#123954,#123955,#123956,#123957,#123958,#123959,#123960,#123961,#123962,
#123963,#123964,#123965,#123966,#123967,#123968,#123969,#123970,#123971,
#123972,#123973,#123974,#123975,#123976,#123977,#123978,#123979,#123980,
#123981,#123982,#123983,#123984,#123985,#123986,#123987,#123988,#123989,
#123990,#123991,#123992,#123993,#123994,#123995,#123996,#123997,#123998,
#123999,#124000,#124001,#124002,#124003,#124004,#124005),.UNSPECIFIED.,
 .F.,.F.)
B_SPLINE_CURVE_WITH_KNOTS((6,1,1,1,1,1,1,1,1,1,1,1,1,1,1,1,1,1,1,1,1,1,
1,1,1,1,1,1,1,1,1,1,1,1,1,1,1,1,1,1,1,1,1,1,1,1,1,1,1,1,1,1,1,1,1,1,1,1,
1,1,1,1,1,1,1,1,1,1,1,1,1,1,1,1,1,1,1,1,1,1,1,1,1,1,1,1,1,1,1,1,1,1,1,1,
1,1,1,1,1,1,1,1,1,1,1,1,1,1,1,1,1,1,1,1,1,1,1,1,1,1,1,1,1,1,1,1,1,1,1,1,
1,1,1,1,1,1,1,1,1,1,1,1,1,1,1,1,1,1,1,1,1,1,1,1,1,1,1,1,1,1,1,1,1,1,1,1,
1,1,1,1,1,1,1,1,1,1,1,1,1,1,1,1,1,1,1,1,1,1,1,6),(0.,0.005,0.01,0.015,0.02,
0.025,0.03,0.035,0.04,0.045,0.05,0.055,0.06,0.065,0.07,0.075,0.08,0.085,
0.09,0.095,0.1,0.105,0.11,0.115,0.12,0.125,0.13,0.135,0.14,0.145,0.15,0.155,
0.16,0.165,0.17,0.175,0.18,0.185,0.19,0.195,0.2,0.205,0.21,0.215,0.22,0.225,
0.23,0.235,0.24,0.245,0.25,0.255,0.26,0.265,0.27,0.275,0.28,0.285,0.29,
0.295,0.3,0.305,0.31,0.315,0.32,0.325,0.33,0.335,0.34,0.345,0.35,0.355,
0.36,0.365,0.37,0.375,0.38,0.385,0.39,0.395,0.4,0.405,0.41,0.415,0.42,0.425,
0.43,0.435,0.44,0.445,0.45,0.455,0.46,0.465,0.47,0.475,0.48,0.485,0.49,
0.495,0.5,0.505,0.51,0.515,0.52,0.525,0.53,0.535,0.54,0.545,0.55,0.555,
0.56,0.565,0.57,0.575,0.58,0.585,0.59,0.595,0.6,0.605,0.61,0.615,0.62,0.625,
0.63,0.635,0.64,0.645,0.65,0.655,0.66,0.665,0.67,0.675,0.68,0.685,0.690000000000001,
0.695000000000001,0.700000000000001,0.705000000000001,0.710000000000001,
0.715000000000001,0.720000000000001,0.725000000000001,0.730000000000001,
0.735000000000001,0.740000000000001,0.745000000000001,0.750000000000001,
0.755000000000001,0.760000000000001,0.765000000000001,0.770000000000001,
0.775000000000001,0.780000000000001,0.785000000000001,0.790000000000001,
0.795000000000001,0.800000000000001,0.805000000000001,0.810000000000001,
0.815000000000001,0.820000000000001,0.825000000000001,0.830000000000001,
0.835000000000001,0.840000000000001,0.845000000000001,0.850000000000001,
0.855000000000001,0.860000000000001,0.865000000000001,0.870000000000001,
0.875000000000001,0.880000000000001,0.885000000000001,0.890000000000001,
0.895000000000001,0.900000000000001,0.905000000000001,0.910000000000001,
0.915000000000001,0.920000000000001,0.925000000000001,0.930000000000001,
0.935000000000001,0.940000000000001,0.941429844437997),.UNSPECIFIED.)
CURVE()
GEOMETRIC_REPRESENTATION_ITEM()
RATIONAL_B_SPLINE_CURVE((1.,1.,1.,1.,1.,1.,1.,1.,1.,1.,1.,1.,1.,1.,1.,1.,
1.,1.,1.,1.,1.,1.,1.,1.,1.,1.,1.,1.,1.,1.,1.,1.,1.,1.,1.,1.,1.,1.,1.,1.,
1.,1.,1.,1.,1.,1.,1.,1.,1.,1.,1.,1.,1.,1.,1.,1.,1.,1.,1.,1.,1.,1.,1.,1.,
1.,1.,1.,1.,1.,1.,1.,1.,1.,1.,1.,1.,1.,1.,1.,1.,1.,1.,1.,1.,1.,1.,1.,1.,
1.,1.,1.,1.,1.,1.,1.,1.,1.,1.,1.,1.,1.,1.,1.,1.,1.,1.,1.,1.,1.,1.,1.,1.,
1.,1.,1.,1.,1.,1.,1.,1.,1.,1.,1.,1.,1.,1.,1.,1.,1.,1.,1.,1.,1.,1.,1.,1.,
1.,1.,1.,1.,1.,1.,1.,1.,1.,1.,1.,1.,1.,1.,1.,1.,1.,1.,1.,1.,1.,1.,1.,1.,
1.,1.,1.,1.,1.,1.,1.,1.,1.,1.,1.,1.,1.,1.,1.,1.,1.,1.,1.,1.,1.,1.,1.,1.,
1.,1.,1.,1.,1.,1.,1.,1.,1.,1.))
REPRESENTATION_ITEM('')
);
#564=(
BOUNDED_CURVE()
B_SPLINE_CURVE(5,(#124008,#124009,#124010,#124011,#124012,#124013,#124014,
#124015,#124016,#124017,#124018,#124019,#124020,#124021,#124022,#124023,
#124024,#124025,#124026,#124027,#124028,#124029,#124030,#124031,#124032,
#124033,#124034,#124035,#124036,#124037,#124038,#124039,#124040,#124041,
#124042,#124043,#124044,#124045,#124046,#124047,#124048,#124049,#124050,
#124051,#124052,#124053,#124054,#124055,#124056,#124057,#124058,#124059,
#124060,#124061,#124062,#124063,#124064,#124065,#124066,#124067,#124068,
#124069,#124070,#124071,#124072,#124073,#124074,#124075,#124076,#124077,
#124078,#124079,#124080,#124081,#124082,#124083,#124084,#124085,#124086,
#124087,#124088,#124089,#124090,#124091,#124092,#124093,#124094,#124095,
#124096,#124097,#124098,#124099,#124100,#124101,#124102,#124103,#124104,
#124105,#124106,#124107,#124108,#124109,#124110,#124111,#124112,#124113,
#124114,#124115,#124116,#124117,#124118,#124119,#124120,#124121,#124122,
#124123,#124124,#124125,#124126,#124127,#124128,#124129,#124130,#124131,
#124132,#124133,#124134,#124135,#124136,#124137,#124138,#124139,#124140,
#124141,#124142,#124143,#124144,#124145,#124146,#124147,#124148,#124149,
#124150,#124151,#124152,#124153,#124154,#124155,#124156,#124157,#124158,
#124159,#124160,#124161,#124162,#124163,#124164,#124165,#124166,#124167,
#124168,#124169,#124170,#124171,#124172,#124173,#124174,#124175,#124176,
#124177,#124178,#124179,#124180,#124181,#124182,#124183,#124184,#124185,
#124186,#124187,#124188,#124189,#124190,#124191,#124192,#124193,#124194,
#124195,#124196,#124197,#124198,#124199,#124200,#124201),.UNSPECIFIED.,
 .F.,.F.)
B_SPLINE_CURVE_WITH_KNOTS((6,1,1,1,1,1,1,1,1,1,1,1,1,1,1,1,1,1,1,1,1,1,
1,1,1,1,1,1,1,1,1,1,1,1,1,1,1,1,1,1,1,1,1,1,1,1,1,1,1,1,1,1,1,1,1,1,1,1,
1,1,1,1,1,1,1,1,1,1,1,1,1,1,1,1,1,1,1,1,1,1,1,1,1,1,1,1,1,1,1,1,1,1,1,1,
1,1,1,1,1,1,1,1,1,1,1,1,1,1,1,1,1,1,1,1,1,1,1,1,1,1,1,1,1,1,1,1,1,1,1,1,
1,1,1,1,1,1,1,1,1,1,1,1,1,1,1,1,1,1,1,1,1,1,1,1,1,1,1,1,1,1,1,1,1,1,1,1,
1,1,1,1,1,1,1,1,1,1,1,1,1,1,1,1,1,1,1,1,1,1,1,6),(-0.941429844437994,-0.940000000000001,
-0.935000000000001,-0.930000000000001,-0.925000000000001,-0.920000000000001,
-0.915000000000001,-0.910000000000001,-0.905000000000001,-0.900000000000001,
-0.895000000000001,-0.890000000000001,-0.885000000000001,-0.880000000000001,
-0.875000000000001,-0.870000000000001,-0.865000000000001,-0.860000000000001,
-0.855000000000001,-0.850000000000001,-0.845000000000001,-0.840000000000001,
-0.835000000000001,-0.830000000000001,-0.825000000000001,-0.820000000000001,
-0.815000000000001,-0.810000000000001,-0.805000000000001,-0.800000000000001,
-0.795000000000001,-0.790000000000001,-0.785000000000001,-0.780000000000001,
-0.775000000000001,-0.770000000000001,-0.765000000000001,-0.760000000000001,
-0.755000000000001,-0.750000000000001,-0.745000000000001,-0.740000000000001,
-0.735000000000001,-0.730000000000001,-0.725000000000001,-0.720000000000001,
-0.715000000000001,-0.710000000000001,-0.705000000000001,-0.700000000000001,
-0.695000000000001,-0.690000000000001,-0.685,-0.68,-0.675,-0.67,-0.665,
-0.66,-0.655,-0.65,-0.645,-0.64,-0.635,-0.63,-0.625,-0.62,-0.615,-0.61,
-0.605,-0.6,-0.595,-0.59,-0.585,-0.58,-0.575,-0.57,-0.565,-0.56,-0.555,
-0.55,-0.545,-0.54,-0.535,-0.53,-0.525,-0.52,-0.515,-0.51,-0.505,-0.5,-0.495,
-0.49,-0.485,-0.48,-0.475,-0.47,-0.465,-0.46,-0.455,-0.45,-0.445,-0.44,
-0.435,-0.43,-0.425,-0.42,-0.415,-0.41,-0.405,-0.4,-0.395,-0.39,-0.385,
-0.38,-0.375,-0.37,-0.365,-0.36,-0.355,-0.35,-0.345,-0.34,-0.335,-0.33,
-0.325,-0.32,-0.315,-0.31,-0.305,-0.3,-0.295,-0.29,-0.285,-0.28,-0.275,
-0.27,-0.265,-0.26,-0.255,-0.25,-0.245,-0.24,-0.235,-0.23,-0.225,-0.22,
-0.215,-0.21,-0.205,-0.2,-0.195,-0.19,-0.185,-0.18,-0.175,-0.17,-0.165,
-0.16,-0.155,-0.15,-0.145,-0.14,-0.135,-0.13,-0.125,-0.12,-0.115,-0.11,
-0.105,-0.1,-0.095,-0.09,-0.085,-0.08,-0.075,-0.07,-0.065,-0.06,-0.055,
-0.05,-0.045,-0.04,-0.035,-0.03,-0.025,-0.02,-0.015,-0.01,-0.005,0.),
 .UNSPECIFIED.)
CURVE()
GEOMETRIC_REPRESENTATION_ITEM()
RATIONAL_B_SPLINE_CURVE((1.,1.,1.,1.,1.,1.,1.,1.,1.,1.,1.,1.,1.,1.,1.,1.,
1.,1.,1.,1.,1.,1.,1.,1.,1.,1.,1.,1.,1.,1.,1.,1.,1.,1.,1.,1.,1.,1.,1.,1.,
1.,1.,1.,1.,1.,1.,1.,1.,1.,1.,1.,1.,1.,1.,1.,1.,1.,1.,1.,1.,1.,1.,1.,1.,
1.,1.,1.,1.,1.,1.,1.,1.,1.,1.,1.,1.,1.,1.,1.,1.,1.,1.,1.,1.,1.,1.,1.,1.,
1.,1.,1.,1.,1.,1.,1.,1.,1.,1.,1.,1.,1.,1.,1.,1.,1.,1.,1.,1.,1.,1.,1.,1.,
1.,1.,1.,1.,1.,1.,1.,1.,1.,1.,1.,1.,1.,1.,1.,1.,1.,1.,1.,1.,1.,1.,1.,1.,
1.,1.,1.,1.,1.,1.,1.,1.,1.,1.,1.,1.,1.,1.,1.,1.,1.,1.,1.,1.,1.,1.,1.,1.,
1.,1.,1.,1.,1.,1.,1.,1.,1.,1.,1.,1.,1.,1.,1.,1.,1.,1.,1.,1.,1.,1.,1.,1.,
1.,1.,1.,1.,1.,1.,1.,1.,1.,1.))
REPRESENTATION_ITEM('')
);
#565=(
BOUNDED_CURVE()
B_SPLINE_CURVE(5,(#124613,#124614,#124615,#124616,#124617,#124618,#124619,
#124620,#124621,#124622,#124623,#124624,#124625,#124626,#124627,#124628,
#124629,#124630,#124631,#124632,#124633,#124634,#124635,#124636,#124637,
#124638,#124639,#124640,#124641,#124642,#124643,#124644,#124645,#124646,
#124647,#124648,#124649,#124650,#124651,#124652,#124653,#124654,#124655,
#124656,#124657,#124658,#124659,#124660,#124661,#124662,#124663,#124664,
#124665,#124666,#124667,#124668,#124669,#124670,#124671,#124672,#124673,
#124674,#124675,#124676,#124677,#124678,#124679,#124680,#124681,#124682,
#124683,#124684,#124685,#124686,#124687,#124688,#124689,#124690,#124691,
#124692,#124693,#124694,#124695,#124696,#124697,#124698,#124699,#124700,
#124701,#124702,#124703,#124704,#124705,#124706,#124707,#124708,#124709,
#124710,#124711,#124712,#124713,#124714,#124715,#124716,#124717,#124718,
#124719,#124720,#124721,#124722,#124723,#124724,#124725,#124726,#124727,
#124728,#124729,#124730,#124731,#124732,#124733,#124734,#124735,#124736,
#124737,#124738,#124739,#124740,#124741,#124742,#124743,#124744,#124745,
#124746,#124747,#124748,#124749,#124750,#124751,#124752,#124753,#124754,
#124755,#124756,#124757,#124758,#124759,#124760,#124761,#124762,#124763,
#124764,#124765,#124766,#124767,#124768,#124769,#124770,#124771,#124772,
#124773,#124774,#124775,#124776,#124777,#124778,#124779,#124780,#124781,
#124782,#124783,#124784,#124785,#124786,#124787,#124788,#124789,#124790,
#124791,#124792,#124793,#124794,#124795,#124796,#124797,#124798,#124799,
#124800,#124801,#124802,#124803,#124804,#124805,#124806),.UNSPECIFIED.,
 .F.,.F.)
B_SPLINE_CURVE_WITH_KNOTS((6,1,1,1,1,1,1,1,1,1,1,1,1,1,1,1,1,1,1,1,1,1,
1,1,1,1,1,1,1,1,1,1,1,1,1,1,1,1,1,1,1,1,1,1,1,1,1,1,1,1,1,1,1,1,1,1,1,1,
1,1,1,1,1,1,1,1,1,1,1,1,1,1,1,1,1,1,1,1,1,1,1,1,1,1,1,1,1,1,1,1,1,1,1,1,
1,1,1,1,1,1,1,1,1,1,1,1,1,1,1,1,1,1,1,1,1,1,1,1,1,1,1,1,1,1,1,1,1,1,1,1,
1,1,1,1,1,1,1,1,1,1,1,1,1,1,1,1,1,1,1,1,1,1,1,1,1,1,1,1,1,1,1,1,1,1,1,1,
1,1,1,1,1,1,1,1,1,1,1,1,1,1,1,1,1,1,1,1,1,1,1,6),(0.,0.005,0.01,0.015,0.02,
0.025,0.03,0.035,0.04,0.045,0.05,0.055,0.06,0.065,0.07,0.075,0.08,0.085,
0.09,0.095,0.1,0.105,0.11,0.115,0.12,0.125,0.13,0.135,0.14,0.145,0.15,0.155,
0.16,0.165,0.17,0.175,0.18,0.185,0.19,0.195,0.2,0.205,0.21,0.215,0.22,0.225,
0.23,0.235,0.24,0.245,0.25,0.255,0.26,0.265,0.27,0.275,0.28,0.285,0.29,
0.295,0.3,0.305,0.31,0.315,0.32,0.325,0.33,0.335,0.34,0.345,0.35,0.355,
0.36,0.365,0.37,0.375,0.38,0.385,0.39,0.395,0.4,0.405,0.41,0.415,0.42,0.425,
0.43,0.435,0.44,0.445,0.45,0.455,0.46,0.465,0.47,0.475,0.48,0.485,0.49,
0.495,0.5,0.505,0.51,0.515,0.52,0.525,0.53,0.535,0.54,0.545,0.55,0.555,
0.56,0.565,0.57,0.575,0.58,0.585,0.59,0.595,0.6,0.605,0.61,0.615,0.62,0.625,
0.63,0.635,0.64,0.645,0.65,0.655,0.66,0.665,0.67,0.675,0.68,0.685,0.690000000000001,
0.695000000000001,0.700000000000001,0.705000000000001,0.710000000000001,
0.715000000000001,0.720000000000001,0.725000000000001,0.730000000000001,
0.735000000000001,0.740000000000001,0.745000000000001,0.750000000000001,
0.755000000000001,0.760000000000001,0.765000000000001,0.770000000000001,
0.775000000000001,0.780000000000001,0.785000000000001,0.790000000000001,
0.795000000000001,0.800000000000001,0.805000000000001,0.810000000000001,
0.815000000000001,0.820000000000001,0.825000000000001,0.830000000000001,
0.835000000000001,0.840000000000001,0.845000000000001,0.850000000000001,
0.855000000000001,0.860000000000001,0.865000000000001,0.870000000000001,
0.875000000000001,0.880000000000001,0.885000000000001,0.890000000000001,
0.895000000000001,0.900000000000001,0.905000000000001,0.910000000000001,
0.915000000000001,0.920000000000001,0.925000000000001,0.930000000000001,
0.935000000000001,0.940000000000001,0.941429844438079),.UNSPECIFIED.)
CURVE()
GEOMETRIC_REPRESENTATION_ITEM()
RATIONAL_B_SPLINE_CURVE((1.,1.,1.,1.,1.,1.,1.,1.,1.,1.,1.,1.,1.,1.,1.,1.,
1.,1.,1.,1.,1.,1.,1.,1.,1.,1.,1.,1.,1.,1.,1.,1.,1.,1.,1.,1.,1.,1.,1.,1.,
1.,1.,1.,1.,1.,1.,1.,1.,1.,1.,1.,1.,1.,1.,1.,1.,1.,1.,1.,1.,1.,1.,1.,1.,
1.,1.,1.,1.,1.,1.,1.,1.,1.,1.,1.,1.,1.,1.,1.,1.,1.,1.,1.,1.,1.,1.,1.,1.,
1.,1.,1.,1.,1.,1.,1.,1.,1.,1.,1.,1.,1.,1.,1.,1.,1.,1.,1.,1.,1.,1.,1.,1.,
1.,1.,1.,1.,1.,1.,1.,1.,1.,1.,1.,1.,1.,1.,1.,1.,1.,1.,1.,1.,1.,1.,1.,1.,
1.,1.,1.,1.,1.,1.,1.,1.,1.,1.,1.,1.,1.,1.,1.,1.,1.,1.,1.,1.,1.,1.,1.,1.,
1.,1.,1.,1.,1.,1.,1.,1.,1.,1.,1.,1.,1.,1.,1.,1.,1.,1.,1.,1.,1.,1.,1.,1.,
1.,1.,1.,1.,1.,1.,1.,1.,1.,1.))
REPRESENTATION_ITEM('')
);
#566=(
BOUNDED_CURVE()
B_SPLINE_CURVE(5,(#124809,#124810,#124811,#124812,#124813,#124814,#124815,
#124816,#124817,#124818,#124819,#124820,#124821,#124822,#124823,#124824,
#124825,#124826,#124827,#124828,#124829,#124830,#124831,#124832,#124833,
#124834,#124835,#124836,#124837,#124838,#124839,#124840,#124841,#124842,
#124843,#124844,#124845,#124846,#124847,#124848,#124849,#124850,#124851,
#124852,#124853,#124854,#124855,#124856,#124857,#124858,#124859,#124860,
#124861,#124862,#124863,#124864,#124865,#124866,#124867,#124868,#124869,
#124870,#124871,#124872,#124873,#124874,#124875,#124876,#124877,#124878,
#124879,#124880,#124881,#124882,#124883,#124884,#124885,#124886,#124887,
#124888,#124889,#124890,#124891,#124892,#124893,#124894,#124895,#124896,
#124897,#124898,#124899,#124900,#124901,#124902,#124903,#124904,#124905,
#124906,#124907,#124908,#124909,#124910,#124911,#124912,#124913,#124914,
#124915,#124916,#124917,#124918,#124919,#124920,#124921,#124922,#124923,
#124924,#124925,#124926,#124927,#124928,#124929,#124930,#124931,#124932,
#124933,#124934,#124935,#124936,#124937,#124938,#124939,#124940,#124941,
#124942,#124943,#124944,#124945,#124946,#124947,#124948,#124949,#124950,
#124951,#124952,#124953,#124954,#124955,#124956,#124957,#124958,#124959,
#124960,#124961,#124962,#124963,#124964,#124965,#124966,#124967,#124968,
#124969,#124970,#124971,#124972,#124973,#124974,#124975,#124976,#124977,
#124978,#124979,#124980,#124981,#124982,#124983,#124984,#124985,#124986,
#124987,#124988,#124989,#124990,#124991,#124992,#124993,#124994,#124995,
#124996,#124997,#124998,#124999,#125000,#125001,#125002),.UNSPECIFIED.,
 .F.,.F.)
B_SPLINE_CURVE_WITH_KNOTS((6,1,1,1,1,1,1,1,1,1,1,1,1,1,1,1,1,1,1,1,1,1,
1,1,1,1,1,1,1,1,1,1,1,1,1,1,1,1,1,1,1,1,1,1,1,1,1,1,1,1,1,1,1,1,1,1,1,1,
1,1,1,1,1,1,1,1,1,1,1,1,1,1,1,1,1,1,1,1,1,1,1,1,1,1,1,1,1,1,1,1,1,1,1,1,
1,1,1,1,1,1,1,1,1,1,1,1,1,1,1,1,1,1,1,1,1,1,1,1,1,1,1,1,1,1,1,1,1,1,1,1,
1,1,1,1,1,1,1,1,1,1,1,1,1,1,1,1,1,1,1,1,1,1,1,1,1,1,1,1,1,1,1,1,1,1,1,1,
1,1,1,1,1,1,1,1,1,1,1,1,1,1,1,1,1,1,1,1,1,1,1,6),(-0.941429844438079,-0.940000000000001,
-0.935000000000001,-0.930000000000001,-0.925000000000001,-0.920000000000001,
-0.915000000000001,-0.910000000000001,-0.905000000000001,-0.900000000000001,
-0.895000000000001,-0.890000000000001,-0.885000000000001,-0.880000000000001,
-0.875000000000001,-0.870000000000001,-0.865000000000001,-0.860000000000001,
-0.855000000000001,-0.850000000000001,-0.845000000000001,-0.840000000000001,
-0.835000000000001,-0.830000000000001,-0.825000000000001,-0.820000000000001,
-0.815000000000001,-0.810000000000001,-0.805000000000001,-0.800000000000001,
-0.795000000000001,-0.790000000000001,-0.785000000000001,-0.780000000000001,
-0.775000000000001,-0.770000000000001,-0.765000000000001,-0.760000000000001,
-0.755000000000001,-0.750000000000001,-0.745000000000001,-0.740000000000001,
-0.735000000000001,-0.730000000000001,-0.725000000000001,-0.720000000000001,
-0.715000000000001,-0.710000000000001,-0.705000000000001,-0.700000000000001,
-0.695000000000001,-0.690000000000001,-0.685,-0.68,-0.675,-0.67,-0.665,
-0.66,-0.655,-0.65,-0.645,-0.64,-0.635,-0.63,-0.625,-0.62,-0.615,-0.61,
-0.605,-0.6,-0.595,-0.59,-0.585,-0.58,-0.575,-0.57,-0.565,-0.56,-0.555,
-0.55,-0.545,-0.54,-0.535,-0.53,-0.525,-0.52,-0.515,-0.51,-0.505,-0.5,-0.495,
-0.49,-0.485,-0.48,-0.475,-0.47,-0.465,-0.46,-0.455,-0.45,-0.445,-0.44,
-0.435,-0.43,-0.425,-0.42,-0.415,-0.41,-0.405,-0.4,-0.395,-0.39,-0.385,
-0.38,-0.375,-0.37,-0.365,-0.36,-0.355,-0.35,-0.345,-0.34,-0.335,-0.33,
-0.325,-0.32,-0.315,-0.31,-0.305,-0.3,-0.295,-0.29,-0.285,-0.28,-0.275,
-0.27,-0.265,-0.26,-0.255,-0.25,-0.245,-0.24,-0.235,-0.23,-0.225,-0.22,
-0.215,-0.21,-0.205,-0.2,-0.195,-0.19,-0.185,-0.18,-0.175,-0.17,-0.165,
-0.16,-0.155,-0.15,-0.145,-0.14,-0.135,-0.13,-0.125,-0.12,-0.115,-0.11,
-0.105,-0.1,-0.095,-0.09,-0.085,-0.08,-0.075,-0.07,-0.065,-0.06,-0.055,
-0.05,-0.045,-0.04,-0.035,-0.03,-0.025,-0.02,-0.015,-0.01,-0.005,0.),
 .UNSPECIFIED.)
CURVE()
GEOMETRIC_REPRESENTATION_ITEM()
RATIONAL_B_SPLINE_CURVE((1.,1.,1.,1.,1.,1.,1.,1.,1.,1.,1.,1.,1.,1.,1.,1.,
1.,1.,1.,1.,1.,1.,1.,1.,1.,1.,1.,1.,1.,1.,1.,1.,1.,1.,1.,1.,1.,1.,1.,1.,
1.,1.,1.,1.,1.,1.,1.,1.,1.,1.,1.,1.,1.,1.,1.,1.,1.,1.,1.,1.,1.,1.,1.,1.,
1.,1.,1.,1.,1.,1.,1.,1.,1.,1.,1.,1.,1.,1.,1.,1.,1.,1.,1.,1.,1.,1.,1.,1.,
1.,1.,1.,1.,1.,1.,1.,1.,1.,1.,1.,1.,1.,1.,1.,1.,1.,1.,1.,1.,1.,1.,1.,1.,
1.,1.,1.,1.,1.,1.,1.,1.,1.,1.,1.,1.,1.,1.,1.,1.,1.,1.,1.,1.,1.,1.,1.,1.,
1.,1.,1.,1.,1.,1.,1.,1.,1.,1.,1.,1.,1.,1.,1.,1.,1.,1.,1.,1.,1.,1.,1.,1.,
1.,1.,1.,1.,1.,1.,1.,1.,1.,1.,1.,1.,1.,1.,1.,1.,1.,1.,1.,1.,1.,1.,1.,1.,
1.,1.,1.,1.,1.,1.,1.,1.,1.,1.))
REPRESENTATION_ITEM('')
);
#567=(
BOUNDED_CURVE()
B_SPLINE_CURVE(5,(#125414,#125415,#125416,#125417,#125418,#125419,#125420,
#125421,#125422,#125423,#125424,#125425,#125426,#125427,#125428,#125429,
#125430,#125431,#125432,#125433,#125434,#125435,#125436,#125437,#125438,
#125439,#125440,#125441,#125442,#125443,#125444,#125445,#125446,#125447,
#125448,#125449,#125450,#125451,#125452,#125453,#125454,#125455,#125456,
#125457,#125458,#125459,#125460,#125461,#125462,#125463,#125464,#125465,
#125466,#125467,#125468,#125469,#125470,#125471,#125472,#125473,#125474,
#125475,#125476,#125477,#125478,#125479,#125480,#125481,#125482,#125483,
#125484,#125485,#125486,#125487,#125488,#125489,#125490,#125491,#125492,
#125493,#125494,#125495,#125496,#125497,#125498,#125499,#125500,#125501,
#125502,#125503,#125504,#125505,#125506,#125507,#125508,#125509,#125510,
#125511,#125512,#125513,#125514,#125515,#125516,#125517,#125518,#125519,
#125520,#125521,#125522,#125523,#125524,#125525,#125526,#125527,#125528,
#125529,#125530,#125531,#125532,#125533,#125534,#125535,#125536,#125537,
#125538,#125539,#125540,#125541,#125542,#125543,#125544,#125545,#125546,
#125547,#125548,#125549,#125550,#125551,#125552,#125553,#125554,#125555,
#125556,#125557,#125558,#125559,#125560,#125561,#125562,#125563,#125564,
#125565,#125566,#125567,#125568,#125569,#125570,#125571,#125572,#125573,
#125574,#125575,#125576,#125577,#125578,#125579,#125580,#125581,#125582,
#125583,#125584,#125585,#125586,#125587,#125588,#125589,#125590,#125591,
#125592,#125593,#125594,#125595,#125596,#125597,#125598,#125599,#125600,
#125601,#125602,#125603,#125604,#125605,#125606,#125607),.UNSPECIFIED.,
 .F.,.F.)
B_SPLINE_CURVE_WITH_KNOTS((6,1,1,1,1,1,1,1,1,1,1,1,1,1,1,1,1,1,1,1,1,1,
1,1,1,1,1,1,1,1,1,1,1,1,1,1,1,1,1,1,1,1,1,1,1,1,1,1,1,1,1,1,1,1,1,1,1,1,
1,1,1,1,1,1,1,1,1,1,1,1,1,1,1,1,1,1,1,1,1,1,1,1,1,1,1,1,1,1,1,1,1,1,1,1,
1,1,1,1,1,1,1,1,1,1,1,1,1,1,1,1,1,1,1,1,1,1,1,1,1,1,1,1,1,1,1,1,1,1,1,1,
1,1,1,1,1,1,1,1,1,1,1,1,1,1,1,1,1,1,1,1,1,1,1,1,1,1,1,1,1,1,1,1,1,1,1,1,
1,1,1,1,1,1,1,1,1,1,1,1,1,1,1,1,1,1,1,1,1,1,1,6),(0.,0.005,0.01,0.015,0.02,
0.025,0.03,0.035,0.04,0.045,0.05,0.055,0.06,0.065,0.07,0.075,0.08,0.085,
0.09,0.095,0.1,0.105,0.11,0.115,0.12,0.125,0.13,0.135,0.14,0.145,0.15,0.155,
0.16,0.165,0.17,0.175,0.18,0.185,0.19,0.195,0.2,0.205,0.21,0.215,0.22,0.225,
0.23,0.235,0.24,0.245,0.25,0.255,0.26,0.265,0.27,0.275,0.28,0.285,0.29,
0.295,0.3,0.305,0.31,0.315,0.32,0.325,0.33,0.335,0.34,0.345,0.35,0.355,
0.36,0.365,0.37,0.375,0.38,0.385,0.39,0.395,0.4,0.405,0.41,0.415,0.42,0.425,
0.43,0.435,0.44,0.445,0.45,0.455,0.46,0.465,0.47,0.475,0.48,0.485,0.49,
0.495,0.5,0.505,0.51,0.515,0.52,0.525,0.53,0.535,0.54,0.545,0.55,0.555,
0.56,0.565,0.57,0.575,0.58,0.585,0.59,0.595,0.6,0.605,0.61,0.615,0.62,0.625,
0.63,0.635,0.64,0.645,0.65,0.655,0.66,0.665,0.67,0.675,0.68,0.685,0.690000000000001,
0.695000000000001,0.700000000000001,0.705000000000001,0.710000000000001,
0.715000000000001,0.720000000000001,0.725000000000001,0.730000000000001,
0.735000000000001,0.740000000000001,0.745000000000001,0.750000000000001,
0.755000000000001,0.760000000000001,0.765000000000001,0.770000000000001,
0.775000000000001,0.780000000000001,0.785000000000001,0.790000000000001,
0.795000000000001,0.800000000000001,0.805000000000001,0.810000000000001,
0.815000000000001,0.820000000000001,0.825000000000001,0.830000000000001,
0.835000000000001,0.840000000000001,0.845000000000001,0.850000000000001,
0.855000000000001,0.860000000000001,0.865000000000001,0.870000000000001,
0.875000000000001,0.880000000000001,0.885000000000001,0.890000000000001,
0.895000000000001,0.900000000000001,0.905000000000001,0.910000000000001,
0.915000000000001,0.920000000000001,0.925000000000001,0.930000000000001,
0.935000000000001,0.940000000000001,0.941429844438073),.UNSPECIFIED.)
CURVE()
GEOMETRIC_REPRESENTATION_ITEM()
RATIONAL_B_SPLINE_CURVE((1.,1.,1.,1.,1.,1.,1.,1.,1.,1.,1.,1.,1.,1.,1.,1.,
1.,1.,1.,1.,1.,1.,1.,1.,1.,1.,1.,1.,1.,1.,1.,1.,1.,1.,1.,1.,1.,1.,1.,1.,
1.,1.,1.,1.,1.,1.,1.,1.,1.,1.,1.,1.,1.,1.,1.,1.,1.,1.,1.,1.,1.,1.,1.,1.,
1.,1.,1.,1.,1.,1.,1.,1.,1.,1.,1.,1.,1.,1.,1.,1.,1.,1.,1.,1.,1.,1.,1.,1.,
1.,1.,1.,1.,1.,1.,1.,1.,1.,1.,1.,1.,1.,1.,1.,1.,1.,1.,1.,1.,1.,1.,1.,1.,
1.,1.,1.,1.,1.,1.,1.,1.,1.,1.,1.,1.,1.,1.,1.,1.,1.,1.,1.,1.,1.,1.,1.,1.,
1.,1.,1.,1.,1.,1.,1.,1.,1.,1.,1.,1.,1.,1.,1.,1.,1.,1.,1.,1.,1.,1.,1.,1.,
1.,1.,1.,1.,1.,1.,1.,1.,1.,1.,1.,1.,1.,1.,1.,1.,1.,1.,1.,1.,1.,1.,1.,1.,
1.,1.,1.,1.,1.,1.,1.,1.,1.,1.))
REPRESENTATION_ITEM('')
);
#568=(
BOUNDED_CURVE()
B_SPLINE_CURVE(5,(#125610,#125611,#125612,#125613,#125614,#125615,#125616,
#125617,#125618,#125619,#125620,#125621,#125622,#125623,#125624,#125625,
#125626,#125627,#125628,#125629,#125630,#125631,#125632,#125633,#125634,
#125635,#125636,#125637,#125638,#125639,#125640,#125641,#125642,#125643,
#125644,#125645,#125646,#125647,#125648,#125649,#125650,#125651,#125652,
#125653,#125654,#125655,#125656,#125657,#125658,#125659,#125660,#125661,
#125662,#125663,#125664,#125665,#125666,#125667,#125668,#125669,#125670,
#125671,#125672,#125673,#125674,#125675,#125676,#125677,#125678,#125679,
#125680,#125681,#125682,#125683,#125684,#125685,#125686,#125687,#125688,
#125689,#125690,#125691,#125692,#125693,#125694,#125695,#125696,#125697,
#125698,#125699,#125700,#125701,#125702,#125703,#125704,#125705,#125706,
#125707,#125708,#125709,#125710,#125711,#125712,#125713,#125714,#125715,
#125716,#125717,#125718,#125719,#125720,#125721,#125722,#125723,#125724,
#125725,#125726,#125727,#125728,#125729,#125730,#125731,#125732,#125733,
#125734,#125735,#125736,#125737,#125738,#125739,#125740,#125741,#125742,
#125743,#125744,#125745,#125746,#125747,#125748,#125749,#125750,#125751,
#125752,#125753,#125754,#125755,#125756,#125757,#125758,#125759,#125760,
#125761,#125762,#125763,#125764,#125765,#125766,#125767,#125768,#125769,
#125770,#125771,#125772,#125773,#125774,#125775,#125776,#125777,#125778,
#125779,#125780,#125781,#125782,#125783,#125784,#125785,#125786,#125787,
#125788,#125789,#125790,#125791,#125792,#125793,#125794,#125795,#125796,
#125797,#125798,#125799,#125800,#125801,#125802,#125803),.UNSPECIFIED.,
 .F.,.F.)
B_SPLINE_CURVE_WITH_KNOTS((6,1,1,1,1,1,1,1,1,1,1,1,1,1,1,1,1,1,1,1,1,1,
1,1,1,1,1,1,1,1,1,1,1,1,1,1,1,1,1,1,1,1,1,1,1,1,1,1,1,1,1,1,1,1,1,1,1,1,
1,1,1,1,1,1,1,1,1,1,1,1,1,1,1,1,1,1,1,1,1,1,1,1,1,1,1,1,1,1,1,1,1,1,1,1,
1,1,1,1,1,1,1,1,1,1,1,1,1,1,1,1,1,1,1,1,1,1,1,1,1,1,1,1,1,1,1,1,1,1,1,1,
1,1,1,1,1,1,1,1,1,1,1,1,1,1,1,1,1,1,1,1,1,1,1,1,1,1,1,1,1,1,1,1,1,1,1,1,
1,1,1,1,1,1,1,1,1,1,1,1,1,1,1,1,1,1,1,1,1,1,1,6),(-0.941429844438069,-0.940000000000001,
-0.935000000000001,-0.930000000000001,-0.925000000000001,-0.920000000000001,
-0.915000000000001,-0.910000000000001,-0.905000000000001,-0.900000000000001,
-0.895000000000001,-0.890000000000001,-0.885000000000001,-0.880000000000001,
-0.875000000000001,-0.870000000000001,-0.865000000000001,-0.860000000000001,
-0.855000000000001,-0.850000000000001,-0.845000000000001,-0.840000000000001,
-0.835000000000001,-0.830000000000001,-0.825000000000001,-0.820000000000001,
-0.815000000000001,-0.810000000000001,-0.805000000000001,-0.800000000000001,
-0.795000000000001,-0.790000000000001,-0.785000000000001,-0.780000000000001,
-0.775000000000001,-0.770000000000001,-0.765000000000001,-0.760000000000001,
-0.755000000000001,-0.750000000000001,-0.745000000000001,-0.740000000000001,
-0.735000000000001,-0.730000000000001,-0.725000000000001,-0.720000000000001,
-0.715000000000001,-0.710000000000001,-0.705000000000001,-0.700000000000001,
-0.695000000000001,-0.690000000000001,-0.685,-0.68,-0.675,-0.67,-0.665,
-0.66,-0.655,-0.65,-0.645,-0.64,-0.635,-0.63,-0.625,-0.62,-0.615,-0.61,
-0.605,-0.6,-0.595,-0.59,-0.585,-0.58,-0.575,-0.57,-0.565,-0.56,-0.555,
-0.55,-0.545,-0.54,-0.535,-0.53,-0.525,-0.52,-0.515,-0.51,-0.505,-0.5,-0.495,
-0.49,-0.485,-0.48,-0.475,-0.47,-0.465,-0.46,-0.455,-0.45,-0.445,-0.44,
-0.435,-0.43,-0.425,-0.42,-0.415,-0.41,-0.405,-0.4,-0.395,-0.39,-0.385,
-0.38,-0.375,-0.37,-0.365,-0.36,-0.355,-0.35,-0.345,-0.34,-0.335,-0.33,
-0.325,-0.32,-0.315,-0.31,-0.305,-0.3,-0.295,-0.29,-0.285,-0.28,-0.275,
-0.27,-0.265,-0.26,-0.255,-0.25,-0.245,-0.24,-0.235,-0.23,-0.225,-0.22,
-0.215,-0.21,-0.205,-0.2,-0.195,-0.19,-0.185,-0.18,-0.175,-0.17,-0.165,
-0.16,-0.155,-0.15,-0.145,-0.14,-0.135,-0.13,-0.125,-0.12,-0.115,-0.11,
-0.105,-0.1,-0.095,-0.09,-0.085,-0.08,-0.075,-0.07,-0.065,-0.06,-0.055,
-0.05,-0.045,-0.04,-0.035,-0.03,-0.025,-0.02,-0.015,-0.01,-0.005,0.),
 .UNSPECIFIED.)
CURVE()
GEOMETRIC_REPRESENTATION_ITEM()
RATIONAL_B_SPLINE_CURVE((1.,1.,1.,1.,1.,1.,1.,1.,1.,1.,1.,1.,1.,1.,1.,1.,
1.,1.,1.,1.,1.,1.,1.,1.,1.,1.,1.,1.,1.,1.,1.,1.,1.,1.,1.,1.,1.,1.,1.,1.,
1.,1.,1.,1.,1.,1.,1.,1.,1.,1.,1.,1.,1.,1.,1.,1.,1.,1.,1.,1.,1.,1.,1.,1.,
1.,1.,1.,1.,1.,1.,1.,1.,1.,1.,1.,1.,1.,1.,1.,1.,1.,1.,1.,1.,1.,1.,1.,1.,
1.,1.,1.,1.,1.,1.,1.,1.,1.,1.,1.,1.,1.,1.,1.,1.,1.,1.,1.,1.,1.,1.,1.,1.,
1.,1.,1.,1.,1.,1.,1.,1.,1.,1.,1.,1.,1.,1.,1.,1.,1.,1.,1.,1.,1.,1.,1.,1.,
1.,1.,1.,1.,1.,1.,1.,1.,1.,1.,1.,1.,1.,1.,1.,1.,1.,1.,1.,1.,1.,1.,1.,1.,
1.,1.,1.,1.,1.,1.,1.,1.,1.,1.,1.,1.,1.,1.,1.,1.,1.,1.,1.,1.,1.,1.,1.,1.,
1.,1.,1.,1.,1.,1.,1.,1.,1.,1.))
REPRESENTATION_ITEM('')
);
#569=(
BOUNDED_CURVE()
B_SPLINE_CURVE(5,(#126215,#126216,#126217,#126218,#126219,#126220,#126221,
#126222,#126223,#126224,#126225,#126226,#126227,#126228,#126229,#126230,
#126231,#126232,#126233,#126234,#126235,#126236,#126237,#126238,#126239,
#126240,#126241,#126242,#126243,#126244,#126245,#126246,#126247,#126248,
#126249,#126250,#126251,#126252,#126253,#126254,#126255,#126256,#126257,
#126258,#126259,#126260,#126261,#126262,#126263,#126264,#126265,#126266,
#126267,#126268,#126269,#126270,#126271,#126272,#126273,#126274,#126275,
#126276,#126277,#126278,#126279,#126280,#126281,#126282,#126283,#126284,
#126285,#126286,#126287,#126288,#126289,#126290,#126291,#126292,#126293,
#126294,#126295,#126296,#126297,#126298,#126299,#126300,#126301,#126302,
#126303,#126304,#126305,#126306,#126307,#126308,#126309,#126310,#126311,
#126312,#126313,#126314,#126315,#126316,#126317,#126318,#126319,#126320,
#126321,#126322,#126323,#126324,#126325,#126326,#126327,#126328,#126329,
#126330,#126331,#126332,#126333,#126334,#126335,#126336,#126337,#126338,
#126339,#126340,#126341,#126342,#126343,#126344,#126345,#126346,#126347,
#126348,#126349,#126350,#126351,#126352,#126353,#126354,#126355,#126356,
#126357,#126358,#126359,#126360,#126361,#126362,#126363,#126364,#126365,
#126366,#126367,#126368,#126369,#126370,#126371,#126372,#126373,#126374,
#126375,#126376,#126377,#126378,#126379,#126380,#126381,#126382,#126383,
#126384,#126385,#126386,#126387,#126388,#126389,#126390,#126391,#126392,
#126393,#126394,#126395,#126396,#126397,#126398,#126399,#126400,#126401,
#126402,#126403,#126404,#126405,#126406,#126407,#126408),.UNSPECIFIED.,
 .F.,.F.)
B_SPLINE_CURVE_WITH_KNOTS((6,1,1,1,1,1,1,1,1,1,1,1,1,1,1,1,1,1,1,1,1,1,
1,1,1,1,1,1,1,1,1,1,1,1,1,1,1,1,1,1,1,1,1,1,1,1,1,1,1,1,1,1,1,1,1,1,1,1,
1,1,1,1,1,1,1,1,1,1,1,1,1,1,1,1,1,1,1,1,1,1,1,1,1,1,1,1,1,1,1,1,1,1,1,1,
1,1,1,1,1,1,1,1,1,1,1,1,1,1,1,1,1,1,1,1,1,1,1,1,1,1,1,1,1,1,1,1,1,1,1,1,
1,1,1,1,1,1,1,1,1,1,1,1,1,1,1,1,1,1,1,1,1,1,1,1,1,1,1,1,1,1,1,1,1,1,1,1,
1,1,1,1,1,1,1,1,1,1,1,1,1,1,1,1,1,1,1,1,1,1,1,6),(0.,0.005,0.01,0.015,0.02,
0.025,0.03,0.035,0.04,0.045,0.05,0.055,0.06,0.065,0.07,0.075,0.08,0.085,
0.09,0.095,0.1,0.105,0.11,0.115,0.12,0.125,0.13,0.135,0.14,0.145,0.15,0.155,
0.16,0.165,0.17,0.175,0.18,0.185,0.19,0.195,0.2,0.205,0.21,0.215,0.22,0.225,
0.23,0.235,0.24,0.245,0.25,0.255,0.26,0.265,0.27,0.275,0.28,0.285,0.29,
0.295,0.3,0.305,0.31,0.315,0.32,0.325,0.33,0.335,0.34,0.345,0.35,0.355,
0.36,0.365,0.37,0.375,0.38,0.385,0.39,0.395,0.4,0.405,0.41,0.415,0.42,0.425,
0.43,0.435,0.44,0.445,0.45,0.455,0.46,0.465,0.47,0.475,0.48,0.485,0.49,
0.495,0.5,0.505,0.51,0.515,0.52,0.525,0.53,0.535,0.54,0.545,0.55,0.555,
0.56,0.565,0.57,0.575,0.58,0.585,0.59,0.595,0.6,0.605,0.61,0.615,0.62,0.625,
0.63,0.635,0.64,0.645,0.65,0.655,0.66,0.665,0.67,0.675,0.68,0.685,0.690000000000001,
0.695000000000001,0.700000000000001,0.705000000000001,0.710000000000001,
0.715000000000001,0.720000000000001,0.725000000000001,0.730000000000001,
0.735000000000001,0.740000000000001,0.745000000000001,0.750000000000001,
0.755000000000001,0.760000000000001,0.765000000000001,0.770000000000001,
0.775000000000001,0.780000000000001,0.785000000000001,0.790000000000001,
0.795000000000001,0.800000000000001,0.805000000000001,0.810000000000001,
0.815000000000001,0.820000000000001,0.825000000000001,0.830000000000001,
0.835000000000001,0.840000000000001,0.845000000000001,0.850000000000001,
0.855000000000001,0.860000000000001,0.865000000000001,0.870000000000001,
0.875000000000001,0.880000000000001,0.885000000000001,0.890000000000001,
0.895000000000001,0.900000000000001,0.905000000000001,0.910000000000001,
0.915000000000001,0.920000000000001,0.925000000000001,0.930000000000001,
0.935000000000001,0.940000000000001,0.941429844438209),.UNSPECIFIED.)
CURVE()
GEOMETRIC_REPRESENTATION_ITEM()
RATIONAL_B_SPLINE_CURVE((1.,1.,1.,1.,1.,1.,1.,1.,1.,1.,1.,1.,1.,1.,1.,1.,
1.,1.,1.,1.,1.,1.,1.,1.,1.,1.,1.,1.,1.,1.,1.,1.,1.,1.,1.,1.,1.,1.,1.,1.,
1.,1.,1.,1.,1.,1.,1.,1.,1.,1.,1.,1.,1.,1.,1.,1.,1.,1.,1.,1.,1.,1.,1.,1.,
1.,1.,1.,1.,1.,1.,1.,1.,1.,1.,1.,1.,1.,1.,1.,1.,1.,1.,1.,1.,1.,1.,1.,1.,
1.,1.,1.,1.,1.,1.,1.,1.,1.,1.,1.,1.,1.,1.,1.,1.,1.,1.,1.,1.,1.,1.,1.,1.,
1.,1.,1.,1.,1.,1.,1.,1.,1.,1.,1.,1.,1.,1.,1.,1.,1.,1.,1.,1.,1.,1.,1.,1.,
1.,1.,1.,1.,1.,1.,1.,1.,1.,1.,1.,1.,1.,1.,1.,1.,1.,1.,1.,1.,1.,1.,1.,1.,
1.,1.,1.,1.,1.,1.,1.,1.,1.,1.,1.,1.,1.,1.,1.,1.,1.,1.,1.,1.,1.,1.,1.,1.,
1.,1.,1.,1.,1.,1.,1.,1.,1.,1.))
REPRESENTATION_ITEM('')
);
#570=(
BOUNDED_CURVE()
B_SPLINE_CURVE(5,(#126411,#126412,#126413,#126414,#126415,#126416,#126417,
#126418,#126419,#126420,#126421,#126422,#126423,#126424,#126425,#126426,
#126427,#126428,#126429,#126430,#126431,#126432,#126433,#126434,#126435,
#126436,#126437,#126438,#126439,#126440,#126441,#126442,#126443,#126444,
#126445,#126446,#126447,#126448,#126449,#126450,#126451,#126452,#126453,
#126454,#126455,#126456,#126457,#126458,#126459,#126460,#126461,#126462,
#126463,#126464,#126465,#126466,#126467,#126468,#126469,#126470,#126471,
#126472,#126473,#126474,#126475,#126476,#126477,#126478,#126479,#126480,
#126481,#126482,#126483,#126484,#126485,#126486,#126487,#126488,#126489,
#126490,#126491,#126492,#126493,#126494,#126495,#126496,#126497,#126498,
#126499,#126500,#126501,#126502,#126503,#126504,#126505,#126506,#126507,
#126508,#126509,#126510,#126511,#126512,#126513,#126514,#126515,#126516,
#126517,#126518,#126519,#126520,#126521,#126522,#126523,#126524,#126525,
#126526,#126527,#126528,#126529,#126530,#126531,#126532,#126533,#126534,
#126535,#126536,#126537,#126538,#126539,#126540,#126541,#126542,#126543,
#126544,#126545,#126546,#126547,#126548,#126549,#126550,#126551,#126552,
#126553,#126554,#126555,#126556,#126557,#126558,#126559,#126560,#126561,
#126562,#126563,#126564,#126565,#126566,#126567,#126568,#126569,#126570,
#126571,#126572,#126573,#126574,#126575,#126576,#126577,#126578,#126579,
#126580,#126581,#126582,#126583,#126584,#126585,#126586,#126587,#126588,
#126589,#126590,#126591,#126592,#126593,#126594,#126595,#126596,#126597,
#126598,#126599,#126600,#126601,#126602,#126603,#126604),.UNSPECIFIED.,
 .F.,.F.)
B_SPLINE_CURVE_WITH_KNOTS((6,1,1,1,1,1,1,1,1,1,1,1,1,1,1,1,1,1,1,1,1,1,
1,1,1,1,1,1,1,1,1,1,1,1,1,1,1,1,1,1,1,1,1,1,1,1,1,1,1,1,1,1,1,1,1,1,1,1,
1,1,1,1,1,1,1,1,1,1,1,1,1,1,1,1,1,1,1,1,1,1,1,1,1,1,1,1,1,1,1,1,1,1,1,1,
1,1,1,1,1,1,1,1,1,1,1,1,1,1,1,1,1,1,1,1,1,1,1,1,1,1,1,1,1,1,1,1,1,1,1,1,
1,1,1,1,1,1,1,1,1,1,1,1,1,1,1,1,1,1,1,1,1,1,1,1,1,1,1,1,1,1,1,1,1,1,1,1,
1,1,1,1,1,1,1,1,1,1,1,1,1,1,1,1,1,1,1,1,1,1,1,6),(-0.941429844438221,-0.940000000000001,
-0.935000000000001,-0.930000000000001,-0.925000000000001,-0.920000000000001,
-0.915000000000001,-0.910000000000001,-0.905000000000001,-0.900000000000001,
-0.895000000000001,-0.890000000000001,-0.885000000000001,-0.880000000000001,
-0.875000000000001,-0.870000000000001,-0.865000000000001,-0.860000000000001,
-0.855000000000001,-0.850000000000001,-0.845000000000001,-0.840000000000001,
-0.835000000000001,-0.830000000000001,-0.825000000000001,-0.820000000000001,
-0.815000000000001,-0.810000000000001,-0.805000000000001,-0.800000000000001,
-0.795000000000001,-0.790000000000001,-0.785000000000001,-0.780000000000001,
-0.775000000000001,-0.770000000000001,-0.765000000000001,-0.760000000000001,
-0.755000000000001,-0.750000000000001,-0.745000000000001,-0.740000000000001,
-0.735000000000001,-0.730000000000001,-0.725000000000001,-0.720000000000001,
-0.715000000000001,-0.710000000000001,-0.705000000000001,-0.700000000000001,
-0.695000000000001,-0.690000000000001,-0.685,-0.68,-0.675,-0.67,-0.665,
-0.66,-0.655,-0.65,-0.645,-0.64,-0.635,-0.63,-0.625,-0.62,-0.615,-0.61,
-0.605,-0.6,-0.595,-0.59,-0.585,-0.58,-0.575,-0.57,-0.565,-0.56,-0.555,
-0.55,-0.545,-0.54,-0.535,-0.53,-0.525,-0.52,-0.515,-0.51,-0.505,-0.5,-0.495,
-0.49,-0.485,-0.48,-0.475,-0.47,-0.465,-0.46,-0.455,-0.45,-0.445,-0.44,
-0.435,-0.43,-0.425,-0.42,-0.415,-0.41,-0.405,-0.4,-0.395,-0.39,-0.385,
-0.38,-0.375,-0.37,-0.365,-0.36,-0.355,-0.35,-0.345,-0.34,-0.335,-0.33,
-0.325,-0.32,-0.315,-0.31,-0.305,-0.3,-0.295,-0.29,-0.285,-0.28,-0.275,
-0.27,-0.265,-0.26,-0.255,-0.25,-0.245,-0.24,-0.235,-0.23,-0.225,-0.22,
-0.215,-0.21,-0.205,-0.2,-0.195,-0.19,-0.185,-0.18,-0.175,-0.17,-0.165,
-0.16,-0.155,-0.15,-0.145,-0.14,-0.135,-0.13,-0.125,-0.12,-0.115,-0.11,
-0.105,-0.1,-0.095,-0.09,-0.085,-0.08,-0.075,-0.07,-0.065,-0.06,-0.055,
-0.05,-0.045,-0.04,-0.035,-0.03,-0.025,-0.02,-0.015,-0.01,-0.005,0.),
 .UNSPECIFIED.)
CURVE()
GEOMETRIC_REPRESENTATION_ITEM()
RATIONAL_B_SPLINE_CURVE((1.,1.,1.,1.,1.,1.,1.,1.,1.,1.,1.,1.,1.,1.,1.,1.,
1.,1.,1.,1.,1.,1.,1.,1.,1.,1.,1.,1.,1.,1.,1.,1.,1.,1.,1.,1.,1.,1.,1.,1.,
1.,1.,1.,1.,1.,1.,1.,1.,1.,1.,1.,1.,1.,1.,1.,1.,1.,1.,1.,1.,1.,1.,1.,1.,
1.,1.,1.,1.,1.,1.,1.,1.,1.,1.,1.,1.,1.,1.,1.,1.,1.,1.,1.,1.,1.,1.,1.,1.,
1.,1.,1.,1.,1.,1.,1.,1.,1.,1.,1.,1.,1.,1.,1.,1.,1.,1.,1.,1.,1.,1.,1.,1.,
1.,1.,1.,1.,1.,1.,1.,1.,1.,1.,1.,1.,1.,1.,1.,1.,1.,1.,1.,1.,1.,1.,1.,1.,
1.,1.,1.,1.,1.,1.,1.,1.,1.,1.,1.,1.,1.,1.,1.,1.,1.,1.,1.,1.,1.,1.,1.,1.,
1.,1.,1.,1.,1.,1.,1.,1.,1.,1.,1.,1.,1.,1.,1.,1.,1.,1.,1.,1.,1.,1.,1.,1.,
1.,1.,1.,1.,1.,1.,1.,1.,1.,1.))
REPRESENTATION_ITEM('')
);
#571=(
BOUNDED_CURVE()
B_SPLINE_CURVE(5,(#127016,#127017,#127018,#127019,#127020,#127021,#127022,
#127023,#127024,#127025,#127026,#127027,#127028,#127029,#127030,#127031,
#127032,#127033,#127034,#127035,#127036,#127037,#127038,#127039,#127040,
#127041,#127042,#127043,#127044,#127045,#127046,#127047,#127048,#127049,
#127050,#127051,#127052,#127053,#127054,#127055,#127056,#127057,#127058,
#127059,#127060,#127061,#127062,#127063,#127064,#127065,#127066,#127067,
#127068,#127069,#127070,#127071,#127072,#127073,#127074,#127075,#127076,
#127077,#127078,#127079,#127080,#127081,#127082,#127083,#127084,#127085,
#127086,#127087,#127088,#127089,#127090,#127091,#127092,#127093,#127094,
#127095,#127096,#127097,#127098,#127099,#127100,#127101,#127102,#127103,
#127104,#127105,#127106,#127107,#127108,#127109,#127110,#127111,#127112,
#127113,#127114,#127115,#127116,#127117,#127118,#127119,#127120,#127121,
#127122,#127123,#127124,#127125,#127126,#127127,#127128,#127129,#127130,
#127131,#127132,#127133,#127134,#127135,#127136,#127137,#127138,#127139,
#127140,#127141,#127142,#127143,#127144,#127145,#127146,#127147,#127148,
#127149,#127150,#127151,#127152,#127153,#127154,#127155,#127156,#127157,
#127158,#127159,#127160,#127161,#127162,#127163,#127164,#127165,#127166,
#127167,#127168,#127169,#127170,#127171,#127172,#127173,#127174,#127175,
#127176,#127177,#127178,#127179,#127180,#127181,#127182,#127183,#127184,
#127185,#127186,#127187,#127188,#127189,#127190,#127191,#127192,#127193,
#127194,#127195,#127196,#127197,#127198,#127199,#127200,#127201,#127202,
#127203,#127204,#127205,#127206,#127207,#127208,#127209),.UNSPECIFIED.,
 .F.,.F.)
B_SPLINE_CURVE_WITH_KNOTS((6,1,1,1,1,1,1,1,1,1,1,1,1,1,1,1,1,1,1,1,1,1,
1,1,1,1,1,1,1,1,1,1,1,1,1,1,1,1,1,1,1,1,1,1,1,1,1,1,1,1,1,1,1,1,1,1,1,1,
1,1,1,1,1,1,1,1,1,1,1,1,1,1,1,1,1,1,1,1,1,1,1,1,1,1,1,1,1,1,1,1,1,1,1,1,
1,1,1,1,1,1,1,1,1,1,1,1,1,1,1,1,1,1,1,1,1,1,1,1,1,1,1,1,1,1,1,1,1,1,1,1,
1,1,1,1,1,1,1,1,1,1,1,1,1,1,1,1,1,1,1,1,1,1,1,1,1,1,1,1,1,1,1,1,1,1,1,1,
1,1,1,1,1,1,1,1,1,1,1,1,1,1,1,1,1,1,1,1,1,1,1,6),(0.,0.005,0.01,0.015,0.02,
0.025,0.03,0.035,0.04,0.045,0.05,0.055,0.06,0.065,0.07,0.075,0.08,0.085,
0.09,0.095,0.1,0.105,0.11,0.115,0.12,0.125,0.13,0.135,0.14,0.145,0.15,0.155,
0.16,0.165,0.17,0.175,0.18,0.185,0.19,0.195,0.2,0.205,0.21,0.215,0.22,0.225,
0.23,0.235,0.24,0.245,0.25,0.255,0.26,0.265,0.27,0.275,0.28,0.285,0.29,
0.295,0.3,0.305,0.31,0.315,0.32,0.325,0.33,0.335,0.34,0.345,0.35,0.355,
0.36,0.365,0.37,0.375,0.38,0.385,0.39,0.395,0.4,0.405,0.41,0.415,0.42,0.425,
0.43,0.435,0.44,0.445,0.45,0.455,0.46,0.465,0.47,0.475,0.48,0.485,0.49,
0.495,0.5,0.505,0.51,0.515,0.52,0.525,0.53,0.535,0.54,0.545,0.55,0.555,
0.56,0.565,0.57,0.575,0.58,0.585,0.59,0.595,0.6,0.605,0.61,0.615,0.62,0.625,
0.63,0.635,0.64,0.645,0.65,0.655,0.66,0.665,0.67,0.675,0.68,0.685,0.690000000000001,
0.695000000000001,0.700000000000001,0.705000000000001,0.710000000000001,
0.715000000000001,0.720000000000001,0.725000000000001,0.730000000000001,
0.735000000000001,0.740000000000001,0.745000000000001,0.750000000000001,
0.755000000000001,0.760000000000001,0.765000000000001,0.770000000000001,
0.775000000000001,0.780000000000001,0.785000000000001,0.790000000000001,
0.795000000000001,0.800000000000001,0.805000000000001,0.810000000000001,
0.815000000000001,0.820000000000001,0.825000000000001,0.830000000000001,
0.835000000000001,0.840000000000001,0.845000000000001,0.850000000000001,
0.855000000000001,0.860000000000001,0.865000000000001,0.870000000000001,
0.875000000000001,0.880000000000001,0.885000000000001,0.890000000000001,
0.895000000000001,0.900000000000001,0.905000000000001,0.910000000000001,
0.915000000000001,0.920000000000001,0.925000000000001,0.930000000000001,
0.935000000000001,0.940000000000001,0.941429844438077),.UNSPECIFIED.)
CURVE()
GEOMETRIC_REPRESENTATION_ITEM()
RATIONAL_B_SPLINE_CURVE((1.,1.,1.,1.,1.,1.,1.,1.,1.,1.,1.,1.,1.,1.,1.,1.,
1.,1.,1.,1.,1.,1.,1.,1.,1.,1.,1.,1.,1.,1.,1.,1.,1.,1.,1.,1.,1.,1.,1.,1.,
1.,1.,1.,1.,1.,1.,1.,1.,1.,1.,1.,1.,1.,1.,1.,1.,1.,1.,1.,1.,1.,1.,1.,1.,
1.,1.,1.,1.,1.,1.,1.,1.,1.,1.,1.,1.,1.,1.,1.,1.,1.,1.,1.,1.,1.,1.,1.,1.,
1.,1.,1.,1.,1.,1.,1.,1.,1.,1.,1.,1.,1.,1.,1.,1.,1.,1.,1.,1.,1.,1.,1.,1.,
1.,1.,1.,1.,1.,1.,1.,1.,1.,1.,1.,1.,1.,1.,1.,1.,1.,1.,1.,1.,1.,1.,1.,1.,
1.,1.,1.,1.,1.,1.,1.,1.,1.,1.,1.,1.,1.,1.,1.,1.,1.,1.,1.,1.,1.,1.,1.,1.,
1.,1.,1.,1.,1.,1.,1.,1.,1.,1.,1.,1.,1.,1.,1.,1.,1.,1.,1.,1.,1.,1.,1.,1.,
1.,1.,1.,1.,1.,1.,1.,1.,1.,1.))
REPRESENTATION_ITEM('')
);
#572=(
BOUNDED_CURVE()
B_SPLINE_CURVE(5,(#127212,#127213,#127214,#127215,#127216,#127217,#127218,
#127219,#127220,#127221,#127222,#127223,#127224,#127225,#127226,#127227,
#127228,#127229,#127230,#127231,#127232,#127233,#127234,#127235,#127236,
#127237,#127238,#127239,#127240,#127241,#127242,#127243,#127244,#127245,
#127246,#127247,#127248,#127249,#127250,#127251,#127252,#127253,#127254,
#127255,#127256,#127257,#127258,#127259,#127260,#127261,#127262,#127263,
#127264,#127265,#127266,#127267,#127268,#127269,#127270,#127271,#127272,
#127273,#127274,#127275,#127276,#127277,#127278,#127279,#127280,#127281,
#127282,#127283,#127284,#127285,#127286,#127287,#127288,#127289,#127290,
#127291,#127292,#127293,#127294,#127295,#127296,#127297,#127298,#127299,
#127300,#127301,#127302,#127303,#127304,#127305,#127306,#127307,#127308,
#127309,#127310,#127311,#127312,#127313,#127314,#127315,#127316,#127317,
#127318,#127319,#127320,#127321,#127322,#127323,#127324,#127325,#127326,
#127327,#127328,#127329,#127330,#127331,#127332,#127333,#127334,#127335,
#127336,#127337,#127338,#127339,#127340,#127341,#127342,#127343,#127344,
#127345,#127346,#127347,#127348,#127349,#127350,#127351,#127352,#127353,
#127354,#127355,#127356,#127357,#127358,#127359,#127360,#127361,#127362,
#127363,#127364,#127365,#127366,#127367,#127368,#127369,#127370,#127371,
#127372,#127373,#127374,#127375,#127376,#127377,#127378,#127379,#127380,
#127381,#127382,#127383,#127384,#127385,#127386,#127387,#127388,#127389,
#127390,#127391,#127392,#127393,#127394,#127395,#127396,#127397,#127398,
#127399,#127400,#127401,#127402,#127403,#127404,#127405),.UNSPECIFIED.,
 .F.,.F.)
B_SPLINE_CURVE_WITH_KNOTS((6,1,1,1,1,1,1,1,1,1,1,1,1,1,1,1,1,1,1,1,1,1,
1,1,1,1,1,1,1,1,1,1,1,1,1,1,1,1,1,1,1,1,1,1,1,1,1,1,1,1,1,1,1,1,1,1,1,1,
1,1,1,1,1,1,1,1,1,1,1,1,1,1,1,1,1,1,1,1,1,1,1,1,1,1,1,1,1,1,1,1,1,1,1,1,
1,1,1,1,1,1,1,1,1,1,1,1,1,1,1,1,1,1,1,1,1,1,1,1,1,1,1,1,1,1,1,1,1,1,1,1,
1,1,1,1,1,1,1,1,1,1,1,1,1,1,1,1,1,1,1,1,1,1,1,1,1,1,1,1,1,1,1,1,1,1,1,1,
1,1,1,1,1,1,1,1,1,1,1,1,1,1,1,1,1,1,1,1,1,1,1,6),(-0.941429844438077,-0.940000000000001,
-0.935000000000001,-0.930000000000001,-0.925000000000001,-0.920000000000001,
-0.915000000000001,-0.910000000000001,-0.905000000000001,-0.900000000000001,
-0.895000000000001,-0.890000000000001,-0.885000000000001,-0.880000000000001,
-0.875000000000001,-0.870000000000001,-0.865000000000001,-0.860000000000001,
-0.855000000000001,-0.850000000000001,-0.845000000000001,-0.840000000000001,
-0.835000000000001,-0.830000000000001,-0.825000000000001,-0.820000000000001,
-0.815000000000001,-0.810000000000001,-0.805000000000001,-0.800000000000001,
-0.795000000000001,-0.790000000000001,-0.785000000000001,-0.780000000000001,
-0.775000000000001,-0.770000000000001,-0.765000000000001,-0.760000000000001,
-0.755000000000001,-0.750000000000001,-0.745000000000001,-0.740000000000001,
-0.735000000000001,-0.730000000000001,-0.725000000000001,-0.720000000000001,
-0.715000000000001,-0.710000000000001,-0.705000000000001,-0.700000000000001,
-0.695000000000001,-0.690000000000001,-0.685,-0.68,-0.675,-0.67,-0.665,
-0.66,-0.655,-0.65,-0.645,-0.64,-0.635,-0.63,-0.625,-0.62,-0.615,-0.61,
-0.605,-0.6,-0.595,-0.59,-0.585,-0.58,-0.575,-0.57,-0.565,-0.56,-0.555,
-0.55,-0.545,-0.54,-0.535,-0.53,-0.525,-0.52,-0.515,-0.51,-0.505,-0.5,-0.495,
-0.49,-0.485,-0.48,-0.475,-0.47,-0.465,-0.46,-0.455,-0.45,-0.445,-0.44,
-0.435,-0.43,-0.425,-0.42,-0.415,-0.41,-0.405,-0.4,-0.395,-0.39,-0.385,
-0.38,-0.375,-0.37,-0.365,-0.36,-0.355,-0.35,-0.345,-0.34,-0.335,-0.33,
-0.325,-0.32,-0.315,-0.31,-0.305,-0.3,-0.295,-0.29,-0.285,-0.28,-0.275,
-0.27,-0.265,-0.26,-0.255,-0.25,-0.245,-0.24,-0.235,-0.23,-0.225,-0.22,
-0.215,-0.21,-0.205,-0.2,-0.195,-0.19,-0.185,-0.18,-0.175,-0.17,-0.165,
-0.16,-0.155,-0.15,-0.145,-0.14,-0.135,-0.13,-0.125,-0.12,-0.115,-0.11,
-0.105,-0.1,-0.095,-0.09,-0.085,-0.08,-0.075,-0.07,-0.065,-0.06,-0.055,
-0.05,-0.045,-0.04,-0.035,-0.03,-0.025,-0.02,-0.015,-0.01,-0.005,0.),
 .UNSPECIFIED.)
CURVE()
GEOMETRIC_REPRESENTATION_ITEM()
RATIONAL_B_SPLINE_CURVE((1.,1.,1.,1.,1.,1.,1.,1.,1.,1.,1.,1.,1.,1.,1.,1.,
1.,1.,1.,1.,1.,1.,1.,1.,1.,1.,1.,1.,1.,1.,1.,1.,1.,1.,1.,1.,1.,1.,1.,1.,
1.,1.,1.,1.,1.,1.,1.,1.,1.,1.,1.,1.,1.,1.,1.,1.,1.,1.,1.,1.,1.,1.,1.,1.,
1.,1.,1.,1.,1.,1.,1.,1.,1.,1.,1.,1.,1.,1.,1.,1.,1.,1.,1.,1.,1.,1.,1.,1.,
1.,1.,1.,1.,1.,1.,1.,1.,1.,1.,1.,1.,1.,1.,1.,1.,1.,1.,1.,1.,1.,1.,1.,1.,
1.,1.,1.,1.,1.,1.,1.,1.,1.,1.,1.,1.,1.,1.,1.,1.,1.,1.,1.,1.,1.,1.,1.,1.,
1.,1.,1.,1.,1.,1.,1.,1.,1.,1.,1.,1.,1.,1.,1.,1.,1.,1.,1.,1.,1.,1.,1.,1.,
1.,1.,1.,1.,1.,1.,1.,1.,1.,1.,1.,1.,1.,1.,1.,1.,1.,1.,1.,1.,1.,1.,1.,1.,
1.,1.,1.,1.,1.,1.,1.,1.,1.,1.))
REPRESENTATION_ITEM('')
);
#573=(
BOUNDED_CURVE()
B_SPLINE_CURVE(5,(#127817,#127818,#127819,#127820,#127821,#127822,#127823,
#127824,#127825,#127826,#127827,#127828,#127829,#127830,#127831,#127832,
#127833,#127834,#127835,#127836,#127837,#127838,#127839,#127840,#127841,
#127842,#127843,#127844,#127845,#127846,#127847,#127848,#127849,#127850,
#127851,#127852,#127853,#127854,#127855,#127856,#127857,#127858,#127859,
#127860,#127861,#127862,#127863,#127864,#127865,#127866,#127867,#127868,
#127869,#127870,#127871,#127872,#127873,#127874,#127875,#127876,#127877,
#127878,#127879,#127880,#127881,#127882,#127883,#127884,#127885,#127886,
#127887,#127888,#127889,#127890,#127891,#127892,#127893,#127894,#127895,
#127896,#127897,#127898,#127899,#127900,#127901,#127902,#127903,#127904,
#127905,#127906,#127907,#127908,#127909,#127910,#127911,#127912,#127913,
#127914,#127915,#127916,#127917,#127918,#127919,#127920,#127921,#127922,
#127923,#127924,#127925,#127926,#127927,#127928,#127929,#127930,#127931,
#127932,#127933,#127934,#127935,#127936,#127937,#127938,#127939,#127940,
#127941,#127942,#127943,#127944,#127945,#127946,#127947,#127948,#127949,
#127950,#127951,#127952,#127953,#127954,#127955,#127956,#127957,#127958,
#127959,#127960,#127961,#127962,#127963,#127964,#127965,#127966,#127967,
#127968,#127969,#127970,#127971,#127972,#127973,#127974,#127975,#127976,
#127977,#127978,#127979,#127980,#127981,#127982,#127983,#127984,#127985,
#127986,#127987,#127988,#127989,#127990,#127991,#127992,#127993,#127994,
#127995,#127996,#127997,#127998,#127999,#128000,#128001,#128002,#128003,
#128004,#128005,#128006,#128007,#128008,#128009,#128010),.UNSPECIFIED.,
 .F.,.F.)
B_SPLINE_CURVE_WITH_KNOTS((6,1,1,1,1,1,1,1,1,1,1,1,1,1,1,1,1,1,1,1,1,1,
1,1,1,1,1,1,1,1,1,1,1,1,1,1,1,1,1,1,1,1,1,1,1,1,1,1,1,1,1,1,1,1,1,1,1,1,
1,1,1,1,1,1,1,1,1,1,1,1,1,1,1,1,1,1,1,1,1,1,1,1,1,1,1,1,1,1,1,1,1,1,1,1,
1,1,1,1,1,1,1,1,1,1,1,1,1,1,1,1,1,1,1,1,1,1,1,1,1,1,1,1,1,1,1,1,1,1,1,1,
1,1,1,1,1,1,1,1,1,1,1,1,1,1,1,1,1,1,1,1,1,1,1,1,1,1,1,1,1,1,1,1,1,1,1,1,
1,1,1,1,1,1,1,1,1,1,1,1,1,1,1,1,1,1,1,1,1,1,1,6),(0.,0.005,0.01,0.015,0.02,
0.025,0.03,0.035,0.04,0.045,0.05,0.055,0.06,0.065,0.07,0.075,0.08,0.085,
0.09,0.095,0.1,0.105,0.11,0.115,0.12,0.125,0.13,0.135,0.14,0.145,0.15,0.155,
0.16,0.165,0.17,0.175,0.18,0.185,0.19,0.195,0.2,0.205,0.21,0.215,0.22,0.225,
0.23,0.235,0.24,0.245,0.25,0.255,0.26,0.265,0.27,0.275,0.28,0.285,0.29,
0.295,0.3,0.305,0.31,0.315,0.32,0.325,0.33,0.335,0.34,0.345,0.35,0.355,
0.36,0.365,0.37,0.375,0.38,0.385,0.39,0.395,0.4,0.405,0.41,0.415,0.42,0.425,
0.43,0.435,0.44,0.445,0.45,0.455,0.46,0.465,0.47,0.475,0.48,0.485,0.49,
0.495,0.5,0.505,0.51,0.515,0.52,0.525,0.53,0.535,0.54,0.545,0.55,0.555,
0.56,0.565,0.57,0.575,0.58,0.585,0.59,0.595,0.6,0.605,0.61,0.615,0.62,0.625,
0.63,0.635,0.64,0.645,0.65,0.655,0.66,0.665,0.67,0.675,0.68,0.685,0.690000000000001,
0.695000000000001,0.700000000000001,0.705000000000001,0.710000000000001,
0.715000000000001,0.720000000000001,0.725000000000001,0.730000000000001,
0.735000000000001,0.740000000000001,0.745000000000001,0.750000000000001,
0.755000000000001,0.760000000000001,0.765000000000001,0.770000000000001,
0.775000000000001,0.780000000000001,0.785000000000001,0.790000000000001,
0.795000000000001,0.800000000000001,0.805000000000001,0.810000000000001,
0.815000000000001,0.820000000000001,0.825000000000001,0.830000000000001,
0.835000000000001,0.840000000000001,0.845000000000001,0.850000000000001,
0.855000000000001,0.860000000000001,0.865000000000001,0.870000000000001,
0.875000000000001,0.880000000000001,0.885000000000001,0.890000000000001,
0.895000000000001,0.900000000000001,0.905000000000001,0.910000000000001,
0.915000000000001,0.920000000000001,0.925000000000001,0.930000000000001,
0.935000000000001,0.940000000000001,0.94142984443807),.UNSPECIFIED.)
CURVE()
GEOMETRIC_REPRESENTATION_ITEM()
RATIONAL_B_SPLINE_CURVE((1.,1.,1.,1.,1.,1.,1.,1.,1.,1.,1.,1.,1.,1.,1.,1.,
1.,1.,1.,1.,1.,1.,1.,1.,1.,1.,1.,1.,1.,1.,1.,1.,1.,1.,1.,1.,1.,1.,1.,1.,
1.,1.,1.,1.,1.,1.,1.,1.,1.,1.,1.,1.,1.,1.,1.,1.,1.,1.,1.,1.,1.,1.,1.,1.,
1.,1.,1.,1.,1.,1.,1.,1.,1.,1.,1.,1.,1.,1.,1.,1.,1.,1.,1.,1.,1.,1.,1.,1.,
1.,1.,1.,1.,1.,1.,1.,1.,1.,1.,1.,1.,1.,1.,1.,1.,1.,1.,1.,1.,1.,1.,1.,1.,
1.,1.,1.,1.,1.,1.,1.,1.,1.,1.,1.,1.,1.,1.,1.,1.,1.,1.,1.,1.,1.,1.,1.,1.,
1.,1.,1.,1.,1.,1.,1.,1.,1.,1.,1.,1.,1.,1.,1.,1.,1.,1.,1.,1.,1.,1.,1.,1.,
1.,1.,1.,1.,1.,1.,1.,1.,1.,1.,1.,1.,1.,1.,1.,1.,1.,1.,1.,1.,1.,1.,1.,1.,
1.,1.,1.,1.,1.,1.,1.,1.,1.,1.))
REPRESENTATION_ITEM('')
);
#574=(
BOUNDED_CURVE()
B_SPLINE_CURVE(5,(#128013,#128014,#128015,#128016,#128017,#128018,#128019,
#128020,#128021,#128022,#128023,#128024,#128025,#128026,#128027,#128028,
#128029,#128030,#128031,#128032,#128033,#128034,#128035,#128036,#128037,
#128038,#128039,#128040,#128041,#128042,#128043,#128044,#128045,#128046,
#128047,#128048,#128049,#128050,#128051,#128052,#128053,#128054,#128055,
#128056,#128057,#128058,#128059,#128060,#128061,#128062,#128063,#128064,
#128065,#128066,#128067,#128068,#128069,#128070,#128071,#128072,#128073,
#128074,#128075,#128076,#128077,#128078,#128079,#128080,#128081,#128082,
#128083,#128084,#128085,#128086,#128087,#128088,#128089,#128090,#128091,
#128092,#128093,#128094,#128095,#128096,#128097,#128098,#128099,#128100,
#128101,#128102,#128103,#128104,#128105,#128106,#128107,#128108,#128109,
#128110,#128111,#128112,#128113,#128114,#128115,#128116,#128117,#128118,
#128119,#128120,#128121,#128122,#128123,#128124,#128125,#128126,#128127,
#128128,#128129,#128130,#128131,#128132,#128133,#128134,#128135,#128136,
#128137,#128138,#128139,#128140,#128141,#128142,#128143,#128144,#128145,
#128146,#128147,#128148,#128149,#128150,#128151,#128152,#128153,#128154,
#128155,#128156,#128157,#128158,#128159,#128160,#128161,#128162,#128163,
#128164,#128165,#128166,#128167,#128168,#128169,#128170,#128171,#128172,
#128173,#128174,#128175,#128176,#128177,#128178,#128179,#128180,#128181,
#128182,#128183,#128184,#128185,#128186,#128187,#128188,#128189,#128190,
#128191,#128192,#128193,#128194,#128195,#128196,#128197,#128198,#128199,
#128200,#128201,#128202,#128203,#128204,#128205,#128206),.UNSPECIFIED.,
 .F.,.F.)
B_SPLINE_CURVE_WITH_KNOTS((6,1,1,1,1,1,1,1,1,1,1,1,1,1,1,1,1,1,1,1,1,1,
1,1,1,1,1,1,1,1,1,1,1,1,1,1,1,1,1,1,1,1,1,1,1,1,1,1,1,1,1,1,1,1,1,1,1,1,
1,1,1,1,1,1,1,1,1,1,1,1,1,1,1,1,1,1,1,1,1,1,1,1,1,1,1,1,1,1,1,1,1,1,1,1,
1,1,1,1,1,1,1,1,1,1,1,1,1,1,1,1,1,1,1,1,1,1,1,1,1,1,1,1,1,1,1,1,1,1,1,1,
1,1,1,1,1,1,1,1,1,1,1,1,1,1,1,1,1,1,1,1,1,1,1,1,1,1,1,1,1,1,1,1,1,1,1,1,
1,1,1,1,1,1,1,1,1,1,1,1,1,1,1,1,1,1,1,1,1,1,1,6),(-0.941429844438071,-0.940000000000001,
-0.935000000000001,-0.930000000000001,-0.925000000000001,-0.920000000000001,
-0.915000000000001,-0.910000000000001,-0.905000000000001,-0.900000000000001,
-0.895000000000001,-0.890000000000001,-0.885000000000001,-0.880000000000001,
-0.875000000000001,-0.870000000000001,-0.865000000000001,-0.860000000000001,
-0.855000000000001,-0.850000000000001,-0.845000000000001,-0.840000000000001,
-0.835000000000001,-0.830000000000001,-0.825000000000001,-0.820000000000001,
-0.815000000000001,-0.810000000000001,-0.805000000000001,-0.800000000000001,
-0.795000000000001,-0.790000000000001,-0.785000000000001,-0.780000000000001,
-0.775000000000001,-0.770000000000001,-0.765000000000001,-0.760000000000001,
-0.755000000000001,-0.750000000000001,-0.745000000000001,-0.740000000000001,
-0.735000000000001,-0.730000000000001,-0.725000000000001,-0.720000000000001,
-0.715000000000001,-0.710000000000001,-0.705000000000001,-0.700000000000001,
-0.695000000000001,-0.690000000000001,-0.685,-0.68,-0.675,-0.67,-0.665,
-0.66,-0.655,-0.65,-0.645,-0.64,-0.635,-0.63,-0.625,-0.62,-0.615,-0.61,
-0.605,-0.6,-0.595,-0.59,-0.585,-0.58,-0.575,-0.57,-0.565,-0.56,-0.555,
-0.55,-0.545,-0.54,-0.535,-0.53,-0.525,-0.52,-0.515,-0.51,-0.505,-0.5,-0.495,
-0.49,-0.485,-0.48,-0.475,-0.47,-0.465,-0.46,-0.455,-0.45,-0.445,-0.44,
-0.435,-0.43,-0.425,-0.42,-0.415,-0.41,-0.405,-0.4,-0.395,-0.39,-0.385,
-0.38,-0.375,-0.37,-0.365,-0.36,-0.355,-0.35,-0.345,-0.34,-0.335,-0.33,
-0.325,-0.32,-0.315,-0.31,-0.305,-0.3,-0.295,-0.29,-0.285,-0.28,-0.275,
-0.27,-0.265,-0.26,-0.255,-0.25,-0.245,-0.24,-0.235,-0.23,-0.225,-0.22,
-0.215,-0.21,-0.205,-0.2,-0.195,-0.19,-0.185,-0.18,-0.175,-0.17,-0.165,
-0.16,-0.155,-0.15,-0.145,-0.14,-0.135,-0.13,-0.125,-0.12,-0.115,-0.11,
-0.105,-0.1,-0.095,-0.09,-0.085,-0.08,-0.075,-0.07,-0.065,-0.06,-0.055,
-0.05,-0.045,-0.04,-0.035,-0.03,-0.025,-0.02,-0.015,-0.01,-0.005,0.),
 .UNSPECIFIED.)
CURVE()
GEOMETRIC_REPRESENTATION_ITEM()
RATIONAL_B_SPLINE_CURVE((1.,1.,1.,1.,1.,1.,1.,1.,1.,1.,1.,1.,1.,1.,1.,1.,
1.,1.,1.,1.,1.,1.,1.,1.,1.,1.,1.,1.,1.,1.,1.,1.,1.,1.,1.,1.,1.,1.,1.,1.,
1.,1.,1.,1.,1.,1.,1.,1.,1.,1.,1.,1.,1.,1.,1.,1.,1.,1.,1.,1.,1.,1.,1.,1.,
1.,1.,1.,1.,1.,1.,1.,1.,1.,1.,1.,1.,1.,1.,1.,1.,1.,1.,1.,1.,1.,1.,1.,1.,
1.,1.,1.,1.,1.,1.,1.,1.,1.,1.,1.,1.,1.,1.,1.,1.,1.,1.,1.,1.,1.,1.,1.,1.,
1.,1.,1.,1.,1.,1.,1.,1.,1.,1.,1.,1.,1.,1.,1.,1.,1.,1.,1.,1.,1.,1.,1.,1.,
1.,1.,1.,1.,1.,1.,1.,1.,1.,1.,1.,1.,1.,1.,1.,1.,1.,1.,1.,1.,1.,1.,1.,1.,
1.,1.,1.,1.,1.,1.,1.,1.,1.,1.,1.,1.,1.,1.,1.,1.,1.,1.,1.,1.,1.,1.,1.,1.,
1.,1.,1.,1.,1.,1.,1.,1.,1.,1.))
REPRESENTATION_ITEM('')
);
#575=(
BOUNDED_CURVE()
B_SPLINE_CURVE(5,(#128618,#128619,#128620,#128621,#128622,#128623,#128624,
#128625,#128626,#128627,#128628,#128629,#128630,#128631,#128632,#128633,
#128634,#128635,#128636,#128637,#128638,#128639,#128640,#128641,#128642,
#128643,#128644,#128645,#128646,#128647,#128648,#128649,#128650,#128651,
#128652,#128653,#128654,#128655,#128656,#128657,#128658,#128659,#128660,
#128661,#128662,#128663,#128664,#128665,#128666,#128667,#128668,#128669,
#128670,#128671,#128672,#128673,#128674,#128675,#128676,#128677,#128678,
#128679,#128680,#128681,#128682,#128683,#128684,#128685,#128686,#128687,
#128688,#128689,#128690,#128691,#128692,#128693,#128694,#128695,#128696,
#128697,#128698,#128699,#128700,#128701,#128702,#128703,#128704,#128705,
#128706,#128707,#128708,#128709,#128710,#128711,#128712,#128713,#128714,
#128715,#128716,#128717,#128718,#128719,#128720,#128721,#128722,#128723,
#128724,#128725,#128726,#128727,#128728,#128729,#128730,#128731,#128732,
#128733,#128734,#128735,#128736,#128737,#128738,#128739,#128740,#128741,
#128742,#128743,#128744,#128745,#128746,#128747,#128748,#128749,#128750,
#128751,#128752,#128753,#128754,#128755,#128756,#128757,#128758,#128759,
#128760,#128761,#128762,#128763,#128764,#128765,#128766,#128767,#128768,
#128769,#128770,#128771,#128772,#128773,#128774,#128775,#128776,#128777,
#128778,#128779,#128780,#128781,#128782,#128783,#128784,#128785,#128786,
#128787,#128788,#128789,#128790,#128791,#128792,#128793,#128794,#128795,
#128796,#128797,#128798,#128799,#128800,#128801,#128802,#128803,#128804,
#128805,#128806,#128807,#128808,#128809,#128810,#128811),.UNSPECIFIED.,
 .F.,.F.)
B_SPLINE_CURVE_WITH_KNOTS((6,1,1,1,1,1,1,1,1,1,1,1,1,1,1,1,1,1,1,1,1,1,
1,1,1,1,1,1,1,1,1,1,1,1,1,1,1,1,1,1,1,1,1,1,1,1,1,1,1,1,1,1,1,1,1,1,1,1,
1,1,1,1,1,1,1,1,1,1,1,1,1,1,1,1,1,1,1,1,1,1,1,1,1,1,1,1,1,1,1,1,1,1,1,1,
1,1,1,1,1,1,1,1,1,1,1,1,1,1,1,1,1,1,1,1,1,1,1,1,1,1,1,1,1,1,1,1,1,1,1,1,
1,1,1,1,1,1,1,1,1,1,1,1,1,1,1,1,1,1,1,1,1,1,1,1,1,1,1,1,1,1,1,1,1,1,1,1,
1,1,1,1,1,1,1,1,1,1,1,1,1,1,1,1,1,1,1,1,1,1,1,6),(0.,0.005,0.01,0.015,0.02,
0.025,0.03,0.035,0.04,0.045,0.05,0.055,0.06,0.065,0.07,0.075,0.08,0.085,
0.09,0.095,0.1,0.105,0.11,0.115,0.12,0.125,0.13,0.135,0.14,0.145,0.15,0.155,
0.16,0.165,0.17,0.175,0.18,0.185,0.19,0.195,0.2,0.205,0.21,0.215,0.22,0.225,
0.23,0.235,0.24,0.245,0.25,0.255,0.26,0.265,0.27,0.275,0.28,0.285,0.29,
0.295,0.3,0.305,0.31,0.315,0.32,0.325,0.33,0.335,0.34,0.345,0.35,0.355,
0.36,0.365,0.37,0.375,0.38,0.385,0.39,0.395,0.4,0.405,0.41,0.415,0.42,0.425,
0.43,0.435,0.44,0.445,0.45,0.455,0.46,0.465,0.47,0.475,0.48,0.485,0.49,
0.495,0.5,0.505,0.51,0.515,0.52,0.525,0.53,0.535,0.54,0.545,0.55,0.555,
0.56,0.565,0.57,0.575,0.58,0.585,0.59,0.595,0.6,0.605,0.61,0.615,0.62,0.625,
0.63,0.635,0.64,0.645,0.65,0.655,0.66,0.665,0.67,0.675,0.68,0.685,0.690000000000001,
0.695000000000001,0.700000000000001,0.705000000000001,0.710000000000001,
0.715000000000001,0.720000000000001,0.725000000000001,0.730000000000001,
0.735000000000001,0.740000000000001,0.745000000000001,0.750000000000001,
0.755000000000001,0.760000000000001,0.765000000000001,0.770000000000001,
0.775000000000001,0.780000000000001,0.785000000000001,0.790000000000001,
0.795000000000001,0.800000000000001,0.805000000000001,0.810000000000001,
0.815000000000001,0.820000000000001,0.825000000000001,0.830000000000001,
0.835000000000001,0.840000000000001,0.845000000000001,0.850000000000001,
0.855000000000001,0.860000000000001,0.865000000000001,0.870000000000001,
0.875000000000001,0.880000000000001,0.885000000000001,0.890000000000001,
0.895000000000001,0.900000000000001,0.905000000000001,0.910000000000001,
0.915000000000001,0.920000000000001,0.925000000000001,0.930000000000001,
0.935000000000001,0.940000000000001,0.94142984443807),.UNSPECIFIED.)
CURVE()
GEOMETRIC_REPRESENTATION_ITEM()
RATIONAL_B_SPLINE_CURVE((1.,1.,1.,1.,1.,1.,1.,1.,1.,1.,1.,1.,1.,1.,1.,1.,
1.,1.,1.,1.,1.,1.,1.,1.,1.,1.,1.,1.,1.,1.,1.,1.,1.,1.,1.,1.,1.,1.,1.,1.,
1.,1.,1.,1.,1.,1.,1.,1.,1.,1.,1.,1.,1.,1.,1.,1.,1.,1.,1.,1.,1.,1.,1.,1.,
1.,1.,1.,1.,1.,1.,1.,1.,1.,1.,1.,1.,1.,1.,1.,1.,1.,1.,1.,1.,1.,1.,1.,1.,
1.,1.,1.,1.,1.,1.,1.,1.,1.,1.,1.,1.,1.,1.,1.,1.,1.,1.,1.,1.,1.,1.,1.,1.,
1.,1.,1.,1.,1.,1.,1.,1.,1.,1.,1.,1.,1.,1.,1.,1.,1.,1.,1.,1.,1.,1.,1.,1.,
1.,1.,1.,1.,1.,1.,1.,1.,1.,1.,1.,1.,1.,1.,1.,1.,1.,1.,1.,1.,1.,1.,1.,1.,
1.,1.,1.,1.,1.,1.,1.,1.,1.,1.,1.,1.,1.,1.,1.,1.,1.,1.,1.,1.,1.,1.,1.,1.,
1.,1.,1.,1.,1.,1.,1.,1.,1.,1.))
REPRESENTATION_ITEM('')
);
#576=(
BOUNDED_CURVE()
B_SPLINE_CURVE(5,(#128814,#128815,#128816,#128817,#128818,#128819,#128820,
#128821,#128822,#128823,#128824,#128825,#128826,#128827,#128828,#128829,
#128830,#128831,#128832,#128833,#128834,#128835,#128836,#128837,#128838,
#128839,#128840,#128841,#128842,#128843,#128844,#128845,#128846,#128847,
#128848,#128849,#128850,#128851,#128852,#128853,#128854,#128855,#128856,
#128857,#128858,#128859,#128860,#128861,#128862,#128863,#128864,#128865,
#128866,#128867,#128868,#128869,#128870,#128871,#128872,#128873,#128874,
#128875,#128876,#128877,#128878,#128879,#128880,#128881,#128882,#128883,
#128884,#128885,#128886,#128887,#128888,#128889,#128890,#128891,#128892,
#128893,#128894,#128895,#128896,#128897,#128898,#128899,#128900,#128901,
#128902,#128903,#128904,#128905,#128906,#128907,#128908,#128909,#128910,
#128911,#128912,#128913,#128914,#128915,#128916,#128917,#128918,#128919,
#128920,#128921,#128922,#128923,#128924,#128925,#128926,#128927,#128928,
#128929,#128930,#128931,#128932,#128933,#128934,#128935,#128936,#128937,
#128938,#128939,#128940,#128941,#128942,#128943,#128944,#128945,#128946,
#128947,#128948,#128949,#128950,#128951,#128952,#128953,#128954,#128955,
#128956,#128957,#128958,#128959,#128960,#128961,#128962,#128963,#128964,
#128965,#128966,#128967,#128968,#128969,#128970,#128971,#128972,#128973,
#128974,#128975,#128976,#128977,#128978,#128979,#128980,#128981,#128982,
#128983,#128984,#128985,#128986,#128987,#128988,#128989,#128990,#128991,
#128992,#128993,#128994,#128995,#128996,#128997,#128998,#128999,#129000,
#129001,#129002,#129003,#129004,#129005,#129006,#129007),.UNSPECIFIED.,
 .F.,.F.)
B_SPLINE_CURVE_WITH_KNOTS((6,1,1,1,1,1,1,1,1,1,1,1,1,1,1,1,1,1,1,1,1,1,
1,1,1,1,1,1,1,1,1,1,1,1,1,1,1,1,1,1,1,1,1,1,1,1,1,1,1,1,1,1,1,1,1,1,1,1,
1,1,1,1,1,1,1,1,1,1,1,1,1,1,1,1,1,1,1,1,1,1,1,1,1,1,1,1,1,1,1,1,1,1,1,1,
1,1,1,1,1,1,1,1,1,1,1,1,1,1,1,1,1,1,1,1,1,1,1,1,1,1,1,1,1,1,1,1,1,1,1,1,
1,1,1,1,1,1,1,1,1,1,1,1,1,1,1,1,1,1,1,1,1,1,1,1,1,1,1,1,1,1,1,1,1,1,1,1,
1,1,1,1,1,1,1,1,1,1,1,1,1,1,1,1,1,1,1,1,1,1,1,6),(-0.941429844438076,-0.940000000000001,
-0.935000000000001,-0.930000000000001,-0.925000000000001,-0.920000000000001,
-0.915000000000001,-0.910000000000001,-0.905000000000001,-0.900000000000001,
-0.895000000000001,-0.890000000000001,-0.885000000000001,-0.880000000000001,
-0.875000000000001,-0.870000000000001,-0.865000000000001,-0.860000000000001,
-0.855000000000001,-0.850000000000001,-0.845000000000001,-0.840000000000001,
-0.835000000000001,-0.830000000000001,-0.825000000000001,-0.820000000000001,
-0.815000000000001,-0.810000000000001,-0.805000000000001,-0.800000000000001,
-0.795000000000001,-0.790000000000001,-0.785000000000001,-0.780000000000001,
-0.775000000000001,-0.770000000000001,-0.765000000000001,-0.760000000000001,
-0.755000000000001,-0.750000000000001,-0.745000000000001,-0.740000000000001,
-0.735000000000001,-0.730000000000001,-0.725000000000001,-0.720000000000001,
-0.715000000000001,-0.710000000000001,-0.705000000000001,-0.700000000000001,
-0.695000000000001,-0.690000000000001,-0.685,-0.68,-0.675,-0.67,-0.665,
-0.66,-0.655,-0.65,-0.645,-0.64,-0.635,-0.63,-0.625,-0.62,-0.615,-0.61,
-0.605,-0.6,-0.595,-0.59,-0.585,-0.58,-0.575,-0.57,-0.565,-0.56,-0.555,
-0.55,-0.545,-0.54,-0.535,-0.53,-0.525,-0.52,-0.515,-0.51,-0.505,-0.5,-0.495,
-0.49,-0.485,-0.48,-0.475,-0.47,-0.465,-0.46,-0.455,-0.45,-0.445,-0.44,
-0.435,-0.43,-0.425,-0.42,-0.415,-0.41,-0.405,-0.4,-0.395,-0.39,-0.385,
-0.38,-0.375,-0.37,-0.365,-0.36,-0.355,-0.35,-0.345,-0.34,-0.335,-0.33,
-0.325,-0.32,-0.315,-0.31,-0.305,-0.3,-0.295,-0.29,-0.285,-0.28,-0.275,
-0.27,-0.265,-0.26,-0.255,-0.25,-0.245,-0.24,-0.235,-0.23,-0.225,-0.22,
-0.215,-0.21,-0.205,-0.2,-0.195,-0.19,-0.185,-0.18,-0.175,-0.17,-0.165,
-0.16,-0.155,-0.15,-0.145,-0.14,-0.135,-0.13,-0.125,-0.12,-0.115,-0.11,
-0.105,-0.1,-0.095,-0.09,-0.085,-0.08,-0.075,-0.07,-0.065,-0.06,-0.055,
-0.05,-0.045,-0.04,-0.035,-0.03,-0.025,-0.02,-0.015,-0.01,-0.005,0.),
 .UNSPECIFIED.)
CURVE()
GEOMETRIC_REPRESENTATION_ITEM()
RATIONAL_B_SPLINE_CURVE((1.,1.,1.,1.,1.,1.,1.,1.,1.,1.,1.,1.,1.,1.,1.,1.,
1.,1.,1.,1.,1.,1.,1.,1.,1.,1.,1.,1.,1.,1.,1.,1.,1.,1.,1.,1.,1.,1.,1.,1.,
1.,1.,1.,1.,1.,1.,1.,1.,1.,1.,1.,1.,1.,1.,1.,1.,1.,1.,1.,1.,1.,1.,1.,1.,
1.,1.,1.,1.,1.,1.,1.,1.,1.,1.,1.,1.,1.,1.,1.,1.,1.,1.,1.,1.,1.,1.,1.,1.,
1.,1.,1.,1.,1.,1.,1.,1.,1.,1.,1.,1.,1.,1.,1.,1.,1.,1.,1.,1.,1.,1.,1.,1.,
1.,1.,1.,1.,1.,1.,1.,1.,1.,1.,1.,1.,1.,1.,1.,1.,1.,1.,1.,1.,1.,1.,1.,1.,
1.,1.,1.,1.,1.,1.,1.,1.,1.,1.,1.,1.,1.,1.,1.,1.,1.,1.,1.,1.,1.,1.,1.,1.,
1.,1.,1.,1.,1.,1.,1.,1.,1.,1.,1.,1.,1.,1.,1.,1.,1.,1.,1.,1.,1.,1.,1.,1.,
1.,1.,1.,1.,1.,1.,1.,1.,1.,1.))
REPRESENTATION_ITEM('')
);
#577=(
BOUNDED_CURVE()
B_SPLINE_CURVE(5,(#129419,#129420,#129421,#129422,#129423,#129424,#129425,
#129426,#129427,#129428,#129429,#129430,#129431,#129432,#129433,#129434,
#129435,#129436,#129437,#129438,#129439,#129440,#129441,#129442,#129443,
#129444,#129445,#129446,#129447,#129448,#129449,#129450,#129451,#129452,
#129453,#129454,#129455,#129456,#129457,#129458,#129459,#129460,#129461,
#129462,#129463,#129464,#129465,#129466,#129467,#129468,#129469,#129470,
#129471,#129472,#129473,#129474,#129475,#129476,#129477,#129478,#129479,
#129480,#129481,#129482,#129483,#129484,#129485,#129486,#129487,#129488,
#129489,#129490,#129491,#129492,#129493,#129494,#129495,#129496,#129497,
#129498,#129499,#129500,#129501,#129502,#129503,#129504,#129505,#129506,
#129507,#129508,#129509,#129510,#129511,#129512,#129513,#129514,#129515,
#129516,#129517,#129518,#129519,#129520,#129521,#129522,#129523,#129524,
#129525,#129526,#129527,#129528,#129529,#129530,#129531,#129532,#129533,
#129534,#129535,#129536,#129537,#129538,#129539,#129540,#129541,#129542,
#129543,#129544,#129545,#129546,#129547,#129548,#129549,#129550,#129551,
#129552,#129553,#129554,#129555,#129556,#129557,#129558,#129559,#129560,
#129561,#129562,#129563,#129564,#129565,#129566,#129567,#129568,#129569,
#129570,#129571,#129572,#129573,#129574,#129575,#129576,#129577,#129578,
#129579,#129580,#129581,#129582,#129583,#129584,#129585,#129586,#129587,
#129588,#129589,#129590,#129591,#129592,#129593,#129594,#129595,#129596,
#129597,#129598,#129599,#129600,#129601,#129602,#129603,#129604,#129605,
#129606,#129607,#129608,#129609,#129610,#129611,#129612),.UNSPECIFIED.,
 .F.,.F.)
B_SPLINE_CURVE_WITH_KNOTS((6,1,1,1,1,1,1,1,1,1,1,1,1,1,1,1,1,1,1,1,1,1,
1,1,1,1,1,1,1,1,1,1,1,1,1,1,1,1,1,1,1,1,1,1,1,1,1,1,1,1,1,1,1,1,1,1,1,1,
1,1,1,1,1,1,1,1,1,1,1,1,1,1,1,1,1,1,1,1,1,1,1,1,1,1,1,1,1,1,1,1,1,1,1,1,
1,1,1,1,1,1,1,1,1,1,1,1,1,1,1,1,1,1,1,1,1,1,1,1,1,1,1,1,1,1,1,1,1,1,1,1,
1,1,1,1,1,1,1,1,1,1,1,1,1,1,1,1,1,1,1,1,1,1,1,1,1,1,1,1,1,1,1,1,1,1,1,1,
1,1,1,1,1,1,1,1,1,1,1,1,1,1,1,1,1,1,1,1,1,1,1,6),(0.,0.005,0.01,0.015,0.02,
0.025,0.03,0.035,0.04,0.045,0.05,0.055,0.06,0.065,0.07,0.075,0.08,0.085,
0.09,0.095,0.1,0.105,0.11,0.115,0.12,0.125,0.13,0.135,0.14,0.145,0.15,0.155,
0.16,0.165,0.17,0.175,0.18,0.185,0.19,0.195,0.2,0.205,0.21,0.215,0.22,0.225,
0.23,0.235,0.24,0.245,0.25,0.255,0.26,0.265,0.27,0.275,0.28,0.285,0.29,
0.295,0.3,0.305,0.31,0.315,0.32,0.325,0.33,0.335,0.34,0.345,0.35,0.355,
0.36,0.365,0.37,0.375,0.38,0.385,0.39,0.395,0.4,0.405,0.41,0.415,0.42,0.425,
0.43,0.435,0.44,0.445,0.45,0.455,0.46,0.465,0.47,0.475,0.48,0.485,0.49,
0.495,0.5,0.505,0.51,0.515,0.52,0.525,0.53,0.535,0.54,0.545,0.55,0.555,
0.56,0.565,0.57,0.575,0.58,0.585,0.59,0.595,0.6,0.605,0.61,0.615,0.62,0.625,
0.63,0.635,0.64,0.645,0.65,0.655,0.66,0.665,0.67,0.675,0.68,0.685,0.690000000000001,
0.695000000000001,0.700000000000001,0.705000000000001,0.710000000000001,
0.715000000000001,0.720000000000001,0.725000000000001,0.730000000000001,
0.735000000000001,0.740000000000001,0.745000000000001,0.750000000000001,
0.755000000000001,0.760000000000001,0.765000000000001,0.770000000000001,
0.775000000000001,0.780000000000001,0.785000000000001,0.790000000000001,
0.795000000000001,0.800000000000001,0.805000000000001,0.810000000000001,
0.815000000000001,0.820000000000001,0.825000000000001,0.830000000000001,
0.835000000000001,0.840000000000001,0.845000000000001,0.850000000000001,
0.855000000000001,0.860000000000001,0.865000000000001,0.870000000000001,
0.875000000000001,0.880000000000001,0.885000000000001,0.890000000000001,
0.895000000000001,0.900000000000001,0.905000000000001,0.910000000000001,
0.915000000000001,0.920000000000001,0.925000000000001,0.930000000000001,
0.935000000000001,0.940000000000001,0.941429844438015),.UNSPECIFIED.)
CURVE()
GEOMETRIC_REPRESENTATION_ITEM()
RATIONAL_B_SPLINE_CURVE((1.,1.,1.,1.,1.,1.,1.,1.,1.,1.,1.,1.,1.,1.,1.,1.,
1.,1.,1.,1.,1.,1.,1.,1.,1.,1.,1.,1.,1.,1.,1.,1.,1.,1.,1.,1.,1.,1.,1.,1.,
1.,1.,1.,1.,1.,1.,1.,1.,1.,1.,1.,1.,1.,1.,1.,1.,1.,1.,1.,1.,1.,1.,1.,1.,
1.,1.,1.,1.,1.,1.,1.,1.,1.,1.,1.,1.,1.,1.,1.,1.,1.,1.,1.,1.,1.,1.,1.,1.,
1.,1.,1.,1.,1.,1.,1.,1.,1.,1.,1.,1.,1.,1.,1.,1.,1.,1.,1.,1.,1.,1.,1.,1.,
1.,1.,1.,1.,1.,1.,1.,1.,1.,1.,1.,1.,1.,1.,1.,1.,1.,1.,1.,1.,1.,1.,1.,1.,
1.,1.,1.,1.,1.,1.,1.,1.,1.,1.,1.,1.,1.,1.,1.,1.,1.,1.,1.,1.,1.,1.,1.,1.,
1.,1.,1.,1.,1.,1.,1.,1.,1.,1.,1.,1.,1.,1.,1.,1.,1.,1.,1.,1.,1.,1.,1.,1.,
1.,1.,1.,1.,1.,1.,1.,1.,1.,1.))
REPRESENTATION_ITEM('')
);
#578=(
BOUNDED_CURVE()
B_SPLINE_CURVE(5,(#129615,#129616,#129617,#129618,#129619,#129620,#129621,
#129622,#129623,#129624,#129625,#129626,#129627,#129628,#129629,#129630,
#129631,#129632,#129633,#129634,#129635,#129636,#129637,#129638,#129639,
#129640,#129641,#129642,#129643,#129644,#129645,#129646,#129647,#129648,
#129649,#129650,#129651,#129652,#129653,#129654,#129655,#129656,#129657,
#129658,#129659,#129660,#129661,#129662,#129663,#129664,#129665,#129666,
#129667,#129668,#129669,#129670,#129671,#129672,#129673,#129674,#129675,
#129676,#129677,#129678,#129679,#129680,#129681,#129682,#129683,#129684,
#129685,#129686,#129687,#129688,#129689,#129690,#129691,#129692,#129693,
#129694,#129695,#129696,#129697,#129698,#129699,#129700,#129701,#129702,
#129703,#129704,#129705,#129706,#129707,#129708,#129709,#129710,#129711,
#129712,#129713,#129714,#129715,#129716,#129717,#129718,#129719,#129720,
#129721,#129722,#129723,#129724,#129725,#129726,#129727,#129728,#129729,
#129730,#129731,#129732,#129733,#129734,#129735,#129736,#129737,#129738,
#129739,#129740,#129741,#129742,#129743,#129744,#129745,#129746,#129747,
#129748,#129749,#129750,#129751,#129752,#129753,#129754,#129755,#129756,
#129757,#129758,#129759,#129760,#129761,#129762,#129763,#129764,#129765,
#129766,#129767,#129768,#129769,#129770,#129771,#129772,#129773,#129774,
#129775,#129776,#129777,#129778,#129779,#129780,#129781,#129782,#129783,
#129784,#129785,#129786,#129787,#129788,#129789,#129790,#129791,#129792,
#129793,#129794,#129795,#129796,#129797,#129798,#129799,#129800,#129801,
#129802,#129803,#129804,#129805,#129806,#129807,#129808),.UNSPECIFIED.,
 .F.,.F.)
B_SPLINE_CURVE_WITH_KNOTS((6,1,1,1,1,1,1,1,1,1,1,1,1,1,1,1,1,1,1,1,1,1,
1,1,1,1,1,1,1,1,1,1,1,1,1,1,1,1,1,1,1,1,1,1,1,1,1,1,1,1,1,1,1,1,1,1,1,1,
1,1,1,1,1,1,1,1,1,1,1,1,1,1,1,1,1,1,1,1,1,1,1,1,1,1,1,1,1,1,1,1,1,1,1,1,
1,1,1,1,1,1,1,1,1,1,1,1,1,1,1,1,1,1,1,1,1,1,1,1,1,1,1,1,1,1,1,1,1,1,1,1,
1,1,1,1,1,1,1,1,1,1,1,1,1,1,1,1,1,1,1,1,1,1,1,1,1,1,1,1,1,1,1,1,1,1,1,1,
1,1,1,1,1,1,1,1,1,1,1,1,1,1,1,1,1,1,1,1,1,1,1,6),(-0.94142984443801,-0.940000000000001,
-0.935000000000001,-0.930000000000001,-0.925000000000001,-0.920000000000001,
-0.915000000000001,-0.910000000000001,-0.905000000000001,-0.900000000000001,
-0.895000000000001,-0.890000000000001,-0.885000000000001,-0.880000000000001,
-0.875000000000001,-0.870000000000001,-0.865000000000001,-0.860000000000001,
-0.855000000000001,-0.850000000000001,-0.845000000000001,-0.840000000000001,
-0.835000000000001,-0.830000000000001,-0.825000000000001,-0.820000000000001,
-0.815000000000001,-0.810000000000001,-0.805000000000001,-0.800000000000001,
-0.795000000000001,-0.790000000000001,-0.785000000000001,-0.780000000000001,
-0.775000000000001,-0.770000000000001,-0.765000000000001,-0.760000000000001,
-0.755000000000001,-0.750000000000001,-0.745000000000001,-0.740000000000001,
-0.735000000000001,-0.730000000000001,-0.725000000000001,-0.720000000000001,
-0.715000000000001,-0.710000000000001,-0.705000000000001,-0.700000000000001,
-0.695000000000001,-0.690000000000001,-0.685,-0.68,-0.675,-0.67,-0.665,
-0.66,-0.655,-0.65,-0.645,-0.64,-0.635,-0.63,-0.625,-0.62,-0.615,-0.61,
-0.605,-0.6,-0.595,-0.59,-0.585,-0.58,-0.575,-0.57,-0.565,-0.56,-0.555,
-0.55,-0.545,-0.54,-0.535,-0.53,-0.525,-0.52,-0.515,-0.51,-0.505,-0.5,-0.495,
-0.49,-0.485,-0.48,-0.475,-0.47,-0.465,-0.46,-0.455,-0.45,-0.445,-0.44,
-0.435,-0.43,-0.425,-0.42,-0.415,-0.41,-0.405,-0.4,-0.395,-0.39,-0.385,
-0.38,-0.375,-0.37,-0.365,-0.36,-0.355,-0.35,-0.345,-0.34,-0.335,-0.33,
-0.325,-0.32,-0.315,-0.31,-0.305,-0.3,-0.295,-0.29,-0.285,-0.28,-0.275,
-0.27,-0.265,-0.26,-0.255,-0.25,-0.245,-0.24,-0.235,-0.23,-0.225,-0.22,
-0.215,-0.21,-0.205,-0.2,-0.195,-0.19,-0.185,-0.18,-0.175,-0.17,-0.165,
-0.16,-0.155,-0.15,-0.145,-0.14,-0.135,-0.13,-0.125,-0.12,-0.115,-0.11,
-0.105,-0.1,-0.095,-0.09,-0.085,-0.08,-0.075,-0.07,-0.065,-0.06,-0.055,
-0.05,-0.045,-0.04,-0.035,-0.03,-0.025,-0.02,-0.015,-0.01,-0.005,0.),
 .UNSPECIFIED.)
CURVE()
GEOMETRIC_REPRESENTATION_ITEM()
RATIONAL_B_SPLINE_CURVE((1.,1.,1.,1.,1.,1.,1.,1.,1.,1.,1.,1.,1.,1.,1.,1.,
1.,1.,1.,1.,1.,1.,1.,1.,1.,1.,1.,1.,1.,1.,1.,1.,1.,1.,1.,1.,1.,1.,1.,1.,
1.,1.,1.,1.,1.,1.,1.,1.,1.,1.,1.,1.,1.,1.,1.,1.,1.,1.,1.,1.,1.,1.,1.,1.,
1.,1.,1.,1.,1.,1.,1.,1.,1.,1.,1.,1.,1.,1.,1.,1.,1.,1.,1.,1.,1.,1.,1.,1.,
1.,1.,1.,1.,1.,1.,1.,1.,1.,1.,1.,1.,1.,1.,1.,1.,1.,1.,1.,1.,1.,1.,1.,1.,
1.,1.,1.,1.,1.,1.,1.,1.,1.,1.,1.,1.,1.,1.,1.,1.,1.,1.,1.,1.,1.,1.,1.,1.,
1.,1.,1.,1.,1.,1.,1.,1.,1.,1.,1.,1.,1.,1.,1.,1.,1.,1.,1.,1.,1.,1.,1.,1.,
1.,1.,1.,1.,1.,1.,1.,1.,1.,1.,1.,1.,1.,1.,1.,1.,1.,1.,1.,1.,1.,1.,1.,1.,
1.,1.,1.,1.,1.,1.,1.,1.,1.,1.))
REPRESENTATION_ITEM('')
);
#579=(
BOUNDED_CURVE()
B_SPLINE_CURVE(5,(#130220,#130221,#130222,#130223,#130224,#130225,#130226,
#130227,#130228,#130229,#130230,#130231,#130232,#130233,#130234,#130235,
#130236,#130237,#130238,#130239,#130240,#130241,#130242,#130243,#130244,
#130245,#130246,#130247,#130248,#130249,#130250,#130251,#130252,#130253,
#130254,#130255,#130256,#130257,#130258,#130259,#130260,#130261,#130262,
#130263,#130264,#130265,#130266,#130267,#130268,#130269,#130270,#130271,
#130272,#130273,#130274,#130275,#130276,#130277,#130278,#130279,#130280,
#130281,#130282,#130283,#130284,#130285,#130286,#130287,#130288,#130289,
#130290,#130291,#130292,#130293,#130294,#130295,#130296,#130297,#130298,
#130299,#130300,#130301,#130302,#130303,#130304,#130305,#130306,#130307,
#130308,#130309,#130310,#130311,#130312,#130313,#130314,#130315,#130316,
#130317,#130318,#130319,#130320,#130321,#130322,#130323,#130324,#130325,
#130326,#130327,#130328,#130329,#130330,#130331,#130332,#130333,#130334,
#130335,#130336,#130337,#130338,#130339,#130340,#130341,#130342,#130343,
#130344,#130345,#130346,#130347,#130348,#130349,#130350,#130351,#130352,
#130353,#130354,#130355,#130356,#130357,#130358,#130359,#130360,#130361,
#130362,#130363,#130364,#130365,#130366,#130367,#130368,#130369,#130370,
#130371,#130372,#130373,#130374,#130375,#130376,#130377,#130378,#130379,
#130380,#130381,#130382,#130383,#130384,#130385,#130386,#130387,#130388,
#130389,#130390,#130391,#130392,#130393,#130394,#130395,#130396,#130397,
#130398,#130399,#130400,#130401,#130402,#130403,#130404,#130405,#130406,
#130407,#130408,#130409,#130410,#130411,#130412,#130413),.UNSPECIFIED.,
 .F.,.F.)
B_SPLINE_CURVE_WITH_KNOTS((6,1,1,1,1,1,1,1,1,1,1,1,1,1,1,1,1,1,1,1,1,1,
1,1,1,1,1,1,1,1,1,1,1,1,1,1,1,1,1,1,1,1,1,1,1,1,1,1,1,1,1,1,1,1,1,1,1,1,
1,1,1,1,1,1,1,1,1,1,1,1,1,1,1,1,1,1,1,1,1,1,1,1,1,1,1,1,1,1,1,1,1,1,1,1,
1,1,1,1,1,1,1,1,1,1,1,1,1,1,1,1,1,1,1,1,1,1,1,1,1,1,1,1,1,1,1,1,1,1,1,1,
1,1,1,1,1,1,1,1,1,1,1,1,1,1,1,1,1,1,1,1,1,1,1,1,1,1,1,1,1,1,1,1,1,1,1,1,
1,1,1,1,1,1,1,1,1,1,1,1,1,1,1,1,1,1,1,1,1,1,1,6),(0.,0.005,0.01,0.015,0.02,
0.025,0.03,0.035,0.04,0.045,0.05,0.055,0.06,0.065,0.07,0.075,0.08,0.085,
0.09,0.095,0.1,0.105,0.11,0.115,0.12,0.125,0.13,0.135,0.14,0.145,0.15,0.155,
0.16,0.165,0.17,0.175,0.18,0.185,0.19,0.195,0.2,0.205,0.21,0.215,0.22,0.225,
0.23,0.235,0.24,0.245,0.25,0.255,0.26,0.265,0.27,0.275,0.28,0.285,0.29,
0.295,0.3,0.305,0.31,0.315,0.32,0.325,0.33,0.335,0.34,0.345,0.35,0.355,
0.36,0.365,0.37,0.375,0.38,0.385,0.39,0.395,0.4,0.405,0.41,0.415,0.42,0.425,
0.43,0.435,0.44,0.445,0.45,0.455,0.46,0.465,0.47,0.475,0.48,0.485,0.49,
0.495,0.5,0.505,0.51,0.515,0.52,0.525,0.53,0.535,0.54,0.545,0.55,0.555,
0.56,0.565,0.57,0.575,0.58,0.585,0.59,0.595,0.6,0.605,0.61,0.615,0.62,0.625,
0.63,0.635,0.64,0.645,0.65,0.655,0.66,0.665,0.67,0.675,0.68,0.685,0.690000000000001,
0.695000000000001,0.700000000000001,0.705000000000001,0.710000000000001,
0.715000000000001,0.720000000000001,0.725000000000001,0.730000000000001,
0.735000000000001,0.740000000000001,0.745000000000001,0.750000000000001,
0.755000000000001,0.760000000000001,0.765000000000001,0.770000000000001,
0.775000000000001,0.780000000000001,0.785000000000001,0.790000000000001,
0.795000000000001,0.800000000000001,0.805000000000001,0.810000000000001,
0.815000000000001,0.820000000000001,0.825000000000001,0.830000000000001,
0.835000000000001,0.840000000000001,0.845000000000001,0.850000000000001,
0.855000000000001,0.860000000000001,0.865000000000001,0.870000000000001,
0.875000000000001,0.880000000000001,0.885000000000001,0.890000000000001,
0.895000000000001,0.900000000000001,0.905000000000001,0.910000000000001,
0.915000000000001,0.920000000000001,0.925000000000001,0.930000000000001,
0.935000000000001,0.940000000000001,0.941429844438042),.UNSPECIFIED.)
CURVE()
GEOMETRIC_REPRESENTATION_ITEM()
RATIONAL_B_SPLINE_CURVE((1.,1.,1.,1.,1.,1.,1.,1.,1.,1.,1.,1.,1.,1.,1.,1.,
1.,1.,1.,1.,1.,1.,1.,1.,1.,1.,1.,1.,1.,1.,1.,1.,1.,1.,1.,1.,1.,1.,1.,1.,
1.,1.,1.,1.,1.,1.,1.,1.,1.,1.,1.,1.,1.,1.,1.,1.,1.,1.,1.,1.,1.,1.,1.,1.,
1.,1.,1.,1.,1.,1.,1.,1.,1.,1.,1.,1.,1.,1.,1.,1.,1.,1.,1.,1.,1.,1.,1.,1.,
1.,1.,1.,1.,1.,1.,1.,1.,1.,1.,1.,1.,1.,1.,1.,1.,1.,1.,1.,1.,1.,1.,1.,1.,
1.,1.,1.,1.,1.,1.,1.,1.,1.,1.,1.,1.,1.,1.,1.,1.,1.,1.,1.,1.,1.,1.,1.,1.,
1.,1.,1.,1.,1.,1.,1.,1.,1.,1.,1.,1.,1.,1.,1.,1.,1.,1.,1.,1.,1.,1.,1.,1.,
1.,1.,1.,1.,1.,1.,1.,1.,1.,1.,1.,1.,1.,1.,1.,1.,1.,1.,1.,1.,1.,1.,1.,1.,
1.,1.,1.,1.,1.,1.,1.,1.,1.,1.))
REPRESENTATION_ITEM('')
);
#580=(
BOUNDED_CURVE()
B_SPLINE_CURVE(5,(#130416,#130417,#130418,#130419,#130420,#130421,#130422,
#130423,#130424,#130425,#130426,#130427,#130428,#130429,#130430,#130431,
#130432,#130433,#130434,#130435,#130436,#130437,#130438,#130439,#130440,
#130441,#130442,#130443,#130444,#130445,#130446,#130447,#130448,#130449,
#130450,#130451,#130452,#130453,#130454,#130455,#130456,#130457,#130458,
#130459,#130460,#130461,#130462,#130463,#130464,#130465,#130466,#130467,
#130468,#130469,#130470,#130471,#130472,#130473,#130474,#130475,#130476,
#130477,#130478,#130479,#130480,#130481,#130482,#130483,#130484,#130485,
#130486,#130487,#130488,#130489,#130490,#130491,#130492,#130493,#130494,
#130495,#130496,#130497,#130498,#130499,#130500,#130501,#130502,#130503,
#130504,#130505,#130506,#130507,#130508,#130509,#130510,#130511,#130512,
#130513,#130514,#130515,#130516,#130517,#130518,#130519,#130520,#130521,
#130522,#130523,#130524,#130525,#130526,#130527,#130528,#130529,#130530,
#130531,#130532,#130533,#130534,#130535,#130536,#130537,#130538,#130539,
#130540,#130541,#130542,#130543,#130544,#130545,#130546,#130547,#130548,
#130549,#130550,#130551,#130552,#130553,#130554,#130555,#130556,#130557,
#130558,#130559,#130560,#130561,#130562,#130563,#130564,#130565,#130566,
#130567,#130568,#130569,#130570,#130571,#130572,#130573,#130574,#130575,
#130576,#130577,#130578,#130579,#130580,#130581,#130582,#130583,#130584,
#130585,#130586,#130587,#130588,#130589,#130590,#130591,#130592,#130593,
#130594,#130595,#130596,#130597,#130598,#130599,#130600,#130601,#130602,
#130603,#130604,#130605,#130606,#130607,#130608,#130609),.UNSPECIFIED.,
 .F.,.F.)
B_SPLINE_CURVE_WITH_KNOTS((6,1,1,1,1,1,1,1,1,1,1,1,1,1,1,1,1,1,1,1,1,1,
1,1,1,1,1,1,1,1,1,1,1,1,1,1,1,1,1,1,1,1,1,1,1,1,1,1,1,1,1,1,1,1,1,1,1,1,
1,1,1,1,1,1,1,1,1,1,1,1,1,1,1,1,1,1,1,1,1,1,1,1,1,1,1,1,1,1,1,1,1,1,1,1,
1,1,1,1,1,1,1,1,1,1,1,1,1,1,1,1,1,1,1,1,1,1,1,1,1,1,1,1,1,1,1,1,1,1,1,1,
1,1,1,1,1,1,1,1,1,1,1,1,1,1,1,1,1,1,1,1,1,1,1,1,1,1,1,1,1,1,1,1,1,1,1,1,
1,1,1,1,1,1,1,1,1,1,1,1,1,1,1,1,1,1,1,1,1,1,1,6),(-0.941429844438034,-0.940000000000001,
-0.935000000000001,-0.930000000000001,-0.925000000000001,-0.920000000000001,
-0.915000000000001,-0.910000000000001,-0.905000000000001,-0.900000000000001,
-0.895000000000001,-0.890000000000001,-0.885000000000001,-0.880000000000001,
-0.875000000000001,-0.870000000000001,-0.865000000000001,-0.860000000000001,
-0.855000000000001,-0.850000000000001,-0.845000000000001,-0.840000000000001,
-0.835000000000001,-0.830000000000001,-0.825000000000001,-0.820000000000001,
-0.815000000000001,-0.810000000000001,-0.805000000000001,-0.800000000000001,
-0.795000000000001,-0.790000000000001,-0.785000000000001,-0.780000000000001,
-0.775000000000001,-0.770000000000001,-0.765000000000001,-0.760000000000001,
-0.755000000000001,-0.750000000000001,-0.745000000000001,-0.740000000000001,
-0.735000000000001,-0.730000000000001,-0.725000000000001,-0.720000000000001,
-0.715000000000001,-0.710000000000001,-0.705000000000001,-0.700000000000001,
-0.695000000000001,-0.690000000000001,-0.685,-0.68,-0.675,-0.67,-0.665,
-0.66,-0.655,-0.65,-0.645,-0.64,-0.635,-0.63,-0.625,-0.62,-0.615,-0.61,
-0.605,-0.6,-0.595,-0.59,-0.585,-0.58,-0.575,-0.57,-0.565,-0.56,-0.555,
-0.55,-0.545,-0.54,-0.535,-0.53,-0.525,-0.52,-0.515,-0.51,-0.505,-0.5,-0.495,
-0.49,-0.485,-0.48,-0.475,-0.47,-0.465,-0.46,-0.455,-0.45,-0.445,-0.44,
-0.435,-0.43,-0.425,-0.42,-0.415,-0.41,-0.405,-0.4,-0.395,-0.39,-0.385,
-0.38,-0.375,-0.37,-0.365,-0.36,-0.355,-0.35,-0.345,-0.34,-0.335,-0.33,
-0.325,-0.32,-0.315,-0.31,-0.305,-0.3,-0.295,-0.29,-0.285,-0.28,-0.275,
-0.27,-0.265,-0.26,-0.255,-0.25,-0.245,-0.24,-0.235,-0.23,-0.225,-0.22,
-0.215,-0.21,-0.205,-0.2,-0.195,-0.19,-0.185,-0.18,-0.175,-0.17,-0.165,
-0.16,-0.155,-0.15,-0.145,-0.14,-0.135,-0.13,-0.125,-0.12,-0.115,-0.11,
-0.105,-0.1,-0.095,-0.09,-0.085,-0.08,-0.075,-0.07,-0.065,-0.06,-0.055,
-0.05,-0.045,-0.04,-0.035,-0.03,-0.025,-0.02,-0.015,-0.01,-0.005,0.),
 .UNSPECIFIED.)
CURVE()
GEOMETRIC_REPRESENTATION_ITEM()
RATIONAL_B_SPLINE_CURVE((1.,1.,1.,1.,1.,1.,1.,1.,1.,1.,1.,1.,1.,1.,1.,1.,
1.,1.,1.,1.,1.,1.,1.,1.,1.,1.,1.,1.,1.,1.,1.,1.,1.,1.,1.,1.,1.,1.,1.,1.,
1.,1.,1.,1.,1.,1.,1.,1.,1.,1.,1.,1.,1.,1.,1.,1.,1.,1.,1.,1.,1.,1.,1.,1.,
1.,1.,1.,1.,1.,1.,1.,1.,1.,1.,1.,1.,1.,1.,1.,1.,1.,1.,1.,1.,1.,1.,1.,1.,
1.,1.,1.,1.,1.,1.,1.,1.,1.,1.,1.,1.,1.,1.,1.,1.,1.,1.,1.,1.,1.,1.,1.,1.,
1.,1.,1.,1.,1.,1.,1.,1.,1.,1.,1.,1.,1.,1.,1.,1.,1.,1.,1.,1.,1.,1.,1.,1.,
1.,1.,1.,1.,1.,1.,1.,1.,1.,1.,1.,1.,1.,1.,1.,1.,1.,1.,1.,1.,1.,1.,1.,1.,
1.,1.,1.,1.,1.,1.,1.,1.,1.,1.,1.,1.,1.,1.,1.,1.,1.,1.,1.,1.,1.,1.,1.,1.,
1.,1.,1.,1.,1.,1.,1.,1.,1.,1.))
REPRESENTATION_ITEM('')
);
#581=(
BOUNDED_CURVE()
B_SPLINE_CURVE(5,(#131021,#131022,#131023,#131024,#131025,#131026,#131027,
#131028,#131029,#131030,#131031,#131032,#131033,#131034,#131035,#131036,
#131037,#131038,#131039,#131040,#131041,#131042,#131043,#131044,#131045,
#131046,#131047,#131048,#131049,#131050,#131051,#131052,#131053,#131054,
#131055,#131056,#131057,#131058,#131059,#131060,#131061,#131062,#131063,
#131064,#131065,#131066,#131067,#131068,#131069,#131070,#131071,#131072,
#131073,#131074,#131075,#131076,#131077,#131078,#131079,#131080,#131081,
#131082,#131083,#131084,#131085,#131086,#131087,#131088,#131089,#131090,
#131091,#131092,#131093,#131094,#131095,#131096,#131097,#131098,#131099,
#131100,#131101,#131102,#131103,#131104,#131105,#131106,#131107,#131108,
#131109,#131110,#131111,#131112,#131113,#131114,#131115,#131116,#131117,
#131118,#131119,#131120,#131121,#131122,#131123,#131124,#131125,#131126,
#131127,#131128,#131129,#131130,#131131,#131132,#131133,#131134,#131135,
#131136,#131137,#131138,#131139,#131140,#131141,#131142,#131143,#131144,
#131145,#131146,#131147,#131148,#131149,#131150,#131151,#131152,#131153,
#131154,#131155,#131156,#131157,#131158,#131159,#131160,#131161,#131162,
#131163,#131164,#131165,#131166,#131167,#131168,#131169,#131170,#131171,
#131172,#131173,#131174,#131175,#131176,#131177,#131178,#131179,#131180,
#131181,#131182,#131183,#131184,#131185,#131186,#131187,#131188,#131189,
#131190,#131191,#131192,#131193,#131194,#131195,#131196,#131197,#131198,
#131199,#131200,#131201,#131202,#131203,#131204,#131205,#131206,#131207,
#131208,#131209,#131210,#131211,#131212,#131213,#131214),.UNSPECIFIED.,
 .F.,.F.)
B_SPLINE_CURVE_WITH_KNOTS((6,1,1,1,1,1,1,1,1,1,1,1,1,1,1,1,1,1,1,1,1,1,
1,1,1,1,1,1,1,1,1,1,1,1,1,1,1,1,1,1,1,1,1,1,1,1,1,1,1,1,1,1,1,1,1,1,1,1,
1,1,1,1,1,1,1,1,1,1,1,1,1,1,1,1,1,1,1,1,1,1,1,1,1,1,1,1,1,1,1,1,1,1,1,1,
1,1,1,1,1,1,1,1,1,1,1,1,1,1,1,1,1,1,1,1,1,1,1,1,1,1,1,1,1,1,1,1,1,1,1,1,
1,1,1,1,1,1,1,1,1,1,1,1,1,1,1,1,1,1,1,1,1,1,1,1,1,1,1,1,1,1,1,1,1,1,1,1,
1,1,1,1,1,1,1,1,1,1,1,1,1,1,1,1,1,1,1,1,1,1,1,6),(0.,0.005,0.01,0.015,0.02,
0.025,0.03,0.035,0.04,0.045,0.05,0.055,0.06,0.065,0.07,0.075,0.08,0.085,
0.09,0.095,0.1,0.105,0.11,0.115,0.12,0.125,0.13,0.135,0.14,0.145,0.15,0.155,
0.16,0.165,0.17,0.175,0.18,0.185,0.19,0.195,0.2,0.205,0.21,0.215,0.22,0.225,
0.23,0.235,0.24,0.245,0.25,0.255,0.26,0.265,0.27,0.275,0.28,0.285,0.29,
0.295,0.3,0.305,0.31,0.315,0.32,0.325,0.33,0.335,0.34,0.345,0.35,0.355,
0.36,0.365,0.37,0.375,0.38,0.385,0.39,0.395,0.4,0.405,0.41,0.415,0.42,0.425,
0.43,0.435,0.44,0.445,0.45,0.455,0.46,0.465,0.47,0.475,0.48,0.485,0.49,
0.495,0.5,0.505,0.51,0.515,0.52,0.525,0.53,0.535,0.54,0.545,0.55,0.555,
0.56,0.565,0.57,0.575,0.58,0.585,0.59,0.595,0.6,0.605,0.61,0.615,0.62,0.625,
0.63,0.635,0.64,0.645,0.65,0.655,0.66,0.665,0.67,0.675,0.68,0.685,0.690000000000001,
0.695000000000001,0.700000000000001,0.705000000000001,0.710000000000001,
0.715000000000001,0.720000000000001,0.725000000000001,0.730000000000001,
0.735000000000001,0.740000000000001,0.745000000000001,0.750000000000001,
0.755000000000001,0.760000000000001,0.765000000000001,0.770000000000001,
0.775000000000001,0.780000000000001,0.785000000000001,0.790000000000001,
0.795000000000001,0.800000000000001,0.805000000000001,0.810000000000001,
0.815000000000001,0.820000000000001,0.825000000000001,0.830000000000001,
0.835000000000001,0.840000000000001,0.845000000000001,0.850000000000001,
0.855000000000001,0.860000000000001,0.865000000000001,0.870000000000001,
0.875000000000001,0.880000000000001,0.885000000000001,0.890000000000001,
0.895000000000001,0.900000000000001,0.905000000000001,0.910000000000001,
0.915000000000001,0.920000000000001,0.925000000000001,0.930000000000001,
0.935000000000001,0.940000000000001,0.94142984443805),.UNSPECIFIED.)
CURVE()
GEOMETRIC_REPRESENTATION_ITEM()
RATIONAL_B_SPLINE_CURVE((1.,1.,1.,1.,1.,1.,1.,1.,1.,1.,1.,1.,1.,1.,1.,1.,
1.,1.,1.,1.,1.,1.,1.,1.,1.,1.,1.,1.,1.,1.,1.,1.,1.,1.,1.,1.,1.,1.,1.,1.,
1.,1.,1.,1.,1.,1.,1.,1.,1.,1.,1.,1.,1.,1.,1.,1.,1.,1.,1.,1.,1.,1.,1.,1.,
1.,1.,1.,1.,1.,1.,1.,1.,1.,1.,1.,1.,1.,1.,1.,1.,1.,1.,1.,1.,1.,1.,1.,1.,
1.,1.,1.,1.,1.,1.,1.,1.,1.,1.,1.,1.,1.,1.,1.,1.,1.,1.,1.,1.,1.,1.,1.,1.,
1.,1.,1.,1.,1.,1.,1.,1.,1.,1.,1.,1.,1.,1.,1.,1.,1.,1.,1.,1.,1.,1.,1.,1.,
1.,1.,1.,1.,1.,1.,1.,1.,1.,1.,1.,1.,1.,1.,1.,1.,1.,1.,1.,1.,1.,1.,1.,1.,
1.,1.,1.,1.,1.,1.,1.,1.,1.,1.,1.,1.,1.,1.,1.,1.,1.,1.,1.,1.,1.,1.,1.,1.,
1.,1.,1.,1.,1.,1.,1.,1.,1.,1.))
REPRESENTATION_ITEM('')
);
#582=(
BOUNDED_CURVE()
B_SPLINE_CURVE(5,(#131217,#131218,#131219,#131220,#131221,#131222,#131223,
#131224,#131225,#131226,#131227,#131228,#131229,#131230,#131231,#131232,
#131233,#131234,#131235,#131236,#131237,#131238,#131239,#131240,#131241,
#131242,#131243,#131244,#131245,#131246,#131247,#131248,#131249,#131250,
#131251,#131252,#131253,#131254,#131255,#131256,#131257,#131258,#131259,
#131260,#131261,#131262,#131263,#131264,#131265,#131266,#131267,#131268,
#131269,#131270,#131271,#131272,#131273,#131274,#131275,#131276,#131277,
#131278,#131279,#131280,#131281,#131282,#131283,#131284,#131285,#131286,
#131287,#131288,#131289,#131290,#131291,#131292,#131293,#131294,#131295,
#131296,#131297,#131298,#131299,#131300,#131301,#131302,#131303,#131304,
#131305,#131306,#131307,#131308,#131309,#131310,#131311,#131312,#131313,
#131314,#131315,#131316,#131317,#131318,#131319,#131320,#131321,#131322,
#131323,#131324,#131325,#131326,#131327,#131328,#131329,#131330,#131331,
#131332,#131333,#131334,#131335,#131336,#131337,#131338,#131339,#131340,
#131341,#131342,#131343,#131344,#131345,#131346,#131347,#131348,#131349,
#131350,#131351,#131352,#131353,#131354,#131355,#131356,#131357,#131358,
#131359,#131360,#131361,#131362,#131363,#131364,#131365,#131366,#131367,
#131368,#131369,#131370,#131371,#131372,#131373,#131374,#131375,#131376,
#131377,#131378,#131379,#131380,#131381,#131382,#131383,#131384,#131385,
#131386,#131387,#131388,#131389,#131390,#131391,#131392,#131393,#131394,
#131395,#131396,#131397,#131398,#131399,#131400,#131401,#131402,#131403,
#131404,#131405,#131406,#131407,#131408,#131409,#131410),.UNSPECIFIED.,
 .F.,.F.)
B_SPLINE_CURVE_WITH_KNOTS((6,1,1,1,1,1,1,1,1,1,1,1,1,1,1,1,1,1,1,1,1,1,
1,1,1,1,1,1,1,1,1,1,1,1,1,1,1,1,1,1,1,1,1,1,1,1,1,1,1,1,1,1,1,1,1,1,1,1,
1,1,1,1,1,1,1,1,1,1,1,1,1,1,1,1,1,1,1,1,1,1,1,1,1,1,1,1,1,1,1,1,1,1,1,1,
1,1,1,1,1,1,1,1,1,1,1,1,1,1,1,1,1,1,1,1,1,1,1,1,1,1,1,1,1,1,1,1,1,1,1,1,
1,1,1,1,1,1,1,1,1,1,1,1,1,1,1,1,1,1,1,1,1,1,1,1,1,1,1,1,1,1,1,1,1,1,1,1,
1,1,1,1,1,1,1,1,1,1,1,1,1,1,1,1,1,1,1,1,1,1,1,6),(-0.941429844438051,-0.940000000000001,
-0.935000000000001,-0.930000000000001,-0.925000000000001,-0.920000000000001,
-0.915000000000001,-0.910000000000001,-0.905000000000001,-0.900000000000001,
-0.895000000000001,-0.890000000000001,-0.885000000000001,-0.880000000000001,
-0.875000000000001,-0.870000000000001,-0.865000000000001,-0.860000000000001,
-0.855000000000001,-0.850000000000001,-0.845000000000001,-0.840000000000001,
-0.835000000000001,-0.830000000000001,-0.825000000000001,-0.820000000000001,
-0.815000000000001,-0.810000000000001,-0.805000000000001,-0.800000000000001,
-0.795000000000001,-0.790000000000001,-0.785000000000001,-0.780000000000001,
-0.775000000000001,-0.770000000000001,-0.765000000000001,-0.760000000000001,
-0.755000000000001,-0.750000000000001,-0.745000000000001,-0.740000000000001,
-0.735000000000001,-0.730000000000001,-0.725000000000001,-0.720000000000001,
-0.715000000000001,-0.710000000000001,-0.705000000000001,-0.700000000000001,
-0.695000000000001,-0.690000000000001,-0.685,-0.68,-0.675,-0.67,-0.665,
-0.66,-0.655,-0.65,-0.645,-0.64,-0.635,-0.63,-0.625,-0.62,-0.615,-0.61,
-0.605,-0.6,-0.595,-0.59,-0.585,-0.58,-0.575,-0.57,-0.565,-0.56,-0.555,
-0.55,-0.545,-0.54,-0.535,-0.53,-0.525,-0.52,-0.515,-0.51,-0.505,-0.5,-0.495,
-0.49,-0.485,-0.48,-0.475,-0.47,-0.465,-0.46,-0.455,-0.45,-0.445,-0.44,
-0.435,-0.43,-0.425,-0.42,-0.415,-0.41,-0.405,-0.4,-0.395,-0.39,-0.385,
-0.38,-0.375,-0.37,-0.365,-0.36,-0.355,-0.35,-0.345,-0.34,-0.335,-0.33,
-0.325,-0.32,-0.315,-0.31,-0.305,-0.3,-0.295,-0.29,-0.285,-0.28,-0.275,
-0.27,-0.265,-0.26,-0.255,-0.25,-0.245,-0.24,-0.235,-0.23,-0.225,-0.22,
-0.215,-0.21,-0.205,-0.2,-0.195,-0.19,-0.185,-0.18,-0.175,-0.17,-0.165,
-0.16,-0.155,-0.15,-0.145,-0.14,-0.135,-0.13,-0.125,-0.12,-0.115,-0.11,
-0.105,-0.1,-0.095,-0.09,-0.085,-0.08,-0.075,-0.07,-0.065,-0.06,-0.055,
-0.05,-0.045,-0.04,-0.035,-0.03,-0.025,-0.02,-0.015,-0.01,-0.005,0.),
 .UNSPECIFIED.)
CURVE()
GEOMETRIC_REPRESENTATION_ITEM()
RATIONAL_B_SPLINE_CURVE((1.,1.,1.,1.,1.,1.,1.,1.,1.,1.,1.,1.,1.,1.,1.,1.,
1.,1.,1.,1.,1.,1.,1.,1.,1.,1.,1.,1.,1.,1.,1.,1.,1.,1.,1.,1.,1.,1.,1.,1.,
1.,1.,1.,1.,1.,1.,1.,1.,1.,1.,1.,1.,1.,1.,1.,1.,1.,1.,1.,1.,1.,1.,1.,1.,
1.,1.,1.,1.,1.,1.,1.,1.,1.,1.,1.,1.,1.,1.,1.,1.,1.,1.,1.,1.,1.,1.,1.,1.,
1.,1.,1.,1.,1.,1.,1.,1.,1.,1.,1.,1.,1.,1.,1.,1.,1.,1.,1.,1.,1.,1.,1.,1.,
1.,1.,1.,1.,1.,1.,1.,1.,1.,1.,1.,1.,1.,1.,1.,1.,1.,1.,1.,1.,1.,1.,1.,1.,
1.,1.,1.,1.,1.,1.,1.,1.,1.,1.,1.,1.,1.,1.,1.,1.,1.,1.,1.,1.,1.,1.,1.,1.,
1.,1.,1.,1.,1.,1.,1.,1.,1.,1.,1.,1.,1.,1.,1.,1.,1.,1.,1.,1.,1.,1.,1.,1.,
1.,1.,1.,1.,1.,1.,1.,1.,1.,1.))
REPRESENTATION_ITEM('')
);
#583=(
BOUNDED_CURVE()
B_SPLINE_CURVE(5,(#131822,#131823,#131824,#131825,#131826,#131827,#131828,
#131829,#131830,#131831,#131832,#131833,#131834,#131835,#131836,#131837,
#131838,#131839,#131840,#131841,#131842,#131843,#131844,#131845,#131846,
#131847,#131848,#131849,#131850,#131851,#131852,#131853,#131854,#131855,
#131856,#131857,#131858,#131859,#131860,#131861,#131862,#131863,#131864,
#131865,#131866,#131867,#131868,#131869,#131870,#131871,#131872,#131873,
#131874,#131875,#131876,#131877,#131878,#131879,#131880,#131881,#131882,
#131883,#131884,#131885,#131886,#131887,#131888,#131889,#131890,#131891,
#131892,#131893,#131894,#131895,#131896,#131897,#131898,#131899,#131900,
#131901,#131902,#131903,#131904,#131905,#131906,#131907,#131908,#131909,
#131910,#131911,#131912,#131913,#131914,#131915,#131916,#131917,#131918,
#131919,#131920,#131921,#131922,#131923,#131924,#131925,#131926,#131927,
#131928,#131929,#131930,#131931,#131932,#131933,#131934,#131935,#131936,
#131937,#131938,#131939,#131940,#131941,#131942,#131943,#131944,#131945,
#131946,#131947,#131948,#131949,#131950,#131951,#131952,#131953,#131954,
#131955,#131956,#131957,#131958,#131959,#131960,#131961,#131962,#131963,
#131964,#131965,#131966,#131967,#131968,#131969,#131970,#131971,#131972,
#131973,#131974,#131975,#131976,#131977,#131978,#131979,#131980,#131981,
#131982,#131983,#131984,#131985,#131986,#131987,#131988,#131989,#131990,
#131991,#131992,#131993,#131994,#131995,#131996,#131997,#131998,#131999,
#132000,#132001,#132002,#132003,#132004,#132005,#132006,#132007,#132008,
#132009,#132010,#132011,#132012,#132013,#132014,#132015),.UNSPECIFIED.,
 .F.,.F.)
B_SPLINE_CURVE_WITH_KNOTS((6,1,1,1,1,1,1,1,1,1,1,1,1,1,1,1,1,1,1,1,1,1,
1,1,1,1,1,1,1,1,1,1,1,1,1,1,1,1,1,1,1,1,1,1,1,1,1,1,1,1,1,1,1,1,1,1,1,1,
1,1,1,1,1,1,1,1,1,1,1,1,1,1,1,1,1,1,1,1,1,1,1,1,1,1,1,1,1,1,1,1,1,1,1,1,
1,1,1,1,1,1,1,1,1,1,1,1,1,1,1,1,1,1,1,1,1,1,1,1,1,1,1,1,1,1,1,1,1,1,1,1,
1,1,1,1,1,1,1,1,1,1,1,1,1,1,1,1,1,1,1,1,1,1,1,1,1,1,1,1,1,1,1,1,1,1,1,1,
1,1,1,1,1,1,1,1,1,1,1,1,1,1,1,1,1,1,1,1,1,1,1,6),(0.,0.005,0.01,0.015,0.02,
0.025,0.03,0.035,0.04,0.045,0.05,0.055,0.06,0.065,0.07,0.075,0.08,0.085,
0.09,0.095,0.1,0.105,0.11,0.115,0.12,0.125,0.13,0.135,0.14,0.145,0.15,0.155,
0.16,0.165,0.17,0.175,0.18,0.185,0.19,0.195,0.2,0.205,0.21,0.215,0.22,0.225,
0.23,0.235,0.24,0.245,0.25,0.255,0.26,0.265,0.27,0.275,0.28,0.285,0.29,
0.295,0.3,0.305,0.31,0.315,0.32,0.325,0.33,0.335,0.34,0.345,0.35,0.355,
0.36,0.365,0.37,0.375,0.38,0.385,0.39,0.395,0.4,0.405,0.41,0.415,0.42,0.425,
0.43,0.435,0.44,0.445,0.45,0.455,0.46,0.465,0.47,0.475,0.48,0.485,0.49,
0.495,0.5,0.505,0.51,0.515,0.52,0.525,0.53,0.535,0.54,0.545,0.55,0.555,
0.56,0.565,0.57,0.575,0.58,0.585,0.59,0.595,0.6,0.605,0.61,0.615,0.62,0.625,
0.63,0.635,0.64,0.645,0.65,0.655,0.66,0.665,0.67,0.675,0.68,0.685,0.690000000000001,
0.695000000000001,0.700000000000001,0.705000000000001,0.710000000000001,
0.715000000000001,0.720000000000001,0.725000000000001,0.730000000000001,
0.735000000000001,0.740000000000001,0.745000000000001,0.750000000000001,
0.755000000000001,0.760000000000001,0.765000000000001,0.770000000000001,
0.775000000000001,0.780000000000001,0.785000000000001,0.790000000000001,
0.795000000000001,0.800000000000001,0.805000000000001,0.810000000000001,
0.815000000000001,0.820000000000001,0.825000000000001,0.830000000000001,
0.835000000000001,0.840000000000001,0.845000000000001,0.850000000000001,
0.855000000000001,0.860000000000001,0.865000000000001,0.870000000000001,
0.875000000000001,0.880000000000001,0.885000000000001,0.890000000000001,
0.895000000000001,0.900000000000001,0.905000000000001,0.910000000000001,
0.915000000000001,0.920000000000001,0.925000000000001,0.930000000000001,
0.935000000000001,0.940000000000001,0.941429844438123),.UNSPECIFIED.)
CURVE()
GEOMETRIC_REPRESENTATION_ITEM()
RATIONAL_B_SPLINE_CURVE((1.,1.,1.,1.,1.,1.,1.,1.,1.,1.,1.,1.,1.,1.,1.,1.,
1.,1.,1.,1.,1.,1.,1.,1.,1.,1.,1.,1.,1.,1.,1.,1.,1.,1.,1.,1.,1.,1.,1.,1.,
1.,1.,1.,1.,1.,1.,1.,1.,1.,1.,1.,1.,1.,1.,1.,1.,1.,1.,1.,1.,1.,1.,1.,1.,
1.,1.,1.,1.,1.,1.,1.,1.,1.,1.,1.,1.,1.,1.,1.,1.,1.,1.,1.,1.,1.,1.,1.,1.,
1.,1.,1.,1.,1.,1.,1.,1.,1.,1.,1.,1.,1.,1.,1.,1.,1.,1.,1.,1.,1.,1.,1.,1.,
1.,1.,1.,1.,1.,1.,1.,1.,1.,1.,1.,1.,1.,1.,1.,1.,1.,1.,1.,1.,1.,1.,1.,1.,
1.,1.,1.,1.,1.,1.,1.,1.,1.,1.,1.,1.,1.,1.,1.,1.,1.,1.,1.,1.,1.,1.,1.,1.,
1.,1.,1.,1.,1.,1.,1.,1.,1.,1.,1.,1.,1.,1.,1.,1.,1.,1.,1.,1.,1.,1.,1.,1.,
1.,1.,1.,1.,1.,1.,1.,1.,1.,1.))
REPRESENTATION_ITEM('')
);
#584=(
BOUNDED_CURVE()
B_SPLINE_CURVE(5,(#132018,#132019,#132020,#132021,#132022,#132023,#132024,
#132025,#132026,#132027,#132028,#132029,#132030,#132031,#132032,#132033,
#132034,#132035,#132036,#132037,#132038,#132039,#132040,#132041,#132042,
#132043,#132044,#132045,#132046,#132047,#132048,#132049,#132050,#132051,
#132052,#132053,#132054,#132055,#132056,#132057,#132058,#132059,#132060,
#132061,#132062,#132063,#132064,#132065,#132066,#132067,#132068,#132069,
#132070,#132071,#132072,#132073,#132074,#132075,#132076,#132077,#132078,
#132079,#132080,#132081,#132082,#132083,#132084,#132085,#132086,#132087,
#132088,#132089,#132090,#132091,#132092,#132093,#132094,#132095,#132096,
#132097,#132098,#132099,#132100,#132101,#132102,#132103,#132104,#132105,
#132106,#132107,#132108,#132109,#132110,#132111,#132112,#132113,#132114,
#132115,#132116,#132117,#132118,#132119,#132120,#132121,#132122,#132123,
#132124,#132125,#132126,#132127,#132128,#132129,#132130,#132131,#132132,
#132133,#132134,#132135,#132136,#132137,#132138,#132139,#132140,#132141,
#132142,#132143,#132144,#132145,#132146,#132147,#132148,#132149,#132150,
#132151,#132152,#132153,#132154,#132155,#132156,#132157,#132158,#132159,
#132160,#132161,#132162,#132163,#132164,#132165,#132166,#132167,#132168,
#132169,#132170,#132171,#132172,#132173,#132174,#132175,#132176,#132177,
#132178,#132179,#132180,#132181,#132182,#132183,#132184,#132185,#132186,
#132187,#132188,#132189,#132190,#132191,#132192,#132193,#132194,#132195,
#132196,#132197,#132198,#132199,#132200,#132201,#132202,#132203,#132204,
#132205,#132206,#132207,#132208,#132209,#132210,#132211),.UNSPECIFIED.,
 .F.,.F.)
B_SPLINE_CURVE_WITH_KNOTS((6,1,1,1,1,1,1,1,1,1,1,1,1,1,1,1,1,1,1,1,1,1,
1,1,1,1,1,1,1,1,1,1,1,1,1,1,1,1,1,1,1,1,1,1,1,1,1,1,1,1,1,1,1,1,1,1,1,1,
1,1,1,1,1,1,1,1,1,1,1,1,1,1,1,1,1,1,1,1,1,1,1,1,1,1,1,1,1,1,1,1,1,1,1,1,
1,1,1,1,1,1,1,1,1,1,1,1,1,1,1,1,1,1,1,1,1,1,1,1,1,1,1,1,1,1,1,1,1,1,1,1,
1,1,1,1,1,1,1,1,1,1,1,1,1,1,1,1,1,1,1,1,1,1,1,1,1,1,1,1,1,1,1,1,1,1,1,1,
1,1,1,1,1,1,1,1,1,1,1,1,1,1,1,1,1,1,1,1,1,1,1,6),(-0.941429844438125,-0.940000000000001,
-0.935000000000001,-0.930000000000001,-0.925000000000001,-0.920000000000001,
-0.915000000000001,-0.910000000000001,-0.905000000000001,-0.900000000000001,
-0.895000000000001,-0.890000000000001,-0.885000000000001,-0.880000000000001,
-0.875000000000001,-0.870000000000001,-0.865000000000001,-0.860000000000001,
-0.855000000000001,-0.850000000000001,-0.845000000000001,-0.840000000000001,
-0.835000000000001,-0.830000000000001,-0.825000000000001,-0.820000000000001,
-0.815000000000001,-0.810000000000001,-0.805000000000001,-0.800000000000001,
-0.795000000000001,-0.790000000000001,-0.785000000000001,-0.780000000000001,
-0.775000000000001,-0.770000000000001,-0.765000000000001,-0.760000000000001,
-0.755000000000001,-0.750000000000001,-0.745000000000001,-0.740000000000001,
-0.735000000000001,-0.730000000000001,-0.725000000000001,-0.720000000000001,
-0.715000000000001,-0.710000000000001,-0.705000000000001,-0.700000000000001,
-0.695000000000001,-0.690000000000001,-0.685,-0.68,-0.675,-0.67,-0.665,
-0.66,-0.655,-0.65,-0.645,-0.64,-0.635,-0.63,-0.625,-0.62,-0.615,-0.61,
-0.605,-0.6,-0.595,-0.59,-0.585,-0.58,-0.575,-0.57,-0.565,-0.56,-0.555,
-0.55,-0.545,-0.54,-0.535,-0.53,-0.525,-0.52,-0.515,-0.51,-0.505,-0.5,-0.495,
-0.49,-0.485,-0.48,-0.475,-0.47,-0.465,-0.46,-0.455,-0.45,-0.445,-0.44,
-0.435,-0.43,-0.425,-0.42,-0.415,-0.41,-0.405,-0.4,-0.395,-0.39,-0.385,
-0.38,-0.375,-0.37,-0.365,-0.36,-0.355,-0.35,-0.345,-0.34,-0.335,-0.33,
-0.325,-0.32,-0.315,-0.31,-0.305,-0.3,-0.295,-0.29,-0.285,-0.28,-0.275,
-0.27,-0.265,-0.26,-0.255,-0.25,-0.245,-0.24,-0.235,-0.23,-0.225,-0.22,
-0.215,-0.21,-0.205,-0.2,-0.195,-0.19,-0.185,-0.18,-0.175,-0.17,-0.165,
-0.16,-0.155,-0.15,-0.145,-0.14,-0.135,-0.13,-0.125,-0.12,-0.115,-0.11,
-0.105,-0.1,-0.095,-0.09,-0.085,-0.08,-0.075,-0.07,-0.065,-0.06,-0.055,
-0.05,-0.045,-0.04,-0.035,-0.03,-0.025,-0.02,-0.015,-0.01,-0.005,0.),
 .UNSPECIFIED.)
CURVE()
GEOMETRIC_REPRESENTATION_ITEM()
RATIONAL_B_SPLINE_CURVE((1.,1.,1.,1.,1.,1.,1.,1.,1.,1.,1.,1.,1.,1.,1.,1.,
1.,1.,1.,1.,1.,1.,1.,1.,1.,1.,1.,1.,1.,1.,1.,1.,1.,1.,1.,1.,1.,1.,1.,1.,
1.,1.,1.,1.,1.,1.,1.,1.,1.,1.,1.,1.,1.,1.,1.,1.,1.,1.,1.,1.,1.,1.,1.,1.,
1.,1.,1.,1.,1.,1.,1.,1.,1.,1.,1.,1.,1.,1.,1.,1.,1.,1.,1.,1.,1.,1.,1.,1.,
1.,1.,1.,1.,1.,1.,1.,1.,1.,1.,1.,1.,1.,1.,1.,1.,1.,1.,1.,1.,1.,1.,1.,1.,
1.,1.,1.,1.,1.,1.,1.,1.,1.,1.,1.,1.,1.,1.,1.,1.,1.,1.,1.,1.,1.,1.,1.,1.,
1.,1.,1.,1.,1.,1.,1.,1.,1.,1.,1.,1.,1.,1.,1.,1.,1.,1.,1.,1.,1.,1.,1.,1.,
1.,1.,1.,1.,1.,1.,1.,1.,1.,1.,1.,1.,1.,1.,1.,1.,1.,1.,1.,1.,1.,1.,1.,1.,
1.,1.,1.,1.,1.,1.,1.,1.,1.,1.))
REPRESENTATION_ITEM('')
);
#585=(
BOUNDED_CURVE()
B_SPLINE_CURVE(5,(#132623,#132624,#132625,#132626,#132627,#132628,#132629,
#132630,#132631,#132632,#132633,#132634,#132635,#132636,#132637,#132638,
#132639,#132640,#132641,#132642,#132643,#132644,#132645,#132646,#132647,
#132648,#132649,#132650,#132651,#132652,#132653,#132654,#132655,#132656,
#132657,#132658,#132659,#132660,#132661,#132662,#132663,#132664,#132665,
#132666,#132667,#132668,#132669,#132670,#132671,#132672,#132673,#132674,
#132675,#132676,#132677,#132678,#132679,#132680,#132681,#132682,#132683,
#132684,#132685,#132686,#132687,#132688,#132689,#132690,#132691,#132692,
#132693,#132694,#132695,#132696,#132697,#132698,#132699,#132700,#132701,
#132702,#132703,#132704,#132705,#132706,#132707,#132708,#132709,#132710,
#132711,#132712,#132713,#132714,#132715,#132716,#132717,#132718,#132719,
#132720,#132721,#132722,#132723,#132724,#132725,#132726,#132727,#132728,
#132729,#132730,#132731,#132732,#132733,#132734,#132735,#132736,#132737,
#132738,#132739,#132740,#132741,#132742,#132743,#132744,#132745,#132746,
#132747,#132748,#132749,#132750,#132751,#132752,#132753,#132754,#132755,
#132756,#132757,#132758,#132759,#132760,#132761,#132762,#132763,#132764,
#132765,#132766,#132767,#132768,#132769,#132770,#132771,#132772,#132773,
#132774,#132775,#132776,#132777,#132778,#132779,#132780,#132781,#132782,
#132783,#132784,#132785,#132786,#132787,#132788,#132789,#132790,#132791,
#132792,#132793,#132794,#132795,#132796,#132797,#132798,#132799,#132800,
#132801,#132802,#132803,#132804,#132805,#132806,#132807,#132808,#132809,
#132810,#132811,#132812,#132813,#132814,#132815,#132816),.UNSPECIFIED.,
 .F.,.F.)
B_SPLINE_CURVE_WITH_KNOTS((6,1,1,1,1,1,1,1,1,1,1,1,1,1,1,1,1,1,1,1,1,1,
1,1,1,1,1,1,1,1,1,1,1,1,1,1,1,1,1,1,1,1,1,1,1,1,1,1,1,1,1,1,1,1,1,1,1,1,
1,1,1,1,1,1,1,1,1,1,1,1,1,1,1,1,1,1,1,1,1,1,1,1,1,1,1,1,1,1,1,1,1,1,1,1,
1,1,1,1,1,1,1,1,1,1,1,1,1,1,1,1,1,1,1,1,1,1,1,1,1,1,1,1,1,1,1,1,1,1,1,1,
1,1,1,1,1,1,1,1,1,1,1,1,1,1,1,1,1,1,1,1,1,1,1,1,1,1,1,1,1,1,1,1,1,1,1,1,
1,1,1,1,1,1,1,1,1,1,1,1,1,1,1,1,1,1,1,1,1,1,1,6),(0.,0.005,0.01,0.015,0.02,
0.025,0.03,0.035,0.04,0.045,0.05,0.055,0.06,0.065,0.07,0.075,0.08,0.085,
0.09,0.095,0.1,0.105,0.11,0.115,0.12,0.125,0.13,0.135,0.14,0.145,0.15,0.155,
0.16,0.165,0.17,0.175,0.18,0.185,0.19,0.195,0.2,0.205,0.21,0.215,0.22,0.225,
0.23,0.235,0.24,0.245,0.25,0.255,0.26,0.265,0.27,0.275,0.28,0.285,0.29,
0.295,0.3,0.305,0.31,0.315,0.32,0.325,0.33,0.335,0.34,0.345,0.35,0.355,
0.36,0.365,0.37,0.375,0.38,0.385,0.39,0.395,0.4,0.405,0.41,0.415,0.42,0.425,
0.43,0.435,0.44,0.445,0.45,0.455,0.46,0.465,0.47,0.475,0.48,0.485,0.49,
0.495,0.5,0.505,0.51,0.515,0.52,0.525,0.53,0.535,0.54,0.545,0.55,0.555,
0.56,0.565,0.57,0.575,0.58,0.585,0.59,0.595,0.6,0.605,0.61,0.615,0.62,0.625,
0.63,0.635,0.64,0.645,0.65,0.655,0.66,0.665,0.67,0.675,0.68,0.685,0.690000000000001,
0.695000000000001,0.700000000000001,0.705000000000001,0.710000000000001,
0.715000000000001,0.720000000000001,0.725000000000001,0.730000000000001,
0.735000000000001,0.740000000000001,0.745000000000001,0.750000000000001,
0.755000000000001,0.760000000000001,0.765000000000001,0.770000000000001,
0.775000000000001,0.780000000000001,0.785000000000001,0.790000000000001,
0.795000000000001,0.800000000000001,0.805000000000001,0.810000000000001,
0.815000000000001,0.820000000000001,0.825000000000001,0.830000000000001,
0.835000000000001,0.840000000000001,0.845000000000001,0.850000000000001,
0.855000000000001,0.860000000000001,0.865000000000001,0.870000000000001,
0.875000000000001,0.880000000000001,0.885000000000001,0.890000000000001,
0.895000000000001,0.900000000000001,0.905000000000001,0.910000000000001,
0.915000000000001,0.920000000000001,0.925000000000001,0.930000000000001,
0.935000000000001,0.940000000000001,0.941429844438013),.UNSPECIFIED.)
CURVE()
GEOMETRIC_REPRESENTATION_ITEM()
RATIONAL_B_SPLINE_CURVE((1.,1.,1.,1.,1.,1.,1.,1.,1.,1.,1.,1.,1.,1.,1.,1.,
1.,1.,1.,1.,1.,1.,1.,1.,1.,1.,1.,1.,1.,1.,1.,1.,1.,1.,1.,1.,1.,1.,1.,1.,
1.,1.,1.,1.,1.,1.,1.,1.,1.,1.,1.,1.,1.,1.,1.,1.,1.,1.,1.,1.,1.,1.,1.,1.,
1.,1.,1.,1.,1.,1.,1.,1.,1.,1.,1.,1.,1.,1.,1.,1.,1.,1.,1.,1.,1.,1.,1.,1.,
1.,1.,1.,1.,1.,1.,1.,1.,1.,1.,1.,1.,1.,1.,1.,1.,1.,1.,1.,1.,1.,1.,1.,1.,
1.,1.,1.,1.,1.,1.,1.,1.,1.,1.,1.,1.,1.,1.,1.,1.,1.,1.,1.,1.,1.,1.,1.,1.,
1.,1.,1.,1.,1.,1.,1.,1.,1.,1.,1.,1.,1.,1.,1.,1.,1.,1.,1.,1.,1.,1.,1.,1.,
1.,1.,1.,1.,1.,1.,1.,1.,1.,1.,1.,1.,1.,1.,1.,1.,1.,1.,1.,1.,1.,1.,1.,1.,
1.,1.,1.,1.,1.,1.,1.,1.,1.,1.))
REPRESENTATION_ITEM('')
);
#586=(
BOUNDED_CURVE()
B_SPLINE_CURVE(5,(#132819,#132820,#132821,#132822,#132823,#132824,#132825,
#132826,#132827,#132828,#132829,#132830,#132831,#132832,#132833,#132834,
#132835,#132836,#132837,#132838,#132839,#132840,#132841,#132842,#132843,
#132844,#132845,#132846,#132847,#132848,#132849,#132850,#132851,#132852,
#132853,#132854,#132855,#132856,#132857,#132858,#132859,#132860,#132861,
#132862,#132863,#132864,#132865,#132866,#132867,#132868,#132869,#132870,
#132871,#132872,#132873,#132874,#132875,#132876,#132877,#132878,#132879,
#132880,#132881,#132882,#132883,#132884,#132885,#132886,#132887,#132888,
#132889,#132890,#132891,#132892,#132893,#132894,#132895,#132896,#132897,
#132898,#132899,#132900,#132901,#132902,#132903,#132904,#132905,#132906,
#132907,#132908,#132909,#132910,#132911,#132912,#132913,#132914,#132915,
#132916,#132917,#132918,#132919,#132920,#132921,#132922,#132923,#132924,
#132925,#132926,#132927,#132928,#132929,#132930,#132931,#132932,#132933,
#132934,#132935,#132936,#132937,#132938,#132939,#132940,#132941,#132942,
#132943,#132944,#132945,#132946,#132947,#132948,#132949,#132950,#132951,
#132952,#132953,#132954,#132955,#132956,#132957,#132958,#132959,#132960,
#132961,#132962,#132963,#132964,#132965,#132966,#132967,#132968,#132969,
#132970,#132971,#132972,#132973,#132974,#132975,#132976,#132977,#132978,
#132979,#132980,#132981,#132982,#132983,#132984,#132985,#132986,#132987,
#132988,#132989,#132990,#132991,#132992,#132993,#132994,#132995,#132996,
#132997,#132998,#132999,#133000,#133001,#133002,#133003,#133004,#133005,
#133006,#133007,#133008,#133009,#133010,#133011,#133012),.UNSPECIFIED.,
 .F.,.F.)
B_SPLINE_CURVE_WITH_KNOTS((6,1,1,1,1,1,1,1,1,1,1,1,1,1,1,1,1,1,1,1,1,1,
1,1,1,1,1,1,1,1,1,1,1,1,1,1,1,1,1,1,1,1,1,1,1,1,1,1,1,1,1,1,1,1,1,1,1,1,
1,1,1,1,1,1,1,1,1,1,1,1,1,1,1,1,1,1,1,1,1,1,1,1,1,1,1,1,1,1,1,1,1,1,1,1,
1,1,1,1,1,1,1,1,1,1,1,1,1,1,1,1,1,1,1,1,1,1,1,1,1,1,1,1,1,1,1,1,1,1,1,1,
1,1,1,1,1,1,1,1,1,1,1,1,1,1,1,1,1,1,1,1,1,1,1,1,1,1,1,1,1,1,1,1,1,1,1,1,
1,1,1,1,1,1,1,1,1,1,1,1,1,1,1,1,1,1,1,1,1,1,1,6),(-0.941429844438012,-0.940000000000001,
-0.935000000000001,-0.930000000000001,-0.925000000000001,-0.920000000000001,
-0.915000000000001,-0.910000000000001,-0.905000000000001,-0.900000000000001,
-0.895000000000001,-0.890000000000001,-0.885000000000001,-0.880000000000001,
-0.875000000000001,-0.870000000000001,-0.865000000000001,-0.860000000000001,
-0.855000000000001,-0.850000000000001,-0.845000000000001,-0.840000000000001,
-0.835000000000001,-0.830000000000001,-0.825000000000001,-0.820000000000001,
-0.815000000000001,-0.810000000000001,-0.805000000000001,-0.800000000000001,
-0.795000000000001,-0.790000000000001,-0.785000000000001,-0.780000000000001,
-0.775000000000001,-0.770000000000001,-0.765000000000001,-0.760000000000001,
-0.755000000000001,-0.750000000000001,-0.745000000000001,-0.740000000000001,
-0.735000000000001,-0.730000000000001,-0.725000000000001,-0.720000000000001,
-0.715000000000001,-0.710000000000001,-0.705000000000001,-0.700000000000001,
-0.695000000000001,-0.690000000000001,-0.685,-0.68,-0.675,-0.67,-0.665,
-0.66,-0.655,-0.65,-0.645,-0.64,-0.635,-0.63,-0.625,-0.62,-0.615,-0.61,
-0.605,-0.6,-0.595,-0.59,-0.585,-0.58,-0.575,-0.57,-0.565,-0.56,-0.555,
-0.55,-0.545,-0.54,-0.535,-0.53,-0.525,-0.52,-0.515,-0.51,-0.505,-0.5,-0.495,
-0.49,-0.485,-0.48,-0.475,-0.47,-0.465,-0.46,-0.455,-0.45,-0.445,-0.44,
-0.435,-0.43,-0.425,-0.42,-0.415,-0.41,-0.405,-0.4,-0.395,-0.39,-0.385,
-0.38,-0.375,-0.37,-0.365,-0.36,-0.355,-0.35,-0.345,-0.34,-0.335,-0.33,
-0.325,-0.32,-0.315,-0.31,-0.305,-0.3,-0.295,-0.29,-0.285,-0.28,-0.275,
-0.27,-0.265,-0.26,-0.255,-0.25,-0.245,-0.24,-0.235,-0.23,-0.225,-0.22,
-0.215,-0.21,-0.205,-0.2,-0.195,-0.19,-0.185,-0.18,-0.175,-0.17,-0.165,
-0.16,-0.155,-0.15,-0.145,-0.14,-0.135,-0.13,-0.125,-0.12,-0.115,-0.11,
-0.105,-0.1,-0.095,-0.09,-0.085,-0.08,-0.075,-0.07,-0.065,-0.06,-0.055,
-0.05,-0.045,-0.04,-0.035,-0.03,-0.025,-0.02,-0.015,-0.01,-0.005,0.),
 .UNSPECIFIED.)
CURVE()
GEOMETRIC_REPRESENTATION_ITEM()
RATIONAL_B_SPLINE_CURVE((1.,1.,1.,1.,1.,1.,1.,1.,1.,1.,1.,1.,1.,1.,1.,1.,
1.,1.,1.,1.,1.,1.,1.,1.,1.,1.,1.,1.,1.,1.,1.,1.,1.,1.,1.,1.,1.,1.,1.,1.,
1.,1.,1.,1.,1.,1.,1.,1.,1.,1.,1.,1.,1.,1.,1.,1.,1.,1.,1.,1.,1.,1.,1.,1.,
1.,1.,1.,1.,1.,1.,1.,1.,1.,1.,1.,1.,1.,1.,1.,1.,1.,1.,1.,1.,1.,1.,1.,1.,
1.,1.,1.,1.,1.,1.,1.,1.,1.,1.,1.,1.,1.,1.,1.,1.,1.,1.,1.,1.,1.,1.,1.,1.,
1.,1.,1.,1.,1.,1.,1.,1.,1.,1.,1.,1.,1.,1.,1.,1.,1.,1.,1.,1.,1.,1.,1.,1.,
1.,1.,1.,1.,1.,1.,1.,1.,1.,1.,1.,1.,1.,1.,1.,1.,1.,1.,1.,1.,1.,1.,1.,1.,
1.,1.,1.,1.,1.,1.,1.,1.,1.,1.,1.,1.,1.,1.,1.,1.,1.,1.,1.,1.,1.,1.,1.,1.,
1.,1.,1.,1.,1.,1.,1.,1.,1.,1.))
REPRESENTATION_ITEM('')
);
#587=(
BOUNDED_CURVE()
B_SPLINE_CURVE(5,(#133424,#133425,#133426,#133427,#133428,#133429,#133430,
#133431,#133432,#133433,#133434,#133435,#133436,#133437,#133438,#133439,
#133440,#133441,#133442,#133443,#133444,#133445,#133446,#133447,#133448,
#133449,#133450,#133451,#133452,#133453,#133454,#133455,#133456,#133457,
#133458,#133459,#133460,#133461,#133462,#133463,#133464,#133465,#133466,
#133467,#133468,#133469,#133470,#133471,#133472,#133473,#133474,#133475,
#133476,#133477,#133478,#133479,#133480,#133481,#133482,#133483,#133484,
#133485,#133486,#133487,#133488,#133489,#133490,#133491,#133492,#133493,
#133494,#133495,#133496,#133497,#133498,#133499,#133500,#133501,#133502,
#133503,#133504,#133505,#133506,#133507,#133508,#133509,#133510,#133511,
#133512,#133513,#133514,#133515,#133516,#133517,#133518,#133519,#133520,
#133521,#133522,#133523,#133524,#133525,#133526,#133527,#133528,#133529,
#133530,#133531,#133532,#133533,#133534,#133535,#133536,#133537,#133538,
#133539,#133540,#133541,#133542,#133543,#133544,#133545,#133546,#133547,
#133548,#133549,#133550,#133551,#133552,#133553,#133554,#133555,#133556,
#133557,#133558,#133559,#133560,#133561,#133562,#133563,#133564,#133565,
#133566,#133567,#133568,#133569,#133570,#133571,#133572,#133573,#133574,
#133575,#133576,#133577,#133578,#133579,#133580,#133581,#133582,#133583,
#133584,#133585,#133586,#133587,#133588,#133589,#133590,#133591,#133592,
#133593,#133594,#133595,#133596,#133597,#133598,#133599,#133600,#133601,
#133602,#133603,#133604,#133605,#133606,#133607,#133608,#133609,#133610,
#133611,#133612,#133613,#133614,#133615,#133616,#133617),.UNSPECIFIED.,
 .F.,.F.)
B_SPLINE_CURVE_WITH_KNOTS((6,1,1,1,1,1,1,1,1,1,1,1,1,1,1,1,1,1,1,1,1,1,
1,1,1,1,1,1,1,1,1,1,1,1,1,1,1,1,1,1,1,1,1,1,1,1,1,1,1,1,1,1,1,1,1,1,1,1,
1,1,1,1,1,1,1,1,1,1,1,1,1,1,1,1,1,1,1,1,1,1,1,1,1,1,1,1,1,1,1,1,1,1,1,1,
1,1,1,1,1,1,1,1,1,1,1,1,1,1,1,1,1,1,1,1,1,1,1,1,1,1,1,1,1,1,1,1,1,1,1,1,
1,1,1,1,1,1,1,1,1,1,1,1,1,1,1,1,1,1,1,1,1,1,1,1,1,1,1,1,1,1,1,1,1,1,1,1,
1,1,1,1,1,1,1,1,1,1,1,1,1,1,1,1,1,1,1,1,1,1,1,6),(0.,0.005,0.01,0.015,0.02,
0.025,0.03,0.035,0.04,0.045,0.05,0.055,0.06,0.065,0.07,0.075,0.08,0.085,
0.09,0.095,0.1,0.105,0.11,0.115,0.12,0.125,0.13,0.135,0.14,0.145,0.15,0.155,
0.16,0.165,0.17,0.175,0.18,0.185,0.19,0.195,0.2,0.205,0.21,0.215,0.22,0.225,
0.23,0.235,0.24,0.245,0.25,0.255,0.26,0.265,0.27,0.275,0.28,0.285,0.29,
0.295,0.3,0.305,0.31,0.315,0.32,0.325,0.33,0.335,0.34,0.345,0.35,0.355,
0.36,0.365,0.37,0.375,0.38,0.385,0.39,0.395,0.4,0.405,0.41,0.415,0.42,0.425,
0.43,0.435,0.44,0.445,0.45,0.455,0.46,0.465,0.47,0.475,0.48,0.485,0.49,
0.495,0.5,0.505,0.51,0.515,0.52,0.525,0.53,0.535,0.54,0.545,0.55,0.555,
0.56,0.565,0.57,0.575,0.58,0.585,0.59,0.595,0.6,0.605,0.61,0.615,0.62,0.625,
0.63,0.635,0.64,0.645,0.65,0.655,0.66,0.665,0.67,0.675,0.68,0.685,0.690000000000001,
0.695000000000001,0.700000000000001,0.705000000000001,0.710000000000001,
0.715000000000001,0.720000000000001,0.725000000000001,0.730000000000001,
0.735000000000001,0.740000000000001,0.745000000000001,0.750000000000001,
0.755000000000001,0.760000000000001,0.765000000000001,0.770000000000001,
0.775000000000001,0.780000000000001,0.785000000000001,0.790000000000001,
0.795000000000001,0.800000000000001,0.805000000000001,0.810000000000001,
0.815000000000001,0.820000000000001,0.825000000000001,0.830000000000001,
0.835000000000001,0.840000000000001,0.845000000000001,0.850000000000001,
0.855000000000001,0.860000000000001,0.865000000000001,0.870000000000001,
0.875000000000001,0.880000000000001,0.885000000000001,0.890000000000001,
0.895000000000001,0.900000000000001,0.905000000000001,0.910000000000001,
0.915000000000001,0.920000000000001,0.925000000000001,0.930000000000001,
0.935000000000001,0.940000000000001,0.941429844438085),.UNSPECIFIED.)
CURVE()
GEOMETRIC_REPRESENTATION_ITEM()
RATIONAL_B_SPLINE_CURVE((1.,1.,1.,1.,1.,1.,1.,1.,1.,1.,1.,1.,1.,1.,1.,1.,
1.,1.,1.,1.,1.,1.,1.,1.,1.,1.,1.,1.,1.,1.,1.,1.,1.,1.,1.,1.,1.,1.,1.,1.,
1.,1.,1.,1.,1.,1.,1.,1.,1.,1.,1.,1.,1.,1.,1.,1.,1.,1.,1.,1.,1.,1.,1.,1.,
1.,1.,1.,1.,1.,1.,1.,1.,1.,1.,1.,1.,1.,1.,1.,1.,1.,1.,1.,1.,1.,1.,1.,1.,
1.,1.,1.,1.,1.,1.,1.,1.,1.,1.,1.,1.,1.,1.,1.,1.,1.,1.,1.,1.,1.,1.,1.,1.,
1.,1.,1.,1.,1.,1.,1.,1.,1.,1.,1.,1.,1.,1.,1.,1.,1.,1.,1.,1.,1.,1.,1.,1.,
1.,1.,1.,1.,1.,1.,1.,1.,1.,1.,1.,1.,1.,1.,1.,1.,1.,1.,1.,1.,1.,1.,1.,1.,
1.,1.,1.,1.,1.,1.,1.,1.,1.,1.,1.,1.,1.,1.,1.,1.,1.,1.,1.,1.,1.,1.,1.,1.,
1.,1.,1.,1.,1.,1.,1.,1.,1.,1.))
REPRESENTATION_ITEM('')
);
#588=(
BOUNDED_CURVE()
B_SPLINE_CURVE(5,(#133620,#133621,#133622,#133623,#133624,#133625,#133626,
#133627,#133628,#133629,#133630,#133631,#133632,#133633,#133634,#133635,
#133636,#133637,#133638,#133639,#133640,#133641,#133642,#133643,#133644,
#133645,#133646,#133647,#133648,#133649,#133650,#133651,#133652,#133653,
#133654,#133655,#133656,#133657,#133658,#133659,#133660,#133661,#133662,
#133663,#133664,#133665,#133666,#133667,#133668,#133669,#133670,#133671,
#133672,#133673,#133674,#133675,#133676,#133677,#133678,#133679,#133680,
#133681,#133682,#133683,#133684,#133685,#133686,#133687,#133688,#133689,
#133690,#133691,#133692,#133693,#133694,#133695,#133696,#133697,#133698,
#133699,#133700,#133701,#133702,#133703,#133704,#133705,#133706,#133707,
#133708,#133709,#133710,#133711,#133712,#133713,#133714,#133715,#133716,
#133717,#133718,#133719,#133720,#133721,#133722,#133723,#133724,#133725,
#133726,#133727,#133728,#133729,#133730,#133731,#133732,#133733,#133734,
#133735,#133736,#133737,#133738,#133739,#133740,#133741,#133742,#133743,
#133744,#133745,#133746,#133747,#133748,#133749,#133750,#133751,#133752,
#133753,#133754,#133755,#133756,#133757,#133758,#133759,#133760,#133761,
#133762,#133763,#133764,#133765,#133766,#133767,#133768,#133769,#133770,
#133771,#133772,#133773,#133774,#133775,#133776,#133777,#133778,#133779,
#133780,#133781,#133782,#133783,#133784,#133785,#133786,#133787,#133788,
#133789,#133790,#133791,#133792,#133793,#133794,#133795,#133796,#133797,
#133798,#133799,#133800,#133801,#133802,#133803,#133804,#133805,#133806,
#133807,#133808,#133809,#133810,#133811,#133812,#133813),.UNSPECIFIED.,
 .F.,.F.)
B_SPLINE_CURVE_WITH_KNOTS((6,1,1,1,1,1,1,1,1,1,1,1,1,1,1,1,1,1,1,1,1,1,
1,1,1,1,1,1,1,1,1,1,1,1,1,1,1,1,1,1,1,1,1,1,1,1,1,1,1,1,1,1,1,1,1,1,1,1,
1,1,1,1,1,1,1,1,1,1,1,1,1,1,1,1,1,1,1,1,1,1,1,1,1,1,1,1,1,1,1,1,1,1,1,1,
1,1,1,1,1,1,1,1,1,1,1,1,1,1,1,1,1,1,1,1,1,1,1,1,1,1,1,1,1,1,1,1,1,1,1,1,
1,1,1,1,1,1,1,1,1,1,1,1,1,1,1,1,1,1,1,1,1,1,1,1,1,1,1,1,1,1,1,1,1,1,1,1,
1,1,1,1,1,1,1,1,1,1,1,1,1,1,1,1,1,1,1,1,1,1,1,6),(-0.941429844438085,-0.940000000000001,
-0.935000000000001,-0.930000000000001,-0.925000000000001,-0.920000000000001,
-0.915000000000001,-0.910000000000001,-0.905000000000001,-0.900000000000001,
-0.895000000000001,-0.890000000000001,-0.885000000000001,-0.880000000000001,
-0.875000000000001,-0.870000000000001,-0.865000000000001,-0.860000000000001,
-0.855000000000001,-0.850000000000001,-0.845000000000001,-0.840000000000001,
-0.835000000000001,-0.830000000000001,-0.825000000000001,-0.820000000000001,
-0.815000000000001,-0.810000000000001,-0.805000000000001,-0.800000000000001,
-0.795000000000001,-0.790000000000001,-0.785000000000001,-0.780000000000001,
-0.775000000000001,-0.770000000000001,-0.765000000000001,-0.760000000000001,
-0.755000000000001,-0.750000000000001,-0.745000000000001,-0.740000000000001,
-0.735000000000001,-0.730000000000001,-0.725000000000001,-0.720000000000001,
-0.715000000000001,-0.710000000000001,-0.705000000000001,-0.700000000000001,
-0.695000000000001,-0.690000000000001,-0.685,-0.68,-0.675,-0.67,-0.665,
-0.66,-0.655,-0.65,-0.645,-0.64,-0.635,-0.63,-0.625,-0.62,-0.615,-0.61,
-0.605,-0.6,-0.595,-0.59,-0.585,-0.58,-0.575,-0.57,-0.565,-0.56,-0.555,
-0.55,-0.545,-0.54,-0.535,-0.53,-0.525,-0.52,-0.515,-0.51,-0.505,-0.5,-0.495,
-0.49,-0.485,-0.48,-0.475,-0.47,-0.465,-0.46,-0.455,-0.45,-0.445,-0.44,
-0.435,-0.43,-0.425,-0.42,-0.415,-0.41,-0.405,-0.4,-0.395,-0.39,-0.385,
-0.38,-0.375,-0.37,-0.365,-0.36,-0.355,-0.35,-0.345,-0.34,-0.335,-0.33,
-0.325,-0.32,-0.315,-0.31,-0.305,-0.3,-0.295,-0.29,-0.285,-0.28,-0.275,
-0.27,-0.265,-0.26,-0.255,-0.25,-0.245,-0.24,-0.235,-0.23,-0.225,-0.22,
-0.215,-0.21,-0.205,-0.2,-0.195,-0.19,-0.185,-0.18,-0.175,-0.17,-0.165,
-0.16,-0.155,-0.15,-0.145,-0.14,-0.135,-0.13,-0.125,-0.12,-0.115,-0.11,
-0.105,-0.1,-0.095,-0.09,-0.085,-0.08,-0.075,-0.07,-0.065,-0.06,-0.055,
-0.05,-0.045,-0.04,-0.035,-0.03,-0.025,-0.02,-0.015,-0.01,-0.005,0.),
 .UNSPECIFIED.)
CURVE()
GEOMETRIC_REPRESENTATION_ITEM()
RATIONAL_B_SPLINE_CURVE((1.,1.,1.,1.,1.,1.,1.,1.,1.,1.,1.,1.,1.,1.,1.,1.,
1.,1.,1.,1.,1.,1.,1.,1.,1.,1.,1.,1.,1.,1.,1.,1.,1.,1.,1.,1.,1.,1.,1.,1.,
1.,1.,1.,1.,1.,1.,1.,1.,1.,1.,1.,1.,1.,1.,1.,1.,1.,1.,1.,1.,1.,1.,1.,1.,
1.,1.,1.,1.,1.,1.,1.,1.,1.,1.,1.,1.,1.,1.,1.,1.,1.,1.,1.,1.,1.,1.,1.,1.,
1.,1.,1.,1.,1.,1.,1.,1.,1.,1.,1.,1.,1.,1.,1.,1.,1.,1.,1.,1.,1.,1.,1.,1.,
1.,1.,1.,1.,1.,1.,1.,1.,1.,1.,1.,1.,1.,1.,1.,1.,1.,1.,1.,1.,1.,1.,1.,1.,
1.,1.,1.,1.,1.,1.,1.,1.,1.,1.,1.,1.,1.,1.,1.,1.,1.,1.,1.,1.,1.,1.,1.,1.,
1.,1.,1.,1.,1.,1.,1.,1.,1.,1.,1.,1.,1.,1.,1.,1.,1.,1.,1.,1.,1.,1.,1.,1.,
1.,1.,1.,1.,1.,1.,1.,1.,1.,1.))
REPRESENTATION_ITEM('')
);
#589=(
BOUNDED_CURVE()
B_SPLINE_CURVE(5,(#134225,#134226,#134227,#134228,#134229,#134230,#134231,
#134232,#134233,#134234,#134235,#134236,#134237,#134238,#134239,#134240,
#134241,#134242,#134243,#134244,#134245,#134246,#134247,#134248,#134249,
#134250,#134251,#134252,#134253,#134254,#134255,#134256,#134257,#134258,
#134259,#134260,#134261,#134262,#134263,#134264,#134265,#134266,#134267,
#134268,#134269,#134270,#134271,#134272,#134273,#134274,#134275,#134276,
#134277,#134278,#134279,#134280,#134281,#134282,#134283,#134284,#134285,
#134286,#134287,#134288,#134289,#134290,#134291,#134292,#134293,#134294,
#134295,#134296,#134297,#134298,#134299,#134300,#134301,#134302,#134303,
#134304,#134305,#134306,#134307,#134308,#134309,#134310,#134311,#134312,
#134313,#134314,#134315,#134316,#134317,#134318,#134319,#134320,#134321,
#134322,#134323,#134324,#134325,#134326,#134327,#134328,#134329,#134330,
#134331,#134332,#134333,#134334,#134335,#134336,#134337,#134338,#134339,
#134340,#134341,#134342,#134343,#134344,#134345,#134346,#134347,#134348,
#134349,#134350,#134351,#134352,#134353,#134354,#134355,#134356,#134357,
#134358,#134359,#134360,#134361,#134362,#134363,#134364,#134365,#134366,
#134367,#134368,#134369,#134370,#134371,#134372,#134373,#134374,#134375,
#134376,#134377,#134378,#134379,#134380,#134381,#134382,#134383,#134384,
#134385,#134386,#134387,#134388,#134389,#134390,#134391,#134392,#134393,
#134394,#134395,#134396,#134397,#134398,#134399,#134400,#134401,#134402,
#134403,#134404,#134405,#134406,#134407,#134408,#134409,#134410,#134411,
#134412,#134413,#134414,#134415,#134416,#134417,#134418),.UNSPECIFIED.,
 .F.,.F.)
B_SPLINE_CURVE_WITH_KNOTS((6,1,1,1,1,1,1,1,1,1,1,1,1,1,1,1,1,1,1,1,1,1,
1,1,1,1,1,1,1,1,1,1,1,1,1,1,1,1,1,1,1,1,1,1,1,1,1,1,1,1,1,1,1,1,1,1,1,1,
1,1,1,1,1,1,1,1,1,1,1,1,1,1,1,1,1,1,1,1,1,1,1,1,1,1,1,1,1,1,1,1,1,1,1,1,
1,1,1,1,1,1,1,1,1,1,1,1,1,1,1,1,1,1,1,1,1,1,1,1,1,1,1,1,1,1,1,1,1,1,1,1,
1,1,1,1,1,1,1,1,1,1,1,1,1,1,1,1,1,1,1,1,1,1,1,1,1,1,1,1,1,1,1,1,1,1,1,1,
1,1,1,1,1,1,1,1,1,1,1,1,1,1,1,1,1,1,1,1,1,1,1,6),(0.,0.005,0.01,0.015,0.02,
0.025,0.03,0.035,0.04,0.045,0.05,0.055,0.06,0.065,0.07,0.075,0.08,0.085,
0.09,0.095,0.1,0.105,0.11,0.115,0.12,0.125,0.13,0.135,0.14,0.145,0.15,0.155,
0.16,0.165,0.17,0.175,0.18,0.185,0.19,0.195,0.2,0.205,0.21,0.215,0.22,0.225,
0.23,0.235,0.24,0.245,0.25,0.255,0.26,0.265,0.27,0.275,0.28,0.285,0.29,
0.295,0.3,0.305,0.31,0.315,0.32,0.325,0.33,0.335,0.34,0.345,0.35,0.355,
0.36,0.365,0.37,0.375,0.38,0.385,0.39,0.395,0.4,0.405,0.41,0.415,0.42,0.425,
0.43,0.435,0.44,0.445,0.45,0.455,0.46,0.465,0.47,0.475,0.48,0.485,0.49,
0.495,0.5,0.505,0.51,0.515,0.52,0.525,0.53,0.535,0.54,0.545,0.55,0.555,
0.56,0.565,0.57,0.575,0.58,0.585,0.59,0.595,0.6,0.605,0.61,0.615,0.62,0.625,
0.63,0.635,0.64,0.645,0.65,0.655,0.66,0.665,0.67,0.675,0.68,0.685,0.690000000000001,
0.695000000000001,0.700000000000001,0.705000000000001,0.710000000000001,
0.715000000000001,0.720000000000001,0.725000000000001,0.730000000000001,
0.735000000000001,0.740000000000001,0.745000000000001,0.750000000000001,
0.755000000000001,0.760000000000001,0.765000000000001,0.770000000000001,
0.775000000000001,0.780000000000001,0.785000000000001,0.790000000000001,
0.795000000000001,0.800000000000001,0.805000000000001,0.810000000000001,
0.815000000000001,0.820000000000001,0.825000000000001,0.830000000000001,
0.835000000000001,0.840000000000001,0.845000000000001,0.850000000000001,
0.855000000000001,0.860000000000001,0.865000000000001,0.870000000000001,
0.875000000000001,0.880000000000001,0.885000000000001,0.890000000000001,
0.895000000000001,0.900000000000001,0.905000000000001,0.910000000000001,
0.915000000000001,0.920000000000001,0.925000000000001,0.930000000000001,
0.935000000000001,0.940000000000001,0.941429844438033),.UNSPECIFIED.)
CURVE()
GEOMETRIC_REPRESENTATION_ITEM()
RATIONAL_B_SPLINE_CURVE((1.,1.,1.,1.,1.,1.,1.,1.,1.,1.,1.,1.,1.,1.,1.,1.,
1.,1.,1.,1.,1.,1.,1.,1.,1.,1.,1.,1.,1.,1.,1.,1.,1.,1.,1.,1.,1.,1.,1.,1.,
1.,1.,1.,1.,1.,1.,1.,1.,1.,1.,1.,1.,1.,1.,1.,1.,1.,1.,1.,1.,1.,1.,1.,1.,
1.,1.,1.,1.,1.,1.,1.,1.,1.,1.,1.,1.,1.,1.,1.,1.,1.,1.,1.,1.,1.,1.,1.,1.,
1.,1.,1.,1.,1.,1.,1.,1.,1.,1.,1.,1.,1.,1.,1.,1.,1.,1.,1.,1.,1.,1.,1.,1.,
1.,1.,1.,1.,1.,1.,1.,1.,1.,1.,1.,1.,1.,1.,1.,1.,1.,1.,1.,1.,1.,1.,1.,1.,
1.,1.,1.,1.,1.,1.,1.,1.,1.,1.,1.,1.,1.,1.,1.,1.,1.,1.,1.,1.,1.,1.,1.,1.,
1.,1.,1.,1.,1.,1.,1.,1.,1.,1.,1.,1.,1.,1.,1.,1.,1.,1.,1.,1.,1.,1.,1.,1.,
1.,1.,1.,1.,1.,1.,1.,1.,1.,1.))
REPRESENTATION_ITEM('')
);
#590=(
BOUNDED_CURVE()
B_SPLINE_CURVE(5,(#134421,#134422,#134423,#134424,#134425,#134426,#134427,
#134428,#134429,#134430,#134431,#134432,#134433,#134434,#134435,#134436,
#134437,#134438,#134439,#134440,#134441,#134442,#134443,#134444,#134445,
#134446,#134447,#134448,#134449,#134450,#134451,#134452,#134453,#134454,
#134455,#134456,#134457,#134458,#134459,#134460,#134461,#134462,#134463,
#134464,#134465,#134466,#134467,#134468,#134469,#134470,#134471,#134472,
#134473,#134474,#134475,#134476,#134477,#134478,#134479,#134480,#134481,
#134482,#134483,#134484,#134485,#134486,#134487,#134488,#134489,#134490,
#134491,#134492,#134493,#134494,#134495,#134496,#134497,#134498,#134499,
#134500,#134501,#134502,#134503,#134504,#134505,#134506,#134507,#134508,
#134509,#134510,#134511,#134512,#134513,#134514,#134515,#134516,#134517,
#134518,#134519,#134520,#134521,#134522,#134523,#134524,#134525,#134526,
#134527,#134528,#134529,#134530,#134531,#134532,#134533,#134534,#134535,
#134536,#134537,#134538,#134539,#134540,#134541,#134542,#134543,#134544,
#134545,#134546,#134547,#134548,#134549,#134550,#134551,#134552,#134553,
#134554,#134555,#134556,#134557,#134558,#134559,#134560,#134561,#134562,
#134563,#134564,#134565,#134566,#134567,#134568,#134569,#134570,#134571,
#134572,#134573,#134574,#134575,#134576,#134577,#134578,#134579,#134580,
#134581,#134582,#134583,#134584,#134585,#134586,#134587,#134588,#134589,
#134590,#134591,#134592,#134593,#134594,#134595,#134596,#134597,#134598,
#134599,#134600,#134601,#134602,#134603,#134604,#134605,#134606,#134607,
#134608,#134609,#134610,#134611,#134612,#134613,#134614),.UNSPECIFIED.,
 .F.,.F.)
B_SPLINE_CURVE_WITH_KNOTS((6,1,1,1,1,1,1,1,1,1,1,1,1,1,1,1,1,1,1,1,1,1,
1,1,1,1,1,1,1,1,1,1,1,1,1,1,1,1,1,1,1,1,1,1,1,1,1,1,1,1,1,1,1,1,1,1,1,1,
1,1,1,1,1,1,1,1,1,1,1,1,1,1,1,1,1,1,1,1,1,1,1,1,1,1,1,1,1,1,1,1,1,1,1,1,
1,1,1,1,1,1,1,1,1,1,1,1,1,1,1,1,1,1,1,1,1,1,1,1,1,1,1,1,1,1,1,1,1,1,1,1,
1,1,1,1,1,1,1,1,1,1,1,1,1,1,1,1,1,1,1,1,1,1,1,1,1,1,1,1,1,1,1,1,1,1,1,1,
1,1,1,1,1,1,1,1,1,1,1,1,1,1,1,1,1,1,1,1,1,1,1,6),(-0.941429844438033,-0.940000000000001,
-0.935000000000001,-0.930000000000001,-0.925000000000001,-0.920000000000001,
-0.915000000000001,-0.910000000000001,-0.905000000000001,-0.900000000000001,
-0.895000000000001,-0.890000000000001,-0.885000000000001,-0.880000000000001,
-0.875000000000001,-0.870000000000001,-0.865000000000001,-0.860000000000001,
-0.855000000000001,-0.850000000000001,-0.845000000000001,-0.840000000000001,
-0.835000000000001,-0.830000000000001,-0.825000000000001,-0.820000000000001,
-0.815000000000001,-0.810000000000001,-0.805000000000001,-0.800000000000001,
-0.795000000000001,-0.790000000000001,-0.785000000000001,-0.780000000000001,
-0.775000000000001,-0.770000000000001,-0.765000000000001,-0.760000000000001,
-0.755000000000001,-0.750000000000001,-0.745000000000001,-0.740000000000001,
-0.735000000000001,-0.730000000000001,-0.725000000000001,-0.720000000000001,
-0.715000000000001,-0.710000000000001,-0.705000000000001,-0.700000000000001,
-0.695000000000001,-0.690000000000001,-0.685,-0.68,-0.675,-0.67,-0.665,
-0.66,-0.655,-0.65,-0.645,-0.64,-0.635,-0.63,-0.625,-0.62,-0.615,-0.61,
-0.605,-0.6,-0.595,-0.59,-0.585,-0.58,-0.575,-0.57,-0.565,-0.56,-0.555,
-0.55,-0.545,-0.54,-0.535,-0.53,-0.525,-0.52,-0.515,-0.51,-0.505,-0.5,-0.495,
-0.49,-0.485,-0.48,-0.475,-0.47,-0.465,-0.46,-0.455,-0.45,-0.445,-0.44,
-0.435,-0.43,-0.425,-0.42,-0.415,-0.41,-0.405,-0.4,-0.395,-0.39,-0.385,
-0.38,-0.375,-0.37,-0.365,-0.36,-0.355,-0.35,-0.345,-0.34,-0.335,-0.33,
-0.325,-0.32,-0.315,-0.31,-0.305,-0.3,-0.295,-0.29,-0.285,-0.28,-0.275,
-0.27,-0.265,-0.26,-0.255,-0.25,-0.245,-0.24,-0.235,-0.23,-0.225,-0.22,
-0.215,-0.21,-0.205,-0.2,-0.195,-0.19,-0.185,-0.18,-0.175,-0.17,-0.165,
-0.16,-0.155,-0.15,-0.145,-0.14,-0.135,-0.13,-0.125,-0.12,-0.115,-0.11,
-0.105,-0.1,-0.095,-0.09,-0.085,-0.08,-0.075,-0.07,-0.065,-0.06,-0.055,
-0.05,-0.045,-0.04,-0.035,-0.03,-0.025,-0.02,-0.015,-0.01,-0.005,0.),
 .UNSPECIFIED.)
CURVE()
GEOMETRIC_REPRESENTATION_ITEM()
RATIONAL_B_SPLINE_CURVE((1.,1.,1.,1.,1.,1.,1.,1.,1.,1.,1.,1.,1.,1.,1.,1.,
1.,1.,1.,1.,1.,1.,1.,1.,1.,1.,1.,1.,1.,1.,1.,1.,1.,1.,1.,1.,1.,1.,1.,1.,
1.,1.,1.,1.,1.,1.,1.,1.,1.,1.,1.,1.,1.,1.,1.,1.,1.,1.,1.,1.,1.,1.,1.,1.,
1.,1.,1.,1.,1.,1.,1.,1.,1.,1.,1.,1.,1.,1.,1.,1.,1.,1.,1.,1.,1.,1.,1.,1.,
1.,1.,1.,1.,1.,1.,1.,1.,1.,1.,1.,1.,1.,1.,1.,1.,1.,1.,1.,1.,1.,1.,1.,1.,
1.,1.,1.,1.,1.,1.,1.,1.,1.,1.,1.,1.,1.,1.,1.,1.,1.,1.,1.,1.,1.,1.,1.,1.,
1.,1.,1.,1.,1.,1.,1.,1.,1.,1.,1.,1.,1.,1.,1.,1.,1.,1.,1.,1.,1.,1.,1.,1.,
1.,1.,1.,1.,1.,1.,1.,1.,1.,1.,1.,1.,1.,1.,1.,1.,1.,1.,1.,1.,1.,1.,1.,1.,
1.,1.,1.,1.,1.,1.,1.,1.,1.,1.))
REPRESENTATION_ITEM('')
);
#591=(
BOUNDED_CURVE()
B_SPLINE_CURVE(5,(#135026,#135027,#135028,#135029,#135030,#135031,#135032,
#135033,#135034,#135035,#135036,#135037,#135038,#135039,#135040,#135041,
#135042,#135043,#135044,#135045,#135046,#135047,#135048,#135049,#135050,
#135051,#135052,#135053,#135054,#135055,#135056,#135057,#135058,#135059,
#135060,#135061,#135062,#135063,#135064,#135065,#135066,#135067,#135068,
#135069,#135070,#135071,#135072,#135073,#135074,#135075,#135076,#135077,
#135078,#135079,#135080,#135081,#135082,#135083,#135084,#135085,#135086,
#135087,#135088,#135089,#135090,#135091,#135092,#135093,#135094,#135095,
#135096,#135097,#135098,#135099,#135100,#135101,#135102,#135103,#135104,
#135105,#135106,#135107,#135108,#135109,#135110,#135111,#135112,#135113,
#135114,#135115,#135116,#135117,#135118,#135119,#135120,#135121,#135122,
#135123,#135124,#135125,#135126,#135127,#135128,#135129,#135130,#135131,
#135132,#135133,#135134,#135135,#135136,#135137,#135138,#135139,#135140,
#135141,#135142,#135143,#135144,#135145,#135146,#135147,#135148,#135149,
#135150,#135151,#135152,#135153,#135154,#135155,#135156,#135157,#135158,
#135159,#135160,#135161,#135162,#135163,#135164,#135165,#135166,#135167,
#135168,#135169,#135170,#135171,#135172,#135173,#135174,#135175,#135176,
#135177,#135178,#135179,#135180,#135181,#135182,#135183,#135184,#135185,
#135186,#135187,#135188,#135189,#135190,#135191,#135192,#135193,#135194,
#135195,#135196,#135197,#135198,#135199,#135200,#135201,#135202,#135203,
#135204,#135205,#135206,#135207,#135208,#135209,#135210,#135211,#135212,
#135213,#135214,#135215,#135216,#135217,#135218,#135219),.UNSPECIFIED.,
 .F.,.F.)
B_SPLINE_CURVE_WITH_KNOTS((6,1,1,1,1,1,1,1,1,1,1,1,1,1,1,1,1,1,1,1,1,1,
1,1,1,1,1,1,1,1,1,1,1,1,1,1,1,1,1,1,1,1,1,1,1,1,1,1,1,1,1,1,1,1,1,1,1,1,
1,1,1,1,1,1,1,1,1,1,1,1,1,1,1,1,1,1,1,1,1,1,1,1,1,1,1,1,1,1,1,1,1,1,1,1,
1,1,1,1,1,1,1,1,1,1,1,1,1,1,1,1,1,1,1,1,1,1,1,1,1,1,1,1,1,1,1,1,1,1,1,1,
1,1,1,1,1,1,1,1,1,1,1,1,1,1,1,1,1,1,1,1,1,1,1,1,1,1,1,1,1,1,1,1,1,1,1,1,
1,1,1,1,1,1,1,1,1,1,1,1,1,1,1,1,1,1,1,1,1,1,1,6),(0.,0.005,0.01,0.015,0.02,
0.025,0.03,0.035,0.04,0.045,0.05,0.055,0.06,0.065,0.07,0.075,0.08,0.085,
0.09,0.095,0.1,0.105,0.11,0.115,0.12,0.125,0.13,0.135,0.14,0.145,0.15,0.155,
0.16,0.165,0.17,0.175,0.18,0.185,0.19,0.195,0.2,0.205,0.21,0.215,0.22,0.225,
0.23,0.235,0.24,0.245,0.25,0.255,0.26,0.265,0.27,0.275,0.28,0.285,0.29,
0.295,0.3,0.305,0.31,0.315,0.32,0.325,0.33,0.335,0.34,0.345,0.35,0.355,
0.36,0.365,0.37,0.375,0.38,0.385,0.39,0.395,0.4,0.405,0.41,0.415,0.42,0.425,
0.43,0.435,0.44,0.445,0.45,0.455,0.46,0.465,0.47,0.475,0.48,0.485,0.49,
0.495,0.5,0.505,0.51,0.515,0.52,0.525,0.53,0.535,0.54,0.545,0.55,0.555,
0.56,0.565,0.57,0.575,0.58,0.585,0.59,0.595,0.6,0.605,0.61,0.615,0.62,0.625,
0.63,0.635,0.64,0.645,0.65,0.655,0.66,0.665,0.67,0.675,0.68,0.685,0.690000000000001,
0.695000000000001,0.700000000000001,0.705000000000001,0.710000000000001,
0.715000000000001,0.720000000000001,0.725000000000001,0.730000000000001,
0.735000000000001,0.740000000000001,0.745000000000001,0.750000000000001,
0.755000000000001,0.760000000000001,0.765000000000001,0.770000000000001,
0.775000000000001,0.780000000000001,0.785000000000001,0.790000000000001,
0.795000000000001,0.800000000000001,0.805000000000001,0.810000000000001,
0.815000000000001,0.820000000000001,0.825000000000001,0.830000000000001,
0.835000000000001,0.840000000000001,0.845000000000001,0.850000000000001,
0.855000000000001,0.860000000000001,0.865000000000001,0.870000000000001,
0.875000000000001,0.880000000000001,0.885000000000001,0.890000000000001,
0.895000000000001,0.900000000000001,0.905000000000001,0.910000000000001,
0.915000000000001,0.920000000000001,0.925000000000001,0.930000000000001,
0.935000000000001,0.940000000000001,0.941429844438099),.UNSPECIFIED.)
CURVE()
GEOMETRIC_REPRESENTATION_ITEM()
RATIONAL_B_SPLINE_CURVE((1.,1.,1.,1.,1.,1.,1.,1.,1.,1.,1.,1.,1.,1.,1.,1.,
1.,1.,1.,1.,1.,1.,1.,1.,1.,1.,1.,1.,1.,1.,1.,1.,1.,1.,1.,1.,1.,1.,1.,1.,
1.,1.,1.,1.,1.,1.,1.,1.,1.,1.,1.,1.,1.,1.,1.,1.,1.,1.,1.,1.,1.,1.,1.,1.,
1.,1.,1.,1.,1.,1.,1.,1.,1.,1.,1.,1.,1.,1.,1.,1.,1.,1.,1.,1.,1.,1.,1.,1.,
1.,1.,1.,1.,1.,1.,1.,1.,1.,1.,1.,1.,1.,1.,1.,1.,1.,1.,1.,1.,1.,1.,1.,1.,
1.,1.,1.,1.,1.,1.,1.,1.,1.,1.,1.,1.,1.,1.,1.,1.,1.,1.,1.,1.,1.,1.,1.,1.,
1.,1.,1.,1.,1.,1.,1.,1.,1.,1.,1.,1.,1.,1.,1.,1.,1.,1.,1.,1.,1.,1.,1.,1.,
1.,1.,1.,1.,1.,1.,1.,1.,1.,1.,1.,1.,1.,1.,1.,1.,1.,1.,1.,1.,1.,1.,1.,1.,
1.,1.,1.,1.,1.,1.,1.,1.,1.,1.))
REPRESENTATION_ITEM('')
);
#592=(
BOUNDED_CURVE()
B_SPLINE_CURVE(5,(#135222,#135223,#135224,#135225,#135226,#135227,#135228,
#135229,#135230,#135231,#135232,#135233,#135234,#135235,#135236,#135237,
#135238,#135239,#135240,#135241,#135242,#135243,#135244,#135245,#135246,
#135247,#135248,#135249,#135250,#135251,#135252,#135253,#135254,#135255,
#135256,#135257,#135258,#135259,#135260,#135261,#135262,#135263,#135264,
#135265,#135266,#135267,#135268,#135269,#135270,#135271,#135272,#135273,
#135274,#135275,#135276,#135277,#135278,#135279,#135280,#135281,#135282,
#135283,#135284,#135285,#135286,#135287,#135288,#135289,#135290,#135291,
#135292,#135293,#135294,#135295,#135296,#135297,#135298,#135299,#135300,
#135301,#135302,#135303,#135304,#135305,#135306,#135307,#135308,#135309,
#135310,#135311,#135312,#135313,#135314,#135315,#135316,#135317,#135318,
#135319,#135320,#135321,#135322,#135323,#135324,#135325,#135326,#135327,
#135328,#135329,#135330,#135331,#135332,#135333,#135334,#135335,#135336,
#135337,#135338,#135339,#135340,#135341,#135342,#135343,#135344,#135345,
#135346,#135347,#135348,#135349,#135350,#135351,#135352,#135353,#135354,
#135355,#135356,#135357,#135358,#135359,#135360,#135361,#135362,#135363,
#135364,#135365,#135366,#135367,#135368,#135369,#135370,#135371,#135372,
#135373,#135374,#135375,#135376,#135377,#135378,#135379,#135380,#135381,
#135382,#135383,#135384,#135385,#135386,#135387,#135388,#135389,#135390,
#135391,#135392,#135393,#135394,#135395,#135396,#135397,#135398,#135399,
#135400,#135401,#135402,#135403,#135404,#135405,#135406,#135407,#135408,
#135409,#135410,#135411,#135412,#135413,#135414,#135415),.UNSPECIFIED.,
 .F.,.F.)
B_SPLINE_CURVE_WITH_KNOTS((6,1,1,1,1,1,1,1,1,1,1,1,1,1,1,1,1,1,1,1,1,1,
1,1,1,1,1,1,1,1,1,1,1,1,1,1,1,1,1,1,1,1,1,1,1,1,1,1,1,1,1,1,1,1,1,1,1,1,
1,1,1,1,1,1,1,1,1,1,1,1,1,1,1,1,1,1,1,1,1,1,1,1,1,1,1,1,1,1,1,1,1,1,1,1,
1,1,1,1,1,1,1,1,1,1,1,1,1,1,1,1,1,1,1,1,1,1,1,1,1,1,1,1,1,1,1,1,1,1,1,1,
1,1,1,1,1,1,1,1,1,1,1,1,1,1,1,1,1,1,1,1,1,1,1,1,1,1,1,1,1,1,1,1,1,1,1,1,
1,1,1,1,1,1,1,1,1,1,1,1,1,1,1,1,1,1,1,1,1,1,1,6),(-0.941429844438094,-0.940000000000001,
-0.935000000000001,-0.930000000000001,-0.925000000000001,-0.920000000000001,
-0.915000000000001,-0.910000000000001,-0.905000000000001,-0.900000000000001,
-0.895000000000001,-0.890000000000001,-0.885000000000001,-0.880000000000001,
-0.875000000000001,-0.870000000000001,-0.865000000000001,-0.860000000000001,
-0.855000000000001,-0.850000000000001,-0.845000000000001,-0.840000000000001,
-0.835000000000001,-0.830000000000001,-0.825000000000001,-0.820000000000001,
-0.815000000000001,-0.810000000000001,-0.805000000000001,-0.800000000000001,
-0.795000000000001,-0.790000000000001,-0.785000000000001,-0.780000000000001,
-0.775000000000001,-0.770000000000001,-0.765000000000001,-0.760000000000001,
-0.755000000000001,-0.750000000000001,-0.745000000000001,-0.740000000000001,
-0.735000000000001,-0.730000000000001,-0.725000000000001,-0.720000000000001,
-0.715000000000001,-0.710000000000001,-0.705000000000001,-0.700000000000001,
-0.695000000000001,-0.690000000000001,-0.685,-0.68,-0.675,-0.67,-0.665,
-0.66,-0.655,-0.65,-0.645,-0.64,-0.635,-0.63,-0.625,-0.62,-0.615,-0.61,
-0.605,-0.6,-0.595,-0.59,-0.585,-0.58,-0.575,-0.57,-0.565,-0.56,-0.555,
-0.55,-0.545,-0.54,-0.535,-0.53,-0.525,-0.52,-0.515,-0.51,-0.505,-0.5,-0.495,
-0.49,-0.485,-0.48,-0.475,-0.47,-0.465,-0.46,-0.455,-0.45,-0.445,-0.44,
-0.435,-0.43,-0.425,-0.42,-0.415,-0.41,-0.405,-0.4,-0.395,-0.39,-0.385,
-0.38,-0.375,-0.37,-0.365,-0.36,-0.355,-0.35,-0.345,-0.34,-0.335,-0.33,
-0.325,-0.32,-0.315,-0.31,-0.305,-0.3,-0.295,-0.29,-0.285,-0.28,-0.275,
-0.27,-0.265,-0.26,-0.255,-0.25,-0.245,-0.24,-0.235,-0.23,-0.225,-0.22,
-0.215,-0.21,-0.205,-0.2,-0.195,-0.19,-0.185,-0.18,-0.175,-0.17,-0.165,
-0.16,-0.155,-0.15,-0.145,-0.14,-0.135,-0.13,-0.125,-0.12,-0.115,-0.11,
-0.105,-0.1,-0.095,-0.09,-0.085,-0.08,-0.075,-0.07,-0.065,-0.06,-0.055,
-0.05,-0.045,-0.04,-0.035,-0.03,-0.025,-0.02,-0.015,-0.01,-0.005,0.),
 .UNSPECIFIED.)
CURVE()
GEOMETRIC_REPRESENTATION_ITEM()
RATIONAL_B_SPLINE_CURVE((1.,1.,1.,1.,1.,1.,1.,1.,1.,1.,1.,1.,1.,1.,1.,1.,
1.,1.,1.,1.,1.,1.,1.,1.,1.,1.,1.,1.,1.,1.,1.,1.,1.,1.,1.,1.,1.,1.,1.,1.,
1.,1.,1.,1.,1.,1.,1.,1.,1.,1.,1.,1.,1.,1.,1.,1.,1.,1.,1.,1.,1.,1.,1.,1.,
1.,1.,1.,1.,1.,1.,1.,1.,1.,1.,1.,1.,1.,1.,1.,1.,1.,1.,1.,1.,1.,1.,1.,1.,
1.,1.,1.,1.,1.,1.,1.,1.,1.,1.,1.,1.,1.,1.,1.,1.,1.,1.,1.,1.,1.,1.,1.,1.,
1.,1.,1.,1.,1.,1.,1.,1.,1.,1.,1.,1.,1.,1.,1.,1.,1.,1.,1.,1.,1.,1.,1.,1.,
1.,1.,1.,1.,1.,1.,1.,1.,1.,1.,1.,1.,1.,1.,1.,1.,1.,1.,1.,1.,1.,1.,1.,1.,
1.,1.,1.,1.,1.,1.,1.,1.,1.,1.,1.,1.,1.,1.,1.,1.,1.,1.,1.,1.,1.,1.,1.,1.,
1.,1.,1.,1.,1.,1.,1.,1.,1.,1.))
REPRESENTATION_ITEM('')
);
#593=(
BOUNDED_CURVE()
B_SPLINE_CURVE(5,(#135827,#135828,#135829,#135830,#135831,#135832,#135833,
#135834,#135835,#135836,#135837,#135838,#135839,#135840,#135841,#135842,
#135843,#135844,#135845,#135846,#135847,#135848,#135849,#135850,#135851,
#135852,#135853,#135854,#135855,#135856,#135857,#135858,#135859,#135860,
#135861,#135862,#135863,#135864,#135865,#135866,#135867,#135868,#135869,
#135870,#135871,#135872,#135873,#135874,#135875,#135876,#135877,#135878,
#135879,#135880,#135881,#135882,#135883,#135884,#135885,#135886,#135887,
#135888,#135889,#135890,#135891,#135892,#135893,#135894,#135895,#135896,
#135897,#135898,#135899,#135900,#135901,#135902,#135903,#135904,#135905,
#135906,#135907,#135908,#135909,#135910,#135911,#135912,#135913,#135914,
#135915,#135916,#135917,#135918,#135919,#135920,#135921,#135922,#135923,
#135924,#135925,#135926,#135927,#135928,#135929,#135930,#135931,#135932,
#135933,#135934,#135935,#135936,#135937,#135938,#135939,#135940,#135941,
#135942,#135943,#135944,#135945,#135946,#135947,#135948,#135949,#135950,
#135951,#135952,#135953,#135954,#135955,#135956,#135957,#135958,#135959,
#135960,#135961,#135962,#135963,#135964,#135965,#135966,#135967,#135968,
#135969,#135970,#135971,#135972,#135973,#135974,#135975,#135976,#135977,
#135978,#135979,#135980,#135981,#135982,#135983,#135984,#135985,#135986,
#135987,#135988,#135989,#135990,#135991,#135992,#135993,#135994,#135995,
#135996,#135997,#135998,#135999,#136000,#136001,#136002,#136003,#136004,
#136005,#136006,#136007,#136008,#136009,#136010,#136011,#136012,#136013,
#136014,#136015,#136016,#136017,#136018,#136019,#136020),.UNSPECIFIED.,
 .F.,.F.)
B_SPLINE_CURVE_WITH_KNOTS((6,1,1,1,1,1,1,1,1,1,1,1,1,1,1,1,1,1,1,1,1,1,
1,1,1,1,1,1,1,1,1,1,1,1,1,1,1,1,1,1,1,1,1,1,1,1,1,1,1,1,1,1,1,1,1,1,1,1,
1,1,1,1,1,1,1,1,1,1,1,1,1,1,1,1,1,1,1,1,1,1,1,1,1,1,1,1,1,1,1,1,1,1,1,1,
1,1,1,1,1,1,1,1,1,1,1,1,1,1,1,1,1,1,1,1,1,1,1,1,1,1,1,1,1,1,1,1,1,1,1,1,
1,1,1,1,1,1,1,1,1,1,1,1,1,1,1,1,1,1,1,1,1,1,1,1,1,1,1,1,1,1,1,1,1,1,1,1,
1,1,1,1,1,1,1,1,1,1,1,1,1,1,1,1,1,1,1,1,1,1,1,6),(0.,0.005,0.01,0.015,0.02,
0.025,0.03,0.035,0.04,0.045,0.05,0.055,0.06,0.065,0.07,0.075,0.08,0.085,
0.09,0.095,0.1,0.105,0.11,0.115,0.12,0.125,0.13,0.135,0.14,0.145,0.15,0.155,
0.16,0.165,0.17,0.175,0.18,0.185,0.19,0.195,0.2,0.205,0.21,0.215,0.22,0.225,
0.23,0.235,0.24,0.245,0.25,0.255,0.26,0.265,0.27,0.275,0.28,0.285,0.29,
0.295,0.3,0.305,0.31,0.315,0.32,0.325,0.33,0.335,0.34,0.345,0.35,0.355,
0.36,0.365,0.37,0.375,0.38,0.385,0.39,0.395,0.4,0.405,0.41,0.415,0.42,0.425,
0.43,0.435,0.44,0.445,0.45,0.455,0.46,0.465,0.47,0.475,0.48,0.485,0.49,
0.495,0.5,0.505,0.51,0.515,0.52,0.525,0.53,0.535,0.54,0.545,0.55,0.555,
0.56,0.565,0.57,0.575,0.58,0.585,0.59,0.595,0.6,0.605,0.61,0.615,0.62,0.625,
0.63,0.635,0.64,0.645,0.65,0.655,0.66,0.665,0.67,0.675,0.68,0.685,0.690000000000001,
0.695000000000001,0.700000000000001,0.705000000000001,0.710000000000001,
0.715000000000001,0.720000000000001,0.725000000000001,0.730000000000001,
0.735000000000001,0.740000000000001,0.745000000000001,0.750000000000001,
0.755000000000001,0.760000000000001,0.765000000000001,0.770000000000001,
0.775000000000001,0.780000000000001,0.785000000000001,0.790000000000001,
0.795000000000001,0.800000000000001,0.805000000000001,0.810000000000001,
0.815000000000001,0.820000000000001,0.825000000000001,0.830000000000001,
0.835000000000001,0.840000000000001,0.845000000000001,0.850000000000001,
0.855000000000001,0.860000000000001,0.865000000000001,0.870000000000001,
0.875000000000001,0.880000000000001,0.885000000000001,0.890000000000001,
0.895000000000001,0.900000000000001,0.905000000000001,0.910000000000001,
0.915000000000001,0.920000000000001,0.925000000000001,0.930000000000001,
0.935000000000001,0.940000000000001,0.941429844438126),.UNSPECIFIED.)
CURVE()
GEOMETRIC_REPRESENTATION_ITEM()
RATIONAL_B_SPLINE_CURVE((1.,1.,1.,1.,1.,1.,1.,1.,1.,1.,1.,1.,1.,1.,1.,1.,
1.,1.,1.,1.,1.,1.,1.,1.,1.,1.,1.,1.,1.,1.,1.,1.,1.,1.,1.,1.,1.,1.,1.,1.,
1.,1.,1.,1.,1.,1.,1.,1.,1.,1.,1.,1.,1.,1.,1.,1.,1.,1.,1.,1.,1.,1.,1.,1.,
1.,1.,1.,1.,1.,1.,1.,1.,1.,1.,1.,1.,1.,1.,1.,1.,1.,1.,1.,1.,1.,1.,1.,1.,
1.,1.,1.,1.,1.,1.,1.,1.,1.,1.,1.,1.,1.,1.,1.,1.,1.,1.,1.,1.,1.,1.,1.,1.,
1.,1.,1.,1.,1.,1.,1.,1.,1.,1.,1.,1.,1.,1.,1.,1.,1.,1.,1.,1.,1.,1.,1.,1.,
1.,1.,1.,1.,1.,1.,1.,1.,1.,1.,1.,1.,1.,1.,1.,1.,1.,1.,1.,1.,1.,1.,1.,1.,
1.,1.,1.,1.,1.,1.,1.,1.,1.,1.,1.,1.,1.,1.,1.,1.,1.,1.,1.,1.,1.,1.,1.,1.,
1.,1.,1.,1.,1.,1.,1.,1.,1.,1.))
REPRESENTATION_ITEM('')
);
#594=(
BOUNDED_CURVE()
B_SPLINE_CURVE(5,(#136023,#136024,#136025,#136026,#136027,#136028,#136029,
#136030,#136031,#136032,#136033,#136034,#136035,#136036,#136037,#136038,
#136039,#136040,#136041,#136042,#136043,#136044,#136045,#136046,#136047,
#136048,#136049,#136050,#136051,#136052,#136053,#136054,#136055,#136056,
#136057,#136058,#136059,#136060,#136061,#136062,#136063,#136064,#136065,
#136066,#136067,#136068,#136069,#136070,#136071,#136072,#136073,#136074,
#136075,#136076,#136077,#136078,#136079,#136080,#136081,#136082,#136083,
#136084,#136085,#136086,#136087,#136088,#136089,#136090,#136091,#136092,
#136093,#136094,#136095,#136096,#136097,#136098,#136099,#136100,#136101,
#136102,#136103,#136104,#136105,#136106,#136107,#136108,#136109,#136110,
#136111,#136112,#136113,#136114,#136115,#136116,#136117,#136118,#136119,
#136120,#136121,#136122,#136123,#136124,#136125,#136126,#136127,#136128,
#136129,#136130,#136131,#136132,#136133,#136134,#136135,#136136,#136137,
#136138,#136139,#136140,#136141,#136142,#136143,#136144,#136145,#136146,
#136147,#136148,#136149,#136150,#136151,#136152,#136153,#136154,#136155,
#136156,#136157,#136158,#136159,#136160,#136161,#136162,#136163,#136164,
#136165,#136166,#136167,#136168,#136169,#136170,#136171,#136172,#136173,
#136174,#136175,#136176,#136177,#136178,#136179,#136180,#136181,#136182,
#136183,#136184,#136185,#136186,#136187,#136188,#136189,#136190,#136191,
#136192,#136193,#136194,#136195,#136196,#136197,#136198,#136199,#136200,
#136201,#136202,#136203,#136204,#136205,#136206,#136207,#136208,#136209,
#136210,#136211,#136212,#136213,#136214,#136215,#136216),.UNSPECIFIED.,
 .F.,.F.)
B_SPLINE_CURVE_WITH_KNOTS((6,1,1,1,1,1,1,1,1,1,1,1,1,1,1,1,1,1,1,1,1,1,
1,1,1,1,1,1,1,1,1,1,1,1,1,1,1,1,1,1,1,1,1,1,1,1,1,1,1,1,1,1,1,1,1,1,1,1,
1,1,1,1,1,1,1,1,1,1,1,1,1,1,1,1,1,1,1,1,1,1,1,1,1,1,1,1,1,1,1,1,1,1,1,1,
1,1,1,1,1,1,1,1,1,1,1,1,1,1,1,1,1,1,1,1,1,1,1,1,1,1,1,1,1,1,1,1,1,1,1,1,
1,1,1,1,1,1,1,1,1,1,1,1,1,1,1,1,1,1,1,1,1,1,1,1,1,1,1,1,1,1,1,1,1,1,1,1,
1,1,1,1,1,1,1,1,1,1,1,1,1,1,1,1,1,1,1,1,1,1,1,6),(-0.9414298444381,-0.940000000000001,
-0.935000000000001,-0.930000000000001,-0.925000000000001,-0.920000000000001,
-0.915000000000001,-0.910000000000001,-0.905000000000001,-0.900000000000001,
-0.895000000000001,-0.890000000000001,-0.885000000000001,-0.880000000000001,
-0.875000000000001,-0.870000000000001,-0.865000000000001,-0.860000000000001,
-0.855000000000001,-0.850000000000001,-0.845000000000001,-0.840000000000001,
-0.835000000000001,-0.830000000000001,-0.825000000000001,-0.820000000000001,
-0.815000000000001,-0.810000000000001,-0.805000000000001,-0.800000000000001,
-0.795000000000001,-0.790000000000001,-0.785000000000001,-0.780000000000001,
-0.775000000000001,-0.770000000000001,-0.765000000000001,-0.760000000000001,
-0.755000000000001,-0.750000000000001,-0.745000000000001,-0.740000000000001,
-0.735000000000001,-0.730000000000001,-0.725000000000001,-0.720000000000001,
-0.715000000000001,-0.710000000000001,-0.705000000000001,-0.700000000000001,
-0.695000000000001,-0.690000000000001,-0.685,-0.68,-0.675,-0.67,-0.665,
-0.66,-0.655,-0.65,-0.645,-0.64,-0.635,-0.63,-0.625,-0.62,-0.615,-0.61,
-0.605,-0.6,-0.595,-0.59,-0.585,-0.58,-0.575,-0.57,-0.565,-0.56,-0.555,
-0.55,-0.545,-0.54,-0.535,-0.53,-0.525,-0.52,-0.515,-0.51,-0.505,-0.5,-0.495,
-0.49,-0.485,-0.48,-0.475,-0.47,-0.465,-0.46,-0.455,-0.45,-0.445,-0.44,
-0.435,-0.43,-0.425,-0.42,-0.415,-0.41,-0.405,-0.4,-0.395,-0.39,-0.385,
-0.38,-0.375,-0.37,-0.365,-0.36,-0.355,-0.35,-0.345,-0.34,-0.335,-0.33,
-0.325,-0.32,-0.315,-0.31,-0.305,-0.3,-0.295,-0.29,-0.285,-0.28,-0.275,
-0.27,-0.265,-0.26,-0.255,-0.25,-0.245,-0.24,-0.235,-0.23,-0.225,-0.22,
-0.215,-0.21,-0.205,-0.2,-0.195,-0.19,-0.185,-0.18,-0.175,-0.17,-0.165,
-0.16,-0.155,-0.15,-0.145,-0.14,-0.135,-0.13,-0.125,-0.12,-0.115,-0.11,
-0.105,-0.1,-0.095,-0.09,-0.085,-0.08,-0.075,-0.07,-0.065,-0.06,-0.055,
-0.05,-0.045,-0.04,-0.035,-0.03,-0.025,-0.02,-0.015,-0.01,-0.005,0.),
 .UNSPECIFIED.)
CURVE()
GEOMETRIC_REPRESENTATION_ITEM()
RATIONAL_B_SPLINE_CURVE((1.,1.,1.,1.,1.,1.,1.,1.,1.,1.,1.,1.,1.,1.,1.,1.,
1.,1.,1.,1.,1.,1.,1.,1.,1.,1.,1.,1.,1.,1.,1.,1.,1.,1.,1.,1.,1.,1.,1.,1.,
1.,1.,1.,1.,1.,1.,1.,1.,1.,1.,1.,1.,1.,1.,1.,1.,1.,1.,1.,1.,1.,1.,1.,1.,
1.,1.,1.,1.,1.,1.,1.,1.,1.,1.,1.,1.,1.,1.,1.,1.,1.,1.,1.,1.,1.,1.,1.,1.,
1.,1.,1.,1.,1.,1.,1.,1.,1.,1.,1.,1.,1.,1.,1.,1.,1.,1.,1.,1.,1.,1.,1.,1.,
1.,1.,1.,1.,1.,1.,1.,1.,1.,1.,1.,1.,1.,1.,1.,1.,1.,1.,1.,1.,1.,1.,1.,1.,
1.,1.,1.,1.,1.,1.,1.,1.,1.,1.,1.,1.,1.,1.,1.,1.,1.,1.,1.,1.,1.,1.,1.,1.,
1.,1.,1.,1.,1.,1.,1.,1.,1.,1.,1.,1.,1.,1.,1.,1.,1.,1.,1.,1.,1.,1.,1.,1.,
1.,1.,1.,1.,1.,1.,1.,1.,1.,1.))
REPRESENTATION_ITEM('')
);
#595=(
BOUNDED_CURVE()
B_SPLINE_CURVE(5,(#136628,#136629,#136630,#136631,#136632,#136633,#136634,
#136635,#136636,#136637,#136638,#136639,#136640,#136641,#136642,#136643,
#136644,#136645,#136646,#136647,#136648,#136649,#136650,#136651,#136652,
#136653,#136654,#136655,#136656,#136657,#136658,#136659,#136660,#136661,
#136662,#136663,#136664,#136665,#136666,#136667,#136668,#136669,#136670,
#136671,#136672,#136673,#136674,#136675,#136676,#136677,#136678,#136679,
#136680,#136681,#136682,#136683,#136684,#136685,#136686,#136687,#136688,
#136689,#136690,#136691,#136692,#136693,#136694,#136695,#136696,#136697,
#136698,#136699,#136700,#136701,#136702,#136703,#136704,#136705,#136706,
#136707,#136708,#136709,#136710,#136711,#136712,#136713,#136714,#136715,
#136716,#136717,#136718,#136719,#136720,#136721,#136722,#136723,#136724,
#136725,#136726,#136727,#136728,#136729,#136730,#136731,#136732,#136733,
#136734,#136735,#136736,#136737,#136738,#136739,#136740,#136741,#136742,
#136743,#136744,#136745,#136746,#136747,#136748,#136749,#136750,#136751,
#136752,#136753,#136754,#136755,#136756,#136757,#136758,#136759,#136760,
#136761,#136762,#136763,#136764,#136765,#136766,#136767,#136768,#136769,
#136770,#136771,#136772,#136773,#136774,#136775,#136776,#136777,#136778,
#136779,#136780,#136781,#136782,#136783,#136784,#136785,#136786,#136787,
#136788,#136789,#136790,#136791,#136792,#136793,#136794,#136795,#136796,
#136797,#136798,#136799,#136800,#136801,#136802,#136803,#136804,#136805,
#136806,#136807,#136808,#136809,#136810,#136811,#136812,#136813,#136814,
#136815,#136816,#136817,#136818,#136819,#136820,#136821),.UNSPECIFIED.,
 .F.,.F.)
B_SPLINE_CURVE_WITH_KNOTS((6,1,1,1,1,1,1,1,1,1,1,1,1,1,1,1,1,1,1,1,1,1,
1,1,1,1,1,1,1,1,1,1,1,1,1,1,1,1,1,1,1,1,1,1,1,1,1,1,1,1,1,1,1,1,1,1,1,1,
1,1,1,1,1,1,1,1,1,1,1,1,1,1,1,1,1,1,1,1,1,1,1,1,1,1,1,1,1,1,1,1,1,1,1,1,
1,1,1,1,1,1,1,1,1,1,1,1,1,1,1,1,1,1,1,1,1,1,1,1,1,1,1,1,1,1,1,1,1,1,1,1,
1,1,1,1,1,1,1,1,1,1,1,1,1,1,1,1,1,1,1,1,1,1,1,1,1,1,1,1,1,1,1,1,1,1,1,1,
1,1,1,1,1,1,1,1,1,1,1,1,1,1,1,1,1,1,1,1,1,1,1,6),(0.,0.005,0.01,0.015,0.02,
0.025,0.03,0.035,0.04,0.045,0.05,0.055,0.06,0.065,0.07,0.075,0.08,0.085,
0.09,0.095,0.1,0.105,0.11,0.115,0.12,0.125,0.13,0.135,0.14,0.145,0.15,0.155,
0.16,0.165,0.17,0.175,0.18,0.185,0.19,0.195,0.2,0.205,0.21,0.215,0.22,0.225,
0.23,0.235,0.24,0.245,0.25,0.255,0.26,0.265,0.27,0.275,0.28,0.285,0.29,
0.295,0.3,0.305,0.31,0.315,0.32,0.325,0.33,0.335,0.34,0.345,0.35,0.355,
0.36,0.365,0.37,0.375,0.38,0.385,0.39,0.395,0.4,0.405,0.41,0.415,0.42,0.425,
0.43,0.435,0.44,0.445,0.45,0.455,0.46,0.465,0.47,0.475,0.48,0.485,0.49,
0.495,0.5,0.505,0.51,0.515,0.52,0.525,0.53,0.535,0.54,0.545,0.55,0.555,
0.56,0.565,0.57,0.575,0.58,0.585,0.59,0.595,0.6,0.605,0.61,0.615,0.62,0.625,
0.63,0.635,0.64,0.645,0.65,0.655,0.66,0.665,0.67,0.675,0.68,0.685,0.690000000000001,
0.695000000000001,0.700000000000001,0.705000000000001,0.710000000000001,
0.715000000000001,0.720000000000001,0.725000000000001,0.730000000000001,
0.735000000000001,0.740000000000001,0.745000000000001,0.750000000000001,
0.755000000000001,0.760000000000001,0.765000000000001,0.770000000000001,
0.775000000000001,0.780000000000001,0.785000000000001,0.790000000000001,
0.795000000000001,0.800000000000001,0.805000000000001,0.810000000000001,
0.815000000000001,0.820000000000001,0.825000000000001,0.830000000000001,
0.835000000000001,0.840000000000001,0.845000000000001,0.850000000000001,
0.855000000000001,0.860000000000001,0.865000000000001,0.870000000000001,
0.875000000000001,0.880000000000001,0.885000000000001,0.890000000000001,
0.895000000000001,0.900000000000001,0.905000000000001,0.910000000000001,
0.915000000000001,0.920000000000001,0.925000000000001,0.930000000000001,
0.935000000000001,0.940000000000001,0.94142984443805),.UNSPECIFIED.)
CURVE()
GEOMETRIC_REPRESENTATION_ITEM()
RATIONAL_B_SPLINE_CURVE((1.,1.,1.,1.,1.,1.,1.,1.,1.,1.,1.,1.,1.,1.,1.,1.,
1.,1.,1.,1.,1.,1.,1.,1.,1.,1.,1.,1.,1.,1.,1.,1.,1.,1.,1.,1.,1.,1.,1.,1.,
1.,1.,1.,1.,1.,1.,1.,1.,1.,1.,1.,1.,1.,1.,1.,1.,1.,1.,1.,1.,1.,1.,1.,1.,
1.,1.,1.,1.,1.,1.,1.,1.,1.,1.,1.,1.,1.,1.,1.,1.,1.,1.,1.,1.,1.,1.,1.,1.,
1.,1.,1.,1.,1.,1.,1.,1.,1.,1.,1.,1.,1.,1.,1.,1.,1.,1.,1.,1.,1.,1.,1.,1.,
1.,1.,1.,1.,1.,1.,1.,1.,1.,1.,1.,1.,1.,1.,1.,1.,1.,1.,1.,1.,1.,1.,1.,1.,
1.,1.,1.,1.,1.,1.,1.,1.,1.,1.,1.,1.,1.,1.,1.,1.,1.,1.,1.,1.,1.,1.,1.,1.,
1.,1.,1.,1.,1.,1.,1.,1.,1.,1.,1.,1.,1.,1.,1.,1.,1.,1.,1.,1.,1.,1.,1.,1.,
1.,1.,1.,1.,1.,1.,1.,1.,1.,1.))
REPRESENTATION_ITEM('')
);
#596=(
BOUNDED_CURVE()
B_SPLINE_CURVE(5,(#136824,#136825,#136826,#136827,#136828,#136829,#136830,
#136831,#136832,#136833,#136834,#136835,#136836,#136837,#136838,#136839,
#136840,#136841,#136842,#136843,#136844,#136845,#136846,#136847,#136848,
#136849,#136850,#136851,#136852,#136853,#136854,#136855,#136856,#136857,
#136858,#136859,#136860,#136861,#136862,#136863,#136864,#136865,#136866,
#136867,#136868,#136869,#136870,#136871,#136872,#136873,#136874,#136875,
#136876,#136877,#136878,#136879,#136880,#136881,#136882,#136883,#136884,
#136885,#136886,#136887,#136888,#136889,#136890,#136891,#136892,#136893,
#136894,#136895,#136896,#136897,#136898,#136899,#136900,#136901,#136902,
#136903,#136904,#136905,#136906,#136907,#136908,#136909,#136910,#136911,
#136912,#136913,#136914,#136915,#136916,#136917,#136918,#136919,#136920,
#136921,#136922,#136923,#136924,#136925,#136926,#136927,#136928,#136929,
#136930,#136931,#136932,#136933,#136934,#136935,#136936,#136937,#136938,
#136939,#136940,#136941,#136942,#136943,#136944,#136945,#136946,#136947,
#136948,#136949,#136950,#136951,#136952,#136953,#136954,#136955,#136956,
#136957,#136958,#136959,#136960,#136961,#136962,#136963,#136964,#136965,
#136966,#136967,#136968,#136969,#136970,#136971,#136972,#136973,#136974,
#136975,#136976,#136977,#136978,#136979,#136980,#136981,#136982,#136983,
#136984,#136985,#136986,#136987,#136988,#136989,#136990,#136991,#136992,
#136993,#136994,#136995,#136996,#136997,#136998,#136999,#137000,#137001,
#137002,#137003,#137004,#137005,#137006,#137007,#137008,#137009,#137010,
#137011,#137012,#137013,#137014,#137015,#137016,#137017),.UNSPECIFIED.,
 .F.,.F.)
B_SPLINE_CURVE_WITH_KNOTS((6,1,1,1,1,1,1,1,1,1,1,1,1,1,1,1,1,1,1,1,1,1,
1,1,1,1,1,1,1,1,1,1,1,1,1,1,1,1,1,1,1,1,1,1,1,1,1,1,1,1,1,1,1,1,1,1,1,1,
1,1,1,1,1,1,1,1,1,1,1,1,1,1,1,1,1,1,1,1,1,1,1,1,1,1,1,1,1,1,1,1,1,1,1,1,
1,1,1,1,1,1,1,1,1,1,1,1,1,1,1,1,1,1,1,1,1,1,1,1,1,1,1,1,1,1,1,1,1,1,1,1,
1,1,1,1,1,1,1,1,1,1,1,1,1,1,1,1,1,1,1,1,1,1,1,1,1,1,1,1,1,1,1,1,1,1,1,1,
1,1,1,1,1,1,1,1,1,1,1,1,1,1,1,1,1,1,1,1,1,1,1,6),(-0.941429844438045,-0.940000000000001,
-0.935000000000001,-0.930000000000001,-0.925000000000001,-0.920000000000001,
-0.915000000000001,-0.910000000000001,-0.905000000000001,-0.900000000000001,
-0.895000000000001,-0.890000000000001,-0.885000000000001,-0.880000000000001,
-0.875000000000001,-0.870000000000001,-0.865000000000001,-0.860000000000001,
-0.855000000000001,-0.850000000000001,-0.845000000000001,-0.840000000000001,
-0.835000000000001,-0.830000000000001,-0.825000000000001,-0.820000000000001,
-0.815000000000001,-0.810000000000001,-0.805000000000001,-0.800000000000001,
-0.795000000000001,-0.790000000000001,-0.785000000000001,-0.780000000000001,
-0.775000000000001,-0.770000000000001,-0.765000000000001,-0.760000000000001,
-0.755000000000001,-0.750000000000001,-0.745000000000001,-0.740000000000001,
-0.735000000000001,-0.730000000000001,-0.725000000000001,-0.720000000000001,
-0.715000000000001,-0.710000000000001,-0.705000000000001,-0.700000000000001,
-0.695000000000001,-0.690000000000001,-0.685,-0.68,-0.675,-0.67,-0.665,
-0.66,-0.655,-0.65,-0.645,-0.64,-0.635,-0.63,-0.625,-0.62,-0.615,-0.61,
-0.605,-0.6,-0.595,-0.59,-0.585,-0.58,-0.575,-0.57,-0.565,-0.56,-0.555,
-0.55,-0.545,-0.54,-0.535,-0.53,-0.525,-0.52,-0.515,-0.51,-0.505,-0.5,-0.495,
-0.49,-0.485,-0.48,-0.475,-0.47,-0.465,-0.46,-0.455,-0.45,-0.445,-0.44,
-0.435,-0.43,-0.425,-0.42,-0.415,-0.41,-0.405,-0.4,-0.395,-0.39,-0.385,
-0.38,-0.375,-0.37,-0.365,-0.36,-0.355,-0.35,-0.345,-0.34,-0.335,-0.33,
-0.325,-0.32,-0.315,-0.31,-0.305,-0.3,-0.295,-0.29,-0.285,-0.28,-0.275,
-0.27,-0.265,-0.26,-0.255,-0.25,-0.245,-0.24,-0.235,-0.23,-0.225,-0.22,
-0.215,-0.21,-0.205,-0.2,-0.195,-0.19,-0.185,-0.18,-0.175,-0.17,-0.165,
-0.16,-0.155,-0.15,-0.145,-0.14,-0.135,-0.13,-0.125,-0.12,-0.115,-0.11,
-0.105,-0.1,-0.095,-0.09,-0.085,-0.08,-0.075,-0.07,-0.065,-0.06,-0.055,
-0.05,-0.045,-0.04,-0.035,-0.03,-0.025,-0.02,-0.015,-0.01,-0.005,0.),
 .UNSPECIFIED.)
CURVE()
GEOMETRIC_REPRESENTATION_ITEM()
RATIONAL_B_SPLINE_CURVE((1.,1.,1.,1.,1.,1.,1.,1.,1.,1.,1.,1.,1.,1.,1.,1.,
1.,1.,1.,1.,1.,1.,1.,1.,1.,1.,1.,1.,1.,1.,1.,1.,1.,1.,1.,1.,1.,1.,1.,1.,
1.,1.,1.,1.,1.,1.,1.,1.,1.,1.,1.,1.,1.,1.,1.,1.,1.,1.,1.,1.,1.,1.,1.,1.,
1.,1.,1.,1.,1.,1.,1.,1.,1.,1.,1.,1.,1.,1.,1.,1.,1.,1.,1.,1.,1.,1.,1.,1.,
1.,1.,1.,1.,1.,1.,1.,1.,1.,1.,1.,1.,1.,1.,1.,1.,1.,1.,1.,1.,1.,1.,1.,1.,
1.,1.,1.,1.,1.,1.,1.,1.,1.,1.,1.,1.,1.,1.,1.,1.,1.,1.,1.,1.,1.,1.,1.,1.,
1.,1.,1.,1.,1.,1.,1.,1.,1.,1.,1.,1.,1.,1.,1.,1.,1.,1.,1.,1.,1.,1.,1.,1.,
1.,1.,1.,1.,1.,1.,1.,1.,1.,1.,1.,1.,1.,1.,1.,1.,1.,1.,1.,1.,1.,1.,1.,1.,
1.,1.,1.,1.,1.,1.,1.,1.,1.,1.))
REPRESENTATION_ITEM('')
);
#597=(
BOUNDED_CURVE()
B_SPLINE_CURVE(5,(#137429,#137430,#137431,#137432,#137433,#137434,#137435,
#137436,#137437,#137438,#137439,#137440,#137441,#137442,#137443,#137444,
#137445,#137446,#137447,#137448,#137449,#137450,#137451,#137452,#137453,
#137454,#137455,#137456,#137457,#137458,#137459,#137460,#137461,#137462,
#137463,#137464,#137465,#137466,#137467,#137468,#137469,#137470,#137471,
#137472,#137473,#137474,#137475,#137476,#137477,#137478,#137479,#137480,
#137481,#137482,#137483,#137484,#137485,#137486,#137487,#137488,#137489,
#137490,#137491,#137492,#137493,#137494,#137495,#137496,#137497,#137498,
#137499,#137500,#137501,#137502,#137503,#137504,#137505,#137506,#137507,
#137508,#137509,#137510,#137511,#137512,#137513,#137514,#137515,#137516,
#137517,#137518,#137519,#137520,#137521,#137522,#137523,#137524,#137525,
#137526,#137527,#137528,#137529,#137530,#137531,#137532,#137533,#137534,
#137535,#137536,#137537,#137538,#137539,#137540,#137541,#137542,#137543,
#137544,#137545,#137546,#137547,#137548,#137549,#137550,#137551,#137552,
#137553,#137554,#137555,#137556,#137557,#137558,#137559,#137560,#137561,
#137562,#137563,#137564,#137565,#137566,#137567,#137568,#137569,#137570,
#137571,#137572,#137573,#137574,#137575,#137576,#137577,#137578,#137579,
#137580,#137581,#137582,#137583,#137584,#137585,#137586,#137587,#137588,
#137589,#137590,#137591,#137592,#137593,#137594,#137595,#137596,#137597,
#137598,#137599,#137600,#137601,#137602,#137603,#137604,#137605,#137606,
#137607,#137608,#137609,#137610,#137611,#137612,#137613,#137614,#137615,
#137616,#137617,#137618,#137619,#137620,#137621,#137622),.UNSPECIFIED.,
 .F.,.F.)
B_SPLINE_CURVE_WITH_KNOTS((6,1,1,1,1,1,1,1,1,1,1,1,1,1,1,1,1,1,1,1,1,1,
1,1,1,1,1,1,1,1,1,1,1,1,1,1,1,1,1,1,1,1,1,1,1,1,1,1,1,1,1,1,1,1,1,1,1,1,
1,1,1,1,1,1,1,1,1,1,1,1,1,1,1,1,1,1,1,1,1,1,1,1,1,1,1,1,1,1,1,1,1,1,1,1,
1,1,1,1,1,1,1,1,1,1,1,1,1,1,1,1,1,1,1,1,1,1,1,1,1,1,1,1,1,1,1,1,1,1,1,1,
1,1,1,1,1,1,1,1,1,1,1,1,1,1,1,1,1,1,1,1,1,1,1,1,1,1,1,1,1,1,1,1,1,1,1,1,
1,1,1,1,1,1,1,1,1,1,1,1,1,1,1,1,1,1,1,1,1,1,1,6),(0.,0.005,0.01,0.015,0.02,
0.025,0.03,0.035,0.04,0.045,0.05,0.055,0.06,0.065,0.07,0.075,0.08,0.085,
0.09,0.095,0.1,0.105,0.11,0.115,0.12,0.125,0.13,0.135,0.14,0.145,0.15,0.155,
0.16,0.165,0.17,0.175,0.18,0.185,0.19,0.195,0.2,0.205,0.21,0.215,0.22,0.225,
0.23,0.235,0.24,0.245,0.25,0.255,0.26,0.265,0.27,0.275,0.28,0.285,0.29,
0.295,0.3,0.305,0.31,0.315,0.32,0.325,0.33,0.335,0.34,0.345,0.35,0.355,
0.36,0.365,0.37,0.375,0.38,0.385,0.39,0.395,0.4,0.405,0.41,0.415,0.42,0.425,
0.43,0.435,0.44,0.445,0.45,0.455,0.46,0.465,0.47,0.475,0.48,0.485,0.49,
0.495,0.5,0.505,0.51,0.515,0.52,0.525,0.53,0.535,0.54,0.545,0.55,0.555,
0.56,0.565,0.57,0.575,0.58,0.585,0.59,0.595,0.6,0.605,0.61,0.615,0.62,0.625,
0.63,0.635,0.64,0.645,0.65,0.655,0.66,0.665,0.67,0.675,0.68,0.685,0.690000000000001,
0.695000000000001,0.700000000000001,0.705000000000001,0.710000000000001,
0.715000000000001,0.720000000000001,0.725000000000001,0.730000000000001,
0.735000000000001,0.740000000000001,0.745000000000001,0.750000000000001,
0.755000000000001,0.760000000000001,0.765000000000001,0.770000000000001,
0.775000000000001,0.780000000000001,0.785000000000001,0.790000000000001,
0.795000000000001,0.800000000000001,0.805000000000001,0.810000000000001,
0.815000000000001,0.820000000000001,0.825000000000001,0.830000000000001,
0.835000000000001,0.840000000000001,0.845000000000001,0.850000000000001,
0.855000000000001,0.860000000000001,0.865000000000001,0.870000000000001,
0.875000000000001,0.880000000000001,0.885000000000001,0.890000000000001,
0.895000000000001,0.900000000000001,0.905000000000001,0.910000000000001,
0.915000000000001,0.920000000000001,0.925000000000001,0.930000000000001,
0.935000000000001,0.940000000000001,0.941429844437968),.UNSPECIFIED.)
CURVE()
GEOMETRIC_REPRESENTATION_ITEM()
RATIONAL_B_SPLINE_CURVE((1.,1.,1.,1.,1.,1.,1.,1.,1.,1.,1.,1.,1.,1.,1.,1.,
1.,1.,1.,1.,1.,1.,1.,1.,1.,1.,1.,1.,1.,1.,1.,1.,1.,1.,1.,1.,1.,1.,1.,1.,
1.,1.,1.,1.,1.,1.,1.,1.,1.,1.,1.,1.,1.,1.,1.,1.,1.,1.,1.,1.,1.,1.,1.,1.,
1.,1.,1.,1.,1.,1.,1.,1.,1.,1.,1.,1.,1.,1.,1.,1.,1.,1.,1.,1.,1.,1.,1.,1.,
1.,1.,1.,1.,1.,1.,1.,1.,1.,1.,1.,1.,1.,1.,1.,1.,1.,1.,1.,1.,1.,1.,1.,1.,
1.,1.,1.,1.,1.,1.,1.,1.,1.,1.,1.,1.,1.,1.,1.,1.,1.,1.,1.,1.,1.,1.,1.,1.,
1.,1.,1.,1.,1.,1.,1.,1.,1.,1.,1.,1.,1.,1.,1.,1.,1.,1.,1.,1.,1.,1.,1.,1.,
1.,1.,1.,1.,1.,1.,1.,1.,1.,1.,1.,1.,1.,1.,1.,1.,1.,1.,1.,1.,1.,1.,1.,1.,
1.,1.,1.,1.,1.,1.,1.,1.,1.,1.))
REPRESENTATION_ITEM('')
);
#598=(
BOUNDED_CURVE()
B_SPLINE_CURVE(5,(#137625,#137626,#137627,#137628,#137629,#137630,#137631,
#137632,#137633,#137634,#137635,#137636,#137637,#137638,#137639,#137640,
#137641,#137642,#137643,#137644,#137645,#137646,#137647,#137648,#137649,
#137650,#137651,#137652,#137653,#137654,#137655,#137656,#137657,#137658,
#137659,#137660,#137661,#137662,#137663,#137664,#137665,#137666,#137667,
#137668,#137669,#137670,#137671,#137672,#137673,#137674,#137675,#137676,
#137677,#137678,#137679,#137680,#137681,#137682,#137683,#137684,#137685,
#137686,#137687,#137688,#137689,#137690,#137691,#137692,#137693,#137694,
#137695,#137696,#137697,#137698,#137699,#137700,#137701,#137702,#137703,
#137704,#137705,#137706,#137707,#137708,#137709,#137710,#137711,#137712,
#137713,#137714,#137715,#137716,#137717,#137718,#137719,#137720,#137721,
#137722,#137723,#137724,#137725,#137726,#137727,#137728,#137729,#137730,
#137731,#137732,#137733,#137734,#137735,#137736,#137737,#137738,#137739,
#137740,#137741,#137742,#137743,#137744,#137745,#137746,#137747,#137748,
#137749,#137750,#137751,#137752,#137753,#137754,#137755,#137756,#137757,
#137758,#137759,#137760,#137761,#137762,#137763,#137764,#137765,#137766,
#137767,#137768,#137769,#137770,#137771,#137772,#137773,#137774,#137775,
#137776,#137777,#137778,#137779,#137780,#137781,#137782,#137783,#137784,
#137785,#137786,#137787,#137788,#137789,#137790,#137791,#137792,#137793,
#137794,#137795,#137796,#137797,#137798,#137799,#137800,#137801,#137802,
#137803,#137804,#137805,#137806,#137807,#137808,#137809,#137810,#137811,
#137812,#137813,#137814,#137815,#137816,#137817,#137818),.UNSPECIFIED.,
 .F.,.F.)
B_SPLINE_CURVE_WITH_KNOTS((6,1,1,1,1,1,1,1,1,1,1,1,1,1,1,1,1,1,1,1,1,1,
1,1,1,1,1,1,1,1,1,1,1,1,1,1,1,1,1,1,1,1,1,1,1,1,1,1,1,1,1,1,1,1,1,1,1,1,
1,1,1,1,1,1,1,1,1,1,1,1,1,1,1,1,1,1,1,1,1,1,1,1,1,1,1,1,1,1,1,1,1,1,1,1,
1,1,1,1,1,1,1,1,1,1,1,1,1,1,1,1,1,1,1,1,1,1,1,1,1,1,1,1,1,1,1,1,1,1,1,1,
1,1,1,1,1,1,1,1,1,1,1,1,1,1,1,1,1,1,1,1,1,1,1,1,1,1,1,1,1,1,1,1,1,1,1,1,
1,1,1,1,1,1,1,1,1,1,1,1,1,1,1,1,1,1,1,1,1,1,1,6),(-0.941429844437971,-0.940000000000001,
-0.935000000000001,-0.930000000000001,-0.925000000000001,-0.920000000000001,
-0.915000000000001,-0.910000000000001,-0.905000000000001,-0.900000000000001,
-0.895000000000001,-0.890000000000001,-0.885000000000001,-0.880000000000001,
-0.875000000000001,-0.870000000000001,-0.865000000000001,-0.860000000000001,
-0.855000000000001,-0.850000000000001,-0.845000000000001,-0.840000000000001,
-0.835000000000001,-0.830000000000001,-0.825000000000001,-0.820000000000001,
-0.815000000000001,-0.810000000000001,-0.805000000000001,-0.800000000000001,
-0.795000000000001,-0.790000000000001,-0.785000000000001,-0.780000000000001,
-0.775000000000001,-0.770000000000001,-0.765000000000001,-0.760000000000001,
-0.755000000000001,-0.750000000000001,-0.745000000000001,-0.740000000000001,
-0.735000000000001,-0.730000000000001,-0.725000000000001,-0.720000000000001,
-0.715000000000001,-0.710000000000001,-0.705000000000001,-0.700000000000001,
-0.695000000000001,-0.690000000000001,-0.685,-0.68,-0.675,-0.67,-0.665,
-0.66,-0.655,-0.65,-0.645,-0.64,-0.635,-0.63,-0.625,-0.62,-0.615,-0.61,
-0.605,-0.6,-0.595,-0.59,-0.585,-0.58,-0.575,-0.57,-0.565,-0.56,-0.555,
-0.55,-0.545,-0.54,-0.535,-0.53,-0.525,-0.52,-0.515,-0.51,-0.505,-0.5,-0.495,
-0.49,-0.485,-0.48,-0.475,-0.47,-0.465,-0.46,-0.455,-0.45,-0.445,-0.44,
-0.435,-0.43,-0.425,-0.42,-0.415,-0.41,-0.405,-0.4,-0.395,-0.39,-0.385,
-0.38,-0.375,-0.37,-0.365,-0.36,-0.355,-0.35,-0.345,-0.34,-0.335,-0.33,
-0.325,-0.32,-0.315,-0.31,-0.305,-0.3,-0.295,-0.29,-0.285,-0.28,-0.275,
-0.27,-0.265,-0.26,-0.255,-0.25,-0.245,-0.24,-0.235,-0.23,-0.225,-0.22,
-0.215,-0.21,-0.205,-0.2,-0.195,-0.19,-0.185,-0.18,-0.175,-0.17,-0.165,
-0.16,-0.155,-0.15,-0.145,-0.14,-0.135,-0.13,-0.125,-0.12,-0.115,-0.11,
-0.105,-0.1,-0.095,-0.09,-0.085,-0.08,-0.075,-0.07,-0.065,-0.06,-0.055,
-0.05,-0.045,-0.04,-0.035,-0.03,-0.025,-0.02,-0.015,-0.01,-0.005,0.),
 .UNSPECIFIED.)
CURVE()
GEOMETRIC_REPRESENTATION_ITEM()
RATIONAL_B_SPLINE_CURVE((1.,1.,1.,1.,1.,1.,1.,1.,1.,1.,1.,1.,1.,1.,1.,1.,
1.,1.,1.,1.,1.,1.,1.,1.,1.,1.,1.,1.,1.,1.,1.,1.,1.,1.,1.,1.,1.,1.,1.,1.,
1.,1.,1.,1.,1.,1.,1.,1.,1.,1.,1.,1.,1.,1.,1.,1.,1.,1.,1.,1.,1.,1.,1.,1.,
1.,1.,1.,1.,1.,1.,1.,1.,1.,1.,1.,1.,1.,1.,1.,1.,1.,1.,1.,1.,1.,1.,1.,1.,
1.,1.,1.,1.,1.,1.,1.,1.,1.,1.,1.,1.,1.,1.,1.,1.,1.,1.,1.,1.,1.,1.,1.,1.,
1.,1.,1.,1.,1.,1.,1.,1.,1.,1.,1.,1.,1.,1.,1.,1.,1.,1.,1.,1.,1.,1.,1.,1.,
1.,1.,1.,1.,1.,1.,1.,1.,1.,1.,1.,1.,1.,1.,1.,1.,1.,1.,1.,1.,1.,1.,1.,1.,
1.,1.,1.,1.,1.,1.,1.,1.,1.,1.,1.,1.,1.,1.,1.,1.,1.,1.,1.,1.,1.,1.,1.,1.,
1.,1.,1.,1.,1.,1.,1.,1.,1.,1.))
REPRESENTATION_ITEM('')
);
#599=(
BOUNDED_CURVE()
B_SPLINE_CURVE(5,(#138230,#138231,#138232,#138233,#138234,#138235,#138236,
#138237,#138238,#138239,#138240,#138241,#138242,#138243,#138244,#138245,
#138246,#138247,#138248,#138249,#138250,#138251,#138252,#138253,#138254,
#138255,#138256,#138257,#138258,#138259,#138260,#138261,#138262,#138263,
#138264,#138265,#138266,#138267,#138268,#138269,#138270,#138271,#138272,
#138273,#138274,#138275,#138276,#138277,#138278,#138279,#138280,#138281,
#138282,#138283,#138284,#138285,#138286,#138287,#138288,#138289,#138290,
#138291,#138292,#138293,#138294,#138295,#138296,#138297,#138298,#138299,
#138300,#138301,#138302,#138303,#138304,#138305,#138306,#138307,#138308,
#138309,#138310,#138311,#138312,#138313,#138314,#138315,#138316,#138317,
#138318,#138319,#138320,#138321,#138322,#138323,#138324,#138325,#138326,
#138327,#138328,#138329,#138330,#138331,#138332,#138333,#138334,#138335,
#138336,#138337,#138338,#138339,#138340,#138341,#138342,#138343,#138344,
#138345,#138346,#138347,#138348,#138349,#138350,#138351,#138352,#138353,
#138354,#138355,#138356,#138357,#138358,#138359,#138360,#138361,#138362,
#138363,#138364,#138365,#138366,#138367,#138368,#138369,#138370,#138371,
#138372,#138373,#138374,#138375,#138376,#138377,#138378,#138379,#138380,
#138381,#138382,#138383,#138384,#138385,#138386,#138387,#138388,#138389,
#138390,#138391,#138392,#138393,#138394,#138395,#138396,#138397,#138398,
#138399,#138400,#138401,#138402,#138403,#138404,#138405,#138406,#138407,
#138408,#138409,#138410,#138411,#138412,#138413,#138414,#138415,#138416,
#138417,#138418,#138419,#138420,#138421,#138422,#138423),.UNSPECIFIED.,
 .F.,.F.)
B_SPLINE_CURVE_WITH_KNOTS((6,1,1,1,1,1,1,1,1,1,1,1,1,1,1,1,1,1,1,1,1,1,
1,1,1,1,1,1,1,1,1,1,1,1,1,1,1,1,1,1,1,1,1,1,1,1,1,1,1,1,1,1,1,1,1,1,1,1,
1,1,1,1,1,1,1,1,1,1,1,1,1,1,1,1,1,1,1,1,1,1,1,1,1,1,1,1,1,1,1,1,1,1,1,1,
1,1,1,1,1,1,1,1,1,1,1,1,1,1,1,1,1,1,1,1,1,1,1,1,1,1,1,1,1,1,1,1,1,1,1,1,
1,1,1,1,1,1,1,1,1,1,1,1,1,1,1,1,1,1,1,1,1,1,1,1,1,1,1,1,1,1,1,1,1,1,1,1,
1,1,1,1,1,1,1,1,1,1,1,1,1,1,1,1,1,1,1,1,1,1,1,6),(0.,0.005,0.01,0.015,0.02,
0.025,0.03,0.035,0.04,0.045,0.05,0.055,0.06,0.065,0.07,0.075,0.08,0.085,
0.09,0.095,0.1,0.105,0.11,0.115,0.12,0.125,0.13,0.135,0.14,0.145,0.15,0.155,
0.16,0.165,0.17,0.175,0.18,0.185,0.19,0.195,0.2,0.205,0.21,0.215,0.22,0.225,
0.23,0.235,0.24,0.245,0.25,0.255,0.26,0.265,0.27,0.275,0.28,0.285,0.29,
0.295,0.3,0.305,0.31,0.315,0.32,0.325,0.33,0.335,0.34,0.345,0.35,0.355,
0.36,0.365,0.37,0.375,0.38,0.385,0.39,0.395,0.4,0.405,0.41,0.415,0.42,0.425,
0.43,0.435,0.44,0.445,0.45,0.455,0.46,0.465,0.47,0.475,0.48,0.485,0.49,
0.495,0.5,0.505,0.51,0.515,0.52,0.525,0.53,0.535,0.54,0.545,0.55,0.555,
0.56,0.565,0.57,0.575,0.58,0.585,0.59,0.595,0.6,0.605,0.61,0.615,0.62,0.625,
0.63,0.635,0.64,0.645,0.65,0.655,0.66,0.665,0.67,0.675,0.68,0.685,0.690000000000001,
0.695000000000001,0.700000000000001,0.705000000000001,0.710000000000001,
0.715000000000001,0.720000000000001,0.725000000000001,0.730000000000001,
0.735000000000001,0.740000000000001,0.745000000000001,0.750000000000001,
0.755000000000001,0.760000000000001,0.765000000000001,0.770000000000001,
0.775000000000001,0.780000000000001,0.785000000000001,0.790000000000001,
0.795000000000001,0.800000000000001,0.805000000000001,0.810000000000001,
0.815000000000001,0.820000000000001,0.825000000000001,0.830000000000001,
0.835000000000001,0.840000000000001,0.845000000000001,0.850000000000001,
0.855000000000001,0.860000000000001,0.865000000000001,0.870000000000001,
0.875000000000001,0.880000000000001,0.885000000000001,0.890000000000001,
0.895000000000001,0.900000000000001,0.905000000000001,0.910000000000001,
0.915000000000001,0.920000000000001,0.925000000000001,0.930000000000001,
0.935000000000001,0.940000000000001,0.941429844438107),.UNSPECIFIED.)
CURVE()
GEOMETRIC_REPRESENTATION_ITEM()
RATIONAL_B_SPLINE_CURVE((1.,1.,1.,1.,1.,1.,1.,1.,1.,1.,1.,1.,1.,1.,1.,1.,
1.,1.,1.,1.,1.,1.,1.,1.,1.,1.,1.,1.,1.,1.,1.,1.,1.,1.,1.,1.,1.,1.,1.,1.,
1.,1.,1.,1.,1.,1.,1.,1.,1.,1.,1.,1.,1.,1.,1.,1.,1.,1.,1.,1.,1.,1.,1.,1.,
1.,1.,1.,1.,1.,1.,1.,1.,1.,1.,1.,1.,1.,1.,1.,1.,1.,1.,1.,1.,1.,1.,1.,1.,
1.,1.,1.,1.,1.,1.,1.,1.,1.,1.,1.,1.,1.,1.,1.,1.,1.,1.,1.,1.,1.,1.,1.,1.,
1.,1.,1.,1.,1.,1.,1.,1.,1.,1.,1.,1.,1.,1.,1.,1.,1.,1.,1.,1.,1.,1.,1.,1.,
1.,1.,1.,1.,1.,1.,1.,1.,1.,1.,1.,1.,1.,1.,1.,1.,1.,1.,1.,1.,1.,1.,1.,1.,
1.,1.,1.,1.,1.,1.,1.,1.,1.,1.,1.,1.,1.,1.,1.,1.,1.,1.,1.,1.,1.,1.,1.,1.,
1.,1.,1.,1.,1.,1.,1.,1.,1.,1.))
REPRESENTATION_ITEM('')
);
#600=(
BOUNDED_CURVE()
B_SPLINE_CURVE(5,(#138426,#138427,#138428,#138429,#138430,#138431,#138432,
#138433,#138434,#138435,#138436,#138437,#138438,#138439,#138440,#138441,
#138442,#138443,#138444,#138445,#138446,#138447,#138448,#138449,#138450,
#138451,#138452,#138453,#138454,#138455,#138456,#138457,#138458,#138459,
#138460,#138461,#138462,#138463,#138464,#138465,#138466,#138467,#138468,
#138469,#138470,#138471,#138472,#138473,#138474,#138475,#138476,#138477,
#138478,#138479,#138480,#138481,#138482,#138483,#138484,#138485,#138486,
#138487,#138488,#138489,#138490,#138491,#138492,#138493,#138494,#138495,
#138496,#138497,#138498,#138499,#138500,#138501,#138502,#138503,#138504,
#138505,#138506,#138507,#138508,#138509,#138510,#138511,#138512,#138513,
#138514,#138515,#138516,#138517,#138518,#138519,#138520,#138521,#138522,
#138523,#138524,#138525,#138526,#138527,#138528,#138529,#138530,#138531,
#138532,#138533,#138534,#138535,#138536,#138537,#138538,#138539,#138540,
#138541,#138542,#138543,#138544,#138545,#138546,#138547,#138548,#138549,
#138550,#138551,#138552,#138553,#138554,#138555,#138556,#138557,#138558,
#138559,#138560,#138561,#138562,#138563,#138564,#138565,#138566,#138567,
#138568,#138569,#138570,#138571,#138572,#138573,#138574,#138575,#138576,
#138577,#138578,#138579,#138580,#138581,#138582,#138583,#138584,#138585,
#138586,#138587,#138588,#138589,#138590,#138591,#138592,#138593,#138594,
#138595,#138596,#138597,#138598,#138599,#138600,#138601,#138602,#138603,
#138604,#138605,#138606,#138607,#138608,#138609,#138610,#138611,#138612,
#138613,#138614,#138615,#138616,#138617,#138618,#138619),.UNSPECIFIED.,
 .F.,.F.)
B_SPLINE_CURVE_WITH_KNOTS((6,1,1,1,1,1,1,1,1,1,1,1,1,1,1,1,1,1,1,1,1,1,
1,1,1,1,1,1,1,1,1,1,1,1,1,1,1,1,1,1,1,1,1,1,1,1,1,1,1,1,1,1,1,1,1,1,1,1,
1,1,1,1,1,1,1,1,1,1,1,1,1,1,1,1,1,1,1,1,1,1,1,1,1,1,1,1,1,1,1,1,1,1,1,1,
1,1,1,1,1,1,1,1,1,1,1,1,1,1,1,1,1,1,1,1,1,1,1,1,1,1,1,1,1,1,1,1,1,1,1,1,
1,1,1,1,1,1,1,1,1,1,1,1,1,1,1,1,1,1,1,1,1,1,1,1,1,1,1,1,1,1,1,1,1,1,1,1,
1,1,1,1,1,1,1,1,1,1,1,1,1,1,1,1,1,1,1,1,1,1,1,6),(-0.941429844438107,-0.940000000000001,
-0.935000000000001,-0.930000000000001,-0.925000000000001,-0.920000000000001,
-0.915000000000001,-0.910000000000001,-0.905000000000001,-0.900000000000001,
-0.895000000000001,-0.890000000000001,-0.885000000000001,-0.880000000000001,
-0.875000000000001,-0.870000000000001,-0.865000000000001,-0.860000000000001,
-0.855000000000001,-0.850000000000001,-0.845000000000001,-0.840000000000001,
-0.835000000000001,-0.830000000000001,-0.825000000000001,-0.820000000000001,
-0.815000000000001,-0.810000000000001,-0.805000000000001,-0.800000000000001,
-0.795000000000001,-0.790000000000001,-0.785000000000001,-0.780000000000001,
-0.775000000000001,-0.770000000000001,-0.765000000000001,-0.760000000000001,
-0.755000000000001,-0.750000000000001,-0.745000000000001,-0.740000000000001,
-0.735000000000001,-0.730000000000001,-0.725000000000001,-0.720000000000001,
-0.715000000000001,-0.710000000000001,-0.705000000000001,-0.700000000000001,
-0.695000000000001,-0.690000000000001,-0.685,-0.68,-0.675,-0.67,-0.665,
-0.66,-0.655,-0.65,-0.645,-0.64,-0.635,-0.63,-0.625,-0.62,-0.615,-0.61,
-0.605,-0.6,-0.595,-0.59,-0.585,-0.58,-0.575,-0.57,-0.565,-0.56,-0.555,
-0.55,-0.545,-0.54,-0.535,-0.53,-0.525,-0.52,-0.515,-0.51,-0.505,-0.5,-0.495,
-0.49,-0.485,-0.48,-0.475,-0.47,-0.465,-0.46,-0.455,-0.45,-0.445,-0.44,
-0.435,-0.43,-0.425,-0.42,-0.415,-0.41,-0.405,-0.4,-0.395,-0.39,-0.385,
-0.38,-0.375,-0.37,-0.365,-0.36,-0.355,-0.35,-0.345,-0.34,-0.335,-0.33,
-0.325,-0.32,-0.315,-0.31,-0.305,-0.3,-0.295,-0.29,-0.285,-0.28,-0.275,
-0.27,-0.265,-0.26,-0.255,-0.25,-0.245,-0.24,-0.235,-0.23,-0.225,-0.22,
-0.215,-0.21,-0.205,-0.2,-0.195,-0.19,-0.185,-0.18,-0.175,-0.17,-0.165,
-0.16,-0.155,-0.15,-0.145,-0.14,-0.135,-0.13,-0.125,-0.12,-0.115,-0.11,
-0.105,-0.1,-0.095,-0.09,-0.085,-0.08,-0.075,-0.07,-0.065,-0.06,-0.055,
-0.05,-0.045,-0.04,-0.035,-0.03,-0.025,-0.02,-0.015,-0.01,-0.005,0.),
 .UNSPECIFIED.)
CURVE()
GEOMETRIC_REPRESENTATION_ITEM()
RATIONAL_B_SPLINE_CURVE((1.,1.,1.,1.,1.,1.,1.,1.,1.,1.,1.,1.,1.,1.,1.,1.,
1.,1.,1.,1.,1.,1.,1.,1.,1.,1.,1.,1.,1.,1.,1.,1.,1.,1.,1.,1.,1.,1.,1.,1.,
1.,1.,1.,1.,1.,1.,1.,1.,1.,1.,1.,1.,1.,1.,1.,1.,1.,1.,1.,1.,1.,1.,1.,1.,
1.,1.,1.,1.,1.,1.,1.,1.,1.,1.,1.,1.,1.,1.,1.,1.,1.,1.,1.,1.,1.,1.,1.,1.,
1.,1.,1.,1.,1.,1.,1.,1.,1.,1.,1.,1.,1.,1.,1.,1.,1.,1.,1.,1.,1.,1.,1.,1.,
1.,1.,1.,1.,1.,1.,1.,1.,1.,1.,1.,1.,1.,1.,1.,1.,1.,1.,1.,1.,1.,1.,1.,1.,
1.,1.,1.,1.,1.,1.,1.,1.,1.,1.,1.,1.,1.,1.,1.,1.,1.,1.,1.,1.,1.,1.,1.,1.,
1.,1.,1.,1.,1.,1.,1.,1.,1.,1.,1.,1.,1.,1.,1.,1.,1.,1.,1.,1.,1.,1.,1.,1.,
1.,1.,1.,1.,1.,1.,1.,1.,1.,1.))
REPRESENTATION_ITEM('')
);
#601=(
BOUNDED_CURVE()
B_SPLINE_CURVE(5,(#139031,#139032,#139033,#139034,#139035,#139036,#139037,
#139038,#139039,#139040,#139041,#139042,#139043,#139044,#139045,#139046,
#139047,#139048,#139049,#139050,#139051,#139052,#139053,#139054,#139055,
#139056,#139057,#139058,#139059,#139060,#139061,#139062,#139063,#139064,
#139065,#139066,#139067,#139068,#139069,#139070,#139071,#139072,#139073,
#139074,#139075,#139076,#139077,#139078,#139079,#139080,#139081,#139082,
#139083,#139084,#139085,#139086,#139087,#139088,#139089,#139090,#139091,
#139092,#139093,#139094,#139095,#139096,#139097,#139098,#139099,#139100,
#139101,#139102,#139103,#139104,#139105,#139106,#139107,#139108,#139109,
#139110,#139111,#139112,#139113,#139114,#139115,#139116,#139117,#139118,
#139119,#139120,#139121,#139122,#139123,#139124,#139125,#139126,#139127,
#139128,#139129,#139130,#139131,#139132,#139133,#139134,#139135,#139136,
#139137,#139138,#139139,#139140,#139141,#139142,#139143,#139144,#139145,
#139146,#139147,#139148,#139149,#139150,#139151,#139152,#139153,#139154,
#139155,#139156,#139157,#139158,#139159,#139160,#139161,#139162,#139163,
#139164,#139165,#139166,#139167,#139168,#139169,#139170,#139171,#139172,
#139173,#139174,#139175,#139176,#139177,#139178,#139179,#139180,#139181,
#139182,#139183,#139184,#139185,#139186,#139187,#139188,#139189,#139190,
#139191,#139192,#139193,#139194,#139195,#139196,#139197,#139198,#139199,
#139200,#139201,#139202,#139203,#139204,#139205,#139206,#139207,#139208,
#139209,#139210,#139211,#139212,#139213,#139214,#139215,#139216,#139217,
#139218,#139219,#139220,#139221,#139222,#139223,#139224),.UNSPECIFIED.,
 .F.,.F.)
B_SPLINE_CURVE_WITH_KNOTS((6,1,1,1,1,1,1,1,1,1,1,1,1,1,1,1,1,1,1,1,1,1,
1,1,1,1,1,1,1,1,1,1,1,1,1,1,1,1,1,1,1,1,1,1,1,1,1,1,1,1,1,1,1,1,1,1,1,1,
1,1,1,1,1,1,1,1,1,1,1,1,1,1,1,1,1,1,1,1,1,1,1,1,1,1,1,1,1,1,1,1,1,1,1,1,
1,1,1,1,1,1,1,1,1,1,1,1,1,1,1,1,1,1,1,1,1,1,1,1,1,1,1,1,1,1,1,1,1,1,1,1,
1,1,1,1,1,1,1,1,1,1,1,1,1,1,1,1,1,1,1,1,1,1,1,1,1,1,1,1,1,1,1,1,1,1,1,1,
1,1,1,1,1,1,1,1,1,1,1,1,1,1,1,1,1,1,1,1,1,1,1,6),(0.,0.005,0.01,0.015,0.02,
0.025,0.03,0.035,0.04,0.045,0.05,0.055,0.06,0.065,0.07,0.075,0.08,0.085,
0.09,0.095,0.1,0.105,0.11,0.115,0.12,0.125,0.13,0.135,0.14,0.145,0.15,0.155,
0.16,0.165,0.17,0.175,0.18,0.185,0.19,0.195,0.2,0.205,0.21,0.215,0.22,0.225,
0.23,0.235,0.24,0.245,0.25,0.255,0.26,0.265,0.27,0.275,0.28,0.285,0.29,
0.295,0.3,0.305,0.31,0.315,0.32,0.325,0.33,0.335,0.34,0.345,0.35,0.355,
0.36,0.365,0.37,0.375,0.38,0.385,0.39,0.395,0.4,0.405,0.41,0.415,0.42,0.425,
0.43,0.435,0.44,0.445,0.45,0.455,0.46,0.465,0.47,0.475,0.48,0.485,0.49,
0.495,0.5,0.505,0.51,0.515,0.52,0.525,0.53,0.535,0.54,0.545,0.55,0.555,
0.56,0.565,0.57,0.575,0.58,0.585,0.59,0.595,0.6,0.605,0.61,0.615,0.62,0.625,
0.63,0.635,0.64,0.645,0.65,0.655,0.66,0.665,0.67,0.675,0.68,0.685,0.690000000000001,
0.695000000000001,0.700000000000001,0.705000000000001,0.710000000000001,
0.715000000000001,0.720000000000001,0.725000000000001,0.730000000000001,
0.735000000000001,0.740000000000001,0.745000000000001,0.750000000000001,
0.755000000000001,0.760000000000001,0.765000000000001,0.770000000000001,
0.775000000000001,0.780000000000001,0.785000000000001,0.790000000000001,
0.795000000000001,0.800000000000001,0.805000000000001,0.810000000000001,
0.815000000000001,0.820000000000001,0.825000000000001,0.830000000000001,
0.835000000000001,0.840000000000001,0.845000000000001,0.850000000000001,
0.855000000000001,0.860000000000001,0.865000000000001,0.870000000000001,
0.875000000000001,0.880000000000001,0.885000000000001,0.890000000000001,
0.895000000000001,0.900000000000001,0.905000000000001,0.910000000000001,
0.915000000000001,0.920000000000001,0.925000000000001,0.930000000000001,
0.935000000000001,0.940000000000001,0.941429844438169),.UNSPECIFIED.)
CURVE()
GEOMETRIC_REPRESENTATION_ITEM()
RATIONAL_B_SPLINE_CURVE((1.,1.,1.,1.,1.,1.,1.,1.,1.,1.,1.,1.,1.,1.,1.,1.,
1.,1.,1.,1.,1.,1.,1.,1.,1.,1.,1.,1.,1.,1.,1.,1.,1.,1.,1.,1.,1.,1.,1.,1.,
1.,1.,1.,1.,1.,1.,1.,1.,1.,1.,1.,1.,1.,1.,1.,1.,1.,1.,1.,1.,1.,1.,1.,1.,
1.,1.,1.,1.,1.,1.,1.,1.,1.,1.,1.,1.,1.,1.,1.,1.,1.,1.,1.,1.,1.,1.,1.,1.,
1.,1.,1.,1.,1.,1.,1.,1.,1.,1.,1.,1.,1.,1.,1.,1.,1.,1.,1.,1.,1.,1.,1.,1.,
1.,1.,1.,1.,1.,1.,1.,1.,1.,1.,1.,1.,1.,1.,1.,1.,1.,1.,1.,1.,1.,1.,1.,1.,
1.,1.,1.,1.,1.,1.,1.,1.,1.,1.,1.,1.,1.,1.,1.,1.,1.,1.,1.,1.,1.,1.,1.,1.,
1.,1.,1.,1.,1.,1.,1.,1.,1.,1.,1.,1.,1.,1.,1.,1.,1.,1.,1.,1.,1.,1.,1.,1.,
1.,1.,1.,1.,1.,1.,1.,1.,1.,1.))
REPRESENTATION_ITEM('')
);
#602=(
BOUNDED_CURVE()
B_SPLINE_CURVE(5,(#139227,#139228,#139229,#139230,#139231,#139232,#139233,
#139234,#139235,#139236,#139237,#139238,#139239,#139240,#139241,#139242,
#139243,#139244,#139245,#139246,#139247,#139248,#139249,#139250,#139251,
#139252,#139253,#139254,#139255,#139256,#139257,#139258,#139259,#139260,
#139261,#139262,#139263,#139264,#139265,#139266,#139267,#139268,#139269,
#139270,#139271,#139272,#139273,#139274,#139275,#139276,#139277,#139278,
#139279,#139280,#139281,#139282,#139283,#139284,#139285,#139286,#139287,
#139288,#139289,#139290,#139291,#139292,#139293,#139294,#139295,#139296,
#139297,#139298,#139299,#139300,#139301,#139302,#139303,#139304,#139305,
#139306,#139307,#139308,#139309,#139310,#139311,#139312,#139313,#139314,
#139315,#139316,#139317,#139318,#139319,#139320,#139321,#139322,#139323,
#139324,#139325,#139326,#139327,#139328,#139329,#139330,#139331,#139332,
#139333,#139334,#139335,#139336,#139337,#139338,#139339,#139340,#139341,
#139342,#139343,#139344,#139345,#139346,#139347,#139348,#139349,#139350,
#139351,#139352,#139353,#139354,#139355,#139356,#139357,#139358,#139359,
#139360,#139361,#139362,#139363,#139364,#139365,#139366,#139367,#139368,
#139369,#139370,#139371,#139372,#139373,#139374,#139375,#139376,#139377,
#139378,#139379,#139380,#139381,#139382,#139383,#139384,#139385,#139386,
#139387,#139388,#139389,#139390,#139391,#139392,#139393,#139394,#139395,
#139396,#139397,#139398,#139399,#139400,#139401,#139402,#139403,#139404,
#139405,#139406,#139407,#139408,#139409,#139410,#139411,#139412,#139413,
#139414,#139415,#139416,#139417,#139418,#139419,#139420),.UNSPECIFIED.,
 .F.,.F.)
B_SPLINE_CURVE_WITH_KNOTS((6,1,1,1,1,1,1,1,1,1,1,1,1,1,1,1,1,1,1,1,1,1,
1,1,1,1,1,1,1,1,1,1,1,1,1,1,1,1,1,1,1,1,1,1,1,1,1,1,1,1,1,1,1,1,1,1,1,1,
1,1,1,1,1,1,1,1,1,1,1,1,1,1,1,1,1,1,1,1,1,1,1,1,1,1,1,1,1,1,1,1,1,1,1,1,
1,1,1,1,1,1,1,1,1,1,1,1,1,1,1,1,1,1,1,1,1,1,1,1,1,1,1,1,1,1,1,1,1,1,1,1,
1,1,1,1,1,1,1,1,1,1,1,1,1,1,1,1,1,1,1,1,1,1,1,1,1,1,1,1,1,1,1,1,1,1,1,1,
1,1,1,1,1,1,1,1,1,1,1,1,1,1,1,1,1,1,1,1,1,1,1,6),(-0.941429844438167,-0.940000000000001,
-0.935000000000001,-0.930000000000001,-0.925000000000001,-0.920000000000001,
-0.915000000000001,-0.910000000000001,-0.905000000000001,-0.900000000000001,
-0.895000000000001,-0.890000000000001,-0.885000000000001,-0.880000000000001,
-0.875000000000001,-0.870000000000001,-0.865000000000001,-0.860000000000001,
-0.855000000000001,-0.850000000000001,-0.845000000000001,-0.840000000000001,
-0.835000000000001,-0.830000000000001,-0.825000000000001,-0.820000000000001,
-0.815000000000001,-0.810000000000001,-0.805000000000001,-0.800000000000001,
-0.795000000000001,-0.790000000000001,-0.785000000000001,-0.780000000000001,
-0.775000000000001,-0.770000000000001,-0.765000000000001,-0.760000000000001,
-0.755000000000001,-0.750000000000001,-0.745000000000001,-0.740000000000001,
-0.735000000000001,-0.730000000000001,-0.725000000000001,-0.720000000000001,
-0.715000000000001,-0.710000000000001,-0.705000000000001,-0.700000000000001,
-0.695000000000001,-0.690000000000001,-0.685,-0.68,-0.675,-0.67,-0.665,
-0.66,-0.655,-0.65,-0.645,-0.64,-0.635,-0.63,-0.625,-0.62,-0.615,-0.61,
-0.605,-0.6,-0.595,-0.59,-0.585,-0.58,-0.575,-0.57,-0.565,-0.56,-0.555,
-0.55,-0.545,-0.54,-0.535,-0.53,-0.525,-0.52,-0.515,-0.51,-0.505,-0.5,-0.495,
-0.49,-0.485,-0.48,-0.475,-0.47,-0.465,-0.46,-0.455,-0.45,-0.445,-0.44,
-0.435,-0.43,-0.425,-0.42,-0.415,-0.41,-0.405,-0.4,-0.395,-0.39,-0.385,
-0.38,-0.375,-0.37,-0.365,-0.36,-0.355,-0.35,-0.345,-0.34,-0.335,-0.33,
-0.325,-0.32,-0.315,-0.31,-0.305,-0.3,-0.295,-0.29,-0.285,-0.28,-0.275,
-0.27,-0.265,-0.26,-0.255,-0.25,-0.245,-0.24,-0.235,-0.23,-0.225,-0.22,
-0.215,-0.21,-0.205,-0.2,-0.195,-0.19,-0.185,-0.18,-0.175,-0.17,-0.165,
-0.16,-0.155,-0.15,-0.145,-0.14,-0.135,-0.13,-0.125,-0.12,-0.115,-0.11,
-0.105,-0.1,-0.095,-0.09,-0.085,-0.08,-0.075,-0.07,-0.065,-0.06,-0.055,
-0.05,-0.045,-0.04,-0.035,-0.03,-0.025,-0.02,-0.015,-0.01,-0.005,0.),
 .UNSPECIFIED.)
CURVE()
GEOMETRIC_REPRESENTATION_ITEM()
RATIONAL_B_SPLINE_CURVE((1.,1.,1.,1.,1.,1.,1.,1.,1.,1.,1.,1.,1.,1.,1.,1.,
1.,1.,1.,1.,1.,1.,1.,1.,1.,1.,1.,1.,1.,1.,1.,1.,1.,1.,1.,1.,1.,1.,1.,1.,
1.,1.,1.,1.,1.,1.,1.,1.,1.,1.,1.,1.,1.,1.,1.,1.,1.,1.,1.,1.,1.,1.,1.,1.,
1.,1.,1.,1.,1.,1.,1.,1.,1.,1.,1.,1.,1.,1.,1.,1.,1.,1.,1.,1.,1.,1.,1.,1.,
1.,1.,1.,1.,1.,1.,1.,1.,1.,1.,1.,1.,1.,1.,1.,1.,1.,1.,1.,1.,1.,1.,1.,1.,
1.,1.,1.,1.,1.,1.,1.,1.,1.,1.,1.,1.,1.,1.,1.,1.,1.,1.,1.,1.,1.,1.,1.,1.,
1.,1.,1.,1.,1.,1.,1.,1.,1.,1.,1.,1.,1.,1.,1.,1.,1.,1.,1.,1.,1.,1.,1.,1.,
1.,1.,1.,1.,1.,1.,1.,1.,1.,1.,1.,1.,1.,1.,1.,1.,1.,1.,1.,1.,1.,1.,1.,1.,
1.,1.,1.,1.,1.,1.,1.,1.,1.,1.))
REPRESENTATION_ITEM('')
);
#603=(
BOUNDED_CURVE()
B_SPLINE_CURVE(5,(#139832,#139833,#139834,#139835,#139836,#139837,#139838,
#139839,#139840,#139841,#139842,#139843,#139844,#139845,#139846,#139847,
#139848,#139849,#139850,#139851,#139852,#139853,#139854,#139855,#139856,
#139857,#139858,#139859,#139860,#139861,#139862,#139863,#139864,#139865,
#139866,#139867,#139868,#139869,#139870,#139871,#139872,#139873,#139874,
#139875,#139876,#139877,#139878,#139879,#139880,#139881,#139882,#139883,
#139884,#139885,#139886,#139887,#139888,#139889,#139890,#139891,#139892,
#139893,#139894,#139895,#139896,#139897,#139898,#139899,#139900,#139901,
#139902,#139903,#139904,#139905,#139906,#139907,#139908,#139909,#139910,
#139911,#139912,#139913,#139914,#139915,#139916,#139917,#139918,#139919,
#139920,#139921,#139922,#139923,#139924,#139925,#139926,#139927,#139928,
#139929,#139930,#139931,#139932,#139933,#139934,#139935,#139936,#139937,
#139938,#139939,#139940,#139941,#139942,#139943,#139944,#139945,#139946,
#139947,#139948,#139949,#139950,#139951,#139952,#139953,#139954,#139955,
#139956,#139957,#139958,#139959,#139960,#139961,#139962,#139963,#139964,
#139965,#139966,#139967,#139968,#139969,#139970,#139971,#139972,#139973,
#139974,#139975,#139976,#139977,#139978,#139979,#139980,#139981,#139982,
#139983,#139984,#139985,#139986,#139987,#139988,#139989,#139990,#139991,
#139992,#139993,#139994,#139995,#139996,#139997,#139998,#139999,#140000,
#140001,#140002,#140003,#140004,#140005,#140006,#140007,#140008,#140009,
#140010,#140011,#140012,#140013,#140014,#140015,#140016,#140017,#140018,
#140019,#140020,#140021,#140022,#140023,#140024,#140025),.UNSPECIFIED.,
 .F.,.F.)
B_SPLINE_CURVE_WITH_KNOTS((6,1,1,1,1,1,1,1,1,1,1,1,1,1,1,1,1,1,1,1,1,1,
1,1,1,1,1,1,1,1,1,1,1,1,1,1,1,1,1,1,1,1,1,1,1,1,1,1,1,1,1,1,1,1,1,1,1,1,
1,1,1,1,1,1,1,1,1,1,1,1,1,1,1,1,1,1,1,1,1,1,1,1,1,1,1,1,1,1,1,1,1,1,1,1,
1,1,1,1,1,1,1,1,1,1,1,1,1,1,1,1,1,1,1,1,1,1,1,1,1,1,1,1,1,1,1,1,1,1,1,1,
1,1,1,1,1,1,1,1,1,1,1,1,1,1,1,1,1,1,1,1,1,1,1,1,1,1,1,1,1,1,1,1,1,1,1,1,
1,1,1,1,1,1,1,1,1,1,1,1,1,1,1,1,1,1,1,1,1,1,1,6),(0.,0.005,0.01,0.015,0.02,
0.025,0.03,0.035,0.04,0.045,0.05,0.055,0.06,0.065,0.07,0.075,0.08,0.085,
0.09,0.095,0.1,0.105,0.11,0.115,0.12,0.125,0.13,0.135,0.14,0.145,0.15,0.155,
0.16,0.165,0.17,0.175,0.18,0.185,0.19,0.195,0.2,0.205,0.21,0.215,0.22,0.225,
0.23,0.235,0.24,0.245,0.25,0.255,0.26,0.265,0.27,0.275,0.28,0.285,0.29,
0.295,0.3,0.305,0.31,0.315,0.32,0.325,0.33,0.335,0.34,0.345,0.35,0.355,
0.36,0.365,0.37,0.375,0.38,0.385,0.39,0.395,0.4,0.405,0.41,0.415,0.42,0.425,
0.43,0.435,0.44,0.445,0.45,0.455,0.46,0.465,0.47,0.475,0.48,0.485,0.49,
0.495,0.5,0.505,0.51,0.515,0.52,0.525,0.53,0.535,0.54,0.545,0.55,0.555,
0.56,0.565,0.57,0.575,0.58,0.585,0.59,0.595,0.6,0.605,0.61,0.615,0.62,0.625,
0.63,0.635,0.64,0.645,0.65,0.655,0.66,0.665,0.67,0.675,0.68,0.685,0.690000000000001,
0.695000000000001,0.700000000000001,0.705000000000001,0.710000000000001,
0.715000000000001,0.720000000000001,0.725000000000001,0.730000000000001,
0.735000000000001,0.740000000000001,0.745000000000001,0.750000000000001,
0.755000000000001,0.760000000000001,0.765000000000001,0.770000000000001,
0.775000000000001,0.780000000000001,0.785000000000001,0.790000000000001,
0.795000000000001,0.800000000000001,0.805000000000001,0.810000000000001,
0.815000000000001,0.820000000000001,0.825000000000001,0.830000000000001,
0.835000000000001,0.840000000000001,0.845000000000001,0.850000000000001,
0.855000000000001,0.860000000000001,0.865000000000001,0.870000000000001,
0.875000000000001,0.880000000000001,0.885000000000001,0.890000000000001,
0.895000000000001,0.900000000000001,0.905000000000001,0.910000000000001,
0.915000000000001,0.920000000000001,0.925000000000001,0.930000000000001,
0.935000000000001,0.940000000000001,0.941429844438156),.UNSPECIFIED.)
CURVE()
GEOMETRIC_REPRESENTATION_ITEM()
RATIONAL_B_SPLINE_CURVE((1.,1.,1.,1.,1.,1.,1.,1.,1.,1.,1.,1.,1.,1.,1.,1.,
1.,1.,1.,1.,1.,1.,1.,1.,1.,1.,1.,1.,1.,1.,1.,1.,1.,1.,1.,1.,1.,1.,1.,1.,
1.,1.,1.,1.,1.,1.,1.,1.,1.,1.,1.,1.,1.,1.,1.,1.,1.,1.,1.,1.,1.,1.,1.,1.,
1.,1.,1.,1.,1.,1.,1.,1.,1.,1.,1.,1.,1.,1.,1.,1.,1.,1.,1.,1.,1.,1.,1.,1.,
1.,1.,1.,1.,1.,1.,1.,1.,1.,1.,1.,1.,1.,1.,1.,1.,1.,1.,1.,1.,1.,1.,1.,1.,
1.,1.,1.,1.,1.,1.,1.,1.,1.,1.,1.,1.,1.,1.,1.,1.,1.,1.,1.,1.,1.,1.,1.,1.,
1.,1.,1.,1.,1.,1.,1.,1.,1.,1.,1.,1.,1.,1.,1.,1.,1.,1.,1.,1.,1.,1.,1.,1.,
1.,1.,1.,1.,1.,1.,1.,1.,1.,1.,1.,1.,1.,1.,1.,1.,1.,1.,1.,1.,1.,1.,1.,1.,
1.,1.,1.,1.,1.,1.,1.,1.,1.,1.))
REPRESENTATION_ITEM('')
);
#604=(
BOUNDED_CURVE()
B_SPLINE_CURVE(5,(#140028,#140029,#140030,#140031,#140032,#140033,#140034,
#140035,#140036,#140037,#140038,#140039,#140040,#140041,#140042,#140043,
#140044,#140045,#140046,#140047,#140048,#140049,#140050,#140051,#140052,
#140053,#140054,#140055,#140056,#140057,#140058,#140059,#140060,#140061,
#140062,#140063,#140064,#140065,#140066,#140067,#140068,#140069,#140070,
#140071,#140072,#140073,#140074,#140075,#140076,#140077,#140078,#140079,
#140080,#140081,#140082,#140083,#140084,#140085,#140086,#140087,#140088,
#140089,#140090,#140091,#140092,#140093,#140094,#140095,#140096,#140097,
#140098,#140099,#140100,#140101,#140102,#140103,#140104,#140105,#140106,
#140107,#140108,#140109,#140110,#140111,#140112,#140113,#140114,#140115,
#140116,#140117,#140118,#140119,#140120,#140121,#140122,#140123,#140124,
#140125,#140126,#140127,#140128,#140129,#140130,#140131,#140132,#140133,
#140134,#140135,#140136,#140137,#140138,#140139,#140140,#140141,#140142,
#140143,#140144,#140145,#140146,#140147,#140148,#140149,#140150,#140151,
#140152,#140153,#140154,#140155,#140156,#140157,#140158,#140159,#140160,
#140161,#140162,#140163,#140164,#140165,#140166,#140167,#140168,#140169,
#140170,#140171,#140172,#140173,#140174,#140175,#140176,#140177,#140178,
#140179,#140180,#140181,#140182,#140183,#140184,#140185,#140186,#140187,
#140188,#140189,#140190,#140191,#140192,#140193,#140194,#140195,#140196,
#140197,#140198,#140199,#140200,#140201,#140202,#140203,#140204,#140205,
#140206,#140207,#140208,#140209,#140210,#140211,#140212,#140213,#140214,
#140215,#140216,#140217,#140218,#140219,#140220,#140221),.UNSPECIFIED.,
 .F.,.F.)
B_SPLINE_CURVE_WITH_KNOTS((6,1,1,1,1,1,1,1,1,1,1,1,1,1,1,1,1,1,1,1,1,1,
1,1,1,1,1,1,1,1,1,1,1,1,1,1,1,1,1,1,1,1,1,1,1,1,1,1,1,1,1,1,1,1,1,1,1,1,
1,1,1,1,1,1,1,1,1,1,1,1,1,1,1,1,1,1,1,1,1,1,1,1,1,1,1,1,1,1,1,1,1,1,1,1,
1,1,1,1,1,1,1,1,1,1,1,1,1,1,1,1,1,1,1,1,1,1,1,1,1,1,1,1,1,1,1,1,1,1,1,1,
1,1,1,1,1,1,1,1,1,1,1,1,1,1,1,1,1,1,1,1,1,1,1,1,1,1,1,1,1,1,1,1,1,1,1,1,
1,1,1,1,1,1,1,1,1,1,1,1,1,1,1,1,1,1,1,1,1,1,1,6),(-0.941429844438138,-0.940000000000001,
-0.935000000000001,-0.930000000000001,-0.925000000000001,-0.920000000000001,
-0.915000000000001,-0.910000000000001,-0.905000000000001,-0.900000000000001,
-0.895000000000001,-0.890000000000001,-0.885000000000001,-0.880000000000001,
-0.875000000000001,-0.870000000000001,-0.865000000000001,-0.860000000000001,
-0.855000000000001,-0.850000000000001,-0.845000000000001,-0.840000000000001,
-0.835000000000001,-0.830000000000001,-0.825000000000001,-0.820000000000001,
-0.815000000000001,-0.810000000000001,-0.805000000000001,-0.800000000000001,
-0.795000000000001,-0.790000000000001,-0.785000000000001,-0.780000000000001,
-0.775000000000001,-0.770000000000001,-0.765000000000001,-0.760000000000001,
-0.755000000000001,-0.750000000000001,-0.745000000000001,-0.740000000000001,
-0.735000000000001,-0.730000000000001,-0.725000000000001,-0.720000000000001,
-0.715000000000001,-0.710000000000001,-0.705000000000001,-0.700000000000001,
-0.695000000000001,-0.690000000000001,-0.685,-0.68,-0.675,-0.67,-0.665,
-0.66,-0.655,-0.65,-0.645,-0.64,-0.635,-0.63,-0.625,-0.62,-0.615,-0.61,
-0.605,-0.6,-0.595,-0.59,-0.585,-0.58,-0.575,-0.57,-0.565,-0.56,-0.555,
-0.55,-0.545,-0.54,-0.535,-0.53,-0.525,-0.52,-0.515,-0.51,-0.505,-0.5,-0.495,
-0.49,-0.485,-0.48,-0.475,-0.47,-0.465,-0.46,-0.455,-0.45,-0.445,-0.44,
-0.435,-0.43,-0.425,-0.42,-0.415,-0.41,-0.405,-0.4,-0.395,-0.39,-0.385,
-0.38,-0.375,-0.37,-0.365,-0.36,-0.355,-0.35,-0.345,-0.34,-0.335,-0.33,
-0.325,-0.32,-0.315,-0.31,-0.305,-0.3,-0.295,-0.29,-0.285,-0.28,-0.275,
-0.27,-0.265,-0.26,-0.255,-0.25,-0.245,-0.24,-0.235,-0.23,-0.225,-0.22,
-0.215,-0.21,-0.205,-0.2,-0.195,-0.19,-0.185,-0.18,-0.175,-0.17,-0.165,
-0.16,-0.155,-0.15,-0.145,-0.14,-0.135,-0.13,-0.125,-0.12,-0.115,-0.11,
-0.105,-0.1,-0.095,-0.09,-0.085,-0.08,-0.075,-0.07,-0.065,-0.06,-0.055,
-0.05,-0.045,-0.04,-0.035,-0.03,-0.025,-0.02,-0.015,-0.01,-0.005,0.),
 .UNSPECIFIED.)
CURVE()
GEOMETRIC_REPRESENTATION_ITEM()
RATIONAL_B_SPLINE_CURVE((1.,1.,1.,1.,1.,1.,1.,1.,1.,1.,1.,1.,1.,1.,1.,1.,
1.,1.,1.,1.,1.,1.,1.,1.,1.,1.,1.,1.,1.,1.,1.,1.,1.,1.,1.,1.,1.,1.,1.,1.,
1.,1.,1.,1.,1.,1.,1.,1.,1.,1.,1.,1.,1.,1.,1.,1.,1.,1.,1.,1.,1.,1.,1.,1.,
1.,1.,1.,1.,1.,1.,1.,1.,1.,1.,1.,1.,1.,1.,1.,1.,1.,1.,1.,1.,1.,1.,1.,1.,
1.,1.,1.,1.,1.,1.,1.,1.,1.,1.,1.,1.,1.,1.,1.,1.,1.,1.,1.,1.,1.,1.,1.,1.,
1.,1.,1.,1.,1.,1.,1.,1.,1.,1.,1.,1.,1.,1.,1.,1.,1.,1.,1.,1.,1.,1.,1.,1.,
1.,1.,1.,1.,1.,1.,1.,1.,1.,1.,1.,1.,1.,1.,1.,1.,1.,1.,1.,1.,1.,1.,1.,1.,
1.,1.,1.,1.,1.,1.,1.,1.,1.,1.,1.,1.,1.,1.,1.,1.,1.,1.,1.,1.,1.,1.,1.,1.,
1.,1.,1.,1.,1.,1.,1.,1.,1.,1.))
REPRESENTATION_ITEM('')
);
#605=(
BOUNDED_CURVE()
B_SPLINE_CURVE(5,(#140633,#140634,#140635,#140636,#140637,#140638,#140639,
#140640,#140641,#140642,#140643,#140644,#140645,#140646,#140647,#140648,
#140649,#140650,#140651,#140652,#140653,#140654,#140655,#140656,#140657,
#140658,#140659,#140660,#140661,#140662,#140663,#140664,#140665,#140666,
#140667,#140668,#140669,#140670,#140671,#140672,#140673,#140674,#140675,
#140676,#140677,#140678,#140679,#140680,#140681,#140682,#140683,#140684,
#140685,#140686,#140687,#140688,#140689,#140690,#140691,#140692,#140693,
#140694,#140695,#140696,#140697,#140698,#140699,#140700,#140701,#140702,
#140703,#140704,#140705,#140706,#140707,#140708,#140709,#140710,#140711,
#140712,#140713,#140714,#140715,#140716,#140717,#140718,#140719,#140720,
#140721,#140722,#140723,#140724,#140725,#140726,#140727,#140728,#140729,
#140730,#140731,#140732,#140733,#140734,#140735,#140736,#140737,#140738,
#140739,#140740,#140741,#140742,#140743,#140744,#140745,#140746,#140747,
#140748,#140749,#140750,#140751,#140752,#140753,#140754,#140755,#140756,
#140757,#140758,#140759,#140760,#140761,#140762,#140763,#140764,#140765,
#140766,#140767,#140768,#140769,#140770,#140771,#140772,#140773,#140774,
#140775,#140776,#140777,#140778,#140779,#140780,#140781,#140782,#140783,
#140784,#140785,#140786,#140787,#140788,#140789,#140790,#140791,#140792,
#140793,#140794,#140795,#140796,#140797,#140798,#140799,#140800,#140801,
#140802,#140803,#140804,#140805,#140806,#140807,#140808,#140809,#140810,
#140811,#140812,#140813,#140814,#140815,#140816,#140817,#140818,#140819,
#140820,#140821,#140822,#140823,#140824,#140825,#140826),.UNSPECIFIED.,
 .F.,.F.)
B_SPLINE_CURVE_WITH_KNOTS((6,1,1,1,1,1,1,1,1,1,1,1,1,1,1,1,1,1,1,1,1,1,
1,1,1,1,1,1,1,1,1,1,1,1,1,1,1,1,1,1,1,1,1,1,1,1,1,1,1,1,1,1,1,1,1,1,1,1,
1,1,1,1,1,1,1,1,1,1,1,1,1,1,1,1,1,1,1,1,1,1,1,1,1,1,1,1,1,1,1,1,1,1,1,1,
1,1,1,1,1,1,1,1,1,1,1,1,1,1,1,1,1,1,1,1,1,1,1,1,1,1,1,1,1,1,1,1,1,1,1,1,
1,1,1,1,1,1,1,1,1,1,1,1,1,1,1,1,1,1,1,1,1,1,1,1,1,1,1,1,1,1,1,1,1,1,1,1,
1,1,1,1,1,1,1,1,1,1,1,1,1,1,1,1,1,1,1,1,1,1,1,6),(0.,0.005,0.01,0.015,0.02,
0.025,0.03,0.035,0.04,0.045,0.05,0.055,0.06,0.065,0.07,0.075,0.08,0.085,
0.09,0.095,0.1,0.105,0.11,0.115,0.12,0.125,0.13,0.135,0.14,0.145,0.15,0.155,
0.16,0.165,0.17,0.175,0.18,0.185,0.19,0.195,0.2,0.205,0.21,0.215,0.22,0.225,
0.23,0.235,0.24,0.245,0.25,0.255,0.26,0.265,0.27,0.275,0.28,0.285,0.29,
0.295,0.3,0.305,0.31,0.315,0.32,0.325,0.33,0.335,0.34,0.345,0.35,0.355,
0.36,0.365,0.37,0.375,0.38,0.385,0.39,0.395,0.4,0.405,0.41,0.415,0.42,0.425,
0.43,0.435,0.44,0.445,0.45,0.455,0.46,0.465,0.47,0.475,0.48,0.485,0.49,
0.495,0.5,0.505,0.51,0.515,0.52,0.525,0.53,0.535,0.54,0.545,0.55,0.555,
0.56,0.565,0.57,0.575,0.58,0.585,0.59,0.595,0.6,0.605,0.61,0.615,0.62,0.625,
0.63,0.635,0.64,0.645,0.65,0.655,0.66,0.665,0.67,0.675,0.68,0.685,0.690000000000001,
0.695000000000001,0.700000000000001,0.705000000000001,0.710000000000001,
0.715000000000001,0.720000000000001,0.725000000000001,0.730000000000001,
0.735000000000001,0.740000000000001,0.745000000000001,0.750000000000001,
0.755000000000001,0.760000000000001,0.765000000000001,0.770000000000001,
0.775000000000001,0.780000000000001,0.785000000000001,0.790000000000001,
0.795000000000001,0.800000000000001,0.805000000000001,0.810000000000001,
0.815000000000001,0.820000000000001,0.825000000000001,0.830000000000001,
0.835000000000001,0.840000000000001,0.845000000000001,0.850000000000001,
0.855000000000001,0.860000000000001,0.865000000000001,0.870000000000001,
0.875000000000001,0.880000000000001,0.885000000000001,0.890000000000001,
0.895000000000001,0.900000000000001,0.905000000000001,0.910000000000001,
0.915000000000001,0.920000000000001,0.925000000000001,0.930000000000001,
0.935000000000001,0.940000000000001,0.941429844438041),.UNSPECIFIED.)
CURVE()
GEOMETRIC_REPRESENTATION_ITEM()
RATIONAL_B_SPLINE_CURVE((1.,1.,1.,1.,1.,1.,1.,1.,1.,1.,1.,1.,1.,1.,1.,1.,
1.,1.,1.,1.,1.,1.,1.,1.,1.,1.,1.,1.,1.,1.,1.,1.,1.,1.,1.,1.,1.,1.,1.,1.,
1.,1.,1.,1.,1.,1.,1.,1.,1.,1.,1.,1.,1.,1.,1.,1.,1.,1.,1.,1.,1.,1.,1.,1.,
1.,1.,1.,1.,1.,1.,1.,1.,1.,1.,1.,1.,1.,1.,1.,1.,1.,1.,1.,1.,1.,1.,1.,1.,
1.,1.,1.,1.,1.,1.,1.,1.,1.,1.,1.,1.,1.,1.,1.,1.,1.,1.,1.,1.,1.,1.,1.,1.,
1.,1.,1.,1.,1.,1.,1.,1.,1.,1.,1.,1.,1.,1.,1.,1.,1.,1.,1.,1.,1.,1.,1.,1.,
1.,1.,1.,1.,1.,1.,1.,1.,1.,1.,1.,1.,1.,1.,1.,1.,1.,1.,1.,1.,1.,1.,1.,1.,
1.,1.,1.,1.,1.,1.,1.,1.,1.,1.,1.,1.,1.,1.,1.,1.,1.,1.,1.,1.,1.,1.,1.,1.,
1.,1.,1.,1.,1.,1.,1.,1.,1.,1.))
REPRESENTATION_ITEM('')
);
#606=(
BOUNDED_CURVE()
B_SPLINE_CURVE(5,(#140829,#140830,#140831,#140832,#140833,#140834,#140835,
#140836,#140837,#140838,#140839,#140840,#140841,#140842,#140843,#140844,
#140845,#140846,#140847,#140848,#140849,#140850,#140851,#140852,#140853,
#140854,#140855,#140856,#140857,#140858,#140859,#140860,#140861,#140862,
#140863,#140864,#140865,#140866,#140867,#140868,#140869,#140870,#140871,
#140872,#140873,#140874,#140875,#140876,#140877,#140878,#140879,#140880,
#140881,#140882,#140883,#140884,#140885,#140886,#140887,#140888,#140889,
#140890,#140891,#140892,#140893,#140894,#140895,#140896,#140897,#140898,
#140899,#140900,#140901,#140902,#140903,#140904,#140905,#140906,#140907,
#140908,#140909,#140910,#140911,#140912,#140913,#140914,#140915,#140916,
#140917,#140918,#140919,#140920,#140921,#140922,#140923,#140924,#140925,
#140926,#140927,#140928,#140929,#140930,#140931,#140932,#140933,#140934,
#140935,#140936,#140937,#140938,#140939,#140940,#140941,#140942,#140943,
#140944,#140945,#140946,#140947,#140948,#140949,#140950,#140951,#140952,
#140953,#140954,#140955,#140956,#140957,#140958,#140959,#140960,#140961,
#140962,#140963,#140964,#140965,#140966,#140967,#140968,#140969,#140970,
#140971,#140972,#140973,#140974,#140975,#140976,#140977,#140978,#140979,
#140980,#140981,#140982,#140983,#140984,#140985,#140986,#140987,#140988,
#140989,#140990,#140991,#140992,#140993,#140994,#140995,#140996,#140997,
#140998,#140999,#141000,#141001,#141002,#141003,#141004,#141005,#141006,
#141007,#141008,#141009,#141010,#141011,#141012,#141013,#141014,#141015,
#141016,#141017,#141018,#141019,#141020,#141021,#141022),.UNSPECIFIED.,
 .F.,.F.)
B_SPLINE_CURVE_WITH_KNOTS((6,1,1,1,1,1,1,1,1,1,1,1,1,1,1,1,1,1,1,1,1,1,
1,1,1,1,1,1,1,1,1,1,1,1,1,1,1,1,1,1,1,1,1,1,1,1,1,1,1,1,1,1,1,1,1,1,1,1,
1,1,1,1,1,1,1,1,1,1,1,1,1,1,1,1,1,1,1,1,1,1,1,1,1,1,1,1,1,1,1,1,1,1,1,1,
1,1,1,1,1,1,1,1,1,1,1,1,1,1,1,1,1,1,1,1,1,1,1,1,1,1,1,1,1,1,1,1,1,1,1,1,
1,1,1,1,1,1,1,1,1,1,1,1,1,1,1,1,1,1,1,1,1,1,1,1,1,1,1,1,1,1,1,1,1,1,1,1,
1,1,1,1,1,1,1,1,1,1,1,1,1,1,1,1,1,1,1,1,1,1,1,6),(-0.941429844438037,-0.940000000000001,
-0.935000000000001,-0.930000000000001,-0.925000000000001,-0.920000000000001,
-0.915000000000001,-0.910000000000001,-0.905000000000001,-0.900000000000001,
-0.895000000000001,-0.890000000000001,-0.885000000000001,-0.880000000000001,
-0.875000000000001,-0.870000000000001,-0.865000000000001,-0.860000000000001,
-0.855000000000001,-0.850000000000001,-0.845000000000001,-0.840000000000001,
-0.835000000000001,-0.830000000000001,-0.825000000000001,-0.820000000000001,
-0.815000000000001,-0.810000000000001,-0.805000000000001,-0.800000000000001,
-0.795000000000001,-0.790000000000001,-0.785000000000001,-0.780000000000001,
-0.775000000000001,-0.770000000000001,-0.765000000000001,-0.760000000000001,
-0.755000000000001,-0.750000000000001,-0.745000000000001,-0.740000000000001,
-0.735000000000001,-0.730000000000001,-0.725000000000001,-0.720000000000001,
-0.715000000000001,-0.710000000000001,-0.705000000000001,-0.700000000000001,
-0.695000000000001,-0.690000000000001,-0.685,-0.68,-0.675,-0.67,-0.665,
-0.66,-0.655,-0.65,-0.645,-0.64,-0.635,-0.63,-0.625,-0.62,-0.615,-0.61,
-0.605,-0.6,-0.595,-0.59,-0.585,-0.58,-0.575,-0.57,-0.565,-0.56,-0.555,
-0.55,-0.545,-0.54,-0.535,-0.53,-0.525,-0.52,-0.515,-0.51,-0.505,-0.5,-0.495,
-0.49,-0.485,-0.48,-0.475,-0.47,-0.465,-0.46,-0.455,-0.45,-0.445,-0.44,
-0.435,-0.43,-0.425,-0.42,-0.415,-0.41,-0.405,-0.4,-0.395,-0.39,-0.385,
-0.38,-0.375,-0.37,-0.365,-0.36,-0.355,-0.35,-0.345,-0.34,-0.335,-0.33,
-0.325,-0.32,-0.315,-0.31,-0.305,-0.3,-0.295,-0.29,-0.285,-0.28,-0.275,
-0.27,-0.265,-0.26,-0.255,-0.25,-0.245,-0.24,-0.235,-0.23,-0.225,-0.22,
-0.215,-0.21,-0.205,-0.2,-0.195,-0.19,-0.185,-0.18,-0.175,-0.17,-0.165,
-0.16,-0.155,-0.15,-0.145,-0.14,-0.135,-0.13,-0.125,-0.12,-0.115,-0.11,
-0.105,-0.1,-0.095,-0.09,-0.085,-0.08,-0.075,-0.07,-0.065,-0.06,-0.055,
-0.05,-0.045,-0.04,-0.035,-0.03,-0.025,-0.02,-0.015,-0.01,-0.005,0.),
 .UNSPECIFIED.)
CURVE()
GEOMETRIC_REPRESENTATION_ITEM()
RATIONAL_B_SPLINE_CURVE((1.,1.,1.,1.,1.,1.,1.,1.,1.,1.,1.,1.,1.,1.,1.,1.,
1.,1.,1.,1.,1.,1.,1.,1.,1.,1.,1.,1.,1.,1.,1.,1.,1.,1.,1.,1.,1.,1.,1.,1.,
1.,1.,1.,1.,1.,1.,1.,1.,1.,1.,1.,1.,1.,1.,1.,1.,1.,1.,1.,1.,1.,1.,1.,1.,
1.,1.,1.,1.,1.,1.,1.,1.,1.,1.,1.,1.,1.,1.,1.,1.,1.,1.,1.,1.,1.,1.,1.,1.,
1.,1.,1.,1.,1.,1.,1.,1.,1.,1.,1.,1.,1.,1.,1.,1.,1.,1.,1.,1.,1.,1.,1.,1.,
1.,1.,1.,1.,1.,1.,1.,1.,1.,1.,1.,1.,1.,1.,1.,1.,1.,1.,1.,1.,1.,1.,1.,1.,
1.,1.,1.,1.,1.,1.,1.,1.,1.,1.,1.,1.,1.,1.,1.,1.,1.,1.,1.,1.,1.,1.,1.,1.,
1.,1.,1.,1.,1.,1.,1.,1.,1.,1.,1.,1.,1.,1.,1.,1.,1.,1.,1.,1.,1.,1.,1.,1.,
1.,1.,1.,1.,1.,1.,1.,1.,1.,1.))
REPRESENTATION_ITEM('')
);
#607=(
BOUNDED_CURVE()
B_SPLINE_CURVE(5,(#141434,#141435,#141436,#141437,#141438,#141439,#141440,
#141441,#141442,#141443,#141444,#141445,#141446,#141447,#141448,#141449,
#141450,#141451,#141452,#141453,#141454,#141455,#141456,#141457,#141458,
#141459,#141460,#141461,#141462,#141463,#141464,#141465,#141466,#141467,
#141468,#141469,#141470,#141471,#141472,#141473,#141474,#141475,#141476,
#141477,#141478,#141479,#141480,#141481,#141482,#141483,#141484,#141485,
#141486,#141487,#141488,#141489,#141490,#141491,#141492,#141493,#141494,
#141495,#141496,#141497,#141498,#141499,#141500,#141501,#141502,#141503,
#141504,#141505,#141506,#141507,#141508,#141509,#141510,#141511,#141512,
#141513,#141514,#141515,#141516,#141517,#141518,#141519,#141520,#141521,
#141522,#141523,#141524,#141525,#141526,#141527,#141528,#141529,#141530,
#141531,#141532,#141533,#141534,#141535,#141536,#141537,#141538,#141539,
#141540,#141541,#141542,#141543,#141544,#141545,#141546,#141547,#141548,
#141549,#141550,#141551,#141552,#141553,#141554,#141555,#141556,#141557,
#141558,#141559,#141560,#141561,#141562,#141563,#141564,#141565,#141566,
#141567,#141568,#141569,#141570,#141571,#141572,#141573,#141574,#141575,
#141576,#141577,#141578,#141579,#141580,#141581,#141582,#141583,#141584,
#141585,#141586,#141587,#141588,#141589,#141590,#141591,#141592,#141593,
#141594,#141595,#141596,#141597,#141598,#141599,#141600,#141601,#141602,
#141603,#141604,#141605,#141606,#141607,#141608,#141609,#141610,#141611,
#141612,#141613,#141614,#141615,#141616,#141617,#141618,#141619,#141620,
#141621,#141622,#141623,#141624,#141625,#141626,#141627),.UNSPECIFIED.,
 .F.,.F.)
B_SPLINE_CURVE_WITH_KNOTS((6,1,1,1,1,1,1,1,1,1,1,1,1,1,1,1,1,1,1,1,1,1,
1,1,1,1,1,1,1,1,1,1,1,1,1,1,1,1,1,1,1,1,1,1,1,1,1,1,1,1,1,1,1,1,1,1,1,1,
1,1,1,1,1,1,1,1,1,1,1,1,1,1,1,1,1,1,1,1,1,1,1,1,1,1,1,1,1,1,1,1,1,1,1,1,
1,1,1,1,1,1,1,1,1,1,1,1,1,1,1,1,1,1,1,1,1,1,1,1,1,1,1,1,1,1,1,1,1,1,1,1,
1,1,1,1,1,1,1,1,1,1,1,1,1,1,1,1,1,1,1,1,1,1,1,1,1,1,1,1,1,1,1,1,1,1,1,1,
1,1,1,1,1,1,1,1,1,1,1,1,1,1,1,1,1,1,1,1,1,1,1,6),(0.,0.005,0.01,0.015,0.02,
0.025,0.03,0.035,0.04,0.045,0.05,0.055,0.06,0.065,0.07,0.075,0.08,0.085,
0.09,0.095,0.1,0.105,0.11,0.115,0.12,0.125,0.13,0.135,0.14,0.145,0.15,0.155,
0.16,0.165,0.17,0.175,0.18,0.185,0.19,0.195,0.2,0.205,0.21,0.215,0.22,0.225,
0.23,0.235,0.24,0.245,0.25,0.255,0.26,0.265,0.27,0.275,0.28,0.285,0.29,
0.295,0.3,0.305,0.31,0.315,0.32,0.325,0.33,0.335,0.34,0.345,0.35,0.355,
0.36,0.365,0.37,0.375,0.38,0.385,0.39,0.395,0.4,0.405,0.41,0.415,0.42,0.425,
0.43,0.435,0.44,0.445,0.45,0.455,0.46,0.465,0.47,0.475,0.48,0.485,0.49,
0.495,0.5,0.505,0.51,0.515,0.52,0.525,0.53,0.535,0.54,0.545,0.55,0.555,
0.56,0.565,0.57,0.575,0.58,0.585,0.59,0.595,0.6,0.605,0.61,0.615,0.62,0.625,
0.63,0.635,0.64,0.645,0.65,0.655,0.66,0.665,0.67,0.675,0.68,0.685,0.690000000000001,
0.695000000000001,0.700000000000001,0.705000000000001,0.710000000000001,
0.715000000000001,0.720000000000001,0.725000000000001,0.730000000000001,
0.735000000000001,0.740000000000001,0.745000000000001,0.750000000000001,
0.755000000000001,0.760000000000001,0.765000000000001,0.770000000000001,
0.775000000000001,0.780000000000001,0.785000000000001,0.790000000000001,
0.795000000000001,0.800000000000001,0.805000000000001,0.810000000000001,
0.815000000000001,0.820000000000001,0.825000000000001,0.830000000000001,
0.835000000000001,0.840000000000001,0.845000000000001,0.850000000000001,
0.855000000000001,0.860000000000001,0.865000000000001,0.870000000000001,
0.875000000000001,0.880000000000001,0.885000000000001,0.890000000000001,
0.895000000000001,0.900000000000001,0.905000000000001,0.910000000000001,
0.915000000000001,0.920000000000001,0.925000000000001,0.930000000000001,
0.935000000000001,0.940000000000001,0.941429844438043),.UNSPECIFIED.)
CURVE()
GEOMETRIC_REPRESENTATION_ITEM()
RATIONAL_B_SPLINE_CURVE((1.,1.,1.,1.,1.,1.,1.,1.,1.,1.,1.,1.,1.,1.,1.,1.,
1.,1.,1.,1.,1.,1.,1.,1.,1.,1.,1.,1.,1.,1.,1.,1.,1.,1.,1.,1.,1.,1.,1.,1.,
1.,1.,1.,1.,1.,1.,1.,1.,1.,1.,1.,1.,1.,1.,1.,1.,1.,1.,1.,1.,1.,1.,1.,1.,
1.,1.,1.,1.,1.,1.,1.,1.,1.,1.,1.,1.,1.,1.,1.,1.,1.,1.,1.,1.,1.,1.,1.,1.,
1.,1.,1.,1.,1.,1.,1.,1.,1.,1.,1.,1.,1.,1.,1.,1.,1.,1.,1.,1.,1.,1.,1.,1.,
1.,1.,1.,1.,1.,1.,1.,1.,1.,1.,1.,1.,1.,1.,1.,1.,1.,1.,1.,1.,1.,1.,1.,1.,
1.,1.,1.,1.,1.,1.,1.,1.,1.,1.,1.,1.,1.,1.,1.,1.,1.,1.,1.,1.,1.,1.,1.,1.,
1.,1.,1.,1.,1.,1.,1.,1.,1.,1.,1.,1.,1.,1.,1.,1.,1.,1.,1.,1.,1.,1.,1.,1.,
1.,1.,1.,1.,1.,1.,1.,1.,1.,1.))
REPRESENTATION_ITEM('')
);
#608=(
BOUNDED_CURVE()
B_SPLINE_CURVE(5,(#141630,#141631,#141632,#141633,#141634,#141635,#141636,
#141637,#141638,#141639,#141640,#141641,#141642,#141643,#141644,#141645,
#141646,#141647,#141648,#141649,#141650,#141651,#141652,#141653,#141654,
#141655,#141656,#141657,#141658,#141659,#141660,#141661,#141662,#141663,
#141664,#141665,#141666,#141667,#141668,#141669,#141670,#141671,#141672,
#141673,#141674,#141675,#141676,#141677,#141678,#141679,#141680,#141681,
#141682,#141683,#141684,#141685,#141686,#141687,#141688,#141689,#141690,
#141691,#141692,#141693,#141694,#141695,#141696,#141697,#141698,#141699,
#141700,#141701,#141702,#141703,#141704,#141705,#141706,#141707,#141708,
#141709,#141710,#141711,#141712,#141713,#141714,#141715,#141716,#141717,
#141718,#141719,#141720,#141721,#141722,#141723,#141724,#141725,#141726,
#141727,#141728,#141729,#141730,#141731,#141732,#141733,#141734,#141735,
#141736,#141737,#141738,#141739,#141740,#141741,#141742,#141743,#141744,
#141745,#141746,#141747,#141748,#141749,#141750,#141751,#141752,#141753,
#141754,#141755,#141756,#141757,#141758,#141759,#141760,#141761,#141762,
#141763,#141764,#141765,#141766,#141767,#141768,#141769,#141770,#141771,
#141772,#141773,#141774,#141775,#141776,#141777,#141778,#141779,#141780,
#141781,#141782,#141783,#141784,#141785,#141786,#141787,#141788,#141789,
#141790,#141791,#141792,#141793,#141794,#141795,#141796,#141797,#141798,
#141799,#141800,#141801,#141802,#141803,#141804,#141805,#141806,#141807,
#141808,#141809,#141810,#141811,#141812,#141813,#141814,#141815,#141816,
#141817,#141818,#141819,#141820,#141821,#141822,#141823),.UNSPECIFIED.,
 .F.,.F.)
B_SPLINE_CURVE_WITH_KNOTS((6,1,1,1,1,1,1,1,1,1,1,1,1,1,1,1,1,1,1,1,1,1,
1,1,1,1,1,1,1,1,1,1,1,1,1,1,1,1,1,1,1,1,1,1,1,1,1,1,1,1,1,1,1,1,1,1,1,1,
1,1,1,1,1,1,1,1,1,1,1,1,1,1,1,1,1,1,1,1,1,1,1,1,1,1,1,1,1,1,1,1,1,1,1,1,
1,1,1,1,1,1,1,1,1,1,1,1,1,1,1,1,1,1,1,1,1,1,1,1,1,1,1,1,1,1,1,1,1,1,1,1,
1,1,1,1,1,1,1,1,1,1,1,1,1,1,1,1,1,1,1,1,1,1,1,1,1,1,1,1,1,1,1,1,1,1,1,1,
1,1,1,1,1,1,1,1,1,1,1,1,1,1,1,1,1,1,1,1,1,1,1,6),(-0.941429844438047,-0.940000000000001,
-0.935000000000001,-0.930000000000001,-0.925000000000001,-0.920000000000001,
-0.915000000000001,-0.910000000000001,-0.905000000000001,-0.900000000000001,
-0.895000000000001,-0.890000000000001,-0.885000000000001,-0.880000000000001,
-0.875000000000001,-0.870000000000001,-0.865000000000001,-0.860000000000001,
-0.855000000000001,-0.850000000000001,-0.845000000000001,-0.840000000000001,
-0.835000000000001,-0.830000000000001,-0.825000000000001,-0.820000000000001,
-0.815000000000001,-0.810000000000001,-0.805000000000001,-0.800000000000001,
-0.795000000000001,-0.790000000000001,-0.785000000000001,-0.780000000000001,
-0.775000000000001,-0.770000000000001,-0.765000000000001,-0.760000000000001,
-0.755000000000001,-0.750000000000001,-0.745000000000001,-0.740000000000001,
-0.735000000000001,-0.730000000000001,-0.725000000000001,-0.720000000000001,
-0.715000000000001,-0.710000000000001,-0.705000000000001,-0.700000000000001,
-0.695000000000001,-0.690000000000001,-0.685,-0.68,-0.675,-0.67,-0.665,
-0.66,-0.655,-0.65,-0.645,-0.64,-0.635,-0.63,-0.625,-0.62,-0.615,-0.61,
-0.605,-0.6,-0.595,-0.59,-0.585,-0.58,-0.575,-0.57,-0.565,-0.56,-0.555,
-0.55,-0.545,-0.54,-0.535,-0.53,-0.525,-0.52,-0.515,-0.51,-0.505,-0.5,-0.495,
-0.49,-0.485,-0.48,-0.475,-0.47,-0.465,-0.46,-0.455,-0.45,-0.445,-0.44,
-0.435,-0.43,-0.425,-0.42,-0.415,-0.41,-0.405,-0.4,-0.395,-0.39,-0.385,
-0.38,-0.375,-0.37,-0.365,-0.36,-0.355,-0.35,-0.345,-0.34,-0.335,-0.33,
-0.325,-0.32,-0.315,-0.31,-0.305,-0.3,-0.295,-0.29,-0.285,-0.28,-0.275,
-0.27,-0.265,-0.26,-0.255,-0.25,-0.245,-0.24,-0.235,-0.23,-0.225,-0.22,
-0.215,-0.21,-0.205,-0.2,-0.195,-0.19,-0.185,-0.18,-0.175,-0.17,-0.165,
-0.16,-0.155,-0.15,-0.145,-0.14,-0.135,-0.13,-0.125,-0.12,-0.115,-0.11,
-0.105,-0.1,-0.095,-0.09,-0.085,-0.08,-0.075,-0.07,-0.065,-0.06,-0.055,
-0.05,-0.045,-0.04,-0.035,-0.03,-0.025,-0.02,-0.015,-0.01,-0.005,0.),
 .UNSPECIFIED.)
CURVE()
GEOMETRIC_REPRESENTATION_ITEM()
RATIONAL_B_SPLINE_CURVE((1.,1.,1.,1.,1.,1.,1.,1.,1.,1.,1.,1.,1.,1.,1.,1.,
1.,1.,1.,1.,1.,1.,1.,1.,1.,1.,1.,1.,1.,1.,1.,1.,1.,1.,1.,1.,1.,1.,1.,1.,
1.,1.,1.,1.,1.,1.,1.,1.,1.,1.,1.,1.,1.,1.,1.,1.,1.,1.,1.,1.,1.,1.,1.,1.,
1.,1.,1.,1.,1.,1.,1.,1.,1.,1.,1.,1.,1.,1.,1.,1.,1.,1.,1.,1.,1.,1.,1.,1.,
1.,1.,1.,1.,1.,1.,1.,1.,1.,1.,1.,1.,1.,1.,1.,1.,1.,1.,1.,1.,1.,1.,1.,1.,
1.,1.,1.,1.,1.,1.,1.,1.,1.,1.,1.,1.,1.,1.,1.,1.,1.,1.,1.,1.,1.,1.,1.,1.,
1.,1.,1.,1.,1.,1.,1.,1.,1.,1.,1.,1.,1.,1.,1.,1.,1.,1.,1.,1.,1.,1.,1.,1.,
1.,1.,1.,1.,1.,1.,1.,1.,1.,1.,1.,1.,1.,1.,1.,1.,1.,1.,1.,1.,1.,1.,1.,1.,
1.,1.,1.,1.,1.,1.,1.,1.,1.,1.))
REPRESENTATION_ITEM('')
);
#609=(
BOUNDED_CURVE()
B_SPLINE_CURVE(5,(#142235,#142236,#142237,#142238,#142239,#142240,#142241,
#142242,#142243,#142244,#142245,#142246,#142247,#142248,#142249,#142250,
#142251,#142252,#142253,#142254,#142255,#142256,#142257,#142258,#142259,
#142260,#142261,#142262,#142263,#142264,#142265,#142266,#142267,#142268,
#142269,#142270,#142271,#142272,#142273,#142274,#142275,#142276,#142277,
#142278,#142279,#142280,#142281,#142282,#142283,#142284,#142285,#142286,
#142287,#142288,#142289,#142290,#142291,#142292,#142293,#142294,#142295,
#142296,#142297,#142298,#142299,#142300,#142301,#142302,#142303,#142304,
#142305,#142306,#142307,#142308,#142309,#142310,#142311,#142312,#142313,
#142314,#142315,#142316,#142317,#142318,#142319,#142320,#142321,#142322,
#142323,#142324,#142325,#142326,#142327,#142328,#142329,#142330,#142331,
#142332,#142333,#142334,#142335,#142336,#142337,#142338,#142339,#142340,
#142341,#142342,#142343,#142344,#142345,#142346,#142347,#142348,#142349,
#142350,#142351,#142352,#142353,#142354,#142355,#142356,#142357,#142358,
#142359,#142360,#142361,#142362,#142363,#142364,#142365,#142366,#142367,
#142368,#142369,#142370,#142371,#142372,#142373,#142374,#142375,#142376,
#142377,#142378,#142379,#142380,#142381,#142382,#142383,#142384,#142385,
#142386,#142387,#142388,#142389,#142390,#142391,#142392,#142393,#142394,
#142395,#142396,#142397,#142398,#142399,#142400,#142401,#142402,#142403,
#142404,#142405,#142406,#142407,#142408,#142409,#142410,#142411,#142412,
#142413,#142414,#142415,#142416,#142417,#142418,#142419,#142420,#142421,
#142422,#142423,#142424,#142425,#142426,#142427,#142428),.UNSPECIFIED.,
 .F.,.F.)
B_SPLINE_CURVE_WITH_KNOTS((6,1,1,1,1,1,1,1,1,1,1,1,1,1,1,1,1,1,1,1,1,1,
1,1,1,1,1,1,1,1,1,1,1,1,1,1,1,1,1,1,1,1,1,1,1,1,1,1,1,1,1,1,1,1,1,1,1,1,
1,1,1,1,1,1,1,1,1,1,1,1,1,1,1,1,1,1,1,1,1,1,1,1,1,1,1,1,1,1,1,1,1,1,1,1,
1,1,1,1,1,1,1,1,1,1,1,1,1,1,1,1,1,1,1,1,1,1,1,1,1,1,1,1,1,1,1,1,1,1,1,1,
1,1,1,1,1,1,1,1,1,1,1,1,1,1,1,1,1,1,1,1,1,1,1,1,1,1,1,1,1,1,1,1,1,1,1,1,
1,1,1,1,1,1,1,1,1,1,1,1,1,1,1,1,1,1,1,1,1,1,1,6),(0.,0.005,0.01,0.015,0.02,
0.025,0.03,0.035,0.04,0.045,0.05,0.055,0.06,0.065,0.07,0.075,0.08,0.085,
0.09,0.095,0.1,0.105,0.11,0.115,0.12,0.125,0.13,0.135,0.14,0.145,0.15,0.155,
0.16,0.165,0.17,0.175,0.18,0.185,0.19,0.195,0.2,0.205,0.21,0.215,0.22,0.225,
0.23,0.235,0.24,0.245,0.25,0.255,0.26,0.265,0.27,0.275,0.28,0.285,0.29,
0.295,0.3,0.305,0.31,0.315,0.32,0.325,0.33,0.335,0.34,0.345,0.35,0.355,
0.36,0.365,0.37,0.375,0.38,0.385,0.39,0.395,0.4,0.405,0.41,0.415,0.42,0.425,
0.43,0.435,0.44,0.445,0.45,0.455,0.46,0.465,0.47,0.475,0.48,0.485,0.49,
0.495,0.5,0.505,0.51,0.515,0.52,0.525,0.53,0.535,0.54,0.545,0.55,0.555,
0.56,0.565,0.57,0.575,0.58,0.585,0.59,0.595,0.6,0.605,0.61,0.615,0.62,0.625,
0.63,0.635,0.64,0.645,0.65,0.655,0.66,0.665,0.67,0.675,0.68,0.685,0.690000000000001,
0.695000000000001,0.700000000000001,0.705000000000001,0.710000000000001,
0.715000000000001,0.720000000000001,0.725000000000001,0.730000000000001,
0.735000000000001,0.740000000000001,0.745000000000001,0.750000000000001,
0.755000000000001,0.760000000000001,0.765000000000001,0.770000000000001,
0.775000000000001,0.780000000000001,0.785000000000001,0.790000000000001,
0.795000000000001,0.800000000000001,0.805000000000001,0.810000000000001,
0.815000000000001,0.820000000000001,0.825000000000001,0.830000000000001,
0.835000000000001,0.840000000000001,0.845000000000001,0.850000000000001,
0.855000000000001,0.860000000000001,0.865000000000001,0.870000000000001,
0.875000000000001,0.880000000000001,0.885000000000001,0.890000000000001,
0.895000000000001,0.900000000000001,0.905000000000001,0.910000000000001,
0.915000000000001,0.920000000000001,0.925000000000001,0.930000000000001,
0.935000000000001,0.940000000000001,0.94142984443807),.UNSPECIFIED.)
CURVE()
GEOMETRIC_REPRESENTATION_ITEM()
RATIONAL_B_SPLINE_CURVE((1.,1.,1.,1.,1.,1.,1.,1.,1.,1.,1.,1.,1.,1.,1.,1.,
1.,1.,1.,1.,1.,1.,1.,1.,1.,1.,1.,1.,1.,1.,1.,1.,1.,1.,1.,1.,1.,1.,1.,1.,
1.,1.,1.,1.,1.,1.,1.,1.,1.,1.,1.,1.,1.,1.,1.,1.,1.,1.,1.,1.,1.,1.,1.,1.,
1.,1.,1.,1.,1.,1.,1.,1.,1.,1.,1.,1.,1.,1.,1.,1.,1.,1.,1.,1.,1.,1.,1.,1.,
1.,1.,1.,1.,1.,1.,1.,1.,1.,1.,1.,1.,1.,1.,1.,1.,1.,1.,1.,1.,1.,1.,1.,1.,
1.,1.,1.,1.,1.,1.,1.,1.,1.,1.,1.,1.,1.,1.,1.,1.,1.,1.,1.,1.,1.,1.,1.,1.,
1.,1.,1.,1.,1.,1.,1.,1.,1.,1.,1.,1.,1.,1.,1.,1.,1.,1.,1.,1.,1.,1.,1.,1.,
1.,1.,1.,1.,1.,1.,1.,1.,1.,1.,1.,1.,1.,1.,1.,1.,1.,1.,1.,1.,1.,1.,1.,1.,
1.,1.,1.,1.,1.,1.,1.,1.,1.,1.))
REPRESENTATION_ITEM('')
);
#610=(
BOUNDED_CURVE()
B_SPLINE_CURVE(5,(#142431,#142432,#142433,#142434,#142435,#142436,#142437,
#142438,#142439,#142440,#142441,#142442,#142443,#142444,#142445,#142446,
#142447,#142448,#142449,#142450,#142451,#142452,#142453,#142454,#142455,
#142456,#142457,#142458,#142459,#142460,#142461,#142462,#142463,#142464,
#142465,#142466,#142467,#142468,#142469,#142470,#142471,#142472,#142473,
#142474,#142475,#142476,#142477,#142478,#142479,#142480,#142481,#142482,
#142483,#142484,#142485,#142486,#142487,#142488,#142489,#142490,#142491,
#142492,#142493,#142494,#142495,#142496,#142497,#142498,#142499,#142500,
#142501,#142502,#142503,#142504,#142505,#142506,#142507,#142508,#142509,
#142510,#142511,#142512,#142513,#142514,#142515,#142516,#142517,#142518,
#142519,#142520,#142521,#142522,#142523,#142524,#142525,#142526,#142527,
#142528,#142529,#142530,#142531,#142532,#142533,#142534,#142535,#142536,
#142537,#142538,#142539,#142540,#142541,#142542,#142543,#142544,#142545,
#142546,#142547,#142548,#142549,#142550,#142551,#142552,#142553,#142554,
#142555,#142556,#142557,#142558,#142559,#142560,#142561,#142562,#142563,
#142564,#142565,#142566,#142567,#142568,#142569,#142570,#142571,#142572,
#142573,#142574,#142575,#142576,#142577,#142578,#142579,#142580,#142581,
#142582,#142583,#142584,#142585,#142586,#142587,#142588,#142589,#142590,
#142591,#142592,#142593,#142594,#142595,#142596,#142597,#142598,#142599,
#142600,#142601,#142602,#142603,#142604,#142605,#142606,#142607,#142608,
#142609,#142610,#142611,#142612,#142613,#142614,#142615,#142616,#142617,
#142618,#142619,#142620,#142621,#142622,#142623,#142624),.UNSPECIFIED.,
 .F.,.F.)
B_SPLINE_CURVE_WITH_KNOTS((6,1,1,1,1,1,1,1,1,1,1,1,1,1,1,1,1,1,1,1,1,1,
1,1,1,1,1,1,1,1,1,1,1,1,1,1,1,1,1,1,1,1,1,1,1,1,1,1,1,1,1,1,1,1,1,1,1,1,
1,1,1,1,1,1,1,1,1,1,1,1,1,1,1,1,1,1,1,1,1,1,1,1,1,1,1,1,1,1,1,1,1,1,1,1,
1,1,1,1,1,1,1,1,1,1,1,1,1,1,1,1,1,1,1,1,1,1,1,1,1,1,1,1,1,1,1,1,1,1,1,1,
1,1,1,1,1,1,1,1,1,1,1,1,1,1,1,1,1,1,1,1,1,1,1,1,1,1,1,1,1,1,1,1,1,1,1,1,
1,1,1,1,1,1,1,1,1,1,1,1,1,1,1,1,1,1,1,1,1,1,1,6),(-0.94142984443807,-0.940000000000001,
-0.935000000000001,-0.930000000000001,-0.925000000000001,-0.920000000000001,
-0.915000000000001,-0.910000000000001,-0.905000000000001,-0.900000000000001,
-0.895000000000001,-0.890000000000001,-0.885000000000001,-0.880000000000001,
-0.875000000000001,-0.870000000000001,-0.865000000000001,-0.860000000000001,
-0.855000000000001,-0.850000000000001,-0.845000000000001,-0.840000000000001,
-0.835000000000001,-0.830000000000001,-0.825000000000001,-0.820000000000001,
-0.815000000000001,-0.810000000000001,-0.805000000000001,-0.800000000000001,
-0.795000000000001,-0.790000000000001,-0.785000000000001,-0.780000000000001,
-0.775000000000001,-0.770000000000001,-0.765000000000001,-0.760000000000001,
-0.755000000000001,-0.750000000000001,-0.745000000000001,-0.740000000000001,
-0.735000000000001,-0.730000000000001,-0.725000000000001,-0.720000000000001,
-0.715000000000001,-0.710000000000001,-0.705000000000001,-0.700000000000001,
-0.695000000000001,-0.690000000000001,-0.685,-0.68,-0.675,-0.67,-0.665,
-0.66,-0.655,-0.65,-0.645,-0.64,-0.635,-0.63,-0.625,-0.62,-0.615,-0.61,
-0.605,-0.6,-0.595,-0.59,-0.585,-0.58,-0.575,-0.57,-0.565,-0.56,-0.555,
-0.55,-0.545,-0.54,-0.535,-0.53,-0.525,-0.52,-0.515,-0.51,-0.505,-0.5,-0.495,
-0.49,-0.485,-0.48,-0.475,-0.47,-0.465,-0.46,-0.455,-0.45,-0.445,-0.44,
-0.435,-0.43,-0.425,-0.42,-0.415,-0.41,-0.405,-0.4,-0.395,-0.39,-0.385,
-0.38,-0.375,-0.37,-0.365,-0.36,-0.355,-0.35,-0.345,-0.34,-0.335,-0.33,
-0.325,-0.32,-0.315,-0.31,-0.305,-0.3,-0.295,-0.29,-0.285,-0.28,-0.275,
-0.27,-0.265,-0.26,-0.255,-0.25,-0.245,-0.24,-0.235,-0.23,-0.225,-0.22,
-0.215,-0.21,-0.205,-0.2,-0.195,-0.19,-0.185,-0.18,-0.175,-0.17,-0.165,
-0.16,-0.155,-0.15,-0.145,-0.14,-0.135,-0.13,-0.125,-0.12,-0.115,-0.11,
-0.105,-0.1,-0.095,-0.09,-0.085,-0.08,-0.075,-0.07,-0.065,-0.06,-0.055,
-0.05,-0.045,-0.04,-0.035,-0.03,-0.025,-0.02,-0.015,-0.01,-0.005,0.),
 .UNSPECIFIED.)
CURVE()
GEOMETRIC_REPRESENTATION_ITEM()
RATIONAL_B_SPLINE_CURVE((1.,1.,1.,1.,1.,1.,1.,1.,1.,1.,1.,1.,1.,1.,1.,1.,
1.,1.,1.,1.,1.,1.,1.,1.,1.,1.,1.,1.,1.,1.,1.,1.,1.,1.,1.,1.,1.,1.,1.,1.,
1.,1.,1.,1.,1.,1.,1.,1.,1.,1.,1.,1.,1.,1.,1.,1.,1.,1.,1.,1.,1.,1.,1.,1.,
1.,1.,1.,1.,1.,1.,1.,1.,1.,1.,1.,1.,1.,1.,1.,1.,1.,1.,1.,1.,1.,1.,1.,1.,
1.,1.,1.,1.,1.,1.,1.,1.,1.,1.,1.,1.,1.,1.,1.,1.,1.,1.,1.,1.,1.,1.,1.,1.,
1.,1.,1.,1.,1.,1.,1.,1.,1.,1.,1.,1.,1.,1.,1.,1.,1.,1.,1.,1.,1.,1.,1.,1.,
1.,1.,1.,1.,1.,1.,1.,1.,1.,1.,1.,1.,1.,1.,1.,1.,1.,1.,1.,1.,1.,1.,1.,1.,
1.,1.,1.,1.,1.,1.,1.,1.,1.,1.,1.,1.,1.,1.,1.,1.,1.,1.,1.,1.,1.,1.,1.,1.,
1.,1.,1.,1.,1.,1.,1.,1.,1.,1.))
REPRESENTATION_ITEM('')
);
#611=(
BOUNDED_CURVE()
B_SPLINE_CURVE(5,(#143036,#143037,#143038,#143039,#143040,#143041,#143042,
#143043,#143044,#143045,#143046,#143047,#143048,#143049,#143050,#143051,
#143052,#143053,#143054,#143055,#143056,#143057,#143058,#143059,#143060,
#143061,#143062,#143063,#143064,#143065,#143066,#143067,#143068,#143069,
#143070,#143071,#143072,#143073,#143074,#143075,#143076,#143077,#143078,
#143079,#143080,#143081,#143082,#143083,#143084,#143085,#143086,#143087,
#143088,#143089,#143090,#143091,#143092,#143093,#143094,#143095,#143096,
#143097,#143098,#143099,#143100,#143101,#143102,#143103,#143104,#143105,
#143106,#143107,#143108,#143109,#143110,#143111,#143112,#143113,#143114,
#143115,#143116,#143117,#143118,#143119,#143120,#143121,#143122,#143123,
#143124,#143125,#143126,#143127,#143128,#143129,#143130,#143131,#143132,
#143133,#143134,#143135,#143136,#143137,#143138,#143139,#143140,#143141,
#143142,#143143,#143144,#143145,#143146,#143147,#143148,#143149,#143150,
#143151,#143152,#143153,#143154,#143155,#143156,#143157,#143158,#143159,
#143160,#143161,#143162,#143163,#143164,#143165,#143166,#143167,#143168,
#143169,#143170,#143171,#143172,#143173,#143174,#143175,#143176,#143177,
#143178,#143179,#143180,#143181,#143182,#143183,#143184,#143185,#143186,
#143187,#143188,#143189,#143190,#143191,#143192,#143193,#143194,#143195,
#143196,#143197,#143198,#143199,#143200,#143201,#143202,#143203,#143204,
#143205,#143206,#143207,#143208,#143209,#143210,#143211,#143212,#143213,
#143214,#143215,#143216,#143217,#143218,#143219,#143220,#143221,#143222,
#143223,#143224,#143225,#143226,#143227,#143228,#143229),.UNSPECIFIED.,
 .F.,.F.)
B_SPLINE_CURVE_WITH_KNOTS((6,1,1,1,1,1,1,1,1,1,1,1,1,1,1,1,1,1,1,1,1,1,
1,1,1,1,1,1,1,1,1,1,1,1,1,1,1,1,1,1,1,1,1,1,1,1,1,1,1,1,1,1,1,1,1,1,1,1,
1,1,1,1,1,1,1,1,1,1,1,1,1,1,1,1,1,1,1,1,1,1,1,1,1,1,1,1,1,1,1,1,1,1,1,1,
1,1,1,1,1,1,1,1,1,1,1,1,1,1,1,1,1,1,1,1,1,1,1,1,1,1,1,1,1,1,1,1,1,1,1,1,
1,1,1,1,1,1,1,1,1,1,1,1,1,1,1,1,1,1,1,1,1,1,1,1,1,1,1,1,1,1,1,1,1,1,1,1,
1,1,1,1,1,1,1,1,1,1,1,1,1,1,1,1,1,1,1,1,1,1,1,6),(0.,0.005,0.01,0.015,0.02,
0.025,0.03,0.035,0.04,0.045,0.05,0.055,0.06,0.065,0.07,0.075,0.08,0.085,
0.09,0.095,0.1,0.105,0.11,0.115,0.12,0.125,0.13,0.135,0.14,0.145,0.15,0.155,
0.16,0.165,0.17,0.175,0.18,0.185,0.19,0.195,0.2,0.205,0.21,0.215,0.22,0.225,
0.23,0.235,0.24,0.245,0.25,0.255,0.26,0.265,0.27,0.275,0.28,0.285,0.29,
0.295,0.3,0.305,0.31,0.315,0.32,0.325,0.33,0.335,0.34,0.345,0.35,0.355,
0.36,0.365,0.37,0.375,0.38,0.385,0.39,0.395,0.4,0.405,0.41,0.415,0.42,0.425,
0.43,0.435,0.44,0.445,0.45,0.455,0.46,0.465,0.47,0.475,0.48,0.485,0.49,
0.495,0.5,0.505,0.51,0.515,0.52,0.525,0.53,0.535,0.54,0.545,0.55,0.555,
0.56,0.565,0.57,0.575,0.58,0.585,0.59,0.595,0.6,0.605,0.61,0.615,0.62,0.625,
0.63,0.635,0.64,0.645,0.65,0.655,0.66,0.665,0.67,0.675,0.68,0.685,0.690000000000001,
0.695000000000001,0.700000000000001,0.705000000000001,0.710000000000001,
0.715000000000001,0.720000000000001,0.725000000000001,0.730000000000001,
0.735000000000001,0.740000000000001,0.745000000000001,0.750000000000001,
0.755000000000001,0.760000000000001,0.765000000000001,0.770000000000001,
0.775000000000001,0.780000000000001,0.785000000000001,0.790000000000001,
0.795000000000001,0.800000000000001,0.805000000000001,0.810000000000001,
0.815000000000001,0.820000000000001,0.825000000000001,0.830000000000001,
0.835000000000001,0.840000000000001,0.845000000000001,0.850000000000001,
0.855000000000001,0.860000000000001,0.865000000000001,0.870000000000001,
0.875000000000001,0.880000000000001,0.885000000000001,0.890000000000001,
0.895000000000001,0.900000000000001,0.905000000000001,0.910000000000001,
0.915000000000001,0.920000000000001,0.925000000000001,0.930000000000001,
0.935000000000001,0.940000000000001,0.941429844437991),.UNSPECIFIED.)
CURVE()
GEOMETRIC_REPRESENTATION_ITEM()
RATIONAL_B_SPLINE_CURVE((1.,1.,1.,1.,1.,1.,1.,1.,1.,1.,1.,1.,1.,1.,1.,1.,
1.,1.,1.,1.,1.,1.,1.,1.,1.,1.,1.,1.,1.,1.,1.,1.,1.,1.,1.,1.,1.,1.,1.,1.,
1.,1.,1.,1.,1.,1.,1.,1.,1.,1.,1.,1.,1.,1.,1.,1.,1.,1.,1.,1.,1.,1.,1.,1.,
1.,1.,1.,1.,1.,1.,1.,1.,1.,1.,1.,1.,1.,1.,1.,1.,1.,1.,1.,1.,1.,1.,1.,1.,
1.,1.,1.,1.,1.,1.,1.,1.,1.,1.,1.,1.,1.,1.,1.,1.,1.,1.,1.,1.,1.,1.,1.,1.,
1.,1.,1.,1.,1.,1.,1.,1.,1.,1.,1.,1.,1.,1.,1.,1.,1.,1.,1.,1.,1.,1.,1.,1.,
1.,1.,1.,1.,1.,1.,1.,1.,1.,1.,1.,1.,1.,1.,1.,1.,1.,1.,1.,1.,1.,1.,1.,1.,
1.,1.,1.,1.,1.,1.,1.,1.,1.,1.,1.,1.,1.,1.,1.,1.,1.,1.,1.,1.,1.,1.,1.,1.,
1.,1.,1.,1.,1.,1.,1.,1.,1.,1.))
REPRESENTATION_ITEM('')
);
#612=(
BOUNDED_CURVE()
B_SPLINE_CURVE(5,(#143232,#143233,#143234,#143235,#143236,#143237,#143238,
#143239,#143240,#143241,#143242,#143243,#143244,#143245,#143246,#143247,
#143248,#143249,#143250,#143251,#143252,#143253,#143254,#143255,#143256,
#143257,#143258,#143259,#143260,#143261,#143262,#143263,#143264,#143265,
#143266,#143267,#143268,#143269,#143270,#143271,#143272,#143273,#143274,
#143275,#143276,#143277,#143278,#143279,#143280,#143281,#143282,#143283,
#143284,#143285,#143286,#143287,#143288,#143289,#143290,#143291,#143292,
#143293,#143294,#143295,#143296,#143297,#143298,#143299,#143300,#143301,
#143302,#143303,#143304,#143305,#143306,#143307,#143308,#143309,#143310,
#143311,#143312,#143313,#143314,#143315,#143316,#143317,#143318,#143319,
#143320,#143321,#143322,#143323,#143324,#143325,#143326,#143327,#143328,
#143329,#143330,#143331,#143332,#143333,#143334,#143335,#143336,#143337,
#143338,#143339,#143340,#143341,#143342,#143343,#143344,#143345,#143346,
#143347,#143348,#143349,#143350,#143351,#143352,#143353,#143354,#143355,
#143356,#143357,#143358,#143359,#143360,#143361,#143362,#143363,#143364,
#143365,#143366,#143367,#143368,#143369,#143370,#143371,#143372,#143373,
#143374,#143375,#143376,#143377,#143378,#143379,#143380,#143381,#143382,
#143383,#143384,#143385,#143386,#143387,#143388,#143389,#143390,#143391,
#143392,#143393,#143394,#143395,#143396,#143397,#143398,#143399,#143400,
#143401,#143402,#143403,#143404,#143405,#143406,#143407,#143408,#143409,
#143410,#143411,#143412,#143413,#143414,#143415,#143416,#143417,#143418,
#143419,#143420,#143421,#143422,#143423,#143424,#143425),.UNSPECIFIED.,
 .F.,.F.)
B_SPLINE_CURVE_WITH_KNOTS((6,1,1,1,1,1,1,1,1,1,1,1,1,1,1,1,1,1,1,1,1,1,
1,1,1,1,1,1,1,1,1,1,1,1,1,1,1,1,1,1,1,1,1,1,1,1,1,1,1,1,1,1,1,1,1,1,1,1,
1,1,1,1,1,1,1,1,1,1,1,1,1,1,1,1,1,1,1,1,1,1,1,1,1,1,1,1,1,1,1,1,1,1,1,1,
1,1,1,1,1,1,1,1,1,1,1,1,1,1,1,1,1,1,1,1,1,1,1,1,1,1,1,1,1,1,1,1,1,1,1,1,
1,1,1,1,1,1,1,1,1,1,1,1,1,1,1,1,1,1,1,1,1,1,1,1,1,1,1,1,1,1,1,1,1,1,1,1,
1,1,1,1,1,1,1,1,1,1,1,1,1,1,1,1,1,1,1,1,1,1,1,6),(-0.94142984443798,-0.940000000000001,
-0.935000000000001,-0.930000000000001,-0.925000000000001,-0.920000000000001,
-0.915000000000001,-0.910000000000001,-0.905000000000001,-0.900000000000001,
-0.895000000000001,-0.890000000000001,-0.885000000000001,-0.880000000000001,
-0.875000000000001,-0.870000000000001,-0.865000000000001,-0.860000000000001,
-0.855000000000001,-0.850000000000001,-0.845000000000001,-0.840000000000001,
-0.835000000000001,-0.830000000000001,-0.825000000000001,-0.820000000000001,
-0.815000000000001,-0.810000000000001,-0.805000000000001,-0.800000000000001,
-0.795000000000001,-0.790000000000001,-0.785000000000001,-0.780000000000001,
-0.775000000000001,-0.770000000000001,-0.765000000000001,-0.760000000000001,
-0.755000000000001,-0.750000000000001,-0.745000000000001,-0.740000000000001,
-0.735000000000001,-0.730000000000001,-0.725000000000001,-0.720000000000001,
-0.715000000000001,-0.710000000000001,-0.705000000000001,-0.700000000000001,
-0.695000000000001,-0.690000000000001,-0.685,-0.68,-0.675,-0.67,-0.665,
-0.66,-0.655,-0.65,-0.645,-0.64,-0.635,-0.63,-0.625,-0.62,-0.615,-0.61,
-0.605,-0.6,-0.595,-0.59,-0.585,-0.58,-0.575,-0.57,-0.565,-0.56,-0.555,
-0.55,-0.545,-0.54,-0.535,-0.53,-0.525,-0.52,-0.515,-0.51,-0.505,-0.5,-0.495,
-0.49,-0.485,-0.48,-0.475,-0.47,-0.465,-0.46,-0.455,-0.45,-0.445,-0.44,
-0.435,-0.43,-0.425,-0.42,-0.415,-0.41,-0.405,-0.4,-0.395,-0.39,-0.385,
-0.38,-0.375,-0.37,-0.365,-0.36,-0.355,-0.35,-0.345,-0.34,-0.335,-0.33,
-0.325,-0.32,-0.315,-0.31,-0.305,-0.3,-0.295,-0.29,-0.285,-0.28,-0.275,
-0.27,-0.265,-0.26,-0.255,-0.25,-0.245,-0.24,-0.235,-0.23,-0.225,-0.22,
-0.215,-0.21,-0.205,-0.2,-0.195,-0.19,-0.185,-0.18,-0.175,-0.17,-0.165,
-0.16,-0.155,-0.15,-0.145,-0.14,-0.135,-0.13,-0.125,-0.12,-0.115,-0.11,
-0.105,-0.1,-0.095,-0.09,-0.085,-0.08,-0.075,-0.07,-0.065,-0.06,-0.055,
-0.05,-0.045,-0.04,-0.035,-0.03,-0.025,-0.02,-0.015,-0.01,-0.005,0.),
 .UNSPECIFIED.)
CURVE()
GEOMETRIC_REPRESENTATION_ITEM()
RATIONAL_B_SPLINE_CURVE((1.,1.,1.,1.,1.,1.,1.,1.,1.,1.,1.,1.,1.,1.,1.,1.,
1.,1.,1.,1.,1.,1.,1.,1.,1.,1.,1.,1.,1.,1.,1.,1.,1.,1.,1.,1.,1.,1.,1.,1.,
1.,1.,1.,1.,1.,1.,1.,1.,1.,1.,1.,1.,1.,1.,1.,1.,1.,1.,1.,1.,1.,1.,1.,1.,
1.,1.,1.,1.,1.,1.,1.,1.,1.,1.,1.,1.,1.,1.,1.,1.,1.,1.,1.,1.,1.,1.,1.,1.,
1.,1.,1.,1.,1.,1.,1.,1.,1.,1.,1.,1.,1.,1.,1.,1.,1.,1.,1.,1.,1.,1.,1.,1.,
1.,1.,1.,1.,1.,1.,1.,1.,1.,1.,1.,1.,1.,1.,1.,1.,1.,1.,1.,1.,1.,1.,1.,1.,
1.,1.,1.,1.,1.,1.,1.,1.,1.,1.,1.,1.,1.,1.,1.,1.,1.,1.,1.,1.,1.,1.,1.,1.,
1.,1.,1.,1.,1.,1.,1.,1.,1.,1.,1.,1.,1.,1.,1.,1.,1.,1.,1.,1.,1.,1.,1.,1.,
1.,1.,1.,1.,1.,1.,1.,1.,1.,1.))
REPRESENTATION_ITEM('')
);
#613=(
BOUNDED_CURVE()
B_SPLINE_CURVE(5,(#143837,#143838,#143839,#143840,#143841,#143842,#143843,
#143844,#143845,#143846,#143847,#143848,#143849,#143850,#143851,#143852,
#143853,#143854,#143855,#143856,#143857,#143858,#143859,#143860,#143861,
#143862,#143863,#143864,#143865,#143866,#143867,#143868,#143869,#143870,
#143871,#143872,#143873,#143874,#143875,#143876,#143877,#143878,#143879,
#143880,#143881,#143882,#143883,#143884,#143885,#143886,#143887,#143888,
#143889,#143890,#143891,#143892,#143893,#143894,#143895,#143896,#143897,
#143898,#143899,#143900,#143901,#143902,#143903,#143904,#143905,#143906,
#143907,#143908,#143909,#143910,#143911,#143912,#143913,#143914,#143915,
#143916,#143917,#143918,#143919,#143920,#143921,#143922,#143923,#143924,
#143925,#143926,#143927,#143928,#143929,#143930,#143931,#143932,#143933,
#143934,#143935,#143936,#143937,#143938,#143939,#143940,#143941,#143942,
#143943,#143944,#143945,#143946,#143947,#143948,#143949,#143950,#143951,
#143952,#143953,#143954,#143955,#143956,#143957,#143958,#143959,#143960,
#143961,#143962,#143963,#143964,#143965,#143966,#143967,#143968,#143969,
#143970,#143971,#143972,#143973,#143974,#143975,#143976,#143977,#143978,
#143979,#143980,#143981,#143982,#143983,#143984,#143985,#143986,#143987,
#143988,#143989,#143990,#143991,#143992,#143993,#143994,#143995,#143996,
#143997,#143998,#143999,#144000,#144001,#144002,#144003,#144004,#144005,
#144006,#144007,#144008,#144009,#144010,#144011,#144012,#144013,#144014,
#144015,#144016,#144017,#144018,#144019,#144020,#144021,#144022,#144023,
#144024,#144025,#144026,#144027,#144028,#144029,#144030),.UNSPECIFIED.,
 .F.,.F.)
B_SPLINE_CURVE_WITH_KNOTS((6,1,1,1,1,1,1,1,1,1,1,1,1,1,1,1,1,1,1,1,1,1,
1,1,1,1,1,1,1,1,1,1,1,1,1,1,1,1,1,1,1,1,1,1,1,1,1,1,1,1,1,1,1,1,1,1,1,1,
1,1,1,1,1,1,1,1,1,1,1,1,1,1,1,1,1,1,1,1,1,1,1,1,1,1,1,1,1,1,1,1,1,1,1,1,
1,1,1,1,1,1,1,1,1,1,1,1,1,1,1,1,1,1,1,1,1,1,1,1,1,1,1,1,1,1,1,1,1,1,1,1,
1,1,1,1,1,1,1,1,1,1,1,1,1,1,1,1,1,1,1,1,1,1,1,1,1,1,1,1,1,1,1,1,1,1,1,1,
1,1,1,1,1,1,1,1,1,1,1,1,1,1,1,1,1,1,1,1,1,1,1,6),(0.,0.005,0.01,0.015,0.02,
0.025,0.03,0.035,0.04,0.045,0.05,0.055,0.06,0.065,0.07,0.075,0.08,0.085,
0.09,0.095,0.1,0.105,0.11,0.115,0.12,0.125,0.13,0.135,0.14,0.145,0.15,0.155,
0.16,0.165,0.17,0.175,0.18,0.185,0.19,0.195,0.2,0.205,0.21,0.215,0.22,0.225,
0.23,0.235,0.24,0.245,0.25,0.255,0.26,0.265,0.27,0.275,0.28,0.285,0.29,
0.295,0.3,0.305,0.31,0.315,0.32,0.325,0.33,0.335,0.34,0.345,0.35,0.355,
0.36,0.365,0.37,0.375,0.38,0.385,0.39,0.395,0.4,0.405,0.41,0.415,0.42,0.425,
0.43,0.435,0.44,0.445,0.45,0.455,0.46,0.465,0.47,0.475,0.48,0.485,0.49,
0.495,0.5,0.505,0.51,0.515,0.52,0.525,0.53,0.535,0.54,0.545,0.55,0.555,
0.56,0.565,0.57,0.575,0.58,0.585,0.59,0.595,0.6,0.605,0.61,0.615,0.62,0.625,
0.63,0.635,0.64,0.645,0.65,0.655,0.66,0.665,0.67,0.675,0.68,0.685,0.690000000000001,
0.695000000000001,0.700000000000001,0.705000000000001,0.710000000000001,
0.715000000000001,0.720000000000001,0.725000000000001,0.730000000000001,
0.735000000000001,0.740000000000001,0.745000000000001,0.750000000000001,
0.755000000000001,0.760000000000001,0.765000000000001,0.770000000000001,
0.775000000000001,0.780000000000001,0.785000000000001,0.790000000000001,
0.795000000000001,0.800000000000001,0.805000000000001,0.810000000000001,
0.815000000000001,0.820000000000001,0.825000000000001,0.830000000000001,
0.835000000000001,0.840000000000001,0.845000000000001,0.850000000000001,
0.855000000000001,0.860000000000001,0.865000000000001,0.870000000000001,
0.875000000000001,0.880000000000001,0.885000000000001,0.890000000000001,
0.895000000000001,0.900000000000001,0.905000000000001,0.910000000000001,
0.915000000000001,0.920000000000001,0.925000000000001,0.930000000000001,
0.935000000000001,0.940000000000001,0.941429844438089),.UNSPECIFIED.)
CURVE()
GEOMETRIC_REPRESENTATION_ITEM()
RATIONAL_B_SPLINE_CURVE((1.,1.,1.,1.,1.,1.,1.,1.,1.,1.,1.,1.,1.,1.,1.,1.,
1.,1.,1.,1.,1.,1.,1.,1.,1.,1.,1.,1.,1.,1.,1.,1.,1.,1.,1.,1.,1.,1.,1.,1.,
1.,1.,1.,1.,1.,1.,1.,1.,1.,1.,1.,1.,1.,1.,1.,1.,1.,1.,1.,1.,1.,1.,1.,1.,
1.,1.,1.,1.,1.,1.,1.,1.,1.,1.,1.,1.,1.,1.,1.,1.,1.,1.,1.,1.,1.,1.,1.,1.,
1.,1.,1.,1.,1.,1.,1.,1.,1.,1.,1.,1.,1.,1.,1.,1.,1.,1.,1.,1.,1.,1.,1.,1.,
1.,1.,1.,1.,1.,1.,1.,1.,1.,1.,1.,1.,1.,1.,1.,1.,1.,1.,1.,1.,1.,1.,1.,1.,
1.,1.,1.,1.,1.,1.,1.,1.,1.,1.,1.,1.,1.,1.,1.,1.,1.,1.,1.,1.,1.,1.,1.,1.,
1.,1.,1.,1.,1.,1.,1.,1.,1.,1.,1.,1.,1.,1.,1.,1.,1.,1.,1.,1.,1.,1.,1.,1.,
1.,1.,1.,1.,1.,1.,1.,1.,1.,1.))
REPRESENTATION_ITEM('')
);
#614=(
BOUNDED_CURVE()
B_SPLINE_CURVE(5,(#144033,#144034,#144035,#144036,#144037,#144038,#144039,
#144040,#144041,#144042,#144043,#144044,#144045,#144046,#144047,#144048,
#144049,#144050,#144051,#144052,#144053,#144054,#144055,#144056,#144057,
#144058,#144059,#144060,#144061,#144062,#144063,#144064,#144065,#144066,
#144067,#144068,#144069,#144070,#144071,#144072,#144073,#144074,#144075,
#144076,#144077,#144078,#144079,#144080,#144081,#144082,#144083,#144084,
#144085,#144086,#144087,#144088,#144089,#144090,#144091,#144092,#144093,
#144094,#144095,#144096,#144097,#144098,#144099,#144100,#144101,#144102,
#144103,#144104,#144105,#144106,#144107,#144108,#144109,#144110,#144111,
#144112,#144113,#144114,#144115,#144116,#144117,#144118,#144119,#144120,
#144121,#144122,#144123,#144124,#144125,#144126,#144127,#144128,#144129,
#144130,#144131,#144132,#144133,#144134,#144135,#144136,#144137,#144138,
#144139,#144140,#144141,#144142,#144143,#144144,#144145,#144146,#144147,
#144148,#144149,#144150,#144151,#144152,#144153,#144154,#144155,#144156,
#144157,#144158,#144159,#144160,#144161,#144162,#144163,#144164,#144165,
#144166,#144167,#144168,#144169,#144170,#144171,#144172,#144173,#144174,
#144175,#144176,#144177,#144178,#144179,#144180,#144181,#144182,#144183,
#144184,#144185,#144186,#144187,#144188,#144189,#144190,#144191,#144192,
#144193,#144194,#144195,#144196,#144197,#144198,#144199,#144200,#144201,
#144202,#144203,#144204,#144205,#144206,#144207,#144208,#144209,#144210,
#144211,#144212,#144213,#144214,#144215,#144216,#144217,#144218,#144219,
#144220,#144221,#144222,#144223,#144224,#144225,#144226),.UNSPECIFIED.,
 .F.,.F.)
B_SPLINE_CURVE_WITH_KNOTS((6,1,1,1,1,1,1,1,1,1,1,1,1,1,1,1,1,1,1,1,1,1,
1,1,1,1,1,1,1,1,1,1,1,1,1,1,1,1,1,1,1,1,1,1,1,1,1,1,1,1,1,1,1,1,1,1,1,1,
1,1,1,1,1,1,1,1,1,1,1,1,1,1,1,1,1,1,1,1,1,1,1,1,1,1,1,1,1,1,1,1,1,1,1,1,
1,1,1,1,1,1,1,1,1,1,1,1,1,1,1,1,1,1,1,1,1,1,1,1,1,1,1,1,1,1,1,1,1,1,1,1,
1,1,1,1,1,1,1,1,1,1,1,1,1,1,1,1,1,1,1,1,1,1,1,1,1,1,1,1,1,1,1,1,1,1,1,1,
1,1,1,1,1,1,1,1,1,1,1,1,1,1,1,1,1,1,1,1,1,1,1,6),(-0.941429844438087,-0.940000000000001,
-0.935000000000001,-0.930000000000001,-0.925000000000001,-0.920000000000001,
-0.915000000000001,-0.910000000000001,-0.905000000000001,-0.900000000000001,
-0.895000000000001,-0.890000000000001,-0.885000000000001,-0.880000000000001,
-0.875000000000001,-0.870000000000001,-0.865000000000001,-0.860000000000001,
-0.855000000000001,-0.850000000000001,-0.845000000000001,-0.840000000000001,
-0.835000000000001,-0.830000000000001,-0.825000000000001,-0.820000000000001,
-0.815000000000001,-0.810000000000001,-0.805000000000001,-0.800000000000001,
-0.795000000000001,-0.790000000000001,-0.785000000000001,-0.780000000000001,
-0.775000000000001,-0.770000000000001,-0.765000000000001,-0.760000000000001,
-0.755000000000001,-0.750000000000001,-0.745000000000001,-0.740000000000001,
-0.735000000000001,-0.730000000000001,-0.725000000000001,-0.720000000000001,
-0.715000000000001,-0.710000000000001,-0.705000000000001,-0.700000000000001,
-0.695000000000001,-0.690000000000001,-0.685,-0.68,-0.675,-0.67,-0.665,
-0.66,-0.655,-0.65,-0.645,-0.64,-0.635,-0.63,-0.625,-0.62,-0.615,-0.61,
-0.605,-0.6,-0.595,-0.59,-0.585,-0.58,-0.575,-0.57,-0.565,-0.56,-0.555,
-0.55,-0.545,-0.54,-0.535,-0.53,-0.525,-0.52,-0.515,-0.51,-0.505,-0.5,-0.495,
-0.49,-0.485,-0.48,-0.475,-0.47,-0.465,-0.46,-0.455,-0.45,-0.445,-0.44,
-0.435,-0.43,-0.425,-0.42,-0.415,-0.41,-0.405,-0.4,-0.395,-0.39,-0.385,
-0.38,-0.375,-0.37,-0.365,-0.36,-0.355,-0.35,-0.345,-0.34,-0.335,-0.33,
-0.325,-0.32,-0.315,-0.31,-0.305,-0.3,-0.295,-0.29,-0.285,-0.28,-0.275,
-0.27,-0.265,-0.26,-0.255,-0.25,-0.245,-0.24,-0.235,-0.23,-0.225,-0.22,
-0.215,-0.21,-0.205,-0.2,-0.195,-0.19,-0.185,-0.18,-0.175,-0.17,-0.165,
-0.16,-0.155,-0.15,-0.145,-0.14,-0.135,-0.13,-0.125,-0.12,-0.115,-0.11,
-0.105,-0.1,-0.095,-0.09,-0.085,-0.08,-0.075,-0.07,-0.065,-0.06,-0.055,
-0.05,-0.045,-0.04,-0.035,-0.03,-0.025,-0.02,-0.015,-0.01,-0.005,0.),
 .UNSPECIFIED.)
CURVE()
GEOMETRIC_REPRESENTATION_ITEM()
RATIONAL_B_SPLINE_CURVE((1.,1.,1.,1.,1.,1.,1.,1.,1.,1.,1.,1.,1.,1.,1.,1.,
1.,1.,1.,1.,1.,1.,1.,1.,1.,1.,1.,1.,1.,1.,1.,1.,1.,1.,1.,1.,1.,1.,1.,1.,
1.,1.,1.,1.,1.,1.,1.,1.,1.,1.,1.,1.,1.,1.,1.,1.,1.,1.,1.,1.,1.,1.,1.,1.,
1.,1.,1.,1.,1.,1.,1.,1.,1.,1.,1.,1.,1.,1.,1.,1.,1.,1.,1.,1.,1.,1.,1.,1.,
1.,1.,1.,1.,1.,1.,1.,1.,1.,1.,1.,1.,1.,1.,1.,1.,1.,1.,1.,1.,1.,1.,1.,1.,
1.,1.,1.,1.,1.,1.,1.,1.,1.,1.,1.,1.,1.,1.,1.,1.,1.,1.,1.,1.,1.,1.,1.,1.,
1.,1.,1.,1.,1.,1.,1.,1.,1.,1.,1.,1.,1.,1.,1.,1.,1.,1.,1.,1.,1.,1.,1.,1.,
1.,1.,1.,1.,1.,1.,1.,1.,1.,1.,1.,1.,1.,1.,1.,1.,1.,1.,1.,1.,1.,1.,1.,1.,
1.,1.,1.,1.,1.,1.,1.,1.,1.,1.))
REPRESENTATION_ITEM('')
);
#615=(
BOUNDED_CURVE()
B_SPLINE_CURVE(5,(#144638,#144639,#144640,#144641,#144642,#144643,#144644,
#144645,#144646,#144647,#144648,#144649,#144650,#144651,#144652,#144653,
#144654,#144655,#144656,#144657,#144658,#144659,#144660,#144661,#144662,
#144663,#144664,#144665,#144666,#144667,#144668,#144669,#144670,#144671,
#144672,#144673,#144674,#144675,#144676,#144677,#144678,#144679,#144680,
#144681,#144682,#144683,#144684,#144685,#144686,#144687,#144688,#144689,
#144690,#144691,#144692,#144693,#144694,#144695,#144696,#144697,#144698,
#144699,#144700,#144701,#144702,#144703,#144704,#144705,#144706,#144707,
#144708,#144709,#144710,#144711,#144712,#144713,#144714,#144715,#144716,
#144717,#144718,#144719,#144720,#144721,#144722,#144723,#144724,#144725,
#144726,#144727,#144728,#144729,#144730,#144731,#144732,#144733,#144734,
#144735,#144736,#144737,#144738,#144739,#144740,#144741,#144742,#144743,
#144744,#144745,#144746,#144747,#144748,#144749,#144750,#144751,#144752,
#144753,#144754,#144755,#144756,#144757,#144758,#144759,#144760,#144761,
#144762,#144763,#144764,#144765,#144766,#144767,#144768,#144769,#144770,
#144771,#144772,#144773,#144774,#144775,#144776,#144777,#144778,#144779,
#144780,#144781,#144782,#144783,#144784,#144785,#144786,#144787,#144788,
#144789,#144790,#144791,#144792,#144793,#144794,#144795,#144796,#144797,
#144798,#144799,#144800,#144801,#144802,#144803,#144804,#144805,#144806,
#144807,#144808,#144809,#144810,#144811,#144812,#144813,#144814,#144815,
#144816,#144817,#144818,#144819,#144820,#144821,#144822,#144823,#144824,
#144825,#144826,#144827,#144828,#144829,#144830,#144831),.UNSPECIFIED.,
 .F.,.F.)
B_SPLINE_CURVE_WITH_KNOTS((6,1,1,1,1,1,1,1,1,1,1,1,1,1,1,1,1,1,1,1,1,1,
1,1,1,1,1,1,1,1,1,1,1,1,1,1,1,1,1,1,1,1,1,1,1,1,1,1,1,1,1,1,1,1,1,1,1,1,
1,1,1,1,1,1,1,1,1,1,1,1,1,1,1,1,1,1,1,1,1,1,1,1,1,1,1,1,1,1,1,1,1,1,1,1,
1,1,1,1,1,1,1,1,1,1,1,1,1,1,1,1,1,1,1,1,1,1,1,1,1,1,1,1,1,1,1,1,1,1,1,1,
1,1,1,1,1,1,1,1,1,1,1,1,1,1,1,1,1,1,1,1,1,1,1,1,1,1,1,1,1,1,1,1,1,1,1,1,
1,1,1,1,1,1,1,1,1,1,1,1,1,1,1,1,1,1,1,1,1,1,1,6),(0.,0.005,0.01,0.015,0.02,
0.025,0.03,0.035,0.04,0.045,0.05,0.055,0.06,0.065,0.07,0.075,0.08,0.085,
0.09,0.095,0.1,0.105,0.11,0.115,0.12,0.125,0.13,0.135,0.14,0.145,0.15,0.155,
0.16,0.165,0.17,0.175,0.18,0.185,0.19,0.195,0.2,0.205,0.21,0.215,0.22,0.225,
0.23,0.235,0.24,0.245,0.25,0.255,0.26,0.265,0.27,0.275,0.28,0.285,0.29,
0.295,0.3,0.305,0.31,0.315,0.32,0.325,0.33,0.335,0.34,0.345,0.35,0.355,
0.36,0.365,0.37,0.375,0.38,0.385,0.39,0.395,0.4,0.405,0.41,0.415,0.42,0.425,
0.43,0.435,0.44,0.445,0.45,0.455,0.46,0.465,0.47,0.475,0.48,0.485,0.49,
0.495,0.5,0.505,0.51,0.515,0.52,0.525,0.53,0.535,0.54,0.545,0.55,0.555,
0.56,0.565,0.57,0.575,0.58,0.585,0.59,0.595,0.6,0.605,0.61,0.615,0.62,0.625,
0.63,0.635,0.64,0.645,0.65,0.655,0.66,0.665,0.67,0.675,0.68,0.685,0.690000000000001,
0.695000000000001,0.700000000000001,0.705000000000001,0.710000000000001,
0.715000000000001,0.720000000000001,0.725000000000001,0.730000000000001,
0.735000000000001,0.740000000000001,0.745000000000001,0.750000000000001,
0.755000000000001,0.760000000000001,0.765000000000001,0.770000000000001,
0.775000000000001,0.780000000000001,0.785000000000001,0.790000000000001,
0.795000000000001,0.800000000000001,0.805000000000001,0.810000000000001,
0.815000000000001,0.820000000000001,0.825000000000001,0.830000000000001,
0.835000000000001,0.840000000000001,0.845000000000001,0.850000000000001,
0.855000000000001,0.860000000000001,0.865000000000001,0.870000000000001,
0.875000000000001,0.880000000000001,0.885000000000001,0.890000000000001,
0.895000000000001,0.900000000000001,0.905000000000001,0.910000000000001,
0.915000000000001,0.920000000000001,0.925000000000001,0.930000000000001,
0.935000000000001,0.940000000000001,0.94142984443808),.UNSPECIFIED.)
CURVE()
GEOMETRIC_REPRESENTATION_ITEM()
RATIONAL_B_SPLINE_CURVE((1.,1.,1.,1.,1.,1.,1.,1.,1.,1.,1.,1.,1.,1.,1.,1.,
1.,1.,1.,1.,1.,1.,1.,1.,1.,1.,1.,1.,1.,1.,1.,1.,1.,1.,1.,1.,1.,1.,1.,1.,
1.,1.,1.,1.,1.,1.,1.,1.,1.,1.,1.,1.,1.,1.,1.,1.,1.,1.,1.,1.,1.,1.,1.,1.,
1.,1.,1.,1.,1.,1.,1.,1.,1.,1.,1.,1.,1.,1.,1.,1.,1.,1.,1.,1.,1.,1.,1.,1.,
1.,1.,1.,1.,1.,1.,1.,1.,1.,1.,1.,1.,1.,1.,1.,1.,1.,1.,1.,1.,1.,1.,1.,1.,
1.,1.,1.,1.,1.,1.,1.,1.,1.,1.,1.,1.,1.,1.,1.,1.,1.,1.,1.,1.,1.,1.,1.,1.,
1.,1.,1.,1.,1.,1.,1.,1.,1.,1.,1.,1.,1.,1.,1.,1.,1.,1.,1.,1.,1.,1.,1.,1.,
1.,1.,1.,1.,1.,1.,1.,1.,1.,1.,1.,1.,1.,1.,1.,1.,1.,1.,1.,1.,1.,1.,1.,1.,
1.,1.,1.,1.,1.,1.,1.,1.,1.,1.))
REPRESENTATION_ITEM('')
);
#616=(
BOUNDED_CURVE()
B_SPLINE_CURVE(5,(#144834,#144835,#144836,#144837,#144838,#144839,#144840,
#144841,#144842,#144843,#144844,#144845,#144846,#144847,#144848,#144849,
#144850,#144851,#144852,#144853,#144854,#144855,#144856,#144857,#144858,
#144859,#144860,#144861,#144862,#144863,#144864,#144865,#144866,#144867,
#144868,#144869,#144870,#144871,#144872,#144873,#144874,#144875,#144876,
#144877,#144878,#144879,#144880,#144881,#144882,#144883,#144884,#144885,
#144886,#144887,#144888,#144889,#144890,#144891,#144892,#144893,#144894,
#144895,#144896,#144897,#144898,#144899,#144900,#144901,#144902,#144903,
#144904,#144905,#144906,#144907,#144908,#144909,#144910,#144911,#144912,
#144913,#144914,#144915,#144916,#144917,#144918,#144919,#144920,#144921,
#144922,#144923,#144924,#144925,#144926,#144927,#144928,#144929,#144930,
#144931,#144932,#144933,#144934,#144935,#144936,#144937,#144938,#144939,
#144940,#144941,#144942,#144943,#144944,#144945,#144946,#144947,#144948,
#144949,#144950,#144951,#144952,#144953,#144954,#144955,#144956,#144957,
#144958,#144959,#144960,#144961,#144962,#144963,#144964,#144965,#144966,
#144967,#144968,#144969,#144970,#144971,#144972,#144973,#144974,#144975,
#144976,#144977,#144978,#144979,#144980,#144981,#144982,#144983,#144984,
#144985,#144986,#144987,#144988,#144989,#144990,#144991,#144992,#144993,
#144994,#144995,#144996,#144997,#144998,#144999,#145000,#145001,#145002,
#145003,#145004,#145005,#145006,#145007,#145008,#145009,#145010,#145011,
#145012,#145013,#145014,#145015,#145016,#145017,#145018,#145019,#145020,
#145021,#145022,#145023,#145024,#145025,#145026,#145027),.UNSPECIFIED.,
 .F.,.F.)
B_SPLINE_CURVE_WITH_KNOTS((6,1,1,1,1,1,1,1,1,1,1,1,1,1,1,1,1,1,1,1,1,1,
1,1,1,1,1,1,1,1,1,1,1,1,1,1,1,1,1,1,1,1,1,1,1,1,1,1,1,1,1,1,1,1,1,1,1,1,
1,1,1,1,1,1,1,1,1,1,1,1,1,1,1,1,1,1,1,1,1,1,1,1,1,1,1,1,1,1,1,1,1,1,1,1,
1,1,1,1,1,1,1,1,1,1,1,1,1,1,1,1,1,1,1,1,1,1,1,1,1,1,1,1,1,1,1,1,1,1,1,1,
1,1,1,1,1,1,1,1,1,1,1,1,1,1,1,1,1,1,1,1,1,1,1,1,1,1,1,1,1,1,1,1,1,1,1,1,
1,1,1,1,1,1,1,1,1,1,1,1,1,1,1,1,1,1,1,1,1,1,1,6),(-0.941429844438077,-0.940000000000001,
-0.935000000000001,-0.930000000000001,-0.925000000000001,-0.920000000000001,
-0.915000000000001,-0.910000000000001,-0.905000000000001,-0.900000000000001,
-0.895000000000001,-0.890000000000001,-0.885000000000001,-0.880000000000001,
-0.875000000000001,-0.870000000000001,-0.865000000000001,-0.860000000000001,
-0.855000000000001,-0.850000000000001,-0.845000000000001,-0.840000000000001,
-0.835000000000001,-0.830000000000001,-0.825000000000001,-0.820000000000001,
-0.815000000000001,-0.810000000000001,-0.805000000000001,-0.800000000000001,
-0.795000000000001,-0.790000000000001,-0.785000000000001,-0.780000000000001,
-0.775000000000001,-0.770000000000001,-0.765000000000001,-0.760000000000001,
-0.755000000000001,-0.750000000000001,-0.745000000000001,-0.740000000000001,
-0.735000000000001,-0.730000000000001,-0.725000000000001,-0.720000000000001,
-0.715000000000001,-0.710000000000001,-0.705000000000001,-0.700000000000001,
-0.695000000000001,-0.690000000000001,-0.685,-0.68,-0.675,-0.67,-0.665,
-0.66,-0.655,-0.65,-0.645,-0.64,-0.635,-0.63,-0.625,-0.62,-0.615,-0.61,
-0.605,-0.6,-0.595,-0.59,-0.585,-0.58,-0.575,-0.57,-0.565,-0.56,-0.555,
-0.55,-0.545,-0.54,-0.535,-0.53,-0.525,-0.52,-0.515,-0.51,-0.505,-0.5,-0.495,
-0.49,-0.485,-0.48,-0.475,-0.47,-0.465,-0.46,-0.455,-0.45,-0.445,-0.44,
-0.435,-0.43,-0.425,-0.42,-0.415,-0.41,-0.405,-0.4,-0.395,-0.39,-0.385,
-0.38,-0.375,-0.37,-0.365,-0.36,-0.355,-0.35,-0.345,-0.34,-0.335,-0.33,
-0.325,-0.32,-0.315,-0.31,-0.305,-0.3,-0.295,-0.29,-0.285,-0.28,-0.275,
-0.27,-0.265,-0.26,-0.255,-0.25,-0.245,-0.24,-0.235,-0.23,-0.225,-0.22,
-0.215,-0.21,-0.205,-0.2,-0.195,-0.19,-0.185,-0.18,-0.175,-0.17,-0.165,
-0.16,-0.155,-0.15,-0.145,-0.14,-0.135,-0.13,-0.125,-0.12,-0.115,-0.11,
-0.105,-0.1,-0.095,-0.09,-0.085,-0.08,-0.075,-0.07,-0.065,-0.06,-0.055,
-0.05,-0.045,-0.04,-0.035,-0.03,-0.025,-0.02,-0.015,-0.01,-0.005,0.),
 .UNSPECIFIED.)
CURVE()
GEOMETRIC_REPRESENTATION_ITEM()
RATIONAL_B_SPLINE_CURVE((1.,1.,1.,1.,1.,1.,1.,1.,1.,1.,1.,1.,1.,1.,1.,1.,
1.,1.,1.,1.,1.,1.,1.,1.,1.,1.,1.,1.,1.,1.,1.,1.,1.,1.,1.,1.,1.,1.,1.,1.,
1.,1.,1.,1.,1.,1.,1.,1.,1.,1.,1.,1.,1.,1.,1.,1.,1.,1.,1.,1.,1.,1.,1.,1.,
1.,1.,1.,1.,1.,1.,1.,1.,1.,1.,1.,1.,1.,1.,1.,1.,1.,1.,1.,1.,1.,1.,1.,1.,
1.,1.,1.,1.,1.,1.,1.,1.,1.,1.,1.,1.,1.,1.,1.,1.,1.,1.,1.,1.,1.,1.,1.,1.,
1.,1.,1.,1.,1.,1.,1.,1.,1.,1.,1.,1.,1.,1.,1.,1.,1.,1.,1.,1.,1.,1.,1.,1.,
1.,1.,1.,1.,1.,1.,1.,1.,1.,1.,1.,1.,1.,1.,1.,1.,1.,1.,1.,1.,1.,1.,1.,1.,
1.,1.,1.,1.,1.,1.,1.,1.,1.,1.,1.,1.,1.,1.,1.,1.,1.,1.,1.,1.,1.,1.,1.,1.,
1.,1.,1.,1.,1.,1.,1.,1.,1.,1.))
REPRESENTATION_ITEM('')
);
#617=(
BOUNDED_CURVE()
B_SPLINE_CURVE(5,(#145439,#145440,#145441,#145442,#145443,#145444,#145445,
#145446,#145447,#145448,#145449,#145450,#145451,#145452,#145453,#145454,
#145455,#145456,#145457,#145458,#145459,#145460,#145461,#145462,#145463,
#145464,#145465,#145466,#145467,#145468,#145469,#145470,#145471,#145472,
#145473,#145474,#145475,#145476,#145477,#145478,#145479,#145480,#145481,
#145482,#145483,#145484,#145485,#145486,#145487,#145488,#145489,#145490,
#145491,#145492,#145493,#145494,#145495,#145496,#145497,#145498,#145499,
#145500,#145501,#145502,#145503,#145504,#145505,#145506,#145507,#145508,
#145509,#145510,#145511,#145512,#145513,#145514,#145515,#145516,#145517,
#145518,#145519,#145520,#145521,#145522,#145523,#145524,#145525,#145526,
#145527,#145528,#145529,#145530,#145531,#145532,#145533,#145534,#145535,
#145536,#145537,#145538,#145539,#145540,#145541,#145542,#145543,#145544,
#145545,#145546,#145547,#145548,#145549,#145550,#145551,#145552,#145553,
#145554,#145555,#145556,#145557,#145558,#145559,#145560,#145561,#145562,
#145563,#145564,#145565,#145566,#145567,#145568,#145569,#145570,#145571,
#145572,#145573,#145574,#145575,#145576,#145577,#145578,#145579,#145580,
#145581,#145582,#145583,#145584,#145585,#145586,#145587,#145588,#145589,
#145590,#145591,#145592,#145593,#145594,#145595,#145596,#145597,#145598,
#145599,#145600,#145601,#145602,#145603,#145604,#145605,#145606,#145607,
#145608,#145609,#145610,#145611,#145612,#145613,#145614,#145615,#145616,
#145617,#145618,#145619,#145620,#145621,#145622,#145623,#145624,#145625,
#145626,#145627,#145628,#145629,#145630,#145631,#145632),.UNSPECIFIED.,
 .F.,.F.)
B_SPLINE_CURVE_WITH_KNOTS((6,1,1,1,1,1,1,1,1,1,1,1,1,1,1,1,1,1,1,1,1,1,
1,1,1,1,1,1,1,1,1,1,1,1,1,1,1,1,1,1,1,1,1,1,1,1,1,1,1,1,1,1,1,1,1,1,1,1,
1,1,1,1,1,1,1,1,1,1,1,1,1,1,1,1,1,1,1,1,1,1,1,1,1,1,1,1,1,1,1,1,1,1,1,1,
1,1,1,1,1,1,1,1,1,1,1,1,1,1,1,1,1,1,1,1,1,1,1,1,1,1,1,1,1,1,1,1,1,1,1,1,
1,1,1,1,1,1,1,1,1,1,1,1,1,1,1,1,1,1,1,1,1,1,1,1,1,1,1,1,1,1,1,1,1,1,1,1,
1,1,1,1,1,1,1,1,1,1,1,1,1,1,1,1,1,1,1,1,1,1,1,6),(0.,0.005,0.01,0.015,0.02,
0.025,0.03,0.035,0.04,0.045,0.05,0.055,0.06,0.065,0.07,0.075,0.08,0.085,
0.09,0.095,0.1,0.105,0.11,0.115,0.12,0.125,0.13,0.135,0.14,0.145,0.15,0.155,
0.16,0.165,0.17,0.175,0.18,0.185,0.19,0.195,0.2,0.205,0.21,0.215,0.22,0.225,
0.23,0.235,0.24,0.245,0.25,0.255,0.26,0.265,0.27,0.275,0.28,0.285,0.29,
0.295,0.3,0.305,0.31,0.315,0.32,0.325,0.33,0.335,0.34,0.345,0.35,0.355,
0.36,0.365,0.37,0.375,0.38,0.385,0.39,0.395,0.4,0.405,0.41,0.415,0.42,0.425,
0.43,0.435,0.44,0.445,0.45,0.455,0.46,0.465,0.47,0.475,0.48,0.485,0.49,
0.495,0.5,0.505,0.51,0.515,0.52,0.525,0.53,0.535,0.54,0.545,0.55,0.555,
0.56,0.565,0.57,0.575,0.58,0.585,0.59,0.595,0.6,0.605,0.61,0.615,0.62,0.625,
0.63,0.635,0.64,0.645,0.65,0.655,0.66,0.665,0.67,0.675,0.68,0.685,0.690000000000001,
0.695000000000001,0.700000000000001,0.705000000000001,0.710000000000001,
0.715000000000001,0.720000000000001,0.725000000000001,0.730000000000001,
0.735000000000001,0.740000000000001,0.745000000000001,0.750000000000001,
0.755000000000001,0.760000000000001,0.765000000000001,0.770000000000001,
0.775000000000001,0.780000000000001,0.785000000000001,0.790000000000001,
0.795000000000001,0.800000000000001,0.805000000000001,0.810000000000001,
0.815000000000001,0.820000000000001,0.825000000000001,0.830000000000001,
0.835000000000001,0.840000000000001,0.845000000000001,0.850000000000001,
0.855000000000001,0.860000000000001,0.865000000000001,0.870000000000001,
0.875000000000001,0.880000000000001,0.885000000000001,0.890000000000001,
0.895000000000001,0.900000000000001,0.905000000000001,0.910000000000001,
0.915000000000001,0.920000000000001,0.925000000000001,0.930000000000001,
0.935000000000001,0.940000000000001,0.941429844438071),.UNSPECIFIED.)
CURVE()
GEOMETRIC_REPRESENTATION_ITEM()
RATIONAL_B_SPLINE_CURVE((1.,1.,1.,1.,1.,1.,1.,1.,1.,1.,1.,1.,1.,1.,1.,1.,
1.,1.,1.,1.,1.,1.,1.,1.,1.,1.,1.,1.,1.,1.,1.,1.,1.,1.,1.,1.,1.,1.,1.,1.,
1.,1.,1.,1.,1.,1.,1.,1.,1.,1.,1.,1.,1.,1.,1.,1.,1.,1.,1.,1.,1.,1.,1.,1.,
1.,1.,1.,1.,1.,1.,1.,1.,1.,1.,1.,1.,1.,1.,1.,1.,1.,1.,1.,1.,1.,1.,1.,1.,
1.,1.,1.,1.,1.,1.,1.,1.,1.,1.,1.,1.,1.,1.,1.,1.,1.,1.,1.,1.,1.,1.,1.,1.,
1.,1.,1.,1.,1.,1.,1.,1.,1.,1.,1.,1.,1.,1.,1.,1.,1.,1.,1.,1.,1.,1.,1.,1.,
1.,1.,1.,1.,1.,1.,1.,1.,1.,1.,1.,1.,1.,1.,1.,1.,1.,1.,1.,1.,1.,1.,1.,1.,
1.,1.,1.,1.,1.,1.,1.,1.,1.,1.,1.,1.,1.,1.,1.,1.,1.,1.,1.,1.,1.,1.,1.,1.,
1.,1.,1.,1.,1.,1.,1.,1.,1.,1.))
REPRESENTATION_ITEM('')
);
#618=(
BOUNDED_CURVE()
B_SPLINE_CURVE(5,(#145635,#145636,#145637,#145638,#145639,#145640,#145641,
#145642,#145643,#145644,#145645,#145646,#145647,#145648,#145649,#145650,
#145651,#145652,#145653,#145654,#145655,#145656,#145657,#145658,#145659,
#145660,#145661,#145662,#145663,#145664,#145665,#145666,#145667,#145668,
#145669,#145670,#145671,#145672,#145673,#145674,#145675,#145676,#145677,
#145678,#145679,#145680,#145681,#145682,#145683,#145684,#145685,#145686,
#145687,#145688,#145689,#145690,#145691,#145692,#145693,#145694,#145695,
#145696,#145697,#145698,#145699,#145700,#145701,#145702,#145703,#145704,
#145705,#145706,#145707,#145708,#145709,#145710,#145711,#145712,#145713,
#145714,#145715,#145716,#145717,#145718,#145719,#145720,#145721,#145722,
#145723,#145724,#145725,#145726,#145727,#145728,#145729,#145730,#145731,
#145732,#145733,#145734,#145735,#145736,#145737,#145738,#145739,#145740,
#145741,#145742,#145743,#145744,#145745,#145746,#145747,#145748,#145749,
#145750,#145751,#145752,#145753,#145754,#145755,#145756,#145757,#145758,
#145759,#145760,#145761,#145762,#145763,#145764,#145765,#145766,#145767,
#145768,#145769,#145770,#145771,#145772,#145773,#145774,#145775,#145776,
#145777,#145778,#145779,#145780,#145781,#145782,#145783,#145784,#145785,
#145786,#145787,#145788,#145789,#145790,#145791,#145792,#145793,#145794,
#145795,#145796,#145797,#145798,#145799,#145800,#145801,#145802,#145803,
#145804,#145805,#145806,#145807,#145808,#145809,#145810,#145811,#145812,
#145813,#145814,#145815,#145816,#145817,#145818,#145819,#145820,#145821,
#145822,#145823,#145824,#145825,#145826,#145827,#145828),.UNSPECIFIED.,
 .F.,.F.)
B_SPLINE_CURVE_WITH_KNOTS((6,1,1,1,1,1,1,1,1,1,1,1,1,1,1,1,1,1,1,1,1,1,
1,1,1,1,1,1,1,1,1,1,1,1,1,1,1,1,1,1,1,1,1,1,1,1,1,1,1,1,1,1,1,1,1,1,1,1,
1,1,1,1,1,1,1,1,1,1,1,1,1,1,1,1,1,1,1,1,1,1,1,1,1,1,1,1,1,1,1,1,1,1,1,1,
1,1,1,1,1,1,1,1,1,1,1,1,1,1,1,1,1,1,1,1,1,1,1,1,1,1,1,1,1,1,1,1,1,1,1,1,
1,1,1,1,1,1,1,1,1,1,1,1,1,1,1,1,1,1,1,1,1,1,1,1,1,1,1,1,1,1,1,1,1,1,1,1,
1,1,1,1,1,1,1,1,1,1,1,1,1,1,1,1,1,1,1,1,1,1,1,6),(-0.941429844438071,-0.940000000000001,
-0.935000000000001,-0.930000000000001,-0.925000000000001,-0.920000000000001,
-0.915000000000001,-0.910000000000001,-0.905000000000001,-0.900000000000001,
-0.895000000000001,-0.890000000000001,-0.885000000000001,-0.880000000000001,
-0.875000000000001,-0.870000000000001,-0.865000000000001,-0.860000000000001,
-0.855000000000001,-0.850000000000001,-0.845000000000001,-0.840000000000001,
-0.835000000000001,-0.830000000000001,-0.825000000000001,-0.820000000000001,
-0.815000000000001,-0.810000000000001,-0.805000000000001,-0.800000000000001,
-0.795000000000001,-0.790000000000001,-0.785000000000001,-0.780000000000001,
-0.775000000000001,-0.770000000000001,-0.765000000000001,-0.760000000000001,
-0.755000000000001,-0.750000000000001,-0.745000000000001,-0.740000000000001,
-0.735000000000001,-0.730000000000001,-0.725000000000001,-0.720000000000001,
-0.715000000000001,-0.710000000000001,-0.705000000000001,-0.700000000000001,
-0.695000000000001,-0.690000000000001,-0.685,-0.68,-0.675,-0.67,-0.665,
-0.66,-0.655,-0.65,-0.645,-0.64,-0.635,-0.63,-0.625,-0.62,-0.615,-0.61,
-0.605,-0.6,-0.595,-0.59,-0.585,-0.58,-0.575,-0.57,-0.565,-0.56,-0.555,
-0.55,-0.545,-0.54,-0.535,-0.53,-0.525,-0.52,-0.515,-0.51,-0.505,-0.5,-0.495,
-0.49,-0.485,-0.48,-0.475,-0.47,-0.465,-0.46,-0.455,-0.45,-0.445,-0.44,
-0.435,-0.43,-0.425,-0.42,-0.415,-0.41,-0.405,-0.4,-0.395,-0.39,-0.385,
-0.38,-0.375,-0.37,-0.365,-0.36,-0.355,-0.35,-0.345,-0.34,-0.335,-0.33,
-0.325,-0.32,-0.315,-0.31,-0.305,-0.3,-0.295,-0.29,-0.285,-0.28,-0.275,
-0.27,-0.265,-0.26,-0.255,-0.25,-0.245,-0.24,-0.235,-0.23,-0.225,-0.22,
-0.215,-0.21,-0.205,-0.2,-0.195,-0.19,-0.185,-0.18,-0.175,-0.17,-0.165,
-0.16,-0.155,-0.15,-0.145,-0.14,-0.135,-0.13,-0.125,-0.12,-0.115,-0.11,
-0.105,-0.1,-0.095,-0.09,-0.085,-0.08,-0.075,-0.07,-0.065,-0.06,-0.055,
-0.05,-0.045,-0.04,-0.035,-0.03,-0.025,-0.02,-0.015,-0.01,-0.005,0.),
 .UNSPECIFIED.)
CURVE()
GEOMETRIC_REPRESENTATION_ITEM()
RATIONAL_B_SPLINE_CURVE((1.,1.,1.,1.,1.,1.,1.,1.,1.,1.,1.,1.,1.,1.,1.,1.,
1.,1.,1.,1.,1.,1.,1.,1.,1.,1.,1.,1.,1.,1.,1.,1.,1.,1.,1.,1.,1.,1.,1.,1.,
1.,1.,1.,1.,1.,1.,1.,1.,1.,1.,1.,1.,1.,1.,1.,1.,1.,1.,1.,1.,1.,1.,1.,1.,
1.,1.,1.,1.,1.,1.,1.,1.,1.,1.,1.,1.,1.,1.,1.,1.,1.,1.,1.,1.,1.,1.,1.,1.,
1.,1.,1.,1.,1.,1.,1.,1.,1.,1.,1.,1.,1.,1.,1.,1.,1.,1.,1.,1.,1.,1.,1.,1.,
1.,1.,1.,1.,1.,1.,1.,1.,1.,1.,1.,1.,1.,1.,1.,1.,1.,1.,1.,1.,1.,1.,1.,1.,
1.,1.,1.,1.,1.,1.,1.,1.,1.,1.,1.,1.,1.,1.,1.,1.,1.,1.,1.,1.,1.,1.,1.,1.,
1.,1.,1.,1.,1.,1.,1.,1.,1.,1.,1.,1.,1.,1.,1.,1.,1.,1.,1.,1.,1.,1.,1.,1.,
1.,1.,1.,1.,1.,1.,1.,1.,1.,1.))
REPRESENTATION_ITEM('')
);
#619=(
BOUNDED_CURVE()
B_SPLINE_CURVE(5,(#146240,#146241,#146242,#146243,#146244,#146245,#146246,
#146247,#146248,#146249,#146250,#146251,#146252,#146253,#146254,#146255,
#146256,#146257,#146258,#146259,#146260,#146261,#146262,#146263,#146264,
#146265,#146266,#146267,#146268,#146269,#146270,#146271,#146272,#146273,
#146274,#146275,#146276,#146277,#146278,#146279,#146280,#146281,#146282,
#146283,#146284,#146285,#146286,#146287,#146288,#146289,#146290,#146291,
#146292,#146293,#146294,#146295,#146296,#146297,#146298,#146299,#146300,
#146301,#146302,#146303,#146304,#146305,#146306,#146307,#146308,#146309,
#146310,#146311,#146312,#146313,#146314,#146315,#146316,#146317,#146318,
#146319,#146320,#146321,#146322,#146323,#146324,#146325,#146326,#146327,
#146328,#146329,#146330,#146331,#146332,#146333,#146334,#146335,#146336,
#146337,#146338,#146339,#146340,#146341,#146342,#146343,#146344,#146345,
#146346,#146347,#146348,#146349,#146350,#146351,#146352,#146353,#146354,
#146355,#146356,#146357,#146358,#146359,#146360,#146361,#146362,#146363,
#146364,#146365,#146366,#146367,#146368,#146369,#146370,#146371,#146372,
#146373,#146374,#146375,#146376,#146377,#146378,#146379,#146380,#146381,
#146382,#146383,#146384,#146385,#146386,#146387,#146388,#146389,#146390,
#146391,#146392,#146393,#146394,#146395,#146396,#146397,#146398,#146399,
#146400,#146401,#146402,#146403,#146404,#146405,#146406,#146407,#146408,
#146409,#146410,#146411,#146412,#146413,#146414,#146415,#146416,#146417,
#146418,#146419,#146420,#146421,#146422,#146423,#146424,#146425,#146426,
#146427,#146428,#146429,#146430,#146431,#146432,#146433),.UNSPECIFIED.,
 .F.,.F.)
B_SPLINE_CURVE_WITH_KNOTS((6,1,1,1,1,1,1,1,1,1,1,1,1,1,1,1,1,1,1,1,1,1,
1,1,1,1,1,1,1,1,1,1,1,1,1,1,1,1,1,1,1,1,1,1,1,1,1,1,1,1,1,1,1,1,1,1,1,1,
1,1,1,1,1,1,1,1,1,1,1,1,1,1,1,1,1,1,1,1,1,1,1,1,1,1,1,1,1,1,1,1,1,1,1,1,
1,1,1,1,1,1,1,1,1,1,1,1,1,1,1,1,1,1,1,1,1,1,1,1,1,1,1,1,1,1,1,1,1,1,1,1,
1,1,1,1,1,1,1,1,1,1,1,1,1,1,1,1,1,1,1,1,1,1,1,1,1,1,1,1,1,1,1,1,1,1,1,1,
1,1,1,1,1,1,1,1,1,1,1,1,1,1,1,1,1,1,1,1,1,1,1,6),(0.,0.005,0.01,0.015,0.02,
0.025,0.03,0.035,0.04,0.045,0.05,0.055,0.06,0.065,0.07,0.075,0.08,0.085,
0.09,0.095,0.1,0.105,0.11,0.115,0.12,0.125,0.13,0.135,0.14,0.145,0.15,0.155,
0.16,0.165,0.17,0.175,0.18,0.185,0.19,0.195,0.2,0.205,0.21,0.215,0.22,0.225,
0.23,0.235,0.24,0.245,0.25,0.255,0.26,0.265,0.27,0.275,0.28,0.285,0.29,
0.295,0.3,0.305,0.31,0.315,0.32,0.325,0.33,0.335,0.34,0.345,0.35,0.355,
0.36,0.365,0.37,0.375,0.38,0.385,0.39,0.395,0.4,0.405,0.41,0.415,0.42,0.425,
0.43,0.435,0.44,0.445,0.45,0.455,0.46,0.465,0.47,0.475,0.48,0.485,0.49,
0.495,0.5,0.505,0.51,0.515,0.52,0.525,0.53,0.535,0.54,0.545,0.55,0.555,
0.56,0.565,0.57,0.575,0.58,0.585,0.59,0.595,0.6,0.605,0.61,0.615,0.62,0.625,
0.63,0.635,0.64,0.645,0.65,0.655,0.66,0.665,0.67,0.675,0.68,0.685,0.690000000000001,
0.695000000000001,0.700000000000001,0.705000000000001,0.710000000000001,
0.715000000000001,0.720000000000001,0.725000000000001,0.730000000000001,
0.735000000000001,0.740000000000001,0.745000000000001,0.750000000000001,
0.755000000000001,0.760000000000001,0.765000000000001,0.770000000000001,
0.775000000000001,0.780000000000001,0.785000000000001,0.790000000000001,
0.795000000000001,0.800000000000001,0.805000000000001,0.810000000000001,
0.815000000000001,0.820000000000001,0.825000000000001,0.830000000000001,
0.835000000000001,0.840000000000001,0.845000000000001,0.850000000000001,
0.855000000000001,0.860000000000001,0.865000000000001,0.870000000000001,
0.875000000000001,0.880000000000001,0.885000000000001,0.890000000000001,
0.895000000000001,0.900000000000001,0.905000000000001,0.910000000000001,
0.915000000000001,0.920000000000001,0.925000000000001,0.930000000000001,
0.935000000000001,0.940000000000001,0.941429844437995),.UNSPECIFIED.)
CURVE()
GEOMETRIC_REPRESENTATION_ITEM()
RATIONAL_B_SPLINE_CURVE((1.,1.,1.,1.,1.,1.,1.,1.,1.,1.,1.,1.,1.,1.,1.,1.,
1.,1.,1.,1.,1.,1.,1.,1.,1.,1.,1.,1.,1.,1.,1.,1.,1.,1.,1.,1.,1.,1.,1.,1.,
1.,1.,1.,1.,1.,1.,1.,1.,1.,1.,1.,1.,1.,1.,1.,1.,1.,1.,1.,1.,1.,1.,1.,1.,
1.,1.,1.,1.,1.,1.,1.,1.,1.,1.,1.,1.,1.,1.,1.,1.,1.,1.,1.,1.,1.,1.,1.,1.,
1.,1.,1.,1.,1.,1.,1.,1.,1.,1.,1.,1.,1.,1.,1.,1.,1.,1.,1.,1.,1.,1.,1.,1.,
1.,1.,1.,1.,1.,1.,1.,1.,1.,1.,1.,1.,1.,1.,1.,1.,1.,1.,1.,1.,1.,1.,1.,1.,
1.,1.,1.,1.,1.,1.,1.,1.,1.,1.,1.,1.,1.,1.,1.,1.,1.,1.,1.,1.,1.,1.,1.,1.,
1.,1.,1.,1.,1.,1.,1.,1.,1.,1.,1.,1.,1.,1.,1.,1.,1.,1.,1.,1.,1.,1.,1.,1.,
1.,1.,1.,1.,1.,1.,1.,1.,1.,1.))
REPRESENTATION_ITEM('')
);
#620=(
BOUNDED_CURVE()
B_SPLINE_CURVE(5,(#146436,#146437,#146438,#146439,#146440,#146441,#146442,
#146443,#146444,#146445,#146446,#146447,#146448,#146449,#146450,#146451,
#146452,#146453,#146454,#146455,#146456,#146457,#146458,#146459,#146460,
#146461,#146462,#146463,#146464,#146465,#146466,#146467,#146468,#146469,
#146470,#146471,#146472,#146473,#146474,#146475,#146476,#146477,#146478,
#146479,#146480,#146481,#146482,#146483,#146484,#146485,#146486,#146487,
#146488,#146489,#146490,#146491,#146492,#146493,#146494,#146495,#146496,
#146497,#146498,#146499,#146500,#146501,#146502,#146503,#146504,#146505,
#146506,#146507,#146508,#146509,#146510,#146511,#146512,#146513,#146514,
#146515,#146516,#146517,#146518,#146519,#146520,#146521,#146522,#146523,
#146524,#146525,#146526,#146527,#146528,#146529,#146530,#146531,#146532,
#146533,#146534,#146535,#146536,#146537,#146538,#146539,#146540,#146541,
#146542,#146543,#146544,#146545,#146546,#146547,#146548,#146549,#146550,
#146551,#146552,#146553,#146554,#146555,#146556,#146557,#146558,#146559,
#146560,#146561,#146562,#146563,#146564,#146565,#146566,#146567,#146568,
#146569,#146570,#146571,#146572,#146573,#146574,#146575,#146576,#146577,
#146578,#146579,#146580,#146581,#146582,#146583,#146584,#146585,#146586,
#146587,#146588,#146589,#146590,#146591,#146592,#146593,#146594,#146595,
#146596,#146597,#146598,#146599,#146600,#146601,#146602,#146603,#146604,
#146605,#146606,#146607,#146608,#146609,#146610,#146611,#146612,#146613,
#146614,#146615,#146616,#146617,#146618,#146619,#146620,#146621,#146622,
#146623,#146624,#146625,#146626,#146627,#146628,#146629),.UNSPECIFIED.,
 .F.,.F.)
B_SPLINE_CURVE_WITH_KNOTS((6,1,1,1,1,1,1,1,1,1,1,1,1,1,1,1,1,1,1,1,1,1,
1,1,1,1,1,1,1,1,1,1,1,1,1,1,1,1,1,1,1,1,1,1,1,1,1,1,1,1,1,1,1,1,1,1,1,1,
1,1,1,1,1,1,1,1,1,1,1,1,1,1,1,1,1,1,1,1,1,1,1,1,1,1,1,1,1,1,1,1,1,1,1,1,
1,1,1,1,1,1,1,1,1,1,1,1,1,1,1,1,1,1,1,1,1,1,1,1,1,1,1,1,1,1,1,1,1,1,1,1,
1,1,1,1,1,1,1,1,1,1,1,1,1,1,1,1,1,1,1,1,1,1,1,1,1,1,1,1,1,1,1,1,1,1,1,1,
1,1,1,1,1,1,1,1,1,1,1,1,1,1,1,1,1,1,1,1,1,1,1,6),(-0.941429844438002,-0.940000000000001,
-0.935000000000001,-0.930000000000001,-0.925000000000001,-0.920000000000001,
-0.915000000000001,-0.910000000000001,-0.905000000000001,-0.900000000000001,
-0.895000000000001,-0.890000000000001,-0.885000000000001,-0.880000000000001,
-0.875000000000001,-0.870000000000001,-0.865000000000001,-0.860000000000001,
-0.855000000000001,-0.850000000000001,-0.845000000000001,-0.840000000000001,
-0.835000000000001,-0.830000000000001,-0.825000000000001,-0.820000000000001,
-0.815000000000001,-0.810000000000001,-0.805000000000001,-0.800000000000001,
-0.795000000000001,-0.790000000000001,-0.785000000000001,-0.780000000000001,
-0.775000000000001,-0.770000000000001,-0.765000000000001,-0.760000000000001,
-0.755000000000001,-0.750000000000001,-0.745000000000001,-0.740000000000001,
-0.735000000000001,-0.730000000000001,-0.725000000000001,-0.720000000000001,
-0.715000000000001,-0.710000000000001,-0.705000000000001,-0.700000000000001,
-0.695000000000001,-0.690000000000001,-0.685,-0.68,-0.675,-0.67,-0.665,
-0.66,-0.655,-0.65,-0.645,-0.64,-0.635,-0.63,-0.625,-0.62,-0.615,-0.61,
-0.605,-0.6,-0.595,-0.59,-0.585,-0.58,-0.575,-0.57,-0.565,-0.56,-0.555,
-0.55,-0.545,-0.54,-0.535,-0.53,-0.525,-0.52,-0.515,-0.51,-0.505,-0.5,-0.495,
-0.49,-0.485,-0.48,-0.475,-0.47,-0.465,-0.46,-0.455,-0.45,-0.445,-0.44,
-0.435,-0.43,-0.425,-0.42,-0.415,-0.41,-0.405,-0.4,-0.395,-0.39,-0.385,
-0.38,-0.375,-0.37,-0.365,-0.36,-0.355,-0.35,-0.345,-0.34,-0.335,-0.33,
-0.325,-0.32,-0.315,-0.31,-0.305,-0.3,-0.295,-0.29,-0.285,-0.28,-0.275,
-0.27,-0.265,-0.26,-0.255,-0.25,-0.245,-0.24,-0.235,-0.23,-0.225,-0.22,
-0.215,-0.21,-0.205,-0.2,-0.195,-0.19,-0.185,-0.18,-0.175,-0.17,-0.165,
-0.16,-0.155,-0.15,-0.145,-0.14,-0.135,-0.13,-0.125,-0.12,-0.115,-0.11,
-0.105,-0.1,-0.095,-0.09,-0.085,-0.08,-0.075,-0.07,-0.065,-0.06,-0.055,
-0.05,-0.045,-0.04,-0.035,-0.03,-0.025,-0.02,-0.015,-0.01,-0.005,0.),
 .UNSPECIFIED.)
CURVE()
GEOMETRIC_REPRESENTATION_ITEM()
RATIONAL_B_SPLINE_CURVE((1.,1.,1.,1.,1.,1.,1.,1.,1.,1.,1.,1.,1.,1.,1.,1.,
1.,1.,1.,1.,1.,1.,1.,1.,1.,1.,1.,1.,1.,1.,1.,1.,1.,1.,1.,1.,1.,1.,1.,1.,
1.,1.,1.,1.,1.,1.,1.,1.,1.,1.,1.,1.,1.,1.,1.,1.,1.,1.,1.,1.,1.,1.,1.,1.,
1.,1.,1.,1.,1.,1.,1.,1.,1.,1.,1.,1.,1.,1.,1.,1.,1.,1.,1.,1.,1.,1.,1.,1.,
1.,1.,1.,1.,1.,1.,1.,1.,1.,1.,1.,1.,1.,1.,1.,1.,1.,1.,1.,1.,1.,1.,1.,1.,
1.,1.,1.,1.,1.,1.,1.,1.,1.,1.,1.,1.,1.,1.,1.,1.,1.,1.,1.,1.,1.,1.,1.,1.,
1.,1.,1.,1.,1.,1.,1.,1.,1.,1.,1.,1.,1.,1.,1.,1.,1.,1.,1.,1.,1.,1.,1.,1.,
1.,1.,1.,1.,1.,1.,1.,1.,1.,1.,1.,1.,1.,1.,1.,1.,1.,1.,1.,1.,1.,1.,1.,1.,
1.,1.,1.,1.,1.,1.,1.,1.,1.,1.))
REPRESENTATION_ITEM('')
);
#621=(
BOUNDED_CURVE()
B_SPLINE_CURVE(5,(#147041,#147042,#147043,#147044,#147045,#147046,#147047,
#147048,#147049,#147050,#147051,#147052,#147053,#147054,#147055,#147056,
#147057,#147058,#147059,#147060,#147061,#147062,#147063,#147064,#147065,
#147066,#147067,#147068,#147069,#147070,#147071,#147072,#147073,#147074,
#147075,#147076,#147077,#147078,#147079,#147080,#147081,#147082,#147083,
#147084,#147085,#147086,#147087,#147088,#147089,#147090,#147091,#147092,
#147093,#147094,#147095,#147096,#147097,#147098,#147099,#147100,#147101,
#147102,#147103,#147104,#147105,#147106,#147107,#147108,#147109,#147110,
#147111,#147112,#147113,#147114,#147115,#147116,#147117,#147118,#147119,
#147120,#147121,#147122,#147123,#147124,#147125,#147126,#147127,#147128,
#147129,#147130,#147131,#147132,#147133,#147134,#147135,#147136,#147137,
#147138,#147139,#147140,#147141,#147142,#147143,#147144,#147145,#147146,
#147147,#147148,#147149,#147150,#147151,#147152,#147153,#147154,#147155,
#147156,#147157,#147158,#147159,#147160,#147161,#147162,#147163,#147164,
#147165,#147166,#147167,#147168,#147169,#147170,#147171,#147172,#147173,
#147174,#147175,#147176,#147177,#147178,#147179,#147180,#147181,#147182,
#147183,#147184,#147185,#147186,#147187,#147188,#147189,#147190,#147191,
#147192,#147193,#147194,#147195,#147196,#147197,#147198,#147199,#147200,
#147201,#147202,#147203,#147204,#147205,#147206,#147207,#147208,#147209,
#147210,#147211,#147212,#147213,#147214,#147215,#147216,#147217,#147218,
#147219,#147220,#147221,#147222,#147223,#147224,#147225,#147226,#147227,
#147228,#147229,#147230,#147231,#147232,#147233,#147234),.UNSPECIFIED.,
 .F.,.F.)
B_SPLINE_CURVE_WITH_KNOTS((6,1,1,1,1,1,1,1,1,1,1,1,1,1,1,1,1,1,1,1,1,1,
1,1,1,1,1,1,1,1,1,1,1,1,1,1,1,1,1,1,1,1,1,1,1,1,1,1,1,1,1,1,1,1,1,1,1,1,
1,1,1,1,1,1,1,1,1,1,1,1,1,1,1,1,1,1,1,1,1,1,1,1,1,1,1,1,1,1,1,1,1,1,1,1,
1,1,1,1,1,1,1,1,1,1,1,1,1,1,1,1,1,1,1,1,1,1,1,1,1,1,1,1,1,1,1,1,1,1,1,1,
1,1,1,1,1,1,1,1,1,1,1,1,1,1,1,1,1,1,1,1,1,1,1,1,1,1,1,1,1,1,1,1,1,1,1,1,
1,1,1,1,1,1,1,1,1,1,1,1,1,1,1,1,1,1,1,1,1,1,1,6),(0.,0.005,0.01,0.015,0.02,
0.025,0.03,0.035,0.04,0.045,0.05,0.055,0.06,0.065,0.07,0.075,0.08,0.085,
0.09,0.095,0.1,0.105,0.11,0.115,0.12,0.125,0.13,0.135,0.14,0.145,0.15,0.155,
0.16,0.165,0.17,0.175,0.18,0.185,0.19,0.195,0.2,0.205,0.21,0.215,0.22,0.225,
0.23,0.235,0.24,0.245,0.25,0.255,0.26,0.265,0.27,0.275,0.28,0.285,0.29,
0.295,0.3,0.305,0.31,0.315,0.32,0.325,0.33,0.335,0.34,0.345,0.35,0.355,
0.36,0.365,0.37,0.375,0.38,0.385,0.39,0.395,0.4,0.405,0.41,0.415,0.42,0.425,
0.43,0.435,0.44,0.445,0.45,0.455,0.46,0.465,0.47,0.475,0.48,0.485,0.49,
0.495,0.5,0.505,0.51,0.515,0.52,0.525,0.53,0.535,0.54,0.545,0.55,0.555,
0.56,0.565,0.57,0.575,0.58,0.585,0.59,0.595,0.6,0.605,0.61,0.615,0.62,0.625,
0.63,0.635,0.64,0.645,0.65,0.655,0.66,0.665,0.67,0.675,0.68,0.685,0.690000000000001,
0.695000000000001,0.700000000000001,0.705000000000001,0.710000000000001,
0.715000000000001,0.720000000000001,0.725000000000001,0.730000000000001,
0.735000000000001,0.740000000000001,0.745000000000001,0.750000000000001,
0.755000000000001,0.760000000000001,0.765000000000001,0.770000000000001,
0.775000000000001,0.780000000000001,0.785000000000001,0.790000000000001,
0.795000000000001,0.800000000000001,0.805000000000001,0.810000000000001,
0.815000000000001,0.820000000000001,0.825000000000001,0.830000000000001,
0.835000000000001,0.840000000000001,0.845000000000001,0.850000000000001,
0.855000000000001,0.860000000000001,0.865000000000001,0.870000000000001,
0.875000000000001,0.880000000000001,0.885000000000001,0.890000000000001,
0.895000000000001,0.900000000000001,0.905000000000001,0.910000000000001,
0.915000000000001,0.920000000000001,0.925000000000001,0.930000000000001,
0.935000000000001,0.940000000000001,0.941429844437957),.UNSPECIFIED.)
CURVE()
GEOMETRIC_REPRESENTATION_ITEM()
RATIONAL_B_SPLINE_CURVE((1.,1.,1.,1.,1.,1.,1.,1.,1.,1.,1.,1.,1.,1.,1.,1.,
1.,1.,1.,1.,1.,1.,1.,1.,1.,1.,1.,1.,1.,1.,1.,1.,1.,1.,1.,1.,1.,1.,1.,1.,
1.,1.,1.,1.,1.,1.,1.,1.,1.,1.,1.,1.,1.,1.,1.,1.,1.,1.,1.,1.,1.,1.,1.,1.,
1.,1.,1.,1.,1.,1.,1.,1.,1.,1.,1.,1.,1.,1.,1.,1.,1.,1.,1.,1.,1.,1.,1.,1.,
1.,1.,1.,1.,1.,1.,1.,1.,1.,1.,1.,1.,1.,1.,1.,1.,1.,1.,1.,1.,1.,1.,1.,1.,
1.,1.,1.,1.,1.,1.,1.,1.,1.,1.,1.,1.,1.,1.,1.,1.,1.,1.,1.,1.,1.,1.,1.,1.,
1.,1.,1.,1.,1.,1.,1.,1.,1.,1.,1.,1.,1.,1.,1.,1.,1.,1.,1.,1.,1.,1.,1.,1.,
1.,1.,1.,1.,1.,1.,1.,1.,1.,1.,1.,1.,1.,1.,1.,1.,1.,1.,1.,1.,1.,1.,1.,1.,
1.,1.,1.,1.,1.,1.,1.,1.,1.,1.))
REPRESENTATION_ITEM('')
);
#622=(
BOUNDED_CURVE()
B_SPLINE_CURVE(5,(#147237,#147238,#147239,#147240,#147241,#147242,#147243,
#147244,#147245,#147246,#147247,#147248,#147249,#147250,#147251,#147252,
#147253,#147254,#147255,#147256,#147257,#147258,#147259,#147260,#147261,
#147262,#147263,#147264,#147265,#147266,#147267,#147268,#147269,#147270,
#147271,#147272,#147273,#147274,#147275,#147276,#147277,#147278,#147279,
#147280,#147281,#147282,#147283,#147284,#147285,#147286,#147287,#147288,
#147289,#147290,#147291,#147292,#147293,#147294,#147295,#147296,#147297,
#147298,#147299,#147300,#147301,#147302,#147303,#147304,#147305,#147306,
#147307,#147308,#147309,#147310,#147311,#147312,#147313,#147314,#147315,
#147316,#147317,#147318,#147319,#147320,#147321,#147322,#147323,#147324,
#147325,#147326,#147327,#147328,#147329,#147330,#147331,#147332,#147333,
#147334,#147335,#147336,#147337,#147338,#147339,#147340,#147341,#147342,
#147343,#147344,#147345,#147346,#147347,#147348,#147349,#147350,#147351,
#147352,#147353,#147354,#147355,#147356,#147357,#147358,#147359,#147360,
#147361,#147362,#147363,#147364,#147365,#147366,#147367,#147368,#147369,
#147370,#147371,#147372,#147373,#147374,#147375,#147376,#147377,#147378,
#147379,#147380,#147381,#147382,#147383,#147384,#147385,#147386,#147387,
#147388,#147389,#147390,#147391,#147392,#147393,#147394,#147395,#147396,
#147397,#147398,#147399,#147400,#147401,#147402,#147403,#147404,#147405,
#147406,#147407,#147408,#147409,#147410,#147411,#147412,#147413,#147414,
#147415,#147416,#147417,#147418,#147419,#147420,#147421,#147422,#147423,
#147424,#147425,#147426,#147427,#147428,#147429,#147430),.UNSPECIFIED.,
 .F.,.F.)
B_SPLINE_CURVE_WITH_KNOTS((6,1,1,1,1,1,1,1,1,1,1,1,1,1,1,1,1,1,1,1,1,1,
1,1,1,1,1,1,1,1,1,1,1,1,1,1,1,1,1,1,1,1,1,1,1,1,1,1,1,1,1,1,1,1,1,1,1,1,
1,1,1,1,1,1,1,1,1,1,1,1,1,1,1,1,1,1,1,1,1,1,1,1,1,1,1,1,1,1,1,1,1,1,1,1,
1,1,1,1,1,1,1,1,1,1,1,1,1,1,1,1,1,1,1,1,1,1,1,1,1,1,1,1,1,1,1,1,1,1,1,1,
1,1,1,1,1,1,1,1,1,1,1,1,1,1,1,1,1,1,1,1,1,1,1,1,1,1,1,1,1,1,1,1,1,1,1,1,
1,1,1,1,1,1,1,1,1,1,1,1,1,1,1,1,1,1,1,1,1,1,1,6),(-0.94142984443796,-0.940000000000001,
-0.935000000000001,-0.930000000000001,-0.925000000000001,-0.920000000000001,
-0.915000000000001,-0.910000000000001,-0.905000000000001,-0.900000000000001,
-0.895000000000001,-0.890000000000001,-0.885000000000001,-0.880000000000001,
-0.875000000000001,-0.870000000000001,-0.865000000000001,-0.860000000000001,
-0.855000000000001,-0.850000000000001,-0.845000000000001,-0.840000000000001,
-0.835000000000001,-0.830000000000001,-0.825000000000001,-0.820000000000001,
-0.815000000000001,-0.810000000000001,-0.805000000000001,-0.800000000000001,
-0.795000000000001,-0.790000000000001,-0.785000000000001,-0.780000000000001,
-0.775000000000001,-0.770000000000001,-0.765000000000001,-0.760000000000001,
-0.755000000000001,-0.750000000000001,-0.745000000000001,-0.740000000000001,
-0.735000000000001,-0.730000000000001,-0.725000000000001,-0.720000000000001,
-0.715000000000001,-0.710000000000001,-0.705000000000001,-0.700000000000001,
-0.695000000000001,-0.690000000000001,-0.685,-0.68,-0.675,-0.67,-0.665,
-0.66,-0.655,-0.65,-0.645,-0.64,-0.635,-0.63,-0.625,-0.62,-0.615,-0.61,
-0.605,-0.6,-0.595,-0.59,-0.585,-0.58,-0.575,-0.57,-0.565,-0.56,-0.555,
-0.55,-0.545,-0.54,-0.535,-0.53,-0.525,-0.52,-0.515,-0.51,-0.505,-0.5,-0.495,
-0.49,-0.485,-0.48,-0.475,-0.47,-0.465,-0.46,-0.455,-0.45,-0.445,-0.44,
-0.435,-0.43,-0.425,-0.42,-0.415,-0.41,-0.405,-0.4,-0.395,-0.39,-0.385,
-0.38,-0.375,-0.37,-0.365,-0.36,-0.355,-0.35,-0.345,-0.34,-0.335,-0.33,
-0.325,-0.32,-0.315,-0.31,-0.305,-0.3,-0.295,-0.29,-0.285,-0.28,-0.275,
-0.27,-0.265,-0.26,-0.255,-0.25,-0.245,-0.24,-0.235,-0.23,-0.225,-0.22,
-0.215,-0.21,-0.205,-0.2,-0.195,-0.19,-0.185,-0.18,-0.175,-0.17,-0.165,
-0.16,-0.155,-0.15,-0.145,-0.14,-0.135,-0.13,-0.125,-0.12,-0.115,-0.11,
-0.105,-0.1,-0.095,-0.09,-0.085,-0.08,-0.075,-0.07,-0.065,-0.06,-0.055,
-0.05,-0.045,-0.04,-0.035,-0.03,-0.025,-0.02,-0.015,-0.01,-0.005,0.),
 .UNSPECIFIED.)
CURVE()
GEOMETRIC_REPRESENTATION_ITEM()
RATIONAL_B_SPLINE_CURVE((1.,1.,1.,1.,1.,1.,1.,1.,1.,1.,1.,1.,1.,1.,1.,1.,
1.,1.,1.,1.,1.,1.,1.,1.,1.,1.,1.,1.,1.,1.,1.,1.,1.,1.,1.,1.,1.,1.,1.,1.,
1.,1.,1.,1.,1.,1.,1.,1.,1.,1.,1.,1.,1.,1.,1.,1.,1.,1.,1.,1.,1.,1.,1.,1.,
1.,1.,1.,1.,1.,1.,1.,1.,1.,1.,1.,1.,1.,1.,1.,1.,1.,1.,1.,1.,1.,1.,1.,1.,
1.,1.,1.,1.,1.,1.,1.,1.,1.,1.,1.,1.,1.,1.,1.,1.,1.,1.,1.,1.,1.,1.,1.,1.,
1.,1.,1.,1.,1.,1.,1.,1.,1.,1.,1.,1.,1.,1.,1.,1.,1.,1.,1.,1.,1.,1.,1.,1.,
1.,1.,1.,1.,1.,1.,1.,1.,1.,1.,1.,1.,1.,1.,1.,1.,1.,1.,1.,1.,1.,1.,1.,1.,
1.,1.,1.,1.,1.,1.,1.,1.,1.,1.,1.,1.,1.,1.,1.,1.,1.,1.,1.,1.,1.,1.,1.,1.,
1.,1.,1.,1.,1.,1.,1.,1.,1.,1.))
REPRESENTATION_ITEM('')
);
#623=(
BOUNDED_CURVE()
B_SPLINE_CURVE(5,(#147842,#147843,#147844,#147845,#147846,#147847,#147848,
#147849,#147850,#147851,#147852,#147853,#147854,#147855,#147856,#147857,
#147858,#147859,#147860,#147861,#147862,#147863,#147864,#147865,#147866,
#147867,#147868,#147869,#147870,#147871,#147872,#147873,#147874,#147875,
#147876,#147877,#147878,#147879,#147880,#147881,#147882,#147883,#147884,
#147885,#147886,#147887,#147888,#147889,#147890,#147891,#147892,#147893,
#147894,#147895,#147896,#147897,#147898,#147899,#147900,#147901,#147902,
#147903,#147904,#147905,#147906,#147907,#147908,#147909,#147910,#147911,
#147912,#147913,#147914,#147915,#147916,#147917,#147918,#147919,#147920,
#147921,#147922,#147923,#147924,#147925,#147926,#147927,#147928,#147929,
#147930,#147931,#147932,#147933,#147934,#147935,#147936,#147937,#147938,
#147939,#147940,#147941,#147942,#147943,#147944,#147945,#147946,#147947,
#147948,#147949,#147950,#147951,#147952,#147953,#147954,#147955,#147956,
#147957,#147958,#147959,#147960,#147961,#147962,#147963,#147964,#147965,
#147966,#147967,#147968,#147969,#147970,#147971,#147972,#147973,#147974,
#147975,#147976,#147977,#147978,#147979,#147980,#147981,#147982,#147983,
#147984,#147985,#147986,#147987,#147988,#147989,#147990,#147991,#147992,
#147993,#147994,#147995,#147996,#147997,#147998,#147999,#148000,#148001,
#148002,#148003,#148004,#148005,#148006,#148007,#148008,#148009,#148010,
#148011,#148012,#148013,#148014,#148015,#148016,#148017,#148018,#148019,
#148020,#148021,#148022,#148023,#148024,#148025,#148026,#148027,#148028,
#148029,#148030,#148031,#148032,#148033,#148034,#148035),.UNSPECIFIED.,
 .F.,.F.)
B_SPLINE_CURVE_WITH_KNOTS((6,1,1,1,1,1,1,1,1,1,1,1,1,1,1,1,1,1,1,1,1,1,
1,1,1,1,1,1,1,1,1,1,1,1,1,1,1,1,1,1,1,1,1,1,1,1,1,1,1,1,1,1,1,1,1,1,1,1,
1,1,1,1,1,1,1,1,1,1,1,1,1,1,1,1,1,1,1,1,1,1,1,1,1,1,1,1,1,1,1,1,1,1,1,1,
1,1,1,1,1,1,1,1,1,1,1,1,1,1,1,1,1,1,1,1,1,1,1,1,1,1,1,1,1,1,1,1,1,1,1,1,
1,1,1,1,1,1,1,1,1,1,1,1,1,1,1,1,1,1,1,1,1,1,1,1,1,1,1,1,1,1,1,1,1,1,1,1,
1,1,1,1,1,1,1,1,1,1,1,1,1,1,1,1,1,1,1,1,1,1,1,6),(0.,0.005,0.01,0.015,0.02,
0.025,0.03,0.035,0.04,0.045,0.05,0.055,0.06,0.065,0.07,0.075,0.08,0.085,
0.09,0.095,0.1,0.105,0.11,0.115,0.12,0.125,0.13,0.135,0.14,0.145,0.15,0.155,
0.16,0.165,0.17,0.175,0.18,0.185,0.19,0.195,0.2,0.205,0.21,0.215,0.22,0.225,
0.23,0.235,0.24,0.245,0.25,0.255,0.26,0.265,0.27,0.275,0.28,0.285,0.29,
0.295,0.3,0.305,0.31,0.315,0.32,0.325,0.33,0.335,0.34,0.345,0.35,0.355,
0.36,0.365,0.37,0.375,0.38,0.385,0.39,0.395,0.4,0.405,0.41,0.415,0.42,0.425,
0.43,0.435,0.44,0.445,0.45,0.455,0.46,0.465,0.47,0.475,0.48,0.485,0.49,
0.495,0.5,0.505,0.51,0.515,0.52,0.525,0.53,0.535,0.54,0.545,0.55,0.555,
0.56,0.565,0.57,0.575,0.58,0.585,0.59,0.595,0.6,0.605,0.61,0.615,0.62,0.625,
0.63,0.635,0.64,0.645,0.65,0.655,0.66,0.665,0.67,0.675,0.68,0.685,0.690000000000001,
0.695000000000001,0.700000000000001,0.705000000000001,0.710000000000001,
0.715000000000001,0.720000000000001,0.725000000000001,0.730000000000001,
0.735000000000001,0.740000000000001,0.745000000000001,0.750000000000001,
0.755000000000001,0.760000000000001,0.765000000000001,0.770000000000001,
0.775000000000001,0.780000000000001,0.785000000000001,0.790000000000001,
0.795000000000001,0.800000000000001,0.805000000000001,0.810000000000001,
0.815000000000001,0.820000000000001,0.825000000000001,0.830000000000001,
0.835000000000001,0.840000000000001,0.845000000000001,0.850000000000001,
0.855000000000001,0.860000000000001,0.865000000000001,0.870000000000001,
0.875000000000001,0.880000000000001,0.885000000000001,0.890000000000001,
0.895000000000001,0.900000000000001,0.905000000000001,0.910000000000001,
0.915000000000001,0.920000000000001,0.925000000000001,0.930000000000001,
0.935000000000001,0.940000000000001,0.941429844437906),.UNSPECIFIED.)
CURVE()
GEOMETRIC_REPRESENTATION_ITEM()
RATIONAL_B_SPLINE_CURVE((1.,1.,1.,1.,1.,1.,1.,1.,1.,1.,1.,1.,1.,1.,1.,1.,
1.,1.,1.,1.,1.,1.,1.,1.,1.,1.,1.,1.,1.,1.,1.,1.,1.,1.,1.,1.,1.,1.,1.,1.,
1.,1.,1.,1.,1.,1.,1.,1.,1.,1.,1.,1.,1.,1.,1.,1.,1.,1.,1.,1.,1.,1.,1.,1.,
1.,1.,1.,1.,1.,1.,1.,1.,1.,1.,1.,1.,1.,1.,1.,1.,1.,1.,1.,1.,1.,1.,1.,1.,
1.,1.,1.,1.,1.,1.,1.,1.,1.,1.,1.,1.,1.,1.,1.,1.,1.,1.,1.,1.,1.,1.,1.,1.,
1.,1.,1.,1.,1.,1.,1.,1.,1.,1.,1.,1.,1.,1.,1.,1.,1.,1.,1.,1.,1.,1.,1.,1.,
1.,1.,1.,1.,1.,1.,1.,1.,1.,1.,1.,1.,1.,1.,1.,1.,1.,1.,1.,1.,1.,1.,1.,1.,
1.,1.,1.,1.,1.,1.,1.,1.,1.,1.,1.,1.,1.,1.,1.,1.,1.,1.,1.,1.,1.,1.,1.,1.,
1.,1.,1.,1.,1.,1.,1.,1.,1.,1.))
REPRESENTATION_ITEM('')
);
#624=(
BOUNDED_CURVE()
B_SPLINE_CURVE(5,(#148038,#148039,#148040,#148041,#148042,#148043,#148044,
#148045,#148046,#148047,#148048,#148049,#148050,#148051,#148052,#148053,
#148054,#148055,#148056,#148057,#148058,#148059,#148060,#148061,#148062,
#148063,#148064,#148065,#148066,#148067,#148068,#148069,#148070,#148071,
#148072,#148073,#148074,#148075,#148076,#148077,#148078,#148079,#148080,
#148081,#148082,#148083,#148084,#148085,#148086,#148087,#148088,#148089,
#148090,#148091,#148092,#148093,#148094,#148095,#148096,#148097,#148098,
#148099,#148100,#148101,#148102,#148103,#148104,#148105,#148106,#148107,
#148108,#148109,#148110,#148111,#148112,#148113,#148114,#148115,#148116,
#148117,#148118,#148119,#148120,#148121,#148122,#148123,#148124,#148125,
#148126,#148127,#148128,#148129,#148130,#148131,#148132,#148133,#148134,
#148135,#148136,#148137,#148138,#148139,#148140,#148141,#148142,#148143,
#148144,#148145,#148146,#148147,#148148,#148149,#148150,#148151,#148152,
#148153,#148154,#148155,#148156,#148157,#148158,#148159,#148160,#148161,
#148162,#148163,#148164,#148165,#148166,#148167,#148168,#148169,#148170,
#148171,#148172,#148173,#148174,#148175,#148176,#148177,#148178,#148179,
#148180,#148181,#148182,#148183,#148184,#148185,#148186,#148187,#148188,
#148189,#148190,#148191,#148192,#148193,#148194,#148195,#148196,#148197,
#148198,#148199,#148200,#148201,#148202,#148203,#148204,#148205,#148206,
#148207,#148208,#148209,#148210,#148211,#148212,#148213,#148214,#148215,
#148216,#148217,#148218,#148219,#148220,#148221,#148222,#148223,#148224,
#148225,#148226,#148227,#148228,#148229,#148230,#148231),.UNSPECIFIED.,
 .F.,.F.)
B_SPLINE_CURVE_WITH_KNOTS((6,1,1,1,1,1,1,1,1,1,1,1,1,1,1,1,1,1,1,1,1,1,
1,1,1,1,1,1,1,1,1,1,1,1,1,1,1,1,1,1,1,1,1,1,1,1,1,1,1,1,1,1,1,1,1,1,1,1,
1,1,1,1,1,1,1,1,1,1,1,1,1,1,1,1,1,1,1,1,1,1,1,1,1,1,1,1,1,1,1,1,1,1,1,1,
1,1,1,1,1,1,1,1,1,1,1,1,1,1,1,1,1,1,1,1,1,1,1,1,1,1,1,1,1,1,1,1,1,1,1,1,
1,1,1,1,1,1,1,1,1,1,1,1,1,1,1,1,1,1,1,1,1,1,1,1,1,1,1,1,1,1,1,1,1,1,1,1,
1,1,1,1,1,1,1,1,1,1,1,1,1,1,1,1,1,1,1,1,1,1,1,6),(-0.941429844437906,-0.940000000000001,
-0.935000000000001,-0.930000000000001,-0.925000000000001,-0.920000000000001,
-0.915000000000001,-0.910000000000001,-0.905000000000001,-0.900000000000001,
-0.895000000000001,-0.890000000000001,-0.885000000000001,-0.880000000000001,
-0.875000000000001,-0.870000000000001,-0.865000000000001,-0.860000000000001,
-0.855000000000001,-0.850000000000001,-0.845000000000001,-0.840000000000001,
-0.835000000000001,-0.830000000000001,-0.825000000000001,-0.820000000000001,
-0.815000000000001,-0.810000000000001,-0.805000000000001,-0.800000000000001,
-0.795000000000001,-0.790000000000001,-0.785000000000001,-0.780000000000001,
-0.775000000000001,-0.770000000000001,-0.765000000000001,-0.760000000000001,
-0.755000000000001,-0.750000000000001,-0.745000000000001,-0.740000000000001,
-0.735000000000001,-0.730000000000001,-0.725000000000001,-0.720000000000001,
-0.715000000000001,-0.710000000000001,-0.705000000000001,-0.700000000000001,
-0.695000000000001,-0.690000000000001,-0.685,-0.68,-0.675,-0.67,-0.665,
-0.66,-0.655,-0.65,-0.645,-0.64,-0.635,-0.63,-0.625,-0.62,-0.615,-0.61,
-0.605,-0.6,-0.595,-0.59,-0.585,-0.58,-0.575,-0.57,-0.565,-0.56,-0.555,
-0.55,-0.545,-0.54,-0.535,-0.53,-0.525,-0.52,-0.515,-0.51,-0.505,-0.5,-0.495,
-0.49,-0.485,-0.48,-0.475,-0.47,-0.465,-0.46,-0.455,-0.45,-0.445,-0.44,
-0.435,-0.43,-0.425,-0.42,-0.415,-0.41,-0.405,-0.4,-0.395,-0.39,-0.385,
-0.38,-0.375,-0.37,-0.365,-0.36,-0.355,-0.35,-0.345,-0.34,-0.335,-0.33,
-0.325,-0.32,-0.315,-0.31,-0.305,-0.3,-0.295,-0.29,-0.285,-0.28,-0.275,
-0.27,-0.265,-0.26,-0.255,-0.25,-0.245,-0.24,-0.235,-0.23,-0.225,-0.22,
-0.215,-0.21,-0.205,-0.2,-0.195,-0.19,-0.185,-0.18,-0.175,-0.17,-0.165,
-0.16,-0.155,-0.15,-0.145,-0.14,-0.135,-0.13,-0.125,-0.12,-0.115,-0.11,
-0.105,-0.1,-0.095,-0.09,-0.085,-0.08,-0.075,-0.07,-0.065,-0.06,-0.055,
-0.05,-0.045,-0.04,-0.035,-0.03,-0.025,-0.02,-0.015,-0.01,-0.005,0.),
 .UNSPECIFIED.)
CURVE()
GEOMETRIC_REPRESENTATION_ITEM()
RATIONAL_B_SPLINE_CURVE((1.,1.,1.,1.,1.,1.,1.,1.,1.,1.,1.,1.,1.,1.,1.,1.,
1.,1.,1.,1.,1.,1.,1.,1.,1.,1.,1.,1.,1.,1.,1.,1.,1.,1.,1.,1.,1.,1.,1.,1.,
1.,1.,1.,1.,1.,1.,1.,1.,1.,1.,1.,1.,1.,1.,1.,1.,1.,1.,1.,1.,1.,1.,1.,1.,
1.,1.,1.,1.,1.,1.,1.,1.,1.,1.,1.,1.,1.,1.,1.,1.,1.,1.,1.,1.,1.,1.,1.,1.,
1.,1.,1.,1.,1.,1.,1.,1.,1.,1.,1.,1.,1.,1.,1.,1.,1.,1.,1.,1.,1.,1.,1.,1.,
1.,1.,1.,1.,1.,1.,1.,1.,1.,1.,1.,1.,1.,1.,1.,1.,1.,1.,1.,1.,1.,1.,1.,1.,
1.,1.,1.,1.,1.,1.,1.,1.,1.,1.,1.,1.,1.,1.,1.,1.,1.,1.,1.,1.,1.,1.,1.,1.,
1.,1.,1.,1.,1.,1.,1.,1.,1.,1.,1.,1.,1.,1.,1.,1.,1.,1.,1.,1.,1.,1.,1.,1.,
1.,1.,1.,1.,1.,1.,1.,1.,1.,1.))
REPRESENTATION_ITEM('')
);
#625=(
BOUNDED_CURVE()
B_SPLINE_CURVE(5,(#148643,#148644,#148645,#148646,#148647,#148648,#148649,
#148650,#148651,#148652,#148653,#148654,#148655,#148656,#148657,#148658,
#148659,#148660,#148661,#148662,#148663,#148664,#148665,#148666,#148667,
#148668,#148669,#148670,#148671,#148672,#148673,#148674,#148675,#148676,
#148677,#148678,#148679,#148680,#148681,#148682,#148683,#148684,#148685,
#148686,#148687,#148688,#148689,#148690,#148691,#148692,#148693,#148694,
#148695,#148696,#148697,#148698,#148699,#148700,#148701,#148702,#148703,
#148704,#148705,#148706,#148707,#148708,#148709,#148710,#148711,#148712,
#148713,#148714,#148715,#148716,#148717,#148718,#148719,#148720,#148721,
#148722,#148723,#148724,#148725,#148726,#148727,#148728,#148729,#148730,
#148731,#148732,#148733,#148734,#148735,#148736,#148737,#148738,#148739,
#148740,#148741,#148742,#148743,#148744,#148745,#148746,#148747,#148748,
#148749,#148750,#148751,#148752,#148753,#148754,#148755,#148756,#148757,
#148758,#148759,#148760,#148761,#148762,#148763,#148764,#148765,#148766,
#148767,#148768,#148769,#148770,#148771,#148772,#148773,#148774,#148775,
#148776,#148777,#148778,#148779,#148780,#148781,#148782,#148783,#148784,
#148785,#148786,#148787,#148788,#148789,#148790,#148791,#148792,#148793,
#148794,#148795,#148796,#148797,#148798,#148799,#148800,#148801,#148802,
#148803,#148804,#148805,#148806,#148807,#148808,#148809,#148810,#148811,
#148812,#148813,#148814,#148815,#148816,#148817,#148818,#148819,#148820,
#148821,#148822,#148823,#148824,#148825,#148826,#148827,#148828,#148829,
#148830,#148831,#148832,#148833,#148834,#148835,#148836),.UNSPECIFIED.,
 .F.,.F.)
B_SPLINE_CURVE_WITH_KNOTS((6,1,1,1,1,1,1,1,1,1,1,1,1,1,1,1,1,1,1,1,1,1,
1,1,1,1,1,1,1,1,1,1,1,1,1,1,1,1,1,1,1,1,1,1,1,1,1,1,1,1,1,1,1,1,1,1,1,1,
1,1,1,1,1,1,1,1,1,1,1,1,1,1,1,1,1,1,1,1,1,1,1,1,1,1,1,1,1,1,1,1,1,1,1,1,
1,1,1,1,1,1,1,1,1,1,1,1,1,1,1,1,1,1,1,1,1,1,1,1,1,1,1,1,1,1,1,1,1,1,1,1,
1,1,1,1,1,1,1,1,1,1,1,1,1,1,1,1,1,1,1,1,1,1,1,1,1,1,1,1,1,1,1,1,1,1,1,1,
1,1,1,1,1,1,1,1,1,1,1,1,1,1,1,1,1,1,1,1,1,1,1,6),(0.,0.005,0.01,0.015,0.02,
0.025,0.03,0.035,0.04,0.045,0.05,0.055,0.06,0.065,0.07,0.075,0.08,0.085,
0.09,0.095,0.1,0.105,0.11,0.115,0.12,0.125,0.13,0.135,0.14,0.145,0.15,0.155,
0.16,0.165,0.17,0.175,0.18,0.185,0.19,0.195,0.2,0.205,0.21,0.215,0.22,0.225,
0.23,0.235,0.24,0.245,0.25,0.255,0.26,0.265,0.27,0.275,0.28,0.285,0.29,
0.295,0.3,0.305,0.31,0.315,0.32,0.325,0.33,0.335,0.34,0.345,0.35,0.355,
0.36,0.365,0.37,0.375,0.38,0.385,0.39,0.395,0.4,0.405,0.41,0.415,0.42,0.425,
0.43,0.435,0.44,0.445,0.45,0.455,0.46,0.465,0.47,0.475,0.48,0.485,0.49,
0.495,0.5,0.505,0.51,0.515,0.52,0.525,0.53,0.535,0.54,0.545,0.55,0.555,
0.56,0.565,0.57,0.575,0.58,0.585,0.59,0.595,0.6,0.605,0.61,0.615,0.62,0.625,
0.63,0.635,0.64,0.645,0.65,0.655,0.66,0.665,0.67,0.675,0.68,0.685,0.690000000000001,
0.695000000000001,0.700000000000001,0.705000000000001,0.710000000000001,
0.715000000000001,0.720000000000001,0.725000000000001,0.730000000000001,
0.735000000000001,0.740000000000001,0.745000000000001,0.750000000000001,
0.755000000000001,0.760000000000001,0.765000000000001,0.770000000000001,
0.775000000000001,0.780000000000001,0.785000000000001,0.790000000000001,
0.795000000000001,0.800000000000001,0.805000000000001,0.810000000000001,
0.815000000000001,0.820000000000001,0.825000000000001,0.830000000000001,
0.835000000000001,0.840000000000001,0.845000000000001,0.850000000000001,
0.855000000000001,0.860000000000001,0.865000000000001,0.870000000000001,
0.875000000000001,0.880000000000001,0.885000000000001,0.890000000000001,
0.895000000000001,0.900000000000001,0.905000000000001,0.910000000000001,
0.915000000000001,0.920000000000001,0.925000000000001,0.930000000000001,
0.935000000000001,0.940000000000001,0.941429844438009),.UNSPECIFIED.)
CURVE()
GEOMETRIC_REPRESENTATION_ITEM()
RATIONAL_B_SPLINE_CURVE((1.,1.,1.,1.,1.,1.,1.,1.,1.,1.,1.,1.,1.,1.,1.,1.,
1.,1.,1.,1.,1.,1.,1.,1.,1.,1.,1.,1.,1.,1.,1.,1.,1.,1.,1.,1.,1.,1.,1.,1.,
1.,1.,1.,1.,1.,1.,1.,1.,1.,1.,1.,1.,1.,1.,1.,1.,1.,1.,1.,1.,1.,1.,1.,1.,
1.,1.,1.,1.,1.,1.,1.,1.,1.,1.,1.,1.,1.,1.,1.,1.,1.,1.,1.,1.,1.,1.,1.,1.,
1.,1.,1.,1.,1.,1.,1.,1.,1.,1.,1.,1.,1.,1.,1.,1.,1.,1.,1.,1.,1.,1.,1.,1.,
1.,1.,1.,1.,1.,1.,1.,1.,1.,1.,1.,1.,1.,1.,1.,1.,1.,1.,1.,1.,1.,1.,1.,1.,
1.,1.,1.,1.,1.,1.,1.,1.,1.,1.,1.,1.,1.,1.,1.,1.,1.,1.,1.,1.,1.,1.,1.,1.,
1.,1.,1.,1.,1.,1.,1.,1.,1.,1.,1.,1.,1.,1.,1.,1.,1.,1.,1.,1.,1.,1.,1.,1.,
1.,1.,1.,1.,1.,1.,1.,1.,1.,1.))
REPRESENTATION_ITEM('')
);
#626=(
BOUNDED_CURVE()
B_SPLINE_CURVE(5,(#148839,#148840,#148841,#148842,#148843,#148844,#148845,
#148846,#148847,#148848,#148849,#148850,#148851,#148852,#148853,#148854,
#148855,#148856,#148857,#148858,#148859,#148860,#148861,#148862,#148863,
#148864,#148865,#148866,#148867,#148868,#148869,#148870,#148871,#148872,
#148873,#148874,#148875,#148876,#148877,#148878,#148879,#148880,#148881,
#148882,#148883,#148884,#148885,#148886,#148887,#148888,#148889,#148890,
#148891,#148892,#148893,#148894,#148895,#148896,#148897,#148898,#148899,
#148900,#148901,#148902,#148903,#148904,#148905,#148906,#148907,#148908,
#148909,#148910,#148911,#148912,#148913,#148914,#148915,#148916,#148917,
#148918,#148919,#148920,#148921,#148922,#148923,#148924,#148925,#148926,
#148927,#148928,#148929,#148930,#148931,#148932,#148933,#148934,#148935,
#148936,#148937,#148938,#148939,#148940,#148941,#148942,#148943,#148944,
#148945,#148946,#148947,#148948,#148949,#148950,#148951,#148952,#148953,
#148954,#148955,#148956,#148957,#148958,#148959,#148960,#148961,#148962,
#148963,#148964,#148965,#148966,#148967,#148968,#148969,#148970,#148971,
#148972,#148973,#148974,#148975,#148976,#148977,#148978,#148979,#148980,
#148981,#148982,#148983,#148984,#148985,#148986,#148987,#148988,#148989,
#148990,#148991,#148992,#148993,#148994,#148995,#148996,#148997,#148998,
#148999,#149000,#149001,#149002,#149003,#149004,#149005,#149006,#149007,
#149008,#149009,#149010,#149011,#149012,#149013,#149014,#149015,#149016,
#149017,#149018,#149019,#149020,#149021,#149022,#149023,#149024,#149025,
#149026,#149027,#149028,#149029,#149030,#149031,#149032),.UNSPECIFIED.,
 .F.,.F.)
B_SPLINE_CURVE_WITH_KNOTS((6,1,1,1,1,1,1,1,1,1,1,1,1,1,1,1,1,1,1,1,1,1,
1,1,1,1,1,1,1,1,1,1,1,1,1,1,1,1,1,1,1,1,1,1,1,1,1,1,1,1,1,1,1,1,1,1,1,1,
1,1,1,1,1,1,1,1,1,1,1,1,1,1,1,1,1,1,1,1,1,1,1,1,1,1,1,1,1,1,1,1,1,1,1,1,
1,1,1,1,1,1,1,1,1,1,1,1,1,1,1,1,1,1,1,1,1,1,1,1,1,1,1,1,1,1,1,1,1,1,1,1,
1,1,1,1,1,1,1,1,1,1,1,1,1,1,1,1,1,1,1,1,1,1,1,1,1,1,1,1,1,1,1,1,1,1,1,1,
1,1,1,1,1,1,1,1,1,1,1,1,1,1,1,1,1,1,1,1,1,1,1,6),(-0.941429844438009,-0.940000000000001,
-0.935000000000001,-0.930000000000001,-0.925000000000001,-0.920000000000001,
-0.915000000000001,-0.910000000000001,-0.905000000000001,-0.900000000000001,
-0.895000000000001,-0.890000000000001,-0.885000000000001,-0.880000000000001,
-0.875000000000001,-0.870000000000001,-0.865000000000001,-0.860000000000001,
-0.855000000000001,-0.850000000000001,-0.845000000000001,-0.840000000000001,
-0.835000000000001,-0.830000000000001,-0.825000000000001,-0.820000000000001,
-0.815000000000001,-0.810000000000001,-0.805000000000001,-0.800000000000001,
-0.795000000000001,-0.790000000000001,-0.785000000000001,-0.780000000000001,
-0.775000000000001,-0.770000000000001,-0.765000000000001,-0.760000000000001,
-0.755000000000001,-0.750000000000001,-0.745000000000001,-0.740000000000001,
-0.735000000000001,-0.730000000000001,-0.725000000000001,-0.720000000000001,
-0.715000000000001,-0.710000000000001,-0.705000000000001,-0.700000000000001,
-0.695000000000001,-0.690000000000001,-0.685,-0.68,-0.675,-0.67,-0.665,
-0.66,-0.655,-0.65,-0.645,-0.64,-0.635,-0.63,-0.625,-0.62,-0.615,-0.61,
-0.605,-0.6,-0.595,-0.59,-0.585,-0.58,-0.575,-0.57,-0.565,-0.56,-0.555,
-0.55,-0.545,-0.54,-0.535,-0.53,-0.525,-0.52,-0.515,-0.51,-0.505,-0.5,-0.495,
-0.49,-0.485,-0.48,-0.475,-0.47,-0.465,-0.46,-0.455,-0.45,-0.445,-0.44,
-0.435,-0.43,-0.425,-0.42,-0.415,-0.41,-0.405,-0.4,-0.395,-0.39,-0.385,
-0.38,-0.375,-0.37,-0.365,-0.36,-0.355,-0.35,-0.345,-0.34,-0.335,-0.33,
-0.325,-0.32,-0.315,-0.31,-0.305,-0.3,-0.295,-0.29,-0.285,-0.28,-0.275,
-0.27,-0.265,-0.26,-0.255,-0.25,-0.245,-0.24,-0.235,-0.23,-0.225,-0.22,
-0.215,-0.21,-0.205,-0.2,-0.195,-0.19,-0.185,-0.18,-0.175,-0.17,-0.165,
-0.16,-0.155,-0.15,-0.145,-0.14,-0.135,-0.13,-0.125,-0.12,-0.115,-0.11,
-0.105,-0.1,-0.095,-0.09,-0.085,-0.08,-0.075,-0.07,-0.065,-0.06,-0.055,
-0.05,-0.045,-0.04,-0.035,-0.03,-0.025,-0.02,-0.015,-0.01,-0.005,0.),
 .UNSPECIFIED.)
CURVE()
GEOMETRIC_REPRESENTATION_ITEM()
RATIONAL_B_SPLINE_CURVE((1.,1.,1.,1.,1.,1.,1.,1.,1.,1.,1.,1.,1.,1.,1.,1.,
1.,1.,1.,1.,1.,1.,1.,1.,1.,1.,1.,1.,1.,1.,1.,1.,1.,1.,1.,1.,1.,1.,1.,1.,
1.,1.,1.,1.,1.,1.,1.,1.,1.,1.,1.,1.,1.,1.,1.,1.,1.,1.,1.,1.,1.,1.,1.,1.,
1.,1.,1.,1.,1.,1.,1.,1.,1.,1.,1.,1.,1.,1.,1.,1.,1.,1.,1.,1.,1.,1.,1.,1.,
1.,1.,1.,1.,1.,1.,1.,1.,1.,1.,1.,1.,1.,1.,1.,1.,1.,1.,1.,1.,1.,1.,1.,1.,
1.,1.,1.,1.,1.,1.,1.,1.,1.,1.,1.,1.,1.,1.,1.,1.,1.,1.,1.,1.,1.,1.,1.,1.,
1.,1.,1.,1.,1.,1.,1.,1.,1.,1.,1.,1.,1.,1.,1.,1.,1.,1.,1.,1.,1.,1.,1.,1.,
1.,1.,1.,1.,1.,1.,1.,1.,1.,1.,1.,1.,1.,1.,1.,1.,1.,1.,1.,1.,1.,1.,1.,1.,
1.,1.,1.,1.,1.,1.,1.,1.,1.,1.))
REPRESENTATION_ITEM('')
);
#627=(
BOUNDED_CURVE()
B_SPLINE_CURVE(5,(#149444,#149445,#149446,#149447,#149448,#149449,#149450,
#149451,#149452,#149453,#149454,#149455,#149456,#149457,#149458,#149459,
#149460,#149461,#149462,#149463,#149464,#149465,#149466,#149467,#149468,
#149469,#149470,#149471,#149472,#149473,#149474,#149475,#149476,#149477,
#149478,#149479,#149480,#149481,#149482,#149483,#149484,#149485,#149486,
#149487,#149488,#149489,#149490,#149491,#149492,#149493,#149494,#149495,
#149496,#149497,#149498,#149499,#149500,#149501,#149502,#149503,#149504,
#149505,#149506,#149507,#149508,#149509,#149510,#149511,#149512,#149513,
#149514,#149515,#149516,#149517,#149518,#149519,#149520,#149521,#149522,
#149523,#149524,#149525,#149526,#149527,#149528,#149529,#149530,#149531,
#149532,#149533,#149534,#149535,#149536,#149537,#149538,#149539,#149540,
#149541,#149542,#149543,#149544,#149545,#149546,#149547,#149548,#149549,
#149550,#149551,#149552,#149553,#149554,#149555,#149556,#149557,#149558,
#149559,#149560,#149561,#149562,#149563,#149564,#149565,#149566,#149567,
#149568,#149569,#149570,#149571,#149572,#149573,#149574,#149575,#149576,
#149577,#149578,#149579,#149580,#149581,#149582,#149583,#149584,#149585,
#149586,#149587,#149588,#149589,#149590,#149591,#149592,#149593,#149594,
#149595,#149596,#149597,#149598,#149599,#149600,#149601,#149602,#149603,
#149604,#149605,#149606,#149607,#149608,#149609,#149610,#149611,#149612,
#149613,#149614,#149615,#149616,#149617,#149618,#149619,#149620,#149621,
#149622,#149623,#149624,#149625,#149626,#149627,#149628,#149629,#149630,
#149631,#149632,#149633,#149634,#149635,#149636,#149637),.UNSPECIFIED.,
 .F.,.F.)
B_SPLINE_CURVE_WITH_KNOTS((6,1,1,1,1,1,1,1,1,1,1,1,1,1,1,1,1,1,1,1,1,1,
1,1,1,1,1,1,1,1,1,1,1,1,1,1,1,1,1,1,1,1,1,1,1,1,1,1,1,1,1,1,1,1,1,1,1,1,
1,1,1,1,1,1,1,1,1,1,1,1,1,1,1,1,1,1,1,1,1,1,1,1,1,1,1,1,1,1,1,1,1,1,1,1,
1,1,1,1,1,1,1,1,1,1,1,1,1,1,1,1,1,1,1,1,1,1,1,1,1,1,1,1,1,1,1,1,1,1,1,1,
1,1,1,1,1,1,1,1,1,1,1,1,1,1,1,1,1,1,1,1,1,1,1,1,1,1,1,1,1,1,1,1,1,1,1,1,
1,1,1,1,1,1,1,1,1,1,1,1,1,1,1,1,1,1,1,1,1,1,1,6),(0.,0.005,0.01,0.015,0.02,
0.025,0.03,0.035,0.04,0.045,0.05,0.055,0.06,0.065,0.07,0.075,0.08,0.085,
0.09,0.095,0.1,0.105,0.11,0.115,0.12,0.125,0.13,0.135,0.14,0.145,0.15,0.155,
0.16,0.165,0.17,0.175,0.18,0.185,0.19,0.195,0.2,0.205,0.21,0.215,0.22,0.225,
0.23,0.235,0.24,0.245,0.25,0.255,0.26,0.265,0.27,0.275,0.28,0.285,0.29,
0.295,0.3,0.305,0.31,0.315,0.32,0.325,0.33,0.335,0.34,0.345,0.35,0.355,
0.36,0.365,0.37,0.375,0.38,0.385,0.39,0.395,0.4,0.405,0.41,0.415,0.42,0.425,
0.43,0.435,0.44,0.445,0.45,0.455,0.46,0.465,0.47,0.475,0.48,0.485,0.49,
0.495,0.5,0.505,0.51,0.515,0.52,0.525,0.53,0.535,0.54,0.545,0.55,0.555,
0.56,0.565,0.57,0.575,0.58,0.585,0.59,0.595,0.6,0.605,0.61,0.615,0.62,0.625,
0.63,0.635,0.64,0.645,0.65,0.655,0.66,0.665,0.67,0.675,0.68,0.685,0.690000000000001,
0.695000000000001,0.700000000000001,0.705000000000001,0.710000000000001,
0.715000000000001,0.720000000000001,0.725000000000001,0.730000000000001,
0.735000000000001,0.740000000000001,0.745000000000001,0.750000000000001,
0.755000000000001,0.760000000000001,0.765000000000001,0.770000000000001,
0.775000000000001,0.780000000000001,0.785000000000001,0.790000000000001,
0.795000000000001,0.800000000000001,0.805000000000001,0.810000000000001,
0.815000000000001,0.820000000000001,0.825000000000001,0.830000000000001,
0.835000000000001,0.840000000000001,0.845000000000001,0.850000000000001,
0.855000000000001,0.860000000000001,0.865000000000001,0.870000000000001,
0.875000000000001,0.880000000000001,0.885000000000001,0.890000000000001,
0.895000000000001,0.900000000000001,0.905000000000001,0.910000000000001,
0.915000000000001,0.920000000000001,0.925000000000001,0.930000000000001,
0.935000000000001,0.940000000000001,0.941429844438207),.UNSPECIFIED.)
CURVE()
GEOMETRIC_REPRESENTATION_ITEM()
RATIONAL_B_SPLINE_CURVE((1.,1.,1.,1.,1.,1.,1.,1.,1.,1.,1.,1.,1.,1.,1.,1.,
1.,1.,1.,1.,1.,1.,1.,1.,1.,1.,1.,1.,1.,1.,1.,1.,1.,1.,1.,1.,1.,1.,1.,1.,
1.,1.,1.,1.,1.,1.,1.,1.,1.,1.,1.,1.,1.,1.,1.,1.,1.,1.,1.,1.,1.,1.,1.,1.,
1.,1.,1.,1.,1.,1.,1.,1.,1.,1.,1.,1.,1.,1.,1.,1.,1.,1.,1.,1.,1.,1.,1.,1.,
1.,1.,1.,1.,1.,1.,1.,1.,1.,1.,1.,1.,1.,1.,1.,1.,1.,1.,1.,1.,1.,1.,1.,1.,
1.,1.,1.,1.,1.,1.,1.,1.,1.,1.,1.,1.,1.,1.,1.,1.,1.,1.,1.,1.,1.,1.,1.,1.,
1.,1.,1.,1.,1.,1.,1.,1.,1.,1.,1.,1.,1.,1.,1.,1.,1.,1.,1.,1.,1.,1.,1.,1.,
1.,1.,1.,1.,1.,1.,1.,1.,1.,1.,1.,1.,1.,1.,1.,1.,1.,1.,1.,1.,1.,1.,1.,1.,
1.,1.,1.,1.,1.,1.,1.,1.,1.,1.))
REPRESENTATION_ITEM('')
);
#628=(
BOUNDED_CURVE()
B_SPLINE_CURVE(5,(#149640,#149641,#149642,#149643,#149644,#149645,#149646,
#149647,#149648,#149649,#149650,#149651,#149652,#149653,#149654,#149655,
#149656,#149657,#149658,#149659,#149660,#149661,#149662,#149663,#149664,
#149665,#149666,#149667,#149668,#149669,#149670,#149671,#149672,#149673,
#149674,#149675,#149676,#149677,#149678,#149679,#149680,#149681,#149682,
#149683,#149684,#149685,#149686,#149687,#149688,#149689,#149690,#149691,
#149692,#149693,#149694,#149695,#149696,#149697,#149698,#149699,#149700,
#149701,#149702,#149703,#149704,#149705,#149706,#149707,#149708,#149709,
#149710,#149711,#149712,#149713,#149714,#149715,#149716,#149717,#149718,
#149719,#149720,#149721,#149722,#149723,#149724,#149725,#149726,#149727,
#149728,#149729,#149730,#149731,#149732,#149733,#149734,#149735,#149736,
#149737,#149738,#149739,#149740,#149741,#149742,#149743,#149744,#149745,
#149746,#149747,#149748,#149749,#149750,#149751,#149752,#149753,#149754,
#149755,#149756,#149757,#149758,#149759,#149760,#149761,#149762,#149763,
#149764,#149765,#149766,#149767,#149768,#149769,#149770,#149771,#149772,
#149773,#149774,#149775,#149776,#149777,#149778,#149779,#149780,#149781,
#149782,#149783,#149784,#149785,#149786,#149787,#149788,#149789,#149790,
#149791,#149792,#149793,#149794,#149795,#149796,#149797,#149798,#149799,
#149800,#149801,#149802,#149803,#149804,#149805,#149806,#149807,#149808,
#149809,#149810,#149811,#149812,#149813,#149814,#149815,#149816,#149817,
#149818,#149819,#149820,#149821,#149822,#149823,#149824,#149825,#149826,
#149827,#149828,#149829,#149830,#149831,#149832,#149833),.UNSPECIFIED.,
 .F.,.F.)
B_SPLINE_CURVE_WITH_KNOTS((6,1,1,1,1,1,1,1,1,1,1,1,1,1,1,1,1,1,1,1,1,1,
1,1,1,1,1,1,1,1,1,1,1,1,1,1,1,1,1,1,1,1,1,1,1,1,1,1,1,1,1,1,1,1,1,1,1,1,
1,1,1,1,1,1,1,1,1,1,1,1,1,1,1,1,1,1,1,1,1,1,1,1,1,1,1,1,1,1,1,1,1,1,1,1,
1,1,1,1,1,1,1,1,1,1,1,1,1,1,1,1,1,1,1,1,1,1,1,1,1,1,1,1,1,1,1,1,1,1,1,1,
1,1,1,1,1,1,1,1,1,1,1,1,1,1,1,1,1,1,1,1,1,1,1,1,1,1,1,1,1,1,1,1,1,1,1,1,
1,1,1,1,1,1,1,1,1,1,1,1,1,1,1,1,1,1,1,1,1,1,1,6),(-0.941429844438208,-0.940000000000001,
-0.935000000000001,-0.930000000000001,-0.925000000000001,-0.920000000000001,
-0.915000000000001,-0.910000000000001,-0.905000000000001,-0.900000000000001,
-0.895000000000001,-0.890000000000001,-0.885000000000001,-0.880000000000001,
-0.875000000000001,-0.870000000000001,-0.865000000000001,-0.860000000000001,
-0.855000000000001,-0.850000000000001,-0.845000000000001,-0.840000000000001,
-0.835000000000001,-0.830000000000001,-0.825000000000001,-0.820000000000001,
-0.815000000000001,-0.810000000000001,-0.805000000000001,-0.800000000000001,
-0.795000000000001,-0.790000000000001,-0.785000000000001,-0.780000000000001,
-0.775000000000001,-0.770000000000001,-0.765000000000001,-0.760000000000001,
-0.755000000000001,-0.750000000000001,-0.745000000000001,-0.740000000000001,
-0.735000000000001,-0.730000000000001,-0.725000000000001,-0.720000000000001,
-0.715000000000001,-0.710000000000001,-0.705000000000001,-0.700000000000001,
-0.695000000000001,-0.690000000000001,-0.685,-0.68,-0.675,-0.67,-0.665,
-0.66,-0.655,-0.65,-0.645,-0.64,-0.635,-0.63,-0.625,-0.62,-0.615,-0.61,
-0.605,-0.6,-0.595,-0.59,-0.585,-0.58,-0.575,-0.57,-0.565,-0.56,-0.555,
-0.55,-0.545,-0.54,-0.535,-0.53,-0.525,-0.52,-0.515,-0.51,-0.505,-0.5,-0.495,
-0.49,-0.485,-0.48,-0.475,-0.47,-0.465,-0.46,-0.455,-0.45,-0.445,-0.44,
-0.435,-0.43,-0.425,-0.42,-0.415,-0.41,-0.405,-0.4,-0.395,-0.39,-0.385,
-0.38,-0.375,-0.37,-0.365,-0.36,-0.355,-0.35,-0.345,-0.34,-0.335,-0.33,
-0.325,-0.32,-0.315,-0.31,-0.305,-0.3,-0.295,-0.29,-0.285,-0.28,-0.275,
-0.27,-0.265,-0.26,-0.255,-0.25,-0.245,-0.24,-0.235,-0.23,-0.225,-0.22,
-0.215,-0.21,-0.205,-0.2,-0.195,-0.19,-0.185,-0.18,-0.175,-0.17,-0.165,
-0.16,-0.155,-0.15,-0.145,-0.14,-0.135,-0.13,-0.125,-0.12,-0.115,-0.11,
-0.105,-0.1,-0.095,-0.09,-0.085,-0.08,-0.075,-0.07,-0.065,-0.06,-0.055,
-0.05,-0.045,-0.04,-0.035,-0.03,-0.025,-0.02,-0.015,-0.01,-0.005,0.),
 .UNSPECIFIED.)
CURVE()
GEOMETRIC_REPRESENTATION_ITEM()
RATIONAL_B_SPLINE_CURVE((1.,1.,1.,1.,1.,1.,1.,1.,1.,1.,1.,1.,1.,1.,1.,1.,
1.,1.,1.,1.,1.,1.,1.,1.,1.,1.,1.,1.,1.,1.,1.,1.,1.,1.,1.,1.,1.,1.,1.,1.,
1.,1.,1.,1.,1.,1.,1.,1.,1.,1.,1.,1.,1.,1.,1.,1.,1.,1.,1.,1.,1.,1.,1.,1.,
1.,1.,1.,1.,1.,1.,1.,1.,1.,1.,1.,1.,1.,1.,1.,1.,1.,1.,1.,1.,1.,1.,1.,1.,
1.,1.,1.,1.,1.,1.,1.,1.,1.,1.,1.,1.,1.,1.,1.,1.,1.,1.,1.,1.,1.,1.,1.,1.,
1.,1.,1.,1.,1.,1.,1.,1.,1.,1.,1.,1.,1.,1.,1.,1.,1.,1.,1.,1.,1.,1.,1.,1.,
1.,1.,1.,1.,1.,1.,1.,1.,1.,1.,1.,1.,1.,1.,1.,1.,1.,1.,1.,1.,1.,1.,1.,1.,
1.,1.,1.,1.,1.,1.,1.,1.,1.,1.,1.,1.,1.,1.,1.,1.,1.,1.,1.,1.,1.,1.,1.,1.,
1.,1.,1.,1.,1.,1.,1.,1.,1.,1.))
REPRESENTATION_ITEM('')
);
#629=(
BOUNDED_CURVE()
B_SPLINE_CURVE(5,(#150245,#150246,#150247,#150248,#150249,#150250,#150251,
#150252,#150253,#150254,#150255,#150256,#150257,#150258,#150259,#150260,
#150261,#150262,#150263,#150264,#150265,#150266,#150267,#150268,#150269,
#150270,#150271,#150272,#150273,#150274,#150275,#150276,#150277,#150278,
#150279,#150280,#150281,#150282,#150283,#150284,#150285,#150286,#150287,
#150288,#150289,#150290,#150291,#150292,#150293,#150294,#150295,#150296,
#150297,#150298,#150299,#150300,#150301,#150302,#150303,#150304,#150305,
#150306,#150307,#150308,#150309,#150310,#150311,#150312,#150313,#150314,
#150315,#150316,#150317,#150318,#150319,#150320,#150321,#150322,#150323,
#150324,#150325,#150326,#150327,#150328,#150329,#150330,#150331,#150332,
#150333,#150334,#150335,#150336,#150337,#150338,#150339,#150340,#150341,
#150342,#150343,#150344,#150345,#150346,#150347,#150348,#150349,#150350,
#150351,#150352,#150353,#150354,#150355,#150356,#150357,#150358,#150359,
#150360,#150361,#150362,#150363,#150364,#150365,#150366,#150367,#150368,
#150369,#150370,#150371,#150372,#150373,#150374,#150375,#150376,#150377,
#150378,#150379,#150380,#150381,#150382,#150383,#150384,#150385,#150386,
#150387,#150388,#150389,#150390,#150391,#150392,#150393,#150394,#150395,
#150396,#150397,#150398,#150399,#150400,#150401,#150402,#150403,#150404,
#150405,#150406,#150407,#150408,#150409,#150410,#150411,#150412,#150413,
#150414,#150415,#150416,#150417,#150418,#150419,#150420,#150421,#150422,
#150423,#150424,#150425,#150426,#150427,#150428,#150429,#150430,#150431,
#150432,#150433,#150434,#150435,#150436,#150437,#150438),.UNSPECIFIED.,
 .F.,.F.)
B_SPLINE_CURVE_WITH_KNOTS((6,1,1,1,1,1,1,1,1,1,1,1,1,1,1,1,1,1,1,1,1,1,
1,1,1,1,1,1,1,1,1,1,1,1,1,1,1,1,1,1,1,1,1,1,1,1,1,1,1,1,1,1,1,1,1,1,1,1,
1,1,1,1,1,1,1,1,1,1,1,1,1,1,1,1,1,1,1,1,1,1,1,1,1,1,1,1,1,1,1,1,1,1,1,1,
1,1,1,1,1,1,1,1,1,1,1,1,1,1,1,1,1,1,1,1,1,1,1,1,1,1,1,1,1,1,1,1,1,1,1,1,
1,1,1,1,1,1,1,1,1,1,1,1,1,1,1,1,1,1,1,1,1,1,1,1,1,1,1,1,1,1,1,1,1,1,1,1,
1,1,1,1,1,1,1,1,1,1,1,1,1,1,1,1,1,1,1,1,1,1,1,6),(0.,0.005,0.01,0.015,0.02,
0.025,0.03,0.035,0.04,0.045,0.05,0.055,0.06,0.065,0.07,0.075,0.08,0.085,
0.09,0.095,0.1,0.105,0.11,0.115,0.12,0.125,0.13,0.135,0.14,0.145,0.15,0.155,
0.16,0.165,0.17,0.175,0.18,0.185,0.19,0.195,0.2,0.205,0.21,0.215,0.22,0.225,
0.23,0.235,0.24,0.245,0.25,0.255,0.26,0.265,0.27,0.275,0.28,0.285,0.29,
0.295,0.3,0.305,0.31,0.315,0.32,0.325,0.33,0.335,0.34,0.345,0.35,0.355,
0.36,0.365,0.37,0.375,0.38,0.385,0.39,0.395,0.4,0.405,0.41,0.415,0.42,0.425,
0.43,0.435,0.44,0.445,0.45,0.455,0.46,0.465,0.47,0.475,0.48,0.485,0.49,
0.495,0.5,0.505,0.51,0.515,0.52,0.525,0.53,0.535,0.54,0.545,0.55,0.555,
0.56,0.565,0.57,0.575,0.58,0.585,0.59,0.595,0.6,0.605,0.61,0.615,0.62,0.625,
0.63,0.635,0.64,0.645,0.65,0.655,0.66,0.665,0.67,0.675,0.68,0.685,0.690000000000001,
0.695000000000001,0.700000000000001,0.705000000000001,0.710000000000001,
0.715000000000001,0.720000000000001,0.725000000000001,0.730000000000001,
0.735000000000001,0.740000000000001,0.745000000000001,0.750000000000001,
0.755000000000001,0.760000000000001,0.765000000000001,0.770000000000001,
0.775000000000001,0.780000000000001,0.785000000000001,0.790000000000001,
0.795000000000001,0.800000000000001,0.805000000000001,0.810000000000001,
0.815000000000001,0.820000000000001,0.825000000000001,0.830000000000001,
0.835000000000001,0.840000000000001,0.845000000000001,0.850000000000001,
0.855000000000001,0.860000000000001,0.865000000000001,0.870000000000001,
0.875000000000001,0.880000000000001,0.885000000000001,0.890000000000001,
0.895000000000001,0.900000000000001,0.905000000000001,0.910000000000001,
0.915000000000001,0.920000000000001,0.925000000000001,0.930000000000001,
0.935000000000001,0.940000000000001,0.941429844437998),.UNSPECIFIED.)
CURVE()
GEOMETRIC_REPRESENTATION_ITEM()
RATIONAL_B_SPLINE_CURVE((1.,1.,1.,1.,1.,1.,1.,1.,1.,1.,1.,1.,1.,1.,1.,1.,
1.,1.,1.,1.,1.,1.,1.,1.,1.,1.,1.,1.,1.,1.,1.,1.,1.,1.,1.,1.,1.,1.,1.,1.,
1.,1.,1.,1.,1.,1.,1.,1.,1.,1.,1.,1.,1.,1.,1.,1.,1.,1.,1.,1.,1.,1.,1.,1.,
1.,1.,1.,1.,1.,1.,1.,1.,1.,1.,1.,1.,1.,1.,1.,1.,1.,1.,1.,1.,1.,1.,1.,1.,
1.,1.,1.,1.,1.,1.,1.,1.,1.,1.,1.,1.,1.,1.,1.,1.,1.,1.,1.,1.,1.,1.,1.,1.,
1.,1.,1.,1.,1.,1.,1.,1.,1.,1.,1.,1.,1.,1.,1.,1.,1.,1.,1.,1.,1.,1.,1.,1.,
1.,1.,1.,1.,1.,1.,1.,1.,1.,1.,1.,1.,1.,1.,1.,1.,1.,1.,1.,1.,1.,1.,1.,1.,
1.,1.,1.,1.,1.,1.,1.,1.,1.,1.,1.,1.,1.,1.,1.,1.,1.,1.,1.,1.,1.,1.,1.,1.,
1.,1.,1.,1.,1.,1.,1.,1.,1.,1.))
REPRESENTATION_ITEM('')
);
#630=(
BOUNDED_CURVE()
B_SPLINE_CURVE(5,(#150441,#150442,#150443,#150444,#150445,#150446,#150447,
#150448,#150449,#150450,#150451,#150452,#150453,#150454,#150455,#150456,
#150457,#150458,#150459,#150460,#150461,#150462,#150463,#150464,#150465,
#150466,#150467,#150468,#150469,#150470,#150471,#150472,#150473,#150474,
#150475,#150476,#150477,#150478,#150479,#150480,#150481,#150482,#150483,
#150484,#150485,#150486,#150487,#150488,#150489,#150490,#150491,#150492,
#150493,#150494,#150495,#150496,#150497,#150498,#150499,#150500,#150501,
#150502,#150503,#150504,#150505,#150506,#150507,#150508,#150509,#150510,
#150511,#150512,#150513,#150514,#150515,#150516,#150517,#150518,#150519,
#150520,#150521,#150522,#150523,#150524,#150525,#150526,#150527,#150528,
#150529,#150530,#150531,#150532,#150533,#150534,#150535,#150536,#150537,
#150538,#150539,#150540,#150541,#150542,#150543,#150544,#150545,#150546,
#150547,#150548,#150549,#150550,#150551,#150552,#150553,#150554,#150555,
#150556,#150557,#150558,#150559,#150560,#150561,#150562,#150563,#150564,
#150565,#150566,#150567,#150568,#150569,#150570,#150571,#150572,#150573,
#150574,#150575,#150576,#150577,#150578,#150579,#150580,#150581,#150582,
#150583,#150584,#150585,#150586,#150587,#150588,#150589,#150590,#150591,
#150592,#150593,#150594,#150595,#150596,#150597,#150598,#150599,#150600,
#150601,#150602,#150603,#150604,#150605,#150606,#150607,#150608,#150609,
#150610,#150611,#150612,#150613,#150614,#150615,#150616,#150617,#150618,
#150619,#150620,#150621,#150622,#150623,#150624,#150625,#150626,#150627,
#150628,#150629,#150630,#150631,#150632,#150633,#150634),.UNSPECIFIED.,
 .F.,.F.)
B_SPLINE_CURVE_WITH_KNOTS((6,1,1,1,1,1,1,1,1,1,1,1,1,1,1,1,1,1,1,1,1,1,
1,1,1,1,1,1,1,1,1,1,1,1,1,1,1,1,1,1,1,1,1,1,1,1,1,1,1,1,1,1,1,1,1,1,1,1,
1,1,1,1,1,1,1,1,1,1,1,1,1,1,1,1,1,1,1,1,1,1,1,1,1,1,1,1,1,1,1,1,1,1,1,1,
1,1,1,1,1,1,1,1,1,1,1,1,1,1,1,1,1,1,1,1,1,1,1,1,1,1,1,1,1,1,1,1,1,1,1,1,
1,1,1,1,1,1,1,1,1,1,1,1,1,1,1,1,1,1,1,1,1,1,1,1,1,1,1,1,1,1,1,1,1,1,1,1,
1,1,1,1,1,1,1,1,1,1,1,1,1,1,1,1,1,1,1,1,1,1,1,6),(-0.941429844437991,-0.940000000000001,
-0.935000000000001,-0.930000000000001,-0.925000000000001,-0.920000000000001,
-0.915000000000001,-0.910000000000001,-0.905000000000001,-0.900000000000001,
-0.895000000000001,-0.890000000000001,-0.885000000000001,-0.880000000000001,
-0.875000000000001,-0.870000000000001,-0.865000000000001,-0.860000000000001,
-0.855000000000001,-0.850000000000001,-0.845000000000001,-0.840000000000001,
-0.835000000000001,-0.830000000000001,-0.825000000000001,-0.820000000000001,
-0.815000000000001,-0.810000000000001,-0.805000000000001,-0.800000000000001,
-0.795000000000001,-0.790000000000001,-0.785000000000001,-0.780000000000001,
-0.775000000000001,-0.770000000000001,-0.765000000000001,-0.760000000000001,
-0.755000000000001,-0.750000000000001,-0.745000000000001,-0.740000000000001,
-0.735000000000001,-0.730000000000001,-0.725000000000001,-0.720000000000001,
-0.715000000000001,-0.710000000000001,-0.705000000000001,-0.700000000000001,
-0.695000000000001,-0.690000000000001,-0.685,-0.68,-0.675,-0.67,-0.665,
-0.66,-0.655,-0.65,-0.645,-0.64,-0.635,-0.63,-0.625,-0.62,-0.615,-0.61,
-0.605,-0.6,-0.595,-0.59,-0.585,-0.58,-0.575,-0.57,-0.565,-0.56,-0.555,
-0.55,-0.545,-0.54,-0.535,-0.53,-0.525,-0.52,-0.515,-0.51,-0.505,-0.5,-0.495,
-0.49,-0.485,-0.48,-0.475,-0.47,-0.465,-0.46,-0.455,-0.45,-0.445,-0.44,
-0.435,-0.43,-0.425,-0.42,-0.415,-0.41,-0.405,-0.4,-0.395,-0.39,-0.385,
-0.38,-0.375,-0.37,-0.365,-0.36,-0.355,-0.35,-0.345,-0.34,-0.335,-0.33,
-0.325,-0.32,-0.315,-0.31,-0.305,-0.3,-0.295,-0.29,-0.285,-0.28,-0.275,
-0.27,-0.265,-0.26,-0.255,-0.25,-0.245,-0.24,-0.235,-0.23,-0.225,-0.22,
-0.215,-0.21,-0.205,-0.2,-0.195,-0.19,-0.185,-0.18,-0.175,-0.17,-0.165,
-0.16,-0.155,-0.15,-0.145,-0.14,-0.135,-0.13,-0.125,-0.12,-0.115,-0.11,
-0.105,-0.1,-0.095,-0.09,-0.085,-0.08,-0.075,-0.07,-0.065,-0.06,-0.055,
-0.05,-0.045,-0.04,-0.035,-0.03,-0.025,-0.02,-0.015,-0.01,-0.005,0.),
 .UNSPECIFIED.)
CURVE()
GEOMETRIC_REPRESENTATION_ITEM()
RATIONAL_B_SPLINE_CURVE((1.,1.,1.,1.,1.,1.,1.,1.,1.,1.,1.,1.,1.,1.,1.,1.,
1.,1.,1.,1.,1.,1.,1.,1.,1.,1.,1.,1.,1.,1.,1.,1.,1.,1.,1.,1.,1.,1.,1.,1.,
1.,1.,1.,1.,1.,1.,1.,1.,1.,1.,1.,1.,1.,1.,1.,1.,1.,1.,1.,1.,1.,1.,1.,1.,
1.,1.,1.,1.,1.,1.,1.,1.,1.,1.,1.,1.,1.,1.,1.,1.,1.,1.,1.,1.,1.,1.,1.,1.,
1.,1.,1.,1.,1.,1.,1.,1.,1.,1.,1.,1.,1.,1.,1.,1.,1.,1.,1.,1.,1.,1.,1.,1.,
1.,1.,1.,1.,1.,1.,1.,1.,1.,1.,1.,1.,1.,1.,1.,1.,1.,1.,1.,1.,1.,1.,1.,1.,
1.,1.,1.,1.,1.,1.,1.,1.,1.,1.,1.,1.,1.,1.,1.,1.,1.,1.,1.,1.,1.,1.,1.,1.,
1.,1.,1.,1.,1.,1.,1.,1.,1.,1.,1.,1.,1.,1.,1.,1.,1.,1.,1.,1.,1.,1.,1.,1.,
1.,1.,1.,1.,1.,1.,1.,1.,1.,1.))
REPRESENTATION_ITEM('')
);
#631=(
BOUNDED_CURVE()
B_SPLINE_CURVE(5,(#151046,#151047,#151048,#151049,#151050,#151051,#151052,
#151053,#151054,#151055,#151056,#151057,#151058,#151059,#151060,#151061,
#151062,#151063,#151064,#151065,#151066,#151067,#151068,#151069,#151070,
#151071,#151072,#151073,#151074,#151075,#151076,#151077,#151078,#151079,
#151080,#151081,#151082,#151083,#151084,#151085,#151086,#151087,#151088,
#151089,#151090,#151091,#151092,#151093,#151094,#151095,#151096,#151097,
#151098,#151099,#151100,#151101,#151102,#151103,#151104,#151105,#151106,
#151107,#151108,#151109,#151110,#151111,#151112,#151113,#151114,#151115,
#151116,#151117,#151118,#151119,#151120,#151121,#151122,#151123,#151124,
#151125,#151126,#151127,#151128,#151129,#151130,#151131,#151132,#151133,
#151134,#151135,#151136,#151137,#151138,#151139,#151140,#151141,#151142,
#151143,#151144,#151145,#151146,#151147,#151148,#151149,#151150,#151151,
#151152,#151153,#151154,#151155,#151156,#151157,#151158,#151159,#151160,
#151161,#151162,#151163,#151164,#151165,#151166,#151167,#151168,#151169,
#151170,#151171,#151172,#151173,#151174,#151175,#151176,#151177,#151178,
#151179,#151180,#151181,#151182,#151183,#151184,#151185,#151186,#151187,
#151188,#151189,#151190,#151191,#151192,#151193,#151194,#151195,#151196,
#151197,#151198,#151199,#151200,#151201,#151202,#151203,#151204,#151205,
#151206,#151207,#151208,#151209,#151210,#151211,#151212,#151213,#151214,
#151215,#151216,#151217,#151218,#151219,#151220,#151221,#151222,#151223,
#151224,#151225,#151226,#151227,#151228,#151229,#151230,#151231,#151232,
#151233,#151234,#151235,#151236,#151237,#151238,#151239),.UNSPECIFIED.,
 .F.,.F.)
B_SPLINE_CURVE_WITH_KNOTS((6,1,1,1,1,1,1,1,1,1,1,1,1,1,1,1,1,1,1,1,1,1,
1,1,1,1,1,1,1,1,1,1,1,1,1,1,1,1,1,1,1,1,1,1,1,1,1,1,1,1,1,1,1,1,1,1,1,1,
1,1,1,1,1,1,1,1,1,1,1,1,1,1,1,1,1,1,1,1,1,1,1,1,1,1,1,1,1,1,1,1,1,1,1,1,
1,1,1,1,1,1,1,1,1,1,1,1,1,1,1,1,1,1,1,1,1,1,1,1,1,1,1,1,1,1,1,1,1,1,1,1,
1,1,1,1,1,1,1,1,1,1,1,1,1,1,1,1,1,1,1,1,1,1,1,1,1,1,1,1,1,1,1,1,1,1,1,1,
1,1,1,1,1,1,1,1,1,1,1,1,1,1,1,1,1,1,1,1,1,1,1,6),(0.,0.005,0.01,0.015,0.02,
0.025,0.03,0.035,0.04,0.045,0.05,0.055,0.06,0.065,0.07,0.075,0.08,0.085,
0.09,0.095,0.1,0.105,0.11,0.115,0.12,0.125,0.13,0.135,0.14,0.145,0.15,0.155,
0.16,0.165,0.17,0.175,0.18,0.185,0.19,0.195,0.2,0.205,0.21,0.215,0.22,0.225,
0.23,0.235,0.24,0.245,0.25,0.255,0.26,0.265,0.27,0.275,0.28,0.285,0.29,
0.295,0.3,0.305,0.31,0.315,0.32,0.325,0.33,0.335,0.34,0.345,0.35,0.355,
0.36,0.365,0.37,0.375,0.38,0.385,0.39,0.395,0.4,0.405,0.41,0.415,0.42,0.425,
0.43,0.435,0.44,0.445,0.45,0.455,0.46,0.465,0.47,0.475,0.48,0.485,0.49,
0.495,0.5,0.505,0.51,0.515,0.52,0.525,0.53,0.535,0.54,0.545,0.55,0.555,
0.56,0.565,0.57,0.575,0.58,0.585,0.59,0.595,0.6,0.605,0.61,0.615,0.62,0.625,
0.63,0.635,0.64,0.645,0.65,0.655,0.66,0.665,0.67,0.675,0.68,0.685,0.690000000000001,
0.695000000000001,0.700000000000001,0.705000000000001,0.710000000000001,
0.715000000000001,0.720000000000001,0.725000000000001,0.730000000000001,
0.735000000000001,0.740000000000001,0.745000000000001,0.750000000000001,
0.755000000000001,0.760000000000001,0.765000000000001,0.770000000000001,
0.775000000000001,0.780000000000001,0.785000000000001,0.790000000000001,
0.795000000000001,0.800000000000001,0.805000000000001,0.810000000000001,
0.815000000000001,0.820000000000001,0.825000000000001,0.830000000000001,
0.835000000000001,0.840000000000001,0.845000000000001,0.850000000000001,
0.855000000000001,0.860000000000001,0.865000000000001,0.870000000000001,
0.875000000000001,0.880000000000001,0.885000000000001,0.890000000000001,
0.895000000000001,0.900000000000001,0.905000000000001,0.910000000000001,
0.915000000000001,0.920000000000001,0.925000000000001,0.930000000000001,
0.935000000000001,0.940000000000001,0.94142984443805),.UNSPECIFIED.)
CURVE()
GEOMETRIC_REPRESENTATION_ITEM()
RATIONAL_B_SPLINE_CURVE((1.,1.,1.,1.,1.,1.,1.,1.,1.,1.,1.,1.,1.,1.,1.,1.,
1.,1.,1.,1.,1.,1.,1.,1.,1.,1.,1.,1.,1.,1.,1.,1.,1.,1.,1.,1.,1.,1.,1.,1.,
1.,1.,1.,1.,1.,1.,1.,1.,1.,1.,1.,1.,1.,1.,1.,1.,1.,1.,1.,1.,1.,1.,1.,1.,
1.,1.,1.,1.,1.,1.,1.,1.,1.,1.,1.,1.,1.,1.,1.,1.,1.,1.,1.,1.,1.,1.,1.,1.,
1.,1.,1.,1.,1.,1.,1.,1.,1.,1.,1.,1.,1.,1.,1.,1.,1.,1.,1.,1.,1.,1.,1.,1.,
1.,1.,1.,1.,1.,1.,1.,1.,1.,1.,1.,1.,1.,1.,1.,1.,1.,1.,1.,1.,1.,1.,1.,1.,
1.,1.,1.,1.,1.,1.,1.,1.,1.,1.,1.,1.,1.,1.,1.,1.,1.,1.,1.,1.,1.,1.,1.,1.,
1.,1.,1.,1.,1.,1.,1.,1.,1.,1.,1.,1.,1.,1.,1.,1.,1.,1.,1.,1.,1.,1.,1.,1.,
1.,1.,1.,1.,1.,1.,1.,1.,1.,1.))
REPRESENTATION_ITEM('')
);
#632=(
BOUNDED_CURVE()
B_SPLINE_CURVE(5,(#151242,#151243,#151244,#151245,#151246,#151247,#151248,
#151249,#151250,#151251,#151252,#151253,#151254,#151255,#151256,#151257,
#151258,#151259,#151260,#151261,#151262,#151263,#151264,#151265,#151266,
#151267,#151268,#151269,#151270,#151271,#151272,#151273,#151274,#151275,
#151276,#151277,#151278,#151279,#151280,#151281,#151282,#151283,#151284,
#151285,#151286,#151287,#151288,#151289,#151290,#151291,#151292,#151293,
#151294,#151295,#151296,#151297,#151298,#151299,#151300,#151301,#151302,
#151303,#151304,#151305,#151306,#151307,#151308,#151309,#151310,#151311,
#151312,#151313,#151314,#151315,#151316,#151317,#151318,#151319,#151320,
#151321,#151322,#151323,#151324,#151325,#151326,#151327,#151328,#151329,
#151330,#151331,#151332,#151333,#151334,#151335,#151336,#151337,#151338,
#151339,#151340,#151341,#151342,#151343,#151344,#151345,#151346,#151347,
#151348,#151349,#151350,#151351,#151352,#151353,#151354,#151355,#151356,
#151357,#151358,#151359,#151360,#151361,#151362,#151363,#151364,#151365,
#151366,#151367,#151368,#151369,#151370,#151371,#151372,#151373,#151374,
#151375,#151376,#151377,#151378,#151379,#151380,#151381,#151382,#151383,
#151384,#151385,#151386,#151387,#151388,#151389,#151390,#151391,#151392,
#151393,#151394,#151395,#151396,#151397,#151398,#151399,#151400,#151401,
#151402,#151403,#151404,#151405,#151406,#151407,#151408,#151409,#151410,
#151411,#151412,#151413,#151414,#151415,#151416,#151417,#151418,#151419,
#151420,#151421,#151422,#151423,#151424,#151425,#151426,#151427,#151428,
#151429,#151430,#151431,#151432,#151433,#151434,#151435),.UNSPECIFIED.,
 .F.,.F.)
B_SPLINE_CURVE_WITH_KNOTS((6,1,1,1,1,1,1,1,1,1,1,1,1,1,1,1,1,1,1,1,1,1,
1,1,1,1,1,1,1,1,1,1,1,1,1,1,1,1,1,1,1,1,1,1,1,1,1,1,1,1,1,1,1,1,1,1,1,1,
1,1,1,1,1,1,1,1,1,1,1,1,1,1,1,1,1,1,1,1,1,1,1,1,1,1,1,1,1,1,1,1,1,1,1,1,
1,1,1,1,1,1,1,1,1,1,1,1,1,1,1,1,1,1,1,1,1,1,1,1,1,1,1,1,1,1,1,1,1,1,1,1,
1,1,1,1,1,1,1,1,1,1,1,1,1,1,1,1,1,1,1,1,1,1,1,1,1,1,1,1,1,1,1,1,1,1,1,1,
1,1,1,1,1,1,1,1,1,1,1,1,1,1,1,1,1,1,1,1,1,1,1,6),(-0.941429844438045,-0.940000000000001,
-0.935000000000001,-0.930000000000001,-0.925000000000001,-0.920000000000001,
-0.915000000000001,-0.910000000000001,-0.905000000000001,-0.900000000000001,
-0.895000000000001,-0.890000000000001,-0.885000000000001,-0.880000000000001,
-0.875000000000001,-0.870000000000001,-0.865000000000001,-0.860000000000001,
-0.855000000000001,-0.850000000000001,-0.845000000000001,-0.840000000000001,
-0.835000000000001,-0.830000000000001,-0.825000000000001,-0.820000000000001,
-0.815000000000001,-0.810000000000001,-0.805000000000001,-0.800000000000001,
-0.795000000000001,-0.790000000000001,-0.785000000000001,-0.780000000000001,
-0.775000000000001,-0.770000000000001,-0.765000000000001,-0.760000000000001,
-0.755000000000001,-0.750000000000001,-0.745000000000001,-0.740000000000001,
-0.735000000000001,-0.730000000000001,-0.725000000000001,-0.720000000000001,
-0.715000000000001,-0.710000000000001,-0.705000000000001,-0.700000000000001,
-0.695000000000001,-0.690000000000001,-0.685,-0.68,-0.675,-0.67,-0.665,
-0.66,-0.655,-0.65,-0.645,-0.64,-0.635,-0.63,-0.625,-0.62,-0.615,-0.61,
-0.605,-0.6,-0.595,-0.59,-0.585,-0.58,-0.575,-0.57,-0.565,-0.56,-0.555,
-0.55,-0.545,-0.54,-0.535,-0.53,-0.525,-0.52,-0.515,-0.51,-0.505,-0.5,-0.495,
-0.49,-0.485,-0.48,-0.475,-0.47,-0.465,-0.46,-0.455,-0.45,-0.445,-0.44,
-0.435,-0.43,-0.425,-0.42,-0.415,-0.41,-0.405,-0.4,-0.395,-0.39,-0.385,
-0.38,-0.375,-0.37,-0.365,-0.36,-0.355,-0.35,-0.345,-0.34,-0.335,-0.33,
-0.325,-0.32,-0.315,-0.31,-0.305,-0.3,-0.295,-0.29,-0.285,-0.28,-0.275,
-0.27,-0.265,-0.26,-0.255,-0.25,-0.245,-0.24,-0.235,-0.23,-0.225,-0.22,
-0.215,-0.21,-0.205,-0.2,-0.195,-0.19,-0.185,-0.18,-0.175,-0.17,-0.165,
-0.16,-0.155,-0.15,-0.145,-0.14,-0.135,-0.13,-0.125,-0.12,-0.115,-0.11,
-0.105,-0.1,-0.095,-0.09,-0.085,-0.08,-0.075,-0.07,-0.065,-0.06,-0.055,
-0.05,-0.045,-0.04,-0.035,-0.03,-0.025,-0.02,-0.015,-0.01,-0.005,0.),
 .UNSPECIFIED.)
CURVE()
GEOMETRIC_REPRESENTATION_ITEM()
RATIONAL_B_SPLINE_CURVE((1.,1.,1.,1.,1.,1.,1.,1.,1.,1.,1.,1.,1.,1.,1.,1.,
1.,1.,1.,1.,1.,1.,1.,1.,1.,1.,1.,1.,1.,1.,1.,1.,1.,1.,1.,1.,1.,1.,1.,1.,
1.,1.,1.,1.,1.,1.,1.,1.,1.,1.,1.,1.,1.,1.,1.,1.,1.,1.,1.,1.,1.,1.,1.,1.,
1.,1.,1.,1.,1.,1.,1.,1.,1.,1.,1.,1.,1.,1.,1.,1.,1.,1.,1.,1.,1.,1.,1.,1.,
1.,1.,1.,1.,1.,1.,1.,1.,1.,1.,1.,1.,1.,1.,1.,1.,1.,1.,1.,1.,1.,1.,1.,1.,
1.,1.,1.,1.,1.,1.,1.,1.,1.,1.,1.,1.,1.,1.,1.,1.,1.,1.,1.,1.,1.,1.,1.,1.,
1.,1.,1.,1.,1.,1.,1.,1.,1.,1.,1.,1.,1.,1.,1.,1.,1.,1.,1.,1.,1.,1.,1.,1.,
1.,1.,1.,1.,1.,1.,1.,1.,1.,1.,1.,1.,1.,1.,1.,1.,1.,1.,1.,1.,1.,1.,1.,1.,
1.,1.,1.,1.,1.,1.,1.,1.,1.,1.))
REPRESENTATION_ITEM('')
);
#633=(
BOUNDED_CURVE()
B_SPLINE_CURVE(5,(#151847,#151848,#151849,#151850,#151851,#151852,#151853,
#151854,#151855,#151856,#151857,#151858,#151859,#151860,#151861,#151862,
#151863,#151864,#151865,#151866,#151867,#151868,#151869,#151870,#151871,
#151872,#151873,#151874,#151875,#151876,#151877,#151878,#151879,#151880,
#151881,#151882,#151883,#151884,#151885,#151886,#151887,#151888,#151889,
#151890,#151891,#151892,#151893,#151894,#151895,#151896,#151897,#151898,
#151899,#151900,#151901,#151902,#151903,#151904,#151905,#151906,#151907,
#151908,#151909,#151910,#151911,#151912,#151913,#151914,#151915,#151916,
#151917,#151918,#151919,#151920,#151921,#151922,#151923,#151924,#151925,
#151926,#151927,#151928,#151929,#151930,#151931,#151932,#151933,#151934,
#151935,#151936,#151937,#151938,#151939,#151940,#151941,#151942,#151943,
#151944,#151945,#151946,#151947,#151948,#151949,#151950,#151951,#151952,
#151953,#151954,#151955,#151956,#151957,#151958,#151959,#151960,#151961,
#151962,#151963,#151964,#151965,#151966,#151967,#151968,#151969,#151970,
#151971,#151972,#151973,#151974,#151975,#151976,#151977,#151978,#151979,
#151980,#151981,#151982,#151983,#151984,#151985,#151986,#151987,#151988,
#151989,#151990,#151991,#151992,#151993,#151994,#151995,#151996,#151997,
#151998,#151999,#152000,#152001,#152002,#152003,#152004,#152005,#152006,
#152007,#152008,#152009,#152010,#152011,#152012,#152013,#152014,#152015,
#152016,#152017,#152018,#152019,#152020,#152021,#152022,#152023,#152024,
#152025,#152026,#152027,#152028,#152029,#152030,#152031,#152032,#152033,
#152034,#152035,#152036,#152037,#152038,#152039,#152040),.UNSPECIFIED.,
 .F.,.F.)
B_SPLINE_CURVE_WITH_KNOTS((6,1,1,1,1,1,1,1,1,1,1,1,1,1,1,1,1,1,1,1,1,1,
1,1,1,1,1,1,1,1,1,1,1,1,1,1,1,1,1,1,1,1,1,1,1,1,1,1,1,1,1,1,1,1,1,1,1,1,
1,1,1,1,1,1,1,1,1,1,1,1,1,1,1,1,1,1,1,1,1,1,1,1,1,1,1,1,1,1,1,1,1,1,1,1,
1,1,1,1,1,1,1,1,1,1,1,1,1,1,1,1,1,1,1,1,1,1,1,1,1,1,1,1,1,1,1,1,1,1,1,1,
1,1,1,1,1,1,1,1,1,1,1,1,1,1,1,1,1,1,1,1,1,1,1,1,1,1,1,1,1,1,1,1,1,1,1,1,
1,1,1,1,1,1,1,1,1,1,1,1,1,1,1,1,1,1,1,1,1,1,1,6),(0.,0.005,0.01,0.015,0.02,
0.025,0.03,0.035,0.04,0.045,0.05,0.055,0.06,0.065,0.07,0.075,0.08,0.085,
0.09,0.095,0.1,0.105,0.11,0.115,0.12,0.125,0.13,0.135,0.14,0.145,0.15,0.155,
0.16,0.165,0.17,0.175,0.18,0.185,0.19,0.195,0.2,0.205,0.21,0.215,0.22,0.225,
0.23,0.235,0.24,0.245,0.25,0.255,0.26,0.265,0.27,0.275,0.28,0.285,0.29,
0.295,0.3,0.305,0.31,0.315,0.32,0.325,0.33,0.335,0.34,0.345,0.35,0.355,
0.36,0.365,0.37,0.375,0.38,0.385,0.39,0.395,0.4,0.405,0.41,0.415,0.42,0.425,
0.43,0.435,0.44,0.445,0.45,0.455,0.46,0.465,0.47,0.475,0.48,0.485,0.49,
0.495,0.5,0.505,0.51,0.515,0.52,0.525,0.53,0.535,0.54,0.545,0.55,0.555,
0.56,0.565,0.57,0.575,0.58,0.585,0.59,0.595,0.6,0.605,0.61,0.615,0.62,0.625,
0.63,0.635,0.64,0.645,0.65,0.655,0.66,0.665,0.67,0.675,0.68,0.685,0.690000000000001,
0.695000000000001,0.700000000000001,0.705000000000001,0.710000000000001,
0.715000000000001,0.720000000000001,0.725000000000001,0.730000000000001,
0.735000000000001,0.740000000000001,0.745000000000001,0.750000000000001,
0.755000000000001,0.760000000000001,0.765000000000001,0.770000000000001,
0.775000000000001,0.780000000000001,0.785000000000001,0.790000000000001,
0.795000000000001,0.800000000000001,0.805000000000001,0.810000000000001,
0.815000000000001,0.820000000000001,0.825000000000001,0.830000000000001,
0.835000000000001,0.840000000000001,0.845000000000001,0.850000000000001,
0.855000000000001,0.860000000000001,0.865000000000001,0.870000000000001,
0.875000000000001,0.880000000000001,0.885000000000001,0.890000000000001,
0.895000000000001,0.900000000000001,0.905000000000001,0.910000000000001,
0.915000000000001,0.920000000000001,0.925000000000001,0.930000000000001,
0.935000000000001,0.940000000000001,0.94142984443799),.UNSPECIFIED.)
CURVE()
GEOMETRIC_REPRESENTATION_ITEM()
RATIONAL_B_SPLINE_CURVE((1.,1.,1.,1.,1.,1.,1.,1.,1.,1.,1.,1.,1.,1.,1.,1.,
1.,1.,1.,1.,1.,1.,1.,1.,1.,1.,1.,1.,1.,1.,1.,1.,1.,1.,1.,1.,1.,1.,1.,1.,
1.,1.,1.,1.,1.,1.,1.,1.,1.,1.,1.,1.,1.,1.,1.,1.,1.,1.,1.,1.,1.,1.,1.,1.,
1.,1.,1.,1.,1.,1.,1.,1.,1.,1.,1.,1.,1.,1.,1.,1.,1.,1.,1.,1.,1.,1.,1.,1.,
1.,1.,1.,1.,1.,1.,1.,1.,1.,1.,1.,1.,1.,1.,1.,1.,1.,1.,1.,1.,1.,1.,1.,1.,
1.,1.,1.,1.,1.,1.,1.,1.,1.,1.,1.,1.,1.,1.,1.,1.,1.,1.,1.,1.,1.,1.,1.,1.,
1.,1.,1.,1.,1.,1.,1.,1.,1.,1.,1.,1.,1.,1.,1.,1.,1.,1.,1.,1.,1.,1.,1.,1.,
1.,1.,1.,1.,1.,1.,1.,1.,1.,1.,1.,1.,1.,1.,1.,1.,1.,1.,1.,1.,1.,1.,1.,1.,
1.,1.,1.,1.,1.,1.,1.,1.,1.,1.))
REPRESENTATION_ITEM('')
);
#634=(
BOUNDED_CURVE()
B_SPLINE_CURVE(5,(#152043,#152044,#152045,#152046,#152047,#152048,#152049,
#152050,#152051,#152052,#152053,#152054,#152055,#152056,#152057,#152058,
#152059,#152060,#152061,#152062,#152063,#152064,#152065,#152066,#152067,
#152068,#152069,#152070,#152071,#152072,#152073,#152074,#152075,#152076,
#152077,#152078,#152079,#152080,#152081,#152082,#152083,#152084,#152085,
#152086,#152087,#152088,#152089,#152090,#152091,#152092,#152093,#152094,
#152095,#152096,#152097,#152098,#152099,#152100,#152101,#152102,#152103,
#152104,#152105,#152106,#152107,#152108,#152109,#152110,#152111,#152112,
#152113,#152114,#152115,#152116,#152117,#152118,#152119,#152120,#152121,
#152122,#152123,#152124,#152125,#152126,#152127,#152128,#152129,#152130,
#152131,#152132,#152133,#152134,#152135,#152136,#152137,#152138,#152139,
#152140,#152141,#152142,#152143,#152144,#152145,#152146,#152147,#152148,
#152149,#152150,#152151,#152152,#152153,#152154,#152155,#152156,#152157,
#152158,#152159,#152160,#152161,#152162,#152163,#152164,#152165,#152166,
#152167,#152168,#152169,#152170,#152171,#152172,#152173,#152174,#152175,
#152176,#152177,#152178,#152179,#152180,#152181,#152182,#152183,#152184,
#152185,#152186,#152187,#152188,#152189,#152190,#152191,#152192,#152193,
#152194,#152195,#152196,#152197,#152198,#152199,#152200,#152201,#152202,
#152203,#152204,#152205,#152206,#152207,#152208,#152209,#152210,#152211,
#152212,#152213,#152214,#152215,#152216,#152217,#152218,#152219,#152220,
#152221,#152222,#152223,#152224,#152225,#152226,#152227,#152228,#152229,
#152230,#152231,#152232,#152233,#152234,#152235,#152236),.UNSPECIFIED.,
 .F.,.F.)
B_SPLINE_CURVE_WITH_KNOTS((6,1,1,1,1,1,1,1,1,1,1,1,1,1,1,1,1,1,1,1,1,1,
1,1,1,1,1,1,1,1,1,1,1,1,1,1,1,1,1,1,1,1,1,1,1,1,1,1,1,1,1,1,1,1,1,1,1,1,
1,1,1,1,1,1,1,1,1,1,1,1,1,1,1,1,1,1,1,1,1,1,1,1,1,1,1,1,1,1,1,1,1,1,1,1,
1,1,1,1,1,1,1,1,1,1,1,1,1,1,1,1,1,1,1,1,1,1,1,1,1,1,1,1,1,1,1,1,1,1,1,1,
1,1,1,1,1,1,1,1,1,1,1,1,1,1,1,1,1,1,1,1,1,1,1,1,1,1,1,1,1,1,1,1,1,1,1,1,
1,1,1,1,1,1,1,1,1,1,1,1,1,1,1,1,1,1,1,1,1,1,1,6),(-0.941429844437991,-0.940000000000001,
-0.935000000000001,-0.930000000000001,-0.925000000000001,-0.920000000000001,
-0.915000000000001,-0.910000000000001,-0.905000000000001,-0.900000000000001,
-0.895000000000001,-0.890000000000001,-0.885000000000001,-0.880000000000001,
-0.875000000000001,-0.870000000000001,-0.865000000000001,-0.860000000000001,
-0.855000000000001,-0.850000000000001,-0.845000000000001,-0.840000000000001,
-0.835000000000001,-0.830000000000001,-0.825000000000001,-0.820000000000001,
-0.815000000000001,-0.810000000000001,-0.805000000000001,-0.800000000000001,
-0.795000000000001,-0.790000000000001,-0.785000000000001,-0.780000000000001,
-0.775000000000001,-0.770000000000001,-0.765000000000001,-0.760000000000001,
-0.755000000000001,-0.750000000000001,-0.745000000000001,-0.740000000000001,
-0.735000000000001,-0.730000000000001,-0.725000000000001,-0.720000000000001,
-0.715000000000001,-0.710000000000001,-0.705000000000001,-0.700000000000001,
-0.695000000000001,-0.690000000000001,-0.685,-0.68,-0.675,-0.67,-0.665,
-0.66,-0.655,-0.65,-0.645,-0.64,-0.635,-0.63,-0.625,-0.62,-0.615,-0.61,
-0.605,-0.6,-0.595,-0.59,-0.585,-0.58,-0.575,-0.57,-0.565,-0.56,-0.555,
-0.55,-0.545,-0.54,-0.535,-0.53,-0.525,-0.52,-0.515,-0.51,-0.505,-0.5,-0.495,
-0.49,-0.485,-0.48,-0.475,-0.47,-0.465,-0.46,-0.455,-0.45,-0.445,-0.44,
-0.435,-0.43,-0.425,-0.42,-0.415,-0.41,-0.405,-0.4,-0.395,-0.39,-0.385,
-0.38,-0.375,-0.37,-0.365,-0.36,-0.355,-0.35,-0.345,-0.34,-0.335,-0.33,
-0.325,-0.32,-0.315,-0.31,-0.305,-0.3,-0.295,-0.29,-0.285,-0.28,-0.275,
-0.27,-0.265,-0.26,-0.255,-0.25,-0.245,-0.24,-0.235,-0.23,-0.225,-0.22,
-0.215,-0.21,-0.205,-0.2,-0.195,-0.19,-0.185,-0.18,-0.175,-0.17,-0.165,
-0.16,-0.155,-0.15,-0.145,-0.14,-0.135,-0.13,-0.125,-0.12,-0.115,-0.11,
-0.105,-0.1,-0.095,-0.09,-0.085,-0.08,-0.075,-0.07,-0.065,-0.06,-0.055,
-0.05,-0.045,-0.04,-0.035,-0.03,-0.025,-0.02,-0.015,-0.01,-0.005,0.),
 .UNSPECIFIED.)
CURVE()
GEOMETRIC_REPRESENTATION_ITEM()
RATIONAL_B_SPLINE_CURVE((1.,1.,1.,1.,1.,1.,1.,1.,1.,1.,1.,1.,1.,1.,1.,1.,
1.,1.,1.,1.,1.,1.,1.,1.,1.,1.,1.,1.,1.,1.,1.,1.,1.,1.,1.,1.,1.,1.,1.,1.,
1.,1.,1.,1.,1.,1.,1.,1.,1.,1.,1.,1.,1.,1.,1.,1.,1.,1.,1.,1.,1.,1.,1.,1.,
1.,1.,1.,1.,1.,1.,1.,1.,1.,1.,1.,1.,1.,1.,1.,1.,1.,1.,1.,1.,1.,1.,1.,1.,
1.,1.,1.,1.,1.,1.,1.,1.,1.,1.,1.,1.,1.,1.,1.,1.,1.,1.,1.,1.,1.,1.,1.,1.,
1.,1.,1.,1.,1.,1.,1.,1.,1.,1.,1.,1.,1.,1.,1.,1.,1.,1.,1.,1.,1.,1.,1.,1.,
1.,1.,1.,1.,1.,1.,1.,1.,1.,1.,1.,1.,1.,1.,1.,1.,1.,1.,1.,1.,1.,1.,1.,1.,
1.,1.,1.,1.,1.,1.,1.,1.,1.,1.,1.,1.,1.,1.,1.,1.,1.,1.,1.,1.,1.,1.,1.,1.,
1.,1.,1.,1.,1.,1.,1.,1.,1.,1.))
REPRESENTATION_ITEM('')
);
#635=(
BOUNDED_CURVE()
B_SPLINE_CURVE(5,(#152648,#152649,#152650,#152651,#152652,#152653,#152654,
#152655,#152656,#152657,#152658,#152659,#152660,#152661,#152662,#152663,
#152664,#152665,#152666,#152667,#152668,#152669,#152670,#152671,#152672,
#152673,#152674,#152675,#152676,#152677,#152678,#152679,#152680,#152681,
#152682,#152683,#152684,#152685,#152686,#152687,#152688,#152689,#152690,
#152691,#152692,#152693,#152694,#152695,#152696,#152697,#152698,#152699,
#152700,#152701,#152702,#152703,#152704,#152705,#152706,#152707,#152708,
#152709,#152710,#152711,#152712,#152713,#152714,#152715,#152716,#152717,
#152718,#152719,#152720,#152721,#152722,#152723,#152724,#152725,#152726,
#152727,#152728,#152729,#152730,#152731,#152732,#152733,#152734,#152735,
#152736,#152737,#152738,#152739,#152740,#152741,#152742,#152743,#152744,
#152745,#152746,#152747,#152748,#152749,#152750,#152751,#152752,#152753,
#152754,#152755,#152756,#152757,#152758,#152759,#152760,#152761,#152762,
#152763,#152764,#152765,#152766,#152767,#152768,#152769,#152770,#152771,
#152772,#152773,#152774,#152775,#152776,#152777,#152778,#152779,#152780,
#152781,#152782,#152783,#152784,#152785,#152786,#152787,#152788,#152789,
#152790,#152791,#152792,#152793,#152794,#152795,#152796,#152797,#152798,
#152799,#152800,#152801,#152802,#152803,#152804,#152805,#152806,#152807,
#152808,#152809,#152810,#152811,#152812,#152813,#152814,#152815,#152816,
#152817,#152818,#152819,#152820,#152821,#152822,#152823,#152824,#152825,
#152826,#152827,#152828,#152829,#152830,#152831,#152832,#152833,#152834,
#152835,#152836,#152837,#152838,#152839,#152840,#152841),.UNSPECIFIED.,
 .F.,.F.)
B_SPLINE_CURVE_WITH_KNOTS((6,1,1,1,1,1,1,1,1,1,1,1,1,1,1,1,1,1,1,1,1,1,
1,1,1,1,1,1,1,1,1,1,1,1,1,1,1,1,1,1,1,1,1,1,1,1,1,1,1,1,1,1,1,1,1,1,1,1,
1,1,1,1,1,1,1,1,1,1,1,1,1,1,1,1,1,1,1,1,1,1,1,1,1,1,1,1,1,1,1,1,1,1,1,1,
1,1,1,1,1,1,1,1,1,1,1,1,1,1,1,1,1,1,1,1,1,1,1,1,1,1,1,1,1,1,1,1,1,1,1,1,
1,1,1,1,1,1,1,1,1,1,1,1,1,1,1,1,1,1,1,1,1,1,1,1,1,1,1,1,1,1,1,1,1,1,1,1,
1,1,1,1,1,1,1,1,1,1,1,1,1,1,1,1,1,1,1,1,1,1,1,6),(0.,0.005,0.01,0.015,0.02,
0.025,0.03,0.035,0.04,0.045,0.05,0.055,0.06,0.065,0.07,0.075,0.08,0.085,
0.09,0.095,0.1,0.105,0.11,0.115,0.12,0.125,0.13,0.135,0.14,0.145,0.15,0.155,
0.16,0.165,0.17,0.175,0.18,0.185,0.19,0.195,0.2,0.205,0.21,0.215,0.22,0.225,
0.23,0.235,0.24,0.245,0.25,0.255,0.26,0.265,0.27,0.275,0.28,0.285,0.29,
0.295,0.3,0.305,0.31,0.315,0.32,0.325,0.33,0.335,0.34,0.345,0.35,0.355,
0.36,0.365,0.37,0.375,0.38,0.385,0.39,0.395,0.4,0.405,0.41,0.415,0.42,0.425,
0.43,0.435,0.44,0.445,0.45,0.455,0.46,0.465,0.47,0.475,0.48,0.485,0.49,
0.495,0.5,0.505,0.51,0.515,0.52,0.525,0.53,0.535,0.54,0.545,0.55,0.555,
0.56,0.565,0.57,0.575,0.58,0.585,0.59,0.595,0.6,0.605,0.61,0.615,0.62,0.625,
0.63,0.635,0.64,0.645,0.65,0.655,0.66,0.665,0.67,0.675,0.68,0.685,0.690000000000001,
0.695000000000001,0.700000000000001,0.705000000000001,0.710000000000001,
0.715000000000001,0.720000000000001,0.725000000000001,0.730000000000001,
0.735000000000001,0.740000000000001,0.745000000000001,0.750000000000001,
0.755000000000001,0.760000000000001,0.765000000000001,0.770000000000001,
0.775000000000001,0.780000000000001,0.785000000000001,0.790000000000001,
0.795000000000001,0.800000000000001,0.805000000000001,0.810000000000001,
0.815000000000001,0.820000000000001,0.825000000000001,0.830000000000001,
0.835000000000001,0.840000000000001,0.845000000000001,0.850000000000001,
0.855000000000001,0.860000000000001,0.865000000000001,0.870000000000001,
0.875000000000001,0.880000000000001,0.885000000000001,0.890000000000001,
0.895000000000001,0.900000000000001,0.905000000000001,0.910000000000001,
0.915000000000001,0.920000000000001,0.925000000000001,0.930000000000001,
0.935000000000001,0.940000000000001,0.941429844438037),.UNSPECIFIED.)
CURVE()
GEOMETRIC_REPRESENTATION_ITEM()
RATIONAL_B_SPLINE_CURVE((1.,1.,1.,1.,1.,1.,1.,1.,1.,1.,1.,1.,1.,1.,1.,1.,
1.,1.,1.,1.,1.,1.,1.,1.,1.,1.,1.,1.,1.,1.,1.,1.,1.,1.,1.,1.,1.,1.,1.,1.,
1.,1.,1.,1.,1.,1.,1.,1.,1.,1.,1.,1.,1.,1.,1.,1.,1.,1.,1.,1.,1.,1.,1.,1.,
1.,1.,1.,1.,1.,1.,1.,1.,1.,1.,1.,1.,1.,1.,1.,1.,1.,1.,1.,1.,1.,1.,1.,1.,
1.,1.,1.,1.,1.,1.,1.,1.,1.,1.,1.,1.,1.,1.,1.,1.,1.,1.,1.,1.,1.,1.,1.,1.,
1.,1.,1.,1.,1.,1.,1.,1.,1.,1.,1.,1.,1.,1.,1.,1.,1.,1.,1.,1.,1.,1.,1.,1.,
1.,1.,1.,1.,1.,1.,1.,1.,1.,1.,1.,1.,1.,1.,1.,1.,1.,1.,1.,1.,1.,1.,1.,1.,
1.,1.,1.,1.,1.,1.,1.,1.,1.,1.,1.,1.,1.,1.,1.,1.,1.,1.,1.,1.,1.,1.,1.,1.,
1.,1.,1.,1.,1.,1.,1.,1.,1.,1.))
REPRESENTATION_ITEM('')
);
#636=(
BOUNDED_CURVE()
B_SPLINE_CURVE(5,(#152844,#152845,#152846,#152847,#152848,#152849,#152850,
#152851,#152852,#152853,#152854,#152855,#152856,#152857,#152858,#152859,
#152860,#152861,#152862,#152863,#152864,#152865,#152866,#152867,#152868,
#152869,#152870,#152871,#152872,#152873,#152874,#152875,#152876,#152877,
#152878,#152879,#152880,#152881,#152882,#152883,#152884,#152885,#152886,
#152887,#152888,#152889,#152890,#152891,#152892,#152893,#152894,#152895,
#152896,#152897,#152898,#152899,#152900,#152901,#152902,#152903,#152904,
#152905,#152906,#152907,#152908,#152909,#152910,#152911,#152912,#152913,
#152914,#152915,#152916,#152917,#152918,#152919,#152920,#152921,#152922,
#152923,#152924,#152925,#152926,#152927,#152928,#152929,#152930,#152931,
#152932,#152933,#152934,#152935,#152936,#152937,#152938,#152939,#152940,
#152941,#152942,#152943,#152944,#152945,#152946,#152947,#152948,#152949,
#152950,#152951,#152952,#152953,#152954,#152955,#152956,#152957,#152958,
#152959,#152960,#152961,#152962,#152963,#152964,#152965,#152966,#152967,
#152968,#152969,#152970,#152971,#152972,#152973,#152974,#152975,#152976,
#152977,#152978,#152979,#152980,#152981,#152982,#152983,#152984,#152985,
#152986,#152987,#152988,#152989,#152990,#152991,#152992,#152993,#152994,
#152995,#152996,#152997,#152998,#152999,#153000,#153001,#153002,#153003,
#153004,#153005,#153006,#153007,#153008,#153009,#153010,#153011,#153012,
#153013,#153014,#153015,#153016,#153017,#153018,#153019,#153020,#153021,
#153022,#153023,#153024,#153025,#153026,#153027,#153028,#153029,#153030,
#153031,#153032,#153033,#153034,#153035,#153036,#153037),.UNSPECIFIED.,
 .F.,.F.)
B_SPLINE_CURVE_WITH_KNOTS((6,1,1,1,1,1,1,1,1,1,1,1,1,1,1,1,1,1,1,1,1,1,
1,1,1,1,1,1,1,1,1,1,1,1,1,1,1,1,1,1,1,1,1,1,1,1,1,1,1,1,1,1,1,1,1,1,1,1,
1,1,1,1,1,1,1,1,1,1,1,1,1,1,1,1,1,1,1,1,1,1,1,1,1,1,1,1,1,1,1,1,1,1,1,1,
1,1,1,1,1,1,1,1,1,1,1,1,1,1,1,1,1,1,1,1,1,1,1,1,1,1,1,1,1,1,1,1,1,1,1,1,
1,1,1,1,1,1,1,1,1,1,1,1,1,1,1,1,1,1,1,1,1,1,1,1,1,1,1,1,1,1,1,1,1,1,1,1,
1,1,1,1,1,1,1,1,1,1,1,1,1,1,1,1,1,1,1,1,1,1,1,6),(-0.941429844438034,-0.940000000000001,
-0.935000000000001,-0.930000000000001,-0.925000000000001,-0.920000000000001,
-0.915000000000001,-0.910000000000001,-0.905000000000001,-0.900000000000001,
-0.895000000000001,-0.890000000000001,-0.885000000000001,-0.880000000000001,
-0.875000000000001,-0.870000000000001,-0.865000000000001,-0.860000000000001,
-0.855000000000001,-0.850000000000001,-0.845000000000001,-0.840000000000001,
-0.835000000000001,-0.830000000000001,-0.825000000000001,-0.820000000000001,
-0.815000000000001,-0.810000000000001,-0.805000000000001,-0.800000000000001,
-0.795000000000001,-0.790000000000001,-0.785000000000001,-0.780000000000001,
-0.775000000000001,-0.770000000000001,-0.765000000000001,-0.760000000000001,
-0.755000000000001,-0.750000000000001,-0.745000000000001,-0.740000000000001,
-0.735000000000001,-0.730000000000001,-0.725000000000001,-0.720000000000001,
-0.715000000000001,-0.710000000000001,-0.705000000000001,-0.700000000000001,
-0.695000000000001,-0.690000000000001,-0.685,-0.68,-0.675,-0.67,-0.665,
-0.66,-0.655,-0.65,-0.645,-0.64,-0.635,-0.63,-0.625,-0.62,-0.615,-0.61,
-0.605,-0.6,-0.595,-0.59,-0.585,-0.58,-0.575,-0.57,-0.565,-0.56,-0.555,
-0.55,-0.545,-0.54,-0.535,-0.53,-0.525,-0.52,-0.515,-0.51,-0.505,-0.5,-0.495,
-0.49,-0.485,-0.48,-0.475,-0.47,-0.465,-0.46,-0.455,-0.45,-0.445,-0.44,
-0.435,-0.43,-0.425,-0.42,-0.415,-0.41,-0.405,-0.4,-0.395,-0.39,-0.385,
-0.38,-0.375,-0.37,-0.365,-0.36,-0.355,-0.35,-0.345,-0.34,-0.335,-0.33,
-0.325,-0.32,-0.315,-0.31,-0.305,-0.3,-0.295,-0.29,-0.285,-0.28,-0.275,
-0.27,-0.265,-0.26,-0.255,-0.25,-0.245,-0.24,-0.235,-0.23,-0.225,-0.22,
-0.215,-0.21,-0.205,-0.2,-0.195,-0.19,-0.185,-0.18,-0.175,-0.17,-0.165,
-0.16,-0.155,-0.15,-0.145,-0.14,-0.135,-0.13,-0.125,-0.12,-0.115,-0.11,
-0.105,-0.1,-0.095,-0.09,-0.085,-0.08,-0.075,-0.07,-0.065,-0.06,-0.055,
-0.05,-0.045,-0.04,-0.035,-0.03,-0.025,-0.02,-0.015,-0.01,-0.005,0.),
 .UNSPECIFIED.)
CURVE()
GEOMETRIC_REPRESENTATION_ITEM()
RATIONAL_B_SPLINE_CURVE((1.,1.,1.,1.,1.,1.,1.,1.,1.,1.,1.,1.,1.,1.,1.,1.,
1.,1.,1.,1.,1.,1.,1.,1.,1.,1.,1.,1.,1.,1.,1.,1.,1.,1.,1.,1.,1.,1.,1.,1.,
1.,1.,1.,1.,1.,1.,1.,1.,1.,1.,1.,1.,1.,1.,1.,1.,1.,1.,1.,1.,1.,1.,1.,1.,
1.,1.,1.,1.,1.,1.,1.,1.,1.,1.,1.,1.,1.,1.,1.,1.,1.,1.,1.,1.,1.,1.,1.,1.,
1.,1.,1.,1.,1.,1.,1.,1.,1.,1.,1.,1.,1.,1.,1.,1.,1.,1.,1.,1.,1.,1.,1.,1.,
1.,1.,1.,1.,1.,1.,1.,1.,1.,1.,1.,1.,1.,1.,1.,1.,1.,1.,1.,1.,1.,1.,1.,1.,
1.,1.,1.,1.,1.,1.,1.,1.,1.,1.,1.,1.,1.,1.,1.,1.,1.,1.,1.,1.,1.,1.,1.,1.,
1.,1.,1.,1.,1.,1.,1.,1.,1.,1.,1.,1.,1.,1.,1.,1.,1.,1.,1.,1.,1.,1.,1.,1.,
1.,1.,1.,1.,1.,1.,1.,1.,1.,1.))
REPRESENTATION_ITEM('')
);
#637=(
BOUNDED_CURVE()
B_SPLINE_CURVE(5,(#153449,#153450,#153451,#153452,#153453,#153454,#153455,
#153456,#153457,#153458,#153459,#153460,#153461,#153462,#153463,#153464,
#153465,#153466,#153467,#153468,#153469,#153470,#153471,#153472,#153473,
#153474,#153475,#153476,#153477,#153478,#153479,#153480,#153481,#153482,
#153483,#153484,#153485,#153486,#153487,#153488,#153489,#153490,#153491,
#153492,#153493,#153494,#153495,#153496,#153497,#153498,#153499,#153500,
#153501,#153502,#153503,#153504,#153505,#153506,#153507,#153508,#153509,
#153510,#153511,#153512,#153513,#153514,#153515,#153516,#153517,#153518,
#153519,#153520,#153521,#153522,#153523,#153524,#153525,#153526,#153527,
#153528,#153529,#153530,#153531,#153532,#153533,#153534,#153535,#153536,
#153537,#153538,#153539,#153540,#153541,#153542,#153543,#153544,#153545,
#153546,#153547,#153548,#153549,#153550,#153551,#153552,#153553,#153554,
#153555,#153556,#153557,#153558,#153559,#153560,#153561,#153562,#153563,
#153564,#153565,#153566,#153567,#153568,#153569,#153570,#153571,#153572,
#153573,#153574,#153575,#153576,#153577,#153578,#153579,#153580,#153581,
#153582,#153583,#153584,#153585,#153586,#153587,#153588,#153589,#153590,
#153591,#153592,#153593,#153594,#153595,#153596,#153597,#153598,#153599,
#153600,#153601,#153602,#153603,#153604,#153605,#153606,#153607,#153608,
#153609,#153610,#153611,#153612,#153613,#153614,#153615,#153616,#153617,
#153618,#153619,#153620,#153621,#153622,#153623,#153624,#153625,#153626,
#153627,#153628,#153629,#153630,#153631,#153632,#153633,#153634,#153635,
#153636,#153637,#153638,#153639,#153640,#153641,#153642),.UNSPECIFIED.,
 .F.,.F.)
B_SPLINE_CURVE_WITH_KNOTS((6,1,1,1,1,1,1,1,1,1,1,1,1,1,1,1,1,1,1,1,1,1,
1,1,1,1,1,1,1,1,1,1,1,1,1,1,1,1,1,1,1,1,1,1,1,1,1,1,1,1,1,1,1,1,1,1,1,1,
1,1,1,1,1,1,1,1,1,1,1,1,1,1,1,1,1,1,1,1,1,1,1,1,1,1,1,1,1,1,1,1,1,1,1,1,
1,1,1,1,1,1,1,1,1,1,1,1,1,1,1,1,1,1,1,1,1,1,1,1,1,1,1,1,1,1,1,1,1,1,1,1,
1,1,1,1,1,1,1,1,1,1,1,1,1,1,1,1,1,1,1,1,1,1,1,1,1,1,1,1,1,1,1,1,1,1,1,1,
1,1,1,1,1,1,1,1,1,1,1,1,1,1,1,1,1,1,1,1,1,1,1,6),(0.,0.005,0.01,0.015,0.02,
0.025,0.03,0.035,0.04,0.045,0.05,0.055,0.06,0.065,0.07,0.075,0.08,0.085,
0.09,0.095,0.1,0.105,0.11,0.115,0.12,0.125,0.13,0.135,0.14,0.145,0.15,0.155,
0.16,0.165,0.17,0.175,0.18,0.185,0.19,0.195,0.2,0.205,0.21,0.215,0.22,0.225,
0.23,0.235,0.24,0.245,0.25,0.255,0.26,0.265,0.27,0.275,0.28,0.285,0.29,
0.295,0.3,0.305,0.31,0.315,0.32,0.325,0.33,0.335,0.34,0.345,0.35,0.355,
0.36,0.365,0.37,0.375,0.38,0.385,0.39,0.395,0.4,0.405,0.41,0.415,0.42,0.425,
0.43,0.435,0.44,0.445,0.45,0.455,0.46,0.465,0.47,0.475,0.48,0.485,0.49,
0.495,0.5,0.505,0.51,0.515,0.52,0.525,0.53,0.535,0.54,0.545,0.55,0.555,
0.56,0.565,0.57,0.575,0.58,0.585,0.59,0.595,0.6,0.605,0.61,0.615,0.62,0.625,
0.63,0.635,0.64,0.645,0.65,0.655,0.66,0.665,0.67,0.675,0.68,0.685,0.690000000000001,
0.695000000000001,0.700000000000001,0.705000000000001,0.710000000000001,
0.715000000000001,0.720000000000001,0.725000000000001,0.730000000000001,
0.735000000000001,0.740000000000001,0.745000000000001,0.750000000000001,
0.755000000000001,0.760000000000001,0.765000000000001,0.770000000000001,
0.775000000000001,0.780000000000001,0.785000000000001,0.790000000000001,
0.795000000000001,0.800000000000001,0.805000000000001,0.810000000000001,
0.815000000000001,0.820000000000001,0.825000000000001,0.830000000000001,
0.835000000000001,0.840000000000001,0.845000000000001,0.850000000000001,
0.855000000000001,0.860000000000001,0.865000000000001,0.870000000000001,
0.875000000000001,0.880000000000001,0.885000000000001,0.890000000000001,
0.895000000000001,0.900000000000001,0.905000000000001,0.910000000000001,
0.915000000000001,0.920000000000001,0.925000000000001,0.930000000000001,
0.935000000000001,0.940000000000001,0.941429844438169),.UNSPECIFIED.)
CURVE()
GEOMETRIC_REPRESENTATION_ITEM()
RATIONAL_B_SPLINE_CURVE((1.,1.,1.,1.,1.,1.,1.,1.,1.,1.,1.,1.,1.,1.,1.,1.,
1.,1.,1.,1.,1.,1.,1.,1.,1.,1.,1.,1.,1.,1.,1.,1.,1.,1.,1.,1.,1.,1.,1.,1.,
1.,1.,1.,1.,1.,1.,1.,1.,1.,1.,1.,1.,1.,1.,1.,1.,1.,1.,1.,1.,1.,1.,1.,1.,
1.,1.,1.,1.,1.,1.,1.,1.,1.,1.,1.,1.,1.,1.,1.,1.,1.,1.,1.,1.,1.,1.,1.,1.,
1.,1.,1.,1.,1.,1.,1.,1.,1.,1.,1.,1.,1.,1.,1.,1.,1.,1.,1.,1.,1.,1.,1.,1.,
1.,1.,1.,1.,1.,1.,1.,1.,1.,1.,1.,1.,1.,1.,1.,1.,1.,1.,1.,1.,1.,1.,1.,1.,
1.,1.,1.,1.,1.,1.,1.,1.,1.,1.,1.,1.,1.,1.,1.,1.,1.,1.,1.,1.,1.,1.,1.,1.,
1.,1.,1.,1.,1.,1.,1.,1.,1.,1.,1.,1.,1.,1.,1.,1.,1.,1.,1.,1.,1.,1.,1.,1.,
1.,1.,1.,1.,1.,1.,1.,1.,1.,1.))
REPRESENTATION_ITEM('')
);
#638=(
BOUNDED_CURVE()
B_SPLINE_CURVE(5,(#153645,#153646,#153647,#153648,#153649,#153650,#153651,
#153652,#153653,#153654,#153655,#153656,#153657,#153658,#153659,#153660,
#153661,#153662,#153663,#153664,#153665,#153666,#153667,#153668,#153669,
#153670,#153671,#153672,#153673,#153674,#153675,#153676,#153677,#153678,
#153679,#153680,#153681,#153682,#153683,#153684,#153685,#153686,#153687,
#153688,#153689,#153690,#153691,#153692,#153693,#153694,#153695,#153696,
#153697,#153698,#153699,#153700,#153701,#153702,#153703,#153704,#153705,
#153706,#153707,#153708,#153709,#153710,#153711,#153712,#153713,#153714,
#153715,#153716,#153717,#153718,#153719,#153720,#153721,#153722,#153723,
#153724,#153725,#153726,#153727,#153728,#153729,#153730,#153731,#153732,
#153733,#153734,#153735,#153736,#153737,#153738,#153739,#153740,#153741,
#153742,#153743,#153744,#153745,#153746,#153747,#153748,#153749,#153750,
#153751,#153752,#153753,#153754,#153755,#153756,#153757,#153758,#153759,
#153760,#153761,#153762,#153763,#153764,#153765,#153766,#153767,#153768,
#153769,#153770,#153771,#153772,#153773,#153774,#153775,#153776,#153777,
#153778,#153779,#153780,#153781,#153782,#153783,#153784,#153785,#153786,
#153787,#153788,#153789,#153790,#153791,#153792,#153793,#153794,#153795,
#153796,#153797,#153798,#153799,#153800,#153801,#153802,#153803,#153804,
#153805,#153806,#153807,#153808,#153809,#153810,#153811,#153812,#153813,
#153814,#153815,#153816,#153817,#153818,#153819,#153820,#153821,#153822,
#153823,#153824,#153825,#153826,#153827,#153828,#153829,#153830,#153831,
#153832,#153833,#153834,#153835,#153836,#153837,#153838),.UNSPECIFIED.,
 .F.,.F.)
B_SPLINE_CURVE_WITH_KNOTS((6,1,1,1,1,1,1,1,1,1,1,1,1,1,1,1,1,1,1,1,1,1,
1,1,1,1,1,1,1,1,1,1,1,1,1,1,1,1,1,1,1,1,1,1,1,1,1,1,1,1,1,1,1,1,1,1,1,1,
1,1,1,1,1,1,1,1,1,1,1,1,1,1,1,1,1,1,1,1,1,1,1,1,1,1,1,1,1,1,1,1,1,1,1,1,
1,1,1,1,1,1,1,1,1,1,1,1,1,1,1,1,1,1,1,1,1,1,1,1,1,1,1,1,1,1,1,1,1,1,1,1,
1,1,1,1,1,1,1,1,1,1,1,1,1,1,1,1,1,1,1,1,1,1,1,1,1,1,1,1,1,1,1,1,1,1,1,1,
1,1,1,1,1,1,1,1,1,1,1,1,1,1,1,1,1,1,1,1,1,1,1,6),(-0.941429844438167,-0.940000000000001,
-0.935000000000001,-0.930000000000001,-0.925000000000001,-0.920000000000001,
-0.915000000000001,-0.910000000000001,-0.905000000000001,-0.900000000000001,
-0.895000000000001,-0.890000000000001,-0.885000000000001,-0.880000000000001,
-0.875000000000001,-0.870000000000001,-0.865000000000001,-0.860000000000001,
-0.855000000000001,-0.850000000000001,-0.845000000000001,-0.840000000000001,
-0.835000000000001,-0.830000000000001,-0.825000000000001,-0.820000000000001,
-0.815000000000001,-0.810000000000001,-0.805000000000001,-0.800000000000001,
-0.795000000000001,-0.790000000000001,-0.785000000000001,-0.780000000000001,
-0.775000000000001,-0.770000000000001,-0.765000000000001,-0.760000000000001,
-0.755000000000001,-0.750000000000001,-0.745000000000001,-0.740000000000001,
-0.735000000000001,-0.730000000000001,-0.725000000000001,-0.720000000000001,
-0.715000000000001,-0.710000000000001,-0.705000000000001,-0.700000000000001,
-0.695000000000001,-0.690000000000001,-0.685,-0.68,-0.675,-0.67,-0.665,
-0.66,-0.655,-0.65,-0.645,-0.64,-0.635,-0.63,-0.625,-0.62,-0.615,-0.61,
-0.605,-0.6,-0.595,-0.59,-0.585,-0.58,-0.575,-0.57,-0.565,-0.56,-0.555,
-0.55,-0.545,-0.54,-0.535,-0.53,-0.525,-0.52,-0.515,-0.51,-0.505,-0.5,-0.495,
-0.49,-0.485,-0.48,-0.475,-0.47,-0.465,-0.46,-0.455,-0.45,-0.445,-0.44,
-0.435,-0.43,-0.425,-0.42,-0.415,-0.41,-0.405,-0.4,-0.395,-0.39,-0.385,
-0.38,-0.375,-0.37,-0.365,-0.36,-0.355,-0.35,-0.345,-0.34,-0.335,-0.33,
-0.325,-0.32,-0.315,-0.31,-0.305,-0.3,-0.295,-0.29,-0.285,-0.28,-0.275,
-0.27,-0.265,-0.26,-0.255,-0.25,-0.245,-0.24,-0.235,-0.23,-0.225,-0.22,
-0.215,-0.21,-0.205,-0.2,-0.195,-0.19,-0.185,-0.18,-0.175,-0.17,-0.165,
-0.16,-0.155,-0.15,-0.145,-0.14,-0.135,-0.13,-0.125,-0.12,-0.115,-0.11,
-0.105,-0.1,-0.095,-0.09,-0.085,-0.08,-0.075,-0.07,-0.065,-0.06,-0.055,
-0.05,-0.045,-0.04,-0.035,-0.03,-0.025,-0.02,-0.015,-0.01,-0.005,0.),
 .UNSPECIFIED.)
CURVE()
GEOMETRIC_REPRESENTATION_ITEM()
RATIONAL_B_SPLINE_CURVE((1.,1.,1.,1.,1.,1.,1.,1.,1.,1.,1.,1.,1.,1.,1.,1.,
1.,1.,1.,1.,1.,1.,1.,1.,1.,1.,1.,1.,1.,1.,1.,1.,1.,1.,1.,1.,1.,1.,1.,1.,
1.,1.,1.,1.,1.,1.,1.,1.,1.,1.,1.,1.,1.,1.,1.,1.,1.,1.,1.,1.,1.,1.,1.,1.,
1.,1.,1.,1.,1.,1.,1.,1.,1.,1.,1.,1.,1.,1.,1.,1.,1.,1.,1.,1.,1.,1.,1.,1.,
1.,1.,1.,1.,1.,1.,1.,1.,1.,1.,1.,1.,1.,1.,1.,1.,1.,1.,1.,1.,1.,1.,1.,1.,
1.,1.,1.,1.,1.,1.,1.,1.,1.,1.,1.,1.,1.,1.,1.,1.,1.,1.,1.,1.,1.,1.,1.,1.,
1.,1.,1.,1.,1.,1.,1.,1.,1.,1.,1.,1.,1.,1.,1.,1.,1.,1.,1.,1.,1.,1.,1.,1.,
1.,1.,1.,1.,1.,1.,1.,1.,1.,1.,1.,1.,1.,1.,1.,1.,1.,1.,1.,1.,1.,1.,1.,1.,
1.,1.,1.,1.,1.,1.,1.,1.,1.,1.))
REPRESENTATION_ITEM('')
);
#639=(
BOUNDED_CURVE()
B_SPLINE_CURVE(5,(#154250,#154251,#154252,#154253,#154254,#154255,#154256,
#154257,#154258,#154259,#154260,#154261,#154262,#154263,#154264,#154265,
#154266,#154267,#154268,#154269,#154270,#154271,#154272,#154273,#154274,
#154275,#154276,#154277,#154278,#154279,#154280,#154281,#154282,#154283,
#154284,#154285,#154286,#154287,#154288,#154289,#154290,#154291,#154292,
#154293,#154294,#154295,#154296,#154297,#154298,#154299,#154300,#154301,
#154302,#154303,#154304,#154305,#154306,#154307,#154308,#154309,#154310,
#154311,#154312,#154313,#154314,#154315,#154316,#154317,#154318,#154319,
#154320,#154321,#154322,#154323,#154324,#154325,#154326,#154327,#154328,
#154329,#154330,#154331,#154332,#154333,#154334,#154335,#154336,#154337,
#154338,#154339,#154340,#154341,#154342,#154343,#154344,#154345,#154346,
#154347,#154348,#154349,#154350,#154351,#154352,#154353,#154354,#154355,
#154356,#154357,#154358,#154359,#154360,#154361,#154362,#154363,#154364,
#154365,#154366,#154367,#154368,#154369,#154370,#154371,#154372,#154373,
#154374,#154375,#154376,#154377,#154378,#154379,#154380,#154381,#154382,
#154383,#154384,#154385,#154386,#154387,#154388,#154389,#154390,#154391,
#154392,#154393,#154394,#154395,#154396,#154397,#154398,#154399,#154400,
#154401,#154402,#154403,#154404,#154405,#154406,#154407,#154408,#154409,
#154410,#154411,#154412,#154413,#154414,#154415,#154416,#154417,#154418,
#154419,#154420,#154421,#154422,#154423,#154424,#154425,#154426,#154427,
#154428,#154429,#154430,#154431,#154432,#154433,#154434,#154435,#154436,
#154437,#154438,#154439,#154440,#154441,#154442,#154443),.UNSPECIFIED.,
 .F.,.F.)
B_SPLINE_CURVE_WITH_KNOTS((6,1,1,1,1,1,1,1,1,1,1,1,1,1,1,1,1,1,1,1,1,1,
1,1,1,1,1,1,1,1,1,1,1,1,1,1,1,1,1,1,1,1,1,1,1,1,1,1,1,1,1,1,1,1,1,1,1,1,
1,1,1,1,1,1,1,1,1,1,1,1,1,1,1,1,1,1,1,1,1,1,1,1,1,1,1,1,1,1,1,1,1,1,1,1,
1,1,1,1,1,1,1,1,1,1,1,1,1,1,1,1,1,1,1,1,1,1,1,1,1,1,1,1,1,1,1,1,1,1,1,1,
1,1,1,1,1,1,1,1,1,1,1,1,1,1,1,1,1,1,1,1,1,1,1,1,1,1,1,1,1,1,1,1,1,1,1,1,
1,1,1,1,1,1,1,1,1,1,1,1,1,1,1,1,1,1,1,1,1,1,1,6),(0.,0.005,0.01,0.015,0.02,
0.025,0.03,0.035,0.04,0.045,0.05,0.055,0.06,0.065,0.07,0.075,0.08,0.085,
0.09,0.095,0.1,0.105,0.11,0.115,0.12,0.125,0.13,0.135,0.14,0.145,0.15,0.155,
0.16,0.165,0.17,0.175,0.18,0.185,0.19,0.195,0.2,0.205,0.21,0.215,0.22,0.225,
0.23,0.235,0.24,0.245,0.25,0.255,0.26,0.265,0.27,0.275,0.28,0.285,0.29,
0.295,0.3,0.305,0.31,0.315,0.32,0.325,0.33,0.335,0.34,0.345,0.35,0.355,
0.36,0.365,0.37,0.375,0.38,0.385,0.39,0.395,0.4,0.405,0.41,0.415,0.42,0.425,
0.43,0.435,0.44,0.445,0.45,0.455,0.46,0.465,0.47,0.475,0.48,0.485,0.49,
0.495,0.5,0.505,0.51,0.515,0.52,0.525,0.53,0.535,0.54,0.545,0.55,0.555,
0.56,0.565,0.57,0.575,0.58,0.585,0.59,0.595,0.6,0.605,0.61,0.615,0.62,0.625,
0.63,0.635,0.64,0.645,0.65,0.655,0.66,0.665,0.67,0.675,0.68,0.685,0.690000000000001,
0.695000000000001,0.700000000000001,0.705000000000001,0.710000000000001,
0.715000000000001,0.720000000000001,0.725000000000001,0.730000000000001,
0.735000000000001,0.740000000000001,0.745000000000001,0.750000000000001,
0.755000000000001,0.760000000000001,0.765000000000001,0.770000000000001,
0.775000000000001,0.780000000000001,0.785000000000001,0.790000000000001,
0.795000000000001,0.800000000000001,0.805000000000001,0.810000000000001,
0.815000000000001,0.820000000000001,0.825000000000001,0.830000000000001,
0.835000000000001,0.840000000000001,0.845000000000001,0.850000000000001,
0.855000000000001,0.860000000000001,0.865000000000001,0.870000000000001,
0.875000000000001,0.880000000000001,0.885000000000001,0.890000000000001,
0.895000000000001,0.900000000000001,0.905000000000001,0.910000000000001,
0.915000000000001,0.920000000000001,0.925000000000001,0.930000000000001,
0.935000000000001,0.940000000000001,0.941429844437968),.UNSPECIFIED.)
CURVE()
GEOMETRIC_REPRESENTATION_ITEM()
RATIONAL_B_SPLINE_CURVE((1.,1.,1.,1.,1.,1.,1.,1.,1.,1.,1.,1.,1.,1.,1.,1.,
1.,1.,1.,1.,1.,1.,1.,1.,1.,1.,1.,1.,1.,1.,1.,1.,1.,1.,1.,1.,1.,1.,1.,1.,
1.,1.,1.,1.,1.,1.,1.,1.,1.,1.,1.,1.,1.,1.,1.,1.,1.,1.,1.,1.,1.,1.,1.,1.,
1.,1.,1.,1.,1.,1.,1.,1.,1.,1.,1.,1.,1.,1.,1.,1.,1.,1.,1.,1.,1.,1.,1.,1.,
1.,1.,1.,1.,1.,1.,1.,1.,1.,1.,1.,1.,1.,1.,1.,1.,1.,1.,1.,1.,1.,1.,1.,1.,
1.,1.,1.,1.,1.,1.,1.,1.,1.,1.,1.,1.,1.,1.,1.,1.,1.,1.,1.,1.,1.,1.,1.,1.,
1.,1.,1.,1.,1.,1.,1.,1.,1.,1.,1.,1.,1.,1.,1.,1.,1.,1.,1.,1.,1.,1.,1.,1.,
1.,1.,1.,1.,1.,1.,1.,1.,1.,1.,1.,1.,1.,1.,1.,1.,1.,1.,1.,1.,1.,1.,1.,1.,
1.,1.,1.,1.,1.,1.,1.,1.,1.,1.))
REPRESENTATION_ITEM('')
);
#640=(
BOUNDED_CURVE()
B_SPLINE_CURVE(5,(#154446,#154447,#154448,#154449,#154450,#154451,#154452,
#154453,#154454,#154455,#154456,#154457,#154458,#154459,#154460,#154461,
#154462,#154463,#154464,#154465,#154466,#154467,#154468,#154469,#154470,
#154471,#154472,#154473,#154474,#154475,#154476,#154477,#154478,#154479,
#154480,#154481,#154482,#154483,#154484,#154485,#154486,#154487,#154488,
#154489,#154490,#154491,#154492,#154493,#154494,#154495,#154496,#154497,
#154498,#154499,#154500,#154501,#154502,#154503,#154504,#154505,#154506,
#154507,#154508,#154509,#154510,#154511,#154512,#154513,#154514,#154515,
#154516,#154517,#154518,#154519,#154520,#154521,#154522,#154523,#154524,
#154525,#154526,#154527,#154528,#154529,#154530,#154531,#154532,#154533,
#154534,#154535,#154536,#154537,#154538,#154539,#154540,#154541,#154542,
#154543,#154544,#154545,#154546,#154547,#154548,#154549,#154550,#154551,
#154552,#154553,#154554,#154555,#154556,#154557,#154558,#154559,#154560,
#154561,#154562,#154563,#154564,#154565,#154566,#154567,#154568,#154569,
#154570,#154571,#154572,#154573,#154574,#154575,#154576,#154577,#154578,
#154579,#154580,#154581,#154582,#154583,#154584,#154585,#154586,#154587,
#154588,#154589,#154590,#154591,#154592,#154593,#154594,#154595,#154596,
#154597,#154598,#154599,#154600,#154601,#154602,#154603,#154604,#154605,
#154606,#154607,#154608,#154609,#154610,#154611,#154612,#154613,#154614,
#154615,#154616,#154617,#154618,#154619,#154620,#154621,#154622,#154623,
#154624,#154625,#154626,#154627,#154628,#154629,#154630,#154631,#154632,
#154633,#154634,#154635,#154636,#154637,#154638,#154639),.UNSPECIFIED.,
 .F.,.F.)
B_SPLINE_CURVE_WITH_KNOTS((6,1,1,1,1,1,1,1,1,1,1,1,1,1,1,1,1,1,1,1,1,1,
1,1,1,1,1,1,1,1,1,1,1,1,1,1,1,1,1,1,1,1,1,1,1,1,1,1,1,1,1,1,1,1,1,1,1,1,
1,1,1,1,1,1,1,1,1,1,1,1,1,1,1,1,1,1,1,1,1,1,1,1,1,1,1,1,1,1,1,1,1,1,1,1,
1,1,1,1,1,1,1,1,1,1,1,1,1,1,1,1,1,1,1,1,1,1,1,1,1,1,1,1,1,1,1,1,1,1,1,1,
1,1,1,1,1,1,1,1,1,1,1,1,1,1,1,1,1,1,1,1,1,1,1,1,1,1,1,1,1,1,1,1,1,1,1,1,
1,1,1,1,1,1,1,1,1,1,1,1,1,1,1,1,1,1,1,1,1,1,1,6),(-0.94142984443797,-0.940000000000001,
-0.935000000000001,-0.930000000000001,-0.925000000000001,-0.920000000000001,
-0.915000000000001,-0.910000000000001,-0.905000000000001,-0.900000000000001,
-0.895000000000001,-0.890000000000001,-0.885000000000001,-0.880000000000001,
-0.875000000000001,-0.870000000000001,-0.865000000000001,-0.860000000000001,
-0.855000000000001,-0.850000000000001,-0.845000000000001,-0.840000000000001,
-0.835000000000001,-0.830000000000001,-0.825000000000001,-0.820000000000001,
-0.815000000000001,-0.810000000000001,-0.805000000000001,-0.800000000000001,
-0.795000000000001,-0.790000000000001,-0.785000000000001,-0.780000000000001,
-0.775000000000001,-0.770000000000001,-0.765000000000001,-0.760000000000001,
-0.755000000000001,-0.750000000000001,-0.745000000000001,-0.740000000000001,
-0.735000000000001,-0.730000000000001,-0.725000000000001,-0.720000000000001,
-0.715000000000001,-0.710000000000001,-0.705000000000001,-0.700000000000001,
-0.695000000000001,-0.690000000000001,-0.685,-0.68,-0.675,-0.67,-0.665,
-0.66,-0.655,-0.65,-0.645,-0.64,-0.635,-0.63,-0.625,-0.62,-0.615,-0.61,
-0.605,-0.6,-0.595,-0.59,-0.585,-0.58,-0.575,-0.57,-0.565,-0.56,-0.555,
-0.55,-0.545,-0.54,-0.535,-0.53,-0.525,-0.52,-0.515,-0.51,-0.505,-0.5,-0.495,
-0.49,-0.485,-0.48,-0.475,-0.47,-0.465,-0.46,-0.455,-0.45,-0.445,-0.44,
-0.435,-0.43,-0.425,-0.42,-0.415,-0.41,-0.405,-0.4,-0.395,-0.39,-0.385,
-0.38,-0.375,-0.37,-0.365,-0.36,-0.355,-0.35,-0.345,-0.34,-0.335,-0.33,
-0.325,-0.32,-0.315,-0.31,-0.305,-0.3,-0.295,-0.29,-0.285,-0.28,-0.275,
-0.27,-0.265,-0.26,-0.255,-0.25,-0.245,-0.24,-0.235,-0.23,-0.225,-0.22,
-0.215,-0.21,-0.205,-0.2,-0.195,-0.19,-0.185,-0.18,-0.175,-0.17,-0.165,
-0.16,-0.155,-0.15,-0.145,-0.14,-0.135,-0.13,-0.125,-0.12,-0.115,-0.11,
-0.105,-0.1,-0.095,-0.09,-0.085,-0.08,-0.075,-0.07,-0.065,-0.06,-0.055,
-0.05,-0.045,-0.04,-0.035,-0.03,-0.025,-0.02,-0.015,-0.01,-0.005,0.),
 .UNSPECIFIED.)
CURVE()
GEOMETRIC_REPRESENTATION_ITEM()
RATIONAL_B_SPLINE_CURVE((1.,1.,1.,1.,1.,1.,1.,1.,1.,1.,1.,1.,1.,1.,1.,1.,
1.,1.,1.,1.,1.,1.,1.,1.,1.,1.,1.,1.,1.,1.,1.,1.,1.,1.,1.,1.,1.,1.,1.,1.,
1.,1.,1.,1.,1.,1.,1.,1.,1.,1.,1.,1.,1.,1.,1.,1.,1.,1.,1.,1.,1.,1.,1.,1.,
1.,1.,1.,1.,1.,1.,1.,1.,1.,1.,1.,1.,1.,1.,1.,1.,1.,1.,1.,1.,1.,1.,1.,1.,
1.,1.,1.,1.,1.,1.,1.,1.,1.,1.,1.,1.,1.,1.,1.,1.,1.,1.,1.,1.,1.,1.,1.,1.,
1.,1.,1.,1.,1.,1.,1.,1.,1.,1.,1.,1.,1.,1.,1.,1.,1.,1.,1.,1.,1.,1.,1.,1.,
1.,1.,1.,1.,1.,1.,1.,1.,1.,1.,1.,1.,1.,1.,1.,1.,1.,1.,1.,1.,1.,1.,1.,1.,
1.,1.,1.,1.,1.,1.,1.,1.,1.,1.,1.,1.,1.,1.,1.,1.,1.,1.,1.,1.,1.,1.,1.,1.,
1.,1.,1.,1.,1.,1.,1.,1.,1.,1.))
REPRESENTATION_ITEM('')
);
#641=(
BOUNDED_CURVE()
B_SPLINE_CURVE(5,(#155051,#155052,#155053,#155054,#155055,#155056,#155057,
#155058,#155059,#155060,#155061,#155062,#155063,#155064,#155065,#155066,
#155067,#155068,#155069,#155070,#155071,#155072,#155073,#155074,#155075,
#155076,#155077,#155078,#155079,#155080,#155081,#155082,#155083,#155084,
#155085,#155086,#155087,#155088,#155089,#155090,#155091,#155092,#155093,
#155094,#155095,#155096,#155097,#155098,#155099,#155100,#155101,#155102,
#155103,#155104,#155105,#155106,#155107,#155108,#155109,#155110,#155111,
#155112,#155113,#155114,#155115,#155116,#155117,#155118,#155119,#155120,
#155121,#155122,#155123,#155124,#155125,#155126,#155127,#155128,#155129,
#155130,#155131,#155132,#155133,#155134,#155135,#155136,#155137,#155138,
#155139,#155140,#155141,#155142,#155143,#155144,#155145,#155146,#155147,
#155148,#155149,#155150,#155151,#155152,#155153,#155154,#155155,#155156,
#155157,#155158,#155159,#155160,#155161,#155162,#155163,#155164,#155165,
#155166,#155167,#155168,#155169,#155170,#155171,#155172,#155173,#155174,
#155175,#155176,#155177,#155178,#155179,#155180,#155181,#155182,#155183,
#155184,#155185,#155186,#155187,#155188,#155189,#155190,#155191,#155192,
#155193,#155194,#155195,#155196,#155197,#155198,#155199,#155200,#155201,
#155202,#155203,#155204,#155205,#155206,#155207,#155208,#155209,#155210,
#155211,#155212,#155213,#155214,#155215,#155216,#155217,#155218,#155219,
#155220,#155221,#155222,#155223,#155224,#155225,#155226,#155227,#155228,
#155229,#155230,#155231,#155232,#155233,#155234,#155235,#155236,#155237,
#155238,#155239,#155240,#155241,#155242,#155243,#155244),.UNSPECIFIED.,
 .F.,.F.)
B_SPLINE_CURVE_WITH_KNOTS((6,1,1,1,1,1,1,1,1,1,1,1,1,1,1,1,1,1,1,1,1,1,
1,1,1,1,1,1,1,1,1,1,1,1,1,1,1,1,1,1,1,1,1,1,1,1,1,1,1,1,1,1,1,1,1,1,1,1,
1,1,1,1,1,1,1,1,1,1,1,1,1,1,1,1,1,1,1,1,1,1,1,1,1,1,1,1,1,1,1,1,1,1,1,1,
1,1,1,1,1,1,1,1,1,1,1,1,1,1,1,1,1,1,1,1,1,1,1,1,1,1,1,1,1,1,1,1,1,1,1,1,
1,1,1,1,1,1,1,1,1,1,1,1,1,1,1,1,1,1,1,1,1,1,1,1,1,1,1,1,1,1,1,1,1,1,1,1,
1,1,1,1,1,1,1,1,1,1,1,1,1,1,1,1,1,1,1,1,1,1,1,6),(0.,0.005,0.01,0.015,0.02,
0.025,0.03,0.035,0.04,0.045,0.05,0.055,0.06,0.065,0.07,0.075,0.08,0.085,
0.09,0.095,0.1,0.105,0.11,0.115,0.12,0.125,0.13,0.135,0.14,0.145,0.15,0.155,
0.16,0.165,0.17,0.175,0.18,0.185,0.19,0.195,0.2,0.205,0.21,0.215,0.22,0.225,
0.23,0.235,0.24,0.245,0.25,0.255,0.26,0.265,0.27,0.275,0.28,0.285,0.29,
0.295,0.3,0.305,0.31,0.315,0.32,0.325,0.33,0.335,0.34,0.345,0.35,0.355,
0.36,0.365,0.37,0.375,0.38,0.385,0.39,0.395,0.4,0.405,0.41,0.415,0.42,0.425,
0.43,0.435,0.44,0.445,0.45,0.455,0.46,0.465,0.47,0.475,0.48,0.485,0.49,
0.495,0.5,0.505,0.51,0.515,0.52,0.525,0.53,0.535,0.54,0.545,0.55,0.555,
0.56,0.565,0.57,0.575,0.58,0.585,0.59,0.595,0.6,0.605,0.61,0.615,0.62,0.625,
0.63,0.635,0.64,0.645,0.65,0.655,0.66,0.665,0.67,0.675,0.68,0.685,0.690000000000001,
0.695000000000001,0.700000000000001,0.705000000000001,0.710000000000001,
0.715000000000001,0.720000000000001,0.725000000000001,0.730000000000001,
0.735000000000001,0.740000000000001,0.745000000000001,0.750000000000001,
0.755000000000001,0.760000000000001,0.765000000000001,0.770000000000001,
0.775000000000001,0.780000000000001,0.785000000000001,0.790000000000001,
0.795000000000001,0.800000000000001,0.805000000000001,0.810000000000001,
0.815000000000001,0.820000000000001,0.825000000000001,0.830000000000001,
0.835000000000001,0.840000000000001,0.845000000000001,0.850000000000001,
0.855000000000001,0.860000000000001,0.865000000000001,0.870000000000001,
0.875000000000001,0.880000000000001,0.885000000000001,0.890000000000001,
0.895000000000001,0.900000000000001,0.905000000000001,0.910000000000001,
0.915000000000001,0.920000000000001,0.925000000000001,0.930000000000001,
0.935000000000001,0.940000000000001,0.941429844438025),.UNSPECIFIED.)
CURVE()
GEOMETRIC_REPRESENTATION_ITEM()
RATIONAL_B_SPLINE_CURVE((1.,1.,1.,1.,1.,1.,1.,1.,1.,1.,1.,1.,1.,1.,1.,1.,
1.,1.,1.,1.,1.,1.,1.,1.,1.,1.,1.,1.,1.,1.,1.,1.,1.,1.,1.,1.,1.,1.,1.,1.,
1.,1.,1.,1.,1.,1.,1.,1.,1.,1.,1.,1.,1.,1.,1.,1.,1.,1.,1.,1.,1.,1.,1.,1.,
1.,1.,1.,1.,1.,1.,1.,1.,1.,1.,1.,1.,1.,1.,1.,1.,1.,1.,1.,1.,1.,1.,1.,1.,
1.,1.,1.,1.,1.,1.,1.,1.,1.,1.,1.,1.,1.,1.,1.,1.,1.,1.,1.,1.,1.,1.,1.,1.,
1.,1.,1.,1.,1.,1.,1.,1.,1.,1.,1.,1.,1.,1.,1.,1.,1.,1.,1.,1.,1.,1.,1.,1.,
1.,1.,1.,1.,1.,1.,1.,1.,1.,1.,1.,1.,1.,1.,1.,1.,1.,1.,1.,1.,1.,1.,1.,1.,
1.,1.,1.,1.,1.,1.,1.,1.,1.,1.,1.,1.,1.,1.,1.,1.,1.,1.,1.,1.,1.,1.,1.,1.,
1.,1.,1.,1.,1.,1.,1.,1.,1.,1.))
REPRESENTATION_ITEM('')
);
#642=(
BOUNDED_CURVE()
B_SPLINE_CURVE(5,(#155247,#155248,#155249,#155250,#155251,#155252,#155253,
#155254,#155255,#155256,#155257,#155258,#155259,#155260,#155261,#155262,
#155263,#155264,#155265,#155266,#155267,#155268,#155269,#155270,#155271,
#155272,#155273,#155274,#155275,#155276,#155277,#155278,#155279,#155280,
#155281,#155282,#155283,#155284,#155285,#155286,#155287,#155288,#155289,
#155290,#155291,#155292,#155293,#155294,#155295,#155296,#155297,#155298,
#155299,#155300,#155301,#155302,#155303,#155304,#155305,#155306,#155307,
#155308,#155309,#155310,#155311,#155312,#155313,#155314,#155315,#155316,
#155317,#155318,#155319,#155320,#155321,#155322,#155323,#155324,#155325,
#155326,#155327,#155328,#155329,#155330,#155331,#155332,#155333,#155334,
#155335,#155336,#155337,#155338,#155339,#155340,#155341,#155342,#155343,
#155344,#155345,#155346,#155347,#155348,#155349,#155350,#155351,#155352,
#155353,#155354,#155355,#155356,#155357,#155358,#155359,#155360,#155361,
#155362,#155363,#155364,#155365,#155366,#155367,#155368,#155369,#155370,
#155371,#155372,#155373,#155374,#155375,#155376,#155377,#155378,#155379,
#155380,#155381,#155382,#155383,#155384,#155385,#155386,#155387,#155388,
#155389,#155390,#155391,#155392,#155393,#155394,#155395,#155396,#155397,
#155398,#155399,#155400,#155401,#155402,#155403,#155404,#155405,#155406,
#155407,#155408,#155409,#155410,#155411,#155412,#155413,#155414,#155415,
#155416,#155417,#155418,#155419,#155420,#155421,#155422,#155423,#155424,
#155425,#155426,#155427,#155428,#155429,#155430,#155431,#155432,#155433,
#155434,#155435,#155436,#155437,#155438,#155439,#155440),.UNSPECIFIED.,
 .F.,.F.)
B_SPLINE_CURVE_WITH_KNOTS((6,1,1,1,1,1,1,1,1,1,1,1,1,1,1,1,1,1,1,1,1,1,
1,1,1,1,1,1,1,1,1,1,1,1,1,1,1,1,1,1,1,1,1,1,1,1,1,1,1,1,1,1,1,1,1,1,1,1,
1,1,1,1,1,1,1,1,1,1,1,1,1,1,1,1,1,1,1,1,1,1,1,1,1,1,1,1,1,1,1,1,1,1,1,1,
1,1,1,1,1,1,1,1,1,1,1,1,1,1,1,1,1,1,1,1,1,1,1,1,1,1,1,1,1,1,1,1,1,1,1,1,
1,1,1,1,1,1,1,1,1,1,1,1,1,1,1,1,1,1,1,1,1,1,1,1,1,1,1,1,1,1,1,1,1,1,1,1,
1,1,1,1,1,1,1,1,1,1,1,1,1,1,1,1,1,1,1,1,1,1,1,6),(-0.941429844438021,-0.940000000000001,
-0.935000000000001,-0.930000000000001,-0.925000000000001,-0.920000000000001,
-0.915000000000001,-0.910000000000001,-0.905000000000001,-0.900000000000001,
-0.895000000000001,-0.890000000000001,-0.885000000000001,-0.880000000000001,
-0.875000000000001,-0.870000000000001,-0.865000000000001,-0.860000000000001,
-0.855000000000001,-0.850000000000001,-0.845000000000001,-0.840000000000001,
-0.835000000000001,-0.830000000000001,-0.825000000000001,-0.820000000000001,
-0.815000000000001,-0.810000000000001,-0.805000000000001,-0.800000000000001,
-0.795000000000001,-0.790000000000001,-0.785000000000001,-0.780000000000001,
-0.775000000000001,-0.770000000000001,-0.765000000000001,-0.760000000000001,
-0.755000000000001,-0.750000000000001,-0.745000000000001,-0.740000000000001,
-0.735000000000001,-0.730000000000001,-0.725000000000001,-0.720000000000001,
-0.715000000000001,-0.710000000000001,-0.705000000000001,-0.700000000000001,
-0.695000000000001,-0.690000000000001,-0.685,-0.68,-0.675,-0.67,-0.665,
-0.66,-0.655,-0.65,-0.645,-0.64,-0.635,-0.63,-0.625,-0.62,-0.615,-0.61,
-0.605,-0.6,-0.595,-0.59,-0.585,-0.58,-0.575,-0.57,-0.565,-0.56,-0.555,
-0.55,-0.545,-0.54,-0.535,-0.53,-0.525,-0.52,-0.515,-0.51,-0.505,-0.5,-0.495,
-0.49,-0.485,-0.48,-0.475,-0.47,-0.465,-0.46,-0.455,-0.45,-0.445,-0.44,
-0.435,-0.43,-0.425,-0.42,-0.415,-0.41,-0.405,-0.4,-0.395,-0.39,-0.385,
-0.38,-0.375,-0.37,-0.365,-0.36,-0.355,-0.35,-0.345,-0.34,-0.335,-0.33,
-0.325,-0.32,-0.315,-0.31,-0.305,-0.3,-0.295,-0.29,-0.285,-0.28,-0.275,
-0.27,-0.265,-0.26,-0.255,-0.25,-0.245,-0.24,-0.235,-0.23,-0.225,-0.22,
-0.215,-0.21,-0.205,-0.2,-0.195,-0.19,-0.185,-0.18,-0.175,-0.17,-0.165,
-0.16,-0.155,-0.15,-0.145,-0.14,-0.135,-0.13,-0.125,-0.12,-0.115,-0.11,
-0.105,-0.1,-0.095,-0.09,-0.085,-0.08,-0.075,-0.07,-0.065,-0.06,-0.055,
-0.05,-0.045,-0.04,-0.035,-0.03,-0.025,-0.02,-0.015,-0.01,-0.005,0.),
 .UNSPECIFIED.)
CURVE()
GEOMETRIC_REPRESENTATION_ITEM()
RATIONAL_B_SPLINE_CURVE((1.,1.,1.,1.,1.,1.,1.,1.,1.,1.,1.,1.,1.,1.,1.,1.,
1.,1.,1.,1.,1.,1.,1.,1.,1.,1.,1.,1.,1.,1.,1.,1.,1.,1.,1.,1.,1.,1.,1.,1.,
1.,1.,1.,1.,1.,1.,1.,1.,1.,1.,1.,1.,1.,1.,1.,1.,1.,1.,1.,1.,1.,1.,1.,1.,
1.,1.,1.,1.,1.,1.,1.,1.,1.,1.,1.,1.,1.,1.,1.,1.,1.,1.,1.,1.,1.,1.,1.,1.,
1.,1.,1.,1.,1.,1.,1.,1.,1.,1.,1.,1.,1.,1.,1.,1.,1.,1.,1.,1.,1.,1.,1.,1.,
1.,1.,1.,1.,1.,1.,1.,1.,1.,1.,1.,1.,1.,1.,1.,1.,1.,1.,1.,1.,1.,1.,1.,1.,
1.,1.,1.,1.,1.,1.,1.,1.,1.,1.,1.,1.,1.,1.,1.,1.,1.,1.,1.,1.,1.,1.,1.,1.,
1.,1.,1.,1.,1.,1.,1.,1.,1.,1.,1.,1.,1.,1.,1.,1.,1.,1.,1.,1.,1.,1.,1.,1.,
1.,1.,1.,1.,1.,1.,1.,1.,1.,1.))
REPRESENTATION_ITEM('')
);
#643=(
BOUNDED_CURVE()
B_SPLINE_CURVE(5,(#155852,#155853,#155854,#155855,#155856,#155857,#155858,
#155859,#155860,#155861,#155862,#155863,#155864,#155865,#155866,#155867,
#155868,#155869,#155870,#155871,#155872,#155873,#155874,#155875,#155876,
#155877,#155878,#155879,#155880,#155881,#155882,#155883,#155884,#155885,
#155886,#155887,#155888,#155889,#155890,#155891,#155892,#155893,#155894,
#155895,#155896,#155897,#155898,#155899,#155900,#155901,#155902,#155903,
#155904,#155905,#155906,#155907,#155908,#155909,#155910,#155911,#155912,
#155913,#155914,#155915,#155916,#155917,#155918,#155919,#155920,#155921,
#155922,#155923,#155924,#155925,#155926,#155927,#155928,#155929,#155930,
#155931,#155932,#155933,#155934,#155935,#155936,#155937,#155938,#155939,
#155940,#155941,#155942,#155943,#155944,#155945,#155946,#155947,#155948,
#155949,#155950,#155951,#155952,#155953,#155954,#155955,#155956,#155957,
#155958,#155959,#155960,#155961,#155962,#155963,#155964,#155965,#155966,
#155967,#155968,#155969,#155970,#155971,#155972,#155973,#155974,#155975,
#155976,#155977,#155978,#155979,#155980,#155981,#155982,#155983,#155984,
#155985,#155986,#155987,#155988,#155989,#155990,#155991,#155992,#155993,
#155994,#155995,#155996,#155997,#155998,#155999,#156000,#156001,#156002,
#156003,#156004,#156005,#156006,#156007,#156008,#156009,#156010,#156011,
#156012,#156013,#156014,#156015,#156016,#156017,#156018,#156019,#156020,
#156021,#156022,#156023,#156024,#156025,#156026,#156027,#156028,#156029,
#156030,#156031,#156032,#156033,#156034,#156035,#156036,#156037,#156038,
#156039,#156040,#156041,#156042,#156043,#156044,#156045),.UNSPECIFIED.,
 .F.,.F.)
B_SPLINE_CURVE_WITH_KNOTS((6,1,1,1,1,1,1,1,1,1,1,1,1,1,1,1,1,1,1,1,1,1,
1,1,1,1,1,1,1,1,1,1,1,1,1,1,1,1,1,1,1,1,1,1,1,1,1,1,1,1,1,1,1,1,1,1,1,1,
1,1,1,1,1,1,1,1,1,1,1,1,1,1,1,1,1,1,1,1,1,1,1,1,1,1,1,1,1,1,1,1,1,1,1,1,
1,1,1,1,1,1,1,1,1,1,1,1,1,1,1,1,1,1,1,1,1,1,1,1,1,1,1,1,1,1,1,1,1,1,1,1,
1,1,1,1,1,1,1,1,1,1,1,1,1,1,1,1,1,1,1,1,1,1,1,1,1,1,1,1,1,1,1,1,1,1,1,1,
1,1,1,1,1,1,1,1,1,1,1,1,1,1,1,1,1,1,1,1,1,1,1,6),(0.,0.005,0.01,0.015,0.02,
0.025,0.03,0.035,0.04,0.045,0.05,0.055,0.06,0.065,0.07,0.075,0.08,0.085,
0.09,0.095,0.1,0.105,0.11,0.115,0.12,0.125,0.13,0.135,0.14,0.145,0.15,0.155,
0.16,0.165,0.17,0.175,0.18,0.185,0.19,0.195,0.2,0.205,0.21,0.215,0.22,0.225,
0.23,0.235,0.24,0.245,0.25,0.255,0.26,0.265,0.27,0.275,0.28,0.285,0.29,
0.295,0.3,0.305,0.31,0.315,0.32,0.325,0.33,0.335,0.34,0.345,0.35,0.355,
0.36,0.365,0.37,0.375,0.38,0.385,0.39,0.395,0.4,0.405,0.41,0.415,0.42,0.425,
0.43,0.435,0.44,0.445,0.45,0.455,0.46,0.465,0.47,0.475,0.48,0.485,0.49,
0.495,0.5,0.505,0.51,0.515,0.52,0.525,0.53,0.535,0.54,0.545,0.55,0.555,
0.56,0.565,0.57,0.575,0.58,0.585,0.59,0.595,0.6,0.605,0.61,0.615,0.62,0.625,
0.63,0.635,0.64,0.645,0.65,0.655,0.66,0.665,0.67,0.675,0.68,0.685,0.690000000000001,
0.695000000000001,0.700000000000001,0.705000000000001,0.710000000000001,
0.715000000000001,0.720000000000001,0.725000000000001,0.730000000000001,
0.735000000000001,0.740000000000001,0.745000000000001,0.750000000000001,
0.755000000000001,0.760000000000001,0.765000000000001,0.770000000000001,
0.775000000000001,0.780000000000001,0.785000000000001,0.790000000000001,
0.795000000000001,0.800000000000001,0.805000000000001,0.810000000000001,
0.815000000000001,0.820000000000001,0.825000000000001,0.830000000000001,
0.835000000000001,0.840000000000001,0.845000000000001,0.850000000000001,
0.855000000000001,0.860000000000001,0.865000000000001,0.870000000000001,
0.875000000000001,0.880000000000001,0.885000000000001,0.890000000000001,
0.895000000000001,0.900000000000001,0.905000000000001,0.910000000000001,
0.915000000000001,0.920000000000001,0.925000000000001,0.930000000000001,
0.935000000000001,0.940000000000001,0.941429844438046),.UNSPECIFIED.)
CURVE()
GEOMETRIC_REPRESENTATION_ITEM()
RATIONAL_B_SPLINE_CURVE((1.,1.,1.,1.,1.,1.,1.,1.,1.,1.,1.,1.,1.,1.,1.,1.,
1.,1.,1.,1.,1.,1.,1.,1.,1.,1.,1.,1.,1.,1.,1.,1.,1.,1.,1.,1.,1.,1.,1.,1.,
1.,1.,1.,1.,1.,1.,1.,1.,1.,1.,1.,1.,1.,1.,1.,1.,1.,1.,1.,1.,1.,1.,1.,1.,
1.,1.,1.,1.,1.,1.,1.,1.,1.,1.,1.,1.,1.,1.,1.,1.,1.,1.,1.,1.,1.,1.,1.,1.,
1.,1.,1.,1.,1.,1.,1.,1.,1.,1.,1.,1.,1.,1.,1.,1.,1.,1.,1.,1.,1.,1.,1.,1.,
1.,1.,1.,1.,1.,1.,1.,1.,1.,1.,1.,1.,1.,1.,1.,1.,1.,1.,1.,1.,1.,1.,1.,1.,
1.,1.,1.,1.,1.,1.,1.,1.,1.,1.,1.,1.,1.,1.,1.,1.,1.,1.,1.,1.,1.,1.,1.,1.,
1.,1.,1.,1.,1.,1.,1.,1.,1.,1.,1.,1.,1.,1.,1.,1.,1.,1.,1.,1.,1.,1.,1.,1.,
1.,1.,1.,1.,1.,1.,1.,1.,1.,1.))
REPRESENTATION_ITEM('')
);
#644=(
BOUNDED_CURVE()
B_SPLINE_CURVE(5,(#156048,#156049,#156050,#156051,#156052,#156053,#156054,
#156055,#156056,#156057,#156058,#156059,#156060,#156061,#156062,#156063,
#156064,#156065,#156066,#156067,#156068,#156069,#156070,#156071,#156072,
#156073,#156074,#156075,#156076,#156077,#156078,#156079,#156080,#156081,
#156082,#156083,#156084,#156085,#156086,#156087,#156088,#156089,#156090,
#156091,#156092,#156093,#156094,#156095,#156096,#156097,#156098,#156099,
#156100,#156101,#156102,#156103,#156104,#156105,#156106,#156107,#156108,
#156109,#156110,#156111,#156112,#156113,#156114,#156115,#156116,#156117,
#156118,#156119,#156120,#156121,#156122,#156123,#156124,#156125,#156126,
#156127,#156128,#156129,#156130,#156131,#156132,#156133,#156134,#156135,
#156136,#156137,#156138,#156139,#156140,#156141,#156142,#156143,#156144,
#156145,#156146,#156147,#156148,#156149,#156150,#156151,#156152,#156153,
#156154,#156155,#156156,#156157,#156158,#156159,#156160,#156161,#156162,
#156163,#156164,#156165,#156166,#156167,#156168,#156169,#156170,#156171,
#156172,#156173,#156174,#156175,#156176,#156177,#156178,#156179,#156180,
#156181,#156182,#156183,#156184,#156185,#156186,#156187,#156188,#156189,
#156190,#156191,#156192,#156193,#156194,#156195,#156196,#156197,#156198,
#156199,#156200,#156201,#156202,#156203,#156204,#156205,#156206,#156207,
#156208,#156209,#156210,#156211,#156212,#156213,#156214,#156215,#156216,
#156217,#156218,#156219,#156220,#156221,#156222,#156223,#156224,#156225,
#156226,#156227,#156228,#156229,#156230,#156231,#156232,#156233,#156234,
#156235,#156236,#156237,#156238,#156239,#156240,#156241),.UNSPECIFIED.,
 .F.,.F.)
B_SPLINE_CURVE_WITH_KNOTS((6,1,1,1,1,1,1,1,1,1,1,1,1,1,1,1,1,1,1,1,1,1,
1,1,1,1,1,1,1,1,1,1,1,1,1,1,1,1,1,1,1,1,1,1,1,1,1,1,1,1,1,1,1,1,1,1,1,1,
1,1,1,1,1,1,1,1,1,1,1,1,1,1,1,1,1,1,1,1,1,1,1,1,1,1,1,1,1,1,1,1,1,1,1,1,
1,1,1,1,1,1,1,1,1,1,1,1,1,1,1,1,1,1,1,1,1,1,1,1,1,1,1,1,1,1,1,1,1,1,1,1,
1,1,1,1,1,1,1,1,1,1,1,1,1,1,1,1,1,1,1,1,1,1,1,1,1,1,1,1,1,1,1,1,1,1,1,1,
1,1,1,1,1,1,1,1,1,1,1,1,1,1,1,1,1,1,1,1,1,1,1,6),(-0.941429844438047,-0.940000000000001,
-0.935000000000001,-0.930000000000001,-0.925000000000001,-0.920000000000001,
-0.915000000000001,-0.910000000000001,-0.905000000000001,-0.900000000000001,
-0.895000000000001,-0.890000000000001,-0.885000000000001,-0.880000000000001,
-0.875000000000001,-0.870000000000001,-0.865000000000001,-0.860000000000001,
-0.855000000000001,-0.850000000000001,-0.845000000000001,-0.840000000000001,
-0.835000000000001,-0.830000000000001,-0.825000000000001,-0.820000000000001,
-0.815000000000001,-0.810000000000001,-0.805000000000001,-0.800000000000001,
-0.795000000000001,-0.790000000000001,-0.785000000000001,-0.780000000000001,
-0.775000000000001,-0.770000000000001,-0.765000000000001,-0.760000000000001,
-0.755000000000001,-0.750000000000001,-0.745000000000001,-0.740000000000001,
-0.735000000000001,-0.730000000000001,-0.725000000000001,-0.720000000000001,
-0.715000000000001,-0.710000000000001,-0.705000000000001,-0.700000000000001,
-0.695000000000001,-0.690000000000001,-0.685,-0.68,-0.675,-0.67,-0.665,
-0.66,-0.655,-0.65,-0.645,-0.64,-0.635,-0.63,-0.625,-0.62,-0.615,-0.61,
-0.605,-0.6,-0.595,-0.59,-0.585,-0.58,-0.575,-0.57,-0.565,-0.56,-0.555,
-0.55,-0.545,-0.54,-0.535,-0.53,-0.525,-0.52,-0.515,-0.51,-0.505,-0.5,-0.495,
-0.49,-0.485,-0.48,-0.475,-0.47,-0.465,-0.46,-0.455,-0.45,-0.445,-0.44,
-0.435,-0.43,-0.425,-0.42,-0.415,-0.41,-0.405,-0.4,-0.395,-0.39,-0.385,
-0.38,-0.375,-0.37,-0.365,-0.36,-0.355,-0.35,-0.345,-0.34,-0.335,-0.33,
-0.325,-0.32,-0.315,-0.31,-0.305,-0.3,-0.295,-0.29,-0.285,-0.28,-0.275,
-0.27,-0.265,-0.26,-0.255,-0.25,-0.245,-0.24,-0.235,-0.23,-0.225,-0.22,
-0.215,-0.21,-0.205,-0.2,-0.195,-0.19,-0.185,-0.18,-0.175,-0.17,-0.165,
-0.16,-0.155,-0.15,-0.145,-0.14,-0.135,-0.13,-0.125,-0.12,-0.115,-0.11,
-0.105,-0.1,-0.095,-0.09,-0.085,-0.08,-0.075,-0.07,-0.065,-0.06,-0.055,
-0.05,-0.045,-0.04,-0.035,-0.03,-0.025,-0.02,-0.015,-0.01,-0.005,0.),
 .UNSPECIFIED.)
CURVE()
GEOMETRIC_REPRESENTATION_ITEM()
RATIONAL_B_SPLINE_CURVE((1.,1.,1.,1.,1.,1.,1.,1.,1.,1.,1.,1.,1.,1.,1.,1.,
1.,1.,1.,1.,1.,1.,1.,1.,1.,1.,1.,1.,1.,1.,1.,1.,1.,1.,1.,1.,1.,1.,1.,1.,
1.,1.,1.,1.,1.,1.,1.,1.,1.,1.,1.,1.,1.,1.,1.,1.,1.,1.,1.,1.,1.,1.,1.,1.,
1.,1.,1.,1.,1.,1.,1.,1.,1.,1.,1.,1.,1.,1.,1.,1.,1.,1.,1.,1.,1.,1.,1.,1.,
1.,1.,1.,1.,1.,1.,1.,1.,1.,1.,1.,1.,1.,1.,1.,1.,1.,1.,1.,1.,1.,1.,1.,1.,
1.,1.,1.,1.,1.,1.,1.,1.,1.,1.,1.,1.,1.,1.,1.,1.,1.,1.,1.,1.,1.,1.,1.,1.,
1.,1.,1.,1.,1.,1.,1.,1.,1.,1.,1.,1.,1.,1.,1.,1.,1.,1.,1.,1.,1.,1.,1.,1.,
1.,1.,1.,1.,1.,1.,1.,1.,1.,1.,1.,1.,1.,1.,1.,1.,1.,1.,1.,1.,1.,1.,1.,1.,
1.,1.,1.,1.,1.,1.,1.,1.,1.,1.))
REPRESENTATION_ITEM('')
);
#645=(
BOUNDED_CURVE()
B_SPLINE_CURVE(5,(#156653,#156654,#156655,#156656,#156657,#156658,#156659,
#156660,#156661,#156662,#156663,#156664,#156665,#156666,#156667,#156668,
#156669,#156670,#156671,#156672,#156673,#156674,#156675,#156676,#156677,
#156678,#156679,#156680,#156681,#156682,#156683,#156684,#156685,#156686,
#156687,#156688,#156689,#156690,#156691,#156692,#156693,#156694,#156695,
#156696,#156697,#156698,#156699,#156700,#156701,#156702,#156703,#156704,
#156705,#156706,#156707,#156708,#156709,#156710,#156711,#156712,#156713,
#156714,#156715,#156716,#156717,#156718,#156719,#156720,#156721,#156722,
#156723,#156724,#156725,#156726,#156727,#156728,#156729,#156730,#156731,
#156732,#156733,#156734,#156735,#156736,#156737,#156738,#156739,#156740,
#156741,#156742,#156743,#156744,#156745,#156746,#156747,#156748,#156749,
#156750,#156751,#156752,#156753,#156754,#156755,#156756,#156757,#156758,
#156759,#156760,#156761,#156762,#156763,#156764,#156765,#156766,#156767,
#156768,#156769,#156770,#156771,#156772,#156773,#156774,#156775,#156776,
#156777,#156778,#156779,#156780,#156781,#156782,#156783,#156784,#156785,
#156786,#156787,#156788,#156789,#156790,#156791,#156792,#156793,#156794,
#156795,#156796,#156797,#156798,#156799,#156800,#156801,#156802,#156803,
#156804,#156805,#156806,#156807,#156808,#156809,#156810,#156811,#156812,
#156813,#156814,#156815,#156816,#156817,#156818,#156819,#156820,#156821,
#156822,#156823,#156824,#156825,#156826,#156827,#156828,#156829,#156830,
#156831,#156832,#156833,#156834,#156835,#156836,#156837,#156838,#156839,
#156840,#156841,#156842,#156843,#156844,#156845,#156846),.UNSPECIFIED.,
 .F.,.F.)
B_SPLINE_CURVE_WITH_KNOTS((6,1,1,1,1,1,1,1,1,1,1,1,1,1,1,1,1,1,1,1,1,1,
1,1,1,1,1,1,1,1,1,1,1,1,1,1,1,1,1,1,1,1,1,1,1,1,1,1,1,1,1,1,1,1,1,1,1,1,
1,1,1,1,1,1,1,1,1,1,1,1,1,1,1,1,1,1,1,1,1,1,1,1,1,1,1,1,1,1,1,1,1,1,1,1,
1,1,1,1,1,1,1,1,1,1,1,1,1,1,1,1,1,1,1,1,1,1,1,1,1,1,1,1,1,1,1,1,1,1,1,1,
1,1,1,1,1,1,1,1,1,1,1,1,1,1,1,1,1,1,1,1,1,1,1,1,1,1,1,1,1,1,1,1,1,1,1,1,
1,1,1,1,1,1,1,1,1,1,1,1,1,1,1,1,1,1,1,1,1,1,1,6),(0.,0.005,0.01,0.015,0.02,
0.025,0.03,0.035,0.04,0.045,0.05,0.055,0.06,0.065,0.07,0.075,0.08,0.085,
0.09,0.095,0.1,0.105,0.11,0.115,0.12,0.125,0.13,0.135,0.14,0.145,0.15,0.155,
0.16,0.165,0.17,0.175,0.18,0.185,0.19,0.195,0.2,0.205,0.21,0.215,0.22,0.225,
0.23,0.235,0.24,0.245,0.25,0.255,0.26,0.265,0.27,0.275,0.28,0.285,0.29,
0.295,0.3,0.305,0.31,0.315,0.32,0.325,0.33,0.335,0.34,0.345,0.35,0.355,
0.36,0.365,0.37,0.375,0.38,0.385,0.39,0.395,0.4,0.405,0.41,0.415,0.42,0.425,
0.43,0.435,0.44,0.445,0.45,0.455,0.46,0.465,0.47,0.475,0.48,0.485,0.49,
0.495,0.5,0.505,0.51,0.515,0.52,0.525,0.53,0.535,0.54,0.545,0.55,0.555,
0.56,0.565,0.57,0.575,0.58,0.585,0.59,0.595,0.6,0.605,0.61,0.615,0.62,0.625,
0.63,0.635,0.64,0.645,0.65,0.655,0.66,0.665,0.67,0.675,0.68,0.685,0.690000000000001,
0.695000000000001,0.700000000000001,0.705000000000001,0.710000000000001,
0.715000000000001,0.720000000000001,0.725000000000001,0.730000000000001,
0.735000000000001,0.740000000000001,0.745000000000001,0.750000000000001,
0.755000000000001,0.760000000000001,0.765000000000001,0.770000000000001,
0.775000000000001,0.780000000000001,0.785000000000001,0.790000000000001,
0.795000000000001,0.800000000000001,0.805000000000001,0.810000000000001,
0.815000000000001,0.820000000000001,0.825000000000001,0.830000000000001,
0.835000000000001,0.840000000000001,0.845000000000001,0.850000000000001,
0.855000000000001,0.860000000000001,0.865000000000001,0.870000000000001,
0.875000000000001,0.880000000000001,0.885000000000001,0.890000000000001,
0.895000000000001,0.900000000000001,0.905000000000001,0.910000000000001,
0.915000000000001,0.920000000000001,0.925000000000001,0.930000000000001,
0.935000000000001,0.940000000000001,0.94142984443804),.UNSPECIFIED.)
CURVE()
GEOMETRIC_REPRESENTATION_ITEM()
RATIONAL_B_SPLINE_CURVE((1.,1.,1.,1.,1.,1.,1.,1.,1.,1.,1.,1.,1.,1.,1.,1.,
1.,1.,1.,1.,1.,1.,1.,1.,1.,1.,1.,1.,1.,1.,1.,1.,1.,1.,1.,1.,1.,1.,1.,1.,
1.,1.,1.,1.,1.,1.,1.,1.,1.,1.,1.,1.,1.,1.,1.,1.,1.,1.,1.,1.,1.,1.,1.,1.,
1.,1.,1.,1.,1.,1.,1.,1.,1.,1.,1.,1.,1.,1.,1.,1.,1.,1.,1.,1.,1.,1.,1.,1.,
1.,1.,1.,1.,1.,1.,1.,1.,1.,1.,1.,1.,1.,1.,1.,1.,1.,1.,1.,1.,1.,1.,1.,1.,
1.,1.,1.,1.,1.,1.,1.,1.,1.,1.,1.,1.,1.,1.,1.,1.,1.,1.,1.,1.,1.,1.,1.,1.,
1.,1.,1.,1.,1.,1.,1.,1.,1.,1.,1.,1.,1.,1.,1.,1.,1.,1.,1.,1.,1.,1.,1.,1.,
1.,1.,1.,1.,1.,1.,1.,1.,1.,1.,1.,1.,1.,1.,1.,1.,1.,1.,1.,1.,1.,1.,1.,1.,
1.,1.,1.,1.,1.,1.,1.,1.,1.,1.))
REPRESENTATION_ITEM('')
);
#646=(
BOUNDED_CURVE()
B_SPLINE_CURVE(5,(#156849,#156850,#156851,#156852,#156853,#156854,#156855,
#156856,#156857,#156858,#156859,#156860,#156861,#156862,#156863,#156864,
#156865,#156866,#156867,#156868,#156869,#156870,#156871,#156872,#156873,
#156874,#156875,#156876,#156877,#156878,#156879,#156880,#156881,#156882,
#156883,#156884,#156885,#156886,#156887,#156888,#156889,#156890,#156891,
#156892,#156893,#156894,#156895,#156896,#156897,#156898,#156899,#156900,
#156901,#156902,#156903,#156904,#156905,#156906,#156907,#156908,#156909,
#156910,#156911,#156912,#156913,#156914,#156915,#156916,#156917,#156918,
#156919,#156920,#156921,#156922,#156923,#156924,#156925,#156926,#156927,
#156928,#156929,#156930,#156931,#156932,#156933,#156934,#156935,#156936,
#156937,#156938,#156939,#156940,#156941,#156942,#156943,#156944,#156945,
#156946,#156947,#156948,#156949,#156950,#156951,#156952,#156953,#156954,
#156955,#156956,#156957,#156958,#156959,#156960,#156961,#156962,#156963,
#156964,#156965,#156966,#156967,#156968,#156969,#156970,#156971,#156972,
#156973,#156974,#156975,#156976,#156977,#156978,#156979,#156980,#156981,
#156982,#156983,#156984,#156985,#156986,#156987,#156988,#156989,#156990,
#156991,#156992,#156993,#156994,#156995,#156996,#156997,#156998,#156999,
#157000,#157001,#157002,#157003,#157004,#157005,#157006,#157007,#157008,
#157009,#157010,#157011,#157012,#157013,#157014,#157015,#157016,#157017,
#157018,#157019,#157020,#157021,#157022,#157023,#157024,#157025,#157026,
#157027,#157028,#157029,#157030,#157031,#157032,#157033,#157034,#157035,
#157036,#157037,#157038,#157039,#157040,#157041,#157042),.UNSPECIFIED.,
 .F.,.F.)
B_SPLINE_CURVE_WITH_KNOTS((6,1,1,1,1,1,1,1,1,1,1,1,1,1,1,1,1,1,1,1,1,1,
1,1,1,1,1,1,1,1,1,1,1,1,1,1,1,1,1,1,1,1,1,1,1,1,1,1,1,1,1,1,1,1,1,1,1,1,
1,1,1,1,1,1,1,1,1,1,1,1,1,1,1,1,1,1,1,1,1,1,1,1,1,1,1,1,1,1,1,1,1,1,1,1,
1,1,1,1,1,1,1,1,1,1,1,1,1,1,1,1,1,1,1,1,1,1,1,1,1,1,1,1,1,1,1,1,1,1,1,1,
1,1,1,1,1,1,1,1,1,1,1,1,1,1,1,1,1,1,1,1,1,1,1,1,1,1,1,1,1,1,1,1,1,1,1,1,
1,1,1,1,1,1,1,1,1,1,1,1,1,1,1,1,1,1,1,1,1,1,1,6),(-0.94142984443804,-0.940000000000001,
-0.935000000000001,-0.930000000000001,-0.925000000000001,-0.920000000000001,
-0.915000000000001,-0.910000000000001,-0.905000000000001,-0.900000000000001,
-0.895000000000001,-0.890000000000001,-0.885000000000001,-0.880000000000001,
-0.875000000000001,-0.870000000000001,-0.865000000000001,-0.860000000000001,
-0.855000000000001,-0.850000000000001,-0.845000000000001,-0.840000000000001,
-0.835000000000001,-0.830000000000001,-0.825000000000001,-0.820000000000001,
-0.815000000000001,-0.810000000000001,-0.805000000000001,-0.800000000000001,
-0.795000000000001,-0.790000000000001,-0.785000000000001,-0.780000000000001,
-0.775000000000001,-0.770000000000001,-0.765000000000001,-0.760000000000001,
-0.755000000000001,-0.750000000000001,-0.745000000000001,-0.740000000000001,
-0.735000000000001,-0.730000000000001,-0.725000000000001,-0.720000000000001,
-0.715000000000001,-0.710000000000001,-0.705000000000001,-0.700000000000001,
-0.695000000000001,-0.690000000000001,-0.685,-0.68,-0.675,-0.67,-0.665,
-0.66,-0.655,-0.65,-0.645,-0.64,-0.635,-0.63,-0.625,-0.62,-0.615,-0.61,
-0.605,-0.6,-0.595,-0.59,-0.585,-0.58,-0.575,-0.57,-0.565,-0.56,-0.555,
-0.55,-0.545,-0.54,-0.535,-0.53,-0.525,-0.52,-0.515,-0.51,-0.505,-0.5,-0.495,
-0.49,-0.485,-0.48,-0.475,-0.47,-0.465,-0.46,-0.455,-0.45,-0.445,-0.44,
-0.435,-0.43,-0.425,-0.42,-0.415,-0.41,-0.405,-0.4,-0.395,-0.39,-0.385,
-0.38,-0.375,-0.37,-0.365,-0.36,-0.355,-0.35,-0.345,-0.34,-0.335,-0.33,
-0.325,-0.32,-0.315,-0.31,-0.305,-0.3,-0.295,-0.29,-0.285,-0.28,-0.275,
-0.27,-0.265,-0.26,-0.255,-0.25,-0.245,-0.24,-0.235,-0.23,-0.225,-0.22,
-0.215,-0.21,-0.205,-0.2,-0.195,-0.19,-0.185,-0.18,-0.175,-0.17,-0.165,
-0.16,-0.155,-0.15,-0.145,-0.14,-0.135,-0.13,-0.125,-0.12,-0.115,-0.11,
-0.105,-0.1,-0.095,-0.09,-0.085,-0.08,-0.075,-0.07,-0.065,-0.06,-0.055,
-0.05,-0.045,-0.04,-0.035,-0.03,-0.025,-0.02,-0.015,-0.01,-0.005,0.),
 .UNSPECIFIED.)
CURVE()
GEOMETRIC_REPRESENTATION_ITEM()
RATIONAL_B_SPLINE_CURVE((1.,1.,1.,1.,1.,1.,1.,1.,1.,1.,1.,1.,1.,1.,1.,1.,
1.,1.,1.,1.,1.,1.,1.,1.,1.,1.,1.,1.,1.,1.,1.,1.,1.,1.,1.,1.,1.,1.,1.,1.,
1.,1.,1.,1.,1.,1.,1.,1.,1.,1.,1.,1.,1.,1.,1.,1.,1.,1.,1.,1.,1.,1.,1.,1.,
1.,1.,1.,1.,1.,1.,1.,1.,1.,1.,1.,1.,1.,1.,1.,1.,1.,1.,1.,1.,1.,1.,1.,1.,
1.,1.,1.,1.,1.,1.,1.,1.,1.,1.,1.,1.,1.,1.,1.,1.,1.,1.,1.,1.,1.,1.,1.,1.,
1.,1.,1.,1.,1.,1.,1.,1.,1.,1.,1.,1.,1.,1.,1.,1.,1.,1.,1.,1.,1.,1.,1.,1.,
1.,1.,1.,1.,1.,1.,1.,1.,1.,1.,1.,1.,1.,1.,1.,1.,1.,1.,1.,1.,1.,1.,1.,1.,
1.,1.,1.,1.,1.,1.,1.,1.,1.,1.,1.,1.,1.,1.,1.,1.,1.,1.,1.,1.,1.,1.,1.,1.,
1.,1.,1.,1.,1.,1.,1.,1.,1.,1.))
REPRESENTATION_ITEM('')
);
#647=(
BOUNDED_CURVE()
B_SPLINE_CURVE(5,(#157454,#157455,#157456,#157457,#157458,#157459,#157460,
#157461,#157462,#157463,#157464,#157465,#157466,#157467,#157468,#157469,
#157470,#157471,#157472,#157473,#157474,#157475,#157476,#157477,#157478,
#157479,#157480,#157481,#157482,#157483,#157484,#157485,#157486,#157487,
#157488,#157489,#157490,#157491,#157492,#157493,#157494,#157495,#157496,
#157497,#157498,#157499,#157500,#157501,#157502,#157503,#157504,#157505,
#157506,#157507,#157508,#157509,#157510,#157511,#157512,#157513,#157514,
#157515,#157516,#157517,#157518,#157519,#157520,#157521,#157522,#157523,
#157524,#157525,#157526,#157527,#157528,#157529,#157530,#157531,#157532,
#157533,#157534,#157535,#157536,#157537,#157538,#157539,#157540,#157541,
#157542,#157543,#157544,#157545,#157546,#157547,#157548,#157549,#157550,
#157551,#157552,#157553,#157554,#157555,#157556,#157557,#157558,#157559,
#157560,#157561,#157562,#157563,#157564,#157565,#157566,#157567,#157568,
#157569,#157570,#157571,#157572,#157573,#157574,#157575,#157576,#157577,
#157578,#157579,#157580,#157581,#157582,#157583,#157584,#157585,#157586,
#157587,#157588,#157589,#157590,#157591,#157592,#157593,#157594,#157595,
#157596,#157597,#157598,#157599,#157600,#157601,#157602,#157603,#157604,
#157605,#157606,#157607,#157608,#157609,#157610,#157611,#157612,#157613,
#157614,#157615,#157616,#157617,#157618,#157619,#157620,#157621,#157622,
#157623,#157624,#157625,#157626,#157627,#157628,#157629,#157630,#157631,
#157632,#157633,#157634,#157635,#157636,#157637,#157638,#157639,#157640,
#157641,#157642,#157643,#157644,#157645,#157646,#157647),.UNSPECIFIED.,
 .F.,.F.)
B_SPLINE_CURVE_WITH_KNOTS((6,1,1,1,1,1,1,1,1,1,1,1,1,1,1,1,1,1,1,1,1,1,
1,1,1,1,1,1,1,1,1,1,1,1,1,1,1,1,1,1,1,1,1,1,1,1,1,1,1,1,1,1,1,1,1,1,1,1,
1,1,1,1,1,1,1,1,1,1,1,1,1,1,1,1,1,1,1,1,1,1,1,1,1,1,1,1,1,1,1,1,1,1,1,1,
1,1,1,1,1,1,1,1,1,1,1,1,1,1,1,1,1,1,1,1,1,1,1,1,1,1,1,1,1,1,1,1,1,1,1,1,
1,1,1,1,1,1,1,1,1,1,1,1,1,1,1,1,1,1,1,1,1,1,1,1,1,1,1,1,1,1,1,1,1,1,1,1,
1,1,1,1,1,1,1,1,1,1,1,1,1,1,1,1,1,1,1,1,1,1,1,6),(0.,0.005,0.01,0.015,0.02,
0.025,0.03,0.035,0.04,0.045,0.05,0.055,0.06,0.065,0.07,0.075,0.08,0.085,
0.09,0.095,0.1,0.105,0.11,0.115,0.12,0.125,0.13,0.135,0.14,0.145,0.15,0.155,
0.16,0.165,0.17,0.175,0.18,0.185,0.19,0.195,0.2,0.205,0.21,0.215,0.22,0.225,
0.23,0.235,0.24,0.245,0.25,0.255,0.26,0.265,0.27,0.275,0.28,0.285,0.29,
0.295,0.3,0.305,0.31,0.315,0.32,0.325,0.33,0.335,0.34,0.345,0.35,0.355,
0.36,0.365,0.37,0.375,0.38,0.385,0.39,0.395,0.4,0.405,0.41,0.415,0.42,0.425,
0.43,0.435,0.44,0.445,0.45,0.455,0.46,0.465,0.47,0.475,0.48,0.485,0.49,
0.495,0.5,0.505,0.51,0.515,0.52,0.525,0.53,0.535,0.54,0.545,0.55,0.555,
0.56,0.565,0.57,0.575,0.58,0.585,0.59,0.595,0.6,0.605,0.61,0.615,0.62,0.625,
0.63,0.635,0.64,0.645,0.65,0.655,0.66,0.665,0.67,0.675,0.68,0.685,0.690000000000001,
0.695000000000001,0.700000000000001,0.705000000000001,0.710000000000001,
0.715000000000001,0.720000000000001,0.725000000000001,0.730000000000001,
0.735000000000001,0.740000000000001,0.745000000000001,0.750000000000001,
0.755000000000001,0.760000000000001,0.765000000000001,0.770000000000001,
0.775000000000001,0.780000000000001,0.785000000000001,0.790000000000001,
0.795000000000001,0.800000000000001,0.805000000000001,0.810000000000001,
0.815000000000001,0.820000000000001,0.825000000000001,0.830000000000001,
0.835000000000001,0.840000000000001,0.845000000000001,0.850000000000001,
0.855000000000001,0.860000000000001,0.865000000000001,0.870000000000001,
0.875000000000001,0.880000000000001,0.885000000000001,0.890000000000001,
0.895000000000001,0.900000000000001,0.905000000000001,0.910000000000001,
0.915000000000001,0.920000000000001,0.925000000000001,0.930000000000001,
0.935000000000001,0.940000000000001,0.941429844438052),.UNSPECIFIED.)
CURVE()
GEOMETRIC_REPRESENTATION_ITEM()
RATIONAL_B_SPLINE_CURVE((1.,1.,1.,1.,1.,1.,1.,1.,1.,1.,1.,1.,1.,1.,1.,1.,
1.,1.,1.,1.,1.,1.,1.,1.,1.,1.,1.,1.,1.,1.,1.,1.,1.,1.,1.,1.,1.,1.,1.,1.,
1.,1.,1.,1.,1.,1.,1.,1.,1.,1.,1.,1.,1.,1.,1.,1.,1.,1.,1.,1.,1.,1.,1.,1.,
1.,1.,1.,1.,1.,1.,1.,1.,1.,1.,1.,1.,1.,1.,1.,1.,1.,1.,1.,1.,1.,1.,1.,1.,
1.,1.,1.,1.,1.,1.,1.,1.,1.,1.,1.,1.,1.,1.,1.,1.,1.,1.,1.,1.,1.,1.,1.,1.,
1.,1.,1.,1.,1.,1.,1.,1.,1.,1.,1.,1.,1.,1.,1.,1.,1.,1.,1.,1.,1.,1.,1.,1.,
1.,1.,1.,1.,1.,1.,1.,1.,1.,1.,1.,1.,1.,1.,1.,1.,1.,1.,1.,1.,1.,1.,1.,1.,
1.,1.,1.,1.,1.,1.,1.,1.,1.,1.,1.,1.,1.,1.,1.,1.,1.,1.,1.,1.,1.,1.,1.,1.,
1.,1.,1.,1.,1.,1.,1.,1.,1.,1.))
REPRESENTATION_ITEM('')
);
#648=(
BOUNDED_CURVE()
B_SPLINE_CURVE(5,(#157650,#157651,#157652,#157653,#157654,#157655,#157656,
#157657,#157658,#157659,#157660,#157661,#157662,#157663,#157664,#157665,
#157666,#157667,#157668,#157669,#157670,#157671,#157672,#157673,#157674,
#157675,#157676,#157677,#157678,#157679,#157680,#157681,#157682,#157683,
#157684,#157685,#157686,#157687,#157688,#157689,#157690,#157691,#157692,
#157693,#157694,#157695,#157696,#157697,#157698,#157699,#157700,#157701,
#157702,#157703,#157704,#157705,#157706,#157707,#157708,#157709,#157710,
#157711,#157712,#157713,#157714,#157715,#157716,#157717,#157718,#157719,
#157720,#157721,#157722,#157723,#157724,#157725,#157726,#157727,#157728,
#157729,#157730,#157731,#157732,#157733,#157734,#157735,#157736,#157737,
#157738,#157739,#157740,#157741,#157742,#157743,#157744,#157745,#157746,
#157747,#157748,#157749,#157750,#157751,#157752,#157753,#157754,#157755,
#157756,#157757,#157758,#157759,#157760,#157761,#157762,#157763,#157764,
#157765,#157766,#157767,#157768,#157769,#157770,#157771,#157772,#157773,
#157774,#157775,#157776,#157777,#157778,#157779,#157780,#157781,#157782,
#157783,#157784,#157785,#157786,#157787,#157788,#157789,#157790,#157791,
#157792,#157793,#157794,#157795,#157796,#157797,#157798,#157799,#157800,
#157801,#157802,#157803,#157804,#157805,#157806,#157807,#157808,#157809,
#157810,#157811,#157812,#157813,#157814,#157815,#157816,#157817,#157818,
#157819,#157820,#157821,#157822,#157823,#157824,#157825,#157826,#157827,
#157828,#157829,#157830,#157831,#157832,#157833,#157834,#157835,#157836,
#157837,#157838,#157839,#157840,#157841,#157842,#157843),.UNSPECIFIED.,
 .F.,.F.)
B_SPLINE_CURVE_WITH_KNOTS((6,1,1,1,1,1,1,1,1,1,1,1,1,1,1,1,1,1,1,1,1,1,
1,1,1,1,1,1,1,1,1,1,1,1,1,1,1,1,1,1,1,1,1,1,1,1,1,1,1,1,1,1,1,1,1,1,1,1,
1,1,1,1,1,1,1,1,1,1,1,1,1,1,1,1,1,1,1,1,1,1,1,1,1,1,1,1,1,1,1,1,1,1,1,1,
1,1,1,1,1,1,1,1,1,1,1,1,1,1,1,1,1,1,1,1,1,1,1,1,1,1,1,1,1,1,1,1,1,1,1,1,
1,1,1,1,1,1,1,1,1,1,1,1,1,1,1,1,1,1,1,1,1,1,1,1,1,1,1,1,1,1,1,1,1,1,1,1,
1,1,1,1,1,1,1,1,1,1,1,1,1,1,1,1,1,1,1,1,1,1,1,6),(-0.941429844438052,-0.940000000000001,
-0.935000000000001,-0.930000000000001,-0.925000000000001,-0.920000000000001,
-0.915000000000001,-0.910000000000001,-0.905000000000001,-0.900000000000001,
-0.895000000000001,-0.890000000000001,-0.885000000000001,-0.880000000000001,
-0.875000000000001,-0.870000000000001,-0.865000000000001,-0.860000000000001,
-0.855000000000001,-0.850000000000001,-0.845000000000001,-0.840000000000001,
-0.835000000000001,-0.830000000000001,-0.825000000000001,-0.820000000000001,
-0.815000000000001,-0.810000000000001,-0.805000000000001,-0.800000000000001,
-0.795000000000001,-0.790000000000001,-0.785000000000001,-0.780000000000001,
-0.775000000000001,-0.770000000000001,-0.765000000000001,-0.760000000000001,
-0.755000000000001,-0.750000000000001,-0.745000000000001,-0.740000000000001,
-0.735000000000001,-0.730000000000001,-0.725000000000001,-0.720000000000001,
-0.715000000000001,-0.710000000000001,-0.705000000000001,-0.700000000000001,
-0.695000000000001,-0.690000000000001,-0.685,-0.68,-0.675,-0.67,-0.665,
-0.66,-0.655,-0.65,-0.645,-0.64,-0.635,-0.63,-0.625,-0.62,-0.615,-0.61,
-0.605,-0.6,-0.595,-0.59,-0.585,-0.58,-0.575,-0.57,-0.565,-0.56,-0.555,
-0.55,-0.545,-0.54,-0.535,-0.53,-0.525,-0.52,-0.515,-0.51,-0.505,-0.5,-0.495,
-0.49,-0.485,-0.48,-0.475,-0.47,-0.465,-0.46,-0.455,-0.45,-0.445,-0.44,
-0.435,-0.43,-0.425,-0.42,-0.415,-0.41,-0.405,-0.4,-0.395,-0.39,-0.385,
-0.38,-0.375,-0.37,-0.365,-0.36,-0.355,-0.35,-0.345,-0.34,-0.335,-0.33,
-0.325,-0.32,-0.315,-0.31,-0.305,-0.3,-0.295,-0.29,-0.285,-0.28,-0.275,
-0.27,-0.265,-0.26,-0.255,-0.25,-0.245,-0.24,-0.235,-0.23,-0.225,-0.22,
-0.215,-0.21,-0.205,-0.2,-0.195,-0.19,-0.185,-0.18,-0.175,-0.17,-0.165,
-0.16,-0.155,-0.15,-0.145,-0.14,-0.135,-0.13,-0.125,-0.12,-0.115,-0.11,
-0.105,-0.1,-0.095,-0.09,-0.085,-0.08,-0.075,-0.07,-0.065,-0.06,-0.055,
-0.05,-0.045,-0.04,-0.035,-0.03,-0.025,-0.02,-0.015,-0.01,-0.005,0.),
 .UNSPECIFIED.)
CURVE()
GEOMETRIC_REPRESENTATION_ITEM()
RATIONAL_B_SPLINE_CURVE((1.,1.,1.,1.,1.,1.,1.,1.,1.,1.,1.,1.,1.,1.,1.,1.,
1.,1.,1.,1.,1.,1.,1.,1.,1.,1.,1.,1.,1.,1.,1.,1.,1.,1.,1.,1.,1.,1.,1.,1.,
1.,1.,1.,1.,1.,1.,1.,1.,1.,1.,1.,1.,1.,1.,1.,1.,1.,1.,1.,1.,1.,1.,1.,1.,
1.,1.,1.,1.,1.,1.,1.,1.,1.,1.,1.,1.,1.,1.,1.,1.,1.,1.,1.,1.,1.,1.,1.,1.,
1.,1.,1.,1.,1.,1.,1.,1.,1.,1.,1.,1.,1.,1.,1.,1.,1.,1.,1.,1.,1.,1.,1.,1.,
1.,1.,1.,1.,1.,1.,1.,1.,1.,1.,1.,1.,1.,1.,1.,1.,1.,1.,1.,1.,1.,1.,1.,1.,
1.,1.,1.,1.,1.,1.,1.,1.,1.,1.,1.,1.,1.,1.,1.,1.,1.,1.,1.,1.,1.,1.,1.,1.,
1.,1.,1.,1.,1.,1.,1.,1.,1.,1.,1.,1.,1.,1.,1.,1.,1.,1.,1.,1.,1.,1.,1.,1.,
1.,1.,1.,1.,1.,1.,1.,1.,1.,1.))
REPRESENTATION_ITEM('')
);
#649=(
BOUNDED_CURVE()
B_SPLINE_CURVE(5,(#158255,#158256,#158257,#158258,#158259,#158260,#158261,
#158262,#158263,#158264,#158265,#158266,#158267,#158268,#158269,#158270,
#158271,#158272,#158273,#158274,#158275,#158276,#158277,#158278,#158279,
#158280,#158281,#158282,#158283,#158284,#158285,#158286,#158287,#158288,
#158289,#158290,#158291,#158292,#158293,#158294,#158295,#158296,#158297,
#158298,#158299,#158300,#158301,#158302,#158303,#158304,#158305,#158306,
#158307,#158308,#158309,#158310,#158311,#158312,#158313,#158314,#158315,
#158316,#158317,#158318,#158319,#158320,#158321,#158322,#158323,#158324,
#158325,#158326,#158327,#158328,#158329,#158330,#158331,#158332,#158333,
#158334,#158335,#158336,#158337,#158338,#158339,#158340,#158341,#158342,
#158343,#158344,#158345,#158346,#158347,#158348,#158349,#158350,#158351,
#158352,#158353,#158354,#158355,#158356,#158357,#158358,#158359,#158360,
#158361,#158362,#158363,#158364,#158365,#158366,#158367,#158368,#158369,
#158370,#158371,#158372,#158373,#158374,#158375,#158376,#158377,#158378,
#158379,#158380,#158381,#158382,#158383,#158384,#158385,#158386,#158387,
#158388,#158389,#158390,#158391,#158392,#158393,#158394,#158395,#158396,
#158397,#158398,#158399,#158400,#158401,#158402,#158403,#158404,#158405,
#158406,#158407,#158408,#158409,#158410,#158411,#158412,#158413,#158414,
#158415,#158416,#158417,#158418,#158419,#158420,#158421,#158422,#158423,
#158424,#158425,#158426,#158427,#158428,#158429,#158430,#158431,#158432,
#158433,#158434,#158435,#158436,#158437,#158438,#158439,#158440,#158441,
#158442,#158443,#158444,#158445,#158446,#158447,#158448),.UNSPECIFIED.,
 .F.,.F.)
B_SPLINE_CURVE_WITH_KNOTS((6,1,1,1,1,1,1,1,1,1,1,1,1,1,1,1,1,1,1,1,1,1,
1,1,1,1,1,1,1,1,1,1,1,1,1,1,1,1,1,1,1,1,1,1,1,1,1,1,1,1,1,1,1,1,1,1,1,1,
1,1,1,1,1,1,1,1,1,1,1,1,1,1,1,1,1,1,1,1,1,1,1,1,1,1,1,1,1,1,1,1,1,1,1,1,
1,1,1,1,1,1,1,1,1,1,1,1,1,1,1,1,1,1,1,1,1,1,1,1,1,1,1,1,1,1,1,1,1,1,1,1,
1,1,1,1,1,1,1,1,1,1,1,1,1,1,1,1,1,1,1,1,1,1,1,1,1,1,1,1,1,1,1,1,1,1,1,1,
1,1,1,1,1,1,1,1,1,1,1,1,1,1,1,1,1,1,1,1,1,1,1,6),(0.,0.005,0.01,0.015,0.02,
0.025,0.03,0.035,0.04,0.045,0.05,0.055,0.06,0.065,0.07,0.075,0.08,0.085,
0.09,0.095,0.1,0.105,0.11,0.115,0.12,0.125,0.13,0.135,0.14,0.145,0.15,0.155,
0.16,0.165,0.17,0.175,0.18,0.185,0.19,0.195,0.2,0.205,0.21,0.215,0.22,0.225,
0.23,0.235,0.24,0.245,0.25,0.255,0.26,0.265,0.27,0.275,0.28,0.285,0.29,
0.295,0.3,0.305,0.31,0.315,0.32,0.325,0.33,0.335,0.34,0.345,0.35,0.355,
0.36,0.365,0.37,0.375,0.38,0.385,0.39,0.395,0.4,0.405,0.41,0.415,0.42,0.425,
0.43,0.435,0.44,0.445,0.45,0.455,0.46,0.465,0.47,0.475,0.48,0.485,0.49,
0.495,0.5,0.505,0.51,0.515,0.52,0.525,0.53,0.535,0.54,0.545,0.55,0.555,
0.56,0.565,0.57,0.575,0.58,0.585,0.59,0.595,0.6,0.605,0.61,0.615,0.62,0.625,
0.63,0.635,0.64,0.645,0.65,0.655,0.66,0.665,0.67,0.675,0.68,0.685,0.690000000000001,
0.695000000000001,0.700000000000001,0.705000000000001,0.710000000000001,
0.715000000000001,0.720000000000001,0.725000000000001,0.730000000000001,
0.735000000000001,0.740000000000001,0.745000000000001,0.750000000000001,
0.755000000000001,0.760000000000001,0.765000000000001,0.770000000000001,
0.775000000000001,0.780000000000001,0.785000000000001,0.790000000000001,
0.795000000000001,0.800000000000001,0.805000000000001,0.810000000000001,
0.815000000000001,0.820000000000001,0.825000000000001,0.830000000000001,
0.835000000000001,0.840000000000001,0.845000000000001,0.850000000000001,
0.855000000000001,0.860000000000001,0.865000000000001,0.870000000000001,
0.875000000000001,0.880000000000001,0.885000000000001,0.890000000000001,
0.895000000000001,0.900000000000001,0.905000000000001,0.910000000000001,
0.915000000000001,0.920000000000001,0.925000000000001,0.930000000000001,
0.935000000000001,0.940000000000001,0.94142984443803),.UNSPECIFIED.)
CURVE()
GEOMETRIC_REPRESENTATION_ITEM()
RATIONAL_B_SPLINE_CURVE((1.,1.,1.,1.,1.,1.,1.,1.,1.,1.,1.,1.,1.,1.,1.,1.,
1.,1.,1.,1.,1.,1.,1.,1.,1.,1.,1.,1.,1.,1.,1.,1.,1.,1.,1.,1.,1.,1.,1.,1.,
1.,1.,1.,1.,1.,1.,1.,1.,1.,1.,1.,1.,1.,1.,1.,1.,1.,1.,1.,1.,1.,1.,1.,1.,
1.,1.,1.,1.,1.,1.,1.,1.,1.,1.,1.,1.,1.,1.,1.,1.,1.,1.,1.,1.,1.,1.,1.,1.,
1.,1.,1.,1.,1.,1.,1.,1.,1.,1.,1.,1.,1.,1.,1.,1.,1.,1.,1.,1.,1.,1.,1.,1.,
1.,1.,1.,1.,1.,1.,1.,1.,1.,1.,1.,1.,1.,1.,1.,1.,1.,1.,1.,1.,1.,1.,1.,1.,
1.,1.,1.,1.,1.,1.,1.,1.,1.,1.,1.,1.,1.,1.,1.,1.,1.,1.,1.,1.,1.,1.,1.,1.,
1.,1.,1.,1.,1.,1.,1.,1.,1.,1.,1.,1.,1.,1.,1.,1.,1.,1.,1.,1.,1.,1.,1.,1.,
1.,1.,1.,1.,1.,1.,1.,1.,1.,1.))
REPRESENTATION_ITEM('')
);
#650=(
BOUNDED_CURVE()
B_SPLINE_CURVE(5,(#158451,#158452,#158453,#158454,#158455,#158456,#158457,
#158458,#158459,#158460,#158461,#158462,#158463,#158464,#158465,#158466,
#158467,#158468,#158469,#158470,#158471,#158472,#158473,#158474,#158475,
#158476,#158477,#158478,#158479,#158480,#158481,#158482,#158483,#158484,
#158485,#158486,#158487,#158488,#158489,#158490,#158491,#158492,#158493,
#158494,#158495,#158496,#158497,#158498,#158499,#158500,#158501,#158502,
#158503,#158504,#158505,#158506,#158507,#158508,#158509,#158510,#158511,
#158512,#158513,#158514,#158515,#158516,#158517,#158518,#158519,#158520,
#158521,#158522,#158523,#158524,#158525,#158526,#158527,#158528,#158529,
#158530,#158531,#158532,#158533,#158534,#158535,#158536,#158537,#158538,
#158539,#158540,#158541,#158542,#158543,#158544,#158545,#158546,#158547,
#158548,#158549,#158550,#158551,#158552,#158553,#158554,#158555,#158556,
#158557,#158558,#158559,#158560,#158561,#158562,#158563,#158564,#158565,
#158566,#158567,#158568,#158569,#158570,#158571,#158572,#158573,#158574,
#158575,#158576,#158577,#158578,#158579,#158580,#158581,#158582,#158583,
#158584,#158585,#158586,#158587,#158588,#158589,#158590,#158591,#158592,
#158593,#158594,#158595,#158596,#158597,#158598,#158599,#158600,#158601,
#158602,#158603,#158604,#158605,#158606,#158607,#158608,#158609,#158610,
#158611,#158612,#158613,#158614,#158615,#158616,#158617,#158618,#158619,
#158620,#158621,#158622,#158623,#158624,#158625,#158626,#158627,#158628,
#158629,#158630,#158631,#158632,#158633,#158634,#158635,#158636,#158637,
#158638,#158639,#158640,#158641,#158642,#158643,#158644),.UNSPECIFIED.,
 .F.,.F.)
B_SPLINE_CURVE_WITH_KNOTS((6,1,1,1,1,1,1,1,1,1,1,1,1,1,1,1,1,1,1,1,1,1,
1,1,1,1,1,1,1,1,1,1,1,1,1,1,1,1,1,1,1,1,1,1,1,1,1,1,1,1,1,1,1,1,1,1,1,1,
1,1,1,1,1,1,1,1,1,1,1,1,1,1,1,1,1,1,1,1,1,1,1,1,1,1,1,1,1,1,1,1,1,1,1,1,
1,1,1,1,1,1,1,1,1,1,1,1,1,1,1,1,1,1,1,1,1,1,1,1,1,1,1,1,1,1,1,1,1,1,1,1,
1,1,1,1,1,1,1,1,1,1,1,1,1,1,1,1,1,1,1,1,1,1,1,1,1,1,1,1,1,1,1,1,1,1,1,1,
1,1,1,1,1,1,1,1,1,1,1,1,1,1,1,1,1,1,1,1,1,1,1,6),(-0.94142984443803,-0.940000000000001,
-0.935000000000001,-0.930000000000001,-0.925000000000001,-0.920000000000001,
-0.915000000000001,-0.910000000000001,-0.905000000000001,-0.900000000000001,
-0.895000000000001,-0.890000000000001,-0.885000000000001,-0.880000000000001,
-0.875000000000001,-0.870000000000001,-0.865000000000001,-0.860000000000001,
-0.855000000000001,-0.850000000000001,-0.845000000000001,-0.840000000000001,
-0.835000000000001,-0.830000000000001,-0.825000000000001,-0.820000000000001,
-0.815000000000001,-0.810000000000001,-0.805000000000001,-0.800000000000001,
-0.795000000000001,-0.790000000000001,-0.785000000000001,-0.780000000000001,
-0.775000000000001,-0.770000000000001,-0.765000000000001,-0.760000000000001,
-0.755000000000001,-0.750000000000001,-0.745000000000001,-0.740000000000001,
-0.735000000000001,-0.730000000000001,-0.725000000000001,-0.720000000000001,
-0.715000000000001,-0.710000000000001,-0.705000000000001,-0.700000000000001,
-0.695000000000001,-0.690000000000001,-0.685,-0.68,-0.675,-0.67,-0.665,
-0.66,-0.655,-0.65,-0.645,-0.64,-0.635,-0.63,-0.625,-0.62,-0.615,-0.61,
-0.605,-0.6,-0.595,-0.59,-0.585,-0.58,-0.575,-0.57,-0.565,-0.56,-0.555,
-0.55,-0.545,-0.54,-0.535,-0.53,-0.525,-0.52,-0.515,-0.51,-0.505,-0.5,-0.495,
-0.49,-0.485,-0.48,-0.475,-0.47,-0.465,-0.46,-0.455,-0.45,-0.445,-0.44,
-0.435,-0.43,-0.425,-0.42,-0.415,-0.41,-0.405,-0.4,-0.395,-0.39,-0.385,
-0.38,-0.375,-0.37,-0.365,-0.36,-0.355,-0.35,-0.345,-0.34,-0.335,-0.33,
-0.325,-0.32,-0.315,-0.31,-0.305,-0.3,-0.295,-0.29,-0.285,-0.28,-0.275,
-0.27,-0.265,-0.26,-0.255,-0.25,-0.245,-0.24,-0.235,-0.23,-0.225,-0.22,
-0.215,-0.21,-0.205,-0.2,-0.195,-0.19,-0.185,-0.18,-0.175,-0.17,-0.165,
-0.16,-0.155,-0.15,-0.145,-0.14,-0.135,-0.13,-0.125,-0.12,-0.115,-0.11,
-0.105,-0.1,-0.095,-0.09,-0.085,-0.08,-0.075,-0.07,-0.065,-0.06,-0.055,
-0.05,-0.045,-0.04,-0.035,-0.03,-0.025,-0.02,-0.015,-0.01,-0.005,0.),
 .UNSPECIFIED.)
CURVE()
GEOMETRIC_REPRESENTATION_ITEM()
RATIONAL_B_SPLINE_CURVE((1.,1.,1.,1.,1.,1.,1.,1.,1.,1.,1.,1.,1.,1.,1.,1.,
1.,1.,1.,1.,1.,1.,1.,1.,1.,1.,1.,1.,1.,1.,1.,1.,1.,1.,1.,1.,1.,1.,1.,1.,
1.,1.,1.,1.,1.,1.,1.,1.,1.,1.,1.,1.,1.,1.,1.,1.,1.,1.,1.,1.,1.,1.,1.,1.,
1.,1.,1.,1.,1.,1.,1.,1.,1.,1.,1.,1.,1.,1.,1.,1.,1.,1.,1.,1.,1.,1.,1.,1.,
1.,1.,1.,1.,1.,1.,1.,1.,1.,1.,1.,1.,1.,1.,1.,1.,1.,1.,1.,1.,1.,1.,1.,1.,
1.,1.,1.,1.,1.,1.,1.,1.,1.,1.,1.,1.,1.,1.,1.,1.,1.,1.,1.,1.,1.,1.,1.,1.,
1.,1.,1.,1.,1.,1.,1.,1.,1.,1.,1.,1.,1.,1.,1.,1.,1.,1.,1.,1.,1.,1.,1.,1.,
1.,1.,1.,1.,1.,1.,1.,1.,1.,1.,1.,1.,1.,1.,1.,1.,1.,1.,1.,1.,1.,1.,1.,1.,
1.,1.,1.,1.,1.,1.,1.,1.,1.,1.))
REPRESENTATION_ITEM('')
);
#651=(
BOUNDED_CURVE()
B_SPLINE_CURVE(5,(#159056,#159057,#159058,#159059,#159060,#159061,#159062,
#159063,#159064,#159065,#159066,#159067,#159068,#159069,#159070,#159071,
#159072,#159073,#159074,#159075,#159076,#159077,#159078,#159079,#159080,
#159081,#159082,#159083,#159084,#159085,#159086,#159087,#159088,#159089,
#159090,#159091,#159092,#159093,#159094,#159095,#159096,#159097,#159098,
#159099,#159100,#159101,#159102,#159103,#159104,#159105,#159106,#159107,
#159108,#159109,#159110,#159111,#159112,#159113,#159114,#159115,#159116,
#159117,#159118,#159119,#159120,#159121,#159122,#159123,#159124,#159125,
#159126,#159127,#159128,#159129,#159130,#159131,#159132,#159133,#159134,
#159135,#159136,#159137,#159138,#159139,#159140,#159141,#159142,#159143,
#159144,#159145,#159146,#159147,#159148,#159149,#159150,#159151,#159152,
#159153,#159154,#159155,#159156,#159157,#159158,#159159,#159160,#159161,
#159162,#159163,#159164,#159165,#159166,#159167,#159168,#159169,#159170,
#159171,#159172,#159173,#159174,#159175,#159176,#159177,#159178,#159179,
#159180,#159181,#159182,#159183,#159184,#159185,#159186,#159187,#159188,
#159189,#159190,#159191,#159192,#159193,#159194,#159195,#159196,#159197,
#159198,#159199,#159200,#159201,#159202,#159203,#159204,#159205,#159206,
#159207,#159208,#159209,#159210,#159211,#159212,#159213,#159214,#159215,
#159216,#159217,#159218,#159219,#159220,#159221,#159222,#159223,#159224,
#159225,#159226,#159227,#159228,#159229,#159230,#159231,#159232,#159233,
#159234,#159235,#159236,#159237,#159238,#159239,#159240,#159241,#159242,
#159243,#159244,#159245,#159246,#159247,#159248,#159249),.UNSPECIFIED.,
 .F.,.F.)
B_SPLINE_CURVE_WITH_KNOTS((6,1,1,1,1,1,1,1,1,1,1,1,1,1,1,1,1,1,1,1,1,1,
1,1,1,1,1,1,1,1,1,1,1,1,1,1,1,1,1,1,1,1,1,1,1,1,1,1,1,1,1,1,1,1,1,1,1,1,
1,1,1,1,1,1,1,1,1,1,1,1,1,1,1,1,1,1,1,1,1,1,1,1,1,1,1,1,1,1,1,1,1,1,1,1,
1,1,1,1,1,1,1,1,1,1,1,1,1,1,1,1,1,1,1,1,1,1,1,1,1,1,1,1,1,1,1,1,1,1,1,1,
1,1,1,1,1,1,1,1,1,1,1,1,1,1,1,1,1,1,1,1,1,1,1,1,1,1,1,1,1,1,1,1,1,1,1,1,
1,1,1,1,1,1,1,1,1,1,1,1,1,1,1,1,1,1,1,1,1,1,1,6),(0.,0.005,0.01,0.015,0.02,
0.025,0.03,0.035,0.04,0.045,0.05,0.055,0.06,0.065,0.07,0.075,0.08,0.085,
0.09,0.095,0.1,0.105,0.11,0.115,0.12,0.125,0.13,0.135,0.14,0.145,0.15,0.155,
0.16,0.165,0.17,0.175,0.18,0.185,0.19,0.195,0.2,0.205,0.21,0.215,0.22,0.225,
0.23,0.235,0.24,0.245,0.25,0.255,0.26,0.265,0.27,0.275,0.28,0.285,0.29,
0.295,0.3,0.305,0.31,0.315,0.32,0.325,0.33,0.335,0.34,0.345,0.35,0.355,
0.36,0.365,0.37,0.375,0.38,0.385,0.39,0.395,0.4,0.405,0.41,0.415,0.42,0.425,
0.43,0.435,0.44,0.445,0.45,0.455,0.46,0.465,0.47,0.475,0.48,0.485,0.49,
0.495,0.5,0.505,0.51,0.515,0.52,0.525,0.53,0.535,0.54,0.545,0.55,0.555,
0.56,0.565,0.57,0.575,0.58,0.585,0.59,0.595,0.6,0.605,0.61,0.615,0.62,0.625,
0.63,0.635,0.64,0.645,0.65,0.655,0.66,0.665,0.67,0.675,0.68,0.685,0.690000000000001,
0.695000000000001,0.700000000000001,0.705000000000001,0.710000000000001,
0.715000000000001,0.720000000000001,0.725000000000001,0.730000000000001,
0.735000000000001,0.740000000000001,0.745000000000001,0.750000000000001,
0.755000000000001,0.760000000000001,0.765000000000001,0.770000000000001,
0.775000000000001,0.780000000000001,0.785000000000001,0.790000000000001,
0.795000000000001,0.800000000000001,0.805000000000001,0.810000000000001,
0.815000000000001,0.820000000000001,0.825000000000001,0.830000000000001,
0.835000000000001,0.840000000000001,0.845000000000001,0.850000000000001,
0.855000000000001,0.860000000000001,0.865000000000001,0.870000000000001,
0.875000000000001,0.880000000000001,0.885000000000001,0.890000000000001,
0.895000000000001,0.900000000000001,0.905000000000001,0.910000000000001,
0.915000000000001,0.920000000000001,0.925000000000001,0.930000000000001,
0.935000000000001,0.940000000000001,0.94142984443804),.UNSPECIFIED.)
CURVE()
GEOMETRIC_REPRESENTATION_ITEM()
RATIONAL_B_SPLINE_CURVE((1.,1.,1.,1.,1.,1.,1.,1.,1.,1.,1.,1.,1.,1.,1.,1.,
1.,1.,1.,1.,1.,1.,1.,1.,1.,1.,1.,1.,1.,1.,1.,1.,1.,1.,1.,1.,1.,1.,1.,1.,
1.,1.,1.,1.,1.,1.,1.,1.,1.,1.,1.,1.,1.,1.,1.,1.,1.,1.,1.,1.,1.,1.,1.,1.,
1.,1.,1.,1.,1.,1.,1.,1.,1.,1.,1.,1.,1.,1.,1.,1.,1.,1.,1.,1.,1.,1.,1.,1.,
1.,1.,1.,1.,1.,1.,1.,1.,1.,1.,1.,1.,1.,1.,1.,1.,1.,1.,1.,1.,1.,1.,1.,1.,
1.,1.,1.,1.,1.,1.,1.,1.,1.,1.,1.,1.,1.,1.,1.,1.,1.,1.,1.,1.,1.,1.,1.,1.,
1.,1.,1.,1.,1.,1.,1.,1.,1.,1.,1.,1.,1.,1.,1.,1.,1.,1.,1.,1.,1.,1.,1.,1.,
1.,1.,1.,1.,1.,1.,1.,1.,1.,1.,1.,1.,1.,1.,1.,1.,1.,1.,1.,1.,1.,1.,1.,1.,
1.,1.,1.,1.,1.,1.,1.,1.,1.,1.))
REPRESENTATION_ITEM('')
);
#652=(
BOUNDED_CURVE()
B_SPLINE_CURVE(5,(#159252,#159253,#159254,#159255,#159256,#159257,#159258,
#159259,#159260,#159261,#159262,#159263,#159264,#159265,#159266,#159267,
#159268,#159269,#159270,#159271,#159272,#159273,#159274,#159275,#159276,
#159277,#159278,#159279,#159280,#159281,#159282,#159283,#159284,#159285,
#159286,#159287,#159288,#159289,#159290,#159291,#159292,#159293,#159294,
#159295,#159296,#159297,#159298,#159299,#159300,#159301,#159302,#159303,
#159304,#159305,#159306,#159307,#159308,#159309,#159310,#159311,#159312,
#159313,#159314,#159315,#159316,#159317,#159318,#159319,#159320,#159321,
#159322,#159323,#159324,#159325,#159326,#159327,#159328,#159329,#159330,
#159331,#159332,#159333,#159334,#159335,#159336,#159337,#159338,#159339,
#159340,#159341,#159342,#159343,#159344,#159345,#159346,#159347,#159348,
#159349,#159350,#159351,#159352,#159353,#159354,#159355,#159356,#159357,
#159358,#159359,#159360,#159361,#159362,#159363,#159364,#159365,#159366,
#159367,#159368,#159369,#159370,#159371,#159372,#159373,#159374,#159375,
#159376,#159377,#159378,#159379,#159380,#159381,#159382,#159383,#159384,
#159385,#159386,#159387,#159388,#159389,#159390,#159391,#159392,#159393,
#159394,#159395,#159396,#159397,#159398,#159399,#159400,#159401,#159402,
#159403,#159404,#159405,#159406,#159407,#159408,#159409,#159410,#159411,
#159412,#159413,#159414,#159415,#159416,#159417,#159418,#159419,#159420,
#159421,#159422,#159423,#159424,#159425,#159426,#159427,#159428,#159429,
#159430,#159431,#159432,#159433,#159434,#159435,#159436,#159437,#159438,
#159439,#159440,#159441,#159442,#159443,#159444,#159445),.UNSPECIFIED.,
 .F.,.F.)
B_SPLINE_CURVE_WITH_KNOTS((6,1,1,1,1,1,1,1,1,1,1,1,1,1,1,1,1,1,1,1,1,1,
1,1,1,1,1,1,1,1,1,1,1,1,1,1,1,1,1,1,1,1,1,1,1,1,1,1,1,1,1,1,1,1,1,1,1,1,
1,1,1,1,1,1,1,1,1,1,1,1,1,1,1,1,1,1,1,1,1,1,1,1,1,1,1,1,1,1,1,1,1,1,1,1,
1,1,1,1,1,1,1,1,1,1,1,1,1,1,1,1,1,1,1,1,1,1,1,1,1,1,1,1,1,1,1,1,1,1,1,1,
1,1,1,1,1,1,1,1,1,1,1,1,1,1,1,1,1,1,1,1,1,1,1,1,1,1,1,1,1,1,1,1,1,1,1,1,
1,1,1,1,1,1,1,1,1,1,1,1,1,1,1,1,1,1,1,1,1,1,1,6),(-0.941429844438064,-0.940000000000001,
-0.935000000000001,-0.930000000000001,-0.925000000000001,-0.920000000000001,
-0.915000000000001,-0.910000000000001,-0.905000000000001,-0.900000000000001,
-0.895000000000001,-0.890000000000001,-0.885000000000001,-0.880000000000001,
-0.875000000000001,-0.870000000000001,-0.865000000000001,-0.860000000000001,
-0.855000000000001,-0.850000000000001,-0.845000000000001,-0.840000000000001,
-0.835000000000001,-0.830000000000001,-0.825000000000001,-0.820000000000001,
-0.815000000000001,-0.810000000000001,-0.805000000000001,-0.800000000000001,
-0.795000000000001,-0.790000000000001,-0.785000000000001,-0.780000000000001,
-0.775000000000001,-0.770000000000001,-0.765000000000001,-0.760000000000001,
-0.755000000000001,-0.750000000000001,-0.745000000000001,-0.740000000000001,
-0.735000000000001,-0.730000000000001,-0.725000000000001,-0.720000000000001,
-0.715000000000001,-0.710000000000001,-0.705000000000001,-0.700000000000001,
-0.695000000000001,-0.690000000000001,-0.685,-0.68,-0.675,-0.67,-0.665,
-0.66,-0.655,-0.65,-0.645,-0.64,-0.635,-0.63,-0.625,-0.62,-0.615,-0.61,
-0.605,-0.6,-0.595,-0.59,-0.585,-0.58,-0.575,-0.57,-0.565,-0.56,-0.555,
-0.55,-0.545,-0.54,-0.535,-0.53,-0.525,-0.52,-0.515,-0.51,-0.505,-0.5,-0.495,
-0.49,-0.485,-0.48,-0.475,-0.47,-0.465,-0.46,-0.455,-0.45,-0.445,-0.44,
-0.435,-0.43,-0.425,-0.42,-0.415,-0.41,-0.405,-0.4,-0.395,-0.39,-0.385,
-0.38,-0.375,-0.37,-0.365,-0.36,-0.355,-0.35,-0.345,-0.34,-0.335,-0.33,
-0.325,-0.32,-0.315,-0.31,-0.305,-0.3,-0.295,-0.29,-0.285,-0.28,-0.275,
-0.27,-0.265,-0.26,-0.255,-0.25,-0.245,-0.24,-0.235,-0.23,-0.225,-0.22,
-0.215,-0.21,-0.205,-0.2,-0.195,-0.19,-0.185,-0.18,-0.175,-0.17,-0.165,
-0.16,-0.155,-0.15,-0.145,-0.14,-0.135,-0.13,-0.125,-0.12,-0.115,-0.11,
-0.105,-0.1,-0.095,-0.09,-0.085,-0.08,-0.075,-0.07,-0.065,-0.06,-0.055,
-0.05,-0.045,-0.04,-0.035,-0.03,-0.025,-0.02,-0.015,-0.01,-0.005,0.),
 .UNSPECIFIED.)
CURVE()
GEOMETRIC_REPRESENTATION_ITEM()
RATIONAL_B_SPLINE_CURVE((1.,1.,1.,1.,1.,1.,1.,1.,1.,1.,1.,1.,1.,1.,1.,1.,
1.,1.,1.,1.,1.,1.,1.,1.,1.,1.,1.,1.,1.,1.,1.,1.,1.,1.,1.,1.,1.,1.,1.,1.,
1.,1.,1.,1.,1.,1.,1.,1.,1.,1.,1.,1.,1.,1.,1.,1.,1.,1.,1.,1.,1.,1.,1.,1.,
1.,1.,1.,1.,1.,1.,1.,1.,1.,1.,1.,1.,1.,1.,1.,1.,1.,1.,1.,1.,1.,1.,1.,1.,
1.,1.,1.,1.,1.,1.,1.,1.,1.,1.,1.,1.,1.,1.,1.,1.,1.,1.,1.,1.,1.,1.,1.,1.,
1.,1.,1.,1.,1.,1.,1.,1.,1.,1.,1.,1.,1.,1.,1.,1.,1.,1.,1.,1.,1.,1.,1.,1.,
1.,1.,1.,1.,1.,1.,1.,1.,1.,1.,1.,1.,1.,1.,1.,1.,1.,1.,1.,1.,1.,1.,1.,1.,
1.,1.,1.,1.,1.,1.,1.,1.,1.,1.,1.,1.,1.,1.,1.,1.,1.,1.,1.,1.,1.,1.,1.,1.,
1.,1.,1.,1.,1.,1.,1.,1.,1.,1.))
REPRESENTATION_ITEM('')
);
#653=(
BOUNDED_CURVE()
B_SPLINE_CURVE(5,(#159857,#159858,#159859,#159860,#159861,#159862,#159863,
#159864,#159865,#159866,#159867,#159868,#159869,#159870,#159871,#159872,
#159873,#159874,#159875,#159876,#159877,#159878,#159879,#159880,#159881,
#159882,#159883,#159884,#159885,#159886,#159887,#159888,#159889,#159890,
#159891,#159892,#159893,#159894,#159895,#159896,#159897,#159898,#159899,
#159900,#159901,#159902,#159903,#159904,#159905,#159906,#159907,#159908,
#159909,#159910,#159911,#159912,#159913,#159914,#159915,#159916,#159917,
#159918,#159919,#159920,#159921,#159922,#159923,#159924,#159925,#159926,
#159927,#159928,#159929,#159930,#159931,#159932,#159933,#159934,#159935,
#159936,#159937,#159938,#159939,#159940,#159941,#159942,#159943,#159944,
#159945,#159946,#159947,#159948,#159949,#159950,#159951,#159952,#159953,
#159954,#159955,#159956,#159957,#159958,#159959,#159960,#159961,#159962,
#159963,#159964,#159965,#159966,#159967,#159968,#159969,#159970,#159971,
#159972,#159973,#159974,#159975,#159976,#159977,#159978,#159979,#159980,
#159981,#159982,#159983,#159984,#159985,#159986,#159987,#159988,#159989,
#159990,#159991,#159992,#159993,#159994,#159995,#159996,#159997,#159998,
#159999,#160000,#160001,#160002,#160003,#160004,#160005,#160006,#160007,
#160008,#160009,#160010,#160011,#160012,#160013,#160014,#160015,#160016,
#160017,#160018,#160019,#160020,#160021,#160022,#160023,#160024,#160025,
#160026,#160027,#160028,#160029,#160030,#160031,#160032,#160033,#160034,
#160035,#160036,#160037,#160038,#160039,#160040,#160041,#160042,#160043,
#160044,#160045,#160046,#160047,#160048,#160049,#160050),.UNSPECIFIED.,
 .F.,.F.)
B_SPLINE_CURVE_WITH_KNOTS((6,1,1,1,1,1,1,1,1,1,1,1,1,1,1,1,1,1,1,1,1,1,
1,1,1,1,1,1,1,1,1,1,1,1,1,1,1,1,1,1,1,1,1,1,1,1,1,1,1,1,1,1,1,1,1,1,1,1,
1,1,1,1,1,1,1,1,1,1,1,1,1,1,1,1,1,1,1,1,1,1,1,1,1,1,1,1,1,1,1,1,1,1,1,1,
1,1,1,1,1,1,1,1,1,1,1,1,1,1,1,1,1,1,1,1,1,1,1,1,1,1,1,1,1,1,1,1,1,1,1,1,
1,1,1,1,1,1,1,1,1,1,1,1,1,1,1,1,1,1,1,1,1,1,1,1,1,1,1,1,1,1,1,1,1,1,1,1,
1,1,1,1,1,1,1,1,1,1,1,1,1,1,1,1,1,1,1,1,1,1,1,6),(0.,0.005,0.01,0.015,0.02,
0.025,0.03,0.035,0.04,0.045,0.05,0.055,0.06,0.065,0.07,0.075,0.08,0.085,
0.09,0.095,0.1,0.105,0.11,0.115,0.12,0.125,0.13,0.135,0.14,0.145,0.15,0.155,
0.16,0.165,0.17,0.175,0.18,0.185,0.19,0.195,0.2,0.205,0.21,0.215,0.22,0.225,
0.23,0.235,0.24,0.245,0.25,0.255,0.26,0.265,0.27,0.275,0.28,0.285,0.29,
0.295,0.3,0.305,0.31,0.315,0.32,0.325,0.33,0.335,0.34,0.345,0.35,0.355,
0.36,0.365,0.37,0.375,0.38,0.385,0.39,0.395,0.4,0.405,0.41,0.415,0.42,0.425,
0.43,0.435,0.44,0.445,0.45,0.455,0.46,0.465,0.47,0.475,0.48,0.485,0.49,
0.495,0.5,0.505,0.51,0.515,0.52,0.525,0.53,0.535,0.54,0.545,0.55,0.555,
0.56,0.565,0.57,0.575,0.58,0.585,0.59,0.595,0.6,0.605,0.61,0.615,0.62,0.625,
0.63,0.635,0.64,0.645,0.65,0.655,0.66,0.665,0.67,0.675,0.68,0.685,0.690000000000001,
0.695000000000001,0.700000000000001,0.705000000000001,0.710000000000001,
0.715000000000001,0.720000000000001,0.725000000000001,0.730000000000001,
0.735000000000001,0.740000000000001,0.745000000000001,0.750000000000001,
0.755000000000001,0.760000000000001,0.765000000000001,0.770000000000001,
0.775000000000001,0.780000000000001,0.785000000000001,0.790000000000001,
0.795000000000001,0.800000000000001,0.805000000000001,0.810000000000001,
0.815000000000001,0.820000000000001,0.825000000000001,0.830000000000001,
0.835000000000001,0.840000000000001,0.845000000000001,0.850000000000001,
0.855000000000001,0.860000000000001,0.865000000000001,0.870000000000001,
0.875000000000001,0.880000000000001,0.885000000000001,0.890000000000001,
0.895000000000001,0.900000000000001,0.905000000000001,0.910000000000001,
0.915000000000001,0.920000000000001,0.925000000000001,0.930000000000001,
0.935000000000001,0.940000000000001,0.941429844438021),.UNSPECIFIED.)
CURVE()
GEOMETRIC_REPRESENTATION_ITEM()
RATIONAL_B_SPLINE_CURVE((1.,1.,1.,1.,1.,1.,1.,1.,1.,1.,1.,1.,1.,1.,1.,1.,
1.,1.,1.,1.,1.,1.,1.,1.,1.,1.,1.,1.,1.,1.,1.,1.,1.,1.,1.,1.,1.,1.,1.,1.,
1.,1.,1.,1.,1.,1.,1.,1.,1.,1.,1.,1.,1.,1.,1.,1.,1.,1.,1.,1.,1.,1.,1.,1.,
1.,1.,1.,1.,1.,1.,1.,1.,1.,1.,1.,1.,1.,1.,1.,1.,1.,1.,1.,1.,1.,1.,1.,1.,
1.,1.,1.,1.,1.,1.,1.,1.,1.,1.,1.,1.,1.,1.,1.,1.,1.,1.,1.,1.,1.,1.,1.,1.,
1.,1.,1.,1.,1.,1.,1.,1.,1.,1.,1.,1.,1.,1.,1.,1.,1.,1.,1.,1.,1.,1.,1.,1.,
1.,1.,1.,1.,1.,1.,1.,1.,1.,1.,1.,1.,1.,1.,1.,1.,1.,1.,1.,1.,1.,1.,1.,1.,
1.,1.,1.,1.,1.,1.,1.,1.,1.,1.,1.,1.,1.,1.,1.,1.,1.,1.,1.,1.,1.,1.,1.,1.,
1.,1.,1.,1.,1.,1.,1.,1.,1.,1.))
REPRESENTATION_ITEM('')
);
#654=(
BOUNDED_CURVE()
B_SPLINE_CURVE(5,(#160053,#160054,#160055,#160056,#160057,#160058,#160059,
#160060,#160061,#160062,#160063,#160064,#160065,#160066,#160067,#160068,
#160069,#160070,#160071,#160072,#160073,#160074,#160075,#160076,#160077,
#160078,#160079,#160080,#160081,#160082,#160083,#160084,#160085,#160086,
#160087,#160088,#160089,#160090,#160091,#160092,#160093,#160094,#160095,
#160096,#160097,#160098,#160099,#160100,#160101,#160102,#160103,#160104,
#160105,#160106,#160107,#160108,#160109,#160110,#160111,#160112,#160113,
#160114,#160115,#160116,#160117,#160118,#160119,#160120,#160121,#160122,
#160123,#160124,#160125,#160126,#160127,#160128,#160129,#160130,#160131,
#160132,#160133,#160134,#160135,#160136,#160137,#160138,#160139,#160140,
#160141,#160142,#160143,#160144,#160145,#160146,#160147,#160148,#160149,
#160150,#160151,#160152,#160153,#160154,#160155,#160156,#160157,#160158,
#160159,#160160,#160161,#160162,#160163,#160164,#160165,#160166,#160167,
#160168,#160169,#160170,#160171,#160172,#160173,#160174,#160175,#160176,
#160177,#160178,#160179,#160180,#160181,#160182,#160183,#160184,#160185,
#160186,#160187,#160188,#160189,#160190,#160191,#160192,#160193,#160194,
#160195,#160196,#160197,#160198,#160199,#160200,#160201,#160202,#160203,
#160204,#160205,#160206,#160207,#160208,#160209,#160210,#160211,#160212,
#160213,#160214,#160215,#160216,#160217,#160218,#160219,#160220,#160221,
#160222,#160223,#160224,#160225,#160226,#160227,#160228,#160229,#160230,
#160231,#160232,#160233,#160234,#160235,#160236,#160237,#160238,#160239,
#160240,#160241,#160242,#160243,#160244,#160245,#160246),.UNSPECIFIED.,
 .F.,.F.)
B_SPLINE_CURVE_WITH_KNOTS((6,1,1,1,1,1,1,1,1,1,1,1,1,1,1,1,1,1,1,1,1,1,
1,1,1,1,1,1,1,1,1,1,1,1,1,1,1,1,1,1,1,1,1,1,1,1,1,1,1,1,1,1,1,1,1,1,1,1,
1,1,1,1,1,1,1,1,1,1,1,1,1,1,1,1,1,1,1,1,1,1,1,1,1,1,1,1,1,1,1,1,1,1,1,1,
1,1,1,1,1,1,1,1,1,1,1,1,1,1,1,1,1,1,1,1,1,1,1,1,1,1,1,1,1,1,1,1,1,1,1,1,
1,1,1,1,1,1,1,1,1,1,1,1,1,1,1,1,1,1,1,1,1,1,1,1,1,1,1,1,1,1,1,1,1,1,1,1,
1,1,1,1,1,1,1,1,1,1,1,1,1,1,1,1,1,1,1,1,1,1,1,6),(-0.941429844438021,-0.940000000000001,
-0.935000000000001,-0.930000000000001,-0.925000000000001,-0.920000000000001,
-0.915000000000001,-0.910000000000001,-0.905000000000001,-0.900000000000001,
-0.895000000000001,-0.890000000000001,-0.885000000000001,-0.880000000000001,
-0.875000000000001,-0.870000000000001,-0.865000000000001,-0.860000000000001,
-0.855000000000001,-0.850000000000001,-0.845000000000001,-0.840000000000001,
-0.835000000000001,-0.830000000000001,-0.825000000000001,-0.820000000000001,
-0.815000000000001,-0.810000000000001,-0.805000000000001,-0.800000000000001,
-0.795000000000001,-0.790000000000001,-0.785000000000001,-0.780000000000001,
-0.775000000000001,-0.770000000000001,-0.765000000000001,-0.760000000000001,
-0.755000000000001,-0.750000000000001,-0.745000000000001,-0.740000000000001,
-0.735000000000001,-0.730000000000001,-0.725000000000001,-0.720000000000001,
-0.715000000000001,-0.710000000000001,-0.705000000000001,-0.700000000000001,
-0.695000000000001,-0.690000000000001,-0.685,-0.68,-0.675,-0.67,-0.665,
-0.66,-0.655,-0.65,-0.645,-0.64,-0.635,-0.63,-0.625,-0.62,-0.615,-0.61,
-0.605,-0.6,-0.595,-0.59,-0.585,-0.58,-0.575,-0.57,-0.565,-0.56,-0.555,
-0.55,-0.545,-0.54,-0.535,-0.53,-0.525,-0.52,-0.515,-0.51,-0.505,-0.5,-0.495,
-0.49,-0.485,-0.48,-0.475,-0.47,-0.465,-0.46,-0.455,-0.45,-0.445,-0.44,
-0.435,-0.43,-0.425,-0.42,-0.415,-0.41,-0.405,-0.4,-0.395,-0.39,-0.385,
-0.38,-0.375,-0.37,-0.365,-0.36,-0.355,-0.35,-0.345,-0.34,-0.335,-0.33,
-0.325,-0.32,-0.315,-0.31,-0.305,-0.3,-0.295,-0.29,-0.285,-0.28,-0.275,
-0.27,-0.265,-0.26,-0.255,-0.25,-0.245,-0.24,-0.235,-0.23,-0.225,-0.22,
-0.215,-0.21,-0.205,-0.2,-0.195,-0.19,-0.185,-0.18,-0.175,-0.17,-0.165,
-0.16,-0.155,-0.15,-0.145,-0.14,-0.135,-0.13,-0.125,-0.12,-0.115,-0.11,
-0.105,-0.1,-0.095,-0.09,-0.085,-0.08,-0.075,-0.07,-0.065,-0.06,-0.055,
-0.05,-0.045,-0.04,-0.035,-0.03,-0.025,-0.02,-0.015,-0.01,-0.005,0.),
 .UNSPECIFIED.)
CURVE()
GEOMETRIC_REPRESENTATION_ITEM()
RATIONAL_B_SPLINE_CURVE((1.,1.,1.,1.,1.,1.,1.,1.,1.,1.,1.,1.,1.,1.,1.,1.,
1.,1.,1.,1.,1.,1.,1.,1.,1.,1.,1.,1.,1.,1.,1.,1.,1.,1.,1.,1.,1.,1.,1.,1.,
1.,1.,1.,1.,1.,1.,1.,1.,1.,1.,1.,1.,1.,1.,1.,1.,1.,1.,1.,1.,1.,1.,1.,1.,
1.,1.,1.,1.,1.,1.,1.,1.,1.,1.,1.,1.,1.,1.,1.,1.,1.,1.,1.,1.,1.,1.,1.,1.,
1.,1.,1.,1.,1.,1.,1.,1.,1.,1.,1.,1.,1.,1.,1.,1.,1.,1.,1.,1.,1.,1.,1.,1.,
1.,1.,1.,1.,1.,1.,1.,1.,1.,1.,1.,1.,1.,1.,1.,1.,1.,1.,1.,1.,1.,1.,1.,1.,
1.,1.,1.,1.,1.,1.,1.,1.,1.,1.,1.,1.,1.,1.,1.,1.,1.,1.,1.,1.,1.,1.,1.,1.,
1.,1.,1.,1.,1.,1.,1.,1.,1.,1.,1.,1.,1.,1.,1.,1.,1.,1.,1.,1.,1.,1.,1.,1.,
1.,1.,1.,1.,1.,1.,1.,1.,1.,1.))
REPRESENTATION_ITEM('')
);
#655=(
BOUNDED_CURVE()
B_SPLINE_CURVE(5,(#160658,#160659,#160660,#160661,#160662,#160663,#160664,
#160665,#160666,#160667,#160668,#160669,#160670,#160671,#160672,#160673,
#160674,#160675,#160676,#160677,#160678,#160679,#160680,#160681,#160682,
#160683,#160684,#160685,#160686,#160687,#160688,#160689,#160690,#160691,
#160692,#160693,#160694,#160695,#160696,#160697,#160698,#160699,#160700,
#160701,#160702,#160703,#160704,#160705,#160706,#160707,#160708,#160709,
#160710,#160711,#160712,#160713,#160714,#160715,#160716,#160717,#160718,
#160719,#160720,#160721,#160722,#160723,#160724,#160725,#160726,#160727,
#160728,#160729,#160730,#160731,#160732,#160733,#160734,#160735,#160736,
#160737,#160738,#160739,#160740,#160741,#160742,#160743,#160744,#160745,
#160746,#160747,#160748,#160749,#160750,#160751,#160752,#160753,#160754,
#160755,#160756,#160757,#160758,#160759,#160760,#160761,#160762,#160763,
#160764,#160765,#160766,#160767,#160768,#160769,#160770,#160771,#160772,
#160773,#160774,#160775,#160776,#160777,#160778,#160779,#160780,#160781,
#160782,#160783,#160784,#160785,#160786,#160787,#160788,#160789,#160790,
#160791,#160792,#160793,#160794,#160795,#160796,#160797,#160798,#160799,
#160800,#160801,#160802,#160803,#160804,#160805,#160806,#160807,#160808,
#160809,#160810,#160811,#160812,#160813,#160814,#160815,#160816,#160817,
#160818,#160819,#160820,#160821,#160822,#160823,#160824,#160825,#160826,
#160827,#160828,#160829,#160830,#160831,#160832,#160833,#160834,#160835,
#160836,#160837,#160838,#160839,#160840,#160841,#160842,#160843,#160844,
#160845,#160846,#160847,#160848,#160849,#160850,#160851),.UNSPECIFIED.,
 .F.,.F.)
B_SPLINE_CURVE_WITH_KNOTS((6,1,1,1,1,1,1,1,1,1,1,1,1,1,1,1,1,1,1,1,1,1,
1,1,1,1,1,1,1,1,1,1,1,1,1,1,1,1,1,1,1,1,1,1,1,1,1,1,1,1,1,1,1,1,1,1,1,1,
1,1,1,1,1,1,1,1,1,1,1,1,1,1,1,1,1,1,1,1,1,1,1,1,1,1,1,1,1,1,1,1,1,1,1,1,
1,1,1,1,1,1,1,1,1,1,1,1,1,1,1,1,1,1,1,1,1,1,1,1,1,1,1,1,1,1,1,1,1,1,1,1,
1,1,1,1,1,1,1,1,1,1,1,1,1,1,1,1,1,1,1,1,1,1,1,1,1,1,1,1,1,1,1,1,1,1,1,1,
1,1,1,1,1,1,1,1,1,1,1,1,1,1,1,1,1,1,1,1,1,1,1,6),(0.,0.005,0.01,0.015,0.02,
0.025,0.03,0.035,0.04,0.045,0.05,0.055,0.06,0.065,0.07,0.075,0.08,0.085,
0.09,0.095,0.1,0.105,0.11,0.115,0.12,0.125,0.13,0.135,0.14,0.145,0.15,0.155,
0.16,0.165,0.17,0.175,0.18,0.185,0.19,0.195,0.2,0.205,0.21,0.215,0.22,0.225,
0.23,0.235,0.24,0.245,0.25,0.255,0.26,0.265,0.27,0.275,0.28,0.285,0.29,
0.295,0.3,0.305,0.31,0.315,0.32,0.325,0.33,0.335,0.34,0.345,0.35,0.355,
0.36,0.365,0.37,0.375,0.38,0.385,0.39,0.395,0.4,0.405,0.41,0.415,0.42,0.425,
0.43,0.435,0.44,0.445,0.45,0.455,0.46,0.465,0.47,0.475,0.48,0.485,0.49,
0.495,0.5,0.505,0.51,0.515,0.52,0.525,0.53,0.535,0.54,0.545,0.55,0.555,
0.56,0.565,0.57,0.575,0.58,0.585,0.59,0.595,0.6,0.605,0.61,0.615,0.62,0.625,
0.63,0.635,0.64,0.645,0.65,0.655,0.66,0.665,0.67,0.675,0.68,0.685,0.690000000000001,
0.695000000000001,0.700000000000001,0.705000000000001,0.710000000000001,
0.715000000000001,0.720000000000001,0.725000000000001,0.730000000000001,
0.735000000000001,0.740000000000001,0.745000000000001,0.750000000000001,
0.755000000000001,0.760000000000001,0.765000000000001,0.770000000000001,
0.775000000000001,0.780000000000001,0.785000000000001,0.790000000000001,
0.795000000000001,0.800000000000001,0.805000000000001,0.810000000000001,
0.815000000000001,0.820000000000001,0.825000000000001,0.830000000000001,
0.835000000000001,0.840000000000001,0.845000000000001,0.850000000000001,
0.855000000000001,0.860000000000001,0.865000000000001,0.870000000000001,
0.875000000000001,0.880000000000001,0.885000000000001,0.890000000000001,
0.895000000000001,0.900000000000001,0.905000000000001,0.910000000000001,
0.915000000000001,0.920000000000001,0.925000000000001,0.930000000000001,
0.935000000000001,0.940000000000001,0.941429844438003),.UNSPECIFIED.)
CURVE()
GEOMETRIC_REPRESENTATION_ITEM()
RATIONAL_B_SPLINE_CURVE((1.,1.,1.,1.,1.,1.,1.,1.,1.,1.,1.,1.,1.,1.,1.,1.,
1.,1.,1.,1.,1.,1.,1.,1.,1.,1.,1.,1.,1.,1.,1.,1.,1.,1.,1.,1.,1.,1.,1.,1.,
1.,1.,1.,1.,1.,1.,1.,1.,1.,1.,1.,1.,1.,1.,1.,1.,1.,1.,1.,1.,1.,1.,1.,1.,
1.,1.,1.,1.,1.,1.,1.,1.,1.,1.,1.,1.,1.,1.,1.,1.,1.,1.,1.,1.,1.,1.,1.,1.,
1.,1.,1.,1.,1.,1.,1.,1.,1.,1.,1.,1.,1.,1.,1.,1.,1.,1.,1.,1.,1.,1.,1.,1.,
1.,1.,1.,1.,1.,1.,1.,1.,1.,1.,1.,1.,1.,1.,1.,1.,1.,1.,1.,1.,1.,1.,1.,1.,
1.,1.,1.,1.,1.,1.,1.,1.,1.,1.,1.,1.,1.,1.,1.,1.,1.,1.,1.,1.,1.,1.,1.,1.,
1.,1.,1.,1.,1.,1.,1.,1.,1.,1.,1.,1.,1.,1.,1.,1.,1.,1.,1.,1.,1.,1.,1.,1.,
1.,1.,1.,1.,1.,1.,1.,1.,1.,1.))
REPRESENTATION_ITEM('')
);
#656=(
BOUNDED_CURVE()
B_SPLINE_CURVE(5,(#160854,#160855,#160856,#160857,#160858,#160859,#160860,
#160861,#160862,#160863,#160864,#160865,#160866,#160867,#160868,#160869,
#160870,#160871,#160872,#160873,#160874,#160875,#160876,#160877,#160878,
#160879,#160880,#160881,#160882,#160883,#160884,#160885,#160886,#160887,
#160888,#160889,#160890,#160891,#160892,#160893,#160894,#160895,#160896,
#160897,#160898,#160899,#160900,#160901,#160902,#160903,#160904,#160905,
#160906,#160907,#160908,#160909,#160910,#160911,#160912,#160913,#160914,
#160915,#160916,#160917,#160918,#160919,#160920,#160921,#160922,#160923,
#160924,#160925,#160926,#160927,#160928,#160929,#160930,#160931,#160932,
#160933,#160934,#160935,#160936,#160937,#160938,#160939,#160940,#160941,
#160942,#160943,#160944,#160945,#160946,#160947,#160948,#160949,#160950,
#160951,#160952,#160953,#160954,#160955,#160956,#160957,#160958,#160959,
#160960,#160961,#160962,#160963,#160964,#160965,#160966,#160967,#160968,
#160969,#160970,#160971,#160972,#160973,#160974,#160975,#160976,#160977,
#160978,#160979,#160980,#160981,#160982,#160983,#160984,#160985,#160986,
#160987,#160988,#160989,#160990,#160991,#160992,#160993,#160994,#160995,
#160996,#160997,#160998,#160999,#161000,#161001,#161002,#161003,#161004,
#161005,#161006,#161007,#161008,#161009,#161010,#161011,#161012,#161013,
#161014,#161015,#161016,#161017,#161018,#161019,#161020,#161021,#161022,
#161023,#161024,#161025,#161026,#161027,#161028,#161029,#161030,#161031,
#161032,#161033,#161034,#161035,#161036,#161037,#161038,#161039,#161040,
#161041,#161042,#161043,#161044,#161045,#161046,#161047),.UNSPECIFIED.,
 .F.,.F.)
B_SPLINE_CURVE_WITH_KNOTS((6,1,1,1,1,1,1,1,1,1,1,1,1,1,1,1,1,1,1,1,1,1,
1,1,1,1,1,1,1,1,1,1,1,1,1,1,1,1,1,1,1,1,1,1,1,1,1,1,1,1,1,1,1,1,1,1,1,1,
1,1,1,1,1,1,1,1,1,1,1,1,1,1,1,1,1,1,1,1,1,1,1,1,1,1,1,1,1,1,1,1,1,1,1,1,
1,1,1,1,1,1,1,1,1,1,1,1,1,1,1,1,1,1,1,1,1,1,1,1,1,1,1,1,1,1,1,1,1,1,1,1,
1,1,1,1,1,1,1,1,1,1,1,1,1,1,1,1,1,1,1,1,1,1,1,1,1,1,1,1,1,1,1,1,1,1,1,1,
1,1,1,1,1,1,1,1,1,1,1,1,1,1,1,1,1,1,1,1,1,1,1,6),(-0.941429844438005,-0.940000000000001,
-0.935000000000001,-0.930000000000001,-0.925000000000001,-0.920000000000001,
-0.915000000000001,-0.910000000000001,-0.905000000000001,-0.900000000000001,
-0.895000000000001,-0.890000000000001,-0.885000000000001,-0.880000000000001,
-0.875000000000001,-0.870000000000001,-0.865000000000001,-0.860000000000001,
-0.855000000000001,-0.850000000000001,-0.845000000000001,-0.840000000000001,
-0.835000000000001,-0.830000000000001,-0.825000000000001,-0.820000000000001,
-0.815000000000001,-0.810000000000001,-0.805000000000001,-0.800000000000001,
-0.795000000000001,-0.790000000000001,-0.785000000000001,-0.780000000000001,
-0.775000000000001,-0.770000000000001,-0.765000000000001,-0.760000000000001,
-0.755000000000001,-0.750000000000001,-0.745000000000001,-0.740000000000001,
-0.735000000000001,-0.730000000000001,-0.725000000000001,-0.720000000000001,
-0.715000000000001,-0.710000000000001,-0.705000000000001,-0.700000000000001,
-0.695000000000001,-0.690000000000001,-0.685,-0.68,-0.675,-0.67,-0.665,
-0.66,-0.655,-0.65,-0.645,-0.64,-0.635,-0.63,-0.625,-0.62,-0.615,-0.61,
-0.605,-0.6,-0.595,-0.59,-0.585,-0.58,-0.575,-0.57,-0.565,-0.56,-0.555,
-0.55,-0.545,-0.54,-0.535,-0.53,-0.525,-0.52,-0.515,-0.51,-0.505,-0.5,-0.495,
-0.49,-0.485,-0.48,-0.475,-0.47,-0.465,-0.46,-0.455,-0.45,-0.445,-0.44,
-0.435,-0.43,-0.425,-0.42,-0.415,-0.41,-0.405,-0.4,-0.395,-0.39,-0.385,
-0.38,-0.375,-0.37,-0.365,-0.36,-0.355,-0.35,-0.345,-0.34,-0.335,-0.33,
-0.325,-0.32,-0.315,-0.31,-0.305,-0.3,-0.295,-0.29,-0.285,-0.28,-0.275,
-0.27,-0.265,-0.26,-0.255,-0.25,-0.245,-0.24,-0.235,-0.23,-0.225,-0.22,
-0.215,-0.21,-0.205,-0.2,-0.195,-0.19,-0.185,-0.18,-0.175,-0.17,-0.165,
-0.16,-0.155,-0.15,-0.145,-0.14,-0.135,-0.13,-0.125,-0.12,-0.115,-0.11,
-0.105,-0.1,-0.095,-0.09,-0.085,-0.08,-0.075,-0.07,-0.065,-0.06,-0.055,
-0.05,-0.045,-0.04,-0.035,-0.03,-0.025,-0.02,-0.015,-0.01,-0.005,0.),
 .UNSPECIFIED.)
CURVE()
GEOMETRIC_REPRESENTATION_ITEM()
RATIONAL_B_SPLINE_CURVE((1.,1.,1.,1.,1.,1.,1.,1.,1.,1.,1.,1.,1.,1.,1.,1.,
1.,1.,1.,1.,1.,1.,1.,1.,1.,1.,1.,1.,1.,1.,1.,1.,1.,1.,1.,1.,1.,1.,1.,1.,
1.,1.,1.,1.,1.,1.,1.,1.,1.,1.,1.,1.,1.,1.,1.,1.,1.,1.,1.,1.,1.,1.,1.,1.,
1.,1.,1.,1.,1.,1.,1.,1.,1.,1.,1.,1.,1.,1.,1.,1.,1.,1.,1.,1.,1.,1.,1.,1.,
1.,1.,1.,1.,1.,1.,1.,1.,1.,1.,1.,1.,1.,1.,1.,1.,1.,1.,1.,1.,1.,1.,1.,1.,
1.,1.,1.,1.,1.,1.,1.,1.,1.,1.,1.,1.,1.,1.,1.,1.,1.,1.,1.,1.,1.,1.,1.,1.,
1.,1.,1.,1.,1.,1.,1.,1.,1.,1.,1.,1.,1.,1.,1.,1.,1.,1.,1.,1.,1.,1.,1.,1.,
1.,1.,1.,1.,1.,1.,1.,1.,1.,1.,1.,1.,1.,1.,1.,1.,1.,1.,1.,1.,1.,1.,1.,1.,
1.,1.,1.,1.,1.,1.,1.,1.,1.,1.))
REPRESENTATION_ITEM('')
);
#657=(
BOUNDED_CURVE()
B_SPLINE_CURVE(5,(#161459,#161460,#161461,#161462,#161463,#161464,#161465,
#161466,#161467,#161468,#161469,#161470,#161471,#161472,#161473,#161474,
#161475,#161476,#161477,#161478,#161479,#161480,#161481,#161482,#161483,
#161484,#161485,#161486,#161487,#161488,#161489,#161490,#161491,#161492,
#161493,#161494,#161495,#161496,#161497,#161498,#161499,#161500,#161501,
#161502,#161503,#161504,#161505,#161506,#161507,#161508,#161509,#161510,
#161511,#161512,#161513,#161514,#161515,#161516,#161517,#161518,#161519,
#161520,#161521,#161522,#161523,#161524,#161525,#161526,#161527,#161528,
#161529,#161530,#161531,#161532,#161533,#161534,#161535,#161536,#161537,
#161538,#161539,#161540,#161541,#161542,#161543,#161544,#161545,#161546,
#161547,#161548,#161549,#161550,#161551,#161552,#161553,#161554,#161555,
#161556,#161557,#161558,#161559,#161560,#161561,#161562,#161563,#161564,
#161565,#161566,#161567,#161568,#161569,#161570,#161571,#161572,#161573,
#161574,#161575,#161576,#161577,#161578,#161579,#161580,#161581,#161582,
#161583,#161584,#161585,#161586,#161587,#161588,#161589,#161590,#161591,
#161592,#161593,#161594,#161595,#161596,#161597,#161598,#161599,#161600,
#161601,#161602,#161603,#161604,#161605,#161606,#161607,#161608,#161609,
#161610,#161611,#161612,#161613,#161614,#161615,#161616,#161617,#161618,
#161619,#161620,#161621,#161622,#161623,#161624,#161625,#161626,#161627,
#161628,#161629,#161630,#161631,#161632,#161633,#161634,#161635,#161636,
#161637,#161638,#161639,#161640,#161641,#161642,#161643,#161644,#161645,
#161646,#161647,#161648,#161649,#161650,#161651,#161652),.UNSPECIFIED.,
 .F.,.F.)
B_SPLINE_CURVE_WITH_KNOTS((6,1,1,1,1,1,1,1,1,1,1,1,1,1,1,1,1,1,1,1,1,1,
1,1,1,1,1,1,1,1,1,1,1,1,1,1,1,1,1,1,1,1,1,1,1,1,1,1,1,1,1,1,1,1,1,1,1,1,
1,1,1,1,1,1,1,1,1,1,1,1,1,1,1,1,1,1,1,1,1,1,1,1,1,1,1,1,1,1,1,1,1,1,1,1,
1,1,1,1,1,1,1,1,1,1,1,1,1,1,1,1,1,1,1,1,1,1,1,1,1,1,1,1,1,1,1,1,1,1,1,1,
1,1,1,1,1,1,1,1,1,1,1,1,1,1,1,1,1,1,1,1,1,1,1,1,1,1,1,1,1,1,1,1,1,1,1,1,
1,1,1,1,1,1,1,1,1,1,1,1,1,1,1,1,1,1,1,1,1,1,1,6),(0.,0.005,0.01,0.015,0.02,
0.025,0.03,0.035,0.04,0.045,0.05,0.055,0.06,0.065,0.07,0.075,0.08,0.085,
0.09,0.095,0.1,0.105,0.11,0.115,0.12,0.125,0.13,0.135,0.14,0.145,0.15,0.155,
0.16,0.165,0.17,0.175,0.18,0.185,0.19,0.195,0.2,0.205,0.21,0.215,0.22,0.225,
0.23,0.235,0.24,0.245,0.25,0.255,0.26,0.265,0.27,0.275,0.28,0.285,0.29,
0.295,0.3,0.305,0.31,0.315,0.32,0.325,0.33,0.335,0.34,0.345,0.35,0.355,
0.36,0.365,0.37,0.375,0.38,0.385,0.39,0.395,0.4,0.405,0.41,0.415,0.42,0.425,
0.43,0.435,0.44,0.445,0.45,0.455,0.46,0.465,0.47,0.475,0.48,0.485,0.49,
0.495,0.5,0.505,0.51,0.515,0.52,0.525,0.53,0.535,0.54,0.545,0.55,0.555,
0.56,0.565,0.57,0.575,0.58,0.585,0.59,0.595,0.6,0.605,0.61,0.615,0.62,0.625,
0.63,0.635,0.64,0.645,0.65,0.655,0.66,0.665,0.67,0.675,0.68,0.685,0.690000000000001,
0.695000000000001,0.700000000000001,0.705000000000001,0.710000000000001,
0.715000000000001,0.720000000000001,0.725000000000001,0.730000000000001,
0.735000000000001,0.740000000000001,0.745000000000001,0.750000000000001,
0.755000000000001,0.760000000000001,0.765000000000001,0.770000000000001,
0.775000000000001,0.780000000000001,0.785000000000001,0.790000000000001,
0.795000000000001,0.800000000000001,0.805000000000001,0.810000000000001,
0.815000000000001,0.820000000000001,0.825000000000001,0.830000000000001,
0.835000000000001,0.840000000000001,0.845000000000001,0.850000000000001,
0.855000000000001,0.860000000000001,0.865000000000001,0.870000000000001,
0.875000000000001,0.880000000000001,0.885000000000001,0.890000000000001,
0.895000000000001,0.900000000000001,0.905000000000001,0.910000000000001,
0.915000000000001,0.920000000000001,0.925000000000001,0.930000000000001,
0.935000000000001,0.940000000000001,0.941429844438118),.UNSPECIFIED.)
CURVE()
GEOMETRIC_REPRESENTATION_ITEM()
RATIONAL_B_SPLINE_CURVE((1.,1.,1.,1.,1.,1.,1.,1.,1.,1.,1.,1.,1.,1.,1.,1.,
1.,1.,1.,1.,1.,1.,1.,1.,1.,1.,1.,1.,1.,1.,1.,1.,1.,1.,1.,1.,1.,1.,1.,1.,
1.,1.,1.,1.,1.,1.,1.,1.,1.,1.,1.,1.,1.,1.,1.,1.,1.,1.,1.,1.,1.,1.,1.,1.,
1.,1.,1.,1.,1.,1.,1.,1.,1.,1.,1.,1.,1.,1.,1.,1.,1.,1.,1.,1.,1.,1.,1.,1.,
1.,1.,1.,1.,1.,1.,1.,1.,1.,1.,1.,1.,1.,1.,1.,1.,1.,1.,1.,1.,1.,1.,1.,1.,
1.,1.,1.,1.,1.,1.,1.,1.,1.,1.,1.,1.,1.,1.,1.,1.,1.,1.,1.,1.,1.,1.,1.,1.,
1.,1.,1.,1.,1.,1.,1.,1.,1.,1.,1.,1.,1.,1.,1.,1.,1.,1.,1.,1.,1.,1.,1.,1.,
1.,1.,1.,1.,1.,1.,1.,1.,1.,1.,1.,1.,1.,1.,1.,1.,1.,1.,1.,1.,1.,1.,1.,1.,
1.,1.,1.,1.,1.,1.,1.,1.,1.,1.))
REPRESENTATION_ITEM('')
);
#658=(
BOUNDED_CURVE()
B_SPLINE_CURVE(5,(#161655,#161656,#161657,#161658,#161659,#161660,#161661,
#161662,#161663,#161664,#161665,#161666,#161667,#161668,#161669,#161670,
#161671,#161672,#161673,#161674,#161675,#161676,#161677,#161678,#161679,
#161680,#161681,#161682,#161683,#161684,#161685,#161686,#161687,#161688,
#161689,#161690,#161691,#161692,#161693,#161694,#161695,#161696,#161697,
#161698,#161699,#161700,#161701,#161702,#161703,#161704,#161705,#161706,
#161707,#161708,#161709,#161710,#161711,#161712,#161713,#161714,#161715,
#161716,#161717,#161718,#161719,#161720,#161721,#161722,#161723,#161724,
#161725,#161726,#161727,#161728,#161729,#161730,#161731,#161732,#161733,
#161734,#161735,#161736,#161737,#161738,#161739,#161740,#161741,#161742,
#161743,#161744,#161745,#161746,#161747,#161748,#161749,#161750,#161751,
#161752,#161753,#161754,#161755,#161756,#161757,#161758,#161759,#161760,
#161761,#161762,#161763,#161764,#161765,#161766,#161767,#161768,#161769,
#161770,#161771,#161772,#161773,#161774,#161775,#161776,#161777,#161778,
#161779,#161780,#161781,#161782,#161783,#161784,#161785,#161786,#161787,
#161788,#161789,#161790,#161791,#161792,#161793,#161794,#161795,#161796,
#161797,#161798,#161799,#161800,#161801,#161802,#161803,#161804,#161805,
#161806,#161807,#161808,#161809,#161810,#161811,#161812,#161813,#161814,
#161815,#161816,#161817,#161818,#161819,#161820,#161821,#161822,#161823,
#161824,#161825,#161826,#161827,#161828,#161829,#161830,#161831,#161832,
#161833,#161834,#161835,#161836,#161837,#161838,#161839,#161840,#161841,
#161842,#161843,#161844,#161845,#161846,#161847,#161848),.UNSPECIFIED.,
 .F.,.F.)
B_SPLINE_CURVE_WITH_KNOTS((6,1,1,1,1,1,1,1,1,1,1,1,1,1,1,1,1,1,1,1,1,1,
1,1,1,1,1,1,1,1,1,1,1,1,1,1,1,1,1,1,1,1,1,1,1,1,1,1,1,1,1,1,1,1,1,1,1,1,
1,1,1,1,1,1,1,1,1,1,1,1,1,1,1,1,1,1,1,1,1,1,1,1,1,1,1,1,1,1,1,1,1,1,1,1,
1,1,1,1,1,1,1,1,1,1,1,1,1,1,1,1,1,1,1,1,1,1,1,1,1,1,1,1,1,1,1,1,1,1,1,1,
1,1,1,1,1,1,1,1,1,1,1,1,1,1,1,1,1,1,1,1,1,1,1,1,1,1,1,1,1,1,1,1,1,1,1,1,
1,1,1,1,1,1,1,1,1,1,1,1,1,1,1,1,1,1,1,1,1,1,1,6),(-0.941429844438121,-0.940000000000001,
-0.935000000000001,-0.930000000000001,-0.925000000000001,-0.920000000000001,
-0.915000000000001,-0.910000000000001,-0.905000000000001,-0.900000000000001,
-0.895000000000001,-0.890000000000001,-0.885000000000001,-0.880000000000001,
-0.875000000000001,-0.870000000000001,-0.865000000000001,-0.860000000000001,
-0.855000000000001,-0.850000000000001,-0.845000000000001,-0.840000000000001,
-0.835000000000001,-0.830000000000001,-0.825000000000001,-0.820000000000001,
-0.815000000000001,-0.810000000000001,-0.805000000000001,-0.800000000000001,
-0.795000000000001,-0.790000000000001,-0.785000000000001,-0.780000000000001,
-0.775000000000001,-0.770000000000001,-0.765000000000001,-0.760000000000001,
-0.755000000000001,-0.750000000000001,-0.745000000000001,-0.740000000000001,
-0.735000000000001,-0.730000000000001,-0.725000000000001,-0.720000000000001,
-0.715000000000001,-0.710000000000001,-0.705000000000001,-0.700000000000001,
-0.695000000000001,-0.690000000000001,-0.685,-0.68,-0.675,-0.67,-0.665,
-0.66,-0.655,-0.65,-0.645,-0.64,-0.635,-0.63,-0.625,-0.62,-0.615,-0.61,
-0.605,-0.6,-0.595,-0.59,-0.585,-0.58,-0.575,-0.57,-0.565,-0.56,-0.555,
-0.55,-0.545,-0.54,-0.535,-0.53,-0.525,-0.52,-0.515,-0.51,-0.505,-0.5,-0.495,
-0.49,-0.485,-0.48,-0.475,-0.47,-0.465,-0.46,-0.455,-0.45,-0.445,-0.44,
-0.435,-0.43,-0.425,-0.42,-0.415,-0.41,-0.405,-0.4,-0.395,-0.39,-0.385,
-0.38,-0.375,-0.37,-0.365,-0.36,-0.355,-0.35,-0.345,-0.34,-0.335,-0.33,
-0.325,-0.32,-0.315,-0.31,-0.305,-0.3,-0.295,-0.29,-0.285,-0.28,-0.275,
-0.27,-0.265,-0.26,-0.255,-0.25,-0.245,-0.24,-0.235,-0.23,-0.225,-0.22,
-0.215,-0.21,-0.205,-0.2,-0.195,-0.19,-0.185,-0.18,-0.175,-0.17,-0.165,
-0.16,-0.155,-0.15,-0.145,-0.14,-0.135,-0.13,-0.125,-0.12,-0.115,-0.11,
-0.105,-0.1,-0.095,-0.09,-0.085,-0.08,-0.075,-0.07,-0.065,-0.06,-0.055,
-0.05,-0.045,-0.04,-0.035,-0.03,-0.025,-0.02,-0.015,-0.01,-0.005,0.),
 .UNSPECIFIED.)
CURVE()
GEOMETRIC_REPRESENTATION_ITEM()
RATIONAL_B_SPLINE_CURVE((1.,1.,1.,1.,1.,1.,1.,1.,1.,1.,1.,1.,1.,1.,1.,1.,
1.,1.,1.,1.,1.,1.,1.,1.,1.,1.,1.,1.,1.,1.,1.,1.,1.,1.,1.,1.,1.,1.,1.,1.,
1.,1.,1.,1.,1.,1.,1.,1.,1.,1.,1.,1.,1.,1.,1.,1.,1.,1.,1.,1.,1.,1.,1.,1.,
1.,1.,1.,1.,1.,1.,1.,1.,1.,1.,1.,1.,1.,1.,1.,1.,1.,1.,1.,1.,1.,1.,1.,1.,
1.,1.,1.,1.,1.,1.,1.,1.,1.,1.,1.,1.,1.,1.,1.,1.,1.,1.,1.,1.,1.,1.,1.,1.,
1.,1.,1.,1.,1.,1.,1.,1.,1.,1.,1.,1.,1.,1.,1.,1.,1.,1.,1.,1.,1.,1.,1.,1.,
1.,1.,1.,1.,1.,1.,1.,1.,1.,1.,1.,1.,1.,1.,1.,1.,1.,1.,1.,1.,1.,1.,1.,1.,
1.,1.,1.,1.,1.,1.,1.,1.,1.,1.,1.,1.,1.,1.,1.,1.,1.,1.,1.,1.,1.,1.,1.,1.,
1.,1.,1.,1.,1.,1.,1.,1.,1.,1.))
REPRESENTATION_ITEM('')
);
#659=(
BOUNDED_CURVE()
B_SPLINE_CURVE(5,(#162260,#162261,#162262,#162263,#162264,#162265,#162266,
#162267,#162268,#162269,#162270,#162271,#162272,#162273,#162274,#162275,
#162276,#162277,#162278,#162279,#162280,#162281,#162282,#162283,#162284,
#162285,#162286,#162287,#162288,#162289,#162290,#162291,#162292,#162293,
#162294,#162295,#162296,#162297,#162298,#162299,#162300,#162301,#162302,
#162303,#162304,#162305,#162306,#162307,#162308,#162309,#162310,#162311,
#162312,#162313,#162314,#162315,#162316,#162317,#162318,#162319,#162320,
#162321,#162322,#162323,#162324,#162325,#162326,#162327,#162328,#162329,
#162330,#162331,#162332,#162333,#162334,#162335,#162336,#162337,#162338,
#162339,#162340,#162341,#162342,#162343,#162344,#162345,#162346,#162347,
#162348,#162349,#162350,#162351,#162352,#162353,#162354,#162355,#162356,
#162357,#162358,#162359,#162360,#162361,#162362,#162363,#162364,#162365,
#162366,#162367,#162368,#162369,#162370,#162371,#162372,#162373,#162374,
#162375,#162376,#162377,#162378,#162379,#162380,#162381,#162382,#162383,
#162384,#162385,#162386,#162387,#162388,#162389,#162390,#162391,#162392,
#162393,#162394,#162395,#162396,#162397,#162398,#162399,#162400,#162401,
#162402,#162403,#162404,#162405,#162406,#162407,#162408,#162409,#162410,
#162411,#162412,#162413,#162414,#162415,#162416,#162417,#162418,#162419,
#162420,#162421,#162422,#162423,#162424,#162425,#162426,#162427,#162428,
#162429,#162430,#162431,#162432,#162433,#162434,#162435,#162436,#162437,
#162438,#162439,#162440,#162441,#162442,#162443,#162444,#162445,#162446,
#162447,#162448,#162449,#162450,#162451,#162452,#162453),.UNSPECIFIED.,
 .F.,.F.)
B_SPLINE_CURVE_WITH_KNOTS((6,1,1,1,1,1,1,1,1,1,1,1,1,1,1,1,1,1,1,1,1,1,
1,1,1,1,1,1,1,1,1,1,1,1,1,1,1,1,1,1,1,1,1,1,1,1,1,1,1,1,1,1,1,1,1,1,1,1,
1,1,1,1,1,1,1,1,1,1,1,1,1,1,1,1,1,1,1,1,1,1,1,1,1,1,1,1,1,1,1,1,1,1,1,1,
1,1,1,1,1,1,1,1,1,1,1,1,1,1,1,1,1,1,1,1,1,1,1,1,1,1,1,1,1,1,1,1,1,1,1,1,
1,1,1,1,1,1,1,1,1,1,1,1,1,1,1,1,1,1,1,1,1,1,1,1,1,1,1,1,1,1,1,1,1,1,1,1,
1,1,1,1,1,1,1,1,1,1,1,1,1,1,1,1,1,1,1,1,1,1,1,6),(0.,0.005,0.01,0.015,0.02,
0.025,0.03,0.035,0.04,0.045,0.05,0.055,0.06,0.065,0.07,0.075,0.08,0.085,
0.09,0.095,0.1,0.105,0.11,0.115,0.12,0.125,0.13,0.135,0.14,0.145,0.15,0.155,
0.16,0.165,0.17,0.175,0.18,0.185,0.19,0.195,0.2,0.205,0.21,0.215,0.22,0.225,
0.23,0.235,0.24,0.245,0.25,0.255,0.26,0.265,0.27,0.275,0.28,0.285,0.29,
0.295,0.3,0.305,0.31,0.315,0.32,0.325,0.33,0.335,0.34,0.345,0.35,0.355,
0.36,0.365,0.37,0.375,0.38,0.385,0.39,0.395,0.4,0.405,0.41,0.415,0.42,0.425,
0.43,0.435,0.44,0.445,0.45,0.455,0.46,0.465,0.47,0.475,0.48,0.485,0.49,
0.495,0.5,0.505,0.51,0.515,0.52,0.525,0.53,0.535,0.54,0.545,0.55,0.555,
0.56,0.565,0.57,0.575,0.58,0.585,0.59,0.595,0.6,0.605,0.61,0.615,0.62,0.625,
0.63,0.635,0.64,0.645,0.65,0.655,0.66,0.665,0.67,0.675,0.68,0.685,0.690000000000001,
0.695000000000001,0.700000000000001,0.705000000000001,0.710000000000001,
0.715000000000001,0.720000000000001,0.725000000000001,0.730000000000001,
0.735000000000001,0.740000000000001,0.745000000000001,0.750000000000001,
0.755000000000001,0.760000000000001,0.765000000000001,0.770000000000001,
0.775000000000001,0.780000000000001,0.785000000000001,0.790000000000001,
0.795000000000001,0.800000000000001,0.805000000000001,0.810000000000001,
0.815000000000001,0.820000000000001,0.825000000000001,0.830000000000001,
0.835000000000001,0.840000000000001,0.845000000000001,0.850000000000001,
0.855000000000001,0.860000000000001,0.865000000000001,0.870000000000001,
0.875000000000001,0.880000000000001,0.885000000000001,0.890000000000001,
0.895000000000001,0.900000000000001,0.905000000000001,0.910000000000001,
0.915000000000001,0.920000000000001,0.925000000000001,0.930000000000001,
0.935000000000001,0.940000000000001,0.941429844438068),.UNSPECIFIED.)
CURVE()
GEOMETRIC_REPRESENTATION_ITEM()
RATIONAL_B_SPLINE_CURVE((1.,1.,1.,1.,1.,1.,1.,1.,1.,1.,1.,1.,1.,1.,1.,1.,
1.,1.,1.,1.,1.,1.,1.,1.,1.,1.,1.,1.,1.,1.,1.,1.,1.,1.,1.,1.,1.,1.,1.,1.,
1.,1.,1.,1.,1.,1.,1.,1.,1.,1.,1.,1.,1.,1.,1.,1.,1.,1.,1.,1.,1.,1.,1.,1.,
1.,1.,1.,1.,1.,1.,1.,1.,1.,1.,1.,1.,1.,1.,1.,1.,1.,1.,1.,1.,1.,1.,1.,1.,
1.,1.,1.,1.,1.,1.,1.,1.,1.,1.,1.,1.,1.,1.,1.,1.,1.,1.,1.,1.,1.,1.,1.,1.,
1.,1.,1.,1.,1.,1.,1.,1.,1.,1.,1.,1.,1.,1.,1.,1.,1.,1.,1.,1.,1.,1.,1.,1.,
1.,1.,1.,1.,1.,1.,1.,1.,1.,1.,1.,1.,1.,1.,1.,1.,1.,1.,1.,1.,1.,1.,1.,1.,
1.,1.,1.,1.,1.,1.,1.,1.,1.,1.,1.,1.,1.,1.,1.,1.,1.,1.,1.,1.,1.,1.,1.,1.,
1.,1.,1.,1.,1.,1.,1.,1.,1.,1.))
REPRESENTATION_ITEM('')
);
#660=(
BOUNDED_CURVE()
B_SPLINE_CURVE(5,(#162456,#162457,#162458,#162459,#162460,#162461,#162462,
#162463,#162464,#162465,#162466,#162467,#162468,#162469,#162470,#162471,
#162472,#162473,#162474,#162475,#162476,#162477,#162478,#162479,#162480,
#162481,#162482,#162483,#162484,#162485,#162486,#162487,#162488,#162489,
#162490,#162491,#162492,#162493,#162494,#162495,#162496,#162497,#162498,
#162499,#162500,#162501,#162502,#162503,#162504,#162505,#162506,#162507,
#162508,#162509,#162510,#162511,#162512,#162513,#162514,#162515,#162516,
#162517,#162518,#162519,#162520,#162521,#162522,#162523,#162524,#162525,
#162526,#162527,#162528,#162529,#162530,#162531,#162532,#162533,#162534,
#162535,#162536,#162537,#162538,#162539,#162540,#162541,#162542,#162543,
#162544,#162545,#162546,#162547,#162548,#162549,#162550,#162551,#162552,
#162553,#162554,#162555,#162556,#162557,#162558,#162559,#162560,#162561,
#162562,#162563,#162564,#162565,#162566,#162567,#162568,#162569,#162570,
#162571,#162572,#162573,#162574,#162575,#162576,#162577,#162578,#162579,
#162580,#162581,#162582,#162583,#162584,#162585,#162586,#162587,#162588,
#162589,#162590,#162591,#162592,#162593,#162594,#162595,#162596,#162597,
#162598,#162599,#162600,#162601,#162602,#162603,#162604,#162605,#162606,
#162607,#162608,#162609,#162610,#162611,#162612,#162613,#162614,#162615,
#162616,#162617,#162618,#162619,#162620,#162621,#162622,#162623,#162624,
#162625,#162626,#162627,#162628,#162629,#162630,#162631,#162632,#162633,
#162634,#162635,#162636,#162637,#162638,#162639,#162640,#162641,#162642,
#162643,#162644,#162645,#162646,#162647,#162648,#162649),.UNSPECIFIED.,
 .F.,.F.)
B_SPLINE_CURVE_WITH_KNOTS((6,1,1,1,1,1,1,1,1,1,1,1,1,1,1,1,1,1,1,1,1,1,
1,1,1,1,1,1,1,1,1,1,1,1,1,1,1,1,1,1,1,1,1,1,1,1,1,1,1,1,1,1,1,1,1,1,1,1,
1,1,1,1,1,1,1,1,1,1,1,1,1,1,1,1,1,1,1,1,1,1,1,1,1,1,1,1,1,1,1,1,1,1,1,1,
1,1,1,1,1,1,1,1,1,1,1,1,1,1,1,1,1,1,1,1,1,1,1,1,1,1,1,1,1,1,1,1,1,1,1,1,
1,1,1,1,1,1,1,1,1,1,1,1,1,1,1,1,1,1,1,1,1,1,1,1,1,1,1,1,1,1,1,1,1,1,1,1,
1,1,1,1,1,1,1,1,1,1,1,1,1,1,1,1,1,1,1,1,1,1,1,6),(-0.941429844438068,-0.940000000000001,
-0.935000000000001,-0.930000000000001,-0.925000000000001,-0.920000000000001,
-0.915000000000001,-0.910000000000001,-0.905000000000001,-0.900000000000001,
-0.895000000000001,-0.890000000000001,-0.885000000000001,-0.880000000000001,
-0.875000000000001,-0.870000000000001,-0.865000000000001,-0.860000000000001,
-0.855000000000001,-0.850000000000001,-0.845000000000001,-0.840000000000001,
-0.835000000000001,-0.830000000000001,-0.825000000000001,-0.820000000000001,
-0.815000000000001,-0.810000000000001,-0.805000000000001,-0.800000000000001,
-0.795000000000001,-0.790000000000001,-0.785000000000001,-0.780000000000001,
-0.775000000000001,-0.770000000000001,-0.765000000000001,-0.760000000000001,
-0.755000000000001,-0.750000000000001,-0.745000000000001,-0.740000000000001,
-0.735000000000001,-0.730000000000001,-0.725000000000001,-0.720000000000001,
-0.715000000000001,-0.710000000000001,-0.705000000000001,-0.700000000000001,
-0.695000000000001,-0.690000000000001,-0.685,-0.68,-0.675,-0.67,-0.665,
-0.66,-0.655,-0.65,-0.645,-0.64,-0.635,-0.63,-0.625,-0.62,-0.615,-0.61,
-0.605,-0.6,-0.595,-0.59,-0.585,-0.58,-0.575,-0.57,-0.565,-0.56,-0.555,
-0.55,-0.545,-0.54,-0.535,-0.53,-0.525,-0.52,-0.515,-0.51,-0.505,-0.5,-0.495,
-0.49,-0.485,-0.48,-0.475,-0.47,-0.465,-0.46,-0.455,-0.45,-0.445,-0.44,
-0.435,-0.43,-0.425,-0.42,-0.415,-0.41,-0.405,-0.4,-0.395,-0.39,-0.385,
-0.38,-0.375,-0.37,-0.365,-0.36,-0.355,-0.35,-0.345,-0.34,-0.335,-0.33,
-0.325,-0.32,-0.315,-0.31,-0.305,-0.3,-0.295,-0.29,-0.285,-0.28,-0.275,
-0.27,-0.265,-0.26,-0.255,-0.25,-0.245,-0.24,-0.235,-0.23,-0.225,-0.22,
-0.215,-0.21,-0.205,-0.2,-0.195,-0.19,-0.185,-0.18,-0.175,-0.17,-0.165,
-0.16,-0.155,-0.15,-0.145,-0.14,-0.135,-0.13,-0.125,-0.12,-0.115,-0.11,
-0.105,-0.1,-0.095,-0.09,-0.085,-0.08,-0.075,-0.07,-0.065,-0.06,-0.055,
-0.05,-0.045,-0.04,-0.035,-0.03,-0.025,-0.02,-0.015,-0.01,-0.005,0.),
 .UNSPECIFIED.)
CURVE()
GEOMETRIC_REPRESENTATION_ITEM()
RATIONAL_B_SPLINE_CURVE((1.,1.,1.,1.,1.,1.,1.,1.,1.,1.,1.,1.,1.,1.,1.,1.,
1.,1.,1.,1.,1.,1.,1.,1.,1.,1.,1.,1.,1.,1.,1.,1.,1.,1.,1.,1.,1.,1.,1.,1.,
1.,1.,1.,1.,1.,1.,1.,1.,1.,1.,1.,1.,1.,1.,1.,1.,1.,1.,1.,1.,1.,1.,1.,1.,
1.,1.,1.,1.,1.,1.,1.,1.,1.,1.,1.,1.,1.,1.,1.,1.,1.,1.,1.,1.,1.,1.,1.,1.,
1.,1.,1.,1.,1.,1.,1.,1.,1.,1.,1.,1.,1.,1.,1.,1.,1.,1.,1.,1.,1.,1.,1.,1.,
1.,1.,1.,1.,1.,1.,1.,1.,1.,1.,1.,1.,1.,1.,1.,1.,1.,1.,1.,1.,1.,1.,1.,1.,
1.,1.,1.,1.,1.,1.,1.,1.,1.,1.,1.,1.,1.,1.,1.,1.,1.,1.,1.,1.,1.,1.,1.,1.,
1.,1.,1.,1.,1.,1.,1.,1.,1.,1.,1.,1.,1.,1.,1.,1.,1.,1.,1.,1.,1.,1.,1.,1.,
1.,1.,1.,1.,1.,1.,1.,1.,1.,1.))
REPRESENTATION_ITEM('')
);
#661=(
BOUNDED_CURVE()
B_SPLINE_CURVE(5,(#163061,#163062,#163063,#163064,#163065,#163066,#163067,
#163068,#163069,#163070,#163071,#163072,#163073,#163074,#163075,#163076,
#163077,#163078,#163079,#163080,#163081,#163082,#163083,#163084,#163085,
#163086,#163087,#163088,#163089,#163090,#163091,#163092,#163093,#163094,
#163095,#163096,#163097,#163098,#163099,#163100,#163101,#163102,#163103,
#163104,#163105,#163106,#163107,#163108,#163109,#163110,#163111,#163112,
#163113,#163114,#163115,#163116,#163117,#163118,#163119,#163120,#163121,
#163122,#163123,#163124,#163125,#163126,#163127,#163128,#163129,#163130,
#163131,#163132,#163133,#163134,#163135,#163136,#163137,#163138,#163139,
#163140,#163141,#163142,#163143,#163144,#163145,#163146,#163147,#163148,
#163149,#163150,#163151,#163152,#163153,#163154,#163155,#163156,#163157,
#163158,#163159,#163160,#163161,#163162,#163163,#163164,#163165,#163166,
#163167,#163168,#163169,#163170,#163171,#163172,#163173,#163174,#163175,
#163176,#163177,#163178,#163179,#163180,#163181,#163182,#163183,#163184,
#163185,#163186,#163187,#163188,#163189,#163190,#163191,#163192,#163193,
#163194,#163195,#163196,#163197,#163198,#163199,#163200,#163201,#163202,
#163203,#163204,#163205,#163206,#163207,#163208,#163209,#163210,#163211,
#163212,#163213,#163214,#163215,#163216,#163217,#163218,#163219,#163220,
#163221,#163222,#163223,#163224,#163225,#163226,#163227,#163228,#163229,
#163230,#163231,#163232,#163233,#163234,#163235,#163236,#163237,#163238,
#163239,#163240,#163241,#163242,#163243,#163244,#163245,#163246,#163247,
#163248,#163249,#163250,#163251,#163252,#163253,#163254),.UNSPECIFIED.,
 .F.,.F.)
B_SPLINE_CURVE_WITH_KNOTS((6,1,1,1,1,1,1,1,1,1,1,1,1,1,1,1,1,1,1,1,1,1,
1,1,1,1,1,1,1,1,1,1,1,1,1,1,1,1,1,1,1,1,1,1,1,1,1,1,1,1,1,1,1,1,1,1,1,1,
1,1,1,1,1,1,1,1,1,1,1,1,1,1,1,1,1,1,1,1,1,1,1,1,1,1,1,1,1,1,1,1,1,1,1,1,
1,1,1,1,1,1,1,1,1,1,1,1,1,1,1,1,1,1,1,1,1,1,1,1,1,1,1,1,1,1,1,1,1,1,1,1,
1,1,1,1,1,1,1,1,1,1,1,1,1,1,1,1,1,1,1,1,1,1,1,1,1,1,1,1,1,1,1,1,1,1,1,1,
1,1,1,1,1,1,1,1,1,1,1,1,1,1,1,1,1,1,1,1,1,1,1,6),(0.,0.005,0.01,0.015,0.02,
0.025,0.03,0.035,0.04,0.045,0.05,0.055,0.06,0.065,0.07,0.075,0.08,0.085,
0.09,0.095,0.1,0.105,0.11,0.115,0.12,0.125,0.13,0.135,0.14,0.145,0.15,0.155,
0.16,0.165,0.17,0.175,0.18,0.185,0.19,0.195,0.2,0.205,0.21,0.215,0.22,0.225,
0.23,0.235,0.24,0.245,0.25,0.255,0.26,0.265,0.27,0.275,0.28,0.285,0.29,
0.295,0.3,0.305,0.31,0.315,0.32,0.325,0.33,0.335,0.34,0.345,0.35,0.355,
0.36,0.365,0.37,0.375,0.38,0.385,0.39,0.395,0.4,0.405,0.41,0.415,0.42,0.425,
0.43,0.435,0.44,0.445,0.45,0.455,0.46,0.465,0.47,0.475,0.48,0.485,0.49,
0.495,0.5,0.505,0.51,0.515,0.52,0.525,0.53,0.535,0.54,0.545,0.55,0.555,
0.56,0.565,0.57,0.575,0.58,0.585,0.59,0.595,0.6,0.605,0.61,0.615,0.62,0.625,
0.63,0.635,0.64,0.645,0.65,0.655,0.66,0.665,0.67,0.675,0.68,0.685,0.690000000000001,
0.695000000000001,0.700000000000001,0.705000000000001,0.710000000000001,
0.715000000000001,0.720000000000001,0.725000000000001,0.730000000000001,
0.735000000000001,0.740000000000001,0.745000000000001,0.750000000000001,
0.755000000000001,0.760000000000001,0.765000000000001,0.770000000000001,
0.775000000000001,0.780000000000001,0.785000000000001,0.790000000000001,
0.795000000000001,0.800000000000001,0.805000000000001,0.810000000000001,
0.815000000000001,0.820000000000001,0.825000000000001,0.830000000000001,
0.835000000000001,0.840000000000001,0.845000000000001,0.850000000000001,
0.855000000000001,0.860000000000001,0.865000000000001,0.870000000000001,
0.875000000000001,0.880000000000001,0.885000000000001,0.890000000000001,
0.895000000000001,0.900000000000001,0.905000000000001,0.910000000000001,
0.915000000000001,0.920000000000001,0.925000000000001,0.930000000000001,
0.935000000000001,0.940000000000001,0.941429844438002),.UNSPECIFIED.)
CURVE()
GEOMETRIC_REPRESENTATION_ITEM()
RATIONAL_B_SPLINE_CURVE((1.,1.,1.,1.,1.,1.,1.,1.,1.,1.,1.,1.,1.,1.,1.,1.,
1.,1.,1.,1.,1.,1.,1.,1.,1.,1.,1.,1.,1.,1.,1.,1.,1.,1.,1.,1.,1.,1.,1.,1.,
1.,1.,1.,1.,1.,1.,1.,1.,1.,1.,1.,1.,1.,1.,1.,1.,1.,1.,1.,1.,1.,1.,1.,1.,
1.,1.,1.,1.,1.,1.,1.,1.,1.,1.,1.,1.,1.,1.,1.,1.,1.,1.,1.,1.,1.,1.,1.,1.,
1.,1.,1.,1.,1.,1.,1.,1.,1.,1.,1.,1.,1.,1.,1.,1.,1.,1.,1.,1.,1.,1.,1.,1.,
1.,1.,1.,1.,1.,1.,1.,1.,1.,1.,1.,1.,1.,1.,1.,1.,1.,1.,1.,1.,1.,1.,1.,1.,
1.,1.,1.,1.,1.,1.,1.,1.,1.,1.,1.,1.,1.,1.,1.,1.,1.,1.,1.,1.,1.,1.,1.,1.,
1.,1.,1.,1.,1.,1.,1.,1.,1.,1.,1.,1.,1.,1.,1.,1.,1.,1.,1.,1.,1.,1.,1.,1.,
1.,1.,1.,1.,1.,1.,1.,1.,1.,1.))
REPRESENTATION_ITEM('')
);
#662=(
BOUNDED_CURVE()
B_SPLINE_CURVE(5,(#163257,#163258,#163259,#163260,#163261,#163262,#163263,
#163264,#163265,#163266,#163267,#163268,#163269,#163270,#163271,#163272,
#163273,#163274,#163275,#163276,#163277,#163278,#163279,#163280,#163281,
#163282,#163283,#163284,#163285,#163286,#163287,#163288,#163289,#163290,
#163291,#163292,#163293,#163294,#163295,#163296,#163297,#163298,#163299,
#163300,#163301,#163302,#163303,#163304,#163305,#163306,#163307,#163308,
#163309,#163310,#163311,#163312,#163313,#163314,#163315,#163316,#163317,
#163318,#163319,#163320,#163321,#163322,#163323,#163324,#163325,#163326,
#163327,#163328,#163329,#163330,#163331,#163332,#163333,#163334,#163335,
#163336,#163337,#163338,#163339,#163340,#163341,#163342,#163343,#163344,
#163345,#163346,#163347,#163348,#163349,#163350,#163351,#163352,#163353,
#163354,#163355,#163356,#163357,#163358,#163359,#163360,#163361,#163362,
#163363,#163364,#163365,#163366,#163367,#163368,#163369,#163370,#163371,
#163372,#163373,#163374,#163375,#163376,#163377,#163378,#163379,#163380,
#163381,#163382,#163383,#163384,#163385,#163386,#163387,#163388,#163389,
#163390,#163391,#163392,#163393,#163394,#163395,#163396,#163397,#163398,
#163399,#163400,#163401,#163402,#163403,#163404,#163405,#163406,#163407,
#163408,#163409,#163410,#163411,#163412,#163413,#163414,#163415,#163416,
#163417,#163418,#163419,#163420,#163421,#163422,#163423,#163424,#163425,
#163426,#163427,#163428,#163429,#163430,#163431,#163432,#163433,#163434,
#163435,#163436,#163437,#163438,#163439,#163440,#163441,#163442,#163443,
#163444,#163445,#163446,#163447,#163448,#163449,#163450),.UNSPECIFIED.,
 .F.,.F.)
B_SPLINE_CURVE_WITH_KNOTS((6,1,1,1,1,1,1,1,1,1,1,1,1,1,1,1,1,1,1,1,1,1,
1,1,1,1,1,1,1,1,1,1,1,1,1,1,1,1,1,1,1,1,1,1,1,1,1,1,1,1,1,1,1,1,1,1,1,1,
1,1,1,1,1,1,1,1,1,1,1,1,1,1,1,1,1,1,1,1,1,1,1,1,1,1,1,1,1,1,1,1,1,1,1,1,
1,1,1,1,1,1,1,1,1,1,1,1,1,1,1,1,1,1,1,1,1,1,1,1,1,1,1,1,1,1,1,1,1,1,1,1,
1,1,1,1,1,1,1,1,1,1,1,1,1,1,1,1,1,1,1,1,1,1,1,1,1,1,1,1,1,1,1,1,1,1,1,1,
1,1,1,1,1,1,1,1,1,1,1,1,1,1,1,1,1,1,1,1,1,1,1,6),(-0.941429844438003,-0.940000000000001,
-0.935000000000001,-0.930000000000001,-0.925000000000001,-0.920000000000001,
-0.915000000000001,-0.910000000000001,-0.905000000000001,-0.900000000000001,
-0.895000000000001,-0.890000000000001,-0.885000000000001,-0.880000000000001,
-0.875000000000001,-0.870000000000001,-0.865000000000001,-0.860000000000001,
-0.855000000000001,-0.850000000000001,-0.845000000000001,-0.840000000000001,
-0.835000000000001,-0.830000000000001,-0.825000000000001,-0.820000000000001,
-0.815000000000001,-0.810000000000001,-0.805000000000001,-0.800000000000001,
-0.795000000000001,-0.790000000000001,-0.785000000000001,-0.780000000000001,
-0.775000000000001,-0.770000000000001,-0.765000000000001,-0.760000000000001,
-0.755000000000001,-0.750000000000001,-0.745000000000001,-0.740000000000001,
-0.735000000000001,-0.730000000000001,-0.725000000000001,-0.720000000000001,
-0.715000000000001,-0.710000000000001,-0.705000000000001,-0.700000000000001,
-0.695000000000001,-0.690000000000001,-0.685,-0.68,-0.675,-0.67,-0.665,
-0.66,-0.655,-0.65,-0.645,-0.64,-0.635,-0.63,-0.625,-0.62,-0.615,-0.61,
-0.605,-0.6,-0.595,-0.59,-0.585,-0.58,-0.575,-0.57,-0.565,-0.56,-0.555,
-0.55,-0.545,-0.54,-0.535,-0.53,-0.525,-0.52,-0.515,-0.51,-0.505,-0.5,-0.495,
-0.49,-0.485,-0.48,-0.475,-0.47,-0.465,-0.46,-0.455,-0.45,-0.445,-0.44,
-0.435,-0.43,-0.425,-0.42,-0.415,-0.41,-0.405,-0.4,-0.395,-0.39,-0.385,
-0.38,-0.375,-0.37,-0.365,-0.36,-0.355,-0.35,-0.345,-0.34,-0.335,-0.33,
-0.325,-0.32,-0.315,-0.31,-0.305,-0.3,-0.295,-0.29,-0.285,-0.28,-0.275,
-0.27,-0.265,-0.26,-0.255,-0.25,-0.245,-0.24,-0.235,-0.23,-0.225,-0.22,
-0.215,-0.21,-0.205,-0.2,-0.195,-0.19,-0.185,-0.18,-0.175,-0.17,-0.165,
-0.16,-0.155,-0.15,-0.145,-0.14,-0.135,-0.13,-0.125,-0.12,-0.115,-0.11,
-0.105,-0.1,-0.095,-0.09,-0.085,-0.08,-0.075,-0.07,-0.065,-0.06,-0.055,
-0.05,-0.045,-0.04,-0.035,-0.03,-0.025,-0.02,-0.015,-0.01,-0.005,0.),
 .UNSPECIFIED.)
CURVE()
GEOMETRIC_REPRESENTATION_ITEM()
RATIONAL_B_SPLINE_CURVE((1.,1.,1.,1.,1.,1.,1.,1.,1.,1.,1.,1.,1.,1.,1.,1.,
1.,1.,1.,1.,1.,1.,1.,1.,1.,1.,1.,1.,1.,1.,1.,1.,1.,1.,1.,1.,1.,1.,1.,1.,
1.,1.,1.,1.,1.,1.,1.,1.,1.,1.,1.,1.,1.,1.,1.,1.,1.,1.,1.,1.,1.,1.,1.,1.,
1.,1.,1.,1.,1.,1.,1.,1.,1.,1.,1.,1.,1.,1.,1.,1.,1.,1.,1.,1.,1.,1.,1.,1.,
1.,1.,1.,1.,1.,1.,1.,1.,1.,1.,1.,1.,1.,1.,1.,1.,1.,1.,1.,1.,1.,1.,1.,1.,
1.,1.,1.,1.,1.,1.,1.,1.,1.,1.,1.,1.,1.,1.,1.,1.,1.,1.,1.,1.,1.,1.,1.,1.,
1.,1.,1.,1.,1.,1.,1.,1.,1.,1.,1.,1.,1.,1.,1.,1.,1.,1.,1.,1.,1.,1.,1.,1.,
1.,1.,1.,1.,1.,1.,1.,1.,1.,1.,1.,1.,1.,1.,1.,1.,1.,1.,1.,1.,1.,1.,1.,1.,
1.,1.,1.,1.,1.,1.,1.,1.,1.,1.))
REPRESENTATION_ITEM('')
);
#663=(
BOUNDED_CURVE()
B_SPLINE_CURVE(5,(#163862,#163863,#163864,#163865,#163866,#163867,#163868,
#163869,#163870,#163871,#163872,#163873,#163874,#163875,#163876,#163877,
#163878,#163879,#163880,#163881,#163882,#163883,#163884,#163885,#163886,
#163887,#163888,#163889,#163890,#163891,#163892,#163893,#163894,#163895,
#163896,#163897,#163898,#163899,#163900,#163901,#163902,#163903,#163904,
#163905,#163906,#163907,#163908,#163909,#163910,#163911,#163912,#163913,
#163914,#163915,#163916,#163917,#163918,#163919,#163920,#163921,#163922,
#163923,#163924,#163925,#163926,#163927,#163928,#163929,#163930,#163931,
#163932,#163933,#163934,#163935,#163936,#163937,#163938,#163939,#163940,
#163941,#163942,#163943,#163944,#163945,#163946,#163947,#163948,#163949,
#163950,#163951,#163952,#163953,#163954,#163955,#163956,#163957,#163958,
#163959,#163960,#163961,#163962,#163963,#163964,#163965,#163966,#163967,
#163968,#163969,#163970,#163971,#163972,#163973,#163974,#163975,#163976,
#163977,#163978,#163979,#163980,#163981,#163982,#163983,#163984,#163985,
#163986,#163987,#163988,#163989,#163990,#163991,#163992,#163993,#163994,
#163995,#163996,#163997,#163998,#163999,#164000,#164001,#164002,#164003,
#164004,#164005,#164006,#164007,#164008,#164009,#164010,#164011,#164012,
#164013,#164014,#164015,#164016,#164017,#164018,#164019,#164020,#164021,
#164022,#164023,#164024,#164025,#164026,#164027,#164028,#164029,#164030,
#164031,#164032,#164033,#164034,#164035,#164036,#164037,#164038,#164039,
#164040,#164041,#164042,#164043,#164044,#164045,#164046,#164047,#164048,
#164049,#164050,#164051,#164052,#164053,#164054,#164055),.UNSPECIFIED.,
 .F.,.F.)
B_SPLINE_CURVE_WITH_KNOTS((6,1,1,1,1,1,1,1,1,1,1,1,1,1,1,1,1,1,1,1,1,1,
1,1,1,1,1,1,1,1,1,1,1,1,1,1,1,1,1,1,1,1,1,1,1,1,1,1,1,1,1,1,1,1,1,1,1,1,
1,1,1,1,1,1,1,1,1,1,1,1,1,1,1,1,1,1,1,1,1,1,1,1,1,1,1,1,1,1,1,1,1,1,1,1,
1,1,1,1,1,1,1,1,1,1,1,1,1,1,1,1,1,1,1,1,1,1,1,1,1,1,1,1,1,1,1,1,1,1,1,1,
1,1,1,1,1,1,1,1,1,1,1,1,1,1,1,1,1,1,1,1,1,1,1,1,1,1,1,1,1,1,1,1,1,1,1,1,
1,1,1,1,1,1,1,1,1,1,1,1,1,1,1,1,1,1,1,1,1,1,1,6),(0.,0.005,0.01,0.015,0.02,
0.025,0.03,0.035,0.04,0.045,0.05,0.055,0.06,0.065,0.07,0.075,0.08,0.085,
0.09,0.095,0.1,0.105,0.11,0.115,0.12,0.125,0.13,0.135,0.14,0.145,0.15,0.155,
0.16,0.165,0.17,0.175,0.18,0.185,0.19,0.195,0.2,0.205,0.21,0.215,0.22,0.225,
0.23,0.235,0.24,0.245,0.25,0.255,0.26,0.265,0.27,0.275,0.28,0.285,0.29,
0.295,0.3,0.305,0.31,0.315,0.32,0.325,0.33,0.335,0.34,0.345,0.35,0.355,
0.36,0.365,0.37,0.375,0.38,0.385,0.39,0.395,0.4,0.405,0.41,0.415,0.42,0.425,
0.43,0.435,0.44,0.445,0.45,0.455,0.46,0.465,0.47,0.475,0.48,0.485,0.49,
0.495,0.5,0.505,0.51,0.515,0.52,0.525,0.53,0.535,0.54,0.545,0.55,0.555,
0.56,0.565,0.57,0.575,0.58,0.585,0.59,0.595,0.6,0.605,0.61,0.615,0.62,0.625,
0.63,0.635,0.64,0.645,0.65,0.655,0.66,0.665,0.67,0.675,0.68,0.685,0.690000000000001,
0.695000000000001,0.700000000000001,0.705000000000001,0.710000000000001,
0.715000000000001,0.720000000000001,0.725000000000001,0.730000000000001,
0.735000000000001,0.740000000000001,0.745000000000001,0.750000000000001,
0.755000000000001,0.760000000000001,0.765000000000001,0.770000000000001,
0.775000000000001,0.780000000000001,0.785000000000001,0.790000000000001,
0.795000000000001,0.800000000000001,0.805000000000001,0.810000000000001,
0.815000000000001,0.820000000000001,0.825000000000001,0.830000000000001,
0.835000000000001,0.840000000000001,0.845000000000001,0.850000000000001,
0.855000000000001,0.860000000000001,0.865000000000001,0.870000000000001,
0.875000000000001,0.880000000000001,0.885000000000001,0.890000000000001,
0.895000000000001,0.900000000000001,0.905000000000001,0.910000000000001,
0.915000000000001,0.920000000000001,0.925000000000001,0.930000000000001,
0.935000000000001,0.940000000000001,0.941429844437967),.UNSPECIFIED.)
CURVE()
GEOMETRIC_REPRESENTATION_ITEM()
RATIONAL_B_SPLINE_CURVE((1.,1.,1.,1.,1.,1.,1.,1.,1.,1.,1.,1.,1.,1.,1.,1.,
1.,1.,1.,1.,1.,1.,1.,1.,1.,1.,1.,1.,1.,1.,1.,1.,1.,1.,1.,1.,1.,1.,1.,1.,
1.,1.,1.,1.,1.,1.,1.,1.,1.,1.,1.,1.,1.,1.,1.,1.,1.,1.,1.,1.,1.,1.,1.,1.,
1.,1.,1.,1.,1.,1.,1.,1.,1.,1.,1.,1.,1.,1.,1.,1.,1.,1.,1.,1.,1.,1.,1.,1.,
1.,1.,1.,1.,1.,1.,1.,1.,1.,1.,1.,1.,1.,1.,1.,1.,1.,1.,1.,1.,1.,1.,1.,1.,
1.,1.,1.,1.,1.,1.,1.,1.,1.,1.,1.,1.,1.,1.,1.,1.,1.,1.,1.,1.,1.,1.,1.,1.,
1.,1.,1.,1.,1.,1.,1.,1.,1.,1.,1.,1.,1.,1.,1.,1.,1.,1.,1.,1.,1.,1.,1.,1.,
1.,1.,1.,1.,1.,1.,1.,1.,1.,1.,1.,1.,1.,1.,1.,1.,1.,1.,1.,1.,1.,1.,1.,1.,
1.,1.,1.,1.,1.,1.,1.,1.,1.,1.))
REPRESENTATION_ITEM('')
);
#664=(
BOUNDED_CURVE()
B_SPLINE_CURVE(5,(#164058,#164059,#164060,#164061,#164062,#164063,#164064,
#164065,#164066,#164067,#164068,#164069,#164070,#164071,#164072,#164073,
#164074,#164075,#164076,#164077,#164078,#164079,#164080,#164081,#164082,
#164083,#164084,#164085,#164086,#164087,#164088,#164089,#164090,#164091,
#164092,#164093,#164094,#164095,#164096,#164097,#164098,#164099,#164100,
#164101,#164102,#164103,#164104,#164105,#164106,#164107,#164108,#164109,
#164110,#164111,#164112,#164113,#164114,#164115,#164116,#164117,#164118,
#164119,#164120,#164121,#164122,#164123,#164124,#164125,#164126,#164127,
#164128,#164129,#164130,#164131,#164132,#164133,#164134,#164135,#164136,
#164137,#164138,#164139,#164140,#164141,#164142,#164143,#164144,#164145,
#164146,#164147,#164148,#164149,#164150,#164151,#164152,#164153,#164154,
#164155,#164156,#164157,#164158,#164159,#164160,#164161,#164162,#164163,
#164164,#164165,#164166,#164167,#164168,#164169,#164170,#164171,#164172,
#164173,#164174,#164175,#164176,#164177,#164178,#164179,#164180,#164181,
#164182,#164183,#164184,#164185,#164186,#164187,#164188,#164189,#164190,
#164191,#164192,#164193,#164194,#164195,#164196,#164197,#164198,#164199,
#164200,#164201,#164202,#164203,#164204,#164205,#164206,#164207,#164208,
#164209,#164210,#164211,#164212,#164213,#164214,#164215,#164216,#164217,
#164218,#164219,#164220,#164221,#164222,#164223,#164224,#164225,#164226,
#164227,#164228,#164229,#164230,#164231,#164232,#164233,#164234,#164235,
#164236,#164237,#164238,#164239,#164240,#164241,#164242,#164243,#164244,
#164245,#164246,#164247,#164248,#164249,#164250,#164251),.UNSPECIFIED.,
 .F.,.F.)
B_SPLINE_CURVE_WITH_KNOTS((6,1,1,1,1,1,1,1,1,1,1,1,1,1,1,1,1,1,1,1,1,1,
1,1,1,1,1,1,1,1,1,1,1,1,1,1,1,1,1,1,1,1,1,1,1,1,1,1,1,1,1,1,1,1,1,1,1,1,
1,1,1,1,1,1,1,1,1,1,1,1,1,1,1,1,1,1,1,1,1,1,1,1,1,1,1,1,1,1,1,1,1,1,1,1,
1,1,1,1,1,1,1,1,1,1,1,1,1,1,1,1,1,1,1,1,1,1,1,1,1,1,1,1,1,1,1,1,1,1,1,1,
1,1,1,1,1,1,1,1,1,1,1,1,1,1,1,1,1,1,1,1,1,1,1,1,1,1,1,1,1,1,1,1,1,1,1,1,
1,1,1,1,1,1,1,1,1,1,1,1,1,1,1,1,1,1,1,1,1,1,1,6),(-0.941429844437967,-0.940000000000001,
-0.935000000000001,-0.930000000000001,-0.925000000000001,-0.920000000000001,
-0.915000000000001,-0.910000000000001,-0.905000000000001,-0.900000000000001,
-0.895000000000001,-0.890000000000001,-0.885000000000001,-0.880000000000001,
-0.875000000000001,-0.870000000000001,-0.865000000000001,-0.860000000000001,
-0.855000000000001,-0.850000000000001,-0.845000000000001,-0.840000000000001,
-0.835000000000001,-0.830000000000001,-0.825000000000001,-0.820000000000001,
-0.815000000000001,-0.810000000000001,-0.805000000000001,-0.800000000000001,
-0.795000000000001,-0.790000000000001,-0.785000000000001,-0.780000000000001,
-0.775000000000001,-0.770000000000001,-0.765000000000001,-0.760000000000001,
-0.755000000000001,-0.750000000000001,-0.745000000000001,-0.740000000000001,
-0.735000000000001,-0.730000000000001,-0.725000000000001,-0.720000000000001,
-0.715000000000001,-0.710000000000001,-0.705000000000001,-0.700000000000001,
-0.695000000000001,-0.690000000000001,-0.685,-0.68,-0.675,-0.67,-0.665,
-0.66,-0.655,-0.65,-0.645,-0.64,-0.635,-0.63,-0.625,-0.62,-0.615,-0.61,
-0.605,-0.6,-0.595,-0.59,-0.585,-0.58,-0.575,-0.57,-0.565,-0.56,-0.555,
-0.55,-0.545,-0.54,-0.535,-0.53,-0.525,-0.52,-0.515,-0.51,-0.505,-0.5,-0.495,
-0.49,-0.485,-0.48,-0.475,-0.47,-0.465,-0.46,-0.455,-0.45,-0.445,-0.44,
-0.435,-0.43,-0.425,-0.42,-0.415,-0.41,-0.405,-0.4,-0.395,-0.39,-0.385,
-0.38,-0.375,-0.37,-0.365,-0.36,-0.355,-0.35,-0.345,-0.34,-0.335,-0.33,
-0.325,-0.32,-0.315,-0.31,-0.305,-0.3,-0.295,-0.29,-0.285,-0.28,-0.275,
-0.27,-0.265,-0.26,-0.255,-0.25,-0.245,-0.24,-0.235,-0.23,-0.225,-0.22,
-0.215,-0.21,-0.205,-0.2,-0.195,-0.19,-0.185,-0.18,-0.175,-0.17,-0.165,
-0.16,-0.155,-0.15,-0.145,-0.14,-0.135,-0.13,-0.125,-0.12,-0.115,-0.11,
-0.105,-0.1,-0.095,-0.09,-0.085,-0.08,-0.075,-0.07,-0.065,-0.06,-0.055,
-0.05,-0.045,-0.04,-0.035,-0.03,-0.025,-0.02,-0.015,-0.01,-0.005,0.),
 .UNSPECIFIED.)
CURVE()
GEOMETRIC_REPRESENTATION_ITEM()
RATIONAL_B_SPLINE_CURVE((1.,1.,1.,1.,1.,1.,1.,1.,1.,1.,1.,1.,1.,1.,1.,1.,
1.,1.,1.,1.,1.,1.,1.,1.,1.,1.,1.,1.,1.,1.,1.,1.,1.,1.,1.,1.,1.,1.,1.,1.,
1.,1.,1.,1.,1.,1.,1.,1.,1.,1.,1.,1.,1.,1.,1.,1.,1.,1.,1.,1.,1.,1.,1.,1.,
1.,1.,1.,1.,1.,1.,1.,1.,1.,1.,1.,1.,1.,1.,1.,1.,1.,1.,1.,1.,1.,1.,1.,1.,
1.,1.,1.,1.,1.,1.,1.,1.,1.,1.,1.,1.,1.,1.,1.,1.,1.,1.,1.,1.,1.,1.,1.,1.,
1.,1.,1.,1.,1.,1.,1.,1.,1.,1.,1.,1.,1.,1.,1.,1.,1.,1.,1.,1.,1.,1.,1.,1.,
1.,1.,1.,1.,1.,1.,1.,1.,1.,1.,1.,1.,1.,1.,1.,1.,1.,1.,1.,1.,1.,1.,1.,1.,
1.,1.,1.,1.,1.,1.,1.,1.,1.,1.,1.,1.,1.,1.,1.,1.,1.,1.,1.,1.,1.,1.,1.,1.,
1.,1.,1.,1.,1.,1.,1.,1.,1.,1.))
REPRESENTATION_ITEM('')
);
#665=(
BOUNDED_CURVE()
B_SPLINE_CURVE(5,(#164663,#164664,#164665,#164666,#164667,#164668,#164669,
#164670,#164671,#164672,#164673,#164674,#164675,#164676,#164677,#164678,
#164679,#164680,#164681,#164682,#164683,#164684,#164685,#164686,#164687,
#164688,#164689,#164690,#164691,#164692,#164693,#164694,#164695,#164696,
#164697,#164698,#164699,#164700,#164701,#164702,#164703,#164704,#164705,
#164706,#164707,#164708,#164709,#164710,#164711,#164712,#164713,#164714,
#164715,#164716,#164717,#164718,#164719,#164720,#164721,#164722,#164723,
#164724,#164725,#164726,#164727,#164728,#164729,#164730,#164731,#164732,
#164733,#164734,#164735,#164736,#164737,#164738,#164739,#164740,#164741,
#164742,#164743,#164744,#164745,#164746,#164747,#164748,#164749,#164750,
#164751,#164752,#164753,#164754,#164755,#164756,#164757,#164758,#164759,
#164760,#164761,#164762,#164763,#164764,#164765,#164766,#164767,#164768,
#164769,#164770,#164771,#164772,#164773,#164774,#164775,#164776,#164777,
#164778,#164779,#164780,#164781,#164782,#164783,#164784,#164785,#164786,
#164787,#164788,#164789,#164790,#164791,#164792,#164793,#164794,#164795,
#164796,#164797,#164798,#164799,#164800,#164801,#164802,#164803,#164804,
#164805,#164806,#164807,#164808,#164809,#164810,#164811,#164812,#164813,
#164814,#164815,#164816,#164817,#164818,#164819,#164820,#164821,#164822,
#164823,#164824,#164825,#164826,#164827,#164828,#164829,#164830,#164831,
#164832,#164833,#164834,#164835,#164836,#164837,#164838,#164839,#164840,
#164841,#164842,#164843,#164844,#164845,#164846,#164847,#164848,#164849,
#164850,#164851,#164852,#164853,#164854,#164855,#164856),.UNSPECIFIED.,
 .F.,.F.)
B_SPLINE_CURVE_WITH_KNOTS((6,1,1,1,1,1,1,1,1,1,1,1,1,1,1,1,1,1,1,1,1,1,
1,1,1,1,1,1,1,1,1,1,1,1,1,1,1,1,1,1,1,1,1,1,1,1,1,1,1,1,1,1,1,1,1,1,1,1,
1,1,1,1,1,1,1,1,1,1,1,1,1,1,1,1,1,1,1,1,1,1,1,1,1,1,1,1,1,1,1,1,1,1,1,1,
1,1,1,1,1,1,1,1,1,1,1,1,1,1,1,1,1,1,1,1,1,1,1,1,1,1,1,1,1,1,1,1,1,1,1,1,
1,1,1,1,1,1,1,1,1,1,1,1,1,1,1,1,1,1,1,1,1,1,1,1,1,1,1,1,1,1,1,1,1,1,1,1,
1,1,1,1,1,1,1,1,1,1,1,1,1,1,1,1,1,1,1,1,1,1,1,6),(0.,0.005,0.01,0.015,0.02,
0.025,0.03,0.035,0.04,0.045,0.05,0.055,0.06,0.065,0.07,0.075,0.08,0.085,
0.09,0.095,0.1,0.105,0.11,0.115,0.12,0.125,0.13,0.135,0.14,0.145,0.15,0.155,
0.16,0.165,0.17,0.175,0.18,0.185,0.19,0.195,0.2,0.205,0.21,0.215,0.22,0.225,
0.23,0.235,0.24,0.245,0.25,0.255,0.26,0.265,0.27,0.275,0.28,0.285,0.29,
0.295,0.3,0.305,0.31,0.315,0.32,0.325,0.33,0.335,0.34,0.345,0.35,0.355,
0.36,0.365,0.37,0.375,0.38,0.385,0.39,0.395,0.4,0.405,0.41,0.415,0.42,0.425,
0.43,0.435,0.44,0.445,0.45,0.455,0.46,0.465,0.47,0.475,0.48,0.485,0.49,
0.495,0.5,0.505,0.51,0.515,0.52,0.525,0.53,0.535,0.54,0.545,0.55,0.555,
0.56,0.565,0.57,0.575,0.58,0.585,0.59,0.595,0.6,0.605,0.61,0.615,0.62,0.625,
0.63,0.635,0.64,0.645,0.65,0.655,0.66,0.665,0.67,0.675,0.68,0.685,0.690000000000001,
0.695000000000001,0.700000000000001,0.705000000000001,0.710000000000001,
0.715000000000001,0.720000000000001,0.725000000000001,0.730000000000001,
0.735000000000001,0.740000000000001,0.745000000000001,0.750000000000001,
0.755000000000001,0.760000000000001,0.765000000000001,0.770000000000001,
0.775000000000001,0.780000000000001,0.785000000000001,0.790000000000001,
0.795000000000001,0.800000000000001,0.805000000000001,0.810000000000001,
0.815000000000001,0.820000000000001,0.825000000000001,0.830000000000001,
0.835000000000001,0.840000000000001,0.845000000000001,0.850000000000001,
0.855000000000001,0.860000000000001,0.865000000000001,0.870000000000001,
0.875000000000001,0.880000000000001,0.885000000000001,0.890000000000001,
0.895000000000001,0.900000000000001,0.905000000000001,0.910000000000001,
0.915000000000001,0.920000000000001,0.925000000000001,0.930000000000001,
0.935000000000001,0.940000000000001,0.941429844438043),.UNSPECIFIED.)
CURVE()
GEOMETRIC_REPRESENTATION_ITEM()
RATIONAL_B_SPLINE_CURVE((1.,1.,1.,1.,1.,1.,1.,1.,1.,1.,1.,1.,1.,1.,1.,1.,
1.,1.,1.,1.,1.,1.,1.,1.,1.,1.,1.,1.,1.,1.,1.,1.,1.,1.,1.,1.,1.,1.,1.,1.,
1.,1.,1.,1.,1.,1.,1.,1.,1.,1.,1.,1.,1.,1.,1.,1.,1.,1.,1.,1.,1.,1.,1.,1.,
1.,1.,1.,1.,1.,1.,1.,1.,1.,1.,1.,1.,1.,1.,1.,1.,1.,1.,1.,1.,1.,1.,1.,1.,
1.,1.,1.,1.,1.,1.,1.,1.,1.,1.,1.,1.,1.,1.,1.,1.,1.,1.,1.,1.,1.,1.,1.,1.,
1.,1.,1.,1.,1.,1.,1.,1.,1.,1.,1.,1.,1.,1.,1.,1.,1.,1.,1.,1.,1.,1.,1.,1.,
1.,1.,1.,1.,1.,1.,1.,1.,1.,1.,1.,1.,1.,1.,1.,1.,1.,1.,1.,1.,1.,1.,1.,1.,
1.,1.,1.,1.,1.,1.,1.,1.,1.,1.,1.,1.,1.,1.,1.,1.,1.,1.,1.,1.,1.,1.,1.,1.,
1.,1.,1.,1.,1.,1.,1.,1.,1.,1.))
REPRESENTATION_ITEM('')
);
#666=(
BOUNDED_CURVE()
B_SPLINE_CURVE(5,(#164859,#164860,#164861,#164862,#164863,#164864,#164865,
#164866,#164867,#164868,#164869,#164870,#164871,#164872,#164873,#164874,
#164875,#164876,#164877,#164878,#164879,#164880,#164881,#164882,#164883,
#164884,#164885,#164886,#164887,#164888,#164889,#164890,#164891,#164892,
#164893,#164894,#164895,#164896,#164897,#164898,#164899,#164900,#164901,
#164902,#164903,#164904,#164905,#164906,#164907,#164908,#164909,#164910,
#164911,#164912,#164913,#164914,#164915,#164916,#164917,#164918,#164919,
#164920,#164921,#164922,#164923,#164924,#164925,#164926,#164927,#164928,
#164929,#164930,#164931,#164932,#164933,#164934,#164935,#164936,#164937,
#164938,#164939,#164940,#164941,#164942,#164943,#164944,#164945,#164946,
#164947,#164948,#164949,#164950,#164951,#164952,#164953,#164954,#164955,
#164956,#164957,#164958,#164959,#164960,#164961,#164962,#164963,#164964,
#164965,#164966,#164967,#164968,#164969,#164970,#164971,#164972,#164973,
#164974,#164975,#164976,#164977,#164978,#164979,#164980,#164981,#164982,
#164983,#164984,#164985,#164986,#164987,#164988,#164989,#164990,#164991,
#164992,#164993,#164994,#164995,#164996,#164997,#164998,#164999,#165000,
#165001,#165002,#165003,#165004,#165005,#165006,#165007,#165008,#165009,
#165010,#165011,#165012,#165013,#165014,#165015,#165016,#165017,#165018,
#165019,#165020,#165021,#165022,#165023,#165024,#165025,#165026,#165027,
#165028,#165029,#165030,#165031,#165032,#165033,#165034,#165035,#165036,
#165037,#165038,#165039,#165040,#165041,#165042,#165043,#165044,#165045,
#165046,#165047,#165048,#165049,#165050,#165051,#165052),.UNSPECIFIED.,
 .F.,.F.)
B_SPLINE_CURVE_WITH_KNOTS((6,1,1,1,1,1,1,1,1,1,1,1,1,1,1,1,1,1,1,1,1,1,
1,1,1,1,1,1,1,1,1,1,1,1,1,1,1,1,1,1,1,1,1,1,1,1,1,1,1,1,1,1,1,1,1,1,1,1,
1,1,1,1,1,1,1,1,1,1,1,1,1,1,1,1,1,1,1,1,1,1,1,1,1,1,1,1,1,1,1,1,1,1,1,1,
1,1,1,1,1,1,1,1,1,1,1,1,1,1,1,1,1,1,1,1,1,1,1,1,1,1,1,1,1,1,1,1,1,1,1,1,
1,1,1,1,1,1,1,1,1,1,1,1,1,1,1,1,1,1,1,1,1,1,1,1,1,1,1,1,1,1,1,1,1,1,1,1,
1,1,1,1,1,1,1,1,1,1,1,1,1,1,1,1,1,1,1,1,1,1,1,6),(-0.941429844438042,-0.940000000000001,
-0.935000000000001,-0.930000000000001,-0.925000000000001,-0.920000000000001,
-0.915000000000001,-0.910000000000001,-0.905000000000001,-0.900000000000001,
-0.895000000000001,-0.890000000000001,-0.885000000000001,-0.880000000000001,
-0.875000000000001,-0.870000000000001,-0.865000000000001,-0.860000000000001,
-0.855000000000001,-0.850000000000001,-0.845000000000001,-0.840000000000001,
-0.835000000000001,-0.830000000000001,-0.825000000000001,-0.820000000000001,
-0.815000000000001,-0.810000000000001,-0.805000000000001,-0.800000000000001,
-0.795000000000001,-0.790000000000001,-0.785000000000001,-0.780000000000001,
-0.775000000000001,-0.770000000000001,-0.765000000000001,-0.760000000000001,
-0.755000000000001,-0.750000000000001,-0.745000000000001,-0.740000000000001,
-0.735000000000001,-0.730000000000001,-0.725000000000001,-0.720000000000001,
-0.715000000000001,-0.710000000000001,-0.705000000000001,-0.700000000000001,
-0.695000000000001,-0.690000000000001,-0.685,-0.68,-0.675,-0.67,-0.665,
-0.66,-0.655,-0.65,-0.645,-0.64,-0.635,-0.63,-0.625,-0.62,-0.615,-0.61,
-0.605,-0.6,-0.595,-0.59,-0.585,-0.58,-0.575,-0.57,-0.565,-0.56,-0.555,
-0.55,-0.545,-0.54,-0.535,-0.53,-0.525,-0.52,-0.515,-0.51,-0.505,-0.5,-0.495,
-0.49,-0.485,-0.48,-0.475,-0.47,-0.465,-0.46,-0.455,-0.45,-0.445,-0.44,
-0.435,-0.43,-0.425,-0.42,-0.415,-0.41,-0.405,-0.4,-0.395,-0.39,-0.385,
-0.38,-0.375,-0.37,-0.365,-0.36,-0.355,-0.35,-0.345,-0.34,-0.335,-0.33,
-0.325,-0.32,-0.315,-0.31,-0.305,-0.3,-0.295,-0.29,-0.285,-0.28,-0.275,
-0.27,-0.265,-0.26,-0.255,-0.25,-0.245,-0.24,-0.235,-0.23,-0.225,-0.22,
-0.215,-0.21,-0.205,-0.2,-0.195,-0.19,-0.185,-0.18,-0.175,-0.17,-0.165,
-0.16,-0.155,-0.15,-0.145,-0.14,-0.135,-0.13,-0.125,-0.12,-0.115,-0.11,
-0.105,-0.1,-0.095,-0.09,-0.085,-0.08,-0.075,-0.07,-0.065,-0.06,-0.055,
-0.05,-0.045,-0.04,-0.035,-0.03,-0.025,-0.02,-0.015,-0.01,-0.005,0.),
 .UNSPECIFIED.)
CURVE()
GEOMETRIC_REPRESENTATION_ITEM()
RATIONAL_B_SPLINE_CURVE((1.,1.,1.,1.,1.,1.,1.,1.,1.,1.,1.,1.,1.,1.,1.,1.,
1.,1.,1.,1.,1.,1.,1.,1.,1.,1.,1.,1.,1.,1.,1.,1.,1.,1.,1.,1.,1.,1.,1.,1.,
1.,1.,1.,1.,1.,1.,1.,1.,1.,1.,1.,1.,1.,1.,1.,1.,1.,1.,1.,1.,1.,1.,1.,1.,
1.,1.,1.,1.,1.,1.,1.,1.,1.,1.,1.,1.,1.,1.,1.,1.,1.,1.,1.,1.,1.,1.,1.,1.,
1.,1.,1.,1.,1.,1.,1.,1.,1.,1.,1.,1.,1.,1.,1.,1.,1.,1.,1.,1.,1.,1.,1.,1.,
1.,1.,1.,1.,1.,1.,1.,1.,1.,1.,1.,1.,1.,1.,1.,1.,1.,1.,1.,1.,1.,1.,1.,1.,
1.,1.,1.,1.,1.,1.,1.,1.,1.,1.,1.,1.,1.,1.,1.,1.,1.,1.,1.,1.,1.,1.,1.,1.,
1.,1.,1.,1.,1.,1.,1.,1.,1.,1.,1.,1.,1.,1.,1.,1.,1.,1.,1.,1.,1.,1.,1.,1.,
1.,1.,1.,1.,1.,1.,1.,1.,1.,1.))
REPRESENTATION_ITEM('')
);
#667=(
BOUNDED_CURVE()
B_SPLINE_CURVE(5,(#165464,#165465,#165466,#165467,#165468,#165469,#165470,
#165471,#165472,#165473,#165474,#165475,#165476,#165477,#165478,#165479,
#165480,#165481,#165482,#165483,#165484,#165485,#165486,#165487,#165488,
#165489,#165490,#165491,#165492,#165493,#165494,#165495,#165496,#165497,
#165498,#165499,#165500,#165501,#165502,#165503,#165504,#165505,#165506,
#165507,#165508,#165509,#165510,#165511,#165512,#165513,#165514,#165515,
#165516,#165517,#165518,#165519,#165520,#165521,#165522,#165523,#165524,
#165525,#165526,#165527,#165528,#165529,#165530,#165531,#165532,#165533,
#165534,#165535,#165536,#165537,#165538,#165539,#165540,#165541,#165542,
#165543,#165544,#165545,#165546,#165547,#165548,#165549,#165550,#165551,
#165552,#165553,#165554,#165555,#165556,#165557,#165558,#165559,#165560,
#165561,#165562,#165563,#165564,#165565,#165566,#165567,#165568,#165569,
#165570,#165571,#165572,#165573,#165574,#165575,#165576,#165577,#165578,
#165579,#165580,#165581,#165582,#165583,#165584,#165585,#165586,#165587,
#165588,#165589,#165590,#165591,#165592,#165593,#165594,#165595,#165596,
#165597,#165598,#165599,#165600,#165601,#165602,#165603,#165604,#165605,
#165606,#165607,#165608,#165609,#165610,#165611,#165612,#165613,#165614,
#165615,#165616,#165617,#165618,#165619,#165620,#165621,#165622,#165623,
#165624,#165625,#165626,#165627,#165628,#165629,#165630,#165631,#165632,
#165633,#165634,#165635,#165636,#165637,#165638,#165639,#165640,#165641,
#165642,#165643,#165644,#165645,#165646,#165647,#165648,#165649,#165650,
#165651,#165652,#165653,#165654,#165655,#165656,#165657),.UNSPECIFIED.,
 .F.,.F.)
B_SPLINE_CURVE_WITH_KNOTS((6,1,1,1,1,1,1,1,1,1,1,1,1,1,1,1,1,1,1,1,1,1,
1,1,1,1,1,1,1,1,1,1,1,1,1,1,1,1,1,1,1,1,1,1,1,1,1,1,1,1,1,1,1,1,1,1,1,1,
1,1,1,1,1,1,1,1,1,1,1,1,1,1,1,1,1,1,1,1,1,1,1,1,1,1,1,1,1,1,1,1,1,1,1,1,
1,1,1,1,1,1,1,1,1,1,1,1,1,1,1,1,1,1,1,1,1,1,1,1,1,1,1,1,1,1,1,1,1,1,1,1,
1,1,1,1,1,1,1,1,1,1,1,1,1,1,1,1,1,1,1,1,1,1,1,1,1,1,1,1,1,1,1,1,1,1,1,1,
1,1,1,1,1,1,1,1,1,1,1,1,1,1,1,1,1,1,1,1,1,1,1,6),(0.,0.005,0.01,0.015,0.02,
0.025,0.03,0.035,0.04,0.045,0.05,0.055,0.06,0.065,0.07,0.075,0.08,0.085,
0.09,0.095,0.1,0.105,0.11,0.115,0.12,0.125,0.13,0.135,0.14,0.145,0.15,0.155,
0.16,0.165,0.17,0.175,0.18,0.185,0.19,0.195,0.2,0.205,0.21,0.215,0.22,0.225,
0.23,0.235,0.24,0.245,0.25,0.255,0.26,0.265,0.27,0.275,0.28,0.285,0.29,
0.295,0.3,0.305,0.31,0.315,0.32,0.325,0.33,0.335,0.34,0.345,0.35,0.355,
0.36,0.365,0.37,0.375,0.38,0.385,0.39,0.395,0.4,0.405,0.41,0.415,0.42,0.425,
0.43,0.435,0.44,0.445,0.45,0.455,0.46,0.465,0.47,0.475,0.48,0.485,0.49,
0.495,0.5,0.505,0.51,0.515,0.52,0.525,0.53,0.535,0.54,0.545,0.55,0.555,
0.56,0.565,0.57,0.575,0.58,0.585,0.59,0.595,0.6,0.605,0.61,0.615,0.62,0.625,
0.63,0.635,0.64,0.645,0.65,0.655,0.66,0.665,0.67,0.675,0.68,0.685,0.690000000000001,
0.695000000000001,0.700000000000001,0.705000000000001,0.710000000000001,
0.715000000000001,0.720000000000001,0.725000000000001,0.730000000000001,
0.735000000000001,0.740000000000001,0.745000000000001,0.750000000000001,
0.755000000000001,0.760000000000001,0.765000000000001,0.770000000000001,
0.775000000000001,0.780000000000001,0.785000000000001,0.790000000000001,
0.795000000000001,0.800000000000001,0.805000000000001,0.810000000000001,
0.815000000000001,0.820000000000001,0.825000000000001,0.830000000000001,
0.835000000000001,0.840000000000001,0.845000000000001,0.850000000000001,
0.855000000000001,0.860000000000001,0.865000000000001,0.870000000000001,
0.875000000000001,0.880000000000001,0.885000000000001,0.890000000000001,
0.895000000000001,0.900000000000001,0.905000000000001,0.910000000000001,
0.915000000000001,0.920000000000001,0.925000000000001,0.930000000000001,
0.935000000000001,0.940000000000001,0.941429844438172),.UNSPECIFIED.)
CURVE()
GEOMETRIC_REPRESENTATION_ITEM()
RATIONAL_B_SPLINE_CURVE((1.,1.,1.,1.,1.,1.,1.,1.,1.,1.,1.,1.,1.,1.,1.,1.,
1.,1.,1.,1.,1.,1.,1.,1.,1.,1.,1.,1.,1.,1.,1.,1.,1.,1.,1.,1.,1.,1.,1.,1.,
1.,1.,1.,1.,1.,1.,1.,1.,1.,1.,1.,1.,1.,1.,1.,1.,1.,1.,1.,1.,1.,1.,1.,1.,
1.,1.,1.,1.,1.,1.,1.,1.,1.,1.,1.,1.,1.,1.,1.,1.,1.,1.,1.,1.,1.,1.,1.,1.,
1.,1.,1.,1.,1.,1.,1.,1.,1.,1.,1.,1.,1.,1.,1.,1.,1.,1.,1.,1.,1.,1.,1.,1.,
1.,1.,1.,1.,1.,1.,1.,1.,1.,1.,1.,1.,1.,1.,1.,1.,1.,1.,1.,1.,1.,1.,1.,1.,
1.,1.,1.,1.,1.,1.,1.,1.,1.,1.,1.,1.,1.,1.,1.,1.,1.,1.,1.,1.,1.,1.,1.,1.,
1.,1.,1.,1.,1.,1.,1.,1.,1.,1.,1.,1.,1.,1.,1.,1.,1.,1.,1.,1.,1.,1.,1.,1.,
1.,1.,1.,1.,1.,1.,1.,1.,1.,1.))
REPRESENTATION_ITEM('')
);
#668=(
BOUNDED_CURVE()
B_SPLINE_CURVE(5,(#165660,#165661,#165662,#165663,#165664,#165665,#165666,
#165667,#165668,#165669,#165670,#165671,#165672,#165673,#165674,#165675,
#165676,#165677,#165678,#165679,#165680,#165681,#165682,#165683,#165684,
#165685,#165686,#165687,#165688,#165689,#165690,#165691,#165692,#165693,
#165694,#165695,#165696,#165697,#165698,#165699,#165700,#165701,#165702,
#165703,#165704,#165705,#165706,#165707,#165708,#165709,#165710,#165711,
#165712,#165713,#165714,#165715,#165716,#165717,#165718,#165719,#165720,
#165721,#165722,#165723,#165724,#165725,#165726,#165727,#165728,#165729,
#165730,#165731,#165732,#165733,#165734,#165735,#165736,#165737,#165738,
#165739,#165740,#165741,#165742,#165743,#165744,#165745,#165746,#165747,
#165748,#165749,#165750,#165751,#165752,#165753,#165754,#165755,#165756,
#165757,#165758,#165759,#165760,#165761,#165762,#165763,#165764,#165765,
#165766,#165767,#165768,#165769,#165770,#165771,#165772,#165773,#165774,
#165775,#165776,#165777,#165778,#165779,#165780,#165781,#165782,#165783,
#165784,#165785,#165786,#165787,#165788,#165789,#165790,#165791,#165792,
#165793,#165794,#165795,#165796,#165797,#165798,#165799,#165800,#165801,
#165802,#165803,#165804,#165805,#165806,#165807,#165808,#165809,#165810,
#165811,#165812,#165813,#165814,#165815,#165816,#165817,#165818,#165819,
#165820,#165821,#165822,#165823,#165824,#165825,#165826,#165827,#165828,
#165829,#165830,#165831,#165832,#165833,#165834,#165835,#165836,#165837,
#165838,#165839,#165840,#165841,#165842,#165843,#165844,#165845,#165846,
#165847,#165848,#165849,#165850,#165851,#165852,#165853),.UNSPECIFIED.,
 .F.,.F.)
B_SPLINE_CURVE_WITH_KNOTS((6,1,1,1,1,1,1,1,1,1,1,1,1,1,1,1,1,1,1,1,1,1,
1,1,1,1,1,1,1,1,1,1,1,1,1,1,1,1,1,1,1,1,1,1,1,1,1,1,1,1,1,1,1,1,1,1,1,1,
1,1,1,1,1,1,1,1,1,1,1,1,1,1,1,1,1,1,1,1,1,1,1,1,1,1,1,1,1,1,1,1,1,1,1,1,
1,1,1,1,1,1,1,1,1,1,1,1,1,1,1,1,1,1,1,1,1,1,1,1,1,1,1,1,1,1,1,1,1,1,1,1,
1,1,1,1,1,1,1,1,1,1,1,1,1,1,1,1,1,1,1,1,1,1,1,1,1,1,1,1,1,1,1,1,1,1,1,1,
1,1,1,1,1,1,1,1,1,1,1,1,1,1,1,1,1,1,1,1,1,1,1,6),(-0.941429844438172,-0.940000000000001,
-0.935000000000001,-0.930000000000001,-0.925000000000001,-0.920000000000001,
-0.915000000000001,-0.910000000000001,-0.905000000000001,-0.900000000000001,
-0.895000000000001,-0.890000000000001,-0.885000000000001,-0.880000000000001,
-0.875000000000001,-0.870000000000001,-0.865000000000001,-0.860000000000001,
-0.855000000000001,-0.850000000000001,-0.845000000000001,-0.840000000000001,
-0.835000000000001,-0.830000000000001,-0.825000000000001,-0.820000000000001,
-0.815000000000001,-0.810000000000001,-0.805000000000001,-0.800000000000001,
-0.795000000000001,-0.790000000000001,-0.785000000000001,-0.780000000000001,
-0.775000000000001,-0.770000000000001,-0.765000000000001,-0.760000000000001,
-0.755000000000001,-0.750000000000001,-0.745000000000001,-0.740000000000001,
-0.735000000000001,-0.730000000000001,-0.725000000000001,-0.720000000000001,
-0.715000000000001,-0.710000000000001,-0.705000000000001,-0.700000000000001,
-0.695000000000001,-0.690000000000001,-0.685,-0.68,-0.675,-0.67,-0.665,
-0.66,-0.655,-0.65,-0.645,-0.64,-0.635,-0.63,-0.625,-0.62,-0.615,-0.61,
-0.605,-0.6,-0.595,-0.59,-0.585,-0.58,-0.575,-0.57,-0.565,-0.56,-0.555,
-0.55,-0.545,-0.54,-0.535,-0.53,-0.525,-0.52,-0.515,-0.51,-0.505,-0.5,-0.495,
-0.49,-0.485,-0.48,-0.475,-0.47,-0.465,-0.46,-0.455,-0.45,-0.445,-0.44,
-0.435,-0.43,-0.425,-0.42,-0.415,-0.41,-0.405,-0.4,-0.395,-0.39,-0.385,
-0.38,-0.375,-0.37,-0.365,-0.36,-0.355,-0.35,-0.345,-0.34,-0.335,-0.33,
-0.325,-0.32,-0.315,-0.31,-0.305,-0.3,-0.295,-0.29,-0.285,-0.28,-0.275,
-0.27,-0.265,-0.26,-0.255,-0.25,-0.245,-0.24,-0.235,-0.23,-0.225,-0.22,
-0.215,-0.21,-0.205,-0.2,-0.195,-0.19,-0.185,-0.18,-0.175,-0.17,-0.165,
-0.16,-0.155,-0.15,-0.145,-0.14,-0.135,-0.13,-0.125,-0.12,-0.115,-0.11,
-0.105,-0.1,-0.095,-0.09,-0.085,-0.08,-0.075,-0.07,-0.065,-0.06,-0.055,
-0.05,-0.045,-0.04,-0.035,-0.03,-0.025,-0.02,-0.015,-0.01,-0.005,0.),
 .UNSPECIFIED.)
CURVE()
GEOMETRIC_REPRESENTATION_ITEM()
RATIONAL_B_SPLINE_CURVE((1.,1.,1.,1.,1.,1.,1.,1.,1.,1.,1.,1.,1.,1.,1.,1.,
1.,1.,1.,1.,1.,1.,1.,1.,1.,1.,1.,1.,1.,1.,1.,1.,1.,1.,1.,1.,1.,1.,1.,1.,
1.,1.,1.,1.,1.,1.,1.,1.,1.,1.,1.,1.,1.,1.,1.,1.,1.,1.,1.,1.,1.,1.,1.,1.,
1.,1.,1.,1.,1.,1.,1.,1.,1.,1.,1.,1.,1.,1.,1.,1.,1.,1.,1.,1.,1.,1.,1.,1.,
1.,1.,1.,1.,1.,1.,1.,1.,1.,1.,1.,1.,1.,1.,1.,1.,1.,1.,1.,1.,1.,1.,1.,1.,
1.,1.,1.,1.,1.,1.,1.,1.,1.,1.,1.,1.,1.,1.,1.,1.,1.,1.,1.,1.,1.,1.,1.,1.,
1.,1.,1.,1.,1.,1.,1.,1.,1.,1.,1.,1.,1.,1.,1.,1.,1.,1.,1.,1.,1.,1.,1.,1.,
1.,1.,1.,1.,1.,1.,1.,1.,1.,1.,1.,1.,1.,1.,1.,1.,1.,1.,1.,1.,1.,1.,1.,1.,
1.,1.,1.,1.,1.,1.,1.,1.,1.,1.))
REPRESENTATION_ITEM('')
);
#669=(
BOUNDED_CURVE()
B_SPLINE_CURVE(5,(#166265,#166266,#166267,#166268,#166269,#166270,#166271,
#166272,#166273,#166274,#166275,#166276,#166277,#166278,#166279,#166280,
#166281,#166282,#166283,#166284,#166285,#166286,#166287,#166288,#166289,
#166290,#166291,#166292,#166293,#166294,#166295,#166296,#166297,#166298,
#166299,#166300,#166301,#166302,#166303,#166304,#166305,#166306,#166307,
#166308,#166309,#166310,#166311,#166312,#166313,#166314,#166315,#166316,
#166317,#166318,#166319,#166320,#166321,#166322,#166323,#166324,#166325,
#166326,#166327,#166328,#166329,#166330,#166331,#166332,#166333,#166334,
#166335,#166336,#166337,#166338,#166339,#166340,#166341,#166342,#166343,
#166344,#166345,#166346,#166347,#166348,#166349,#166350,#166351,#166352,
#166353,#166354,#166355,#166356,#166357,#166358,#166359,#166360,#166361,
#166362,#166363,#166364,#166365,#166366,#166367,#166368,#166369,#166370,
#166371,#166372,#166373,#166374,#166375,#166376,#166377,#166378,#166379,
#166380,#166381,#166382,#166383,#166384,#166385,#166386,#166387,#166388,
#166389,#166390,#166391,#166392,#166393,#166394,#166395,#166396,#166397,
#166398,#166399,#166400,#166401,#166402,#166403,#166404,#166405,#166406,
#166407,#166408,#166409,#166410,#166411,#166412,#166413,#166414,#166415,
#166416,#166417,#166418,#166419,#166420,#166421,#166422,#166423,#166424,
#166425,#166426,#166427,#166428,#166429,#166430,#166431,#166432,#166433,
#166434,#166435,#166436,#166437,#166438,#166439,#166440,#166441,#166442,
#166443,#166444,#166445,#166446,#166447,#166448,#166449,#166450,#166451,
#166452,#166453,#166454,#166455,#166456,#166457,#166458),.UNSPECIFIED.,
 .F.,.F.)
B_SPLINE_CURVE_WITH_KNOTS((6,1,1,1,1,1,1,1,1,1,1,1,1,1,1,1,1,1,1,1,1,1,
1,1,1,1,1,1,1,1,1,1,1,1,1,1,1,1,1,1,1,1,1,1,1,1,1,1,1,1,1,1,1,1,1,1,1,1,
1,1,1,1,1,1,1,1,1,1,1,1,1,1,1,1,1,1,1,1,1,1,1,1,1,1,1,1,1,1,1,1,1,1,1,1,
1,1,1,1,1,1,1,1,1,1,1,1,1,1,1,1,1,1,1,1,1,1,1,1,1,1,1,1,1,1,1,1,1,1,1,1,
1,1,1,1,1,1,1,1,1,1,1,1,1,1,1,1,1,1,1,1,1,1,1,1,1,1,1,1,1,1,1,1,1,1,1,1,
1,1,1,1,1,1,1,1,1,1,1,1,1,1,1,1,1,1,1,1,1,1,1,6),(0.,0.005,0.01,0.015,0.02,
0.025,0.03,0.035,0.04,0.045,0.05,0.055,0.06,0.065,0.07,0.075,0.08,0.085,
0.09,0.095,0.1,0.105,0.11,0.115,0.12,0.125,0.13,0.135,0.14,0.145,0.15,0.155,
0.16,0.165,0.17,0.175,0.18,0.185,0.19,0.195,0.2,0.205,0.21,0.215,0.22,0.225,
0.23,0.235,0.24,0.245,0.25,0.255,0.26,0.265,0.27,0.275,0.28,0.285,0.29,
0.295,0.3,0.305,0.31,0.315,0.32,0.325,0.33,0.335,0.34,0.345,0.35,0.355,
0.36,0.365,0.37,0.375,0.38,0.385,0.39,0.395,0.4,0.405,0.41,0.415,0.42,0.425,
0.43,0.435,0.44,0.445,0.45,0.455,0.46,0.465,0.47,0.475,0.48,0.485,0.49,
0.495,0.5,0.505,0.51,0.515,0.52,0.525,0.53,0.535,0.54,0.545,0.55,0.555,
0.56,0.565,0.57,0.575,0.58,0.585,0.59,0.595,0.6,0.605,0.61,0.615,0.62,0.625,
0.63,0.635,0.64,0.645,0.65,0.655,0.66,0.665,0.67,0.675,0.68,0.685,0.690000000000001,
0.695000000000001,0.700000000000001,0.705000000000001,0.710000000000001,
0.715000000000001,0.720000000000001,0.725000000000001,0.730000000000001,
0.735000000000001,0.740000000000001,0.745000000000001,0.750000000000001,
0.755000000000001,0.760000000000001,0.765000000000001,0.770000000000001,
0.775000000000001,0.780000000000001,0.785000000000001,0.790000000000001,
0.795000000000001,0.800000000000001,0.805000000000001,0.810000000000001,
0.815000000000001,0.820000000000001,0.825000000000001,0.830000000000001,
0.835000000000001,0.840000000000001,0.845000000000001,0.850000000000001,
0.855000000000001,0.860000000000001,0.865000000000001,0.870000000000001,
0.875000000000001,0.880000000000001,0.885000000000001,0.890000000000001,
0.895000000000001,0.900000000000001,0.905000000000001,0.910000000000001,
0.915000000000001,0.920000000000001,0.925000000000001,0.930000000000001,
0.935000000000001,0.940000000000001,0.94142984443799),.UNSPECIFIED.)
CURVE()
GEOMETRIC_REPRESENTATION_ITEM()
RATIONAL_B_SPLINE_CURVE((1.,1.,1.,1.,1.,1.,1.,1.,1.,1.,1.,1.,1.,1.,1.,1.,
1.,1.,1.,1.,1.,1.,1.,1.,1.,1.,1.,1.,1.,1.,1.,1.,1.,1.,1.,1.,1.,1.,1.,1.,
1.,1.,1.,1.,1.,1.,1.,1.,1.,1.,1.,1.,1.,1.,1.,1.,1.,1.,1.,1.,1.,1.,1.,1.,
1.,1.,1.,1.,1.,1.,1.,1.,1.,1.,1.,1.,1.,1.,1.,1.,1.,1.,1.,1.,1.,1.,1.,1.,
1.,1.,1.,1.,1.,1.,1.,1.,1.,1.,1.,1.,1.,1.,1.,1.,1.,1.,1.,1.,1.,1.,1.,1.,
1.,1.,1.,1.,1.,1.,1.,1.,1.,1.,1.,1.,1.,1.,1.,1.,1.,1.,1.,1.,1.,1.,1.,1.,
1.,1.,1.,1.,1.,1.,1.,1.,1.,1.,1.,1.,1.,1.,1.,1.,1.,1.,1.,1.,1.,1.,1.,1.,
1.,1.,1.,1.,1.,1.,1.,1.,1.,1.,1.,1.,1.,1.,1.,1.,1.,1.,1.,1.,1.,1.,1.,1.,
1.,1.,1.,1.,1.,1.,1.,1.,1.,1.))
REPRESENTATION_ITEM('')
);
#670=(
BOUNDED_CURVE()
B_SPLINE_CURVE(5,(#166461,#166462,#166463,#166464,#166465,#166466,#166467,
#166468,#166469,#166470,#166471,#166472,#166473,#166474,#166475,#166476,
#166477,#166478,#166479,#166480,#166481,#166482,#166483,#166484,#166485,
#166486,#166487,#166488,#166489,#166490,#166491,#166492,#166493,#166494,
#166495,#166496,#166497,#166498,#166499,#166500,#166501,#166502,#166503,
#166504,#166505,#166506,#166507,#166508,#166509,#166510,#166511,#166512,
#166513,#166514,#166515,#166516,#166517,#166518,#166519,#166520,#166521,
#166522,#166523,#166524,#166525,#166526,#166527,#166528,#166529,#166530,
#166531,#166532,#166533,#166534,#166535,#166536,#166537,#166538,#166539,
#166540,#166541,#166542,#166543,#166544,#166545,#166546,#166547,#166548,
#166549,#166550,#166551,#166552,#166553,#166554,#166555,#166556,#166557,
#166558,#166559,#166560,#166561,#166562,#166563,#166564,#166565,#166566,
#166567,#166568,#166569,#166570,#166571,#166572,#166573,#166574,#166575,
#166576,#166577,#166578,#166579,#166580,#166581,#166582,#166583,#166584,
#166585,#166586,#166587,#166588,#166589,#166590,#166591,#166592,#166593,
#166594,#166595,#166596,#166597,#166598,#166599,#166600,#166601,#166602,
#166603,#166604,#166605,#166606,#166607,#166608,#166609,#166610,#166611,
#166612,#166613,#166614,#166615,#166616,#166617,#166618,#166619,#166620,
#166621,#166622,#166623,#166624,#166625,#166626,#166627,#166628,#166629,
#166630,#166631,#166632,#166633,#166634,#166635,#166636,#166637,#166638,
#166639,#166640,#166641,#166642,#166643,#166644,#166645,#166646,#166647,
#166648,#166649,#166650,#166651,#166652,#166653,#166654),.UNSPECIFIED.,
 .F.,.F.)
B_SPLINE_CURVE_WITH_KNOTS((6,1,1,1,1,1,1,1,1,1,1,1,1,1,1,1,1,1,1,1,1,1,
1,1,1,1,1,1,1,1,1,1,1,1,1,1,1,1,1,1,1,1,1,1,1,1,1,1,1,1,1,1,1,1,1,1,1,1,
1,1,1,1,1,1,1,1,1,1,1,1,1,1,1,1,1,1,1,1,1,1,1,1,1,1,1,1,1,1,1,1,1,1,1,1,
1,1,1,1,1,1,1,1,1,1,1,1,1,1,1,1,1,1,1,1,1,1,1,1,1,1,1,1,1,1,1,1,1,1,1,1,
1,1,1,1,1,1,1,1,1,1,1,1,1,1,1,1,1,1,1,1,1,1,1,1,1,1,1,1,1,1,1,1,1,1,1,1,
1,1,1,1,1,1,1,1,1,1,1,1,1,1,1,1,1,1,1,1,1,1,1,6),(-0.941429844437991,-0.940000000000001,
-0.935000000000001,-0.930000000000001,-0.925000000000001,-0.920000000000001,
-0.915000000000001,-0.910000000000001,-0.905000000000001,-0.900000000000001,
-0.895000000000001,-0.890000000000001,-0.885000000000001,-0.880000000000001,
-0.875000000000001,-0.870000000000001,-0.865000000000001,-0.860000000000001,
-0.855000000000001,-0.850000000000001,-0.845000000000001,-0.840000000000001,
-0.835000000000001,-0.830000000000001,-0.825000000000001,-0.820000000000001,
-0.815000000000001,-0.810000000000001,-0.805000000000001,-0.800000000000001,
-0.795000000000001,-0.790000000000001,-0.785000000000001,-0.780000000000001,
-0.775000000000001,-0.770000000000001,-0.765000000000001,-0.760000000000001,
-0.755000000000001,-0.750000000000001,-0.745000000000001,-0.740000000000001,
-0.735000000000001,-0.730000000000001,-0.725000000000001,-0.720000000000001,
-0.715000000000001,-0.710000000000001,-0.705000000000001,-0.700000000000001,
-0.695000000000001,-0.690000000000001,-0.685,-0.68,-0.675,-0.67,-0.665,
-0.66,-0.655,-0.65,-0.645,-0.64,-0.635,-0.63,-0.625,-0.62,-0.615,-0.61,
-0.605,-0.6,-0.595,-0.59,-0.585,-0.58,-0.575,-0.57,-0.565,-0.56,-0.555,
-0.55,-0.545,-0.54,-0.535,-0.53,-0.525,-0.52,-0.515,-0.51,-0.505,-0.5,-0.495,
-0.49,-0.485,-0.48,-0.475,-0.47,-0.465,-0.46,-0.455,-0.45,-0.445,-0.44,
-0.435,-0.43,-0.425,-0.42,-0.415,-0.41,-0.405,-0.4,-0.395,-0.39,-0.385,
-0.38,-0.375,-0.37,-0.365,-0.36,-0.355,-0.35,-0.345,-0.34,-0.335,-0.33,
-0.325,-0.32,-0.315,-0.31,-0.305,-0.3,-0.295,-0.29,-0.285,-0.28,-0.275,
-0.27,-0.265,-0.26,-0.255,-0.25,-0.245,-0.24,-0.235,-0.23,-0.225,-0.22,
-0.215,-0.21,-0.205,-0.2,-0.195,-0.19,-0.185,-0.18,-0.175,-0.17,-0.165,
-0.16,-0.155,-0.15,-0.145,-0.14,-0.135,-0.13,-0.125,-0.12,-0.115,-0.11,
-0.105,-0.1,-0.095,-0.09,-0.085,-0.08,-0.075,-0.07,-0.065,-0.06,-0.055,
-0.05,-0.045,-0.04,-0.035,-0.03,-0.025,-0.02,-0.015,-0.01,-0.005,0.),
 .UNSPECIFIED.)
CURVE()
GEOMETRIC_REPRESENTATION_ITEM()
RATIONAL_B_SPLINE_CURVE((1.,1.,1.,1.,1.,1.,1.,1.,1.,1.,1.,1.,1.,1.,1.,1.,
1.,1.,1.,1.,1.,1.,1.,1.,1.,1.,1.,1.,1.,1.,1.,1.,1.,1.,1.,1.,1.,1.,1.,1.,
1.,1.,1.,1.,1.,1.,1.,1.,1.,1.,1.,1.,1.,1.,1.,1.,1.,1.,1.,1.,1.,1.,1.,1.,
1.,1.,1.,1.,1.,1.,1.,1.,1.,1.,1.,1.,1.,1.,1.,1.,1.,1.,1.,1.,1.,1.,1.,1.,
1.,1.,1.,1.,1.,1.,1.,1.,1.,1.,1.,1.,1.,1.,1.,1.,1.,1.,1.,1.,1.,1.,1.,1.,
1.,1.,1.,1.,1.,1.,1.,1.,1.,1.,1.,1.,1.,1.,1.,1.,1.,1.,1.,1.,1.,1.,1.,1.,
1.,1.,1.,1.,1.,1.,1.,1.,1.,1.,1.,1.,1.,1.,1.,1.,1.,1.,1.,1.,1.,1.,1.,1.,
1.,1.,1.,1.,1.,1.,1.,1.,1.,1.,1.,1.,1.,1.,1.,1.,1.,1.,1.,1.,1.,1.,1.,1.,
1.,1.,1.,1.,1.,1.,1.,1.,1.,1.))
REPRESENTATION_ITEM('')
);
#671=(
BOUNDED_CURVE()
B_SPLINE_CURVE(5,(#167066,#167067,#167068,#167069,#167070,#167071,#167072,
#167073,#167074,#167075,#167076,#167077,#167078,#167079,#167080,#167081,
#167082,#167083,#167084,#167085,#167086,#167087,#167088,#167089,#167090,
#167091,#167092,#167093,#167094,#167095,#167096,#167097,#167098,#167099,
#167100,#167101,#167102,#167103,#167104,#167105,#167106,#167107,#167108,
#167109,#167110,#167111,#167112,#167113,#167114,#167115,#167116,#167117,
#167118,#167119,#167120,#167121,#167122,#167123,#167124,#167125,#167126,
#167127,#167128,#167129,#167130,#167131,#167132,#167133,#167134,#167135,
#167136,#167137,#167138,#167139,#167140,#167141,#167142,#167143,#167144,
#167145,#167146,#167147,#167148,#167149,#167150,#167151,#167152,#167153,
#167154,#167155,#167156,#167157,#167158,#167159,#167160,#167161,#167162,
#167163,#167164,#167165,#167166,#167167,#167168,#167169,#167170,#167171,
#167172,#167173,#167174,#167175,#167176,#167177,#167178,#167179,#167180,
#167181,#167182,#167183,#167184,#167185,#167186,#167187,#167188,#167189,
#167190,#167191,#167192,#167193,#167194,#167195,#167196,#167197,#167198,
#167199,#167200,#167201,#167202,#167203,#167204,#167205,#167206,#167207,
#167208,#167209,#167210,#167211,#167212,#167213,#167214,#167215,#167216,
#167217,#167218,#167219,#167220,#167221,#167222,#167223,#167224,#167225,
#167226,#167227,#167228,#167229,#167230,#167231,#167232,#167233,#167234,
#167235,#167236,#167237,#167238,#167239,#167240,#167241,#167242,#167243,
#167244,#167245,#167246,#167247,#167248,#167249,#167250,#167251,#167252,
#167253,#167254,#167255,#167256,#167257,#167258,#167259),.UNSPECIFIED.,
 .F.,.F.)
B_SPLINE_CURVE_WITH_KNOTS((6,1,1,1,1,1,1,1,1,1,1,1,1,1,1,1,1,1,1,1,1,1,
1,1,1,1,1,1,1,1,1,1,1,1,1,1,1,1,1,1,1,1,1,1,1,1,1,1,1,1,1,1,1,1,1,1,1,1,
1,1,1,1,1,1,1,1,1,1,1,1,1,1,1,1,1,1,1,1,1,1,1,1,1,1,1,1,1,1,1,1,1,1,1,1,
1,1,1,1,1,1,1,1,1,1,1,1,1,1,1,1,1,1,1,1,1,1,1,1,1,1,1,1,1,1,1,1,1,1,1,1,
1,1,1,1,1,1,1,1,1,1,1,1,1,1,1,1,1,1,1,1,1,1,1,1,1,1,1,1,1,1,1,1,1,1,1,1,
1,1,1,1,1,1,1,1,1,1,1,1,1,1,1,1,1,1,1,1,1,1,1,6),(0.,0.005,0.01,0.015,0.02,
0.025,0.03,0.035,0.04,0.045,0.05,0.055,0.06,0.065,0.07,0.075,0.08,0.085,
0.09,0.095,0.1,0.105,0.11,0.115,0.12,0.125,0.13,0.135,0.14,0.145,0.15,0.155,
0.16,0.165,0.17,0.175,0.18,0.185,0.19,0.195,0.2,0.205,0.21,0.215,0.22,0.225,
0.23,0.235,0.24,0.245,0.25,0.255,0.26,0.265,0.27,0.275,0.28,0.285,0.29,
0.295,0.3,0.305,0.31,0.315,0.32,0.325,0.33,0.335,0.34,0.345,0.35,0.355,
0.36,0.365,0.37,0.375,0.38,0.385,0.39,0.395,0.4,0.405,0.41,0.415,0.42,0.425,
0.43,0.435,0.44,0.445,0.45,0.455,0.46,0.465,0.47,0.475,0.48,0.485,0.49,
0.495,0.5,0.505,0.51,0.515,0.52,0.525,0.53,0.535,0.54,0.545,0.55,0.555,
0.56,0.565,0.57,0.575,0.58,0.585,0.59,0.595,0.6,0.605,0.61,0.615,0.62,0.625,
0.63,0.635,0.64,0.645,0.65,0.655,0.66,0.665,0.67,0.675,0.68,0.685,0.690000000000001,
0.695000000000001,0.700000000000001,0.705000000000001,0.710000000000001,
0.715000000000001,0.720000000000001,0.725000000000001,0.730000000000001,
0.735000000000001,0.740000000000001,0.745000000000001,0.750000000000001,
0.755000000000001,0.760000000000001,0.765000000000001,0.770000000000001,
0.775000000000001,0.780000000000001,0.785000000000001,0.790000000000001,
0.795000000000001,0.800000000000001,0.805000000000001,0.810000000000001,
0.815000000000001,0.820000000000001,0.825000000000001,0.830000000000001,
0.835000000000001,0.840000000000001,0.845000000000001,0.850000000000001,
0.855000000000001,0.860000000000001,0.865000000000001,0.870000000000001,
0.875000000000001,0.880000000000001,0.885000000000001,0.890000000000001,
0.895000000000001,0.900000000000001,0.905000000000001,0.910000000000001,
0.915000000000001,0.920000000000001,0.925000000000001,0.930000000000001,
0.935000000000001,0.940000000000001,0.941429844438107),.UNSPECIFIED.)
CURVE()
GEOMETRIC_REPRESENTATION_ITEM()
RATIONAL_B_SPLINE_CURVE((1.,1.,1.,1.,1.,1.,1.,1.,1.,1.,1.,1.,1.,1.,1.,1.,
1.,1.,1.,1.,1.,1.,1.,1.,1.,1.,1.,1.,1.,1.,1.,1.,1.,1.,1.,1.,1.,1.,1.,1.,
1.,1.,1.,1.,1.,1.,1.,1.,1.,1.,1.,1.,1.,1.,1.,1.,1.,1.,1.,1.,1.,1.,1.,1.,
1.,1.,1.,1.,1.,1.,1.,1.,1.,1.,1.,1.,1.,1.,1.,1.,1.,1.,1.,1.,1.,1.,1.,1.,
1.,1.,1.,1.,1.,1.,1.,1.,1.,1.,1.,1.,1.,1.,1.,1.,1.,1.,1.,1.,1.,1.,1.,1.,
1.,1.,1.,1.,1.,1.,1.,1.,1.,1.,1.,1.,1.,1.,1.,1.,1.,1.,1.,1.,1.,1.,1.,1.,
1.,1.,1.,1.,1.,1.,1.,1.,1.,1.,1.,1.,1.,1.,1.,1.,1.,1.,1.,1.,1.,1.,1.,1.,
1.,1.,1.,1.,1.,1.,1.,1.,1.,1.,1.,1.,1.,1.,1.,1.,1.,1.,1.,1.,1.,1.,1.,1.,
1.,1.,1.,1.,1.,1.,1.,1.,1.,1.))
REPRESENTATION_ITEM('')
);
#672=(
BOUNDED_CURVE()
B_SPLINE_CURVE(5,(#167262,#167263,#167264,#167265,#167266,#167267,#167268,
#167269,#167270,#167271,#167272,#167273,#167274,#167275,#167276,#167277,
#167278,#167279,#167280,#167281,#167282,#167283,#167284,#167285,#167286,
#167287,#167288,#167289,#167290,#167291,#167292,#167293,#167294,#167295,
#167296,#167297,#167298,#167299,#167300,#167301,#167302,#167303,#167304,
#167305,#167306,#167307,#167308,#167309,#167310,#167311,#167312,#167313,
#167314,#167315,#167316,#167317,#167318,#167319,#167320,#167321,#167322,
#167323,#167324,#167325,#167326,#167327,#167328,#167329,#167330,#167331,
#167332,#167333,#167334,#167335,#167336,#167337,#167338,#167339,#167340,
#167341,#167342,#167343,#167344,#167345,#167346,#167347,#167348,#167349,
#167350,#167351,#167352,#167353,#167354,#167355,#167356,#167357,#167358,
#167359,#167360,#167361,#167362,#167363,#167364,#167365,#167366,#167367,
#167368,#167369,#167370,#167371,#167372,#167373,#167374,#167375,#167376,
#167377,#167378,#167379,#167380,#167381,#167382,#167383,#167384,#167385,
#167386,#167387,#167388,#167389,#167390,#167391,#167392,#167393,#167394,
#167395,#167396,#167397,#167398,#167399,#167400,#167401,#167402,#167403,
#167404,#167405,#167406,#167407,#167408,#167409,#167410,#167411,#167412,
#167413,#167414,#167415,#167416,#167417,#167418,#167419,#167420,#167421,
#167422,#167423,#167424,#167425,#167426,#167427,#167428,#167429,#167430,
#167431,#167432,#167433,#167434,#167435,#167436,#167437,#167438,#167439,
#167440,#167441,#167442,#167443,#167444,#167445,#167446,#167447,#167448,
#167449,#167450,#167451,#167452,#167453,#167454,#167455),.UNSPECIFIED.,
 .F.,.F.)
B_SPLINE_CURVE_WITH_KNOTS((6,1,1,1,1,1,1,1,1,1,1,1,1,1,1,1,1,1,1,1,1,1,
1,1,1,1,1,1,1,1,1,1,1,1,1,1,1,1,1,1,1,1,1,1,1,1,1,1,1,1,1,1,1,1,1,1,1,1,
1,1,1,1,1,1,1,1,1,1,1,1,1,1,1,1,1,1,1,1,1,1,1,1,1,1,1,1,1,1,1,1,1,1,1,1,
1,1,1,1,1,1,1,1,1,1,1,1,1,1,1,1,1,1,1,1,1,1,1,1,1,1,1,1,1,1,1,1,1,1,1,1,
1,1,1,1,1,1,1,1,1,1,1,1,1,1,1,1,1,1,1,1,1,1,1,1,1,1,1,1,1,1,1,1,1,1,1,1,
1,1,1,1,1,1,1,1,1,1,1,1,1,1,1,1,1,1,1,1,1,1,1,6),(-0.941429844438107,-0.940000000000001,
-0.935000000000001,-0.930000000000001,-0.925000000000001,-0.920000000000001,
-0.915000000000001,-0.910000000000001,-0.905000000000001,-0.900000000000001,
-0.895000000000001,-0.890000000000001,-0.885000000000001,-0.880000000000001,
-0.875000000000001,-0.870000000000001,-0.865000000000001,-0.860000000000001,
-0.855000000000001,-0.850000000000001,-0.845000000000001,-0.840000000000001,
-0.835000000000001,-0.830000000000001,-0.825000000000001,-0.820000000000001,
-0.815000000000001,-0.810000000000001,-0.805000000000001,-0.800000000000001,
-0.795000000000001,-0.790000000000001,-0.785000000000001,-0.780000000000001,
-0.775000000000001,-0.770000000000001,-0.765000000000001,-0.760000000000001,
-0.755000000000001,-0.750000000000001,-0.745000000000001,-0.740000000000001,
-0.735000000000001,-0.730000000000001,-0.725000000000001,-0.720000000000001,
-0.715000000000001,-0.710000000000001,-0.705000000000001,-0.700000000000001,
-0.695000000000001,-0.690000000000001,-0.685,-0.68,-0.675,-0.67,-0.665,
-0.66,-0.655,-0.65,-0.645,-0.64,-0.635,-0.63,-0.625,-0.62,-0.615,-0.61,
-0.605,-0.6,-0.595,-0.59,-0.585,-0.58,-0.575,-0.57,-0.565,-0.56,-0.555,
-0.55,-0.545,-0.54,-0.535,-0.53,-0.525,-0.52,-0.515,-0.51,-0.505,-0.5,-0.495,
-0.49,-0.485,-0.48,-0.475,-0.47,-0.465,-0.46,-0.455,-0.45,-0.445,-0.44,
-0.435,-0.43,-0.425,-0.42,-0.415,-0.41,-0.405,-0.4,-0.395,-0.39,-0.385,
-0.38,-0.375,-0.37,-0.365,-0.36,-0.355,-0.35,-0.345,-0.34,-0.335,-0.33,
-0.325,-0.32,-0.315,-0.31,-0.305,-0.3,-0.295,-0.29,-0.285,-0.28,-0.275,
-0.27,-0.265,-0.26,-0.255,-0.25,-0.245,-0.24,-0.235,-0.23,-0.225,-0.22,
-0.215,-0.21,-0.205,-0.2,-0.195,-0.19,-0.185,-0.18,-0.175,-0.17,-0.165,
-0.16,-0.155,-0.15,-0.145,-0.14,-0.135,-0.13,-0.125,-0.12,-0.115,-0.11,
-0.105,-0.1,-0.095,-0.09,-0.085,-0.08,-0.075,-0.07,-0.065,-0.06,-0.055,
-0.05,-0.045,-0.04,-0.035,-0.03,-0.025,-0.02,-0.015,-0.01,-0.005,0.),
 .UNSPECIFIED.)
CURVE()
GEOMETRIC_REPRESENTATION_ITEM()
RATIONAL_B_SPLINE_CURVE((1.,1.,1.,1.,1.,1.,1.,1.,1.,1.,1.,1.,1.,1.,1.,1.,
1.,1.,1.,1.,1.,1.,1.,1.,1.,1.,1.,1.,1.,1.,1.,1.,1.,1.,1.,1.,1.,1.,1.,1.,
1.,1.,1.,1.,1.,1.,1.,1.,1.,1.,1.,1.,1.,1.,1.,1.,1.,1.,1.,1.,1.,1.,1.,1.,
1.,1.,1.,1.,1.,1.,1.,1.,1.,1.,1.,1.,1.,1.,1.,1.,1.,1.,1.,1.,1.,1.,1.,1.,
1.,1.,1.,1.,1.,1.,1.,1.,1.,1.,1.,1.,1.,1.,1.,1.,1.,1.,1.,1.,1.,1.,1.,1.,
1.,1.,1.,1.,1.,1.,1.,1.,1.,1.,1.,1.,1.,1.,1.,1.,1.,1.,1.,1.,1.,1.,1.,1.,
1.,1.,1.,1.,1.,1.,1.,1.,1.,1.,1.,1.,1.,1.,1.,1.,1.,1.,1.,1.,1.,1.,1.,1.,
1.,1.,1.,1.,1.,1.,1.,1.,1.,1.,1.,1.,1.,1.,1.,1.,1.,1.,1.,1.,1.,1.,1.,1.,
1.,1.,1.,1.,1.,1.,1.,1.,1.,1.))
REPRESENTATION_ITEM('')
);
#673=(
BOUNDED_CURVE()
B_SPLINE_CURVE(5,(#167867,#167868,#167869,#167870,#167871,#167872,#167873,
#167874,#167875,#167876,#167877,#167878,#167879,#167880,#167881,#167882,
#167883,#167884,#167885,#167886,#167887,#167888,#167889,#167890,#167891,
#167892,#167893,#167894,#167895,#167896,#167897,#167898,#167899,#167900,
#167901,#167902,#167903,#167904,#167905,#167906,#167907,#167908,#167909,
#167910,#167911,#167912,#167913,#167914,#167915,#167916,#167917,#167918,
#167919,#167920,#167921,#167922,#167923,#167924,#167925,#167926,#167927,
#167928,#167929,#167930,#167931,#167932,#167933,#167934,#167935,#167936,
#167937,#167938,#167939,#167940,#167941,#167942,#167943,#167944,#167945,
#167946,#167947,#167948,#167949,#167950,#167951,#167952,#167953,#167954,
#167955,#167956,#167957,#167958,#167959,#167960,#167961,#167962,#167963,
#167964,#167965,#167966,#167967,#167968,#167969,#167970,#167971,#167972,
#167973,#167974,#167975,#167976,#167977,#167978,#167979,#167980,#167981,
#167982,#167983,#167984,#167985,#167986,#167987,#167988,#167989,#167990,
#167991,#167992,#167993,#167994,#167995,#167996,#167997,#167998,#167999,
#168000,#168001,#168002,#168003,#168004,#168005,#168006,#168007,#168008,
#168009,#168010,#168011,#168012,#168013,#168014,#168015,#168016,#168017,
#168018,#168019,#168020,#168021,#168022,#168023,#168024,#168025,#168026,
#168027,#168028,#168029,#168030,#168031,#168032,#168033,#168034,#168035,
#168036,#168037,#168038,#168039,#168040,#168041,#168042,#168043,#168044,
#168045,#168046,#168047,#168048,#168049,#168050,#168051,#168052,#168053,
#168054,#168055,#168056,#168057,#168058,#168059,#168060),.UNSPECIFIED.,
 .F.,.F.)
B_SPLINE_CURVE_WITH_KNOTS((6,1,1,1,1,1,1,1,1,1,1,1,1,1,1,1,1,1,1,1,1,1,
1,1,1,1,1,1,1,1,1,1,1,1,1,1,1,1,1,1,1,1,1,1,1,1,1,1,1,1,1,1,1,1,1,1,1,1,
1,1,1,1,1,1,1,1,1,1,1,1,1,1,1,1,1,1,1,1,1,1,1,1,1,1,1,1,1,1,1,1,1,1,1,1,
1,1,1,1,1,1,1,1,1,1,1,1,1,1,1,1,1,1,1,1,1,1,1,1,1,1,1,1,1,1,1,1,1,1,1,1,
1,1,1,1,1,1,1,1,1,1,1,1,1,1,1,1,1,1,1,1,1,1,1,1,1,1,1,1,1,1,1,1,1,1,1,1,
1,1,1,1,1,1,1,1,1,1,1,1,1,1,1,1,1,1,1,1,1,1,1,6),(0.,0.005,0.01,0.015,0.02,
0.025,0.03,0.035,0.04,0.045,0.05,0.055,0.06,0.065,0.07,0.075,0.08,0.085,
0.09,0.095,0.1,0.105,0.11,0.115,0.12,0.125,0.13,0.135,0.14,0.145,0.15,0.155,
0.16,0.165,0.17,0.175,0.18,0.185,0.19,0.195,0.2,0.205,0.21,0.215,0.22,0.225,
0.23,0.235,0.24,0.245,0.25,0.255,0.26,0.265,0.27,0.275,0.28,0.285,0.29,
0.295,0.3,0.305,0.31,0.315,0.32,0.325,0.33,0.335,0.34,0.345,0.35,0.355,
0.36,0.365,0.37,0.375,0.38,0.385,0.39,0.395,0.4,0.405,0.41,0.415,0.42,0.425,
0.43,0.435,0.44,0.445,0.45,0.455,0.46,0.465,0.47,0.475,0.48,0.485,0.49,
0.495,0.5,0.505,0.51,0.515,0.52,0.525,0.53,0.535,0.54,0.545,0.55,0.555,
0.56,0.565,0.57,0.575,0.58,0.585,0.59,0.595,0.6,0.605,0.61,0.615,0.62,0.625,
0.63,0.635,0.64,0.645,0.65,0.655,0.66,0.665,0.67,0.675,0.68,0.685,0.690000000000001,
0.695000000000001,0.700000000000001,0.705000000000001,0.710000000000001,
0.715000000000001,0.720000000000001,0.725000000000001,0.730000000000001,
0.735000000000001,0.740000000000001,0.745000000000001,0.750000000000001,
0.755000000000001,0.760000000000001,0.765000000000001,0.770000000000001,
0.775000000000001,0.780000000000001,0.785000000000001,0.790000000000001,
0.795000000000001,0.800000000000001,0.805000000000001,0.810000000000001,
0.815000000000001,0.820000000000001,0.825000000000001,0.830000000000001,
0.835000000000001,0.840000000000001,0.845000000000001,0.850000000000001,
0.855000000000001,0.860000000000001,0.865000000000001,0.870000000000001,
0.875000000000001,0.880000000000001,0.885000000000001,0.890000000000001,
0.895000000000001,0.900000000000001,0.905000000000001,0.910000000000001,
0.915000000000001,0.920000000000001,0.925000000000001,0.930000000000001,
0.935000000000001,0.940000000000001,0.941429844438079),.UNSPECIFIED.)
CURVE()
GEOMETRIC_REPRESENTATION_ITEM()
RATIONAL_B_SPLINE_CURVE((1.,1.,1.,1.,1.,1.,1.,1.,1.,1.,1.,1.,1.,1.,1.,1.,
1.,1.,1.,1.,1.,1.,1.,1.,1.,1.,1.,1.,1.,1.,1.,1.,1.,1.,1.,1.,1.,1.,1.,1.,
1.,1.,1.,1.,1.,1.,1.,1.,1.,1.,1.,1.,1.,1.,1.,1.,1.,1.,1.,1.,1.,1.,1.,1.,
1.,1.,1.,1.,1.,1.,1.,1.,1.,1.,1.,1.,1.,1.,1.,1.,1.,1.,1.,1.,1.,1.,1.,1.,
1.,1.,1.,1.,1.,1.,1.,1.,1.,1.,1.,1.,1.,1.,1.,1.,1.,1.,1.,1.,1.,1.,1.,1.,
1.,1.,1.,1.,1.,1.,1.,1.,1.,1.,1.,1.,1.,1.,1.,1.,1.,1.,1.,1.,1.,1.,1.,1.,
1.,1.,1.,1.,1.,1.,1.,1.,1.,1.,1.,1.,1.,1.,1.,1.,1.,1.,1.,1.,1.,1.,1.,1.,
1.,1.,1.,1.,1.,1.,1.,1.,1.,1.,1.,1.,1.,1.,1.,1.,1.,1.,1.,1.,1.,1.,1.,1.,
1.,1.,1.,1.,1.,1.,1.,1.,1.,1.))
REPRESENTATION_ITEM('')
);
#674=(
BOUNDED_CURVE()
B_SPLINE_CURVE(5,(#168063,#168064,#168065,#168066,#168067,#168068,#168069,
#168070,#168071,#168072,#168073,#168074,#168075,#168076,#168077,#168078,
#168079,#168080,#168081,#168082,#168083,#168084,#168085,#168086,#168087,
#168088,#168089,#168090,#168091,#168092,#168093,#168094,#168095,#168096,
#168097,#168098,#168099,#168100,#168101,#168102,#168103,#168104,#168105,
#168106,#168107,#168108,#168109,#168110,#168111,#168112,#168113,#168114,
#168115,#168116,#168117,#168118,#168119,#168120,#168121,#168122,#168123,
#168124,#168125,#168126,#168127,#168128,#168129,#168130,#168131,#168132,
#168133,#168134,#168135,#168136,#168137,#168138,#168139,#168140,#168141,
#168142,#168143,#168144,#168145,#168146,#168147,#168148,#168149,#168150,
#168151,#168152,#168153,#168154,#168155,#168156,#168157,#168158,#168159,
#168160,#168161,#168162,#168163,#168164,#168165,#168166,#168167,#168168,
#168169,#168170,#168171,#168172,#168173,#168174,#168175,#168176,#168177,
#168178,#168179,#168180,#168181,#168182,#168183,#168184,#168185,#168186,
#168187,#168188,#168189,#168190,#168191,#168192,#168193,#168194,#168195,
#168196,#168197,#168198,#168199,#168200,#168201,#168202,#168203,#168204,
#168205,#168206,#168207,#168208,#168209,#168210,#168211,#168212,#168213,
#168214,#168215,#168216,#168217,#168218,#168219,#168220,#168221,#168222,
#168223,#168224,#168225,#168226,#168227,#168228,#168229,#168230,#168231,
#168232,#168233,#168234,#168235,#168236,#168237,#168238,#168239,#168240,
#168241,#168242,#168243,#168244,#168245,#168246,#168247,#168248,#168249,
#168250,#168251,#168252,#168253,#168254,#168255,#168256),.UNSPECIFIED.,
 .F.,.F.)
B_SPLINE_CURVE_WITH_KNOTS((6,1,1,1,1,1,1,1,1,1,1,1,1,1,1,1,1,1,1,1,1,1,
1,1,1,1,1,1,1,1,1,1,1,1,1,1,1,1,1,1,1,1,1,1,1,1,1,1,1,1,1,1,1,1,1,1,1,1,
1,1,1,1,1,1,1,1,1,1,1,1,1,1,1,1,1,1,1,1,1,1,1,1,1,1,1,1,1,1,1,1,1,1,1,1,
1,1,1,1,1,1,1,1,1,1,1,1,1,1,1,1,1,1,1,1,1,1,1,1,1,1,1,1,1,1,1,1,1,1,1,1,
1,1,1,1,1,1,1,1,1,1,1,1,1,1,1,1,1,1,1,1,1,1,1,1,1,1,1,1,1,1,1,1,1,1,1,1,
1,1,1,1,1,1,1,1,1,1,1,1,1,1,1,1,1,1,1,1,1,1,1,6),(-0.941429844438079,-0.940000000000001,
-0.935000000000001,-0.930000000000001,-0.925000000000001,-0.920000000000001,
-0.915000000000001,-0.910000000000001,-0.905000000000001,-0.900000000000001,
-0.895000000000001,-0.890000000000001,-0.885000000000001,-0.880000000000001,
-0.875000000000001,-0.870000000000001,-0.865000000000001,-0.860000000000001,
-0.855000000000001,-0.850000000000001,-0.845000000000001,-0.840000000000001,
-0.835000000000001,-0.830000000000001,-0.825000000000001,-0.820000000000001,
-0.815000000000001,-0.810000000000001,-0.805000000000001,-0.800000000000001,
-0.795000000000001,-0.790000000000001,-0.785000000000001,-0.780000000000001,
-0.775000000000001,-0.770000000000001,-0.765000000000001,-0.760000000000001,
-0.755000000000001,-0.750000000000001,-0.745000000000001,-0.740000000000001,
-0.735000000000001,-0.730000000000001,-0.725000000000001,-0.720000000000001,
-0.715000000000001,-0.710000000000001,-0.705000000000001,-0.700000000000001,
-0.695000000000001,-0.690000000000001,-0.685,-0.68,-0.675,-0.67,-0.665,
-0.66,-0.655,-0.65,-0.645,-0.64,-0.635,-0.63,-0.625,-0.62,-0.615,-0.61,
-0.605,-0.6,-0.595,-0.59,-0.585,-0.58,-0.575,-0.57,-0.565,-0.56,-0.555,
-0.55,-0.545,-0.54,-0.535,-0.53,-0.525,-0.52,-0.515,-0.51,-0.505,-0.5,-0.495,
-0.49,-0.485,-0.48,-0.475,-0.47,-0.465,-0.46,-0.455,-0.45,-0.445,-0.44,
-0.435,-0.43,-0.425,-0.42,-0.415,-0.41,-0.405,-0.4,-0.395,-0.39,-0.385,
-0.38,-0.375,-0.37,-0.365,-0.36,-0.355,-0.35,-0.345,-0.34,-0.335,-0.33,
-0.325,-0.32,-0.315,-0.31,-0.305,-0.3,-0.295,-0.29,-0.285,-0.28,-0.275,
-0.27,-0.265,-0.26,-0.255,-0.25,-0.245,-0.24,-0.235,-0.23,-0.225,-0.22,
-0.215,-0.21,-0.205,-0.2,-0.195,-0.19,-0.185,-0.18,-0.175,-0.17,-0.165,
-0.16,-0.155,-0.15,-0.145,-0.14,-0.135,-0.13,-0.125,-0.12,-0.115,-0.11,
-0.105,-0.1,-0.095,-0.09,-0.085,-0.08,-0.075,-0.07,-0.065,-0.06,-0.055,
-0.05,-0.045,-0.04,-0.035,-0.03,-0.025,-0.02,-0.015,-0.01,-0.005,0.),
 .UNSPECIFIED.)
CURVE()
GEOMETRIC_REPRESENTATION_ITEM()
RATIONAL_B_SPLINE_CURVE((1.,1.,1.,1.,1.,1.,1.,1.,1.,1.,1.,1.,1.,1.,1.,1.,
1.,1.,1.,1.,1.,1.,1.,1.,1.,1.,1.,1.,1.,1.,1.,1.,1.,1.,1.,1.,1.,1.,1.,1.,
1.,1.,1.,1.,1.,1.,1.,1.,1.,1.,1.,1.,1.,1.,1.,1.,1.,1.,1.,1.,1.,1.,1.,1.,
1.,1.,1.,1.,1.,1.,1.,1.,1.,1.,1.,1.,1.,1.,1.,1.,1.,1.,1.,1.,1.,1.,1.,1.,
1.,1.,1.,1.,1.,1.,1.,1.,1.,1.,1.,1.,1.,1.,1.,1.,1.,1.,1.,1.,1.,1.,1.,1.,
1.,1.,1.,1.,1.,1.,1.,1.,1.,1.,1.,1.,1.,1.,1.,1.,1.,1.,1.,1.,1.,1.,1.,1.,
1.,1.,1.,1.,1.,1.,1.,1.,1.,1.,1.,1.,1.,1.,1.,1.,1.,1.,1.,1.,1.,1.,1.,1.,
1.,1.,1.,1.,1.,1.,1.,1.,1.,1.,1.,1.,1.,1.,1.,1.,1.,1.,1.,1.,1.,1.,1.,1.,
1.,1.,1.,1.,1.,1.,1.,1.,1.,1.))
REPRESENTATION_ITEM('')
);
#675=(
BOUNDED_CURVE()
B_SPLINE_CURVE(5,(#168668,#168669,#168670,#168671,#168672,#168673,#168674,
#168675,#168676,#168677,#168678,#168679,#168680,#168681,#168682,#168683,
#168684,#168685,#168686,#168687,#168688,#168689,#168690,#168691,#168692,
#168693,#168694,#168695,#168696,#168697,#168698,#168699,#168700,#168701,
#168702,#168703,#168704,#168705,#168706,#168707,#168708,#168709,#168710,
#168711,#168712,#168713,#168714,#168715,#168716,#168717,#168718,#168719,
#168720,#168721,#168722,#168723,#168724,#168725,#168726,#168727,#168728,
#168729,#168730,#168731,#168732,#168733,#168734,#168735,#168736,#168737,
#168738,#168739,#168740,#168741,#168742,#168743,#168744,#168745,#168746,
#168747,#168748,#168749,#168750,#168751,#168752,#168753,#168754,#168755,
#168756,#168757,#168758,#168759,#168760,#168761,#168762,#168763,#168764,
#168765,#168766,#168767,#168768,#168769,#168770,#168771,#168772,#168773,
#168774,#168775,#168776,#168777,#168778,#168779,#168780,#168781,#168782,
#168783,#168784,#168785,#168786,#168787,#168788,#168789,#168790,#168791,
#168792,#168793,#168794,#168795,#168796,#168797,#168798,#168799,#168800,
#168801,#168802,#168803,#168804,#168805,#168806,#168807,#168808,#168809,
#168810,#168811,#168812,#168813,#168814,#168815,#168816,#168817,#168818,
#168819,#168820,#168821,#168822,#168823,#168824,#168825,#168826,#168827,
#168828,#168829,#168830,#168831,#168832,#168833,#168834,#168835,#168836,
#168837,#168838,#168839,#168840,#168841,#168842,#168843,#168844,#168845,
#168846,#168847,#168848,#168849,#168850,#168851,#168852,#168853,#168854,
#168855,#168856,#168857,#168858,#168859,#168860,#168861),.UNSPECIFIED.,
 .F.,.F.)
B_SPLINE_CURVE_WITH_KNOTS((6,1,1,1,1,1,1,1,1,1,1,1,1,1,1,1,1,1,1,1,1,1,
1,1,1,1,1,1,1,1,1,1,1,1,1,1,1,1,1,1,1,1,1,1,1,1,1,1,1,1,1,1,1,1,1,1,1,1,
1,1,1,1,1,1,1,1,1,1,1,1,1,1,1,1,1,1,1,1,1,1,1,1,1,1,1,1,1,1,1,1,1,1,1,1,
1,1,1,1,1,1,1,1,1,1,1,1,1,1,1,1,1,1,1,1,1,1,1,1,1,1,1,1,1,1,1,1,1,1,1,1,
1,1,1,1,1,1,1,1,1,1,1,1,1,1,1,1,1,1,1,1,1,1,1,1,1,1,1,1,1,1,1,1,1,1,1,1,
1,1,1,1,1,1,1,1,1,1,1,1,1,1,1,1,1,1,1,1,1,1,1,6),(0.,0.005,0.01,0.015,0.02,
0.025,0.03,0.035,0.04,0.045,0.05,0.055,0.06,0.065,0.07,0.075,0.08,0.085,
0.09,0.095,0.1,0.105,0.11,0.115,0.12,0.125,0.13,0.135,0.14,0.145,0.15,0.155,
0.16,0.165,0.17,0.175,0.18,0.185,0.19,0.195,0.2,0.205,0.21,0.215,0.22,0.225,
0.23,0.235,0.24,0.245,0.25,0.255,0.26,0.265,0.27,0.275,0.28,0.285,0.29,
0.295,0.3,0.305,0.31,0.315,0.32,0.325,0.33,0.335,0.34,0.345,0.35,0.355,
0.36,0.365,0.37,0.375,0.38,0.385,0.39,0.395,0.4,0.405,0.41,0.415,0.42,0.425,
0.43,0.435,0.44,0.445,0.45,0.455,0.46,0.465,0.47,0.475,0.48,0.485,0.49,
0.495,0.5,0.505,0.51,0.515,0.52,0.525,0.53,0.535,0.54,0.545,0.55,0.555,
0.56,0.565,0.57,0.575,0.58,0.585,0.59,0.595,0.6,0.605,0.61,0.615,0.62,0.625,
0.63,0.635,0.64,0.645,0.65,0.655,0.66,0.665,0.67,0.675,0.68,0.685,0.690000000000001,
0.695000000000001,0.700000000000001,0.705000000000001,0.710000000000001,
0.715000000000001,0.720000000000001,0.725000000000001,0.730000000000001,
0.735000000000001,0.740000000000001,0.745000000000001,0.750000000000001,
0.755000000000001,0.760000000000001,0.765000000000001,0.770000000000001,
0.775000000000001,0.780000000000001,0.785000000000001,0.790000000000001,
0.795000000000001,0.800000000000001,0.805000000000001,0.810000000000001,
0.815000000000001,0.820000000000001,0.825000000000001,0.830000000000001,
0.835000000000001,0.840000000000001,0.845000000000001,0.850000000000001,
0.855000000000001,0.860000000000001,0.865000000000001,0.870000000000001,
0.875000000000001,0.880000000000001,0.885000000000001,0.890000000000001,
0.895000000000001,0.900000000000001,0.905000000000001,0.910000000000001,
0.915000000000001,0.920000000000001,0.925000000000001,0.930000000000001,
0.935000000000001,0.940000000000001,0.941429844438012),.UNSPECIFIED.)
CURVE()
GEOMETRIC_REPRESENTATION_ITEM()
RATIONAL_B_SPLINE_CURVE((1.,1.,1.,1.,1.,1.,1.,1.,1.,1.,1.,1.,1.,1.,1.,1.,
1.,1.,1.,1.,1.,1.,1.,1.,1.,1.,1.,1.,1.,1.,1.,1.,1.,1.,1.,1.,1.,1.,1.,1.,
1.,1.,1.,1.,1.,1.,1.,1.,1.,1.,1.,1.,1.,1.,1.,1.,1.,1.,1.,1.,1.,1.,1.,1.,
1.,1.,1.,1.,1.,1.,1.,1.,1.,1.,1.,1.,1.,1.,1.,1.,1.,1.,1.,1.,1.,1.,1.,1.,
1.,1.,1.,1.,1.,1.,1.,1.,1.,1.,1.,1.,1.,1.,1.,1.,1.,1.,1.,1.,1.,1.,1.,1.,
1.,1.,1.,1.,1.,1.,1.,1.,1.,1.,1.,1.,1.,1.,1.,1.,1.,1.,1.,1.,1.,1.,1.,1.,
1.,1.,1.,1.,1.,1.,1.,1.,1.,1.,1.,1.,1.,1.,1.,1.,1.,1.,1.,1.,1.,1.,1.,1.,
1.,1.,1.,1.,1.,1.,1.,1.,1.,1.,1.,1.,1.,1.,1.,1.,1.,1.,1.,1.,1.,1.,1.,1.,
1.,1.,1.,1.,1.,1.,1.,1.,1.,1.))
REPRESENTATION_ITEM('')
);
#676=(
BOUNDED_CURVE()
B_SPLINE_CURVE(5,(#168864,#168865,#168866,#168867,#168868,#168869,#168870,
#168871,#168872,#168873,#168874,#168875,#168876,#168877,#168878,#168879,
#168880,#168881,#168882,#168883,#168884,#168885,#168886,#168887,#168888,
#168889,#168890,#168891,#168892,#168893,#168894,#168895,#168896,#168897,
#168898,#168899,#168900,#168901,#168902,#168903,#168904,#168905,#168906,
#168907,#168908,#168909,#168910,#168911,#168912,#168913,#168914,#168915,
#168916,#168917,#168918,#168919,#168920,#168921,#168922,#168923,#168924,
#168925,#168926,#168927,#168928,#168929,#168930,#168931,#168932,#168933,
#168934,#168935,#168936,#168937,#168938,#168939,#168940,#168941,#168942,
#168943,#168944,#168945,#168946,#168947,#168948,#168949,#168950,#168951,
#168952,#168953,#168954,#168955,#168956,#168957,#168958,#168959,#168960,
#168961,#168962,#168963,#168964,#168965,#168966,#168967,#168968,#168969,
#168970,#168971,#168972,#168973,#168974,#168975,#168976,#168977,#168978,
#168979,#168980,#168981,#168982,#168983,#168984,#168985,#168986,#168987,
#168988,#168989,#168990,#168991,#168992,#168993,#168994,#168995,#168996,
#168997,#168998,#168999,#169000,#169001,#169002,#169003,#169004,#169005,
#169006,#169007,#169008,#169009,#169010,#169011,#169012,#169013,#169014,
#169015,#169016,#169017,#169018,#169019,#169020,#169021,#169022,#169023,
#169024,#169025,#169026,#169027,#169028,#169029,#169030,#169031,#169032,
#169033,#169034,#169035,#169036,#169037,#169038,#169039,#169040,#169041,
#169042,#169043,#169044,#169045,#169046,#169047,#169048,#169049,#169050,
#169051,#169052,#169053,#169054,#169055,#169056,#169057),.UNSPECIFIED.,
 .F.,.F.)
B_SPLINE_CURVE_WITH_KNOTS((6,1,1,1,1,1,1,1,1,1,1,1,1,1,1,1,1,1,1,1,1,1,
1,1,1,1,1,1,1,1,1,1,1,1,1,1,1,1,1,1,1,1,1,1,1,1,1,1,1,1,1,1,1,1,1,1,1,1,
1,1,1,1,1,1,1,1,1,1,1,1,1,1,1,1,1,1,1,1,1,1,1,1,1,1,1,1,1,1,1,1,1,1,1,1,
1,1,1,1,1,1,1,1,1,1,1,1,1,1,1,1,1,1,1,1,1,1,1,1,1,1,1,1,1,1,1,1,1,1,1,1,
1,1,1,1,1,1,1,1,1,1,1,1,1,1,1,1,1,1,1,1,1,1,1,1,1,1,1,1,1,1,1,1,1,1,1,1,
1,1,1,1,1,1,1,1,1,1,1,1,1,1,1,1,1,1,1,1,1,1,1,6),(-0.941429844438006,-0.940000000000001,
-0.935000000000001,-0.930000000000001,-0.925000000000001,-0.920000000000001,
-0.915000000000001,-0.910000000000001,-0.905000000000001,-0.900000000000001,
-0.895000000000001,-0.890000000000001,-0.885000000000001,-0.880000000000001,
-0.875000000000001,-0.870000000000001,-0.865000000000001,-0.860000000000001,
-0.855000000000001,-0.850000000000001,-0.845000000000001,-0.840000000000001,
-0.835000000000001,-0.830000000000001,-0.825000000000001,-0.820000000000001,
-0.815000000000001,-0.810000000000001,-0.805000000000001,-0.800000000000001,
-0.795000000000001,-0.790000000000001,-0.785000000000001,-0.780000000000001,
-0.775000000000001,-0.770000000000001,-0.765000000000001,-0.760000000000001,
-0.755000000000001,-0.750000000000001,-0.745000000000001,-0.740000000000001,
-0.735000000000001,-0.730000000000001,-0.725000000000001,-0.720000000000001,
-0.715000000000001,-0.710000000000001,-0.705000000000001,-0.700000000000001,
-0.695000000000001,-0.690000000000001,-0.685,-0.68,-0.675,-0.67,-0.665,
-0.66,-0.655,-0.65,-0.645,-0.64,-0.635,-0.63,-0.625,-0.62,-0.615,-0.61,
-0.605,-0.6,-0.595,-0.59,-0.585,-0.58,-0.575,-0.57,-0.565,-0.56,-0.555,
-0.55,-0.545,-0.54,-0.535,-0.53,-0.525,-0.52,-0.515,-0.51,-0.505,-0.5,-0.495,
-0.49,-0.485,-0.48,-0.475,-0.47,-0.465,-0.46,-0.455,-0.45,-0.445,-0.44,
-0.435,-0.43,-0.425,-0.42,-0.415,-0.41,-0.405,-0.4,-0.395,-0.39,-0.385,
-0.38,-0.375,-0.37,-0.365,-0.36,-0.355,-0.35,-0.345,-0.34,-0.335,-0.33,
-0.325,-0.32,-0.315,-0.31,-0.305,-0.3,-0.295,-0.29,-0.285,-0.28,-0.275,
-0.27,-0.265,-0.26,-0.255,-0.25,-0.245,-0.24,-0.235,-0.23,-0.225,-0.22,
-0.215,-0.21,-0.205,-0.2,-0.195,-0.19,-0.185,-0.18,-0.175,-0.17,-0.165,
-0.16,-0.155,-0.15,-0.145,-0.14,-0.135,-0.13,-0.125,-0.12,-0.115,-0.11,
-0.105,-0.1,-0.095,-0.09,-0.085,-0.08,-0.075,-0.07,-0.065,-0.06,-0.055,
-0.05,-0.045,-0.04,-0.035,-0.03,-0.025,-0.02,-0.015,-0.01,-0.005,0.),
 .UNSPECIFIED.)
CURVE()
GEOMETRIC_REPRESENTATION_ITEM()
RATIONAL_B_SPLINE_CURVE((1.,1.,1.,1.,1.,1.,1.,1.,1.,1.,1.,1.,1.,1.,1.,1.,
1.,1.,1.,1.,1.,1.,1.,1.,1.,1.,1.,1.,1.,1.,1.,1.,1.,1.,1.,1.,1.,1.,1.,1.,
1.,1.,1.,1.,1.,1.,1.,1.,1.,1.,1.,1.,1.,1.,1.,1.,1.,1.,1.,1.,1.,1.,1.,1.,
1.,1.,1.,1.,1.,1.,1.,1.,1.,1.,1.,1.,1.,1.,1.,1.,1.,1.,1.,1.,1.,1.,1.,1.,
1.,1.,1.,1.,1.,1.,1.,1.,1.,1.,1.,1.,1.,1.,1.,1.,1.,1.,1.,1.,1.,1.,1.,1.,
1.,1.,1.,1.,1.,1.,1.,1.,1.,1.,1.,1.,1.,1.,1.,1.,1.,1.,1.,1.,1.,1.,1.,1.,
1.,1.,1.,1.,1.,1.,1.,1.,1.,1.,1.,1.,1.,1.,1.,1.,1.,1.,1.,1.,1.,1.,1.,1.,
1.,1.,1.,1.,1.,1.,1.,1.,1.,1.,1.,1.,1.,1.,1.,1.,1.,1.,1.,1.,1.,1.,1.,1.,
1.,1.,1.,1.,1.,1.,1.,1.,1.,1.))
REPRESENTATION_ITEM('')
);
#677=(
BOUNDED_CURVE()
B_SPLINE_CURVE(5,(#169469,#169470,#169471,#169472,#169473,#169474,#169475,
#169476,#169477,#169478,#169479,#169480,#169481,#169482,#169483,#169484,
#169485,#169486,#169487,#169488,#169489,#169490,#169491,#169492,#169493,
#169494,#169495,#169496,#169497,#169498,#169499,#169500,#169501,#169502,
#169503,#169504,#169505,#169506,#169507,#169508,#169509,#169510,#169511,
#169512,#169513,#169514,#169515,#169516,#169517,#169518,#169519,#169520,
#169521,#169522,#169523,#169524,#169525,#169526,#169527,#169528,#169529,
#169530,#169531,#169532,#169533,#169534,#169535,#169536,#169537,#169538,
#169539,#169540,#169541,#169542,#169543,#169544,#169545,#169546,#169547,
#169548,#169549,#169550,#169551,#169552,#169553,#169554,#169555,#169556,
#169557,#169558,#169559,#169560,#169561,#169562,#169563,#169564,#169565,
#169566,#169567,#169568,#169569,#169570,#169571,#169572,#169573,#169574,
#169575,#169576,#169577,#169578,#169579,#169580,#169581,#169582,#169583,
#169584,#169585,#169586,#169587,#169588,#169589,#169590,#169591,#169592,
#169593,#169594,#169595,#169596,#169597,#169598,#169599,#169600,#169601,
#169602,#169603,#169604,#169605,#169606,#169607,#169608,#169609,#169610,
#169611,#169612,#169613,#169614,#169615,#169616,#169617,#169618,#169619,
#169620,#169621,#169622,#169623,#169624,#169625,#169626,#169627,#169628,
#169629,#169630,#169631,#169632,#169633,#169634,#169635,#169636,#169637,
#169638,#169639,#169640,#169641,#169642,#169643,#169644,#169645,#169646,
#169647,#169648,#169649,#169650,#169651,#169652,#169653,#169654,#169655,
#169656,#169657,#169658,#169659,#169660,#169661,#169662),.UNSPECIFIED.,
 .F.,.F.)
B_SPLINE_CURVE_WITH_KNOTS((6,1,1,1,1,1,1,1,1,1,1,1,1,1,1,1,1,1,1,1,1,1,
1,1,1,1,1,1,1,1,1,1,1,1,1,1,1,1,1,1,1,1,1,1,1,1,1,1,1,1,1,1,1,1,1,1,1,1,
1,1,1,1,1,1,1,1,1,1,1,1,1,1,1,1,1,1,1,1,1,1,1,1,1,1,1,1,1,1,1,1,1,1,1,1,
1,1,1,1,1,1,1,1,1,1,1,1,1,1,1,1,1,1,1,1,1,1,1,1,1,1,1,1,1,1,1,1,1,1,1,1,
1,1,1,1,1,1,1,1,1,1,1,1,1,1,1,1,1,1,1,1,1,1,1,1,1,1,1,1,1,1,1,1,1,1,1,1,
1,1,1,1,1,1,1,1,1,1,1,1,1,1,1,1,1,1,1,1,1,1,1,6),(0.,0.005,0.01,0.015,0.02,
0.025,0.03,0.035,0.04,0.045,0.05,0.055,0.06,0.065,0.07,0.075,0.08,0.085,
0.09,0.095,0.1,0.105,0.11,0.115,0.12,0.125,0.13,0.135,0.14,0.145,0.15,0.155,
0.16,0.165,0.17,0.175,0.18,0.185,0.19,0.195,0.2,0.205,0.21,0.215,0.22,0.225,
0.23,0.235,0.24,0.245,0.25,0.255,0.26,0.265,0.27,0.275,0.28,0.285,0.29,
0.295,0.3,0.305,0.31,0.315,0.32,0.325,0.33,0.335,0.34,0.345,0.35,0.355,
0.36,0.365,0.37,0.375,0.38,0.385,0.39,0.395,0.4,0.405,0.41,0.415,0.42,0.425,
0.43,0.435,0.44,0.445,0.45,0.455,0.46,0.465,0.47,0.475,0.48,0.485,0.49,
0.495,0.5,0.505,0.51,0.515,0.52,0.525,0.53,0.535,0.54,0.545,0.55,0.555,
0.56,0.565,0.57,0.575,0.58,0.585,0.59,0.595,0.6,0.605,0.61,0.615,0.62,0.625,
0.63,0.635,0.64,0.645,0.65,0.655,0.66,0.665,0.67,0.675,0.68,0.685,0.690000000000001,
0.695000000000001,0.700000000000001,0.705000000000001,0.710000000000001,
0.715000000000001,0.720000000000001,0.725000000000001,0.730000000000001,
0.735000000000001,0.740000000000001,0.745000000000001,0.750000000000001,
0.755000000000001,0.760000000000001,0.765000000000001,0.770000000000001,
0.775000000000001,0.780000000000001,0.785000000000001,0.790000000000001,
0.795000000000001,0.800000000000001,0.805000000000001,0.810000000000001,
0.815000000000001,0.820000000000001,0.825000000000001,0.830000000000001,
0.835000000000001,0.840000000000001,0.845000000000001,0.850000000000001,
0.855000000000001,0.860000000000001,0.865000000000001,0.870000000000001,
0.875000000000001,0.880000000000001,0.885000000000001,0.890000000000001,
0.895000000000001,0.900000000000001,0.905000000000001,0.910000000000001,
0.915000000000001,0.920000000000001,0.925000000000001,0.930000000000001,
0.935000000000001,0.940000000000001,0.94142984443808),.UNSPECIFIED.)
CURVE()
GEOMETRIC_REPRESENTATION_ITEM()
RATIONAL_B_SPLINE_CURVE((1.,1.,1.,1.,1.,1.,1.,1.,1.,1.,1.,1.,1.,1.,1.,1.,
1.,1.,1.,1.,1.,1.,1.,1.,1.,1.,1.,1.,1.,1.,1.,1.,1.,1.,1.,1.,1.,1.,1.,1.,
1.,1.,1.,1.,1.,1.,1.,1.,1.,1.,1.,1.,1.,1.,1.,1.,1.,1.,1.,1.,1.,1.,1.,1.,
1.,1.,1.,1.,1.,1.,1.,1.,1.,1.,1.,1.,1.,1.,1.,1.,1.,1.,1.,1.,1.,1.,1.,1.,
1.,1.,1.,1.,1.,1.,1.,1.,1.,1.,1.,1.,1.,1.,1.,1.,1.,1.,1.,1.,1.,1.,1.,1.,
1.,1.,1.,1.,1.,1.,1.,1.,1.,1.,1.,1.,1.,1.,1.,1.,1.,1.,1.,1.,1.,1.,1.,1.,
1.,1.,1.,1.,1.,1.,1.,1.,1.,1.,1.,1.,1.,1.,1.,1.,1.,1.,1.,1.,1.,1.,1.,1.,
1.,1.,1.,1.,1.,1.,1.,1.,1.,1.,1.,1.,1.,1.,1.,1.,1.,1.,1.,1.,1.,1.,1.,1.,
1.,1.,1.,1.,1.,1.,1.,1.,1.,1.))
REPRESENTATION_ITEM('')
);
#678=(
BOUNDED_CURVE()
B_SPLINE_CURVE(5,(#169665,#169666,#169667,#169668,#169669,#169670,#169671,
#169672,#169673,#169674,#169675,#169676,#169677,#169678,#169679,#169680,
#169681,#169682,#169683,#169684,#169685,#169686,#169687,#169688,#169689,
#169690,#169691,#169692,#169693,#169694,#169695,#169696,#169697,#169698,
#169699,#169700,#169701,#169702,#169703,#169704,#169705,#169706,#169707,
#169708,#169709,#169710,#169711,#169712,#169713,#169714,#169715,#169716,
#169717,#169718,#169719,#169720,#169721,#169722,#169723,#169724,#169725,
#169726,#169727,#169728,#169729,#169730,#169731,#169732,#169733,#169734,
#169735,#169736,#169737,#169738,#169739,#169740,#169741,#169742,#169743,
#169744,#169745,#169746,#169747,#169748,#169749,#169750,#169751,#169752,
#169753,#169754,#169755,#169756,#169757,#169758,#169759,#169760,#169761,
#169762,#169763,#169764,#169765,#169766,#169767,#169768,#169769,#169770,
#169771,#169772,#169773,#169774,#169775,#169776,#169777,#169778,#169779,
#169780,#169781,#169782,#169783,#169784,#169785,#169786,#169787,#169788,
#169789,#169790,#169791,#169792,#169793,#169794,#169795,#169796,#169797,
#169798,#169799,#169800,#169801,#169802,#169803,#169804,#169805,#169806,
#169807,#169808,#169809,#169810,#169811,#169812,#169813,#169814,#169815,
#169816,#169817,#169818,#169819,#169820,#169821,#169822,#169823,#169824,
#169825,#169826,#169827,#169828,#169829,#169830,#169831,#169832,#169833,
#169834,#169835,#169836,#169837,#169838,#169839,#169840,#169841,#169842,
#169843,#169844,#169845,#169846,#169847,#169848,#169849,#169850,#169851,
#169852,#169853,#169854,#169855,#169856,#169857,#169858),.UNSPECIFIED.,
 .F.,.F.)
B_SPLINE_CURVE_WITH_KNOTS((6,1,1,1,1,1,1,1,1,1,1,1,1,1,1,1,1,1,1,1,1,1,
1,1,1,1,1,1,1,1,1,1,1,1,1,1,1,1,1,1,1,1,1,1,1,1,1,1,1,1,1,1,1,1,1,1,1,1,
1,1,1,1,1,1,1,1,1,1,1,1,1,1,1,1,1,1,1,1,1,1,1,1,1,1,1,1,1,1,1,1,1,1,1,1,
1,1,1,1,1,1,1,1,1,1,1,1,1,1,1,1,1,1,1,1,1,1,1,1,1,1,1,1,1,1,1,1,1,1,1,1,
1,1,1,1,1,1,1,1,1,1,1,1,1,1,1,1,1,1,1,1,1,1,1,1,1,1,1,1,1,1,1,1,1,1,1,1,
1,1,1,1,1,1,1,1,1,1,1,1,1,1,1,1,1,1,1,1,1,1,1,6),(-0.941429844438109,-0.940000000000001,
-0.935000000000001,-0.930000000000001,-0.925000000000001,-0.920000000000001,
-0.915000000000001,-0.910000000000001,-0.905000000000001,-0.900000000000001,
-0.895000000000001,-0.890000000000001,-0.885000000000001,-0.880000000000001,
-0.875000000000001,-0.870000000000001,-0.865000000000001,-0.860000000000001,
-0.855000000000001,-0.850000000000001,-0.845000000000001,-0.840000000000001,
-0.835000000000001,-0.830000000000001,-0.825000000000001,-0.820000000000001,
-0.815000000000001,-0.810000000000001,-0.805000000000001,-0.800000000000001,
-0.795000000000001,-0.790000000000001,-0.785000000000001,-0.780000000000001,
-0.775000000000001,-0.770000000000001,-0.765000000000001,-0.760000000000001,
-0.755000000000001,-0.750000000000001,-0.745000000000001,-0.740000000000001,
-0.735000000000001,-0.730000000000001,-0.725000000000001,-0.720000000000001,
-0.715000000000001,-0.710000000000001,-0.705000000000001,-0.700000000000001,
-0.695000000000001,-0.690000000000001,-0.685,-0.68,-0.675,-0.67,-0.665,
-0.66,-0.655,-0.65,-0.645,-0.64,-0.635,-0.63,-0.625,-0.62,-0.615,-0.61,
-0.605,-0.6,-0.595,-0.59,-0.585,-0.58,-0.575,-0.57,-0.565,-0.56,-0.555,
-0.55,-0.545,-0.54,-0.535,-0.53,-0.525,-0.52,-0.515,-0.51,-0.505,-0.5,-0.495,
-0.49,-0.485,-0.48,-0.475,-0.47,-0.465,-0.46,-0.455,-0.45,-0.445,-0.44,
-0.435,-0.43,-0.425,-0.42,-0.415,-0.41,-0.405,-0.4,-0.395,-0.39,-0.385,
-0.38,-0.375,-0.37,-0.365,-0.36,-0.355,-0.35,-0.345,-0.34,-0.335,-0.33,
-0.325,-0.32,-0.315,-0.31,-0.305,-0.3,-0.295,-0.29,-0.285,-0.28,-0.275,
-0.27,-0.265,-0.26,-0.255,-0.25,-0.245,-0.24,-0.235,-0.23,-0.225,-0.22,
-0.215,-0.21,-0.205,-0.2,-0.195,-0.19,-0.185,-0.18,-0.175,-0.17,-0.165,
-0.16,-0.155,-0.15,-0.145,-0.14,-0.135,-0.13,-0.125,-0.12,-0.115,-0.11,
-0.105,-0.1,-0.095,-0.09,-0.085,-0.08,-0.075,-0.07,-0.065,-0.06,-0.055,
-0.05,-0.045,-0.04,-0.035,-0.03,-0.025,-0.02,-0.015,-0.01,-0.005,0.),
 .UNSPECIFIED.)
CURVE()
GEOMETRIC_REPRESENTATION_ITEM()
RATIONAL_B_SPLINE_CURVE((1.,1.,1.,1.,1.,1.,1.,1.,1.,1.,1.,1.,1.,1.,1.,1.,
1.,1.,1.,1.,1.,1.,1.,1.,1.,1.,1.,1.,1.,1.,1.,1.,1.,1.,1.,1.,1.,1.,1.,1.,
1.,1.,1.,1.,1.,1.,1.,1.,1.,1.,1.,1.,1.,1.,1.,1.,1.,1.,1.,1.,1.,1.,1.,1.,
1.,1.,1.,1.,1.,1.,1.,1.,1.,1.,1.,1.,1.,1.,1.,1.,1.,1.,1.,1.,1.,1.,1.,1.,
1.,1.,1.,1.,1.,1.,1.,1.,1.,1.,1.,1.,1.,1.,1.,1.,1.,1.,1.,1.,1.,1.,1.,1.,
1.,1.,1.,1.,1.,1.,1.,1.,1.,1.,1.,1.,1.,1.,1.,1.,1.,1.,1.,1.,1.,1.,1.,1.,
1.,1.,1.,1.,1.,1.,1.,1.,1.,1.,1.,1.,1.,1.,1.,1.,1.,1.,1.,1.,1.,1.,1.,1.,
1.,1.,1.,1.,1.,1.,1.,1.,1.,1.,1.,1.,1.,1.,1.,1.,1.,1.,1.,1.,1.,1.,1.,1.,
1.,1.,1.,1.,1.,1.,1.,1.,1.,1.))
REPRESENTATION_ITEM('')
);
#679=(
BOUNDED_CURVE()
B_SPLINE_CURVE(5,(#170270,#170271,#170272,#170273,#170274,#170275,#170276,
#170277,#170278,#170279,#170280,#170281,#170282,#170283,#170284,#170285,
#170286,#170287,#170288,#170289,#170290,#170291,#170292,#170293,#170294,
#170295,#170296,#170297,#170298,#170299,#170300,#170301,#170302,#170303,
#170304,#170305,#170306,#170307,#170308,#170309,#170310,#170311,#170312,
#170313,#170314,#170315,#170316,#170317,#170318,#170319,#170320,#170321,
#170322,#170323,#170324,#170325,#170326,#170327,#170328,#170329,#170330,
#170331,#170332,#170333,#170334,#170335,#170336,#170337,#170338,#170339,
#170340,#170341,#170342,#170343,#170344,#170345,#170346,#170347,#170348,
#170349,#170350,#170351,#170352,#170353,#170354,#170355,#170356,#170357,
#170358,#170359,#170360,#170361,#170362,#170363,#170364,#170365,#170366,
#170367,#170368,#170369,#170370,#170371,#170372,#170373,#170374,#170375,
#170376,#170377,#170378,#170379,#170380,#170381,#170382,#170383,#170384,
#170385,#170386,#170387,#170388,#170389,#170390,#170391,#170392,#170393,
#170394,#170395,#170396,#170397,#170398,#170399,#170400,#170401,#170402,
#170403,#170404,#170405,#170406,#170407,#170408,#170409,#170410,#170411,
#170412,#170413,#170414,#170415,#170416,#170417,#170418,#170419,#170420,
#170421,#170422,#170423,#170424,#170425,#170426,#170427,#170428,#170429,
#170430,#170431,#170432,#170433,#170434,#170435,#170436,#170437,#170438,
#170439,#170440,#170441,#170442,#170443,#170444,#170445,#170446,#170447,
#170448,#170449,#170450,#170451,#170452,#170453,#170454,#170455,#170456,
#170457,#170458,#170459,#170460,#170461,#170462,#170463),.UNSPECIFIED.,
 .F.,.F.)
B_SPLINE_CURVE_WITH_KNOTS((6,1,1,1,1,1,1,1,1,1,1,1,1,1,1,1,1,1,1,1,1,1,
1,1,1,1,1,1,1,1,1,1,1,1,1,1,1,1,1,1,1,1,1,1,1,1,1,1,1,1,1,1,1,1,1,1,1,1,
1,1,1,1,1,1,1,1,1,1,1,1,1,1,1,1,1,1,1,1,1,1,1,1,1,1,1,1,1,1,1,1,1,1,1,1,
1,1,1,1,1,1,1,1,1,1,1,1,1,1,1,1,1,1,1,1,1,1,1,1,1,1,1,1,1,1,1,1,1,1,1,1,
1,1,1,1,1,1,1,1,1,1,1,1,1,1,1,1,1,1,1,1,1,1,1,1,1,1,1,1,1,1,1,1,1,1,1,1,
1,1,1,1,1,1,1,1,1,1,1,1,1,1,1,1,1,1,1,1,1,1,1,6),(0.,0.005,0.01,0.015,0.02,
0.025,0.03,0.035,0.04,0.045,0.05,0.055,0.06,0.065,0.07,0.075,0.08,0.085,
0.09,0.095,0.1,0.105,0.11,0.115,0.12,0.125,0.13,0.135,0.14,0.145,0.15,0.155,
0.16,0.165,0.17,0.175,0.18,0.185,0.19,0.195,0.2,0.205,0.21,0.215,0.22,0.225,
0.23,0.235,0.24,0.245,0.25,0.255,0.26,0.265,0.27,0.275,0.28,0.285,0.29,
0.295,0.3,0.305,0.31,0.315,0.32,0.325,0.33,0.335,0.34,0.345,0.35,0.355,
0.36,0.365,0.37,0.375,0.38,0.385,0.39,0.395,0.4,0.405,0.41,0.415,0.42,0.425,
0.43,0.435,0.44,0.445,0.45,0.455,0.46,0.465,0.47,0.475,0.48,0.485,0.49,
0.495,0.5,0.505,0.51,0.515,0.52,0.525,0.53,0.535,0.54,0.545,0.55,0.555,
0.56,0.565,0.57,0.575,0.58,0.585,0.59,0.595,0.6,0.605,0.61,0.615,0.62,0.625,
0.63,0.635,0.64,0.645,0.65,0.655,0.66,0.665,0.67,0.675,0.68,0.685,0.690000000000001,
0.695000000000001,0.700000000000001,0.705000000000001,0.710000000000001,
0.715000000000001,0.720000000000001,0.725000000000001,0.730000000000001,
0.735000000000001,0.740000000000001,0.745000000000001,0.750000000000001,
0.755000000000001,0.760000000000001,0.765000000000001,0.770000000000001,
0.775000000000001,0.780000000000001,0.785000000000001,0.790000000000001,
0.795000000000001,0.800000000000001,0.805000000000001,0.810000000000001,
0.815000000000001,0.820000000000001,0.825000000000001,0.830000000000001,
0.835000000000001,0.840000000000001,0.845000000000001,0.850000000000001,
0.855000000000001,0.860000000000001,0.865000000000001,0.870000000000001,
0.875000000000001,0.880000000000001,0.885000000000001,0.890000000000001,
0.895000000000001,0.900000000000001,0.905000000000001,0.910000000000001,
0.915000000000001,0.920000000000001,0.925000000000001,0.930000000000001,
0.935000000000001,0.940000000000001,0.941429844438046),.UNSPECIFIED.)
CURVE()
GEOMETRIC_REPRESENTATION_ITEM()
RATIONAL_B_SPLINE_CURVE((1.,1.,1.,1.,1.,1.,1.,1.,1.,1.,1.,1.,1.,1.,1.,1.,
1.,1.,1.,1.,1.,1.,1.,1.,1.,1.,1.,1.,1.,1.,1.,1.,1.,1.,1.,1.,1.,1.,1.,1.,
1.,1.,1.,1.,1.,1.,1.,1.,1.,1.,1.,1.,1.,1.,1.,1.,1.,1.,1.,1.,1.,1.,1.,1.,
1.,1.,1.,1.,1.,1.,1.,1.,1.,1.,1.,1.,1.,1.,1.,1.,1.,1.,1.,1.,1.,1.,1.,1.,
1.,1.,1.,1.,1.,1.,1.,1.,1.,1.,1.,1.,1.,1.,1.,1.,1.,1.,1.,1.,1.,1.,1.,1.,
1.,1.,1.,1.,1.,1.,1.,1.,1.,1.,1.,1.,1.,1.,1.,1.,1.,1.,1.,1.,1.,1.,1.,1.,
1.,1.,1.,1.,1.,1.,1.,1.,1.,1.,1.,1.,1.,1.,1.,1.,1.,1.,1.,1.,1.,1.,1.,1.,
1.,1.,1.,1.,1.,1.,1.,1.,1.,1.,1.,1.,1.,1.,1.,1.,1.,1.,1.,1.,1.,1.,1.,1.,
1.,1.,1.,1.,1.,1.,1.,1.,1.,1.))
REPRESENTATION_ITEM('')
);
#680=(
BOUNDED_CURVE()
B_SPLINE_CURVE(5,(#170466,#170467,#170468,#170469,#170470,#170471,#170472,
#170473,#170474,#170475,#170476,#170477,#170478,#170479,#170480,#170481,
#170482,#170483,#170484,#170485,#170486,#170487,#170488,#170489,#170490,
#170491,#170492,#170493,#170494,#170495,#170496,#170497,#170498,#170499,
#170500,#170501,#170502,#170503,#170504,#170505,#170506,#170507,#170508,
#170509,#170510,#170511,#170512,#170513,#170514,#170515,#170516,#170517,
#170518,#170519,#170520,#170521,#170522,#170523,#170524,#170525,#170526,
#170527,#170528,#170529,#170530,#170531,#170532,#170533,#170534,#170535,
#170536,#170537,#170538,#170539,#170540,#170541,#170542,#170543,#170544,
#170545,#170546,#170547,#170548,#170549,#170550,#170551,#170552,#170553,
#170554,#170555,#170556,#170557,#170558,#170559,#170560,#170561,#170562,
#170563,#170564,#170565,#170566,#170567,#170568,#170569,#170570,#170571,
#170572,#170573,#170574,#170575,#170576,#170577,#170578,#170579,#170580,
#170581,#170582,#170583,#170584,#170585,#170586,#170587,#170588,#170589,
#170590,#170591,#170592,#170593,#170594,#170595,#170596,#170597,#170598,
#170599,#170600,#170601,#170602,#170603,#170604,#170605,#170606,#170607,
#170608,#170609,#170610,#170611,#170612,#170613,#170614,#170615,#170616,
#170617,#170618,#170619,#170620,#170621,#170622,#170623,#170624,#170625,
#170626,#170627,#170628,#170629,#170630,#170631,#170632,#170633,#170634,
#170635,#170636,#170637,#170638,#170639,#170640,#170641,#170642,#170643,
#170644,#170645,#170646,#170647,#170648,#170649,#170650,#170651,#170652,
#170653,#170654,#170655,#170656,#170657,#170658,#170659),.UNSPECIFIED.,
 .F.,.F.)
B_SPLINE_CURVE_WITH_KNOTS((6,1,1,1,1,1,1,1,1,1,1,1,1,1,1,1,1,1,1,1,1,1,
1,1,1,1,1,1,1,1,1,1,1,1,1,1,1,1,1,1,1,1,1,1,1,1,1,1,1,1,1,1,1,1,1,1,1,1,
1,1,1,1,1,1,1,1,1,1,1,1,1,1,1,1,1,1,1,1,1,1,1,1,1,1,1,1,1,1,1,1,1,1,1,1,
1,1,1,1,1,1,1,1,1,1,1,1,1,1,1,1,1,1,1,1,1,1,1,1,1,1,1,1,1,1,1,1,1,1,1,1,
1,1,1,1,1,1,1,1,1,1,1,1,1,1,1,1,1,1,1,1,1,1,1,1,1,1,1,1,1,1,1,1,1,1,1,1,
1,1,1,1,1,1,1,1,1,1,1,1,1,1,1,1,1,1,1,1,1,1,1,6),(-0.941429844438047,-0.940000000000001,
-0.935000000000001,-0.930000000000001,-0.925000000000001,-0.920000000000001,
-0.915000000000001,-0.910000000000001,-0.905000000000001,-0.900000000000001,
-0.895000000000001,-0.890000000000001,-0.885000000000001,-0.880000000000001,
-0.875000000000001,-0.870000000000001,-0.865000000000001,-0.860000000000001,
-0.855000000000001,-0.850000000000001,-0.845000000000001,-0.840000000000001,
-0.835000000000001,-0.830000000000001,-0.825000000000001,-0.820000000000001,
-0.815000000000001,-0.810000000000001,-0.805000000000001,-0.800000000000001,
-0.795000000000001,-0.790000000000001,-0.785000000000001,-0.780000000000001,
-0.775000000000001,-0.770000000000001,-0.765000000000001,-0.760000000000001,
-0.755000000000001,-0.750000000000001,-0.745000000000001,-0.740000000000001,
-0.735000000000001,-0.730000000000001,-0.725000000000001,-0.720000000000001,
-0.715000000000001,-0.710000000000001,-0.705000000000001,-0.700000000000001,
-0.695000000000001,-0.690000000000001,-0.685,-0.68,-0.675,-0.67,-0.665,
-0.66,-0.655,-0.65,-0.645,-0.64,-0.635,-0.63,-0.625,-0.62,-0.615,-0.61,
-0.605,-0.6,-0.595,-0.59,-0.585,-0.58,-0.575,-0.57,-0.565,-0.56,-0.555,
-0.55,-0.545,-0.54,-0.535,-0.53,-0.525,-0.52,-0.515,-0.51,-0.505,-0.5,-0.495,
-0.49,-0.485,-0.48,-0.475,-0.47,-0.465,-0.46,-0.455,-0.45,-0.445,-0.44,
-0.435,-0.43,-0.425,-0.42,-0.415,-0.41,-0.405,-0.4,-0.395,-0.39,-0.385,
-0.38,-0.375,-0.37,-0.365,-0.36,-0.355,-0.35,-0.345,-0.34,-0.335,-0.33,
-0.325,-0.32,-0.315,-0.31,-0.305,-0.3,-0.295,-0.29,-0.285,-0.28,-0.275,
-0.27,-0.265,-0.26,-0.255,-0.25,-0.245,-0.24,-0.235,-0.23,-0.225,-0.22,
-0.215,-0.21,-0.205,-0.2,-0.195,-0.19,-0.185,-0.18,-0.175,-0.17,-0.165,
-0.16,-0.155,-0.15,-0.145,-0.14,-0.135,-0.13,-0.125,-0.12,-0.115,-0.11,
-0.105,-0.1,-0.095,-0.09,-0.085,-0.08,-0.075,-0.07,-0.065,-0.06,-0.055,
-0.05,-0.045,-0.04,-0.035,-0.03,-0.025,-0.02,-0.015,-0.01,-0.005,0.),
 .UNSPECIFIED.)
CURVE()
GEOMETRIC_REPRESENTATION_ITEM()
RATIONAL_B_SPLINE_CURVE((1.,1.,1.,1.,1.,1.,1.,1.,1.,1.,1.,1.,1.,1.,1.,1.,
1.,1.,1.,1.,1.,1.,1.,1.,1.,1.,1.,1.,1.,1.,1.,1.,1.,1.,1.,1.,1.,1.,1.,1.,
1.,1.,1.,1.,1.,1.,1.,1.,1.,1.,1.,1.,1.,1.,1.,1.,1.,1.,1.,1.,1.,1.,1.,1.,
1.,1.,1.,1.,1.,1.,1.,1.,1.,1.,1.,1.,1.,1.,1.,1.,1.,1.,1.,1.,1.,1.,1.,1.,
1.,1.,1.,1.,1.,1.,1.,1.,1.,1.,1.,1.,1.,1.,1.,1.,1.,1.,1.,1.,1.,1.,1.,1.,
1.,1.,1.,1.,1.,1.,1.,1.,1.,1.,1.,1.,1.,1.,1.,1.,1.,1.,1.,1.,1.,1.,1.,1.,
1.,1.,1.,1.,1.,1.,1.,1.,1.,1.,1.,1.,1.,1.,1.,1.,1.,1.,1.,1.,1.,1.,1.,1.,
1.,1.,1.,1.,1.,1.,1.,1.,1.,1.,1.,1.,1.,1.,1.,1.,1.,1.,1.,1.,1.,1.,1.,1.,
1.,1.,1.,1.,1.,1.,1.,1.,1.,1.))
REPRESENTATION_ITEM('')
);
#681=(
BOUNDED_CURVE()
B_SPLINE_CURVE(5,(#171071,#171072,#171073,#171074,#171075,#171076,#171077,
#171078,#171079,#171080,#171081,#171082,#171083,#171084,#171085,#171086,
#171087,#171088,#171089,#171090,#171091,#171092,#171093,#171094,#171095,
#171096,#171097,#171098,#171099,#171100,#171101,#171102,#171103,#171104,
#171105,#171106,#171107,#171108,#171109,#171110,#171111,#171112,#171113,
#171114,#171115,#171116,#171117,#171118,#171119,#171120,#171121,#171122,
#171123,#171124,#171125,#171126,#171127,#171128,#171129,#171130,#171131,
#171132,#171133,#171134,#171135,#171136,#171137,#171138,#171139,#171140,
#171141,#171142,#171143,#171144,#171145,#171146,#171147,#171148,#171149,
#171150,#171151,#171152,#171153,#171154,#171155,#171156,#171157,#171158,
#171159,#171160,#171161,#171162,#171163,#171164,#171165,#171166,#171167,
#171168,#171169,#171170,#171171,#171172,#171173,#171174,#171175,#171176,
#171177,#171178,#171179,#171180,#171181,#171182,#171183,#171184,#171185,
#171186,#171187,#171188,#171189,#171190,#171191,#171192,#171193,#171194,
#171195,#171196,#171197,#171198,#171199,#171200,#171201,#171202,#171203,
#171204,#171205,#171206,#171207,#171208,#171209,#171210,#171211,#171212,
#171213,#171214,#171215,#171216,#171217,#171218,#171219,#171220,#171221,
#171222,#171223,#171224,#171225,#171226,#171227,#171228,#171229,#171230,
#171231,#171232,#171233,#171234,#171235,#171236,#171237,#171238,#171239,
#171240,#171241,#171242,#171243,#171244,#171245,#171246,#171247,#171248,
#171249,#171250,#171251,#171252,#171253,#171254,#171255,#171256,#171257,
#171258,#171259,#171260,#171261,#171262,#171263,#171264),.UNSPECIFIED.,
 .F.,.F.)
B_SPLINE_CURVE_WITH_KNOTS((6,1,1,1,1,1,1,1,1,1,1,1,1,1,1,1,1,1,1,1,1,1,
1,1,1,1,1,1,1,1,1,1,1,1,1,1,1,1,1,1,1,1,1,1,1,1,1,1,1,1,1,1,1,1,1,1,1,1,
1,1,1,1,1,1,1,1,1,1,1,1,1,1,1,1,1,1,1,1,1,1,1,1,1,1,1,1,1,1,1,1,1,1,1,1,
1,1,1,1,1,1,1,1,1,1,1,1,1,1,1,1,1,1,1,1,1,1,1,1,1,1,1,1,1,1,1,1,1,1,1,1,
1,1,1,1,1,1,1,1,1,1,1,1,1,1,1,1,1,1,1,1,1,1,1,1,1,1,1,1,1,1,1,1,1,1,1,1,
1,1,1,1,1,1,1,1,1,1,1,1,1,1,1,1,1,1,1,1,1,1,1,6),(0.,0.005,0.01,0.015,0.02,
0.025,0.03,0.035,0.04,0.045,0.05,0.055,0.06,0.065,0.07,0.075,0.08,0.085,
0.09,0.095,0.1,0.105,0.11,0.115,0.12,0.125,0.13,0.135,0.14,0.145,0.15,0.155,
0.16,0.165,0.17,0.175,0.18,0.185,0.19,0.195,0.2,0.205,0.21,0.215,0.22,0.225,
0.23,0.235,0.24,0.245,0.25,0.255,0.26,0.265,0.27,0.275,0.28,0.285,0.29,
0.295,0.3,0.305,0.31,0.315,0.32,0.325,0.33,0.335,0.34,0.345,0.35,0.355,
0.36,0.365,0.37,0.375,0.38,0.385,0.39,0.395,0.4,0.405,0.41,0.415,0.42,0.425,
0.43,0.435,0.44,0.445,0.45,0.455,0.46,0.465,0.47,0.475,0.48,0.485,0.49,
0.495,0.5,0.505,0.51,0.515,0.52,0.525,0.53,0.535,0.54,0.545,0.55,0.555,
0.56,0.565,0.57,0.575,0.58,0.585,0.59,0.595,0.6,0.605,0.61,0.615,0.62,0.625,
0.63,0.635,0.64,0.645,0.65,0.655,0.66,0.665,0.67,0.675,0.68,0.685,0.690000000000001,
0.695000000000001,0.700000000000001,0.705000000000001,0.710000000000001,
0.715000000000001,0.720000000000001,0.725000000000001,0.730000000000001,
0.735000000000001,0.740000000000001,0.745000000000001,0.750000000000001,
0.755000000000001,0.760000000000001,0.765000000000001,0.770000000000001,
0.775000000000001,0.780000000000001,0.785000000000001,0.790000000000001,
0.795000000000001,0.800000000000001,0.805000000000001,0.810000000000001,
0.815000000000001,0.820000000000001,0.825000000000001,0.830000000000001,
0.835000000000001,0.840000000000001,0.845000000000001,0.850000000000001,
0.855000000000001,0.860000000000001,0.865000000000001,0.870000000000001,
0.875000000000001,0.880000000000001,0.885000000000001,0.890000000000001,
0.895000000000001,0.900000000000001,0.905000000000001,0.910000000000001,
0.915000000000001,0.920000000000001,0.925000000000001,0.930000000000001,
0.935000000000001,0.940000000000001,0.94142984443807),.UNSPECIFIED.)
CURVE()
GEOMETRIC_REPRESENTATION_ITEM()
RATIONAL_B_SPLINE_CURVE((1.,1.,1.,1.,1.,1.,1.,1.,1.,1.,1.,1.,1.,1.,1.,1.,
1.,1.,1.,1.,1.,1.,1.,1.,1.,1.,1.,1.,1.,1.,1.,1.,1.,1.,1.,1.,1.,1.,1.,1.,
1.,1.,1.,1.,1.,1.,1.,1.,1.,1.,1.,1.,1.,1.,1.,1.,1.,1.,1.,1.,1.,1.,1.,1.,
1.,1.,1.,1.,1.,1.,1.,1.,1.,1.,1.,1.,1.,1.,1.,1.,1.,1.,1.,1.,1.,1.,1.,1.,
1.,1.,1.,1.,1.,1.,1.,1.,1.,1.,1.,1.,1.,1.,1.,1.,1.,1.,1.,1.,1.,1.,1.,1.,
1.,1.,1.,1.,1.,1.,1.,1.,1.,1.,1.,1.,1.,1.,1.,1.,1.,1.,1.,1.,1.,1.,1.,1.,
1.,1.,1.,1.,1.,1.,1.,1.,1.,1.,1.,1.,1.,1.,1.,1.,1.,1.,1.,1.,1.,1.,1.,1.,
1.,1.,1.,1.,1.,1.,1.,1.,1.,1.,1.,1.,1.,1.,1.,1.,1.,1.,1.,1.,1.,1.,1.,1.,
1.,1.,1.,1.,1.,1.,1.,1.,1.,1.))
REPRESENTATION_ITEM('')
);
#682=(
BOUNDED_CURVE()
B_SPLINE_CURVE(5,(#171267,#171268,#171269,#171270,#171271,#171272,#171273,
#171274,#171275,#171276,#171277,#171278,#171279,#171280,#171281,#171282,
#171283,#171284,#171285,#171286,#171287,#171288,#171289,#171290,#171291,
#171292,#171293,#171294,#171295,#171296,#171297,#171298,#171299,#171300,
#171301,#171302,#171303,#171304,#171305,#171306,#171307,#171308,#171309,
#171310,#171311,#171312,#171313,#171314,#171315,#171316,#171317,#171318,
#171319,#171320,#171321,#171322,#171323,#171324,#171325,#171326,#171327,
#171328,#171329,#171330,#171331,#171332,#171333,#171334,#171335,#171336,
#171337,#171338,#171339,#171340,#171341,#171342,#171343,#171344,#171345,
#171346,#171347,#171348,#171349,#171350,#171351,#171352,#171353,#171354,
#171355,#171356,#171357,#171358,#171359,#171360,#171361,#171362,#171363,
#171364,#171365,#171366,#171367,#171368,#171369,#171370,#171371,#171372,
#171373,#171374,#171375,#171376,#171377,#171378,#171379,#171380,#171381,
#171382,#171383,#171384,#171385,#171386,#171387,#171388,#171389,#171390,
#171391,#171392,#171393,#171394,#171395,#171396,#171397,#171398,#171399,
#171400,#171401,#171402,#171403,#171404,#171405,#171406,#171407,#171408,
#171409,#171410,#171411,#171412,#171413,#171414,#171415,#171416,#171417,
#171418,#171419,#171420,#171421,#171422,#171423,#171424,#171425,#171426,
#171427,#171428,#171429,#171430,#171431,#171432,#171433,#171434,#171435,
#171436,#171437,#171438,#171439,#171440,#171441,#171442,#171443,#171444,
#171445,#171446,#171447,#171448,#171449,#171450,#171451,#171452,#171453,
#171454,#171455,#171456,#171457,#171458,#171459,#171460),.UNSPECIFIED.,
 .F.,.F.)
B_SPLINE_CURVE_WITH_KNOTS((6,1,1,1,1,1,1,1,1,1,1,1,1,1,1,1,1,1,1,1,1,1,
1,1,1,1,1,1,1,1,1,1,1,1,1,1,1,1,1,1,1,1,1,1,1,1,1,1,1,1,1,1,1,1,1,1,1,1,
1,1,1,1,1,1,1,1,1,1,1,1,1,1,1,1,1,1,1,1,1,1,1,1,1,1,1,1,1,1,1,1,1,1,1,1,
1,1,1,1,1,1,1,1,1,1,1,1,1,1,1,1,1,1,1,1,1,1,1,1,1,1,1,1,1,1,1,1,1,1,1,1,
1,1,1,1,1,1,1,1,1,1,1,1,1,1,1,1,1,1,1,1,1,1,1,1,1,1,1,1,1,1,1,1,1,1,1,1,
1,1,1,1,1,1,1,1,1,1,1,1,1,1,1,1,1,1,1,1,1,1,1,6),(-0.941429844438063,-0.940000000000001,
-0.935000000000001,-0.930000000000001,-0.925000000000001,-0.920000000000001,
-0.915000000000001,-0.910000000000001,-0.905000000000001,-0.900000000000001,
-0.895000000000001,-0.890000000000001,-0.885000000000001,-0.880000000000001,
-0.875000000000001,-0.870000000000001,-0.865000000000001,-0.860000000000001,
-0.855000000000001,-0.850000000000001,-0.845000000000001,-0.840000000000001,
-0.835000000000001,-0.830000000000001,-0.825000000000001,-0.820000000000001,
-0.815000000000001,-0.810000000000001,-0.805000000000001,-0.800000000000001,
-0.795000000000001,-0.790000000000001,-0.785000000000001,-0.780000000000001,
-0.775000000000001,-0.770000000000001,-0.765000000000001,-0.760000000000001,
-0.755000000000001,-0.750000000000001,-0.745000000000001,-0.740000000000001,
-0.735000000000001,-0.730000000000001,-0.725000000000001,-0.720000000000001,
-0.715000000000001,-0.710000000000001,-0.705000000000001,-0.700000000000001,
-0.695000000000001,-0.690000000000001,-0.685,-0.68,-0.675,-0.67,-0.665,
-0.66,-0.655,-0.65,-0.645,-0.64,-0.635,-0.63,-0.625,-0.62,-0.615,-0.61,
-0.605,-0.6,-0.595,-0.59,-0.585,-0.58,-0.575,-0.57,-0.565,-0.56,-0.555,
-0.55,-0.545,-0.54,-0.535,-0.53,-0.525,-0.52,-0.515,-0.51,-0.505,-0.5,-0.495,
-0.49,-0.485,-0.48,-0.475,-0.47,-0.465,-0.46,-0.455,-0.45,-0.445,-0.44,
-0.435,-0.43,-0.425,-0.42,-0.415,-0.41,-0.405,-0.4,-0.395,-0.39,-0.385,
-0.38,-0.375,-0.37,-0.365,-0.36,-0.355,-0.35,-0.345,-0.34,-0.335,-0.33,
-0.325,-0.32,-0.315,-0.31,-0.305,-0.3,-0.295,-0.29,-0.285,-0.28,-0.275,
-0.27,-0.265,-0.26,-0.255,-0.25,-0.245,-0.24,-0.235,-0.23,-0.225,-0.22,
-0.215,-0.21,-0.205,-0.2,-0.195,-0.19,-0.185,-0.18,-0.175,-0.17,-0.165,
-0.16,-0.155,-0.15,-0.145,-0.14,-0.135,-0.13,-0.125,-0.12,-0.115,-0.11,
-0.105,-0.1,-0.095,-0.09,-0.085,-0.08,-0.075,-0.07,-0.065,-0.06,-0.055,
-0.05,-0.045,-0.04,-0.035,-0.03,-0.025,-0.02,-0.015,-0.01,-0.005,0.),
 .UNSPECIFIED.)
CURVE()
GEOMETRIC_REPRESENTATION_ITEM()
RATIONAL_B_SPLINE_CURVE((1.,1.,1.,1.,1.,1.,1.,1.,1.,1.,1.,1.,1.,1.,1.,1.,
1.,1.,1.,1.,1.,1.,1.,1.,1.,1.,1.,1.,1.,1.,1.,1.,1.,1.,1.,1.,1.,1.,1.,1.,
1.,1.,1.,1.,1.,1.,1.,1.,1.,1.,1.,1.,1.,1.,1.,1.,1.,1.,1.,1.,1.,1.,1.,1.,
1.,1.,1.,1.,1.,1.,1.,1.,1.,1.,1.,1.,1.,1.,1.,1.,1.,1.,1.,1.,1.,1.,1.,1.,
1.,1.,1.,1.,1.,1.,1.,1.,1.,1.,1.,1.,1.,1.,1.,1.,1.,1.,1.,1.,1.,1.,1.,1.,
1.,1.,1.,1.,1.,1.,1.,1.,1.,1.,1.,1.,1.,1.,1.,1.,1.,1.,1.,1.,1.,1.,1.,1.,
1.,1.,1.,1.,1.,1.,1.,1.,1.,1.,1.,1.,1.,1.,1.,1.,1.,1.,1.,1.,1.,1.,1.,1.,
1.,1.,1.,1.,1.,1.,1.,1.,1.,1.,1.,1.,1.,1.,1.,1.,1.,1.,1.,1.,1.,1.,1.,1.,
1.,1.,1.,1.,1.,1.,1.,1.,1.,1.))
REPRESENTATION_ITEM('')
);
#683=(
BOUNDED_CURVE()
B_SPLINE_CURVE(5,(#171872,#171873,#171874,#171875,#171876,#171877,#171878,
#171879,#171880,#171881,#171882,#171883,#171884,#171885,#171886,#171887,
#171888,#171889,#171890,#171891,#171892,#171893,#171894,#171895,#171896,
#171897,#171898,#171899,#171900,#171901,#171902,#171903,#171904,#171905,
#171906,#171907,#171908,#171909,#171910,#171911,#171912,#171913,#171914,
#171915,#171916,#171917,#171918,#171919,#171920,#171921,#171922,#171923,
#171924,#171925,#171926,#171927,#171928,#171929,#171930,#171931,#171932,
#171933,#171934,#171935,#171936,#171937,#171938,#171939,#171940,#171941,
#171942,#171943,#171944,#171945,#171946,#171947,#171948,#171949,#171950,
#171951,#171952,#171953,#171954,#171955,#171956,#171957,#171958,#171959,
#171960,#171961,#171962,#171963,#171964,#171965,#171966,#171967,#171968,
#171969,#171970,#171971,#171972,#171973,#171974,#171975,#171976,#171977,
#171978,#171979,#171980,#171981,#171982,#171983,#171984,#171985,#171986,
#171987,#171988,#171989,#171990,#171991,#171992,#171993,#171994,#171995,
#171996,#171997,#171998,#171999,#172000,#172001,#172002,#172003,#172004,
#172005,#172006,#172007,#172008,#172009,#172010,#172011,#172012,#172013,
#172014,#172015,#172016,#172017,#172018,#172019,#172020,#172021,#172022,
#172023,#172024,#172025,#172026,#172027,#172028,#172029,#172030,#172031,
#172032,#172033,#172034,#172035,#172036,#172037,#172038,#172039,#172040,
#172041,#172042,#172043,#172044,#172045,#172046,#172047,#172048,#172049,
#172050,#172051,#172052,#172053,#172054,#172055,#172056,#172057,#172058,
#172059,#172060,#172061,#172062,#172063,#172064,#172065),.UNSPECIFIED.,
 .F.,.F.)
B_SPLINE_CURVE_WITH_KNOTS((6,1,1,1,1,1,1,1,1,1,1,1,1,1,1,1,1,1,1,1,1,1,
1,1,1,1,1,1,1,1,1,1,1,1,1,1,1,1,1,1,1,1,1,1,1,1,1,1,1,1,1,1,1,1,1,1,1,1,
1,1,1,1,1,1,1,1,1,1,1,1,1,1,1,1,1,1,1,1,1,1,1,1,1,1,1,1,1,1,1,1,1,1,1,1,
1,1,1,1,1,1,1,1,1,1,1,1,1,1,1,1,1,1,1,1,1,1,1,1,1,1,1,1,1,1,1,1,1,1,1,1,
1,1,1,1,1,1,1,1,1,1,1,1,1,1,1,1,1,1,1,1,1,1,1,1,1,1,1,1,1,1,1,1,1,1,1,1,
1,1,1,1,1,1,1,1,1,1,1,1,1,1,1,1,1,1,1,1,1,1,1,6),(0.,0.005,0.01,0.015,0.02,
0.025,0.03,0.035,0.04,0.045,0.05,0.055,0.06,0.065,0.07,0.075,0.08,0.085,
0.09,0.095,0.1,0.105,0.11,0.115,0.12,0.125,0.13,0.135,0.14,0.145,0.15,0.155,
0.16,0.165,0.17,0.175,0.18,0.185,0.19,0.195,0.2,0.205,0.21,0.215,0.22,0.225,
0.23,0.235,0.24,0.245,0.25,0.255,0.26,0.265,0.27,0.275,0.28,0.285,0.29,
0.295,0.3,0.305,0.31,0.315,0.32,0.325,0.33,0.335,0.34,0.345,0.35,0.355,
0.36,0.365,0.37,0.375,0.38,0.385,0.39,0.395,0.4,0.405,0.41,0.415,0.42,0.425,
0.43,0.435,0.44,0.445,0.45,0.455,0.46,0.465,0.47,0.475,0.48,0.485,0.49,
0.495,0.5,0.505,0.51,0.515,0.52,0.525,0.53,0.535,0.54,0.545,0.55,0.555,
0.56,0.565,0.57,0.575,0.58,0.585,0.59,0.595,0.6,0.605,0.61,0.615,0.62,0.625,
0.63,0.635,0.64,0.645,0.65,0.655,0.66,0.665,0.67,0.675,0.68,0.685,0.690000000000001,
0.695000000000001,0.700000000000001,0.705000000000001,0.710000000000001,
0.715000000000001,0.720000000000001,0.725000000000001,0.730000000000001,
0.735000000000001,0.740000000000001,0.745000000000001,0.750000000000001,
0.755000000000001,0.760000000000001,0.765000000000001,0.770000000000001,
0.775000000000001,0.780000000000001,0.785000000000001,0.790000000000001,
0.795000000000001,0.800000000000001,0.805000000000001,0.810000000000001,
0.815000000000001,0.820000000000001,0.825000000000001,0.830000000000001,
0.835000000000001,0.840000000000001,0.845000000000001,0.850000000000001,
0.855000000000001,0.860000000000001,0.865000000000001,0.870000000000001,
0.875000000000001,0.880000000000001,0.885000000000001,0.890000000000001,
0.895000000000001,0.900000000000001,0.905000000000001,0.910000000000001,
0.915000000000001,0.920000000000001,0.925000000000001,0.930000000000001,
0.935000000000001,0.940000000000001,0.94142984443804),.UNSPECIFIED.)
CURVE()
GEOMETRIC_REPRESENTATION_ITEM()
RATIONAL_B_SPLINE_CURVE((1.,1.,1.,1.,1.,1.,1.,1.,1.,1.,1.,1.,1.,1.,1.,1.,
1.,1.,1.,1.,1.,1.,1.,1.,1.,1.,1.,1.,1.,1.,1.,1.,1.,1.,1.,1.,1.,1.,1.,1.,
1.,1.,1.,1.,1.,1.,1.,1.,1.,1.,1.,1.,1.,1.,1.,1.,1.,1.,1.,1.,1.,1.,1.,1.,
1.,1.,1.,1.,1.,1.,1.,1.,1.,1.,1.,1.,1.,1.,1.,1.,1.,1.,1.,1.,1.,1.,1.,1.,
1.,1.,1.,1.,1.,1.,1.,1.,1.,1.,1.,1.,1.,1.,1.,1.,1.,1.,1.,1.,1.,1.,1.,1.,
1.,1.,1.,1.,1.,1.,1.,1.,1.,1.,1.,1.,1.,1.,1.,1.,1.,1.,1.,1.,1.,1.,1.,1.,
1.,1.,1.,1.,1.,1.,1.,1.,1.,1.,1.,1.,1.,1.,1.,1.,1.,1.,1.,1.,1.,1.,1.,1.,
1.,1.,1.,1.,1.,1.,1.,1.,1.,1.,1.,1.,1.,1.,1.,1.,1.,1.,1.,1.,1.,1.,1.,1.,
1.,1.,1.,1.,1.,1.,1.,1.,1.,1.))
REPRESENTATION_ITEM('')
);
#684=(
BOUNDED_CURVE()
B_SPLINE_CURVE(5,(#172068,#172069,#172070,#172071,#172072,#172073,#172074,
#172075,#172076,#172077,#172078,#172079,#172080,#172081,#172082,#172083,
#172084,#172085,#172086,#172087,#172088,#172089,#172090,#172091,#172092,
#172093,#172094,#172095,#172096,#172097,#172098,#172099,#172100,#172101,
#172102,#172103,#172104,#172105,#172106,#172107,#172108,#172109,#172110,
#172111,#172112,#172113,#172114,#172115,#172116,#172117,#172118,#172119,
#172120,#172121,#172122,#172123,#172124,#172125,#172126,#172127,#172128,
#172129,#172130,#172131,#172132,#172133,#172134,#172135,#172136,#172137,
#172138,#172139,#172140,#172141,#172142,#172143,#172144,#172145,#172146,
#172147,#172148,#172149,#172150,#172151,#172152,#172153,#172154,#172155,
#172156,#172157,#172158,#172159,#172160,#172161,#172162,#172163,#172164,
#172165,#172166,#172167,#172168,#172169,#172170,#172171,#172172,#172173,
#172174,#172175,#172176,#172177,#172178,#172179,#172180,#172181,#172182,
#172183,#172184,#172185,#172186,#172187,#172188,#172189,#172190,#172191,
#172192,#172193,#172194,#172195,#172196,#172197,#172198,#172199,#172200,
#172201,#172202,#172203,#172204,#172205,#172206,#172207,#172208,#172209,
#172210,#172211,#172212,#172213,#172214,#172215,#172216,#172217,#172218,
#172219,#172220,#172221,#172222,#172223,#172224,#172225,#172226,#172227,
#172228,#172229,#172230,#172231,#172232,#172233,#172234,#172235,#172236,
#172237,#172238,#172239,#172240,#172241,#172242,#172243,#172244,#172245,
#172246,#172247,#172248,#172249,#172250,#172251,#172252,#172253,#172254,
#172255,#172256,#172257,#172258,#172259,#172260,#172261),.UNSPECIFIED.,
 .F.,.F.)
B_SPLINE_CURVE_WITH_KNOTS((6,1,1,1,1,1,1,1,1,1,1,1,1,1,1,1,1,1,1,1,1,1,
1,1,1,1,1,1,1,1,1,1,1,1,1,1,1,1,1,1,1,1,1,1,1,1,1,1,1,1,1,1,1,1,1,1,1,1,
1,1,1,1,1,1,1,1,1,1,1,1,1,1,1,1,1,1,1,1,1,1,1,1,1,1,1,1,1,1,1,1,1,1,1,1,
1,1,1,1,1,1,1,1,1,1,1,1,1,1,1,1,1,1,1,1,1,1,1,1,1,1,1,1,1,1,1,1,1,1,1,1,
1,1,1,1,1,1,1,1,1,1,1,1,1,1,1,1,1,1,1,1,1,1,1,1,1,1,1,1,1,1,1,1,1,1,1,1,
1,1,1,1,1,1,1,1,1,1,1,1,1,1,1,1,1,1,1,1,1,1,1,6),(-0.94142984443804,-0.940000000000001,
-0.935000000000001,-0.930000000000001,-0.925000000000001,-0.920000000000001,
-0.915000000000001,-0.910000000000001,-0.905000000000001,-0.900000000000001,
-0.895000000000001,-0.890000000000001,-0.885000000000001,-0.880000000000001,
-0.875000000000001,-0.870000000000001,-0.865000000000001,-0.860000000000001,
-0.855000000000001,-0.850000000000001,-0.845000000000001,-0.840000000000001,
-0.835000000000001,-0.830000000000001,-0.825000000000001,-0.820000000000001,
-0.815000000000001,-0.810000000000001,-0.805000000000001,-0.800000000000001,
-0.795000000000001,-0.790000000000001,-0.785000000000001,-0.780000000000001,
-0.775000000000001,-0.770000000000001,-0.765000000000001,-0.760000000000001,
-0.755000000000001,-0.750000000000001,-0.745000000000001,-0.740000000000001,
-0.735000000000001,-0.730000000000001,-0.725000000000001,-0.720000000000001,
-0.715000000000001,-0.710000000000001,-0.705000000000001,-0.700000000000001,
-0.695000000000001,-0.690000000000001,-0.685,-0.68,-0.675,-0.67,-0.665,
-0.66,-0.655,-0.65,-0.645,-0.64,-0.635,-0.63,-0.625,-0.62,-0.615,-0.61,
-0.605,-0.6,-0.595,-0.59,-0.585,-0.58,-0.575,-0.57,-0.565,-0.56,-0.555,
-0.55,-0.545,-0.54,-0.535,-0.53,-0.525,-0.52,-0.515,-0.51,-0.505,-0.5,-0.495,
-0.49,-0.485,-0.48,-0.475,-0.47,-0.465,-0.46,-0.455,-0.45,-0.445,-0.44,
-0.435,-0.43,-0.425,-0.42,-0.415,-0.41,-0.405,-0.4,-0.395,-0.39,-0.385,
-0.38,-0.375,-0.37,-0.365,-0.36,-0.355,-0.35,-0.345,-0.34,-0.335,-0.33,
-0.325,-0.32,-0.315,-0.31,-0.305,-0.3,-0.295,-0.29,-0.285,-0.28,-0.275,
-0.27,-0.265,-0.26,-0.255,-0.25,-0.245,-0.24,-0.235,-0.23,-0.225,-0.22,
-0.215,-0.21,-0.205,-0.2,-0.195,-0.19,-0.185,-0.18,-0.175,-0.17,-0.165,
-0.16,-0.155,-0.15,-0.145,-0.14,-0.135,-0.13,-0.125,-0.12,-0.115,-0.11,
-0.105,-0.1,-0.095,-0.09,-0.085,-0.08,-0.075,-0.07,-0.065,-0.06,-0.055,
-0.05,-0.045,-0.04,-0.035,-0.03,-0.025,-0.02,-0.015,-0.01,-0.005,0.),
 .UNSPECIFIED.)
CURVE()
GEOMETRIC_REPRESENTATION_ITEM()
RATIONAL_B_SPLINE_CURVE((1.,1.,1.,1.,1.,1.,1.,1.,1.,1.,1.,1.,1.,1.,1.,1.,
1.,1.,1.,1.,1.,1.,1.,1.,1.,1.,1.,1.,1.,1.,1.,1.,1.,1.,1.,1.,1.,1.,1.,1.,
1.,1.,1.,1.,1.,1.,1.,1.,1.,1.,1.,1.,1.,1.,1.,1.,1.,1.,1.,1.,1.,1.,1.,1.,
1.,1.,1.,1.,1.,1.,1.,1.,1.,1.,1.,1.,1.,1.,1.,1.,1.,1.,1.,1.,1.,1.,1.,1.,
1.,1.,1.,1.,1.,1.,1.,1.,1.,1.,1.,1.,1.,1.,1.,1.,1.,1.,1.,1.,1.,1.,1.,1.,
1.,1.,1.,1.,1.,1.,1.,1.,1.,1.,1.,1.,1.,1.,1.,1.,1.,1.,1.,1.,1.,1.,1.,1.,
1.,1.,1.,1.,1.,1.,1.,1.,1.,1.,1.,1.,1.,1.,1.,1.,1.,1.,1.,1.,1.,1.,1.,1.,
1.,1.,1.,1.,1.,1.,1.,1.,1.,1.,1.,1.,1.,1.,1.,1.,1.,1.,1.,1.,1.,1.,1.,1.,
1.,1.,1.,1.,1.,1.,1.,1.,1.,1.))
REPRESENTATION_ITEM('')
);
#685=(
BOUNDED_CURVE()
B_SPLINE_CURVE(5,(#172673,#172674,#172675,#172676,#172677,#172678,#172679,
#172680,#172681,#172682,#172683,#172684,#172685,#172686,#172687,#172688,
#172689,#172690,#172691,#172692,#172693,#172694,#172695,#172696,#172697,
#172698,#172699,#172700,#172701,#172702,#172703,#172704,#172705,#172706,
#172707,#172708,#172709,#172710,#172711,#172712,#172713,#172714,#172715,
#172716,#172717,#172718,#172719,#172720,#172721,#172722,#172723,#172724,
#172725,#172726,#172727,#172728,#172729,#172730,#172731,#172732,#172733,
#172734,#172735,#172736,#172737,#172738,#172739,#172740,#172741,#172742,
#172743,#172744,#172745,#172746,#172747,#172748,#172749,#172750,#172751,
#172752,#172753,#172754,#172755,#172756,#172757,#172758,#172759,#172760,
#172761,#172762,#172763,#172764,#172765,#172766,#172767,#172768,#172769,
#172770,#172771,#172772,#172773,#172774,#172775,#172776,#172777,#172778,
#172779,#172780,#172781,#172782,#172783,#172784,#172785,#172786,#172787,
#172788,#172789,#172790,#172791,#172792,#172793,#172794,#172795,#172796,
#172797,#172798,#172799,#172800,#172801,#172802,#172803,#172804,#172805,
#172806,#172807,#172808,#172809,#172810,#172811,#172812,#172813,#172814,
#172815,#172816,#172817,#172818,#172819,#172820,#172821,#172822,#172823,
#172824,#172825,#172826,#172827,#172828,#172829,#172830,#172831,#172832,
#172833,#172834,#172835,#172836,#172837,#172838,#172839,#172840,#172841,
#172842,#172843,#172844,#172845,#172846,#172847,#172848,#172849,#172850,
#172851,#172852,#172853,#172854,#172855,#172856,#172857,#172858,#172859,
#172860,#172861,#172862,#172863,#172864,#172865,#172866),.UNSPECIFIED.,
 .F.,.F.)
B_SPLINE_CURVE_WITH_KNOTS((6,1,1,1,1,1,1,1,1,1,1,1,1,1,1,1,1,1,1,1,1,1,
1,1,1,1,1,1,1,1,1,1,1,1,1,1,1,1,1,1,1,1,1,1,1,1,1,1,1,1,1,1,1,1,1,1,1,1,
1,1,1,1,1,1,1,1,1,1,1,1,1,1,1,1,1,1,1,1,1,1,1,1,1,1,1,1,1,1,1,1,1,1,1,1,
1,1,1,1,1,1,1,1,1,1,1,1,1,1,1,1,1,1,1,1,1,1,1,1,1,1,1,1,1,1,1,1,1,1,1,1,
1,1,1,1,1,1,1,1,1,1,1,1,1,1,1,1,1,1,1,1,1,1,1,1,1,1,1,1,1,1,1,1,1,1,1,1,
1,1,1,1,1,1,1,1,1,1,1,1,1,1,1,1,1,1,1,1,1,1,1,6),(0.,0.005,0.01,0.015,0.02,
0.025,0.03,0.035,0.04,0.045,0.05,0.055,0.06,0.065,0.07,0.075,0.08,0.085,
0.09,0.095,0.1,0.105,0.11,0.115,0.12,0.125,0.13,0.135,0.14,0.145,0.15,0.155,
0.16,0.165,0.17,0.175,0.18,0.185,0.19,0.195,0.2,0.205,0.21,0.215,0.22,0.225,
0.23,0.235,0.24,0.245,0.25,0.255,0.26,0.265,0.27,0.275,0.28,0.285,0.29,
0.295,0.3,0.305,0.31,0.315,0.32,0.325,0.33,0.335,0.34,0.345,0.35,0.355,
0.36,0.365,0.37,0.375,0.38,0.385,0.39,0.395,0.4,0.405,0.41,0.415,0.42,0.425,
0.43,0.435,0.44,0.445,0.45,0.455,0.46,0.465,0.47,0.475,0.48,0.485,0.49,
0.495,0.5,0.505,0.51,0.515,0.52,0.525,0.53,0.535,0.54,0.545,0.55,0.555,
0.56,0.565,0.57,0.575,0.58,0.585,0.59,0.595,0.6,0.605,0.61,0.615,0.62,0.625,
0.63,0.635,0.64,0.645,0.65,0.655,0.66,0.665,0.67,0.675,0.68,0.685,0.690000000000001,
0.695000000000001,0.700000000000001,0.705000000000001,0.710000000000001,
0.715000000000001,0.720000000000001,0.725000000000001,0.730000000000001,
0.735000000000001,0.740000000000001,0.745000000000001,0.750000000000001,
0.755000000000001,0.760000000000001,0.765000000000001,0.770000000000001,
0.775000000000001,0.780000000000001,0.785000000000001,0.790000000000001,
0.795000000000001,0.800000000000001,0.805000000000001,0.810000000000001,
0.815000000000001,0.820000000000001,0.825000000000001,0.830000000000001,
0.835000000000001,0.840000000000001,0.845000000000001,0.850000000000001,
0.855000000000001,0.860000000000001,0.865000000000001,0.870000000000001,
0.875000000000001,0.880000000000001,0.885000000000001,0.890000000000001,
0.895000000000001,0.900000000000001,0.905000000000001,0.910000000000001,
0.915000000000001,0.920000000000001,0.925000000000001,0.930000000000001,
0.935000000000001,0.940000000000001,0.94142984443804),.UNSPECIFIED.)
CURVE()
GEOMETRIC_REPRESENTATION_ITEM()
RATIONAL_B_SPLINE_CURVE((1.,1.,1.,1.,1.,1.,1.,1.,1.,1.,1.,1.,1.,1.,1.,1.,
1.,1.,1.,1.,1.,1.,1.,1.,1.,1.,1.,1.,1.,1.,1.,1.,1.,1.,1.,1.,1.,1.,1.,1.,
1.,1.,1.,1.,1.,1.,1.,1.,1.,1.,1.,1.,1.,1.,1.,1.,1.,1.,1.,1.,1.,1.,1.,1.,
1.,1.,1.,1.,1.,1.,1.,1.,1.,1.,1.,1.,1.,1.,1.,1.,1.,1.,1.,1.,1.,1.,1.,1.,
1.,1.,1.,1.,1.,1.,1.,1.,1.,1.,1.,1.,1.,1.,1.,1.,1.,1.,1.,1.,1.,1.,1.,1.,
1.,1.,1.,1.,1.,1.,1.,1.,1.,1.,1.,1.,1.,1.,1.,1.,1.,1.,1.,1.,1.,1.,1.,1.,
1.,1.,1.,1.,1.,1.,1.,1.,1.,1.,1.,1.,1.,1.,1.,1.,1.,1.,1.,1.,1.,1.,1.,1.,
1.,1.,1.,1.,1.,1.,1.,1.,1.,1.,1.,1.,1.,1.,1.,1.,1.,1.,1.,1.,1.,1.,1.,1.,
1.,1.,1.,1.,1.,1.,1.,1.,1.,1.))
REPRESENTATION_ITEM('')
);
#686=(
BOUNDED_CURVE()
B_SPLINE_CURVE(5,(#172869,#172870,#172871,#172872,#172873,#172874,#172875,
#172876,#172877,#172878,#172879,#172880,#172881,#172882,#172883,#172884,
#172885,#172886,#172887,#172888,#172889,#172890,#172891,#172892,#172893,
#172894,#172895,#172896,#172897,#172898,#172899,#172900,#172901,#172902,
#172903,#172904,#172905,#172906,#172907,#172908,#172909,#172910,#172911,
#172912,#172913,#172914,#172915,#172916,#172917,#172918,#172919,#172920,
#172921,#172922,#172923,#172924,#172925,#172926,#172927,#172928,#172929,
#172930,#172931,#172932,#172933,#172934,#172935,#172936,#172937,#172938,
#172939,#172940,#172941,#172942,#172943,#172944,#172945,#172946,#172947,
#172948,#172949,#172950,#172951,#172952,#172953,#172954,#172955,#172956,
#172957,#172958,#172959,#172960,#172961,#172962,#172963,#172964,#172965,
#172966,#172967,#172968,#172969,#172970,#172971,#172972,#172973,#172974,
#172975,#172976,#172977,#172978,#172979,#172980,#172981,#172982,#172983,
#172984,#172985,#172986,#172987,#172988,#172989,#172990,#172991,#172992,
#172993,#172994,#172995,#172996,#172997,#172998,#172999,#173000,#173001,
#173002,#173003,#173004,#173005,#173006,#173007,#173008,#173009,#173010,
#173011,#173012,#173013,#173014,#173015,#173016,#173017,#173018,#173019,
#173020,#173021,#173022,#173023,#173024,#173025,#173026,#173027,#173028,
#173029,#173030,#173031,#173032,#173033,#173034,#173035,#173036,#173037,
#173038,#173039,#173040,#173041,#173042,#173043,#173044,#173045,#173046,
#173047,#173048,#173049,#173050,#173051,#173052,#173053,#173054,#173055,
#173056,#173057,#173058,#173059,#173060,#173061,#173062),.UNSPECIFIED.,
 .F.,.F.)
B_SPLINE_CURVE_WITH_KNOTS((6,1,1,1,1,1,1,1,1,1,1,1,1,1,1,1,1,1,1,1,1,1,
1,1,1,1,1,1,1,1,1,1,1,1,1,1,1,1,1,1,1,1,1,1,1,1,1,1,1,1,1,1,1,1,1,1,1,1,
1,1,1,1,1,1,1,1,1,1,1,1,1,1,1,1,1,1,1,1,1,1,1,1,1,1,1,1,1,1,1,1,1,1,1,1,
1,1,1,1,1,1,1,1,1,1,1,1,1,1,1,1,1,1,1,1,1,1,1,1,1,1,1,1,1,1,1,1,1,1,1,1,
1,1,1,1,1,1,1,1,1,1,1,1,1,1,1,1,1,1,1,1,1,1,1,1,1,1,1,1,1,1,1,1,1,1,1,1,
1,1,1,1,1,1,1,1,1,1,1,1,1,1,1,1,1,1,1,1,1,1,1,6),(-0.941429844438057,-0.940000000000001,
-0.935000000000001,-0.930000000000001,-0.925000000000001,-0.920000000000001,
-0.915000000000001,-0.910000000000001,-0.905000000000001,-0.900000000000001,
-0.895000000000001,-0.890000000000001,-0.885000000000001,-0.880000000000001,
-0.875000000000001,-0.870000000000001,-0.865000000000001,-0.860000000000001,
-0.855000000000001,-0.850000000000001,-0.845000000000001,-0.840000000000001,
-0.835000000000001,-0.830000000000001,-0.825000000000001,-0.820000000000001,
-0.815000000000001,-0.810000000000001,-0.805000000000001,-0.800000000000001,
-0.795000000000001,-0.790000000000001,-0.785000000000001,-0.780000000000001,
-0.775000000000001,-0.770000000000001,-0.765000000000001,-0.760000000000001,
-0.755000000000001,-0.750000000000001,-0.745000000000001,-0.740000000000001,
-0.735000000000001,-0.730000000000001,-0.725000000000001,-0.720000000000001,
-0.715000000000001,-0.710000000000001,-0.705000000000001,-0.700000000000001,
-0.695000000000001,-0.690000000000001,-0.685,-0.68,-0.675,-0.67,-0.665,
-0.66,-0.655,-0.65,-0.645,-0.64,-0.635,-0.63,-0.625,-0.62,-0.615,-0.61,
-0.605,-0.6,-0.595,-0.59,-0.585,-0.58,-0.575,-0.57,-0.565,-0.56,-0.555,
-0.55,-0.545,-0.54,-0.535,-0.53,-0.525,-0.52,-0.515,-0.51,-0.505,-0.5,-0.495,
-0.49,-0.485,-0.48,-0.475,-0.47,-0.465,-0.46,-0.455,-0.45,-0.445,-0.44,
-0.435,-0.43,-0.425,-0.42,-0.415,-0.41,-0.405,-0.4,-0.395,-0.39,-0.385,
-0.38,-0.375,-0.37,-0.365,-0.36,-0.355,-0.35,-0.345,-0.34,-0.335,-0.33,
-0.325,-0.32,-0.315,-0.31,-0.305,-0.3,-0.295,-0.29,-0.285,-0.28,-0.275,
-0.27,-0.265,-0.26,-0.255,-0.25,-0.245,-0.24,-0.235,-0.23,-0.225,-0.22,
-0.215,-0.21,-0.205,-0.2,-0.195,-0.19,-0.185,-0.18,-0.175,-0.17,-0.165,
-0.16,-0.155,-0.15,-0.145,-0.14,-0.135,-0.13,-0.125,-0.12,-0.115,-0.11,
-0.105,-0.1,-0.095,-0.09,-0.085,-0.08,-0.075,-0.07,-0.065,-0.06,-0.055,
-0.05,-0.045,-0.04,-0.035,-0.03,-0.025,-0.02,-0.015,-0.01,-0.005,0.),
 .UNSPECIFIED.)
CURVE()
GEOMETRIC_REPRESENTATION_ITEM()
RATIONAL_B_SPLINE_CURVE((1.,1.,1.,1.,1.,1.,1.,1.,1.,1.,1.,1.,1.,1.,1.,1.,
1.,1.,1.,1.,1.,1.,1.,1.,1.,1.,1.,1.,1.,1.,1.,1.,1.,1.,1.,1.,1.,1.,1.,1.,
1.,1.,1.,1.,1.,1.,1.,1.,1.,1.,1.,1.,1.,1.,1.,1.,1.,1.,1.,1.,1.,1.,1.,1.,
1.,1.,1.,1.,1.,1.,1.,1.,1.,1.,1.,1.,1.,1.,1.,1.,1.,1.,1.,1.,1.,1.,1.,1.,
1.,1.,1.,1.,1.,1.,1.,1.,1.,1.,1.,1.,1.,1.,1.,1.,1.,1.,1.,1.,1.,1.,1.,1.,
1.,1.,1.,1.,1.,1.,1.,1.,1.,1.,1.,1.,1.,1.,1.,1.,1.,1.,1.,1.,1.,1.,1.,1.,
1.,1.,1.,1.,1.,1.,1.,1.,1.,1.,1.,1.,1.,1.,1.,1.,1.,1.,1.,1.,1.,1.,1.,1.,
1.,1.,1.,1.,1.,1.,1.,1.,1.,1.,1.,1.,1.,1.,1.,1.,1.,1.,1.,1.,1.,1.,1.,1.,
1.,1.,1.,1.,1.,1.,1.,1.,1.,1.))
REPRESENTATION_ITEM('')
);
#687=(
BOUNDED_CURVE()
B_SPLINE_CURVE(5,(#173738,#173739,#173740,#173741,#173742,#173743,#173744,
#173745,#173746,#173747,#173748,#173749,#173750,#173751,#173752,#173753,
#173754,#173755,#173756,#173757,#173758,#173759,#173760,#173761,#173762,
#173763,#173764,#173765,#173766,#173767,#173768,#173769,#173770,#173771,
#173772,#173773,#173774,#173775,#173776,#173777,#173778,#173779,#173780,
#173781,#173782,#173783,#173784,#173785,#173786,#173787,#173788,#173789,
#173790,#173791,#173792,#173793,#173794,#173795,#173796,#173797,#173798,
#173799,#173800,#173801,#173802,#173803,#173804,#173805,#173806,#173807,
#173808,#173809,#173810,#173811,#173812,#173813,#173814,#173815,#173816,
#173817,#173818,#173819,#173820,#173821,#173822,#173823,#173824,#173825,
#173826,#173827,#173828,#173829,#173830,#173831,#173832,#173833,#173834,
#173835,#173836,#173837,#173838,#173839,#173840,#173841,#173842,#173843,
#173844,#173845,#173846,#173847,#173848,#173849,#173850,#173851,#173852,
#173853,#173854,#173855,#173856,#173857,#173858,#173859,#173860,#173861,
#173862,#173863,#173864,#173865,#173866,#173867,#173868,#173869,#173870,
#173871,#173872,#173873,#173874,#173875,#173876,#173877,#173878,#173879,
#173880,#173881,#173882,#173883,#173884,#173885,#173886,#173887,#173888,
#173889,#173890,#173891,#173892,#173893,#173894,#173895,#173896,#173897,
#173898,#173899,#173900,#173901,#173902,#173903,#173904,#173905,#173906,
#173907,#173908,#173909,#173910,#173911,#173912,#173913,#173914,#173915,
#173916,#173917,#173918,#173919,#173920,#173921,#173922,#173923,#173924,
#173925,#173926,#173927,#173928,#173929,#173930,#173931),.UNSPECIFIED.,
 .F.,.F.)
B_SPLINE_CURVE_WITH_KNOTS((6,1,1,1,1,1,1,1,1,1,1,1,1,1,1,1,1,1,1,1,1,1,
1,1,1,1,1,1,1,1,1,1,1,1,1,1,1,1,1,1,1,1,1,1,1,1,1,1,1,1,1,1,1,1,1,1,1,1,
1,1,1,1,1,1,1,1,1,1,1,1,1,1,1,1,1,1,1,1,1,1,1,1,1,1,1,1,1,1,1,1,1,1,1,1,
1,1,1,1,1,1,1,1,1,1,1,1,1,1,1,1,1,1,1,1,1,1,1,1,1,1,1,1,1,1,1,1,1,1,1,1,
1,1,1,1,1,1,1,1,1,1,1,1,1,1,1,1,1,1,1,1,1,1,1,1,1,1,1,1,1,1,1,1,1,1,1,1,
1,1,1,1,1,1,1,1,1,1,1,1,1,1,1,1,1,1,1,1,1,1,1,6),(0.,0.005,0.01,0.015,0.02,
0.025,0.03,0.035,0.04,0.045,0.05,0.055,0.06,0.065,0.07,0.075,0.08,0.085,
0.09,0.095,0.1,0.105,0.11,0.115,0.12,0.125,0.13,0.135,0.14,0.145,0.15,0.155,
0.16,0.165,0.17,0.175,0.18,0.185,0.19,0.195,0.2,0.205,0.21,0.215,0.22,0.225,
0.23,0.235,0.24,0.245,0.25,0.255,0.26,0.265,0.27,0.275,0.28,0.285,0.29,
0.295,0.3,0.305,0.31,0.315,0.32,0.325,0.33,0.335,0.34,0.345,0.35,0.355,
0.36,0.365,0.37,0.375,0.38,0.385,0.39,0.395,0.4,0.405,0.41,0.415,0.42,0.425,
0.43,0.435,0.44,0.445,0.45,0.455,0.46,0.465,0.47,0.475,0.48,0.485,0.49,
0.495,0.5,0.505,0.51,0.515,0.52,0.525,0.53,0.535,0.54,0.545,0.55,0.555,
0.56,0.565,0.57,0.575,0.58,0.585,0.59,0.595,0.6,0.605,0.61,0.615,0.62,0.625,
0.63,0.635,0.64,0.645,0.65,0.655,0.66,0.665,0.67,0.675,0.68,0.685,0.690000000000001,
0.695000000000001,0.700000000000001,0.705000000000001,0.710000000000001,
0.715000000000001,0.720000000000001,0.725000000000001,0.730000000000001,
0.735000000000001,0.740000000000001,0.745000000000001,0.750000000000001,
0.755000000000001,0.760000000000001,0.765000000000001,0.770000000000001,
0.775000000000001,0.780000000000001,0.785000000000001,0.790000000000001,
0.795000000000001,0.800000000000001,0.805000000000001,0.810000000000001,
0.815000000000001,0.820000000000001,0.825000000000001,0.830000000000001,
0.835000000000001,0.840000000000001,0.845000000000001,0.850000000000001,
0.855000000000001,0.860000000000001,0.865000000000001,0.870000000000001,
0.875000000000001,0.880000000000001,0.885000000000001,0.890000000000001,
0.895000000000001,0.900000000000001,0.905000000000001,0.910000000000001,
0.915000000000001,0.920000000000001,0.925000000000001,0.930000000000001,
0.935000000000001,0.940000000000001,0.941429844431361),.UNSPECIFIED.)
CURVE()
GEOMETRIC_REPRESENTATION_ITEM()
RATIONAL_B_SPLINE_CURVE((1.,1.,1.,1.,1.,1.,1.,1.,1.,1.,1.,1.,1.,1.,1.,1.,
1.,1.,1.,1.,1.,1.,1.,1.,1.,1.,1.,1.,1.,1.,1.,1.,1.,1.,1.,1.,1.,1.,1.,1.,
1.,1.,1.,1.,1.,1.,1.,1.,1.,1.,1.,1.,1.,1.,1.,1.,1.,1.,1.,1.,1.,1.,1.,1.,
1.,1.,1.,1.,1.,1.,1.,1.,1.,1.,1.,1.,1.,1.,1.,1.,1.,1.,1.,1.,1.,1.,1.,1.,
1.,1.,1.,1.,1.,1.,1.,1.,1.,1.,1.,1.,1.,1.,1.,1.,1.,1.,1.,1.,1.,1.,1.,1.,
1.,1.,1.,1.,1.,1.,1.,1.,1.,1.,1.,1.,1.,1.,1.,1.,1.,1.,1.,1.,1.,1.,1.,1.,
1.,1.,1.,1.,1.,1.,1.,1.,1.,1.,1.,1.,1.,1.,1.,1.,1.,1.,1.,1.,1.,1.,1.,1.,
1.,1.,1.,1.,1.,1.,1.,1.,1.,1.,1.,1.,1.,1.,1.,1.,1.,1.,1.,1.,1.,1.,1.,1.,
1.,1.,1.,1.,1.,1.,1.,1.,1.,1.))
REPRESENTATION_ITEM('')
);
#688=(
BOUNDED_CURVE()
B_SPLINE_CURVE(5,(#173932,#173933,#173934,#173935,#173936,#173937,#173938,
#173939,#173940,#173941,#173942,#173943,#173944,#173945,#173946,#173947,
#173948,#173949,#173950,#173951,#173952,#173953,#173954,#173955,#173956,
#173957,#173958,#173959,#173960,#173961,#173962,#173963,#173964,#173965,
#173966,#173967,#173968,#173969,#173970,#173971,#173972,#173973,#173974,
#173975,#173976,#173977,#173978,#173979,#173980,#173981,#173982,#173983,
#173984,#173985,#173986,#173987,#173988,#173989,#173990,#173991,#173992,
#173993,#173994,#173995,#173996,#173997,#173998,#173999,#174000,#174001,
#174002,#174003,#174004,#174005,#174006,#174007,#174008,#174009,#174010,
#174011,#174012,#174013,#174014,#174015,#174016,#174017,#174018,#174019,
#174020,#174021,#174022,#174023,#174024,#174025,#174026,#174027,#174028,
#174029,#174030,#174031,#174032,#174033,#174034,#174035,#174036,#174037,
#174038,#174039,#174040,#174041,#174042,#174043,#174044,#174045,#174046,
#174047,#174048,#174049,#174050,#174051,#174052,#174053,#174054,#174055,
#174056,#174057,#174058,#174059,#174060,#174061,#174062,#174063,#174064,
#174065,#174066,#174067,#174068,#174069,#174070,#174071,#174072,#174073,
#174074,#174075,#174076,#174077,#174078,#174079,#174080,#174081,#174082,
#174083,#174084,#174085,#174086,#174087,#174088,#174089,#174090,#174091,
#174092,#174093,#174094,#174095,#174096,#174097,#174098,#174099,#174100,
#174101,#174102,#174103,#174104,#174105,#174106,#174107,#174108,#174109,
#174110,#174111,#174112,#174113,#174114,#174115,#174116,#174117,#174118,
#174119,#174120,#174121,#174122,#174123,#174124,#174125),.UNSPECIFIED.,
 .F.,.F.)
B_SPLINE_CURVE_WITH_KNOTS((6,1,1,1,1,1,1,1,1,1,1,1,1,1,1,1,1,1,1,1,1,1,
1,1,1,1,1,1,1,1,1,1,1,1,1,1,1,1,1,1,1,1,1,1,1,1,1,1,1,1,1,1,1,1,1,1,1,1,
1,1,1,1,1,1,1,1,1,1,1,1,1,1,1,1,1,1,1,1,1,1,1,1,1,1,1,1,1,1,1,1,1,1,1,1,
1,1,1,1,1,1,1,1,1,1,1,1,1,1,1,1,1,1,1,1,1,1,1,1,1,1,1,1,1,1,1,1,1,1,1,1,
1,1,1,1,1,1,1,1,1,1,1,1,1,1,1,1,1,1,1,1,1,1,1,1,1,1,1,1,1,1,1,1,1,1,1,1,
1,1,1,1,1,1,1,1,1,1,1,1,1,1,1,1,1,1,1,1,1,1,1,6),(-0.941429844431347,-0.940000000000001,
-0.935000000000001,-0.930000000000001,-0.925000000000001,-0.920000000000001,
-0.915000000000001,-0.910000000000001,-0.905000000000001,-0.900000000000001,
-0.895000000000001,-0.890000000000001,-0.885000000000001,-0.880000000000001,
-0.875000000000001,-0.870000000000001,-0.865000000000001,-0.860000000000001,
-0.855000000000001,-0.850000000000001,-0.845000000000001,-0.840000000000001,
-0.835000000000001,-0.830000000000001,-0.825000000000001,-0.820000000000001,
-0.815000000000001,-0.810000000000001,-0.805000000000001,-0.800000000000001,
-0.795000000000001,-0.790000000000001,-0.785000000000001,-0.780000000000001,
-0.775000000000001,-0.770000000000001,-0.765000000000001,-0.760000000000001,
-0.755000000000001,-0.750000000000001,-0.745000000000001,-0.740000000000001,
-0.735000000000001,-0.730000000000001,-0.725000000000001,-0.720000000000001,
-0.715000000000001,-0.710000000000001,-0.705000000000001,-0.700000000000001,
-0.695000000000001,-0.690000000000001,-0.685,-0.68,-0.675,-0.67,-0.665,
-0.66,-0.655,-0.65,-0.645,-0.64,-0.635,-0.63,-0.625,-0.62,-0.615,-0.61,
-0.605,-0.6,-0.595,-0.59,-0.585,-0.58,-0.575,-0.57,-0.565,-0.56,-0.555,
-0.55,-0.545,-0.54,-0.535,-0.53,-0.525,-0.52,-0.515,-0.51,-0.505,-0.5,-0.495,
-0.49,-0.485,-0.48,-0.475,-0.47,-0.465,-0.46,-0.455,-0.45,-0.445,-0.44,
-0.435,-0.43,-0.425,-0.42,-0.415,-0.41,-0.405,-0.4,-0.395,-0.39,-0.385,
-0.38,-0.375,-0.37,-0.365,-0.36,-0.355,-0.35,-0.345,-0.34,-0.335,-0.33,
-0.325,-0.32,-0.315,-0.31,-0.305,-0.3,-0.295,-0.29,-0.285,-0.28,-0.275,
-0.27,-0.265,-0.26,-0.255,-0.25,-0.245,-0.24,-0.235,-0.23,-0.225,-0.22,
-0.215,-0.21,-0.205,-0.2,-0.195,-0.19,-0.185,-0.18,-0.175,-0.17,-0.165,
-0.16,-0.155,-0.15,-0.145,-0.14,-0.135,-0.13,-0.125,-0.12,-0.115,-0.11,
-0.105,-0.1,-0.095,-0.09,-0.085,-0.08,-0.075,-0.07,-0.065,-0.06,-0.055,
-0.05,-0.045,-0.04,-0.035,-0.03,-0.025,-0.02,-0.015,-0.01,-0.005,0.),
 .UNSPECIFIED.)
CURVE()
GEOMETRIC_REPRESENTATION_ITEM()
RATIONAL_B_SPLINE_CURVE((1.,1.,1.,1.,1.,1.,1.,1.,1.,1.,1.,1.,1.,1.,1.,1.,
1.,1.,1.,1.,1.,1.,1.,1.,1.,1.,1.,1.,1.,1.,1.,1.,1.,1.,1.,1.,1.,1.,1.,1.,
1.,1.,1.,1.,1.,1.,1.,1.,1.,1.,1.,1.,1.,1.,1.,1.,1.,1.,1.,1.,1.,1.,1.,1.,
1.,1.,1.,1.,1.,1.,1.,1.,1.,1.,1.,1.,1.,1.,1.,1.,1.,1.,1.,1.,1.,1.,1.,1.,
1.,1.,1.,1.,1.,1.,1.,1.,1.,1.,1.,1.,1.,1.,1.,1.,1.,1.,1.,1.,1.,1.,1.,1.,
1.,1.,1.,1.,1.,1.,1.,1.,1.,1.,1.,1.,1.,1.,1.,1.,1.,1.,1.,1.,1.,1.,1.,1.,
1.,1.,1.,1.,1.,1.,1.,1.,1.,1.,1.,1.,1.,1.,1.,1.,1.,1.,1.,1.,1.,1.,1.,1.,
1.,1.,1.,1.,1.,1.,1.,1.,1.,1.,1.,1.,1.,1.,1.,1.,1.,1.,1.,1.,1.,1.,1.,1.,
1.,1.,1.,1.,1.,1.,1.,1.,1.,1.))
REPRESENTATION_ITEM('')
);
#689=(
BOUNDED_CURVE()
B_SPLINE_CURVE(5,(#174585,#174586,#174587,#174588,#174589,#174590,#174591,
#174592,#174593,#174594,#174595,#174596,#174597,#174598,#174599,#174600,
#174601,#174602,#174603,#174604,#174605,#174606,#174607,#174608,#174609,
#174610,#174611,#174612,#174613,#174614,#174615,#174616,#174617,#174618,
#174619,#174620,#174621,#174622,#174623,#174624,#174625,#174626,#174627,
#174628,#174629,#174630,#174631,#174632,#174633,#174634,#174635,#174636,
#174637,#174638,#174639,#174640,#174641,#174642,#174643,#174644,#174645,
#174646,#174647,#174648,#174649,#174650,#174651,#174652,#174653,#174654,
#174655,#174656,#174657,#174658,#174659,#174660,#174661,#174662,#174663,
#174664,#174665,#174666,#174667,#174668,#174669,#174670,#174671,#174672,
#174673,#174674,#174675,#174676,#174677,#174678,#174679,#174680,#174681,
#174682,#174683,#174684,#174685,#174686,#174687,#174688,#174689,#174690,
#174691,#174692,#174693,#174694,#174695,#174696,#174697,#174698,#174699,
#174700,#174701,#174702,#174703,#174704,#174705,#174706,#174707,#174708,
#174709,#174710,#174711,#174712,#174713,#174714,#174715,#174716,#174717,
#174718,#174719,#174720,#174721,#174722,#174723,#174724,#174725,#174726,
#174727,#174728,#174729,#174730,#174731,#174732,#174733,#174734,#174735,
#174736,#174737,#174738,#174739,#174740,#174741,#174742,#174743,#174744,
#174745,#174746,#174747,#174748,#174749,#174750,#174751,#174752,#174753,
#174754,#174755,#174756,#174757,#174758,#174759,#174760,#174761,#174762,
#174763,#174764,#174765,#174766,#174767,#174768,#174769,#174770,#174771,
#174772,#174773,#174774,#174775,#174776,#174777,#174778),.UNSPECIFIED.,
 .F.,.F.)
B_SPLINE_CURVE_WITH_KNOTS((6,1,1,1,1,1,1,1,1,1,1,1,1,1,1,1,1,1,1,1,1,1,
1,1,1,1,1,1,1,1,1,1,1,1,1,1,1,1,1,1,1,1,1,1,1,1,1,1,1,1,1,1,1,1,1,1,1,1,
1,1,1,1,1,1,1,1,1,1,1,1,1,1,1,1,1,1,1,1,1,1,1,1,1,1,1,1,1,1,1,1,1,1,1,1,
1,1,1,1,1,1,1,1,1,1,1,1,1,1,1,1,1,1,1,1,1,1,1,1,1,1,1,1,1,1,1,1,1,1,1,1,
1,1,1,1,1,1,1,1,1,1,1,1,1,1,1,1,1,1,1,1,1,1,1,1,1,1,1,1,1,1,1,1,1,1,1,1,
1,1,1,1,1,1,1,1,1,1,1,1,1,1,1,1,1,1,1,1,1,1,1,6),(0.,0.005,0.01,0.015,0.02,
0.025,0.03,0.035,0.04,0.045,0.05,0.055,0.06,0.065,0.07,0.075,0.08,0.085,
0.09,0.095,0.1,0.105,0.11,0.115,0.12,0.125,0.13,0.135,0.14,0.145,0.15,0.155,
0.16,0.165,0.17,0.175,0.18,0.185,0.19,0.195,0.2,0.205,0.21,0.215,0.22,0.225,
0.23,0.235,0.24,0.245,0.25,0.255,0.26,0.265,0.27,0.275,0.28,0.285,0.29,
0.295,0.3,0.305,0.31,0.315,0.32,0.325,0.33,0.335,0.34,0.345,0.35,0.355,
0.36,0.365,0.37,0.375,0.38,0.385,0.39,0.395,0.4,0.405,0.41,0.415,0.42,0.425,
0.43,0.435,0.44,0.445,0.45,0.455,0.46,0.465,0.47,0.475,0.48,0.485,0.49,
0.495,0.5,0.505,0.51,0.515,0.52,0.525,0.53,0.535,0.54,0.545,0.55,0.555,
0.56,0.565,0.57,0.575,0.58,0.585,0.59,0.595,0.6,0.605,0.61,0.615,0.62,0.625,
0.63,0.635,0.64,0.645,0.65,0.655,0.66,0.665,0.67,0.675,0.68,0.685,0.690000000000001,
0.695000000000001,0.700000000000001,0.705000000000001,0.710000000000001,
0.715000000000001,0.720000000000001,0.725000000000001,0.730000000000001,
0.735000000000001,0.740000000000001,0.745000000000001,0.750000000000001,
0.755000000000001,0.760000000000001,0.765000000000001,0.770000000000001,
0.775000000000001,0.780000000000001,0.785000000000001,0.790000000000001,
0.795000000000001,0.800000000000001,0.805000000000001,0.810000000000001,
0.815000000000001,0.820000000000001,0.825000000000001,0.830000000000001,
0.835000000000001,0.840000000000001,0.845000000000001,0.850000000000001,
0.855000000000001,0.860000000000001,0.865000000000001,0.870000000000001,
0.875000000000001,0.880000000000001,0.885000000000001,0.890000000000001,
0.895000000000001,0.900000000000001,0.905000000000001,0.910000000000001,
0.915000000000001,0.920000000000001,0.925000000000001,0.930000000000001,
0.935000000000001,0.940000000000001,0.941429844438059),.UNSPECIFIED.)
CURVE()
GEOMETRIC_REPRESENTATION_ITEM()
RATIONAL_B_SPLINE_CURVE((1.,1.,1.,1.,1.,1.,1.,1.,1.,1.,1.,1.,1.,1.,1.,1.,
1.,1.,1.,1.,1.,1.,1.,1.,1.,1.,1.,1.,1.,1.,1.,1.,1.,1.,1.,1.,1.,1.,1.,1.,
1.,1.,1.,1.,1.,1.,1.,1.,1.,1.,1.,1.,1.,1.,1.,1.,1.,1.,1.,1.,1.,1.,1.,1.,
1.,1.,1.,1.,1.,1.,1.,1.,1.,1.,1.,1.,1.,1.,1.,1.,1.,1.,1.,1.,1.,1.,1.,1.,
1.,1.,1.,1.,1.,1.,1.,1.,1.,1.,1.,1.,1.,1.,1.,1.,1.,1.,1.,1.,1.,1.,1.,1.,
1.,1.,1.,1.,1.,1.,1.,1.,1.,1.,1.,1.,1.,1.,1.,1.,1.,1.,1.,1.,1.,1.,1.,1.,
1.,1.,1.,1.,1.,1.,1.,1.,1.,1.,1.,1.,1.,1.,1.,1.,1.,1.,1.,1.,1.,1.,1.,1.,
1.,1.,1.,1.,1.,1.,1.,1.,1.,1.,1.,1.,1.,1.,1.,1.,1.,1.,1.,1.,1.,1.,1.,1.,
1.,1.,1.,1.,1.,1.,1.,1.,1.,1.))
REPRESENTATION_ITEM('')
);
#690=(
BOUNDED_CURVE()
B_SPLINE_CURVE(5,(#174779,#174780,#174781,#174782,#174783,#174784,#174785,
#174786,#174787,#174788,#174789,#174790,#174791,#174792,#174793,#174794,
#174795,#174796,#174797,#174798,#174799,#174800,#174801,#174802,#174803,
#174804,#174805,#174806,#174807,#174808,#174809,#174810,#174811,#174812,
#174813,#174814,#174815,#174816,#174817,#174818,#174819,#174820,#174821,
#174822,#174823,#174824,#174825,#174826,#174827,#174828,#174829,#174830,
#174831,#174832,#174833,#174834,#174835,#174836,#174837,#174838,#174839,
#174840,#174841,#174842,#174843,#174844,#174845,#174846,#174847,#174848,
#174849,#174850,#174851,#174852,#174853,#174854,#174855,#174856,#174857,
#174858,#174859,#174860,#174861,#174862,#174863,#174864,#174865,#174866,
#174867,#174868,#174869,#174870,#174871,#174872,#174873,#174874,#174875,
#174876,#174877,#174878,#174879,#174880,#174881,#174882,#174883,#174884,
#174885,#174886,#174887,#174888,#174889,#174890,#174891,#174892,#174893,
#174894,#174895,#174896,#174897,#174898,#174899,#174900,#174901,#174902,
#174903,#174904,#174905,#174906,#174907,#174908,#174909,#174910,#174911,
#174912,#174913,#174914,#174915,#174916,#174917,#174918,#174919,#174920,
#174921,#174922,#174923,#174924,#174925,#174926,#174927,#174928,#174929,
#174930,#174931,#174932,#174933,#174934,#174935,#174936,#174937,#174938,
#174939,#174940,#174941,#174942,#174943,#174944,#174945,#174946,#174947,
#174948,#174949,#174950,#174951,#174952,#174953,#174954,#174955,#174956,
#174957,#174958,#174959,#174960,#174961,#174962,#174963,#174964,#174965,
#174966,#174967,#174968,#174969,#174970,#174971,#174972),.UNSPECIFIED.,
 .F.,.F.)
B_SPLINE_CURVE_WITH_KNOTS((6,1,1,1,1,1,1,1,1,1,1,1,1,1,1,1,1,1,1,1,1,1,
1,1,1,1,1,1,1,1,1,1,1,1,1,1,1,1,1,1,1,1,1,1,1,1,1,1,1,1,1,1,1,1,1,1,1,1,
1,1,1,1,1,1,1,1,1,1,1,1,1,1,1,1,1,1,1,1,1,1,1,1,1,1,1,1,1,1,1,1,1,1,1,1,
1,1,1,1,1,1,1,1,1,1,1,1,1,1,1,1,1,1,1,1,1,1,1,1,1,1,1,1,1,1,1,1,1,1,1,1,
1,1,1,1,1,1,1,1,1,1,1,1,1,1,1,1,1,1,1,1,1,1,1,1,1,1,1,1,1,1,1,1,1,1,1,1,
1,1,1,1,1,1,1,1,1,1,1,1,1,1,1,1,1,1,1,1,1,1,1,6),(-0.941429844438049,-0.940000000000001,
-0.935000000000001,-0.930000000000001,-0.925000000000001,-0.920000000000001,
-0.915000000000001,-0.910000000000001,-0.905000000000001,-0.900000000000001,
-0.895000000000001,-0.890000000000001,-0.885000000000001,-0.880000000000001,
-0.875000000000001,-0.870000000000001,-0.865000000000001,-0.860000000000001,
-0.855000000000001,-0.850000000000001,-0.845000000000001,-0.840000000000001,
-0.835000000000001,-0.830000000000001,-0.825000000000001,-0.820000000000001,
-0.815000000000001,-0.810000000000001,-0.805000000000001,-0.800000000000001,
-0.795000000000001,-0.790000000000001,-0.785000000000001,-0.780000000000001,
-0.775000000000001,-0.770000000000001,-0.765000000000001,-0.760000000000001,
-0.755000000000001,-0.750000000000001,-0.745000000000001,-0.740000000000001,
-0.735000000000001,-0.730000000000001,-0.725000000000001,-0.720000000000001,
-0.715000000000001,-0.710000000000001,-0.705000000000001,-0.700000000000001,
-0.695000000000001,-0.690000000000001,-0.685,-0.68,-0.675,-0.67,-0.665,
-0.66,-0.655,-0.65,-0.645,-0.64,-0.635,-0.63,-0.625,-0.62,-0.615,-0.61,
-0.605,-0.6,-0.595,-0.59,-0.585,-0.58,-0.575,-0.57,-0.565,-0.56,-0.555,
-0.55,-0.545,-0.54,-0.535,-0.53,-0.525,-0.52,-0.515,-0.51,-0.505,-0.5,-0.495,
-0.49,-0.485,-0.48,-0.475,-0.47,-0.465,-0.46,-0.455,-0.45,-0.445,-0.44,
-0.435,-0.43,-0.425,-0.42,-0.415,-0.41,-0.405,-0.4,-0.395,-0.39,-0.385,
-0.38,-0.375,-0.37,-0.365,-0.36,-0.355,-0.35,-0.345,-0.34,-0.335,-0.33,
-0.325,-0.32,-0.315,-0.31,-0.305,-0.3,-0.295,-0.29,-0.285,-0.28,-0.275,
-0.27,-0.265,-0.26,-0.255,-0.25,-0.245,-0.24,-0.235,-0.23,-0.225,-0.22,
-0.215,-0.21,-0.205,-0.2,-0.195,-0.19,-0.185,-0.18,-0.175,-0.17,-0.165,
-0.16,-0.155,-0.15,-0.145,-0.14,-0.135,-0.13,-0.125,-0.12,-0.115,-0.11,
-0.105,-0.1,-0.095,-0.09,-0.085,-0.08,-0.075,-0.07,-0.065,-0.06,-0.055,
-0.05,-0.045,-0.04,-0.035,-0.03,-0.025,-0.02,-0.015,-0.01,-0.005,0.),
 .UNSPECIFIED.)
CURVE()
GEOMETRIC_REPRESENTATION_ITEM()
RATIONAL_B_SPLINE_CURVE((1.,1.,1.,1.,1.,1.,1.,1.,1.,1.,1.,1.,1.,1.,1.,1.,
1.,1.,1.,1.,1.,1.,1.,1.,1.,1.,1.,1.,1.,1.,1.,1.,1.,1.,1.,1.,1.,1.,1.,1.,
1.,1.,1.,1.,1.,1.,1.,1.,1.,1.,1.,1.,1.,1.,1.,1.,1.,1.,1.,1.,1.,1.,1.,1.,
1.,1.,1.,1.,1.,1.,1.,1.,1.,1.,1.,1.,1.,1.,1.,1.,1.,1.,1.,1.,1.,1.,1.,1.,
1.,1.,1.,1.,1.,1.,1.,1.,1.,1.,1.,1.,1.,1.,1.,1.,1.,1.,1.,1.,1.,1.,1.,1.,
1.,1.,1.,1.,1.,1.,1.,1.,1.,1.,1.,1.,1.,1.,1.,1.,1.,1.,1.,1.,1.,1.,1.,1.,
1.,1.,1.,1.,1.,1.,1.,1.,1.,1.,1.,1.,1.,1.,1.,1.,1.,1.,1.,1.,1.,1.,1.,1.,
1.,1.,1.,1.,1.,1.,1.,1.,1.,1.,1.,1.,1.,1.,1.,1.,1.,1.,1.,1.,1.,1.,1.,1.,
1.,1.,1.,1.,1.,1.,1.,1.,1.,1.))
REPRESENTATION_ITEM('')
);
#883=(
BOUNDED_SURFACE()
B_SPLINE_SURFACE(5,1,((#52622,#52623),(#52624,#52625),(#52626,#52627),(#52628,
#52629),(#52630,#52631),(#52632,#52633),(#52634,#52635),(#52636,#52637),
(#52638,#52639),(#52640,#52641),(#52642,#52643),(#52644,#52645),(#52646,
#52647),(#52648,#52649),(#52650,#52651),(#52652,#52653),(#52654,#52655),
(#52656,#52657),(#52658,#52659),(#52660,#52661),(#52662,#52663),(#52664,
#52665),(#52666,#52667),(#52668,#52669),(#52670,#52671),(#52672,#52673),
(#52674,#52675),(#52676,#52677),(#52678,#52679),(#52680,#52681),(#52682,
#52683),(#52684,#52685),(#52686,#52687),(#52688,#52689),(#52690,#52691),
(#52692,#52693),(#52694,#52695),(#52696,#52697),(#52698,#52699),(#52700,
#52701),(#52702,#52703),(#52704,#52705),(#52706,#52707),(#52708,#52709),
(#52710,#52711),(#52712,#52713),(#52714,#52715),(#52716,#52717),(#52718,
#52719),(#52720,#52721),(#52722,#52723),(#52724,#52725),(#52726,#52727),
(#52728,#52729),(#52730,#52731),(#52732,#52733),(#52734,#52735),(#52736,
#52737),(#52738,#52739),(#52740,#52741),(#52742,#52743),(#52744,#52745),
(#52746,#52747),(#52748,#52749),(#52750,#52751),(#52752,#52753),(#52754,
#52755),(#52756,#52757),(#52758,#52759),(#52760,#52761),(#52762,#52763),
(#52764,#52765),(#52766,#52767),(#52768,#52769),(#52770,#52771),(#52772,
#52773),(#52774,#52775),(#52776,#52777),(#52778,#52779),(#52780,#52781),
(#52782,#52783),(#52784,#52785),(#52786,#52787),(#52788,#52789),(#52790,
#52791),(#52792,#52793),(#52794,#52795),(#52796,#52797),(#52798,#52799),
(#52800,#52801),(#52802,#52803),(#52804,#52805),(#52806,#52807),(#52808,
#52809),(#52810,#52811),(#52812,#52813),(#52814,#52815),(#52816,#52817),
(#52818,#52819),(#52820,#52821),(#52822,#52823),(#52824,#52825),(#52826,
#52827),(#52828,#52829),(#52830,#52831),(#52832,#52833),(#52834,#52835),
(#52836,#52837),(#52838,#52839),(#52840,#52841),(#52842,#52843),(#52844,
#52845),(#52846,#52847),(#52848,#52849),(#52850,#52851),(#52852,#52853),
(#52854,#52855),(#52856,#52857),(#52858,#52859),(#52860,#52861),(#52862,
#52863),(#52864,#52865),(#52866,#52867),(#52868,#52869),(#52870,#52871),
(#52872,#52873),(#52874,#52875),(#52876,#52877),(#52878,#52879),(#52880,
#52881),(#52882,#52883),(#52884,#52885),(#52886,#52887),(#52888,#52889),
(#52890,#52891),(#52892,#52893),(#52894,#52895),(#52896,#52897),(#52898,
#52899),(#52900,#52901),(#52902,#52903),(#52904,#52905),(#52906,#52907),
(#52908,#52909),(#52910,#52911),(#52912,#52913),(#52914,#52915),(#52916,
#52917),(#52918,#52919),(#52920,#52921),(#52922,#52923),(#52924,#52925),
(#52926,#52927),(#52928,#52929),(#52930,#52931),(#52932,#52933),(#52934,
#52935),(#52936,#52937),(#52938,#52939),(#52940,#52941),(#52942,#52943),
(#52944,#52945),(#52946,#52947),(#52948,#52949),(#52950,#52951),(#52952,
#52953),(#52954,#52955),(#52956,#52957),(#52958,#52959),(#52960,#52961),
(#52962,#52963),(#52964,#52965),(#52966,#52967),(#52968,#52969),(#52970,
#52971),(#52972,#52973),(#52974,#52975),(#52976,#52977),(#52978,#52979),
(#52980,#52981),(#52982,#52983),(#52984,#52985),(#52986,#52987),(#52988,
#52989),(#52990,#52991),(#52992,#52993),(#52994,#52995),(#52996,#52997),
(#52998,#52999),(#53000,#53001),(#53002,#53003),(#53004,#53005),(#53006,
#53007),(#53008,#53009),(#53010,#53011),(#53012,#53013),(#53014,#53015),
(#53016,#53017),(#53018,#53019),(#53020,#53021),(#53022,#53023),(#53024,
#53025),(#53026,#53027),(#53028,#53029),(#53030,#53031)),.UNSPECIFIED.,
 .F.,.F.,.F.)
B_SPLINE_SURFACE_WITH_KNOTS((6,1,1,1,1,1,1,1,1,1,1,1,1,1,1,1,1,1,1,1,1,
1,1,1,1,1,1,1,1,1,1,1,1,1,1,1,1,1,1,1,1,1,1,1,1,1,1,1,1,1,1,1,1,1,1,1,1,
1,1,1,1,1,1,1,1,1,1,1,1,1,1,1,1,1,1,1,1,1,1,1,1,1,1,1,1,1,1,1,1,1,1,1,1,
1,1,1,1,1,1,1,1,1,1,1,1,1,1,1,1,1,1,1,1,1,1,1,1,1,1,1,1,1,1,1,1,1,1,1,1,
1,1,1,1,1,1,1,1,1,1,1,1,1,1,1,1,1,1,1,1,1,1,1,1,1,1,1,1,1,1,1,1,1,1,1,1,
1,1,1,1,1,1,1,1,1,1,1,1,1,1,1,1,1,1,1,1,1,1,1,1,1,1,1,1,1,1,1,1,1,1,1,6),
(2,2),(0.,0.005,0.01,0.015,0.02,0.025,0.03,0.035,0.04,0.045,0.05,0.055,
0.06,0.065,0.07,0.075,0.08,0.085,0.09,0.095,0.1,0.105,0.11,0.115,0.12,0.125,
0.13,0.135,0.14,0.145,0.15,0.155,0.16,0.165,0.17,0.175,0.18,0.185,0.19,
0.195,0.2,0.205,0.21,0.215,0.22,0.225,0.23,0.235,0.24,0.245,0.25,0.255,
0.26,0.265,0.27,0.275,0.28,0.285,0.29,0.295,0.3,0.305,0.31,0.315,0.32,0.325,
0.33,0.335,0.34,0.345,0.35,0.355,0.36,0.365,0.37,0.375,0.38,0.385,0.39,
0.395,0.4,0.405,0.41,0.415,0.42,0.425,0.43,0.435,0.44,0.445,0.45,0.455,
0.46,0.465,0.47,0.475,0.48,0.485,0.49,0.495,0.5,0.505,0.51,0.515,0.52,0.525,
0.53,0.535,0.54,0.545,0.55,0.555,0.56,0.565,0.57,0.575,0.58,0.585,0.59,
0.595,0.6,0.605,0.61,0.615,0.62,0.625,0.63,0.635,0.64,0.645,0.65,0.655,
0.66,0.665,0.67,0.675,0.68,0.685,0.690000000000001,0.695000000000001,0.700000000000001,
0.705000000000001,0.710000000000001,0.715000000000001,0.720000000000001,
0.725000000000001,0.730000000000001,0.735000000000001,0.740000000000001,
0.745000000000001,0.750000000000001,0.755000000000001,0.760000000000001,
0.765000000000001,0.770000000000001,0.775000000000001,0.780000000000001,
0.785000000000001,0.790000000000001,0.795000000000001,0.800000000000001,
0.805000000000001,0.810000000000001,0.815000000000001,0.820000000000001,
0.825000000000001,0.830000000000001,0.835000000000001,0.840000000000001,
0.845000000000001,0.850000000000001,0.855000000000001,0.860000000000001,
0.865000000000001,0.870000000000001,0.875000000000001,0.880000000000001,
0.885000000000001,0.890000000000001,0.895000000000001,0.900000000000001,
0.905000000000001,0.910000000000001,0.915000000000001,0.920000000000001,
0.925000000000001,0.930000000000001,0.935000000000001,0.940000000000001,
0.945000000000001,0.950000000000001,0.955000000000001,0.960000000000001,
0.965000000000001,0.970000000000001,0.975000000000001,0.980000000000001,
0.985000000000001,0.990000000000001,0.995000000000001,1.),(0.,1.2),
 .UNSPECIFIED.)
GEOMETRIC_REPRESENTATION_ITEM()
RATIONAL_B_SPLINE_SURFACE(((1.,1.),(1.,1.),(1.,1.),(1.,1.),(1.,1.),(1.,
1.),(1.,1.),(1.,1.),(1.,1.),(1.,1.),(1.,1.),(1.,1.),(1.,1.),(1.,1.),(1.,
1.),(1.,1.),(1.,1.),(1.,1.),(1.,1.),(1.,1.),(1.,1.),(1.,1.),(1.,1.),(1.,
1.),(1.,1.),(1.,1.),(1.,1.),(1.,1.),(1.,1.),(1.,1.),(1.,1.),(1.,1.),(1.,
1.),(1.,1.),(1.,1.),(1.,1.),(1.,1.),(1.,1.),(1.,1.),(1.,1.),(1.,1.),(1.,
1.),(1.,1.),(1.,1.),(1.,1.),(1.,1.),(1.,1.),(1.,1.),(1.,1.),(1.,1.),(1.,
1.),(1.,1.),(1.,1.),(1.,1.),(1.,1.),(1.,1.),(1.,1.),(1.,1.),(1.,1.),(1.,
1.),(1.,1.),(1.,1.),(1.,1.),(1.,1.),(1.,1.),(1.,1.),(1.,1.),(1.,1.),(1.,
1.),(1.,1.),(1.,1.),(1.,1.),(1.,1.),(1.,1.),(1.,1.),(1.,1.),(1.,1.),(1.,
1.),(1.,1.),(1.,1.),(1.,1.),(1.,1.),(1.,1.),(1.,1.),(1.,1.),(1.,1.),(1.,
1.),(1.,1.),(1.,1.),(1.,1.),(1.,1.),(1.,1.),(1.,1.),(1.,1.),(1.,1.),(1.,
1.),(1.,1.),(1.,1.),(1.,1.),(1.,1.),(1.,1.),(1.,1.),(1.,1.),(1.,1.),(1.,
1.),(1.,1.),(1.,1.),(1.,1.),(1.,1.),(1.,1.),(1.,1.),(1.,1.),(1.,1.),(1.,
1.),(1.,1.),(1.,1.),(1.,1.),(1.,1.),(1.,1.),(1.,1.),(1.,1.),(1.,1.),(1.,
1.),(1.,1.),(1.,1.),(1.,1.),(1.,1.),(1.,1.),(1.,1.),(1.,1.),(1.,1.),(1.,
1.),(1.,1.),(1.,1.),(1.,1.),(1.,1.),(1.,1.),(1.,1.),(1.,1.),(1.,1.),(1.,
1.),(1.,1.),(1.,1.),(1.,1.),(1.,1.),(1.,1.),(1.,1.),(1.,1.),(1.,1.),(1.,
1.),(1.,1.),(1.,1.),(1.,1.),(1.,1.),(1.,1.),(1.,1.),(1.,1.),(1.,1.),(1.,
1.),(1.,1.),(1.,1.),(1.,1.),(1.,1.),(1.,1.),(1.,1.),(1.,1.),(1.,1.),(1.,
1.),(1.,1.),(1.,1.),(1.,1.),(1.,1.),(1.,1.),(1.,1.),(1.,1.),(1.,1.),(1.,
1.),(1.,1.),(1.,1.),(1.,1.),(1.,1.),(1.,1.),(1.,1.),(1.,1.),(1.,1.),(1.,
1.),(1.,1.),(1.,1.),(1.,1.),(1.,1.),(1.,1.),(1.,1.),(1.,1.),(1.,1.),(1.,
1.),(1.,1.),(1.,1.),(1.,1.),(1.,1.),(1.,1.),(1.,1.),(1.,1.),(1.,1.),(1.,
1.),(1.,1.)))
REPRESENTATION_ITEM('')
SURFACE()
);
#884=(
BOUNDED_SURFACE()
B_SPLINE_SURFACE(5,1,((#53518,#53519),(#53520,#53521),(#53522,#53523),(#53524,
#53525),(#53526,#53527),(#53528,#53529),(#53530,#53531),(#53532,#53533),
(#53534,#53535),(#53536,#53537),(#53538,#53539),(#53540,#53541),(#53542,
#53543),(#53544,#53545),(#53546,#53547),(#53548,#53549),(#53550,#53551),
(#53552,#53553),(#53554,#53555),(#53556,#53557),(#53558,#53559),(#53560,
#53561),(#53562,#53563),(#53564,#53565),(#53566,#53567),(#53568,#53569),
(#53570,#53571),(#53572,#53573),(#53574,#53575),(#53576,#53577),(#53578,
#53579),(#53580,#53581),(#53582,#53583),(#53584,#53585),(#53586,#53587),
(#53588,#53589),(#53590,#53591),(#53592,#53593),(#53594,#53595),(#53596,
#53597),(#53598,#53599),(#53600,#53601),(#53602,#53603),(#53604,#53605),
(#53606,#53607),(#53608,#53609),(#53610,#53611),(#53612,#53613),(#53614,
#53615),(#53616,#53617),(#53618,#53619),(#53620,#53621),(#53622,#53623),
(#53624,#53625),(#53626,#53627),(#53628,#53629),(#53630,#53631),(#53632,
#53633),(#53634,#53635),(#53636,#53637),(#53638,#53639),(#53640,#53641),
(#53642,#53643),(#53644,#53645),(#53646,#53647),(#53648,#53649),(#53650,
#53651),(#53652,#53653),(#53654,#53655),(#53656,#53657),(#53658,#53659),
(#53660,#53661),(#53662,#53663),(#53664,#53665),(#53666,#53667),(#53668,
#53669),(#53670,#53671),(#53672,#53673),(#53674,#53675),(#53676,#53677),
(#53678,#53679),(#53680,#53681),(#53682,#53683),(#53684,#53685),(#53686,
#53687),(#53688,#53689),(#53690,#53691),(#53692,#53693),(#53694,#53695),
(#53696,#53697),(#53698,#53699),(#53700,#53701),(#53702,#53703),(#53704,
#53705),(#53706,#53707),(#53708,#53709),(#53710,#53711),(#53712,#53713),
(#53714,#53715),(#53716,#53717),(#53718,#53719),(#53720,#53721),(#53722,
#53723),(#53724,#53725),(#53726,#53727),(#53728,#53729),(#53730,#53731),
(#53732,#53733),(#53734,#53735),(#53736,#53737),(#53738,#53739),(#53740,
#53741),(#53742,#53743),(#53744,#53745),(#53746,#53747),(#53748,#53749),
(#53750,#53751),(#53752,#53753),(#53754,#53755),(#53756,#53757),(#53758,
#53759),(#53760,#53761),(#53762,#53763),(#53764,#53765),(#53766,#53767),
(#53768,#53769),(#53770,#53771),(#53772,#53773),(#53774,#53775),(#53776,
#53777),(#53778,#53779),(#53780,#53781),(#53782,#53783),(#53784,#53785),
(#53786,#53787),(#53788,#53789),(#53790,#53791),(#53792,#53793),(#53794,
#53795),(#53796,#53797),(#53798,#53799),(#53800,#53801),(#53802,#53803),
(#53804,#53805),(#53806,#53807),(#53808,#53809),(#53810,#53811),(#53812,
#53813),(#53814,#53815),(#53816,#53817),(#53818,#53819),(#53820,#53821),
(#53822,#53823),(#53824,#53825),(#53826,#53827),(#53828,#53829),(#53830,
#53831),(#53832,#53833),(#53834,#53835),(#53836,#53837),(#53838,#53839),
(#53840,#53841),(#53842,#53843),(#53844,#53845),(#53846,#53847),(#53848,
#53849),(#53850,#53851),(#53852,#53853),(#53854,#53855),(#53856,#53857),
(#53858,#53859),(#53860,#53861),(#53862,#53863),(#53864,#53865),(#53866,
#53867),(#53868,#53869),(#53870,#53871),(#53872,#53873),(#53874,#53875),
(#53876,#53877),(#53878,#53879),(#53880,#53881),(#53882,#53883),(#53884,
#53885),(#53886,#53887),(#53888,#53889),(#53890,#53891),(#53892,#53893),
(#53894,#53895),(#53896,#53897),(#53898,#53899),(#53900,#53901),(#53902,
#53903),(#53904,#53905),(#53906,#53907),(#53908,#53909),(#53910,#53911),
(#53912,#53913),(#53914,#53915),(#53916,#53917),(#53918,#53919),(#53920,
#53921),(#53922,#53923),(#53924,#53925),(#53926,#53927)),.UNSPECIFIED.,
 .F.,.F.,.F.)
B_SPLINE_SURFACE_WITH_KNOTS((6,1,1,1,1,1,1,1,1,1,1,1,1,1,1,1,1,1,1,1,1,
1,1,1,1,1,1,1,1,1,1,1,1,1,1,1,1,1,1,1,1,1,1,1,1,1,1,1,1,1,1,1,1,1,1,1,1,
1,1,1,1,1,1,1,1,1,1,1,1,1,1,1,1,1,1,1,1,1,1,1,1,1,1,1,1,1,1,1,1,1,1,1,1,
1,1,1,1,1,1,1,1,1,1,1,1,1,1,1,1,1,1,1,1,1,1,1,1,1,1,1,1,1,1,1,1,1,1,1,1,
1,1,1,1,1,1,1,1,1,1,1,1,1,1,1,1,1,1,1,1,1,1,1,1,1,1,1,1,1,1,1,1,1,1,1,1,
1,1,1,1,1,1,1,1,1,1,1,1,1,1,1,1,1,1,1,1,1,1,1,1,1,1,1,1,1,1,1,1,1,1,1,6),
(2,2),(0.,0.005,0.01,0.015,0.02,0.025,0.03,0.035,0.04,0.045,0.05,0.055,
0.06,0.065,0.07,0.075,0.08,0.085,0.09,0.095,0.1,0.105,0.11,0.115,0.12,0.125,
0.13,0.135,0.14,0.145,0.15,0.155,0.16,0.165,0.17,0.175,0.18,0.185,0.19,
0.195,0.2,0.205,0.21,0.215,0.22,0.225,0.23,0.235,0.24,0.245,0.25,0.255,
0.26,0.265,0.27,0.275,0.28,0.285,0.29,0.295,0.3,0.305,0.31,0.315,0.32,0.325,
0.33,0.335,0.34,0.345,0.35,0.355,0.36,0.365,0.37,0.375,0.38,0.385,0.39,
0.395,0.4,0.405,0.41,0.415,0.42,0.425,0.43,0.435,0.44,0.445,0.45,0.455,
0.46,0.465,0.47,0.475,0.48,0.485,0.49,0.495,0.5,0.505,0.51,0.515,0.52,0.525,
0.53,0.535,0.54,0.545,0.55,0.555,0.56,0.565,0.57,0.575,0.58,0.585,0.59,
0.595,0.6,0.605,0.61,0.615,0.62,0.625,0.63,0.635,0.64,0.645,0.65,0.655,
0.66,0.665,0.67,0.675,0.68,0.685,0.690000000000001,0.695000000000001,0.700000000000001,
0.705000000000001,0.710000000000001,0.715000000000001,0.720000000000001,
0.725000000000001,0.730000000000001,0.735000000000001,0.740000000000001,
0.745000000000001,0.750000000000001,0.755000000000001,0.760000000000001,
0.765000000000001,0.770000000000001,0.775000000000001,0.780000000000001,
0.785000000000001,0.790000000000001,0.795000000000001,0.800000000000001,
0.805000000000001,0.810000000000001,0.815000000000001,0.820000000000001,
0.825000000000001,0.830000000000001,0.835000000000001,0.840000000000001,
0.845000000000001,0.850000000000001,0.855000000000001,0.860000000000001,
0.865000000000001,0.870000000000001,0.875000000000001,0.880000000000001,
0.885000000000001,0.890000000000001,0.895000000000001,0.900000000000001,
0.905000000000001,0.910000000000001,0.915000000000001,0.920000000000001,
0.925000000000001,0.930000000000001,0.935000000000001,0.940000000000001,
0.945000000000001,0.950000000000001,0.955000000000001,0.960000000000001,
0.965000000000001,0.970000000000001,0.975000000000001,0.980000000000001,
0.985000000000001,0.990000000000001,0.995000000000001,1.),(0.,1.2),
 .UNSPECIFIED.)
GEOMETRIC_REPRESENTATION_ITEM()
RATIONAL_B_SPLINE_SURFACE(((1.,1.),(1.,1.),(1.,1.),(1.,1.),(1.,1.),(1.,
1.),(1.,1.),(1.,1.),(1.,1.),(1.,1.),(1.,1.),(1.,1.),(1.,1.),(1.,1.),(1.,
1.),(1.,1.),(1.,1.),(1.,1.),(1.,1.),(1.,1.),(1.,1.),(1.,1.),(1.,1.),(1.,
1.),(1.,1.),(1.,1.),(1.,1.),(1.,1.),(1.,1.),(1.,1.),(1.,1.),(1.,1.),(1.,
1.),(1.,1.),(1.,1.),(1.,1.),(1.,1.),(1.,1.),(1.,1.),(1.,1.),(1.,1.),(1.,
1.),(1.,1.),(1.,1.),(1.,1.),(1.,1.),(1.,1.),(1.,1.),(1.,1.),(1.,1.),(1.,
1.),(1.,1.),(1.,1.),(1.,1.),(1.,1.),(1.,1.),(1.,1.),(1.,1.),(1.,1.),(1.,
1.),(1.,1.),(1.,1.),(1.,1.),(1.,1.),(1.,1.),(1.,1.),(1.,1.),(1.,1.),(1.,
1.),(1.,1.),(1.,1.),(1.,1.),(1.,1.),(1.,1.),(1.,1.),(1.,1.),(1.,1.),(1.,
1.),(1.,1.),(1.,1.),(1.,1.),(1.,1.),(1.,1.),(1.,1.),(1.,1.),(1.,1.),(1.,
1.),(1.,1.),(1.,1.),(1.,1.),(1.,1.),(1.,1.),(1.,1.),(1.,1.),(1.,1.),(1.,
1.),(1.,1.),(1.,1.),(1.,1.),(1.,1.),(1.,1.),(1.,1.),(1.,1.),(1.,1.),(1.,
1.),(1.,1.),(1.,1.),(1.,1.),(1.,1.),(1.,1.),(1.,1.),(1.,1.),(1.,1.),(1.,
1.),(1.,1.),(1.,1.),(1.,1.),(1.,1.),(1.,1.),(1.,1.),(1.,1.),(1.,1.),(1.,
1.),(1.,1.),(1.,1.),(1.,1.),(1.,1.),(1.,1.),(1.,1.),(1.,1.),(1.,1.),(1.,
1.),(1.,1.),(1.,1.),(1.,1.),(1.,1.),(1.,1.),(1.,1.),(1.,1.),(1.,1.),(1.,
1.),(1.,1.),(1.,1.),(1.,1.),(1.,1.),(1.,1.),(1.,1.),(1.,1.),(1.,1.),(1.,
1.),(1.,1.),(1.,1.),(1.,1.),(1.,1.),(1.,1.),(1.,1.),(1.,1.),(1.,1.),(1.,
1.),(1.,1.),(1.,1.),(1.,1.),(1.,1.),(1.,1.),(1.,1.),(1.,1.),(1.,1.),(1.,
1.),(1.,1.),(1.,1.),(1.,1.),(1.,1.),(1.,1.),(1.,1.),(1.,1.),(1.,1.),(1.,
1.),(1.,1.),(1.,1.),(1.,1.),(1.,1.),(1.,1.),(1.,1.),(1.,1.),(1.,1.),(1.,
1.),(1.,1.),(1.,1.),(1.,1.),(1.,1.),(1.,1.),(1.,1.),(1.,1.),(1.,1.),(1.,
1.),(1.,1.),(1.,1.),(1.,1.),(1.,1.),(1.,1.),(1.,1.),(1.,1.),(1.,1.),(1.,
1.),(1.,1.)))
REPRESENTATION_ITEM('')
SURFACE()
);
#885=(
BOUNDED_SURFACE()
B_SPLINE_SURFACE(5,1,((#54414,#54415),(#54416,#54417),(#54418,#54419),(#54420,
#54421),(#54422,#54423),(#54424,#54425),(#54426,#54427),(#54428,#54429),
(#54430,#54431),(#54432,#54433),(#54434,#54435),(#54436,#54437),(#54438,
#54439),(#54440,#54441),(#54442,#54443),(#54444,#54445),(#54446,#54447),
(#54448,#54449),(#54450,#54451),(#54452,#54453),(#54454,#54455),(#54456,
#54457),(#54458,#54459),(#54460,#54461),(#54462,#54463),(#54464,#54465),
(#54466,#54467),(#54468,#54469),(#54470,#54471),(#54472,#54473),(#54474,
#54475),(#54476,#54477),(#54478,#54479),(#54480,#54481),(#54482,#54483),
(#54484,#54485),(#54486,#54487),(#54488,#54489),(#54490,#54491),(#54492,
#54493),(#54494,#54495),(#54496,#54497),(#54498,#54499),(#54500,#54501),
(#54502,#54503),(#54504,#54505),(#54506,#54507),(#54508,#54509),(#54510,
#54511),(#54512,#54513),(#54514,#54515),(#54516,#54517),(#54518,#54519),
(#54520,#54521),(#54522,#54523),(#54524,#54525),(#54526,#54527),(#54528,
#54529),(#54530,#54531),(#54532,#54533),(#54534,#54535),(#54536,#54537),
(#54538,#54539),(#54540,#54541),(#54542,#54543),(#54544,#54545),(#54546,
#54547),(#54548,#54549),(#54550,#54551),(#54552,#54553),(#54554,#54555),
(#54556,#54557),(#54558,#54559),(#54560,#54561),(#54562,#54563),(#54564,
#54565),(#54566,#54567),(#54568,#54569),(#54570,#54571),(#54572,#54573),
(#54574,#54575),(#54576,#54577),(#54578,#54579),(#54580,#54581),(#54582,
#54583),(#54584,#54585),(#54586,#54587),(#54588,#54589),(#54590,#54591),
(#54592,#54593),(#54594,#54595),(#54596,#54597),(#54598,#54599),(#54600,
#54601),(#54602,#54603),(#54604,#54605),(#54606,#54607),(#54608,#54609),
(#54610,#54611),(#54612,#54613),(#54614,#54615),(#54616,#54617),(#54618,
#54619),(#54620,#54621),(#54622,#54623),(#54624,#54625),(#54626,#54627),
(#54628,#54629),(#54630,#54631),(#54632,#54633),(#54634,#54635),(#54636,
#54637),(#54638,#54639),(#54640,#54641),(#54642,#54643),(#54644,#54645),
(#54646,#54647),(#54648,#54649),(#54650,#54651),(#54652,#54653),(#54654,
#54655),(#54656,#54657),(#54658,#54659),(#54660,#54661),(#54662,#54663),
(#54664,#54665),(#54666,#54667),(#54668,#54669),(#54670,#54671),(#54672,
#54673),(#54674,#54675),(#54676,#54677),(#54678,#54679),(#54680,#54681),
(#54682,#54683),(#54684,#54685),(#54686,#54687),(#54688,#54689),(#54690,
#54691),(#54692,#54693),(#54694,#54695),(#54696,#54697),(#54698,#54699),
(#54700,#54701),(#54702,#54703),(#54704,#54705),(#54706,#54707),(#54708,
#54709),(#54710,#54711),(#54712,#54713),(#54714,#54715),(#54716,#54717),
(#54718,#54719),(#54720,#54721),(#54722,#54723),(#54724,#54725),(#54726,
#54727),(#54728,#54729),(#54730,#54731),(#54732,#54733),(#54734,#54735),
(#54736,#54737),(#54738,#54739),(#54740,#54741),(#54742,#54743),(#54744,
#54745),(#54746,#54747),(#54748,#54749),(#54750,#54751),(#54752,#54753),
(#54754,#54755),(#54756,#54757),(#54758,#54759),(#54760,#54761),(#54762,
#54763),(#54764,#54765),(#54766,#54767),(#54768,#54769),(#54770,#54771),
(#54772,#54773),(#54774,#54775),(#54776,#54777),(#54778,#54779),(#54780,
#54781),(#54782,#54783),(#54784,#54785),(#54786,#54787),(#54788,#54789),
(#54790,#54791),(#54792,#54793),(#54794,#54795),(#54796,#54797),(#54798,
#54799),(#54800,#54801),(#54802,#54803),(#54804,#54805),(#54806,#54807),
(#54808,#54809),(#54810,#54811),(#54812,#54813),(#54814,#54815),(#54816,
#54817),(#54818,#54819),(#54820,#54821),(#54822,#54823)),.UNSPECIFIED.,
 .F.,.F.,.F.)
B_SPLINE_SURFACE_WITH_KNOTS((6,1,1,1,1,1,1,1,1,1,1,1,1,1,1,1,1,1,1,1,1,
1,1,1,1,1,1,1,1,1,1,1,1,1,1,1,1,1,1,1,1,1,1,1,1,1,1,1,1,1,1,1,1,1,1,1,1,
1,1,1,1,1,1,1,1,1,1,1,1,1,1,1,1,1,1,1,1,1,1,1,1,1,1,1,1,1,1,1,1,1,1,1,1,
1,1,1,1,1,1,1,1,1,1,1,1,1,1,1,1,1,1,1,1,1,1,1,1,1,1,1,1,1,1,1,1,1,1,1,1,
1,1,1,1,1,1,1,1,1,1,1,1,1,1,1,1,1,1,1,1,1,1,1,1,1,1,1,1,1,1,1,1,1,1,1,1,
1,1,1,1,1,1,1,1,1,1,1,1,1,1,1,1,1,1,1,1,1,1,1,1,1,1,1,1,1,1,1,1,1,1,1,6),
(2,2),(0.,0.005,0.01,0.015,0.02,0.025,0.03,0.035,0.04,0.045,0.05,0.055,
0.06,0.065,0.07,0.075,0.08,0.085,0.09,0.095,0.1,0.105,0.11,0.115,0.12,0.125,
0.13,0.135,0.14,0.145,0.15,0.155,0.16,0.165,0.17,0.175,0.18,0.185,0.19,
0.195,0.2,0.205,0.21,0.215,0.22,0.225,0.23,0.235,0.24,0.245,0.25,0.255,
0.26,0.265,0.27,0.275,0.28,0.285,0.29,0.295,0.3,0.305,0.31,0.315,0.32,0.325,
0.33,0.335,0.34,0.345,0.35,0.355,0.36,0.365,0.37,0.375,0.38,0.385,0.39,
0.395,0.4,0.405,0.41,0.415,0.42,0.425,0.43,0.435,0.44,0.445,0.45,0.455,
0.46,0.465,0.47,0.475,0.48,0.485,0.49,0.495,0.5,0.505,0.51,0.515,0.52,0.525,
0.53,0.535,0.54,0.545,0.55,0.555,0.56,0.565,0.57,0.575,0.58,0.585,0.59,
0.595,0.6,0.605,0.61,0.615,0.62,0.625,0.63,0.635,0.64,0.645,0.65,0.655,
0.66,0.665,0.67,0.675,0.68,0.685,0.690000000000001,0.695000000000001,0.700000000000001,
0.705000000000001,0.710000000000001,0.715000000000001,0.720000000000001,
0.725000000000001,0.730000000000001,0.735000000000001,0.740000000000001,
0.745000000000001,0.750000000000001,0.755000000000001,0.760000000000001,
0.765000000000001,0.770000000000001,0.775000000000001,0.780000000000001,
0.785000000000001,0.790000000000001,0.795000000000001,0.800000000000001,
0.805000000000001,0.810000000000001,0.815000000000001,0.820000000000001,
0.825000000000001,0.830000000000001,0.835000000000001,0.840000000000001,
0.845000000000001,0.850000000000001,0.855000000000001,0.860000000000001,
0.865000000000001,0.870000000000001,0.875000000000001,0.880000000000001,
0.885000000000001,0.890000000000001,0.895000000000001,0.900000000000001,
0.905000000000001,0.910000000000001,0.915000000000001,0.920000000000001,
0.925000000000001,0.930000000000001,0.935000000000001,0.940000000000001,
0.945000000000001,0.950000000000001,0.955000000000001,0.960000000000001,
0.965000000000001,0.970000000000001,0.975000000000001,0.980000000000001,
0.985000000000001,0.990000000000001,0.995000000000001,1.),(0.,1.2),
 .UNSPECIFIED.)
GEOMETRIC_REPRESENTATION_ITEM()
RATIONAL_B_SPLINE_SURFACE(((1.,1.),(1.,1.),(1.,1.),(1.,1.),(1.,1.),(1.,
1.),(1.,1.),(1.,1.),(1.,1.),(1.,1.),(1.,1.),(1.,1.),(1.,1.),(1.,1.),(1.,
1.),(1.,1.),(1.,1.),(1.,1.),(1.,1.),(1.,1.),(1.,1.),(1.,1.),(1.,1.),(1.,
1.),(1.,1.),(1.,1.),(1.,1.),(1.,1.),(1.,1.),(1.,1.),(1.,1.),(1.,1.),(1.,
1.),(1.,1.),(1.,1.),(1.,1.),(1.,1.),(1.,1.),(1.,1.),(1.,1.),(1.,1.),(1.,
1.),(1.,1.),(1.,1.),(1.,1.),(1.,1.),(1.,1.),(1.,1.),(1.,1.),(1.,1.),(1.,
1.),(1.,1.),(1.,1.),(1.,1.),(1.,1.),(1.,1.),(1.,1.),(1.,1.),(1.,1.),(1.,
1.),(1.,1.),(1.,1.),(1.,1.),(1.,1.),(1.,1.),(1.,1.),(1.,1.),(1.,1.),(1.,
1.),(1.,1.),(1.,1.),(1.,1.),(1.,1.),(1.,1.),(1.,1.),(1.,1.),(1.,1.),(1.,
1.),(1.,1.),(1.,1.),(1.,1.),(1.,1.),(1.,1.),(1.,1.),(1.,1.),(1.,1.),(1.,
1.),(1.,1.),(1.,1.),(1.,1.),(1.,1.),(1.,1.),(1.,1.),(1.,1.),(1.,1.),(1.,
1.),(1.,1.),(1.,1.),(1.,1.),(1.,1.),(1.,1.),(1.,1.),(1.,1.),(1.,1.),(1.,
1.),(1.,1.),(1.,1.),(1.,1.),(1.,1.),(1.,1.),(1.,1.),(1.,1.),(1.,1.),(1.,
1.),(1.,1.),(1.,1.),(1.,1.),(1.,1.),(1.,1.),(1.,1.),(1.,1.),(1.,1.),(1.,
1.),(1.,1.),(1.,1.),(1.,1.),(1.,1.),(1.,1.),(1.,1.),(1.,1.),(1.,1.),(1.,
1.),(1.,1.),(1.,1.),(1.,1.),(1.,1.),(1.,1.),(1.,1.),(1.,1.),(1.,1.),(1.,
1.),(1.,1.),(1.,1.),(1.,1.),(1.,1.),(1.,1.),(1.,1.),(1.,1.),(1.,1.),(1.,
1.),(1.,1.),(1.,1.),(1.,1.),(1.,1.),(1.,1.),(1.,1.),(1.,1.),(1.,1.),(1.,
1.),(1.,1.),(1.,1.),(1.,1.),(1.,1.),(1.,1.),(1.,1.),(1.,1.),(1.,1.),(1.,
1.),(1.,1.),(1.,1.),(1.,1.),(1.,1.),(1.,1.),(1.,1.),(1.,1.),(1.,1.),(1.,
1.),(1.,1.),(1.,1.),(1.,1.),(1.,1.),(1.,1.),(1.,1.),(1.,1.),(1.,1.),(1.,
1.),(1.,1.),(1.,1.),(1.,1.),(1.,1.),(1.,1.),(1.,1.),(1.,1.),(1.,1.),(1.,
1.),(1.,1.),(1.,1.),(1.,1.),(1.,1.),(1.,1.),(1.,1.),(1.,1.),(1.,1.),(1.,
1.),(1.,1.)))
REPRESENTATION_ITEM('')
SURFACE()
);
#886=(
BOUNDED_SURFACE()
B_SPLINE_SURFACE(5,1,((#55310,#55311),(#55312,#55313),(#55314,#55315),(#55316,
#55317),(#55318,#55319),(#55320,#55321),(#55322,#55323),(#55324,#55325),
(#55326,#55327),(#55328,#55329),(#55330,#55331),(#55332,#55333),(#55334,
#55335),(#55336,#55337),(#55338,#55339),(#55340,#55341),(#55342,#55343),
(#55344,#55345),(#55346,#55347),(#55348,#55349),(#55350,#55351),(#55352,
#55353),(#55354,#55355),(#55356,#55357),(#55358,#55359),(#55360,#55361),
(#55362,#55363),(#55364,#55365),(#55366,#55367),(#55368,#55369),(#55370,
#55371),(#55372,#55373),(#55374,#55375),(#55376,#55377),(#55378,#55379),
(#55380,#55381),(#55382,#55383),(#55384,#55385),(#55386,#55387),(#55388,
#55389),(#55390,#55391),(#55392,#55393),(#55394,#55395),(#55396,#55397),
(#55398,#55399),(#55400,#55401),(#55402,#55403),(#55404,#55405),(#55406,
#55407),(#55408,#55409),(#55410,#55411),(#55412,#55413),(#55414,#55415),
(#55416,#55417),(#55418,#55419),(#55420,#55421),(#55422,#55423),(#55424,
#55425),(#55426,#55427),(#55428,#55429),(#55430,#55431),(#55432,#55433),
(#55434,#55435),(#55436,#55437),(#55438,#55439),(#55440,#55441),(#55442,
#55443),(#55444,#55445),(#55446,#55447),(#55448,#55449),(#55450,#55451),
(#55452,#55453),(#55454,#55455),(#55456,#55457),(#55458,#55459),(#55460,
#55461),(#55462,#55463),(#55464,#55465),(#55466,#55467),(#55468,#55469),
(#55470,#55471),(#55472,#55473),(#55474,#55475),(#55476,#55477),(#55478,
#55479),(#55480,#55481),(#55482,#55483),(#55484,#55485),(#55486,#55487),
(#55488,#55489),(#55490,#55491),(#55492,#55493),(#55494,#55495),(#55496,
#55497),(#55498,#55499),(#55500,#55501),(#55502,#55503),(#55504,#55505),
(#55506,#55507),(#55508,#55509),(#55510,#55511),(#55512,#55513),(#55514,
#55515),(#55516,#55517),(#55518,#55519),(#55520,#55521),(#55522,#55523),
(#55524,#55525),(#55526,#55527),(#55528,#55529),(#55530,#55531),(#55532,
#55533),(#55534,#55535),(#55536,#55537),(#55538,#55539),(#55540,#55541),
(#55542,#55543),(#55544,#55545),(#55546,#55547),(#55548,#55549),(#55550,
#55551),(#55552,#55553),(#55554,#55555),(#55556,#55557),(#55558,#55559),
(#55560,#55561),(#55562,#55563),(#55564,#55565),(#55566,#55567),(#55568,
#55569),(#55570,#55571),(#55572,#55573),(#55574,#55575),(#55576,#55577),
(#55578,#55579),(#55580,#55581),(#55582,#55583),(#55584,#55585),(#55586,
#55587),(#55588,#55589),(#55590,#55591),(#55592,#55593),(#55594,#55595),
(#55596,#55597),(#55598,#55599),(#55600,#55601),(#55602,#55603),(#55604,
#55605),(#55606,#55607),(#55608,#55609),(#55610,#55611),(#55612,#55613),
(#55614,#55615),(#55616,#55617),(#55618,#55619),(#55620,#55621),(#55622,
#55623),(#55624,#55625),(#55626,#55627),(#55628,#55629),(#55630,#55631),
(#55632,#55633),(#55634,#55635),(#55636,#55637),(#55638,#55639),(#55640,
#55641),(#55642,#55643),(#55644,#55645),(#55646,#55647),(#55648,#55649),
(#55650,#55651),(#55652,#55653),(#55654,#55655),(#55656,#55657),(#55658,
#55659),(#55660,#55661),(#55662,#55663),(#55664,#55665),(#55666,#55667),
(#55668,#55669),(#55670,#55671),(#55672,#55673),(#55674,#55675),(#55676,
#55677),(#55678,#55679),(#55680,#55681),(#55682,#55683),(#55684,#55685),
(#55686,#55687),(#55688,#55689),(#55690,#55691),(#55692,#55693),(#55694,
#55695),(#55696,#55697),(#55698,#55699),(#55700,#55701),(#55702,#55703),
(#55704,#55705),(#55706,#55707),(#55708,#55709),(#55710,#55711),(#55712,
#55713),(#55714,#55715),(#55716,#55717),(#55718,#55719)),.UNSPECIFIED.,
 .F.,.F.,.F.)
B_SPLINE_SURFACE_WITH_KNOTS((6,1,1,1,1,1,1,1,1,1,1,1,1,1,1,1,1,1,1,1,1,
1,1,1,1,1,1,1,1,1,1,1,1,1,1,1,1,1,1,1,1,1,1,1,1,1,1,1,1,1,1,1,1,1,1,1,1,
1,1,1,1,1,1,1,1,1,1,1,1,1,1,1,1,1,1,1,1,1,1,1,1,1,1,1,1,1,1,1,1,1,1,1,1,
1,1,1,1,1,1,1,1,1,1,1,1,1,1,1,1,1,1,1,1,1,1,1,1,1,1,1,1,1,1,1,1,1,1,1,1,
1,1,1,1,1,1,1,1,1,1,1,1,1,1,1,1,1,1,1,1,1,1,1,1,1,1,1,1,1,1,1,1,1,1,1,1,
1,1,1,1,1,1,1,1,1,1,1,1,1,1,1,1,1,1,1,1,1,1,1,1,1,1,1,1,1,1,1,1,1,1,1,6),
(2,2),(0.,0.005,0.01,0.015,0.02,0.025,0.03,0.035,0.04,0.045,0.05,0.055,
0.06,0.065,0.07,0.075,0.08,0.085,0.09,0.095,0.1,0.105,0.11,0.115,0.12,0.125,
0.13,0.135,0.14,0.145,0.15,0.155,0.16,0.165,0.17,0.175,0.18,0.185,0.19,
0.195,0.2,0.205,0.21,0.215,0.22,0.225,0.23,0.235,0.24,0.245,0.25,0.255,
0.26,0.265,0.27,0.275,0.28,0.285,0.29,0.295,0.3,0.305,0.31,0.315,0.32,0.325,
0.33,0.335,0.34,0.345,0.35,0.355,0.36,0.365,0.37,0.375,0.38,0.385,0.39,
0.395,0.4,0.405,0.41,0.415,0.42,0.425,0.43,0.435,0.44,0.445,0.45,0.455,
0.46,0.465,0.47,0.475,0.48,0.485,0.49,0.495,0.5,0.505,0.51,0.515,0.52,0.525,
0.53,0.535,0.54,0.545,0.55,0.555,0.56,0.565,0.57,0.575,0.58,0.585,0.59,
0.595,0.6,0.605,0.61,0.615,0.62,0.625,0.63,0.635,0.64,0.645,0.65,0.655,
0.66,0.665,0.67,0.675,0.68,0.685,0.690000000000001,0.695000000000001,0.700000000000001,
0.705000000000001,0.710000000000001,0.715000000000001,0.720000000000001,
0.725000000000001,0.730000000000001,0.735000000000001,0.740000000000001,
0.745000000000001,0.750000000000001,0.755000000000001,0.760000000000001,
0.765000000000001,0.770000000000001,0.775000000000001,0.780000000000001,
0.785000000000001,0.790000000000001,0.795000000000001,0.800000000000001,
0.805000000000001,0.810000000000001,0.815000000000001,0.820000000000001,
0.825000000000001,0.830000000000001,0.835000000000001,0.840000000000001,
0.845000000000001,0.850000000000001,0.855000000000001,0.860000000000001,
0.865000000000001,0.870000000000001,0.875000000000001,0.880000000000001,
0.885000000000001,0.890000000000001,0.895000000000001,0.900000000000001,
0.905000000000001,0.910000000000001,0.915000000000001,0.920000000000001,
0.925000000000001,0.930000000000001,0.935000000000001,0.940000000000001,
0.945000000000001,0.950000000000001,0.955000000000001,0.960000000000001,
0.965000000000001,0.970000000000001,0.975000000000001,0.980000000000001,
0.985000000000001,0.990000000000001,0.995000000000001,1.),(0.,1.2),
 .UNSPECIFIED.)
GEOMETRIC_REPRESENTATION_ITEM()
RATIONAL_B_SPLINE_SURFACE(((1.,1.),(1.,1.),(1.,1.),(1.,1.),(1.,1.),(1.,
1.),(1.,1.),(1.,1.),(1.,1.),(1.,1.),(1.,1.),(1.,1.),(1.,1.),(1.,1.),(1.,
1.),(1.,1.),(1.,1.),(1.,1.),(1.,1.),(1.,1.),(1.,1.),(1.,1.),(1.,1.),(1.,
1.),(1.,1.),(1.,1.),(1.,1.),(1.,1.),(1.,1.),(1.,1.),(1.,1.),(1.,1.),(1.,
1.),(1.,1.),(1.,1.),(1.,1.),(1.,1.),(1.,1.),(1.,1.),(1.,1.),(1.,1.),(1.,
1.),(1.,1.),(1.,1.),(1.,1.),(1.,1.),(1.,1.),(1.,1.),(1.,1.),(1.,1.),(1.,
1.),(1.,1.),(1.,1.),(1.,1.),(1.,1.),(1.,1.),(1.,1.),(1.,1.),(1.,1.),(1.,
1.),(1.,1.),(1.,1.),(1.,1.),(1.,1.),(1.,1.),(1.,1.),(1.,1.),(1.,1.),(1.,
1.),(1.,1.),(1.,1.),(1.,1.),(1.,1.),(1.,1.),(1.,1.),(1.,1.),(1.,1.),(1.,
1.),(1.,1.),(1.,1.),(1.,1.),(1.,1.),(1.,1.),(1.,1.),(1.,1.),(1.,1.),(1.,
1.),(1.,1.),(1.,1.),(1.,1.),(1.,1.),(1.,1.),(1.,1.),(1.,1.),(1.,1.),(1.,
1.),(1.,1.),(1.,1.),(1.,1.),(1.,1.),(1.,1.),(1.,1.),(1.,1.),(1.,1.),(1.,
1.),(1.,1.),(1.,1.),(1.,1.),(1.,1.),(1.,1.),(1.,1.),(1.,1.),(1.,1.),(1.,
1.),(1.,1.),(1.,1.),(1.,1.),(1.,1.),(1.,1.),(1.,1.),(1.,1.),(1.,1.),(1.,
1.),(1.,1.),(1.,1.),(1.,1.),(1.,1.),(1.,1.),(1.,1.),(1.,1.),(1.,1.),(1.,
1.),(1.,1.),(1.,1.),(1.,1.),(1.,1.),(1.,1.),(1.,1.),(1.,1.),(1.,1.),(1.,
1.),(1.,1.),(1.,1.),(1.,1.),(1.,1.),(1.,1.),(1.,1.),(1.,1.),(1.,1.),(1.,
1.),(1.,1.),(1.,1.),(1.,1.),(1.,1.),(1.,1.),(1.,1.),(1.,1.),(1.,1.),(1.,
1.),(1.,1.),(1.,1.),(1.,1.),(1.,1.),(1.,1.),(1.,1.),(1.,1.),(1.,1.),(1.,
1.),(1.,1.),(1.,1.),(1.,1.),(1.,1.),(1.,1.),(1.,1.),(1.,1.),(1.,1.),(1.,
1.),(1.,1.),(1.,1.),(1.,1.),(1.,1.),(1.,1.),(1.,1.),(1.,1.),(1.,1.),(1.,
1.),(1.,1.),(1.,1.),(1.,1.),(1.,1.),(1.,1.),(1.,1.),(1.,1.),(1.,1.),(1.,
1.),(1.,1.),(1.,1.),(1.,1.),(1.,1.),(1.,1.),(1.,1.),(1.,1.),(1.,1.),(1.,
1.),(1.,1.)))
REPRESENTATION_ITEM('')
SURFACE()
);
#887=(
BOUNDED_SURFACE()
B_SPLINE_SURFACE(5,1,((#56206,#56207),(#56208,#56209),(#56210,#56211),(#56212,
#56213),(#56214,#56215),(#56216,#56217),(#56218,#56219),(#56220,#56221),
(#56222,#56223),(#56224,#56225),(#56226,#56227),(#56228,#56229),(#56230,
#56231),(#56232,#56233),(#56234,#56235),(#56236,#56237),(#56238,#56239),
(#56240,#56241),(#56242,#56243),(#56244,#56245),(#56246,#56247),(#56248,
#56249),(#56250,#56251),(#56252,#56253),(#56254,#56255),(#56256,#56257),
(#56258,#56259),(#56260,#56261),(#56262,#56263),(#56264,#56265),(#56266,
#56267),(#56268,#56269),(#56270,#56271),(#56272,#56273),(#56274,#56275),
(#56276,#56277),(#56278,#56279),(#56280,#56281),(#56282,#56283),(#56284,
#56285),(#56286,#56287),(#56288,#56289),(#56290,#56291),(#56292,#56293),
(#56294,#56295),(#56296,#56297),(#56298,#56299),(#56300,#56301),(#56302,
#56303),(#56304,#56305),(#56306,#56307),(#56308,#56309),(#56310,#56311),
(#56312,#56313),(#56314,#56315),(#56316,#56317),(#56318,#56319),(#56320,
#56321),(#56322,#56323),(#56324,#56325),(#56326,#56327),(#56328,#56329),
(#56330,#56331),(#56332,#56333),(#56334,#56335),(#56336,#56337),(#56338,
#56339),(#56340,#56341),(#56342,#56343),(#56344,#56345),(#56346,#56347),
(#56348,#56349),(#56350,#56351),(#56352,#56353),(#56354,#56355),(#56356,
#56357),(#56358,#56359),(#56360,#56361),(#56362,#56363),(#56364,#56365),
(#56366,#56367),(#56368,#56369),(#56370,#56371),(#56372,#56373),(#56374,
#56375),(#56376,#56377),(#56378,#56379),(#56380,#56381),(#56382,#56383),
(#56384,#56385),(#56386,#56387),(#56388,#56389),(#56390,#56391),(#56392,
#56393),(#56394,#56395),(#56396,#56397),(#56398,#56399),(#56400,#56401),
(#56402,#56403),(#56404,#56405),(#56406,#56407),(#56408,#56409),(#56410,
#56411),(#56412,#56413),(#56414,#56415),(#56416,#56417),(#56418,#56419),
(#56420,#56421),(#56422,#56423),(#56424,#56425),(#56426,#56427),(#56428,
#56429),(#56430,#56431),(#56432,#56433),(#56434,#56435),(#56436,#56437),
(#56438,#56439),(#56440,#56441),(#56442,#56443),(#56444,#56445),(#56446,
#56447),(#56448,#56449),(#56450,#56451),(#56452,#56453),(#56454,#56455),
(#56456,#56457),(#56458,#56459),(#56460,#56461),(#56462,#56463),(#56464,
#56465),(#56466,#56467),(#56468,#56469),(#56470,#56471),(#56472,#56473),
(#56474,#56475),(#56476,#56477),(#56478,#56479),(#56480,#56481),(#56482,
#56483),(#56484,#56485),(#56486,#56487),(#56488,#56489),(#56490,#56491),
(#56492,#56493),(#56494,#56495),(#56496,#56497),(#56498,#56499),(#56500,
#56501),(#56502,#56503),(#56504,#56505),(#56506,#56507),(#56508,#56509),
(#56510,#56511),(#56512,#56513),(#56514,#56515),(#56516,#56517),(#56518,
#56519),(#56520,#56521),(#56522,#56523),(#56524,#56525),(#56526,#56527),
(#56528,#56529),(#56530,#56531),(#56532,#56533),(#56534,#56535),(#56536,
#56537),(#56538,#56539),(#56540,#56541),(#56542,#56543),(#56544,#56545),
(#56546,#56547),(#56548,#56549),(#56550,#56551),(#56552,#56553),(#56554,
#56555),(#56556,#56557),(#56558,#56559),(#56560,#56561),(#56562,#56563),
(#56564,#56565),(#56566,#56567),(#56568,#56569),(#56570,#56571),(#56572,
#56573),(#56574,#56575),(#56576,#56577),(#56578,#56579),(#56580,#56581),
(#56582,#56583),(#56584,#56585),(#56586,#56587),(#56588,#56589),(#56590,
#56591),(#56592,#56593),(#56594,#56595),(#56596,#56597),(#56598,#56599),
(#56600,#56601),(#56602,#56603),(#56604,#56605),(#56606,#56607),(#56608,
#56609),(#56610,#56611),(#56612,#56613),(#56614,#56615)),.UNSPECIFIED.,
 .F.,.F.,.F.)
B_SPLINE_SURFACE_WITH_KNOTS((6,1,1,1,1,1,1,1,1,1,1,1,1,1,1,1,1,1,1,1,1,
1,1,1,1,1,1,1,1,1,1,1,1,1,1,1,1,1,1,1,1,1,1,1,1,1,1,1,1,1,1,1,1,1,1,1,1,
1,1,1,1,1,1,1,1,1,1,1,1,1,1,1,1,1,1,1,1,1,1,1,1,1,1,1,1,1,1,1,1,1,1,1,1,
1,1,1,1,1,1,1,1,1,1,1,1,1,1,1,1,1,1,1,1,1,1,1,1,1,1,1,1,1,1,1,1,1,1,1,1,
1,1,1,1,1,1,1,1,1,1,1,1,1,1,1,1,1,1,1,1,1,1,1,1,1,1,1,1,1,1,1,1,1,1,1,1,
1,1,1,1,1,1,1,1,1,1,1,1,1,1,1,1,1,1,1,1,1,1,1,1,1,1,1,1,1,1,1,1,1,1,1,6),
(2,2),(0.,0.005,0.01,0.015,0.02,0.025,0.03,0.035,0.04,0.045,0.05,0.055,
0.06,0.065,0.07,0.075,0.08,0.085,0.09,0.095,0.1,0.105,0.11,0.115,0.12,0.125,
0.13,0.135,0.14,0.145,0.15,0.155,0.16,0.165,0.17,0.175,0.18,0.185,0.19,
0.195,0.2,0.205,0.21,0.215,0.22,0.225,0.23,0.235,0.24,0.245,0.25,0.255,
0.26,0.265,0.27,0.275,0.28,0.285,0.29,0.295,0.3,0.305,0.31,0.315,0.32,0.325,
0.33,0.335,0.34,0.345,0.35,0.355,0.36,0.365,0.37,0.375,0.38,0.385,0.39,
0.395,0.4,0.405,0.41,0.415,0.42,0.425,0.43,0.435,0.44,0.445,0.45,0.455,
0.46,0.465,0.47,0.475,0.48,0.485,0.49,0.495,0.5,0.505,0.51,0.515,0.52,0.525,
0.53,0.535,0.54,0.545,0.55,0.555,0.56,0.565,0.57,0.575,0.58,0.585,0.59,
0.595,0.6,0.605,0.61,0.615,0.62,0.625,0.63,0.635,0.64,0.645,0.65,0.655,
0.66,0.665,0.67,0.675,0.68,0.685,0.690000000000001,0.695000000000001,0.700000000000001,
0.705000000000001,0.710000000000001,0.715000000000001,0.720000000000001,
0.725000000000001,0.730000000000001,0.735000000000001,0.740000000000001,
0.745000000000001,0.750000000000001,0.755000000000001,0.760000000000001,
0.765000000000001,0.770000000000001,0.775000000000001,0.780000000000001,
0.785000000000001,0.790000000000001,0.795000000000001,0.800000000000001,
0.805000000000001,0.810000000000001,0.815000000000001,0.820000000000001,
0.825000000000001,0.830000000000001,0.835000000000001,0.840000000000001,
0.845000000000001,0.850000000000001,0.855000000000001,0.860000000000001,
0.865000000000001,0.870000000000001,0.875000000000001,0.880000000000001,
0.885000000000001,0.890000000000001,0.895000000000001,0.900000000000001,
0.905000000000001,0.910000000000001,0.915000000000001,0.920000000000001,
0.925000000000001,0.930000000000001,0.935000000000001,0.940000000000001,
0.945000000000001,0.950000000000001,0.955000000000001,0.960000000000001,
0.965000000000001,0.970000000000001,0.975000000000001,0.980000000000001,
0.985000000000001,0.990000000000001,0.995000000000001,1.),(0.,1.2),
 .UNSPECIFIED.)
GEOMETRIC_REPRESENTATION_ITEM()
RATIONAL_B_SPLINE_SURFACE(((1.,1.),(1.,1.),(1.,1.),(1.,1.),(1.,1.),(1.,
1.),(1.,1.),(1.,1.),(1.,1.),(1.,1.),(1.,1.),(1.,1.),(1.,1.),(1.,1.),(1.,
1.),(1.,1.),(1.,1.),(1.,1.),(1.,1.),(1.,1.),(1.,1.),(1.,1.),(1.,1.),(1.,
1.),(1.,1.),(1.,1.),(1.,1.),(1.,1.),(1.,1.),(1.,1.),(1.,1.),(1.,1.),(1.,
1.),(1.,1.),(1.,1.),(1.,1.),(1.,1.),(1.,1.),(1.,1.),(1.,1.),(1.,1.),(1.,
1.),(1.,1.),(1.,1.),(1.,1.),(1.,1.),(1.,1.),(1.,1.),(1.,1.),(1.,1.),(1.,
1.),(1.,1.),(1.,1.),(1.,1.),(1.,1.),(1.,1.),(1.,1.),(1.,1.),(1.,1.),(1.,
1.),(1.,1.),(1.,1.),(1.,1.),(1.,1.),(1.,1.),(1.,1.),(1.,1.),(1.,1.),(1.,
1.),(1.,1.),(1.,1.),(1.,1.),(1.,1.),(1.,1.),(1.,1.),(1.,1.),(1.,1.),(1.,
1.),(1.,1.),(1.,1.),(1.,1.),(1.,1.),(1.,1.),(1.,1.),(1.,1.),(1.,1.),(1.,
1.),(1.,1.),(1.,1.),(1.,1.),(1.,1.),(1.,1.),(1.,1.),(1.,1.),(1.,1.),(1.,
1.),(1.,1.),(1.,1.),(1.,1.),(1.,1.),(1.,1.),(1.,1.),(1.,1.),(1.,1.),(1.,
1.),(1.,1.),(1.,1.),(1.,1.),(1.,1.),(1.,1.),(1.,1.),(1.,1.),(1.,1.),(1.,
1.),(1.,1.),(1.,1.),(1.,1.),(1.,1.),(1.,1.),(1.,1.),(1.,1.),(1.,1.),(1.,
1.),(1.,1.),(1.,1.),(1.,1.),(1.,1.),(1.,1.),(1.,1.),(1.,1.),(1.,1.),(1.,
1.),(1.,1.),(1.,1.),(1.,1.),(1.,1.),(1.,1.),(1.,1.),(1.,1.),(1.,1.),(1.,
1.),(1.,1.),(1.,1.),(1.,1.),(1.,1.),(1.,1.),(1.,1.),(1.,1.),(1.,1.),(1.,
1.),(1.,1.),(1.,1.),(1.,1.),(1.,1.),(1.,1.),(1.,1.),(1.,1.),(1.,1.),(1.,
1.),(1.,1.),(1.,1.),(1.,1.),(1.,1.),(1.,1.),(1.,1.),(1.,1.),(1.,1.),(1.,
1.),(1.,1.),(1.,1.),(1.,1.),(1.,1.),(1.,1.),(1.,1.),(1.,1.),(1.,1.),(1.,
1.),(1.,1.),(1.,1.),(1.,1.),(1.,1.),(1.,1.),(1.,1.),(1.,1.),(1.,1.),(1.,
1.),(1.,1.),(1.,1.),(1.,1.),(1.,1.),(1.,1.),(1.,1.),(1.,1.),(1.,1.),(1.,
1.),(1.,1.),(1.,1.),(1.,1.),(1.,1.),(1.,1.),(1.,1.),(1.,1.),(1.,1.),(1.,
1.),(1.,1.)))
REPRESENTATION_ITEM('')
SURFACE()
);
#888=(
BOUNDED_SURFACE()
B_SPLINE_SURFACE(5,1,((#57102,#57103),(#57104,#57105),(#57106,#57107),(#57108,
#57109),(#57110,#57111),(#57112,#57113),(#57114,#57115),(#57116,#57117),
(#57118,#57119),(#57120,#57121),(#57122,#57123),(#57124,#57125),(#57126,
#57127),(#57128,#57129),(#57130,#57131),(#57132,#57133),(#57134,#57135),
(#57136,#57137),(#57138,#57139),(#57140,#57141),(#57142,#57143),(#57144,
#57145),(#57146,#57147),(#57148,#57149),(#57150,#57151),(#57152,#57153),
(#57154,#57155),(#57156,#57157),(#57158,#57159),(#57160,#57161),(#57162,
#57163),(#57164,#57165),(#57166,#57167),(#57168,#57169),(#57170,#57171),
(#57172,#57173),(#57174,#57175),(#57176,#57177),(#57178,#57179),(#57180,
#57181),(#57182,#57183),(#57184,#57185),(#57186,#57187),(#57188,#57189),
(#57190,#57191),(#57192,#57193),(#57194,#57195),(#57196,#57197),(#57198,
#57199),(#57200,#57201),(#57202,#57203),(#57204,#57205),(#57206,#57207),
(#57208,#57209),(#57210,#57211),(#57212,#57213),(#57214,#57215),(#57216,
#57217),(#57218,#57219),(#57220,#57221),(#57222,#57223),(#57224,#57225),
(#57226,#57227),(#57228,#57229),(#57230,#57231),(#57232,#57233),(#57234,
#57235),(#57236,#57237),(#57238,#57239),(#57240,#57241),(#57242,#57243),
(#57244,#57245),(#57246,#57247),(#57248,#57249),(#57250,#57251),(#57252,
#57253),(#57254,#57255),(#57256,#57257),(#57258,#57259),(#57260,#57261),
(#57262,#57263),(#57264,#57265),(#57266,#57267),(#57268,#57269),(#57270,
#57271),(#57272,#57273),(#57274,#57275),(#57276,#57277),(#57278,#57279),
(#57280,#57281),(#57282,#57283),(#57284,#57285),(#57286,#57287),(#57288,
#57289),(#57290,#57291),(#57292,#57293),(#57294,#57295),(#57296,#57297),
(#57298,#57299),(#57300,#57301),(#57302,#57303),(#57304,#57305),(#57306,
#57307),(#57308,#57309),(#57310,#57311),(#57312,#57313),(#57314,#57315),
(#57316,#57317),(#57318,#57319),(#57320,#57321),(#57322,#57323),(#57324,
#57325),(#57326,#57327),(#57328,#57329),(#57330,#57331),(#57332,#57333),
(#57334,#57335),(#57336,#57337),(#57338,#57339),(#57340,#57341),(#57342,
#57343),(#57344,#57345),(#57346,#57347),(#57348,#57349),(#57350,#57351),
(#57352,#57353),(#57354,#57355),(#57356,#57357),(#57358,#57359),(#57360,
#57361),(#57362,#57363),(#57364,#57365),(#57366,#57367),(#57368,#57369),
(#57370,#57371),(#57372,#57373),(#57374,#57375),(#57376,#57377),(#57378,
#57379),(#57380,#57381),(#57382,#57383),(#57384,#57385),(#57386,#57387),
(#57388,#57389),(#57390,#57391),(#57392,#57393),(#57394,#57395),(#57396,
#57397),(#57398,#57399),(#57400,#57401),(#57402,#57403),(#57404,#57405),
(#57406,#57407),(#57408,#57409),(#57410,#57411),(#57412,#57413),(#57414,
#57415),(#57416,#57417),(#57418,#57419),(#57420,#57421),(#57422,#57423),
(#57424,#57425),(#57426,#57427),(#57428,#57429),(#57430,#57431),(#57432,
#57433),(#57434,#57435),(#57436,#57437),(#57438,#57439),(#57440,#57441),
(#57442,#57443),(#57444,#57445),(#57446,#57447),(#57448,#57449),(#57450,
#57451),(#57452,#57453),(#57454,#57455),(#57456,#57457),(#57458,#57459),
(#57460,#57461),(#57462,#57463),(#57464,#57465),(#57466,#57467),(#57468,
#57469),(#57470,#57471),(#57472,#57473),(#57474,#57475),(#57476,#57477),
(#57478,#57479),(#57480,#57481),(#57482,#57483),(#57484,#57485),(#57486,
#57487),(#57488,#57489),(#57490,#57491),(#57492,#57493),(#57494,#57495),
(#57496,#57497),(#57498,#57499),(#57500,#57501),(#57502,#57503),(#57504,
#57505),(#57506,#57507),(#57508,#57509),(#57510,#57511)),.UNSPECIFIED.,
 .F.,.F.,.F.)
B_SPLINE_SURFACE_WITH_KNOTS((6,1,1,1,1,1,1,1,1,1,1,1,1,1,1,1,1,1,1,1,1,
1,1,1,1,1,1,1,1,1,1,1,1,1,1,1,1,1,1,1,1,1,1,1,1,1,1,1,1,1,1,1,1,1,1,1,1,
1,1,1,1,1,1,1,1,1,1,1,1,1,1,1,1,1,1,1,1,1,1,1,1,1,1,1,1,1,1,1,1,1,1,1,1,
1,1,1,1,1,1,1,1,1,1,1,1,1,1,1,1,1,1,1,1,1,1,1,1,1,1,1,1,1,1,1,1,1,1,1,1,
1,1,1,1,1,1,1,1,1,1,1,1,1,1,1,1,1,1,1,1,1,1,1,1,1,1,1,1,1,1,1,1,1,1,1,1,
1,1,1,1,1,1,1,1,1,1,1,1,1,1,1,1,1,1,1,1,1,1,1,1,1,1,1,1,1,1,1,1,1,1,1,6),
(2,2),(0.,0.005,0.01,0.015,0.02,0.025,0.03,0.035,0.04,0.045,0.05,0.055,
0.06,0.065,0.07,0.075,0.08,0.085,0.09,0.095,0.1,0.105,0.11,0.115,0.12,0.125,
0.13,0.135,0.14,0.145,0.15,0.155,0.16,0.165,0.17,0.175,0.18,0.185,0.19,
0.195,0.2,0.205,0.21,0.215,0.22,0.225,0.23,0.235,0.24,0.245,0.25,0.255,
0.26,0.265,0.27,0.275,0.28,0.285,0.29,0.295,0.3,0.305,0.31,0.315,0.32,0.325,
0.33,0.335,0.34,0.345,0.35,0.355,0.36,0.365,0.37,0.375,0.38,0.385,0.39,
0.395,0.4,0.405,0.41,0.415,0.42,0.425,0.43,0.435,0.44,0.445,0.45,0.455,
0.46,0.465,0.47,0.475,0.48,0.485,0.49,0.495,0.5,0.505,0.51,0.515,0.52,0.525,
0.53,0.535,0.54,0.545,0.55,0.555,0.56,0.565,0.57,0.575,0.58,0.585,0.59,
0.595,0.6,0.605,0.61,0.615,0.62,0.625,0.63,0.635,0.64,0.645,0.65,0.655,
0.66,0.665,0.67,0.675,0.68,0.685,0.690000000000001,0.695000000000001,0.700000000000001,
0.705000000000001,0.710000000000001,0.715000000000001,0.720000000000001,
0.725000000000001,0.730000000000001,0.735000000000001,0.740000000000001,
0.745000000000001,0.750000000000001,0.755000000000001,0.760000000000001,
0.765000000000001,0.770000000000001,0.775000000000001,0.780000000000001,
0.785000000000001,0.790000000000001,0.795000000000001,0.800000000000001,
0.805000000000001,0.810000000000001,0.815000000000001,0.820000000000001,
0.825000000000001,0.830000000000001,0.835000000000001,0.840000000000001,
0.845000000000001,0.850000000000001,0.855000000000001,0.860000000000001,
0.865000000000001,0.870000000000001,0.875000000000001,0.880000000000001,
0.885000000000001,0.890000000000001,0.895000000000001,0.900000000000001,
0.905000000000001,0.910000000000001,0.915000000000001,0.920000000000001,
0.925000000000001,0.930000000000001,0.935000000000001,0.940000000000001,
0.945000000000001,0.950000000000001,0.955000000000001,0.960000000000001,
0.965000000000001,0.970000000000001,0.975000000000001,0.980000000000001,
0.985000000000001,0.990000000000001,0.995000000000001,1.),(0.,1.2),
 .UNSPECIFIED.)
GEOMETRIC_REPRESENTATION_ITEM()
RATIONAL_B_SPLINE_SURFACE(((1.,1.),(1.,1.),(1.,1.),(1.,1.),(1.,1.),(1.,
1.),(1.,1.),(1.,1.),(1.,1.),(1.,1.),(1.,1.),(1.,1.),(1.,1.),(1.,1.),(1.,
1.),(1.,1.),(1.,1.),(1.,1.),(1.,1.),(1.,1.),(1.,1.),(1.,1.),(1.,1.),(1.,
1.),(1.,1.),(1.,1.),(1.,1.),(1.,1.),(1.,1.),(1.,1.),(1.,1.),(1.,1.),(1.,
1.),(1.,1.),(1.,1.),(1.,1.),(1.,1.),(1.,1.),(1.,1.),(1.,1.),(1.,1.),(1.,
1.),(1.,1.),(1.,1.),(1.,1.),(1.,1.),(1.,1.),(1.,1.),(1.,1.),(1.,1.),(1.,
1.),(1.,1.),(1.,1.),(1.,1.),(1.,1.),(1.,1.),(1.,1.),(1.,1.),(1.,1.),(1.,
1.),(1.,1.),(1.,1.),(1.,1.),(1.,1.),(1.,1.),(1.,1.),(1.,1.),(1.,1.),(1.,
1.),(1.,1.),(1.,1.),(1.,1.),(1.,1.),(1.,1.),(1.,1.),(1.,1.),(1.,1.),(1.,
1.),(1.,1.),(1.,1.),(1.,1.),(1.,1.),(1.,1.),(1.,1.),(1.,1.),(1.,1.),(1.,
1.),(1.,1.),(1.,1.),(1.,1.),(1.,1.),(1.,1.),(1.,1.),(1.,1.),(1.,1.),(1.,
1.),(1.,1.),(1.,1.),(1.,1.),(1.,1.),(1.,1.),(1.,1.),(1.,1.),(1.,1.),(1.,
1.),(1.,1.),(1.,1.),(1.,1.),(1.,1.),(1.,1.),(1.,1.),(1.,1.),(1.,1.),(1.,
1.),(1.,1.),(1.,1.),(1.,1.),(1.,1.),(1.,1.),(1.,1.),(1.,1.),(1.,1.),(1.,
1.),(1.,1.),(1.,1.),(1.,1.),(1.,1.),(1.,1.),(1.,1.),(1.,1.),(1.,1.),(1.,
1.),(1.,1.),(1.,1.),(1.,1.),(1.,1.),(1.,1.),(1.,1.),(1.,1.),(1.,1.),(1.,
1.),(1.,1.),(1.,1.),(1.,1.),(1.,1.),(1.,1.),(1.,1.),(1.,1.),(1.,1.),(1.,
1.),(1.,1.),(1.,1.),(1.,1.),(1.,1.),(1.,1.),(1.,1.),(1.,1.),(1.,1.),(1.,
1.),(1.,1.),(1.,1.),(1.,1.),(1.,1.),(1.,1.),(1.,1.),(1.,1.),(1.,1.),(1.,
1.),(1.,1.),(1.,1.),(1.,1.),(1.,1.),(1.,1.),(1.,1.),(1.,1.),(1.,1.),(1.,
1.),(1.,1.),(1.,1.),(1.,1.),(1.,1.),(1.,1.),(1.,1.),(1.,1.),(1.,1.),(1.,
1.),(1.,1.),(1.,1.),(1.,1.),(1.,1.),(1.,1.),(1.,1.),(1.,1.),(1.,1.),(1.,
1.),(1.,1.),(1.,1.),(1.,1.),(1.,1.),(1.,1.),(1.,1.),(1.,1.),(1.,1.),(1.,
1.),(1.,1.)))
REPRESENTATION_ITEM('')
SURFACE()
);
#889=(
BOUNDED_SURFACE()
B_SPLINE_SURFACE(5,1,((#57998,#57999),(#58000,#58001),(#58002,#58003),(#58004,
#58005),(#58006,#58007),(#58008,#58009),(#58010,#58011),(#58012,#58013),
(#58014,#58015),(#58016,#58017),(#58018,#58019),(#58020,#58021),(#58022,
#58023),(#58024,#58025),(#58026,#58027),(#58028,#58029),(#58030,#58031),
(#58032,#58033),(#58034,#58035),(#58036,#58037),(#58038,#58039),(#58040,
#58041),(#58042,#58043),(#58044,#58045),(#58046,#58047),(#58048,#58049),
(#58050,#58051),(#58052,#58053),(#58054,#58055),(#58056,#58057),(#58058,
#58059),(#58060,#58061),(#58062,#58063),(#58064,#58065),(#58066,#58067),
(#58068,#58069),(#58070,#58071),(#58072,#58073),(#58074,#58075),(#58076,
#58077),(#58078,#58079),(#58080,#58081),(#58082,#58083),(#58084,#58085),
(#58086,#58087),(#58088,#58089),(#58090,#58091),(#58092,#58093),(#58094,
#58095),(#58096,#58097),(#58098,#58099),(#58100,#58101),(#58102,#58103),
(#58104,#58105),(#58106,#58107),(#58108,#58109),(#58110,#58111),(#58112,
#58113),(#58114,#58115),(#58116,#58117),(#58118,#58119),(#58120,#58121),
(#58122,#58123),(#58124,#58125),(#58126,#58127),(#58128,#58129),(#58130,
#58131),(#58132,#58133),(#58134,#58135),(#58136,#58137),(#58138,#58139),
(#58140,#58141),(#58142,#58143),(#58144,#58145),(#58146,#58147),(#58148,
#58149),(#58150,#58151),(#58152,#58153),(#58154,#58155),(#58156,#58157),
(#58158,#58159),(#58160,#58161),(#58162,#58163),(#58164,#58165),(#58166,
#58167),(#58168,#58169),(#58170,#58171),(#58172,#58173),(#58174,#58175),
(#58176,#58177),(#58178,#58179),(#58180,#58181),(#58182,#58183),(#58184,
#58185),(#58186,#58187),(#58188,#58189),(#58190,#58191),(#58192,#58193),
(#58194,#58195),(#58196,#58197),(#58198,#58199),(#58200,#58201),(#58202,
#58203),(#58204,#58205),(#58206,#58207),(#58208,#58209),(#58210,#58211),
(#58212,#58213),(#58214,#58215),(#58216,#58217),(#58218,#58219),(#58220,
#58221),(#58222,#58223),(#58224,#58225),(#58226,#58227),(#58228,#58229),
(#58230,#58231),(#58232,#58233),(#58234,#58235),(#58236,#58237),(#58238,
#58239),(#58240,#58241),(#58242,#58243),(#58244,#58245),(#58246,#58247),
(#58248,#58249),(#58250,#58251),(#58252,#58253),(#58254,#58255),(#58256,
#58257),(#58258,#58259),(#58260,#58261),(#58262,#58263),(#58264,#58265),
(#58266,#58267),(#58268,#58269),(#58270,#58271),(#58272,#58273),(#58274,
#58275),(#58276,#58277),(#58278,#58279),(#58280,#58281),(#58282,#58283),
(#58284,#58285),(#58286,#58287),(#58288,#58289),(#58290,#58291),(#58292,
#58293),(#58294,#58295),(#58296,#58297),(#58298,#58299),(#58300,#58301),
(#58302,#58303),(#58304,#58305),(#58306,#58307),(#58308,#58309),(#58310,
#58311),(#58312,#58313),(#58314,#58315),(#58316,#58317),(#58318,#58319),
(#58320,#58321),(#58322,#58323),(#58324,#58325),(#58326,#58327),(#58328,
#58329),(#58330,#58331),(#58332,#58333),(#58334,#58335),(#58336,#58337),
(#58338,#58339),(#58340,#58341),(#58342,#58343),(#58344,#58345),(#58346,
#58347),(#58348,#58349),(#58350,#58351),(#58352,#58353),(#58354,#58355),
(#58356,#58357),(#58358,#58359),(#58360,#58361),(#58362,#58363),(#58364,
#58365),(#58366,#58367),(#58368,#58369),(#58370,#58371),(#58372,#58373),
(#58374,#58375),(#58376,#58377),(#58378,#58379),(#58380,#58381),(#58382,
#58383),(#58384,#58385),(#58386,#58387),(#58388,#58389),(#58390,#58391),
(#58392,#58393),(#58394,#58395),(#58396,#58397),(#58398,#58399),(#58400,
#58401),(#58402,#58403),(#58404,#58405),(#58406,#58407)),.UNSPECIFIED.,
 .F.,.F.,.F.)
B_SPLINE_SURFACE_WITH_KNOTS((6,1,1,1,1,1,1,1,1,1,1,1,1,1,1,1,1,1,1,1,1,
1,1,1,1,1,1,1,1,1,1,1,1,1,1,1,1,1,1,1,1,1,1,1,1,1,1,1,1,1,1,1,1,1,1,1,1,
1,1,1,1,1,1,1,1,1,1,1,1,1,1,1,1,1,1,1,1,1,1,1,1,1,1,1,1,1,1,1,1,1,1,1,1,
1,1,1,1,1,1,1,1,1,1,1,1,1,1,1,1,1,1,1,1,1,1,1,1,1,1,1,1,1,1,1,1,1,1,1,1,
1,1,1,1,1,1,1,1,1,1,1,1,1,1,1,1,1,1,1,1,1,1,1,1,1,1,1,1,1,1,1,1,1,1,1,1,
1,1,1,1,1,1,1,1,1,1,1,1,1,1,1,1,1,1,1,1,1,1,1,1,1,1,1,1,1,1,1,1,1,1,1,6),
(2,2),(0.,0.005,0.01,0.015,0.02,0.025,0.03,0.035,0.04,0.045,0.05,0.055,
0.06,0.065,0.07,0.075,0.08,0.085,0.09,0.095,0.1,0.105,0.11,0.115,0.12,0.125,
0.13,0.135,0.14,0.145,0.15,0.155,0.16,0.165,0.17,0.175,0.18,0.185,0.19,
0.195,0.2,0.205,0.21,0.215,0.22,0.225,0.23,0.235,0.24,0.245,0.25,0.255,
0.26,0.265,0.27,0.275,0.28,0.285,0.29,0.295,0.3,0.305,0.31,0.315,0.32,0.325,
0.33,0.335,0.34,0.345,0.35,0.355,0.36,0.365,0.37,0.375,0.38,0.385,0.39,
0.395,0.4,0.405,0.41,0.415,0.42,0.425,0.43,0.435,0.44,0.445,0.45,0.455,
0.46,0.465,0.47,0.475,0.48,0.485,0.49,0.495,0.5,0.505,0.51,0.515,0.52,0.525,
0.53,0.535,0.54,0.545,0.55,0.555,0.56,0.565,0.57,0.575,0.58,0.585,0.59,
0.595,0.6,0.605,0.61,0.615,0.62,0.625,0.63,0.635,0.64,0.645,0.65,0.655,
0.66,0.665,0.67,0.675,0.68,0.685,0.690000000000001,0.695000000000001,0.700000000000001,
0.705000000000001,0.710000000000001,0.715000000000001,0.720000000000001,
0.725000000000001,0.730000000000001,0.735000000000001,0.740000000000001,
0.745000000000001,0.750000000000001,0.755000000000001,0.760000000000001,
0.765000000000001,0.770000000000001,0.775000000000001,0.780000000000001,
0.785000000000001,0.790000000000001,0.795000000000001,0.800000000000001,
0.805000000000001,0.810000000000001,0.815000000000001,0.820000000000001,
0.825000000000001,0.830000000000001,0.835000000000001,0.840000000000001,
0.845000000000001,0.850000000000001,0.855000000000001,0.860000000000001,
0.865000000000001,0.870000000000001,0.875000000000001,0.880000000000001,
0.885000000000001,0.890000000000001,0.895000000000001,0.900000000000001,
0.905000000000001,0.910000000000001,0.915000000000001,0.920000000000001,
0.925000000000001,0.930000000000001,0.935000000000001,0.940000000000001,
0.945000000000001,0.950000000000001,0.955000000000001,0.960000000000001,
0.965000000000001,0.970000000000001,0.975000000000001,0.980000000000001,
0.985000000000001,0.990000000000001,0.995000000000001,1.),(0.,1.2),
 .UNSPECIFIED.)
GEOMETRIC_REPRESENTATION_ITEM()
RATIONAL_B_SPLINE_SURFACE(((1.,1.),(1.,1.),(1.,1.),(1.,1.),(1.,1.),(1.,
1.),(1.,1.),(1.,1.),(1.,1.),(1.,1.),(1.,1.),(1.,1.),(1.,1.),(1.,1.),(1.,
1.),(1.,1.),(1.,1.),(1.,1.),(1.,1.),(1.,1.),(1.,1.),(1.,1.),(1.,1.),(1.,
1.),(1.,1.),(1.,1.),(1.,1.),(1.,1.),(1.,1.),(1.,1.),(1.,1.),(1.,1.),(1.,
1.),(1.,1.),(1.,1.),(1.,1.),(1.,1.),(1.,1.),(1.,1.),(1.,1.),(1.,1.),(1.,
1.),(1.,1.),(1.,1.),(1.,1.),(1.,1.),(1.,1.),(1.,1.),(1.,1.),(1.,1.),(1.,
1.),(1.,1.),(1.,1.),(1.,1.),(1.,1.),(1.,1.),(1.,1.),(1.,1.),(1.,1.),(1.,
1.),(1.,1.),(1.,1.),(1.,1.),(1.,1.),(1.,1.),(1.,1.),(1.,1.),(1.,1.),(1.,
1.),(1.,1.),(1.,1.),(1.,1.),(1.,1.),(1.,1.),(1.,1.),(1.,1.),(1.,1.),(1.,
1.),(1.,1.),(1.,1.),(1.,1.),(1.,1.),(1.,1.),(1.,1.),(1.,1.),(1.,1.),(1.,
1.),(1.,1.),(1.,1.),(1.,1.),(1.,1.),(1.,1.),(1.,1.),(1.,1.),(1.,1.),(1.,
1.),(1.,1.),(1.,1.),(1.,1.),(1.,1.),(1.,1.),(1.,1.),(1.,1.),(1.,1.),(1.,
1.),(1.,1.),(1.,1.),(1.,1.),(1.,1.),(1.,1.),(1.,1.),(1.,1.),(1.,1.),(1.,
1.),(1.,1.),(1.,1.),(1.,1.),(1.,1.),(1.,1.),(1.,1.),(1.,1.),(1.,1.),(1.,
1.),(1.,1.),(1.,1.),(1.,1.),(1.,1.),(1.,1.),(1.,1.),(1.,1.),(1.,1.),(1.,
1.),(1.,1.),(1.,1.),(1.,1.),(1.,1.),(1.,1.),(1.,1.),(1.,1.),(1.,1.),(1.,
1.),(1.,1.),(1.,1.),(1.,1.),(1.,1.),(1.,1.),(1.,1.),(1.,1.),(1.,1.),(1.,
1.),(1.,1.),(1.,1.),(1.,1.),(1.,1.),(1.,1.),(1.,1.),(1.,1.),(1.,1.),(1.,
1.),(1.,1.),(1.,1.),(1.,1.),(1.,1.),(1.,1.),(1.,1.),(1.,1.),(1.,1.),(1.,
1.),(1.,1.),(1.,1.),(1.,1.),(1.,1.),(1.,1.),(1.,1.),(1.,1.),(1.,1.),(1.,
1.),(1.,1.),(1.,1.),(1.,1.),(1.,1.),(1.,1.),(1.,1.),(1.,1.),(1.,1.),(1.,
1.),(1.,1.),(1.,1.),(1.,1.),(1.,1.),(1.,1.),(1.,1.),(1.,1.),(1.,1.),(1.,
1.),(1.,1.),(1.,1.),(1.,1.),(1.,1.),(1.,1.),(1.,1.),(1.,1.),(1.,1.),(1.,
1.),(1.,1.)))
REPRESENTATION_ITEM('')
SURFACE()
);
#890=(
BOUNDED_SURFACE()
B_SPLINE_SURFACE(5,1,((#58894,#58895),(#58896,#58897),(#58898,#58899),(#58900,
#58901),(#58902,#58903),(#58904,#58905),(#58906,#58907),(#58908,#58909),
(#58910,#58911),(#58912,#58913),(#58914,#58915),(#58916,#58917),(#58918,
#58919),(#58920,#58921),(#58922,#58923),(#58924,#58925),(#58926,#58927),
(#58928,#58929),(#58930,#58931),(#58932,#58933),(#58934,#58935),(#58936,
#58937),(#58938,#58939),(#58940,#58941),(#58942,#58943),(#58944,#58945),
(#58946,#58947),(#58948,#58949),(#58950,#58951),(#58952,#58953),(#58954,
#58955),(#58956,#58957),(#58958,#58959),(#58960,#58961),(#58962,#58963),
(#58964,#58965),(#58966,#58967),(#58968,#58969),(#58970,#58971),(#58972,
#58973),(#58974,#58975),(#58976,#58977),(#58978,#58979),(#58980,#58981),
(#58982,#58983),(#58984,#58985),(#58986,#58987),(#58988,#58989),(#58990,
#58991),(#58992,#58993),(#58994,#58995),(#58996,#58997),(#58998,#58999),
(#59000,#59001),(#59002,#59003),(#59004,#59005),(#59006,#59007),(#59008,
#59009),(#59010,#59011),(#59012,#59013),(#59014,#59015),(#59016,#59017),
(#59018,#59019),(#59020,#59021),(#59022,#59023),(#59024,#59025),(#59026,
#59027),(#59028,#59029),(#59030,#59031),(#59032,#59033),(#59034,#59035),
(#59036,#59037),(#59038,#59039),(#59040,#59041),(#59042,#59043),(#59044,
#59045),(#59046,#59047),(#59048,#59049),(#59050,#59051),(#59052,#59053),
(#59054,#59055),(#59056,#59057),(#59058,#59059),(#59060,#59061),(#59062,
#59063),(#59064,#59065),(#59066,#59067),(#59068,#59069),(#59070,#59071),
(#59072,#59073),(#59074,#59075),(#59076,#59077),(#59078,#59079),(#59080,
#59081),(#59082,#59083),(#59084,#59085),(#59086,#59087),(#59088,#59089),
(#59090,#59091),(#59092,#59093),(#59094,#59095),(#59096,#59097),(#59098,
#59099),(#59100,#59101),(#59102,#59103),(#59104,#59105),(#59106,#59107),
(#59108,#59109),(#59110,#59111),(#59112,#59113),(#59114,#59115),(#59116,
#59117),(#59118,#59119),(#59120,#59121),(#59122,#59123),(#59124,#59125),
(#59126,#59127),(#59128,#59129),(#59130,#59131),(#59132,#59133),(#59134,
#59135),(#59136,#59137),(#59138,#59139),(#59140,#59141),(#59142,#59143),
(#59144,#59145),(#59146,#59147),(#59148,#59149),(#59150,#59151),(#59152,
#59153),(#59154,#59155),(#59156,#59157),(#59158,#59159),(#59160,#59161),
(#59162,#59163),(#59164,#59165),(#59166,#59167),(#59168,#59169),(#59170,
#59171),(#59172,#59173),(#59174,#59175),(#59176,#59177),(#59178,#59179),
(#59180,#59181),(#59182,#59183),(#59184,#59185),(#59186,#59187),(#59188,
#59189),(#59190,#59191),(#59192,#59193),(#59194,#59195),(#59196,#59197),
(#59198,#59199),(#59200,#59201),(#59202,#59203),(#59204,#59205),(#59206,
#59207),(#59208,#59209),(#59210,#59211),(#59212,#59213),(#59214,#59215),
(#59216,#59217),(#59218,#59219),(#59220,#59221),(#59222,#59223),(#59224,
#59225),(#59226,#59227),(#59228,#59229),(#59230,#59231),(#59232,#59233),
(#59234,#59235),(#59236,#59237),(#59238,#59239),(#59240,#59241),(#59242,
#59243),(#59244,#59245),(#59246,#59247),(#59248,#59249),(#59250,#59251),
(#59252,#59253),(#59254,#59255),(#59256,#59257),(#59258,#59259),(#59260,
#59261),(#59262,#59263),(#59264,#59265),(#59266,#59267),(#59268,#59269),
(#59270,#59271),(#59272,#59273),(#59274,#59275),(#59276,#59277),(#59278,
#59279),(#59280,#59281),(#59282,#59283),(#59284,#59285),(#59286,#59287),
(#59288,#59289),(#59290,#59291),(#59292,#59293),(#59294,#59295),(#59296,
#59297),(#59298,#59299),(#59300,#59301),(#59302,#59303)),.UNSPECIFIED.,
 .F.,.F.,.F.)
B_SPLINE_SURFACE_WITH_KNOTS((6,1,1,1,1,1,1,1,1,1,1,1,1,1,1,1,1,1,1,1,1,
1,1,1,1,1,1,1,1,1,1,1,1,1,1,1,1,1,1,1,1,1,1,1,1,1,1,1,1,1,1,1,1,1,1,1,1,
1,1,1,1,1,1,1,1,1,1,1,1,1,1,1,1,1,1,1,1,1,1,1,1,1,1,1,1,1,1,1,1,1,1,1,1,
1,1,1,1,1,1,1,1,1,1,1,1,1,1,1,1,1,1,1,1,1,1,1,1,1,1,1,1,1,1,1,1,1,1,1,1,
1,1,1,1,1,1,1,1,1,1,1,1,1,1,1,1,1,1,1,1,1,1,1,1,1,1,1,1,1,1,1,1,1,1,1,1,
1,1,1,1,1,1,1,1,1,1,1,1,1,1,1,1,1,1,1,1,1,1,1,1,1,1,1,1,1,1,1,1,1,1,1,6),
(2,2),(0.,0.005,0.01,0.015,0.02,0.025,0.03,0.035,0.04,0.045,0.05,0.055,
0.06,0.065,0.07,0.075,0.08,0.085,0.09,0.095,0.1,0.105,0.11,0.115,0.12,0.125,
0.13,0.135,0.14,0.145,0.15,0.155,0.16,0.165,0.17,0.175,0.18,0.185,0.19,
0.195,0.2,0.205,0.21,0.215,0.22,0.225,0.23,0.235,0.24,0.245,0.25,0.255,
0.26,0.265,0.27,0.275,0.28,0.285,0.29,0.295,0.3,0.305,0.31,0.315,0.32,0.325,
0.33,0.335,0.34,0.345,0.35,0.355,0.36,0.365,0.37,0.375,0.38,0.385,0.39,
0.395,0.4,0.405,0.41,0.415,0.42,0.425,0.43,0.435,0.44,0.445,0.45,0.455,
0.46,0.465,0.47,0.475,0.48,0.485,0.49,0.495,0.5,0.505,0.51,0.515,0.52,0.525,
0.53,0.535,0.54,0.545,0.55,0.555,0.56,0.565,0.57,0.575,0.58,0.585,0.59,
0.595,0.6,0.605,0.61,0.615,0.62,0.625,0.63,0.635,0.64,0.645,0.65,0.655,
0.66,0.665,0.67,0.675,0.68,0.685,0.690000000000001,0.695000000000001,0.700000000000001,
0.705000000000001,0.710000000000001,0.715000000000001,0.720000000000001,
0.725000000000001,0.730000000000001,0.735000000000001,0.740000000000001,
0.745000000000001,0.750000000000001,0.755000000000001,0.760000000000001,
0.765000000000001,0.770000000000001,0.775000000000001,0.780000000000001,
0.785000000000001,0.790000000000001,0.795000000000001,0.800000000000001,
0.805000000000001,0.810000000000001,0.815000000000001,0.820000000000001,
0.825000000000001,0.830000000000001,0.835000000000001,0.840000000000001,
0.845000000000001,0.850000000000001,0.855000000000001,0.860000000000001,
0.865000000000001,0.870000000000001,0.875000000000001,0.880000000000001,
0.885000000000001,0.890000000000001,0.895000000000001,0.900000000000001,
0.905000000000001,0.910000000000001,0.915000000000001,0.920000000000001,
0.925000000000001,0.930000000000001,0.935000000000001,0.940000000000001,
0.945000000000001,0.950000000000001,0.955000000000001,0.960000000000001,
0.965000000000001,0.970000000000001,0.975000000000001,0.980000000000001,
0.985000000000001,0.990000000000001,0.995000000000001,1.),(0.,1.2),
 .UNSPECIFIED.)
GEOMETRIC_REPRESENTATION_ITEM()
RATIONAL_B_SPLINE_SURFACE(((1.,1.),(1.,1.),(1.,1.),(1.,1.),(1.,1.),(1.,
1.),(1.,1.),(1.,1.),(1.,1.),(1.,1.),(1.,1.),(1.,1.),(1.,1.),(1.,1.),(1.,
1.),(1.,1.),(1.,1.),(1.,1.),(1.,1.),(1.,1.),(1.,1.),(1.,1.),(1.,1.),(1.,
1.),(1.,1.),(1.,1.),(1.,1.),(1.,1.),(1.,1.),(1.,1.),(1.,1.),(1.,1.),(1.,
1.),(1.,1.),(1.,1.),(1.,1.),(1.,1.),(1.,1.),(1.,1.),(1.,1.),(1.,1.),(1.,
1.),(1.,1.),(1.,1.),(1.,1.),(1.,1.),(1.,1.),(1.,1.),(1.,1.),(1.,1.),(1.,
1.),(1.,1.),(1.,1.),(1.,1.),(1.,1.),(1.,1.),(1.,1.),(1.,1.),(1.,1.),(1.,
1.),(1.,1.),(1.,1.),(1.,1.),(1.,1.),(1.,1.),(1.,1.),(1.,1.),(1.,1.),(1.,
1.),(1.,1.),(1.,1.),(1.,1.),(1.,1.),(1.,1.),(1.,1.),(1.,1.),(1.,1.),(1.,
1.),(1.,1.),(1.,1.),(1.,1.),(1.,1.),(1.,1.),(1.,1.),(1.,1.),(1.,1.),(1.,
1.),(1.,1.),(1.,1.),(1.,1.),(1.,1.),(1.,1.),(1.,1.),(1.,1.),(1.,1.),(1.,
1.),(1.,1.),(1.,1.),(1.,1.),(1.,1.),(1.,1.),(1.,1.),(1.,1.),(1.,1.),(1.,
1.),(1.,1.),(1.,1.),(1.,1.),(1.,1.),(1.,1.),(1.,1.),(1.,1.),(1.,1.),(1.,
1.),(1.,1.),(1.,1.),(1.,1.),(1.,1.),(1.,1.),(1.,1.),(1.,1.),(1.,1.),(1.,
1.),(1.,1.),(1.,1.),(1.,1.),(1.,1.),(1.,1.),(1.,1.),(1.,1.),(1.,1.),(1.,
1.),(1.,1.),(1.,1.),(1.,1.),(1.,1.),(1.,1.),(1.,1.),(1.,1.),(1.,1.),(1.,
1.),(1.,1.),(1.,1.),(1.,1.),(1.,1.),(1.,1.),(1.,1.),(1.,1.),(1.,1.),(1.,
1.),(1.,1.),(1.,1.),(1.,1.),(1.,1.),(1.,1.),(1.,1.),(1.,1.),(1.,1.),(1.,
1.),(1.,1.),(1.,1.),(1.,1.),(1.,1.),(1.,1.),(1.,1.),(1.,1.),(1.,1.),(1.,
1.),(1.,1.),(1.,1.),(1.,1.),(1.,1.),(1.,1.),(1.,1.),(1.,1.),(1.,1.),(1.,
1.),(1.,1.),(1.,1.),(1.,1.),(1.,1.),(1.,1.),(1.,1.),(1.,1.),(1.,1.),(1.,
1.),(1.,1.),(1.,1.),(1.,1.),(1.,1.),(1.,1.),(1.,1.),(1.,1.),(1.,1.),(1.,
1.),(1.,1.),(1.,1.),(1.,1.),(1.,1.),(1.,1.),(1.,1.),(1.,1.),(1.,1.),(1.,
1.),(1.,1.)))
REPRESENTATION_ITEM('')
SURFACE()
);
#891=(
BOUNDED_SURFACE()
B_SPLINE_SURFACE(5,1,((#59790,#59791),(#59792,#59793),(#59794,#59795),(#59796,
#59797),(#59798,#59799),(#59800,#59801),(#59802,#59803),(#59804,#59805),
(#59806,#59807),(#59808,#59809),(#59810,#59811),(#59812,#59813),(#59814,
#59815),(#59816,#59817),(#59818,#59819),(#59820,#59821),(#59822,#59823),
(#59824,#59825),(#59826,#59827),(#59828,#59829),(#59830,#59831),(#59832,
#59833),(#59834,#59835),(#59836,#59837),(#59838,#59839),(#59840,#59841),
(#59842,#59843),(#59844,#59845),(#59846,#59847),(#59848,#59849),(#59850,
#59851),(#59852,#59853),(#59854,#59855),(#59856,#59857),(#59858,#59859),
(#59860,#59861),(#59862,#59863),(#59864,#59865),(#59866,#59867),(#59868,
#59869),(#59870,#59871),(#59872,#59873),(#59874,#59875),(#59876,#59877),
(#59878,#59879),(#59880,#59881),(#59882,#59883),(#59884,#59885),(#59886,
#59887),(#59888,#59889),(#59890,#59891),(#59892,#59893),(#59894,#59895),
(#59896,#59897),(#59898,#59899),(#59900,#59901),(#59902,#59903),(#59904,
#59905),(#59906,#59907),(#59908,#59909),(#59910,#59911),(#59912,#59913),
(#59914,#59915),(#59916,#59917),(#59918,#59919),(#59920,#59921),(#59922,
#59923),(#59924,#59925),(#59926,#59927),(#59928,#59929),(#59930,#59931),
(#59932,#59933),(#59934,#59935),(#59936,#59937),(#59938,#59939),(#59940,
#59941),(#59942,#59943),(#59944,#59945),(#59946,#59947),(#59948,#59949),
(#59950,#59951),(#59952,#59953),(#59954,#59955),(#59956,#59957),(#59958,
#59959),(#59960,#59961),(#59962,#59963),(#59964,#59965),(#59966,#59967),
(#59968,#59969),(#59970,#59971),(#59972,#59973),(#59974,#59975),(#59976,
#59977),(#59978,#59979),(#59980,#59981),(#59982,#59983),(#59984,#59985),
(#59986,#59987),(#59988,#59989),(#59990,#59991),(#59992,#59993),(#59994,
#59995),(#59996,#59997),(#59998,#59999),(#60000,#60001),(#60002,#60003),
(#60004,#60005),(#60006,#60007),(#60008,#60009),(#60010,#60011),(#60012,
#60013),(#60014,#60015),(#60016,#60017),(#60018,#60019),(#60020,#60021),
(#60022,#60023),(#60024,#60025),(#60026,#60027),(#60028,#60029),(#60030,
#60031),(#60032,#60033),(#60034,#60035),(#60036,#60037),(#60038,#60039),
(#60040,#60041),(#60042,#60043),(#60044,#60045),(#60046,#60047),(#60048,
#60049),(#60050,#60051),(#60052,#60053),(#60054,#60055),(#60056,#60057),
(#60058,#60059),(#60060,#60061),(#60062,#60063),(#60064,#60065),(#60066,
#60067),(#60068,#60069),(#60070,#60071),(#60072,#60073),(#60074,#60075),
(#60076,#60077),(#60078,#60079),(#60080,#60081),(#60082,#60083),(#60084,
#60085),(#60086,#60087),(#60088,#60089),(#60090,#60091),(#60092,#60093),
(#60094,#60095),(#60096,#60097),(#60098,#60099),(#60100,#60101),(#60102,
#60103),(#60104,#60105),(#60106,#60107),(#60108,#60109),(#60110,#60111),
(#60112,#60113),(#60114,#60115),(#60116,#60117),(#60118,#60119),(#60120,
#60121),(#60122,#60123),(#60124,#60125),(#60126,#60127),(#60128,#60129),
(#60130,#60131),(#60132,#60133),(#60134,#60135),(#60136,#60137),(#60138,
#60139),(#60140,#60141),(#60142,#60143),(#60144,#60145),(#60146,#60147),
(#60148,#60149),(#60150,#60151),(#60152,#60153),(#60154,#60155),(#60156,
#60157),(#60158,#60159),(#60160,#60161),(#60162,#60163),(#60164,#60165),
(#60166,#60167),(#60168,#60169),(#60170,#60171),(#60172,#60173),(#60174,
#60175),(#60176,#60177),(#60178,#60179),(#60180,#60181),(#60182,#60183),
(#60184,#60185),(#60186,#60187),(#60188,#60189),(#60190,#60191),(#60192,
#60193),(#60194,#60195),(#60196,#60197),(#60198,#60199)),.UNSPECIFIED.,
 .F.,.F.,.F.)
B_SPLINE_SURFACE_WITH_KNOTS((6,1,1,1,1,1,1,1,1,1,1,1,1,1,1,1,1,1,1,1,1,
1,1,1,1,1,1,1,1,1,1,1,1,1,1,1,1,1,1,1,1,1,1,1,1,1,1,1,1,1,1,1,1,1,1,1,1,
1,1,1,1,1,1,1,1,1,1,1,1,1,1,1,1,1,1,1,1,1,1,1,1,1,1,1,1,1,1,1,1,1,1,1,1,
1,1,1,1,1,1,1,1,1,1,1,1,1,1,1,1,1,1,1,1,1,1,1,1,1,1,1,1,1,1,1,1,1,1,1,1,
1,1,1,1,1,1,1,1,1,1,1,1,1,1,1,1,1,1,1,1,1,1,1,1,1,1,1,1,1,1,1,1,1,1,1,1,
1,1,1,1,1,1,1,1,1,1,1,1,1,1,1,1,1,1,1,1,1,1,1,1,1,1,1,1,1,1,1,1,1,1,1,6),
(2,2),(0.,0.005,0.01,0.015,0.02,0.025,0.03,0.035,0.04,0.045,0.05,0.055,
0.06,0.065,0.07,0.075,0.08,0.085,0.09,0.095,0.1,0.105,0.11,0.115,0.12,0.125,
0.13,0.135,0.14,0.145,0.15,0.155,0.16,0.165,0.17,0.175,0.18,0.185,0.19,
0.195,0.2,0.205,0.21,0.215,0.22,0.225,0.23,0.235,0.24,0.245,0.25,0.255,
0.26,0.265,0.27,0.275,0.28,0.285,0.29,0.295,0.3,0.305,0.31,0.315,0.32,0.325,
0.33,0.335,0.34,0.345,0.35,0.355,0.36,0.365,0.37,0.375,0.38,0.385,0.39,
0.395,0.4,0.405,0.41,0.415,0.42,0.425,0.43,0.435,0.44,0.445,0.45,0.455,
0.46,0.465,0.47,0.475,0.48,0.485,0.49,0.495,0.5,0.505,0.51,0.515,0.52,0.525,
0.53,0.535,0.54,0.545,0.55,0.555,0.56,0.565,0.57,0.575,0.58,0.585,0.59,
0.595,0.6,0.605,0.61,0.615,0.62,0.625,0.63,0.635,0.64,0.645,0.65,0.655,
0.66,0.665,0.67,0.675,0.68,0.685,0.690000000000001,0.695000000000001,0.700000000000001,
0.705000000000001,0.710000000000001,0.715000000000001,0.720000000000001,
0.725000000000001,0.730000000000001,0.735000000000001,0.740000000000001,
0.745000000000001,0.750000000000001,0.755000000000001,0.760000000000001,
0.765000000000001,0.770000000000001,0.775000000000001,0.780000000000001,
0.785000000000001,0.790000000000001,0.795000000000001,0.800000000000001,
0.805000000000001,0.810000000000001,0.815000000000001,0.820000000000001,
0.825000000000001,0.830000000000001,0.835000000000001,0.840000000000001,
0.845000000000001,0.850000000000001,0.855000000000001,0.860000000000001,
0.865000000000001,0.870000000000001,0.875000000000001,0.880000000000001,
0.885000000000001,0.890000000000001,0.895000000000001,0.900000000000001,
0.905000000000001,0.910000000000001,0.915000000000001,0.920000000000001,
0.925000000000001,0.930000000000001,0.935000000000001,0.940000000000001,
0.945000000000001,0.950000000000001,0.955000000000001,0.960000000000001,
0.965000000000001,0.970000000000001,0.975000000000001,0.980000000000001,
0.985000000000001,0.990000000000001,0.995000000000001,1.),(0.,1.2),
 .UNSPECIFIED.)
GEOMETRIC_REPRESENTATION_ITEM()
RATIONAL_B_SPLINE_SURFACE(((1.,1.),(1.,1.),(1.,1.),(1.,1.),(1.,1.),(1.,
1.),(1.,1.),(1.,1.),(1.,1.),(1.,1.),(1.,1.),(1.,1.),(1.,1.),(1.,1.),(1.,
1.),(1.,1.),(1.,1.),(1.,1.),(1.,1.),(1.,1.),(1.,1.),(1.,1.),(1.,1.),(1.,
1.),(1.,1.),(1.,1.),(1.,1.),(1.,1.),(1.,1.),(1.,1.),(1.,1.),(1.,1.),(1.,
1.),(1.,1.),(1.,1.),(1.,1.),(1.,1.),(1.,1.),(1.,1.),(1.,1.),(1.,1.),(1.,
1.),(1.,1.),(1.,1.),(1.,1.),(1.,1.),(1.,1.),(1.,1.),(1.,1.),(1.,1.),(1.,
1.),(1.,1.),(1.,1.),(1.,1.),(1.,1.),(1.,1.),(1.,1.),(1.,1.),(1.,1.),(1.,
1.),(1.,1.),(1.,1.),(1.,1.),(1.,1.),(1.,1.),(1.,1.),(1.,1.),(1.,1.),(1.,
1.),(1.,1.),(1.,1.),(1.,1.),(1.,1.),(1.,1.),(1.,1.),(1.,1.),(1.,1.),(1.,
1.),(1.,1.),(1.,1.),(1.,1.),(1.,1.),(1.,1.),(1.,1.),(1.,1.),(1.,1.),(1.,
1.),(1.,1.),(1.,1.),(1.,1.),(1.,1.),(1.,1.),(1.,1.),(1.,1.),(1.,1.),(1.,
1.),(1.,1.),(1.,1.),(1.,1.),(1.,1.),(1.,1.),(1.,1.),(1.,1.),(1.,1.),(1.,
1.),(1.,1.),(1.,1.),(1.,1.),(1.,1.),(1.,1.),(1.,1.),(1.,1.),(1.,1.),(1.,
1.),(1.,1.),(1.,1.),(1.,1.),(1.,1.),(1.,1.),(1.,1.),(1.,1.),(1.,1.),(1.,
1.),(1.,1.),(1.,1.),(1.,1.),(1.,1.),(1.,1.),(1.,1.),(1.,1.),(1.,1.),(1.,
1.),(1.,1.),(1.,1.),(1.,1.),(1.,1.),(1.,1.),(1.,1.),(1.,1.),(1.,1.),(1.,
1.),(1.,1.),(1.,1.),(1.,1.),(1.,1.),(1.,1.),(1.,1.),(1.,1.),(1.,1.),(1.,
1.),(1.,1.),(1.,1.),(1.,1.),(1.,1.),(1.,1.),(1.,1.),(1.,1.),(1.,1.),(1.,
1.),(1.,1.),(1.,1.),(1.,1.),(1.,1.),(1.,1.),(1.,1.),(1.,1.),(1.,1.),(1.,
1.),(1.,1.),(1.,1.),(1.,1.),(1.,1.),(1.,1.),(1.,1.),(1.,1.),(1.,1.),(1.,
1.),(1.,1.),(1.,1.),(1.,1.),(1.,1.),(1.,1.),(1.,1.),(1.,1.),(1.,1.),(1.,
1.),(1.,1.),(1.,1.),(1.,1.),(1.,1.),(1.,1.),(1.,1.),(1.,1.),(1.,1.),(1.,
1.),(1.,1.),(1.,1.),(1.,1.),(1.,1.),(1.,1.),(1.,1.),(1.,1.),(1.,1.),(1.,
1.),(1.,1.)))
REPRESENTATION_ITEM('')
SURFACE()
);
#892=(
BOUNDED_SURFACE()
B_SPLINE_SURFACE(5,1,((#60686,#60687),(#60688,#60689),(#60690,#60691),(#60692,
#60693),(#60694,#60695),(#60696,#60697),(#60698,#60699),(#60700,#60701),
(#60702,#60703),(#60704,#60705),(#60706,#60707),(#60708,#60709),(#60710,
#60711),(#60712,#60713),(#60714,#60715),(#60716,#60717),(#60718,#60719),
(#60720,#60721),(#60722,#60723),(#60724,#60725),(#60726,#60727),(#60728,
#60729),(#60730,#60731),(#60732,#60733),(#60734,#60735),(#60736,#60737),
(#60738,#60739),(#60740,#60741),(#60742,#60743),(#60744,#60745),(#60746,
#60747),(#60748,#60749),(#60750,#60751),(#60752,#60753),(#60754,#60755),
(#60756,#60757),(#60758,#60759),(#60760,#60761),(#60762,#60763),(#60764,
#60765),(#60766,#60767),(#60768,#60769),(#60770,#60771),(#60772,#60773),
(#60774,#60775),(#60776,#60777),(#60778,#60779),(#60780,#60781),(#60782,
#60783),(#60784,#60785),(#60786,#60787),(#60788,#60789),(#60790,#60791),
(#60792,#60793),(#60794,#60795),(#60796,#60797),(#60798,#60799),(#60800,
#60801),(#60802,#60803),(#60804,#60805),(#60806,#60807),(#60808,#60809),
(#60810,#60811),(#60812,#60813),(#60814,#60815),(#60816,#60817),(#60818,
#60819),(#60820,#60821),(#60822,#60823),(#60824,#60825),(#60826,#60827),
(#60828,#60829),(#60830,#60831),(#60832,#60833),(#60834,#60835),(#60836,
#60837),(#60838,#60839),(#60840,#60841),(#60842,#60843),(#60844,#60845),
(#60846,#60847),(#60848,#60849),(#60850,#60851),(#60852,#60853),(#60854,
#60855),(#60856,#60857),(#60858,#60859),(#60860,#60861),(#60862,#60863),
(#60864,#60865),(#60866,#60867),(#60868,#60869),(#60870,#60871),(#60872,
#60873),(#60874,#60875),(#60876,#60877),(#60878,#60879),(#60880,#60881),
(#60882,#60883),(#60884,#60885),(#60886,#60887),(#60888,#60889),(#60890,
#60891),(#60892,#60893),(#60894,#60895),(#60896,#60897),(#60898,#60899),
(#60900,#60901),(#60902,#60903),(#60904,#60905),(#60906,#60907),(#60908,
#60909),(#60910,#60911),(#60912,#60913),(#60914,#60915),(#60916,#60917),
(#60918,#60919),(#60920,#60921),(#60922,#60923),(#60924,#60925),(#60926,
#60927),(#60928,#60929),(#60930,#60931),(#60932,#60933),(#60934,#60935),
(#60936,#60937),(#60938,#60939),(#60940,#60941),(#60942,#60943),(#60944,
#60945),(#60946,#60947),(#60948,#60949),(#60950,#60951),(#60952,#60953),
(#60954,#60955),(#60956,#60957),(#60958,#60959),(#60960,#60961),(#60962,
#60963),(#60964,#60965),(#60966,#60967),(#60968,#60969),(#60970,#60971),
(#60972,#60973),(#60974,#60975),(#60976,#60977),(#60978,#60979),(#60980,
#60981),(#60982,#60983),(#60984,#60985),(#60986,#60987),(#60988,#60989),
(#60990,#60991),(#60992,#60993),(#60994,#60995),(#60996,#60997),(#60998,
#60999),(#61000,#61001),(#61002,#61003),(#61004,#61005),(#61006,#61007),
(#61008,#61009),(#61010,#61011),(#61012,#61013),(#61014,#61015),(#61016,
#61017),(#61018,#61019),(#61020,#61021),(#61022,#61023),(#61024,#61025),
(#61026,#61027),(#61028,#61029),(#61030,#61031),(#61032,#61033),(#61034,
#61035),(#61036,#61037),(#61038,#61039),(#61040,#61041),(#61042,#61043),
(#61044,#61045),(#61046,#61047),(#61048,#61049),(#61050,#61051),(#61052,
#61053),(#61054,#61055),(#61056,#61057),(#61058,#61059),(#61060,#61061),
(#61062,#61063),(#61064,#61065),(#61066,#61067),(#61068,#61069),(#61070,
#61071),(#61072,#61073),(#61074,#61075),(#61076,#61077),(#61078,#61079),
(#61080,#61081),(#61082,#61083),(#61084,#61085),(#61086,#61087),(#61088,
#61089),(#61090,#61091),(#61092,#61093),(#61094,#61095)),.UNSPECIFIED.,
 .F.,.F.,.F.)
B_SPLINE_SURFACE_WITH_KNOTS((6,1,1,1,1,1,1,1,1,1,1,1,1,1,1,1,1,1,1,1,1,
1,1,1,1,1,1,1,1,1,1,1,1,1,1,1,1,1,1,1,1,1,1,1,1,1,1,1,1,1,1,1,1,1,1,1,1,
1,1,1,1,1,1,1,1,1,1,1,1,1,1,1,1,1,1,1,1,1,1,1,1,1,1,1,1,1,1,1,1,1,1,1,1,
1,1,1,1,1,1,1,1,1,1,1,1,1,1,1,1,1,1,1,1,1,1,1,1,1,1,1,1,1,1,1,1,1,1,1,1,
1,1,1,1,1,1,1,1,1,1,1,1,1,1,1,1,1,1,1,1,1,1,1,1,1,1,1,1,1,1,1,1,1,1,1,1,
1,1,1,1,1,1,1,1,1,1,1,1,1,1,1,1,1,1,1,1,1,1,1,1,1,1,1,1,1,1,1,1,1,1,1,6),
(2,2),(0.,0.005,0.01,0.015,0.02,0.025,0.03,0.035,0.04,0.045,0.05,0.055,
0.06,0.065,0.07,0.075,0.08,0.085,0.09,0.095,0.1,0.105,0.11,0.115,0.12,0.125,
0.13,0.135,0.14,0.145,0.15,0.155,0.16,0.165,0.17,0.175,0.18,0.185,0.19,
0.195,0.2,0.205,0.21,0.215,0.22,0.225,0.23,0.235,0.24,0.245,0.25,0.255,
0.26,0.265,0.27,0.275,0.28,0.285,0.29,0.295,0.3,0.305,0.31,0.315,0.32,0.325,
0.33,0.335,0.34,0.345,0.35,0.355,0.36,0.365,0.37,0.375,0.38,0.385,0.39,
0.395,0.4,0.405,0.41,0.415,0.42,0.425,0.43,0.435,0.44,0.445,0.45,0.455,
0.46,0.465,0.47,0.475,0.48,0.485,0.49,0.495,0.5,0.505,0.51,0.515,0.52,0.525,
0.53,0.535,0.54,0.545,0.55,0.555,0.56,0.565,0.57,0.575,0.58,0.585,0.59,
0.595,0.6,0.605,0.61,0.615,0.62,0.625,0.63,0.635,0.64,0.645,0.65,0.655,
0.66,0.665,0.67,0.675,0.68,0.685,0.690000000000001,0.695000000000001,0.700000000000001,
0.705000000000001,0.710000000000001,0.715000000000001,0.720000000000001,
0.725000000000001,0.730000000000001,0.735000000000001,0.740000000000001,
0.745000000000001,0.750000000000001,0.755000000000001,0.760000000000001,
0.765000000000001,0.770000000000001,0.775000000000001,0.780000000000001,
0.785000000000001,0.790000000000001,0.795000000000001,0.800000000000001,
0.805000000000001,0.810000000000001,0.815000000000001,0.820000000000001,
0.825000000000001,0.830000000000001,0.835000000000001,0.840000000000001,
0.845000000000001,0.850000000000001,0.855000000000001,0.860000000000001,
0.865000000000001,0.870000000000001,0.875000000000001,0.880000000000001,
0.885000000000001,0.890000000000001,0.895000000000001,0.900000000000001,
0.905000000000001,0.910000000000001,0.915000000000001,0.920000000000001,
0.925000000000001,0.930000000000001,0.935000000000001,0.940000000000001,
0.945000000000001,0.950000000000001,0.955000000000001,0.960000000000001,
0.965000000000001,0.970000000000001,0.975000000000001,0.980000000000001,
0.985000000000001,0.990000000000001,0.995000000000001,1.),(0.,1.2),
 .UNSPECIFIED.)
GEOMETRIC_REPRESENTATION_ITEM()
RATIONAL_B_SPLINE_SURFACE(((1.,1.),(1.,1.),(1.,1.),(1.,1.),(1.,1.),(1.,
1.),(1.,1.),(1.,1.),(1.,1.),(1.,1.),(1.,1.),(1.,1.),(1.,1.),(1.,1.),(1.,
1.),(1.,1.),(1.,1.),(1.,1.),(1.,1.),(1.,1.),(1.,1.),(1.,1.),(1.,1.),(1.,
1.),(1.,1.),(1.,1.),(1.,1.),(1.,1.),(1.,1.),(1.,1.),(1.,1.),(1.,1.),(1.,
1.),(1.,1.),(1.,1.),(1.,1.),(1.,1.),(1.,1.),(1.,1.),(1.,1.),(1.,1.),(1.,
1.),(1.,1.),(1.,1.),(1.,1.),(1.,1.),(1.,1.),(1.,1.),(1.,1.),(1.,1.),(1.,
1.),(1.,1.),(1.,1.),(1.,1.),(1.,1.),(1.,1.),(1.,1.),(1.,1.),(1.,1.),(1.,
1.),(1.,1.),(1.,1.),(1.,1.),(1.,1.),(1.,1.),(1.,1.),(1.,1.),(1.,1.),(1.,
1.),(1.,1.),(1.,1.),(1.,1.),(1.,1.),(1.,1.),(1.,1.),(1.,1.),(1.,1.),(1.,
1.),(1.,1.),(1.,1.),(1.,1.),(1.,1.),(1.,1.),(1.,1.),(1.,1.),(1.,1.),(1.,
1.),(1.,1.),(1.,1.),(1.,1.),(1.,1.),(1.,1.),(1.,1.),(1.,1.),(1.,1.),(1.,
1.),(1.,1.),(1.,1.),(1.,1.),(1.,1.),(1.,1.),(1.,1.),(1.,1.),(1.,1.),(1.,
1.),(1.,1.),(1.,1.),(1.,1.),(1.,1.),(1.,1.),(1.,1.),(1.,1.),(1.,1.),(1.,
1.),(1.,1.),(1.,1.),(1.,1.),(1.,1.),(1.,1.),(1.,1.),(1.,1.),(1.,1.),(1.,
1.),(1.,1.),(1.,1.),(1.,1.),(1.,1.),(1.,1.),(1.,1.),(1.,1.),(1.,1.),(1.,
1.),(1.,1.),(1.,1.),(1.,1.),(1.,1.),(1.,1.),(1.,1.),(1.,1.),(1.,1.),(1.,
1.),(1.,1.),(1.,1.),(1.,1.),(1.,1.),(1.,1.),(1.,1.),(1.,1.),(1.,1.),(1.,
1.),(1.,1.),(1.,1.),(1.,1.),(1.,1.),(1.,1.),(1.,1.),(1.,1.),(1.,1.),(1.,
1.),(1.,1.),(1.,1.),(1.,1.),(1.,1.),(1.,1.),(1.,1.),(1.,1.),(1.,1.),(1.,
1.),(1.,1.),(1.,1.),(1.,1.),(1.,1.),(1.,1.),(1.,1.),(1.,1.),(1.,1.),(1.,
1.),(1.,1.),(1.,1.),(1.,1.),(1.,1.),(1.,1.),(1.,1.),(1.,1.),(1.,1.),(1.,
1.),(1.,1.),(1.,1.),(1.,1.),(1.,1.),(1.,1.),(1.,1.),(1.,1.),(1.,1.),(1.,
1.),(1.,1.),(1.,1.),(1.,1.),(1.,1.),(1.,1.),(1.,1.),(1.,1.),(1.,1.),(1.,
1.),(1.,1.)))
REPRESENTATION_ITEM('')
SURFACE()
);
#893=(
BOUNDED_SURFACE()
B_SPLINE_SURFACE(5,1,((#61582,#61583),(#61584,#61585),(#61586,#61587),(#61588,
#61589),(#61590,#61591),(#61592,#61593),(#61594,#61595),(#61596,#61597),
(#61598,#61599),(#61600,#61601),(#61602,#61603),(#61604,#61605),(#61606,
#61607),(#61608,#61609),(#61610,#61611),(#61612,#61613),(#61614,#61615),
(#61616,#61617),(#61618,#61619),(#61620,#61621),(#61622,#61623),(#61624,
#61625),(#61626,#61627),(#61628,#61629),(#61630,#61631),(#61632,#61633),
(#61634,#61635),(#61636,#61637),(#61638,#61639),(#61640,#61641),(#61642,
#61643),(#61644,#61645),(#61646,#61647),(#61648,#61649),(#61650,#61651),
(#61652,#61653),(#61654,#61655),(#61656,#61657),(#61658,#61659),(#61660,
#61661),(#61662,#61663),(#61664,#61665),(#61666,#61667),(#61668,#61669),
(#61670,#61671),(#61672,#61673),(#61674,#61675),(#61676,#61677),(#61678,
#61679),(#61680,#61681),(#61682,#61683),(#61684,#61685),(#61686,#61687),
(#61688,#61689),(#61690,#61691),(#61692,#61693),(#61694,#61695),(#61696,
#61697),(#61698,#61699),(#61700,#61701),(#61702,#61703),(#61704,#61705),
(#61706,#61707),(#61708,#61709),(#61710,#61711),(#61712,#61713),(#61714,
#61715),(#61716,#61717),(#61718,#61719),(#61720,#61721),(#61722,#61723),
(#61724,#61725),(#61726,#61727),(#61728,#61729),(#61730,#61731),(#61732,
#61733),(#61734,#61735),(#61736,#61737),(#61738,#61739),(#61740,#61741),
(#61742,#61743),(#61744,#61745),(#61746,#61747),(#61748,#61749),(#61750,
#61751),(#61752,#61753),(#61754,#61755),(#61756,#61757),(#61758,#61759),
(#61760,#61761),(#61762,#61763),(#61764,#61765),(#61766,#61767),(#61768,
#61769),(#61770,#61771),(#61772,#61773),(#61774,#61775),(#61776,#61777),
(#61778,#61779),(#61780,#61781),(#61782,#61783),(#61784,#61785),(#61786,
#61787),(#61788,#61789),(#61790,#61791),(#61792,#61793),(#61794,#61795),
(#61796,#61797),(#61798,#61799),(#61800,#61801),(#61802,#61803),(#61804,
#61805),(#61806,#61807),(#61808,#61809),(#61810,#61811),(#61812,#61813),
(#61814,#61815),(#61816,#61817),(#61818,#61819),(#61820,#61821),(#61822,
#61823),(#61824,#61825),(#61826,#61827),(#61828,#61829),(#61830,#61831),
(#61832,#61833),(#61834,#61835),(#61836,#61837),(#61838,#61839),(#61840,
#61841),(#61842,#61843),(#61844,#61845),(#61846,#61847),(#61848,#61849),
(#61850,#61851),(#61852,#61853),(#61854,#61855),(#61856,#61857),(#61858,
#61859),(#61860,#61861),(#61862,#61863),(#61864,#61865),(#61866,#61867),
(#61868,#61869),(#61870,#61871),(#61872,#61873),(#61874,#61875),(#61876,
#61877),(#61878,#61879),(#61880,#61881),(#61882,#61883),(#61884,#61885),
(#61886,#61887),(#61888,#61889),(#61890,#61891),(#61892,#61893),(#61894,
#61895),(#61896,#61897),(#61898,#61899),(#61900,#61901),(#61902,#61903),
(#61904,#61905),(#61906,#61907),(#61908,#61909),(#61910,#61911),(#61912,
#61913),(#61914,#61915),(#61916,#61917),(#61918,#61919),(#61920,#61921),
(#61922,#61923),(#61924,#61925),(#61926,#61927),(#61928,#61929),(#61930,
#61931),(#61932,#61933),(#61934,#61935),(#61936,#61937),(#61938,#61939),
(#61940,#61941),(#61942,#61943),(#61944,#61945),(#61946,#61947),(#61948,
#61949),(#61950,#61951),(#61952,#61953),(#61954,#61955),(#61956,#61957),
(#61958,#61959),(#61960,#61961),(#61962,#61963),(#61964,#61965),(#61966,
#61967),(#61968,#61969),(#61970,#61971),(#61972,#61973),(#61974,#61975),
(#61976,#61977),(#61978,#61979),(#61980,#61981),(#61982,#61983),(#61984,
#61985),(#61986,#61987),(#61988,#61989),(#61990,#61991)),.UNSPECIFIED.,
 .F.,.F.,.F.)
B_SPLINE_SURFACE_WITH_KNOTS((6,1,1,1,1,1,1,1,1,1,1,1,1,1,1,1,1,1,1,1,1,
1,1,1,1,1,1,1,1,1,1,1,1,1,1,1,1,1,1,1,1,1,1,1,1,1,1,1,1,1,1,1,1,1,1,1,1,
1,1,1,1,1,1,1,1,1,1,1,1,1,1,1,1,1,1,1,1,1,1,1,1,1,1,1,1,1,1,1,1,1,1,1,1,
1,1,1,1,1,1,1,1,1,1,1,1,1,1,1,1,1,1,1,1,1,1,1,1,1,1,1,1,1,1,1,1,1,1,1,1,
1,1,1,1,1,1,1,1,1,1,1,1,1,1,1,1,1,1,1,1,1,1,1,1,1,1,1,1,1,1,1,1,1,1,1,1,
1,1,1,1,1,1,1,1,1,1,1,1,1,1,1,1,1,1,1,1,1,1,1,1,1,1,1,1,1,1,1,1,1,1,1,6),
(2,2),(0.,0.005,0.01,0.015,0.02,0.025,0.03,0.035,0.04,0.045,0.05,0.055,
0.06,0.065,0.07,0.075,0.08,0.085,0.09,0.095,0.1,0.105,0.11,0.115,0.12,0.125,
0.13,0.135,0.14,0.145,0.15,0.155,0.16,0.165,0.17,0.175,0.18,0.185,0.19,
0.195,0.2,0.205,0.21,0.215,0.22,0.225,0.23,0.235,0.24,0.245,0.25,0.255,
0.26,0.265,0.27,0.275,0.28,0.285,0.29,0.295,0.3,0.305,0.31,0.315,0.32,0.325,
0.33,0.335,0.34,0.345,0.35,0.355,0.36,0.365,0.37,0.375,0.38,0.385,0.39,
0.395,0.4,0.405,0.41,0.415,0.42,0.425,0.43,0.435,0.44,0.445,0.45,0.455,
0.46,0.465,0.47,0.475,0.48,0.485,0.49,0.495,0.5,0.505,0.51,0.515,0.52,0.525,
0.53,0.535,0.54,0.545,0.55,0.555,0.56,0.565,0.57,0.575,0.58,0.585,0.59,
0.595,0.6,0.605,0.61,0.615,0.62,0.625,0.63,0.635,0.64,0.645,0.65,0.655,
0.66,0.665,0.67,0.675,0.68,0.685,0.690000000000001,0.695000000000001,0.700000000000001,
0.705000000000001,0.710000000000001,0.715000000000001,0.720000000000001,
0.725000000000001,0.730000000000001,0.735000000000001,0.740000000000001,
0.745000000000001,0.750000000000001,0.755000000000001,0.760000000000001,
0.765000000000001,0.770000000000001,0.775000000000001,0.780000000000001,
0.785000000000001,0.790000000000001,0.795000000000001,0.800000000000001,
0.805000000000001,0.810000000000001,0.815000000000001,0.820000000000001,
0.825000000000001,0.830000000000001,0.835000000000001,0.840000000000001,
0.845000000000001,0.850000000000001,0.855000000000001,0.860000000000001,
0.865000000000001,0.870000000000001,0.875000000000001,0.880000000000001,
0.885000000000001,0.890000000000001,0.895000000000001,0.900000000000001,
0.905000000000001,0.910000000000001,0.915000000000001,0.920000000000001,
0.925000000000001,0.930000000000001,0.935000000000001,0.940000000000001,
0.945000000000001,0.950000000000001,0.955000000000001,0.960000000000001,
0.965000000000001,0.970000000000001,0.975000000000001,0.980000000000001,
0.985000000000001,0.990000000000001,0.995000000000001,1.),(0.,1.2),
 .UNSPECIFIED.)
GEOMETRIC_REPRESENTATION_ITEM()
RATIONAL_B_SPLINE_SURFACE(((1.,1.),(1.,1.),(1.,1.),(1.,1.),(1.,1.),(1.,
1.),(1.,1.),(1.,1.),(1.,1.),(1.,1.),(1.,1.),(1.,1.),(1.,1.),(1.,1.),(1.,
1.),(1.,1.),(1.,1.),(1.,1.),(1.,1.),(1.,1.),(1.,1.),(1.,1.),(1.,1.),(1.,
1.),(1.,1.),(1.,1.),(1.,1.),(1.,1.),(1.,1.),(1.,1.),(1.,1.),(1.,1.),(1.,
1.),(1.,1.),(1.,1.),(1.,1.),(1.,1.),(1.,1.),(1.,1.),(1.,1.),(1.,1.),(1.,
1.),(1.,1.),(1.,1.),(1.,1.),(1.,1.),(1.,1.),(1.,1.),(1.,1.),(1.,1.),(1.,
1.),(1.,1.),(1.,1.),(1.,1.),(1.,1.),(1.,1.),(1.,1.),(1.,1.),(1.,1.),(1.,
1.),(1.,1.),(1.,1.),(1.,1.),(1.,1.),(1.,1.),(1.,1.),(1.,1.),(1.,1.),(1.,
1.),(1.,1.),(1.,1.),(1.,1.),(1.,1.),(1.,1.),(1.,1.),(1.,1.),(1.,1.),(1.,
1.),(1.,1.),(1.,1.),(1.,1.),(1.,1.),(1.,1.),(1.,1.),(1.,1.),(1.,1.),(1.,
1.),(1.,1.),(1.,1.),(1.,1.),(1.,1.),(1.,1.),(1.,1.),(1.,1.),(1.,1.),(1.,
1.),(1.,1.),(1.,1.),(1.,1.),(1.,1.),(1.,1.),(1.,1.),(1.,1.),(1.,1.),(1.,
1.),(1.,1.),(1.,1.),(1.,1.),(1.,1.),(1.,1.),(1.,1.),(1.,1.),(1.,1.),(1.,
1.),(1.,1.),(1.,1.),(1.,1.),(1.,1.),(1.,1.),(1.,1.),(1.,1.),(1.,1.),(1.,
1.),(1.,1.),(1.,1.),(1.,1.),(1.,1.),(1.,1.),(1.,1.),(1.,1.),(1.,1.),(1.,
1.),(1.,1.),(1.,1.),(1.,1.),(1.,1.),(1.,1.),(1.,1.),(1.,1.),(1.,1.),(1.,
1.),(1.,1.),(1.,1.),(1.,1.),(1.,1.),(1.,1.),(1.,1.),(1.,1.),(1.,1.),(1.,
1.),(1.,1.),(1.,1.),(1.,1.),(1.,1.),(1.,1.),(1.,1.),(1.,1.),(1.,1.),(1.,
1.),(1.,1.),(1.,1.),(1.,1.),(1.,1.),(1.,1.),(1.,1.),(1.,1.),(1.,1.),(1.,
1.),(1.,1.),(1.,1.),(1.,1.),(1.,1.),(1.,1.),(1.,1.),(1.,1.),(1.,1.),(1.,
1.),(1.,1.),(1.,1.),(1.,1.),(1.,1.),(1.,1.),(1.,1.),(1.,1.),(1.,1.),(1.,
1.),(1.,1.),(1.,1.),(1.,1.),(1.,1.),(1.,1.),(1.,1.),(1.,1.),(1.,1.),(1.,
1.),(1.,1.),(1.,1.),(1.,1.),(1.,1.),(1.,1.),(1.,1.),(1.,1.),(1.,1.),(1.,
1.),(1.,1.)))
REPRESENTATION_ITEM('')
SURFACE()
);
#894=(
BOUNDED_SURFACE()
B_SPLINE_SURFACE(5,1,((#62478,#62479),(#62480,#62481),(#62482,#62483),(#62484,
#62485),(#62486,#62487),(#62488,#62489),(#62490,#62491),(#62492,#62493),
(#62494,#62495),(#62496,#62497),(#62498,#62499),(#62500,#62501),(#62502,
#62503),(#62504,#62505),(#62506,#62507),(#62508,#62509),(#62510,#62511),
(#62512,#62513),(#62514,#62515),(#62516,#62517),(#62518,#62519),(#62520,
#62521),(#62522,#62523),(#62524,#62525),(#62526,#62527),(#62528,#62529),
(#62530,#62531),(#62532,#62533),(#62534,#62535),(#62536,#62537),(#62538,
#62539),(#62540,#62541),(#62542,#62543),(#62544,#62545),(#62546,#62547),
(#62548,#62549),(#62550,#62551),(#62552,#62553),(#62554,#62555),(#62556,
#62557),(#62558,#62559),(#62560,#62561),(#62562,#62563),(#62564,#62565),
(#62566,#62567),(#62568,#62569),(#62570,#62571),(#62572,#62573),(#62574,
#62575),(#62576,#62577),(#62578,#62579),(#62580,#62581),(#62582,#62583),
(#62584,#62585),(#62586,#62587),(#62588,#62589),(#62590,#62591),(#62592,
#62593),(#62594,#62595),(#62596,#62597),(#62598,#62599),(#62600,#62601),
(#62602,#62603),(#62604,#62605),(#62606,#62607),(#62608,#62609),(#62610,
#62611),(#62612,#62613),(#62614,#62615),(#62616,#62617),(#62618,#62619),
(#62620,#62621),(#62622,#62623),(#62624,#62625),(#62626,#62627),(#62628,
#62629),(#62630,#62631),(#62632,#62633),(#62634,#62635),(#62636,#62637),
(#62638,#62639),(#62640,#62641),(#62642,#62643),(#62644,#62645),(#62646,
#62647),(#62648,#62649),(#62650,#62651),(#62652,#62653),(#62654,#62655),
(#62656,#62657),(#62658,#62659),(#62660,#62661),(#62662,#62663),(#62664,
#62665),(#62666,#62667),(#62668,#62669),(#62670,#62671),(#62672,#62673),
(#62674,#62675),(#62676,#62677),(#62678,#62679),(#62680,#62681),(#62682,
#62683),(#62684,#62685),(#62686,#62687),(#62688,#62689),(#62690,#62691),
(#62692,#62693),(#62694,#62695),(#62696,#62697),(#62698,#62699),(#62700,
#62701),(#62702,#62703),(#62704,#62705),(#62706,#62707),(#62708,#62709),
(#62710,#62711),(#62712,#62713),(#62714,#62715),(#62716,#62717),(#62718,
#62719),(#62720,#62721),(#62722,#62723),(#62724,#62725),(#62726,#62727),
(#62728,#62729),(#62730,#62731),(#62732,#62733),(#62734,#62735),(#62736,
#62737),(#62738,#62739),(#62740,#62741),(#62742,#62743),(#62744,#62745),
(#62746,#62747),(#62748,#62749),(#62750,#62751),(#62752,#62753),(#62754,
#62755),(#62756,#62757),(#62758,#62759),(#62760,#62761),(#62762,#62763),
(#62764,#62765),(#62766,#62767),(#62768,#62769),(#62770,#62771),(#62772,
#62773),(#62774,#62775),(#62776,#62777),(#62778,#62779),(#62780,#62781),
(#62782,#62783),(#62784,#62785),(#62786,#62787),(#62788,#62789),(#62790,
#62791),(#62792,#62793),(#62794,#62795),(#62796,#62797),(#62798,#62799),
(#62800,#62801),(#62802,#62803),(#62804,#62805),(#62806,#62807),(#62808,
#62809),(#62810,#62811),(#62812,#62813),(#62814,#62815),(#62816,#62817),
(#62818,#62819),(#62820,#62821),(#62822,#62823),(#62824,#62825),(#62826,
#62827),(#62828,#62829),(#62830,#62831),(#62832,#62833),(#62834,#62835),
(#62836,#62837),(#62838,#62839),(#62840,#62841),(#62842,#62843),(#62844,
#62845),(#62846,#62847),(#62848,#62849),(#62850,#62851),(#62852,#62853),
(#62854,#62855),(#62856,#62857),(#62858,#62859),(#62860,#62861),(#62862,
#62863),(#62864,#62865),(#62866,#62867),(#62868,#62869),(#62870,#62871),
(#62872,#62873),(#62874,#62875),(#62876,#62877),(#62878,#62879),(#62880,
#62881),(#62882,#62883),(#62884,#62885),(#62886,#62887)),.UNSPECIFIED.,
 .F.,.F.,.F.)
B_SPLINE_SURFACE_WITH_KNOTS((6,1,1,1,1,1,1,1,1,1,1,1,1,1,1,1,1,1,1,1,1,
1,1,1,1,1,1,1,1,1,1,1,1,1,1,1,1,1,1,1,1,1,1,1,1,1,1,1,1,1,1,1,1,1,1,1,1,
1,1,1,1,1,1,1,1,1,1,1,1,1,1,1,1,1,1,1,1,1,1,1,1,1,1,1,1,1,1,1,1,1,1,1,1,
1,1,1,1,1,1,1,1,1,1,1,1,1,1,1,1,1,1,1,1,1,1,1,1,1,1,1,1,1,1,1,1,1,1,1,1,
1,1,1,1,1,1,1,1,1,1,1,1,1,1,1,1,1,1,1,1,1,1,1,1,1,1,1,1,1,1,1,1,1,1,1,1,
1,1,1,1,1,1,1,1,1,1,1,1,1,1,1,1,1,1,1,1,1,1,1,1,1,1,1,1,1,1,1,1,1,1,1,6),
(2,2),(0.,0.005,0.01,0.015,0.02,0.025,0.03,0.035,0.04,0.045,0.05,0.055,
0.06,0.065,0.07,0.075,0.08,0.085,0.09,0.095,0.1,0.105,0.11,0.115,0.12,0.125,
0.13,0.135,0.14,0.145,0.15,0.155,0.16,0.165,0.17,0.175,0.18,0.185,0.19,
0.195,0.2,0.205,0.21,0.215,0.22,0.225,0.23,0.235,0.24,0.245,0.25,0.255,
0.26,0.265,0.27,0.275,0.28,0.285,0.29,0.295,0.3,0.305,0.31,0.315,0.32,0.325,
0.33,0.335,0.34,0.345,0.35,0.355,0.36,0.365,0.37,0.375,0.38,0.385,0.39,
0.395,0.4,0.405,0.41,0.415,0.42,0.425,0.43,0.435,0.44,0.445,0.45,0.455,
0.46,0.465,0.47,0.475,0.48,0.485,0.49,0.495,0.5,0.505,0.51,0.515,0.52,0.525,
0.53,0.535,0.54,0.545,0.55,0.555,0.56,0.565,0.57,0.575,0.58,0.585,0.59,
0.595,0.6,0.605,0.61,0.615,0.62,0.625,0.63,0.635,0.64,0.645,0.65,0.655,
0.66,0.665,0.67,0.675,0.68,0.685,0.690000000000001,0.695000000000001,0.700000000000001,
0.705000000000001,0.710000000000001,0.715000000000001,0.720000000000001,
0.725000000000001,0.730000000000001,0.735000000000001,0.740000000000001,
0.745000000000001,0.750000000000001,0.755000000000001,0.760000000000001,
0.765000000000001,0.770000000000001,0.775000000000001,0.780000000000001,
0.785000000000001,0.790000000000001,0.795000000000001,0.800000000000001,
0.805000000000001,0.810000000000001,0.815000000000001,0.820000000000001,
0.825000000000001,0.830000000000001,0.835000000000001,0.840000000000001,
0.845000000000001,0.850000000000001,0.855000000000001,0.860000000000001,
0.865000000000001,0.870000000000001,0.875000000000001,0.880000000000001,
0.885000000000001,0.890000000000001,0.895000000000001,0.900000000000001,
0.905000000000001,0.910000000000001,0.915000000000001,0.920000000000001,
0.925000000000001,0.930000000000001,0.935000000000001,0.940000000000001,
0.945000000000001,0.950000000000001,0.955000000000001,0.960000000000001,
0.965000000000001,0.970000000000001,0.975000000000001,0.980000000000001,
0.985000000000001,0.990000000000001,0.995000000000001,1.),(0.,1.2),
 .UNSPECIFIED.)
GEOMETRIC_REPRESENTATION_ITEM()
RATIONAL_B_SPLINE_SURFACE(((1.,1.),(1.,1.),(1.,1.),(1.,1.),(1.,1.),(1.,
1.),(1.,1.),(1.,1.),(1.,1.),(1.,1.),(1.,1.),(1.,1.),(1.,1.),(1.,1.),(1.,
1.),(1.,1.),(1.,1.),(1.,1.),(1.,1.),(1.,1.),(1.,1.),(1.,1.),(1.,1.),(1.,
1.),(1.,1.),(1.,1.),(1.,1.),(1.,1.),(1.,1.),(1.,1.),(1.,1.),(1.,1.),(1.,
1.),(1.,1.),(1.,1.),(1.,1.),(1.,1.),(1.,1.),(1.,1.),(1.,1.),(1.,1.),(1.,
1.),(1.,1.),(1.,1.),(1.,1.),(1.,1.),(1.,1.),(1.,1.),(1.,1.),(1.,1.),(1.,
1.),(1.,1.),(1.,1.),(1.,1.),(1.,1.),(1.,1.),(1.,1.),(1.,1.),(1.,1.),(1.,
1.),(1.,1.),(1.,1.),(1.,1.),(1.,1.),(1.,1.),(1.,1.),(1.,1.),(1.,1.),(1.,
1.),(1.,1.),(1.,1.),(1.,1.),(1.,1.),(1.,1.),(1.,1.),(1.,1.),(1.,1.),(1.,
1.),(1.,1.),(1.,1.),(1.,1.),(1.,1.),(1.,1.),(1.,1.),(1.,1.),(1.,1.),(1.,
1.),(1.,1.),(1.,1.),(1.,1.),(1.,1.),(1.,1.),(1.,1.),(1.,1.),(1.,1.),(1.,
1.),(1.,1.),(1.,1.),(1.,1.),(1.,1.),(1.,1.),(1.,1.),(1.,1.),(1.,1.),(1.,
1.),(1.,1.),(1.,1.),(1.,1.),(1.,1.),(1.,1.),(1.,1.),(1.,1.),(1.,1.),(1.,
1.),(1.,1.),(1.,1.),(1.,1.),(1.,1.),(1.,1.),(1.,1.),(1.,1.),(1.,1.),(1.,
1.),(1.,1.),(1.,1.),(1.,1.),(1.,1.),(1.,1.),(1.,1.),(1.,1.),(1.,1.),(1.,
1.),(1.,1.),(1.,1.),(1.,1.),(1.,1.),(1.,1.),(1.,1.),(1.,1.),(1.,1.),(1.,
1.),(1.,1.),(1.,1.),(1.,1.),(1.,1.),(1.,1.),(1.,1.),(1.,1.),(1.,1.),(1.,
1.),(1.,1.),(1.,1.),(1.,1.),(1.,1.),(1.,1.),(1.,1.),(1.,1.),(1.,1.),(1.,
1.),(1.,1.),(1.,1.),(1.,1.),(1.,1.),(1.,1.),(1.,1.),(1.,1.),(1.,1.),(1.,
1.),(1.,1.),(1.,1.),(1.,1.),(1.,1.),(1.,1.),(1.,1.),(1.,1.),(1.,1.),(1.,
1.),(1.,1.),(1.,1.),(1.,1.),(1.,1.),(1.,1.),(1.,1.),(1.,1.),(1.,1.),(1.,
1.),(1.,1.),(1.,1.),(1.,1.),(1.,1.),(1.,1.),(1.,1.),(1.,1.),(1.,1.),(1.,
1.),(1.,1.),(1.,1.),(1.,1.),(1.,1.),(1.,1.),(1.,1.),(1.,1.),(1.,1.),(1.,
1.),(1.,1.)))
REPRESENTATION_ITEM('')
SURFACE()
);
#895=(
BOUNDED_SURFACE()
B_SPLINE_SURFACE(5,1,((#63374,#63375),(#63376,#63377),(#63378,#63379),(#63380,
#63381),(#63382,#63383),(#63384,#63385),(#63386,#63387),(#63388,#63389),
(#63390,#63391),(#63392,#63393),(#63394,#63395),(#63396,#63397),(#63398,
#63399),(#63400,#63401),(#63402,#63403),(#63404,#63405),(#63406,#63407),
(#63408,#63409),(#63410,#63411),(#63412,#63413),(#63414,#63415),(#63416,
#63417),(#63418,#63419),(#63420,#63421),(#63422,#63423),(#63424,#63425),
(#63426,#63427),(#63428,#63429),(#63430,#63431),(#63432,#63433),(#63434,
#63435),(#63436,#63437),(#63438,#63439),(#63440,#63441),(#63442,#63443),
(#63444,#63445),(#63446,#63447),(#63448,#63449),(#63450,#63451),(#63452,
#63453),(#63454,#63455),(#63456,#63457),(#63458,#63459),(#63460,#63461),
(#63462,#63463),(#63464,#63465),(#63466,#63467),(#63468,#63469),(#63470,
#63471),(#63472,#63473),(#63474,#63475),(#63476,#63477),(#63478,#63479),
(#63480,#63481),(#63482,#63483),(#63484,#63485),(#63486,#63487),(#63488,
#63489),(#63490,#63491),(#63492,#63493),(#63494,#63495),(#63496,#63497),
(#63498,#63499),(#63500,#63501),(#63502,#63503),(#63504,#63505),(#63506,
#63507),(#63508,#63509),(#63510,#63511),(#63512,#63513),(#63514,#63515),
(#63516,#63517),(#63518,#63519),(#63520,#63521),(#63522,#63523),(#63524,
#63525),(#63526,#63527),(#63528,#63529),(#63530,#63531),(#63532,#63533),
(#63534,#63535),(#63536,#63537),(#63538,#63539),(#63540,#63541),(#63542,
#63543),(#63544,#63545),(#63546,#63547),(#63548,#63549),(#63550,#63551),
(#63552,#63553),(#63554,#63555),(#63556,#63557),(#63558,#63559),(#63560,
#63561),(#63562,#63563),(#63564,#63565),(#63566,#63567),(#63568,#63569),
(#63570,#63571),(#63572,#63573),(#63574,#63575),(#63576,#63577),(#63578,
#63579),(#63580,#63581),(#63582,#63583),(#63584,#63585),(#63586,#63587),
(#63588,#63589),(#63590,#63591),(#63592,#63593),(#63594,#63595),(#63596,
#63597),(#63598,#63599),(#63600,#63601),(#63602,#63603),(#63604,#63605),
(#63606,#63607),(#63608,#63609),(#63610,#63611),(#63612,#63613),(#63614,
#63615),(#63616,#63617),(#63618,#63619),(#63620,#63621),(#63622,#63623),
(#63624,#63625),(#63626,#63627),(#63628,#63629),(#63630,#63631),(#63632,
#63633),(#63634,#63635),(#63636,#63637),(#63638,#63639),(#63640,#63641),
(#63642,#63643),(#63644,#63645),(#63646,#63647),(#63648,#63649),(#63650,
#63651),(#63652,#63653),(#63654,#63655),(#63656,#63657),(#63658,#63659),
(#63660,#63661),(#63662,#63663),(#63664,#63665),(#63666,#63667),(#63668,
#63669),(#63670,#63671),(#63672,#63673),(#63674,#63675),(#63676,#63677),
(#63678,#63679),(#63680,#63681),(#63682,#63683),(#63684,#63685),(#63686,
#63687),(#63688,#63689),(#63690,#63691),(#63692,#63693),(#63694,#63695),
(#63696,#63697),(#63698,#63699),(#63700,#63701),(#63702,#63703),(#63704,
#63705),(#63706,#63707),(#63708,#63709),(#63710,#63711),(#63712,#63713),
(#63714,#63715),(#63716,#63717),(#63718,#63719),(#63720,#63721),(#63722,
#63723),(#63724,#63725),(#63726,#63727),(#63728,#63729),(#63730,#63731),
(#63732,#63733),(#63734,#63735),(#63736,#63737),(#63738,#63739),(#63740,
#63741),(#63742,#63743),(#63744,#63745),(#63746,#63747),(#63748,#63749),
(#63750,#63751),(#63752,#63753),(#63754,#63755),(#63756,#63757),(#63758,
#63759),(#63760,#63761),(#63762,#63763),(#63764,#63765),(#63766,#63767),
(#63768,#63769),(#63770,#63771),(#63772,#63773),(#63774,#63775),(#63776,
#63777),(#63778,#63779),(#63780,#63781),(#63782,#63783)),.UNSPECIFIED.,
 .F.,.F.,.F.)
B_SPLINE_SURFACE_WITH_KNOTS((6,1,1,1,1,1,1,1,1,1,1,1,1,1,1,1,1,1,1,1,1,
1,1,1,1,1,1,1,1,1,1,1,1,1,1,1,1,1,1,1,1,1,1,1,1,1,1,1,1,1,1,1,1,1,1,1,1,
1,1,1,1,1,1,1,1,1,1,1,1,1,1,1,1,1,1,1,1,1,1,1,1,1,1,1,1,1,1,1,1,1,1,1,1,
1,1,1,1,1,1,1,1,1,1,1,1,1,1,1,1,1,1,1,1,1,1,1,1,1,1,1,1,1,1,1,1,1,1,1,1,
1,1,1,1,1,1,1,1,1,1,1,1,1,1,1,1,1,1,1,1,1,1,1,1,1,1,1,1,1,1,1,1,1,1,1,1,
1,1,1,1,1,1,1,1,1,1,1,1,1,1,1,1,1,1,1,1,1,1,1,1,1,1,1,1,1,1,1,1,1,1,1,6),
(2,2),(0.,0.005,0.01,0.015,0.02,0.025,0.03,0.035,0.04,0.045,0.05,0.055,
0.06,0.065,0.07,0.075,0.08,0.085,0.09,0.095,0.1,0.105,0.11,0.115,0.12,0.125,
0.13,0.135,0.14,0.145,0.15,0.155,0.16,0.165,0.17,0.175,0.18,0.185,0.19,
0.195,0.2,0.205,0.21,0.215,0.22,0.225,0.23,0.235,0.24,0.245,0.25,0.255,
0.26,0.265,0.27,0.275,0.28,0.285,0.29,0.295,0.3,0.305,0.31,0.315,0.32,0.325,
0.33,0.335,0.34,0.345,0.35,0.355,0.36,0.365,0.37,0.375,0.38,0.385,0.39,
0.395,0.4,0.405,0.41,0.415,0.42,0.425,0.43,0.435,0.44,0.445,0.45,0.455,
0.46,0.465,0.47,0.475,0.48,0.485,0.49,0.495,0.5,0.505,0.51,0.515,0.52,0.525,
0.53,0.535,0.54,0.545,0.55,0.555,0.56,0.565,0.57,0.575,0.58,0.585,0.59,
0.595,0.6,0.605,0.61,0.615,0.62,0.625,0.63,0.635,0.64,0.645,0.65,0.655,
0.66,0.665,0.67,0.675,0.68,0.685,0.690000000000001,0.695000000000001,0.700000000000001,
0.705000000000001,0.710000000000001,0.715000000000001,0.720000000000001,
0.725000000000001,0.730000000000001,0.735000000000001,0.740000000000001,
0.745000000000001,0.750000000000001,0.755000000000001,0.760000000000001,
0.765000000000001,0.770000000000001,0.775000000000001,0.780000000000001,
0.785000000000001,0.790000000000001,0.795000000000001,0.800000000000001,
0.805000000000001,0.810000000000001,0.815000000000001,0.820000000000001,
0.825000000000001,0.830000000000001,0.835000000000001,0.840000000000001,
0.845000000000001,0.850000000000001,0.855000000000001,0.860000000000001,
0.865000000000001,0.870000000000001,0.875000000000001,0.880000000000001,
0.885000000000001,0.890000000000001,0.895000000000001,0.900000000000001,
0.905000000000001,0.910000000000001,0.915000000000001,0.920000000000001,
0.925000000000001,0.930000000000001,0.935000000000001,0.940000000000001,
0.945000000000001,0.950000000000001,0.955000000000001,0.960000000000001,
0.965000000000001,0.970000000000001,0.975000000000001,0.980000000000001,
0.985000000000001,0.990000000000001,0.995000000000001,1.),(0.,1.2),
 .UNSPECIFIED.)
GEOMETRIC_REPRESENTATION_ITEM()
RATIONAL_B_SPLINE_SURFACE(((1.,1.),(1.,1.),(1.,1.),(1.,1.),(1.,1.),(1.,
1.),(1.,1.),(1.,1.),(1.,1.),(1.,1.),(1.,1.),(1.,1.),(1.,1.),(1.,1.),(1.,
1.),(1.,1.),(1.,1.),(1.,1.),(1.,1.),(1.,1.),(1.,1.),(1.,1.),(1.,1.),(1.,
1.),(1.,1.),(1.,1.),(1.,1.),(1.,1.),(1.,1.),(1.,1.),(1.,1.),(1.,1.),(1.,
1.),(1.,1.),(1.,1.),(1.,1.),(1.,1.),(1.,1.),(1.,1.),(1.,1.),(1.,1.),(1.,
1.),(1.,1.),(1.,1.),(1.,1.),(1.,1.),(1.,1.),(1.,1.),(1.,1.),(1.,1.),(1.,
1.),(1.,1.),(1.,1.),(1.,1.),(1.,1.),(1.,1.),(1.,1.),(1.,1.),(1.,1.),(1.,
1.),(1.,1.),(1.,1.),(1.,1.),(1.,1.),(1.,1.),(1.,1.),(1.,1.),(1.,1.),(1.,
1.),(1.,1.),(1.,1.),(1.,1.),(1.,1.),(1.,1.),(1.,1.),(1.,1.),(1.,1.),(1.,
1.),(1.,1.),(1.,1.),(1.,1.),(1.,1.),(1.,1.),(1.,1.),(1.,1.),(1.,1.),(1.,
1.),(1.,1.),(1.,1.),(1.,1.),(1.,1.),(1.,1.),(1.,1.),(1.,1.),(1.,1.),(1.,
1.),(1.,1.),(1.,1.),(1.,1.),(1.,1.),(1.,1.),(1.,1.),(1.,1.),(1.,1.),(1.,
1.),(1.,1.),(1.,1.),(1.,1.),(1.,1.),(1.,1.),(1.,1.),(1.,1.),(1.,1.),(1.,
1.),(1.,1.),(1.,1.),(1.,1.),(1.,1.),(1.,1.),(1.,1.),(1.,1.),(1.,1.),(1.,
1.),(1.,1.),(1.,1.),(1.,1.),(1.,1.),(1.,1.),(1.,1.),(1.,1.),(1.,1.),(1.,
1.),(1.,1.),(1.,1.),(1.,1.),(1.,1.),(1.,1.),(1.,1.),(1.,1.),(1.,1.),(1.,
1.),(1.,1.),(1.,1.),(1.,1.),(1.,1.),(1.,1.),(1.,1.),(1.,1.),(1.,1.),(1.,
1.),(1.,1.),(1.,1.),(1.,1.),(1.,1.),(1.,1.),(1.,1.),(1.,1.),(1.,1.),(1.,
1.),(1.,1.),(1.,1.),(1.,1.),(1.,1.),(1.,1.),(1.,1.),(1.,1.),(1.,1.),(1.,
1.),(1.,1.),(1.,1.),(1.,1.),(1.,1.),(1.,1.),(1.,1.),(1.,1.),(1.,1.),(1.,
1.),(1.,1.),(1.,1.),(1.,1.),(1.,1.),(1.,1.),(1.,1.),(1.,1.),(1.,1.),(1.,
1.),(1.,1.),(1.,1.),(1.,1.),(1.,1.),(1.,1.),(1.,1.),(1.,1.),(1.,1.),(1.,
1.),(1.,1.),(1.,1.),(1.,1.),(1.,1.),(1.,1.),(1.,1.),(1.,1.),(1.,1.),(1.,
1.),(1.,1.)))
REPRESENTATION_ITEM('')
SURFACE()
);
#896=(
BOUNDED_SURFACE()
B_SPLINE_SURFACE(5,1,((#64270,#64271),(#64272,#64273),(#64274,#64275),(#64276,
#64277),(#64278,#64279),(#64280,#64281),(#64282,#64283),(#64284,#64285),
(#64286,#64287),(#64288,#64289),(#64290,#64291),(#64292,#64293),(#64294,
#64295),(#64296,#64297),(#64298,#64299),(#64300,#64301),(#64302,#64303),
(#64304,#64305),(#64306,#64307),(#64308,#64309),(#64310,#64311),(#64312,
#64313),(#64314,#64315),(#64316,#64317),(#64318,#64319),(#64320,#64321),
(#64322,#64323),(#64324,#64325),(#64326,#64327),(#64328,#64329),(#64330,
#64331),(#64332,#64333),(#64334,#64335),(#64336,#64337),(#64338,#64339),
(#64340,#64341),(#64342,#64343),(#64344,#64345),(#64346,#64347),(#64348,
#64349),(#64350,#64351),(#64352,#64353),(#64354,#64355),(#64356,#64357),
(#64358,#64359),(#64360,#64361),(#64362,#64363),(#64364,#64365),(#64366,
#64367),(#64368,#64369),(#64370,#64371),(#64372,#64373),(#64374,#64375),
(#64376,#64377),(#64378,#64379),(#64380,#64381),(#64382,#64383),(#64384,
#64385),(#64386,#64387),(#64388,#64389),(#64390,#64391),(#64392,#64393),
(#64394,#64395),(#64396,#64397),(#64398,#64399),(#64400,#64401),(#64402,
#64403),(#64404,#64405),(#64406,#64407),(#64408,#64409),(#64410,#64411),
(#64412,#64413),(#64414,#64415),(#64416,#64417),(#64418,#64419),(#64420,
#64421),(#64422,#64423),(#64424,#64425),(#64426,#64427),(#64428,#64429),
(#64430,#64431),(#64432,#64433),(#64434,#64435),(#64436,#64437),(#64438,
#64439),(#64440,#64441),(#64442,#64443),(#64444,#64445),(#64446,#64447),
(#64448,#64449),(#64450,#64451),(#64452,#64453),(#64454,#64455),(#64456,
#64457),(#64458,#64459),(#64460,#64461),(#64462,#64463),(#64464,#64465),
(#64466,#64467),(#64468,#64469),(#64470,#64471),(#64472,#64473),(#64474,
#64475),(#64476,#64477),(#64478,#64479),(#64480,#64481),(#64482,#64483),
(#64484,#64485),(#64486,#64487),(#64488,#64489),(#64490,#64491),(#64492,
#64493),(#64494,#64495),(#64496,#64497),(#64498,#64499),(#64500,#64501),
(#64502,#64503),(#64504,#64505),(#64506,#64507),(#64508,#64509),(#64510,
#64511),(#64512,#64513),(#64514,#64515),(#64516,#64517),(#64518,#64519),
(#64520,#64521),(#64522,#64523),(#64524,#64525),(#64526,#64527),(#64528,
#64529),(#64530,#64531),(#64532,#64533),(#64534,#64535),(#64536,#64537),
(#64538,#64539),(#64540,#64541),(#64542,#64543),(#64544,#64545),(#64546,
#64547),(#64548,#64549),(#64550,#64551),(#64552,#64553),(#64554,#64555),
(#64556,#64557),(#64558,#64559),(#64560,#64561),(#64562,#64563),(#64564,
#64565),(#64566,#64567),(#64568,#64569),(#64570,#64571),(#64572,#64573),
(#64574,#64575),(#64576,#64577),(#64578,#64579),(#64580,#64581),(#64582,
#64583),(#64584,#64585),(#64586,#64587),(#64588,#64589),(#64590,#64591),
(#64592,#64593),(#64594,#64595),(#64596,#64597),(#64598,#64599),(#64600,
#64601),(#64602,#64603),(#64604,#64605),(#64606,#64607),(#64608,#64609),
(#64610,#64611),(#64612,#64613),(#64614,#64615),(#64616,#64617),(#64618,
#64619),(#64620,#64621),(#64622,#64623),(#64624,#64625),(#64626,#64627),
(#64628,#64629),(#64630,#64631),(#64632,#64633),(#64634,#64635),(#64636,
#64637),(#64638,#64639),(#64640,#64641),(#64642,#64643),(#64644,#64645),
(#64646,#64647),(#64648,#64649),(#64650,#64651),(#64652,#64653),(#64654,
#64655),(#64656,#64657),(#64658,#64659),(#64660,#64661),(#64662,#64663),
(#64664,#64665),(#64666,#64667),(#64668,#64669),(#64670,#64671),(#64672,
#64673),(#64674,#64675),(#64676,#64677),(#64678,#64679)),.UNSPECIFIED.,
 .F.,.F.,.F.)
B_SPLINE_SURFACE_WITH_KNOTS((6,1,1,1,1,1,1,1,1,1,1,1,1,1,1,1,1,1,1,1,1,
1,1,1,1,1,1,1,1,1,1,1,1,1,1,1,1,1,1,1,1,1,1,1,1,1,1,1,1,1,1,1,1,1,1,1,1,
1,1,1,1,1,1,1,1,1,1,1,1,1,1,1,1,1,1,1,1,1,1,1,1,1,1,1,1,1,1,1,1,1,1,1,1,
1,1,1,1,1,1,1,1,1,1,1,1,1,1,1,1,1,1,1,1,1,1,1,1,1,1,1,1,1,1,1,1,1,1,1,1,
1,1,1,1,1,1,1,1,1,1,1,1,1,1,1,1,1,1,1,1,1,1,1,1,1,1,1,1,1,1,1,1,1,1,1,1,
1,1,1,1,1,1,1,1,1,1,1,1,1,1,1,1,1,1,1,1,1,1,1,1,1,1,1,1,1,1,1,1,1,1,1,6),
(2,2),(0.,0.005,0.01,0.015,0.02,0.025,0.03,0.035,0.04,0.045,0.05,0.055,
0.06,0.065,0.07,0.075,0.08,0.085,0.09,0.095,0.1,0.105,0.11,0.115,0.12,0.125,
0.13,0.135,0.14,0.145,0.15,0.155,0.16,0.165,0.17,0.175,0.18,0.185,0.19,
0.195,0.2,0.205,0.21,0.215,0.22,0.225,0.23,0.235,0.24,0.245,0.25,0.255,
0.26,0.265,0.27,0.275,0.28,0.285,0.29,0.295,0.3,0.305,0.31,0.315,0.32,0.325,
0.33,0.335,0.34,0.345,0.35,0.355,0.36,0.365,0.37,0.375,0.38,0.385,0.39,
0.395,0.4,0.405,0.41,0.415,0.42,0.425,0.43,0.435,0.44,0.445,0.45,0.455,
0.46,0.465,0.47,0.475,0.48,0.485,0.49,0.495,0.5,0.505,0.51,0.515,0.52,0.525,
0.53,0.535,0.54,0.545,0.55,0.555,0.56,0.565,0.57,0.575,0.58,0.585,0.59,
0.595,0.6,0.605,0.61,0.615,0.62,0.625,0.63,0.635,0.64,0.645,0.65,0.655,
0.66,0.665,0.67,0.675,0.68,0.685,0.690000000000001,0.695000000000001,0.700000000000001,
0.705000000000001,0.710000000000001,0.715000000000001,0.720000000000001,
0.725000000000001,0.730000000000001,0.735000000000001,0.740000000000001,
0.745000000000001,0.750000000000001,0.755000000000001,0.760000000000001,
0.765000000000001,0.770000000000001,0.775000000000001,0.780000000000001,
0.785000000000001,0.790000000000001,0.795000000000001,0.800000000000001,
0.805000000000001,0.810000000000001,0.815000000000001,0.820000000000001,
0.825000000000001,0.830000000000001,0.835000000000001,0.840000000000001,
0.845000000000001,0.850000000000001,0.855000000000001,0.860000000000001,
0.865000000000001,0.870000000000001,0.875000000000001,0.880000000000001,
0.885000000000001,0.890000000000001,0.895000000000001,0.900000000000001,
0.905000000000001,0.910000000000001,0.915000000000001,0.920000000000001,
0.925000000000001,0.930000000000001,0.935000000000001,0.940000000000001,
0.945000000000001,0.950000000000001,0.955000000000001,0.960000000000001,
0.965000000000001,0.970000000000001,0.975000000000001,0.980000000000001,
0.985000000000001,0.990000000000001,0.995000000000001,1.),(0.,1.2),
 .UNSPECIFIED.)
GEOMETRIC_REPRESENTATION_ITEM()
RATIONAL_B_SPLINE_SURFACE(((1.,1.),(1.,1.),(1.,1.),(1.,1.),(1.,1.),(1.,
1.),(1.,1.),(1.,1.),(1.,1.),(1.,1.),(1.,1.),(1.,1.),(1.,1.),(1.,1.),(1.,
1.),(1.,1.),(1.,1.),(1.,1.),(1.,1.),(1.,1.),(1.,1.),(1.,1.),(1.,1.),(1.,
1.),(1.,1.),(1.,1.),(1.,1.),(1.,1.),(1.,1.),(1.,1.),(1.,1.),(1.,1.),(1.,
1.),(1.,1.),(1.,1.),(1.,1.),(1.,1.),(1.,1.),(1.,1.),(1.,1.),(1.,1.),(1.,
1.),(1.,1.),(1.,1.),(1.,1.),(1.,1.),(1.,1.),(1.,1.),(1.,1.),(1.,1.),(1.,
1.),(1.,1.),(1.,1.),(1.,1.),(1.,1.),(1.,1.),(1.,1.),(1.,1.),(1.,1.),(1.,
1.),(1.,1.),(1.,1.),(1.,1.),(1.,1.),(1.,1.),(1.,1.),(1.,1.),(1.,1.),(1.,
1.),(1.,1.),(1.,1.),(1.,1.),(1.,1.),(1.,1.),(1.,1.),(1.,1.),(1.,1.),(1.,
1.),(1.,1.),(1.,1.),(1.,1.),(1.,1.),(1.,1.),(1.,1.),(1.,1.),(1.,1.),(1.,
1.),(1.,1.),(1.,1.),(1.,1.),(1.,1.),(1.,1.),(1.,1.),(1.,1.),(1.,1.),(1.,
1.),(1.,1.),(1.,1.),(1.,1.),(1.,1.),(1.,1.),(1.,1.),(1.,1.),(1.,1.),(1.,
1.),(1.,1.),(1.,1.),(1.,1.),(1.,1.),(1.,1.),(1.,1.),(1.,1.),(1.,1.),(1.,
1.),(1.,1.),(1.,1.),(1.,1.),(1.,1.),(1.,1.),(1.,1.),(1.,1.),(1.,1.),(1.,
1.),(1.,1.),(1.,1.),(1.,1.),(1.,1.),(1.,1.),(1.,1.),(1.,1.),(1.,1.),(1.,
1.),(1.,1.),(1.,1.),(1.,1.),(1.,1.),(1.,1.),(1.,1.),(1.,1.),(1.,1.),(1.,
1.),(1.,1.),(1.,1.),(1.,1.),(1.,1.),(1.,1.),(1.,1.),(1.,1.),(1.,1.),(1.,
1.),(1.,1.),(1.,1.),(1.,1.),(1.,1.),(1.,1.),(1.,1.),(1.,1.),(1.,1.),(1.,
1.),(1.,1.),(1.,1.),(1.,1.),(1.,1.),(1.,1.),(1.,1.),(1.,1.),(1.,1.),(1.,
1.),(1.,1.),(1.,1.),(1.,1.),(1.,1.),(1.,1.),(1.,1.),(1.,1.),(1.,1.),(1.,
1.),(1.,1.),(1.,1.),(1.,1.),(1.,1.),(1.,1.),(1.,1.),(1.,1.),(1.,1.),(1.,
1.),(1.,1.),(1.,1.),(1.,1.),(1.,1.),(1.,1.),(1.,1.),(1.,1.),(1.,1.),(1.,
1.),(1.,1.),(1.,1.),(1.,1.),(1.,1.),(1.,1.),(1.,1.),(1.,1.),(1.,1.),(1.,
1.),(1.,1.)))
REPRESENTATION_ITEM('')
SURFACE()
);
#897=(
BOUNDED_SURFACE()
B_SPLINE_SURFACE(5,1,((#65166,#65167),(#65168,#65169),(#65170,#65171),(#65172,
#65173),(#65174,#65175),(#65176,#65177),(#65178,#65179),(#65180,#65181),
(#65182,#65183),(#65184,#65185),(#65186,#65187),(#65188,#65189),(#65190,
#65191),(#65192,#65193),(#65194,#65195),(#65196,#65197),(#65198,#65199),
(#65200,#65201),(#65202,#65203),(#65204,#65205),(#65206,#65207),(#65208,
#65209),(#65210,#65211),(#65212,#65213),(#65214,#65215),(#65216,#65217),
(#65218,#65219),(#65220,#65221),(#65222,#65223),(#65224,#65225),(#65226,
#65227),(#65228,#65229),(#65230,#65231),(#65232,#65233),(#65234,#65235),
(#65236,#65237),(#65238,#65239),(#65240,#65241),(#65242,#65243),(#65244,
#65245),(#65246,#65247),(#65248,#65249),(#65250,#65251),(#65252,#65253),
(#65254,#65255),(#65256,#65257),(#65258,#65259),(#65260,#65261),(#65262,
#65263),(#65264,#65265),(#65266,#65267),(#65268,#65269),(#65270,#65271),
(#65272,#65273),(#65274,#65275),(#65276,#65277),(#65278,#65279),(#65280,
#65281),(#65282,#65283),(#65284,#65285),(#65286,#65287),(#65288,#65289),
(#65290,#65291),(#65292,#65293),(#65294,#65295),(#65296,#65297),(#65298,
#65299),(#65300,#65301),(#65302,#65303),(#65304,#65305),(#65306,#65307),
(#65308,#65309),(#65310,#65311),(#65312,#65313),(#65314,#65315),(#65316,
#65317),(#65318,#65319),(#65320,#65321),(#65322,#65323),(#65324,#65325),
(#65326,#65327),(#65328,#65329),(#65330,#65331),(#65332,#65333),(#65334,
#65335),(#65336,#65337),(#65338,#65339),(#65340,#65341),(#65342,#65343),
(#65344,#65345),(#65346,#65347),(#65348,#65349),(#65350,#65351),(#65352,
#65353),(#65354,#65355),(#65356,#65357),(#65358,#65359),(#65360,#65361),
(#65362,#65363),(#65364,#65365),(#65366,#65367),(#65368,#65369),(#65370,
#65371),(#65372,#65373),(#65374,#65375),(#65376,#65377),(#65378,#65379),
(#65380,#65381),(#65382,#65383),(#65384,#65385),(#65386,#65387),(#65388,
#65389),(#65390,#65391),(#65392,#65393),(#65394,#65395),(#65396,#65397),
(#65398,#65399),(#65400,#65401),(#65402,#65403),(#65404,#65405),(#65406,
#65407),(#65408,#65409),(#65410,#65411),(#65412,#65413),(#65414,#65415),
(#65416,#65417),(#65418,#65419),(#65420,#65421),(#65422,#65423),(#65424,
#65425),(#65426,#65427),(#65428,#65429),(#65430,#65431),(#65432,#65433),
(#65434,#65435),(#65436,#65437),(#65438,#65439),(#65440,#65441),(#65442,
#65443),(#65444,#65445),(#65446,#65447),(#65448,#65449),(#65450,#65451),
(#65452,#65453),(#65454,#65455),(#65456,#65457),(#65458,#65459),(#65460,
#65461),(#65462,#65463),(#65464,#65465),(#65466,#65467),(#65468,#65469),
(#65470,#65471),(#65472,#65473),(#65474,#65475),(#65476,#65477),(#65478,
#65479),(#65480,#65481),(#65482,#65483),(#65484,#65485),(#65486,#65487),
(#65488,#65489),(#65490,#65491),(#65492,#65493),(#65494,#65495),(#65496,
#65497),(#65498,#65499),(#65500,#65501),(#65502,#65503),(#65504,#65505),
(#65506,#65507),(#65508,#65509),(#65510,#65511),(#65512,#65513),(#65514,
#65515),(#65516,#65517),(#65518,#65519),(#65520,#65521),(#65522,#65523),
(#65524,#65525),(#65526,#65527),(#65528,#65529),(#65530,#65531),(#65532,
#65533),(#65534,#65535),(#65536,#65537),(#65538,#65539),(#65540,#65541),
(#65542,#65543),(#65544,#65545),(#65546,#65547),(#65548,#65549),(#65550,
#65551),(#65552,#65553),(#65554,#65555),(#65556,#65557),(#65558,#65559),
(#65560,#65561),(#65562,#65563),(#65564,#65565),(#65566,#65567),(#65568,
#65569),(#65570,#65571),(#65572,#65573),(#65574,#65575)),.UNSPECIFIED.,
 .F.,.F.,.F.)
B_SPLINE_SURFACE_WITH_KNOTS((6,1,1,1,1,1,1,1,1,1,1,1,1,1,1,1,1,1,1,1,1,
1,1,1,1,1,1,1,1,1,1,1,1,1,1,1,1,1,1,1,1,1,1,1,1,1,1,1,1,1,1,1,1,1,1,1,1,
1,1,1,1,1,1,1,1,1,1,1,1,1,1,1,1,1,1,1,1,1,1,1,1,1,1,1,1,1,1,1,1,1,1,1,1,
1,1,1,1,1,1,1,1,1,1,1,1,1,1,1,1,1,1,1,1,1,1,1,1,1,1,1,1,1,1,1,1,1,1,1,1,
1,1,1,1,1,1,1,1,1,1,1,1,1,1,1,1,1,1,1,1,1,1,1,1,1,1,1,1,1,1,1,1,1,1,1,1,
1,1,1,1,1,1,1,1,1,1,1,1,1,1,1,1,1,1,1,1,1,1,1,1,1,1,1,1,1,1,1,1,1,1,1,6),
(2,2),(0.,0.005,0.01,0.015,0.02,0.025,0.03,0.035,0.04,0.045,0.05,0.055,
0.06,0.065,0.07,0.075,0.08,0.085,0.09,0.095,0.1,0.105,0.11,0.115,0.12,0.125,
0.13,0.135,0.14,0.145,0.15,0.155,0.16,0.165,0.17,0.175,0.18,0.185,0.19,
0.195,0.2,0.205,0.21,0.215,0.22,0.225,0.23,0.235,0.24,0.245,0.25,0.255,
0.26,0.265,0.27,0.275,0.28,0.285,0.29,0.295,0.3,0.305,0.31,0.315,0.32,0.325,
0.33,0.335,0.34,0.345,0.35,0.355,0.36,0.365,0.37,0.375,0.38,0.385,0.39,
0.395,0.4,0.405,0.41,0.415,0.42,0.425,0.43,0.435,0.44,0.445,0.45,0.455,
0.46,0.465,0.47,0.475,0.48,0.485,0.49,0.495,0.5,0.505,0.51,0.515,0.52,0.525,
0.53,0.535,0.54,0.545,0.55,0.555,0.56,0.565,0.57,0.575,0.58,0.585,0.59,
0.595,0.6,0.605,0.61,0.615,0.62,0.625,0.63,0.635,0.64,0.645,0.65,0.655,
0.66,0.665,0.67,0.675,0.68,0.685,0.690000000000001,0.695000000000001,0.700000000000001,
0.705000000000001,0.710000000000001,0.715000000000001,0.720000000000001,
0.725000000000001,0.730000000000001,0.735000000000001,0.740000000000001,
0.745000000000001,0.750000000000001,0.755000000000001,0.760000000000001,
0.765000000000001,0.770000000000001,0.775000000000001,0.780000000000001,
0.785000000000001,0.790000000000001,0.795000000000001,0.800000000000001,
0.805000000000001,0.810000000000001,0.815000000000001,0.820000000000001,
0.825000000000001,0.830000000000001,0.835000000000001,0.840000000000001,
0.845000000000001,0.850000000000001,0.855000000000001,0.860000000000001,
0.865000000000001,0.870000000000001,0.875000000000001,0.880000000000001,
0.885000000000001,0.890000000000001,0.895000000000001,0.900000000000001,
0.905000000000001,0.910000000000001,0.915000000000001,0.920000000000001,
0.925000000000001,0.930000000000001,0.935000000000001,0.940000000000001,
0.945000000000001,0.950000000000001,0.955000000000001,0.960000000000001,
0.965000000000001,0.970000000000001,0.975000000000001,0.980000000000001,
0.985000000000001,0.990000000000001,0.995000000000001,1.),(0.,1.2),
 .UNSPECIFIED.)
GEOMETRIC_REPRESENTATION_ITEM()
RATIONAL_B_SPLINE_SURFACE(((1.,1.),(1.,1.),(1.,1.),(1.,1.),(1.,1.),(1.,
1.),(1.,1.),(1.,1.),(1.,1.),(1.,1.),(1.,1.),(1.,1.),(1.,1.),(1.,1.),(1.,
1.),(1.,1.),(1.,1.),(1.,1.),(1.,1.),(1.,1.),(1.,1.),(1.,1.),(1.,1.),(1.,
1.),(1.,1.),(1.,1.),(1.,1.),(1.,1.),(1.,1.),(1.,1.),(1.,1.),(1.,1.),(1.,
1.),(1.,1.),(1.,1.),(1.,1.),(1.,1.),(1.,1.),(1.,1.),(1.,1.),(1.,1.),(1.,
1.),(1.,1.),(1.,1.),(1.,1.),(1.,1.),(1.,1.),(1.,1.),(1.,1.),(1.,1.),(1.,
1.),(1.,1.),(1.,1.),(1.,1.),(1.,1.),(1.,1.),(1.,1.),(1.,1.),(1.,1.),(1.,
1.),(1.,1.),(1.,1.),(1.,1.),(1.,1.),(1.,1.),(1.,1.),(1.,1.),(1.,1.),(1.,
1.),(1.,1.),(1.,1.),(1.,1.),(1.,1.),(1.,1.),(1.,1.),(1.,1.),(1.,1.),(1.,
1.),(1.,1.),(1.,1.),(1.,1.),(1.,1.),(1.,1.),(1.,1.),(1.,1.),(1.,1.),(1.,
1.),(1.,1.),(1.,1.),(1.,1.),(1.,1.),(1.,1.),(1.,1.),(1.,1.),(1.,1.),(1.,
1.),(1.,1.),(1.,1.),(1.,1.),(1.,1.),(1.,1.),(1.,1.),(1.,1.),(1.,1.),(1.,
1.),(1.,1.),(1.,1.),(1.,1.),(1.,1.),(1.,1.),(1.,1.),(1.,1.),(1.,1.),(1.,
1.),(1.,1.),(1.,1.),(1.,1.),(1.,1.),(1.,1.),(1.,1.),(1.,1.),(1.,1.),(1.,
1.),(1.,1.),(1.,1.),(1.,1.),(1.,1.),(1.,1.),(1.,1.),(1.,1.),(1.,1.),(1.,
1.),(1.,1.),(1.,1.),(1.,1.),(1.,1.),(1.,1.),(1.,1.),(1.,1.),(1.,1.),(1.,
1.),(1.,1.),(1.,1.),(1.,1.),(1.,1.),(1.,1.),(1.,1.),(1.,1.),(1.,1.),(1.,
1.),(1.,1.),(1.,1.),(1.,1.),(1.,1.),(1.,1.),(1.,1.),(1.,1.),(1.,1.),(1.,
1.),(1.,1.),(1.,1.),(1.,1.),(1.,1.),(1.,1.),(1.,1.),(1.,1.),(1.,1.),(1.,
1.),(1.,1.),(1.,1.),(1.,1.),(1.,1.),(1.,1.),(1.,1.),(1.,1.),(1.,1.),(1.,
1.),(1.,1.),(1.,1.),(1.,1.),(1.,1.),(1.,1.),(1.,1.),(1.,1.),(1.,1.),(1.,
1.),(1.,1.),(1.,1.),(1.,1.),(1.,1.),(1.,1.),(1.,1.),(1.,1.),(1.,1.),(1.,
1.),(1.,1.),(1.,1.),(1.,1.),(1.,1.),(1.,1.),(1.,1.),(1.,1.),(1.,1.),(1.,
1.),(1.,1.)))
REPRESENTATION_ITEM('')
SURFACE()
);
#898=(
BOUNDED_SURFACE()
B_SPLINE_SURFACE(5,1,((#66062,#66063),(#66064,#66065),(#66066,#66067),(#66068,
#66069),(#66070,#66071),(#66072,#66073),(#66074,#66075),(#66076,#66077),
(#66078,#66079),(#66080,#66081),(#66082,#66083),(#66084,#66085),(#66086,
#66087),(#66088,#66089),(#66090,#66091),(#66092,#66093),(#66094,#66095),
(#66096,#66097),(#66098,#66099),(#66100,#66101),(#66102,#66103),(#66104,
#66105),(#66106,#66107),(#66108,#66109),(#66110,#66111),(#66112,#66113),
(#66114,#66115),(#66116,#66117),(#66118,#66119),(#66120,#66121),(#66122,
#66123),(#66124,#66125),(#66126,#66127),(#66128,#66129),(#66130,#66131),
(#66132,#66133),(#66134,#66135),(#66136,#66137),(#66138,#66139),(#66140,
#66141),(#66142,#66143),(#66144,#66145),(#66146,#66147),(#66148,#66149),
(#66150,#66151),(#66152,#66153),(#66154,#66155),(#66156,#66157),(#66158,
#66159),(#66160,#66161),(#66162,#66163),(#66164,#66165),(#66166,#66167),
(#66168,#66169),(#66170,#66171),(#66172,#66173),(#66174,#66175),(#66176,
#66177),(#66178,#66179),(#66180,#66181),(#66182,#66183),(#66184,#66185),
(#66186,#66187),(#66188,#66189),(#66190,#66191),(#66192,#66193),(#66194,
#66195),(#66196,#66197),(#66198,#66199),(#66200,#66201),(#66202,#66203),
(#66204,#66205),(#66206,#66207),(#66208,#66209),(#66210,#66211),(#66212,
#66213),(#66214,#66215),(#66216,#66217),(#66218,#66219),(#66220,#66221),
(#66222,#66223),(#66224,#66225),(#66226,#66227),(#66228,#66229),(#66230,
#66231),(#66232,#66233),(#66234,#66235),(#66236,#66237),(#66238,#66239),
(#66240,#66241),(#66242,#66243),(#66244,#66245),(#66246,#66247),(#66248,
#66249),(#66250,#66251),(#66252,#66253),(#66254,#66255),(#66256,#66257),
(#66258,#66259),(#66260,#66261),(#66262,#66263),(#66264,#66265),(#66266,
#66267),(#66268,#66269),(#66270,#66271),(#66272,#66273),(#66274,#66275),
(#66276,#66277),(#66278,#66279),(#66280,#66281),(#66282,#66283),(#66284,
#66285),(#66286,#66287),(#66288,#66289),(#66290,#66291),(#66292,#66293),
(#66294,#66295),(#66296,#66297),(#66298,#66299),(#66300,#66301),(#66302,
#66303),(#66304,#66305),(#66306,#66307),(#66308,#66309),(#66310,#66311),
(#66312,#66313),(#66314,#66315),(#66316,#66317),(#66318,#66319),(#66320,
#66321),(#66322,#66323),(#66324,#66325),(#66326,#66327),(#66328,#66329),
(#66330,#66331),(#66332,#66333),(#66334,#66335),(#66336,#66337),(#66338,
#66339),(#66340,#66341),(#66342,#66343),(#66344,#66345),(#66346,#66347),
(#66348,#66349),(#66350,#66351),(#66352,#66353),(#66354,#66355),(#66356,
#66357),(#66358,#66359),(#66360,#66361),(#66362,#66363),(#66364,#66365),
(#66366,#66367),(#66368,#66369),(#66370,#66371),(#66372,#66373),(#66374,
#66375),(#66376,#66377),(#66378,#66379),(#66380,#66381),(#66382,#66383),
(#66384,#66385),(#66386,#66387),(#66388,#66389),(#66390,#66391),(#66392,
#66393),(#66394,#66395),(#66396,#66397),(#66398,#66399),(#66400,#66401),
(#66402,#66403),(#66404,#66405),(#66406,#66407),(#66408,#66409),(#66410,
#66411),(#66412,#66413),(#66414,#66415),(#66416,#66417),(#66418,#66419),
(#66420,#66421),(#66422,#66423),(#66424,#66425),(#66426,#66427),(#66428,
#66429),(#66430,#66431),(#66432,#66433),(#66434,#66435),(#66436,#66437),
(#66438,#66439),(#66440,#66441),(#66442,#66443),(#66444,#66445),(#66446,
#66447),(#66448,#66449),(#66450,#66451),(#66452,#66453),(#66454,#66455),
(#66456,#66457),(#66458,#66459),(#66460,#66461),(#66462,#66463),(#66464,
#66465),(#66466,#66467),(#66468,#66469),(#66470,#66471)),.UNSPECIFIED.,
 .F.,.F.,.F.)
B_SPLINE_SURFACE_WITH_KNOTS((6,1,1,1,1,1,1,1,1,1,1,1,1,1,1,1,1,1,1,1,1,
1,1,1,1,1,1,1,1,1,1,1,1,1,1,1,1,1,1,1,1,1,1,1,1,1,1,1,1,1,1,1,1,1,1,1,1,
1,1,1,1,1,1,1,1,1,1,1,1,1,1,1,1,1,1,1,1,1,1,1,1,1,1,1,1,1,1,1,1,1,1,1,1,
1,1,1,1,1,1,1,1,1,1,1,1,1,1,1,1,1,1,1,1,1,1,1,1,1,1,1,1,1,1,1,1,1,1,1,1,
1,1,1,1,1,1,1,1,1,1,1,1,1,1,1,1,1,1,1,1,1,1,1,1,1,1,1,1,1,1,1,1,1,1,1,1,
1,1,1,1,1,1,1,1,1,1,1,1,1,1,1,1,1,1,1,1,1,1,1,1,1,1,1,1,1,1,1,1,1,1,1,6),
(2,2),(0.,0.005,0.01,0.015,0.02,0.025,0.03,0.035,0.04,0.045,0.05,0.055,
0.06,0.065,0.07,0.075,0.08,0.085,0.09,0.095,0.1,0.105,0.11,0.115,0.12,0.125,
0.13,0.135,0.14,0.145,0.15,0.155,0.16,0.165,0.17,0.175,0.18,0.185,0.19,
0.195,0.2,0.205,0.21,0.215,0.22,0.225,0.23,0.235,0.24,0.245,0.25,0.255,
0.26,0.265,0.27,0.275,0.28,0.285,0.29,0.295,0.3,0.305,0.31,0.315,0.32,0.325,
0.33,0.335,0.34,0.345,0.35,0.355,0.36,0.365,0.37,0.375,0.38,0.385,0.39,
0.395,0.4,0.405,0.41,0.415,0.42,0.425,0.43,0.435,0.44,0.445,0.45,0.455,
0.46,0.465,0.47,0.475,0.48,0.485,0.49,0.495,0.5,0.505,0.51,0.515,0.52,0.525,
0.53,0.535,0.54,0.545,0.55,0.555,0.56,0.565,0.57,0.575,0.58,0.585,0.59,
0.595,0.6,0.605,0.61,0.615,0.62,0.625,0.63,0.635,0.64,0.645,0.65,0.655,
0.66,0.665,0.67,0.675,0.68,0.685,0.690000000000001,0.695000000000001,0.700000000000001,
0.705000000000001,0.710000000000001,0.715000000000001,0.720000000000001,
0.725000000000001,0.730000000000001,0.735000000000001,0.740000000000001,
0.745000000000001,0.750000000000001,0.755000000000001,0.760000000000001,
0.765000000000001,0.770000000000001,0.775000000000001,0.780000000000001,
0.785000000000001,0.790000000000001,0.795000000000001,0.800000000000001,
0.805000000000001,0.810000000000001,0.815000000000001,0.820000000000001,
0.825000000000001,0.830000000000001,0.835000000000001,0.840000000000001,
0.845000000000001,0.850000000000001,0.855000000000001,0.860000000000001,
0.865000000000001,0.870000000000001,0.875000000000001,0.880000000000001,
0.885000000000001,0.890000000000001,0.895000000000001,0.900000000000001,
0.905000000000001,0.910000000000001,0.915000000000001,0.920000000000001,
0.925000000000001,0.930000000000001,0.935000000000001,0.940000000000001,
0.945000000000001,0.950000000000001,0.955000000000001,0.960000000000001,
0.965000000000001,0.970000000000001,0.975000000000001,0.980000000000001,
0.985000000000001,0.990000000000001,0.995000000000001,1.),(0.,1.2),
 .UNSPECIFIED.)
GEOMETRIC_REPRESENTATION_ITEM()
RATIONAL_B_SPLINE_SURFACE(((1.,1.),(1.,1.),(1.,1.),(1.,1.),(1.,1.),(1.,
1.),(1.,1.),(1.,1.),(1.,1.),(1.,1.),(1.,1.),(1.,1.),(1.,1.),(1.,1.),(1.,
1.),(1.,1.),(1.,1.),(1.,1.),(1.,1.),(1.,1.),(1.,1.),(1.,1.),(1.,1.),(1.,
1.),(1.,1.),(1.,1.),(1.,1.),(1.,1.),(1.,1.),(1.,1.),(1.,1.),(1.,1.),(1.,
1.),(1.,1.),(1.,1.),(1.,1.),(1.,1.),(1.,1.),(1.,1.),(1.,1.),(1.,1.),(1.,
1.),(1.,1.),(1.,1.),(1.,1.),(1.,1.),(1.,1.),(1.,1.),(1.,1.),(1.,1.),(1.,
1.),(1.,1.),(1.,1.),(1.,1.),(1.,1.),(1.,1.),(1.,1.),(1.,1.),(1.,1.),(1.,
1.),(1.,1.),(1.,1.),(1.,1.),(1.,1.),(1.,1.),(1.,1.),(1.,1.),(1.,1.),(1.,
1.),(1.,1.),(1.,1.),(1.,1.),(1.,1.),(1.,1.),(1.,1.),(1.,1.),(1.,1.),(1.,
1.),(1.,1.),(1.,1.),(1.,1.),(1.,1.),(1.,1.),(1.,1.),(1.,1.),(1.,1.),(1.,
1.),(1.,1.),(1.,1.),(1.,1.),(1.,1.),(1.,1.),(1.,1.),(1.,1.),(1.,1.),(1.,
1.),(1.,1.),(1.,1.),(1.,1.),(1.,1.),(1.,1.),(1.,1.),(1.,1.),(1.,1.),(1.,
1.),(1.,1.),(1.,1.),(1.,1.),(1.,1.),(1.,1.),(1.,1.),(1.,1.),(1.,1.),(1.,
1.),(1.,1.),(1.,1.),(1.,1.),(1.,1.),(1.,1.),(1.,1.),(1.,1.),(1.,1.),(1.,
1.),(1.,1.),(1.,1.),(1.,1.),(1.,1.),(1.,1.),(1.,1.),(1.,1.),(1.,1.),(1.,
1.),(1.,1.),(1.,1.),(1.,1.),(1.,1.),(1.,1.),(1.,1.),(1.,1.),(1.,1.),(1.,
1.),(1.,1.),(1.,1.),(1.,1.),(1.,1.),(1.,1.),(1.,1.),(1.,1.),(1.,1.),(1.,
1.),(1.,1.),(1.,1.),(1.,1.),(1.,1.),(1.,1.),(1.,1.),(1.,1.),(1.,1.),(1.,
1.),(1.,1.),(1.,1.),(1.,1.),(1.,1.),(1.,1.),(1.,1.),(1.,1.),(1.,1.),(1.,
1.),(1.,1.),(1.,1.),(1.,1.),(1.,1.),(1.,1.),(1.,1.),(1.,1.),(1.,1.),(1.,
1.),(1.,1.),(1.,1.),(1.,1.),(1.,1.),(1.,1.),(1.,1.),(1.,1.),(1.,1.),(1.,
1.),(1.,1.),(1.,1.),(1.,1.),(1.,1.),(1.,1.),(1.,1.),(1.,1.),(1.,1.),(1.,
1.),(1.,1.),(1.,1.),(1.,1.),(1.,1.),(1.,1.),(1.,1.),(1.,1.),(1.,1.),(1.,
1.),(1.,1.)))
REPRESENTATION_ITEM('')
SURFACE()
);
#899=(
BOUNDED_SURFACE()
B_SPLINE_SURFACE(5,1,((#66958,#66959),(#66960,#66961),(#66962,#66963),(#66964,
#66965),(#66966,#66967),(#66968,#66969),(#66970,#66971),(#66972,#66973),
(#66974,#66975),(#66976,#66977),(#66978,#66979),(#66980,#66981),(#66982,
#66983),(#66984,#66985),(#66986,#66987),(#66988,#66989),(#66990,#66991),
(#66992,#66993),(#66994,#66995),(#66996,#66997),(#66998,#66999),(#67000,
#67001),(#67002,#67003),(#67004,#67005),(#67006,#67007),(#67008,#67009),
(#67010,#67011),(#67012,#67013),(#67014,#67015),(#67016,#67017),(#67018,
#67019),(#67020,#67021),(#67022,#67023),(#67024,#67025),(#67026,#67027),
(#67028,#67029),(#67030,#67031),(#67032,#67033),(#67034,#67035),(#67036,
#67037),(#67038,#67039),(#67040,#67041),(#67042,#67043),(#67044,#67045),
(#67046,#67047),(#67048,#67049),(#67050,#67051),(#67052,#67053),(#67054,
#67055),(#67056,#67057),(#67058,#67059),(#67060,#67061),(#67062,#67063),
(#67064,#67065),(#67066,#67067),(#67068,#67069),(#67070,#67071),(#67072,
#67073),(#67074,#67075),(#67076,#67077),(#67078,#67079),(#67080,#67081),
(#67082,#67083),(#67084,#67085),(#67086,#67087),(#67088,#67089),(#67090,
#67091),(#67092,#67093),(#67094,#67095),(#67096,#67097),(#67098,#67099),
(#67100,#67101),(#67102,#67103),(#67104,#67105),(#67106,#67107),(#67108,
#67109),(#67110,#67111),(#67112,#67113),(#67114,#67115),(#67116,#67117),
(#67118,#67119),(#67120,#67121),(#67122,#67123),(#67124,#67125),(#67126,
#67127),(#67128,#67129),(#67130,#67131),(#67132,#67133),(#67134,#67135),
(#67136,#67137),(#67138,#67139),(#67140,#67141),(#67142,#67143),(#67144,
#67145),(#67146,#67147),(#67148,#67149),(#67150,#67151),(#67152,#67153),
(#67154,#67155),(#67156,#67157),(#67158,#67159),(#67160,#67161),(#67162,
#67163),(#67164,#67165),(#67166,#67167),(#67168,#67169),(#67170,#67171),
(#67172,#67173),(#67174,#67175),(#67176,#67177),(#67178,#67179),(#67180,
#67181),(#67182,#67183),(#67184,#67185),(#67186,#67187),(#67188,#67189),
(#67190,#67191),(#67192,#67193),(#67194,#67195),(#67196,#67197),(#67198,
#67199),(#67200,#67201),(#67202,#67203),(#67204,#67205),(#67206,#67207),
(#67208,#67209),(#67210,#67211),(#67212,#67213),(#67214,#67215),(#67216,
#67217),(#67218,#67219),(#67220,#67221),(#67222,#67223),(#67224,#67225),
(#67226,#67227),(#67228,#67229),(#67230,#67231),(#67232,#67233),(#67234,
#67235),(#67236,#67237),(#67238,#67239),(#67240,#67241),(#67242,#67243),
(#67244,#67245),(#67246,#67247),(#67248,#67249),(#67250,#67251),(#67252,
#67253),(#67254,#67255),(#67256,#67257),(#67258,#67259),(#67260,#67261),
(#67262,#67263),(#67264,#67265),(#67266,#67267),(#67268,#67269),(#67270,
#67271),(#67272,#67273),(#67274,#67275),(#67276,#67277),(#67278,#67279),
(#67280,#67281),(#67282,#67283),(#67284,#67285),(#67286,#67287),(#67288,
#67289),(#67290,#67291),(#67292,#67293),(#67294,#67295),(#67296,#67297),
(#67298,#67299),(#67300,#67301),(#67302,#67303),(#67304,#67305),(#67306,
#67307),(#67308,#67309),(#67310,#67311),(#67312,#67313),(#67314,#67315),
(#67316,#67317),(#67318,#67319),(#67320,#67321),(#67322,#67323),(#67324,
#67325),(#67326,#67327),(#67328,#67329),(#67330,#67331),(#67332,#67333),
(#67334,#67335),(#67336,#67337),(#67338,#67339),(#67340,#67341),(#67342,
#67343),(#67344,#67345),(#67346,#67347),(#67348,#67349),(#67350,#67351),
(#67352,#67353),(#67354,#67355),(#67356,#67357),(#67358,#67359),(#67360,
#67361),(#67362,#67363),(#67364,#67365),(#67366,#67367)),.UNSPECIFIED.,
 .F.,.F.,.F.)
B_SPLINE_SURFACE_WITH_KNOTS((6,1,1,1,1,1,1,1,1,1,1,1,1,1,1,1,1,1,1,1,1,
1,1,1,1,1,1,1,1,1,1,1,1,1,1,1,1,1,1,1,1,1,1,1,1,1,1,1,1,1,1,1,1,1,1,1,1,
1,1,1,1,1,1,1,1,1,1,1,1,1,1,1,1,1,1,1,1,1,1,1,1,1,1,1,1,1,1,1,1,1,1,1,1,
1,1,1,1,1,1,1,1,1,1,1,1,1,1,1,1,1,1,1,1,1,1,1,1,1,1,1,1,1,1,1,1,1,1,1,1,
1,1,1,1,1,1,1,1,1,1,1,1,1,1,1,1,1,1,1,1,1,1,1,1,1,1,1,1,1,1,1,1,1,1,1,1,
1,1,1,1,1,1,1,1,1,1,1,1,1,1,1,1,1,1,1,1,1,1,1,1,1,1,1,1,1,1,1,1,1,1,1,6),
(2,2),(0.,0.005,0.01,0.015,0.02,0.025,0.03,0.035,0.04,0.045,0.05,0.055,
0.06,0.065,0.07,0.075,0.08,0.085,0.09,0.095,0.1,0.105,0.11,0.115,0.12,0.125,
0.13,0.135,0.14,0.145,0.15,0.155,0.16,0.165,0.17,0.175,0.18,0.185,0.19,
0.195,0.2,0.205,0.21,0.215,0.22,0.225,0.23,0.235,0.24,0.245,0.25,0.255,
0.26,0.265,0.27,0.275,0.28,0.285,0.29,0.295,0.3,0.305,0.31,0.315,0.32,0.325,
0.33,0.335,0.34,0.345,0.35,0.355,0.36,0.365,0.37,0.375,0.38,0.385,0.39,
0.395,0.4,0.405,0.41,0.415,0.42,0.425,0.43,0.435,0.44,0.445,0.45,0.455,
0.46,0.465,0.47,0.475,0.48,0.485,0.49,0.495,0.5,0.505,0.51,0.515,0.52,0.525,
0.53,0.535,0.54,0.545,0.55,0.555,0.56,0.565,0.57,0.575,0.58,0.585,0.59,
0.595,0.6,0.605,0.61,0.615,0.62,0.625,0.63,0.635,0.64,0.645,0.65,0.655,
0.66,0.665,0.67,0.675,0.68,0.685,0.690000000000001,0.695000000000001,0.700000000000001,
0.705000000000001,0.710000000000001,0.715000000000001,0.720000000000001,
0.725000000000001,0.730000000000001,0.735000000000001,0.740000000000001,
0.745000000000001,0.750000000000001,0.755000000000001,0.760000000000001,
0.765000000000001,0.770000000000001,0.775000000000001,0.780000000000001,
0.785000000000001,0.790000000000001,0.795000000000001,0.800000000000001,
0.805000000000001,0.810000000000001,0.815000000000001,0.820000000000001,
0.825000000000001,0.830000000000001,0.835000000000001,0.840000000000001,
0.845000000000001,0.850000000000001,0.855000000000001,0.860000000000001,
0.865000000000001,0.870000000000001,0.875000000000001,0.880000000000001,
0.885000000000001,0.890000000000001,0.895000000000001,0.900000000000001,
0.905000000000001,0.910000000000001,0.915000000000001,0.920000000000001,
0.925000000000001,0.930000000000001,0.935000000000001,0.940000000000001,
0.945000000000001,0.950000000000001,0.955000000000001,0.960000000000001,
0.965000000000001,0.970000000000001,0.975000000000001,0.980000000000001,
0.985000000000001,0.990000000000001,0.995000000000001,1.),(0.,1.2),
 .UNSPECIFIED.)
GEOMETRIC_REPRESENTATION_ITEM()
RATIONAL_B_SPLINE_SURFACE(((1.,1.),(1.,1.),(1.,1.),(1.,1.),(1.,1.),(1.,
1.),(1.,1.),(1.,1.),(1.,1.),(1.,1.),(1.,1.),(1.,1.),(1.,1.),(1.,1.),(1.,
1.),(1.,1.),(1.,1.),(1.,1.),(1.,1.),(1.,1.),(1.,1.),(1.,1.),(1.,1.),(1.,
1.),(1.,1.),(1.,1.),(1.,1.),(1.,1.),(1.,1.),(1.,1.),(1.,1.),(1.,1.),(1.,
1.),(1.,1.),(1.,1.),(1.,1.),(1.,1.),(1.,1.),(1.,1.),(1.,1.),(1.,1.),(1.,
1.),(1.,1.),(1.,1.),(1.,1.),(1.,1.),(1.,1.),(1.,1.),(1.,1.),(1.,1.),(1.,
1.),(1.,1.),(1.,1.),(1.,1.),(1.,1.),(1.,1.),(1.,1.),(1.,1.),(1.,1.),(1.,
1.),(1.,1.),(1.,1.),(1.,1.),(1.,1.),(1.,1.),(1.,1.),(1.,1.),(1.,1.),(1.,
1.),(1.,1.),(1.,1.),(1.,1.),(1.,1.),(1.,1.),(1.,1.),(1.,1.),(1.,1.),(1.,
1.),(1.,1.),(1.,1.),(1.,1.),(1.,1.),(1.,1.),(1.,1.),(1.,1.),(1.,1.),(1.,
1.),(1.,1.),(1.,1.),(1.,1.),(1.,1.),(1.,1.),(1.,1.),(1.,1.),(1.,1.),(1.,
1.),(1.,1.),(1.,1.),(1.,1.),(1.,1.),(1.,1.),(1.,1.),(1.,1.),(1.,1.),(1.,
1.),(1.,1.),(1.,1.),(1.,1.),(1.,1.),(1.,1.),(1.,1.),(1.,1.),(1.,1.),(1.,
1.),(1.,1.),(1.,1.),(1.,1.),(1.,1.),(1.,1.),(1.,1.),(1.,1.),(1.,1.),(1.,
1.),(1.,1.),(1.,1.),(1.,1.),(1.,1.),(1.,1.),(1.,1.),(1.,1.),(1.,1.),(1.,
1.),(1.,1.),(1.,1.),(1.,1.),(1.,1.),(1.,1.),(1.,1.),(1.,1.),(1.,1.),(1.,
1.),(1.,1.),(1.,1.),(1.,1.),(1.,1.),(1.,1.),(1.,1.),(1.,1.),(1.,1.),(1.,
1.),(1.,1.),(1.,1.),(1.,1.),(1.,1.),(1.,1.),(1.,1.),(1.,1.),(1.,1.),(1.,
1.),(1.,1.),(1.,1.),(1.,1.),(1.,1.),(1.,1.),(1.,1.),(1.,1.),(1.,1.),(1.,
1.),(1.,1.),(1.,1.),(1.,1.),(1.,1.),(1.,1.),(1.,1.),(1.,1.),(1.,1.),(1.,
1.),(1.,1.),(1.,1.),(1.,1.),(1.,1.),(1.,1.),(1.,1.),(1.,1.),(1.,1.),(1.,
1.),(1.,1.),(1.,1.),(1.,1.),(1.,1.),(1.,1.),(1.,1.),(1.,1.),(1.,1.),(1.,
1.),(1.,1.),(1.,1.),(1.,1.),(1.,1.),(1.,1.),(1.,1.),(1.,1.),(1.,1.),(1.,
1.),(1.,1.)))
REPRESENTATION_ITEM('')
SURFACE()
);
#900=(
BOUNDED_SURFACE()
B_SPLINE_SURFACE(5,1,((#67854,#67855),(#67856,#67857),(#67858,#67859),(#67860,
#67861),(#67862,#67863),(#67864,#67865),(#67866,#67867),(#67868,#67869),
(#67870,#67871),(#67872,#67873),(#67874,#67875),(#67876,#67877),(#67878,
#67879),(#67880,#67881),(#67882,#67883),(#67884,#67885),(#67886,#67887),
(#67888,#67889),(#67890,#67891),(#67892,#67893),(#67894,#67895),(#67896,
#67897),(#67898,#67899),(#67900,#67901),(#67902,#67903),(#67904,#67905),
(#67906,#67907),(#67908,#67909),(#67910,#67911),(#67912,#67913),(#67914,
#67915),(#67916,#67917),(#67918,#67919),(#67920,#67921),(#67922,#67923),
(#67924,#67925),(#67926,#67927),(#67928,#67929),(#67930,#67931),(#67932,
#67933),(#67934,#67935),(#67936,#67937),(#67938,#67939),(#67940,#67941),
(#67942,#67943),(#67944,#67945),(#67946,#67947),(#67948,#67949),(#67950,
#67951),(#67952,#67953),(#67954,#67955),(#67956,#67957),(#67958,#67959),
(#67960,#67961),(#67962,#67963),(#67964,#67965),(#67966,#67967),(#67968,
#67969),(#67970,#67971),(#67972,#67973),(#67974,#67975),(#67976,#67977),
(#67978,#67979),(#67980,#67981),(#67982,#67983),(#67984,#67985),(#67986,
#67987),(#67988,#67989),(#67990,#67991),(#67992,#67993),(#67994,#67995),
(#67996,#67997),(#67998,#67999),(#68000,#68001),(#68002,#68003),(#68004,
#68005),(#68006,#68007),(#68008,#68009),(#68010,#68011),(#68012,#68013),
(#68014,#68015),(#68016,#68017),(#68018,#68019),(#68020,#68021),(#68022,
#68023),(#68024,#68025),(#68026,#68027),(#68028,#68029),(#68030,#68031),
(#68032,#68033),(#68034,#68035),(#68036,#68037),(#68038,#68039),(#68040,
#68041),(#68042,#68043),(#68044,#68045),(#68046,#68047),(#68048,#68049),
(#68050,#68051),(#68052,#68053),(#68054,#68055),(#68056,#68057),(#68058,
#68059),(#68060,#68061),(#68062,#68063),(#68064,#68065),(#68066,#68067),
(#68068,#68069),(#68070,#68071),(#68072,#68073),(#68074,#68075),(#68076,
#68077),(#68078,#68079),(#68080,#68081),(#68082,#68083),(#68084,#68085),
(#68086,#68087),(#68088,#68089),(#68090,#68091),(#68092,#68093),(#68094,
#68095),(#68096,#68097),(#68098,#68099),(#68100,#68101),(#68102,#68103),
(#68104,#68105),(#68106,#68107),(#68108,#68109),(#68110,#68111),(#68112,
#68113),(#68114,#68115),(#68116,#68117),(#68118,#68119),(#68120,#68121),
(#68122,#68123),(#68124,#68125),(#68126,#68127),(#68128,#68129),(#68130,
#68131),(#68132,#68133),(#68134,#68135),(#68136,#68137),(#68138,#68139),
(#68140,#68141),(#68142,#68143),(#68144,#68145),(#68146,#68147),(#68148,
#68149),(#68150,#68151),(#68152,#68153),(#68154,#68155),(#68156,#68157),
(#68158,#68159),(#68160,#68161),(#68162,#68163),(#68164,#68165),(#68166,
#68167),(#68168,#68169),(#68170,#68171),(#68172,#68173),(#68174,#68175),
(#68176,#68177),(#68178,#68179),(#68180,#68181),(#68182,#68183),(#68184,
#68185),(#68186,#68187),(#68188,#68189),(#68190,#68191),(#68192,#68193),
(#68194,#68195),(#68196,#68197),(#68198,#68199),(#68200,#68201),(#68202,
#68203),(#68204,#68205),(#68206,#68207),(#68208,#68209),(#68210,#68211),
(#68212,#68213),(#68214,#68215),(#68216,#68217),(#68218,#68219),(#68220,
#68221),(#68222,#68223),(#68224,#68225),(#68226,#68227),(#68228,#68229),
(#68230,#68231),(#68232,#68233),(#68234,#68235),(#68236,#68237),(#68238,
#68239),(#68240,#68241),(#68242,#68243),(#68244,#68245),(#68246,#68247),
(#68248,#68249),(#68250,#68251),(#68252,#68253),(#68254,#68255),(#68256,
#68257),(#68258,#68259),(#68260,#68261),(#68262,#68263)),.UNSPECIFIED.,
 .F.,.F.,.F.)
B_SPLINE_SURFACE_WITH_KNOTS((6,1,1,1,1,1,1,1,1,1,1,1,1,1,1,1,1,1,1,1,1,
1,1,1,1,1,1,1,1,1,1,1,1,1,1,1,1,1,1,1,1,1,1,1,1,1,1,1,1,1,1,1,1,1,1,1,1,
1,1,1,1,1,1,1,1,1,1,1,1,1,1,1,1,1,1,1,1,1,1,1,1,1,1,1,1,1,1,1,1,1,1,1,1,
1,1,1,1,1,1,1,1,1,1,1,1,1,1,1,1,1,1,1,1,1,1,1,1,1,1,1,1,1,1,1,1,1,1,1,1,
1,1,1,1,1,1,1,1,1,1,1,1,1,1,1,1,1,1,1,1,1,1,1,1,1,1,1,1,1,1,1,1,1,1,1,1,
1,1,1,1,1,1,1,1,1,1,1,1,1,1,1,1,1,1,1,1,1,1,1,1,1,1,1,1,1,1,1,1,1,1,1,6),
(2,2),(0.,0.005,0.01,0.015,0.02,0.025,0.03,0.035,0.04,0.045,0.05,0.055,
0.06,0.065,0.07,0.075,0.08,0.085,0.09,0.095,0.1,0.105,0.11,0.115,0.12,0.125,
0.13,0.135,0.14,0.145,0.15,0.155,0.16,0.165,0.17,0.175,0.18,0.185,0.19,
0.195,0.2,0.205,0.21,0.215,0.22,0.225,0.23,0.235,0.24,0.245,0.25,0.255,
0.26,0.265,0.27,0.275,0.28,0.285,0.29,0.295,0.3,0.305,0.31,0.315,0.32,0.325,
0.33,0.335,0.34,0.345,0.35,0.355,0.36,0.365,0.37,0.375,0.38,0.385,0.39,
0.395,0.4,0.405,0.41,0.415,0.42,0.425,0.43,0.435,0.44,0.445,0.45,0.455,
0.46,0.465,0.47,0.475,0.48,0.485,0.49,0.495,0.5,0.505,0.51,0.515,0.52,0.525,
0.53,0.535,0.54,0.545,0.55,0.555,0.56,0.565,0.57,0.575,0.58,0.585,0.59,
0.595,0.6,0.605,0.61,0.615,0.62,0.625,0.63,0.635,0.64,0.645,0.65,0.655,
0.66,0.665,0.67,0.675,0.68,0.685,0.690000000000001,0.695000000000001,0.700000000000001,
0.705000000000001,0.710000000000001,0.715000000000001,0.720000000000001,
0.725000000000001,0.730000000000001,0.735000000000001,0.740000000000001,
0.745000000000001,0.750000000000001,0.755000000000001,0.760000000000001,
0.765000000000001,0.770000000000001,0.775000000000001,0.780000000000001,
0.785000000000001,0.790000000000001,0.795000000000001,0.800000000000001,
0.805000000000001,0.810000000000001,0.815000000000001,0.820000000000001,
0.825000000000001,0.830000000000001,0.835000000000001,0.840000000000001,
0.845000000000001,0.850000000000001,0.855000000000001,0.860000000000001,
0.865000000000001,0.870000000000001,0.875000000000001,0.880000000000001,
0.885000000000001,0.890000000000001,0.895000000000001,0.900000000000001,
0.905000000000001,0.910000000000001,0.915000000000001,0.920000000000001,
0.925000000000001,0.930000000000001,0.935000000000001,0.940000000000001,
0.945000000000001,0.950000000000001,0.955000000000001,0.960000000000001,
0.965000000000001,0.970000000000001,0.975000000000001,0.980000000000001,
0.985000000000001,0.990000000000001,0.995000000000001,1.),(0.,1.2),
 .UNSPECIFIED.)
GEOMETRIC_REPRESENTATION_ITEM()
RATIONAL_B_SPLINE_SURFACE(((1.,1.),(1.,1.),(1.,1.),(1.,1.),(1.,1.),(1.,
1.),(1.,1.),(1.,1.),(1.,1.),(1.,1.),(1.,1.),(1.,1.),(1.,1.),(1.,1.),(1.,
1.),(1.,1.),(1.,1.),(1.,1.),(1.,1.),(1.,1.),(1.,1.),(1.,1.),(1.,1.),(1.,
1.),(1.,1.),(1.,1.),(1.,1.),(1.,1.),(1.,1.),(1.,1.),(1.,1.),(1.,1.),(1.,
1.),(1.,1.),(1.,1.),(1.,1.),(1.,1.),(1.,1.),(1.,1.),(1.,1.),(1.,1.),(1.,
1.),(1.,1.),(1.,1.),(1.,1.),(1.,1.),(1.,1.),(1.,1.),(1.,1.),(1.,1.),(1.,
1.),(1.,1.),(1.,1.),(1.,1.),(1.,1.),(1.,1.),(1.,1.),(1.,1.),(1.,1.),(1.,
1.),(1.,1.),(1.,1.),(1.,1.),(1.,1.),(1.,1.),(1.,1.),(1.,1.),(1.,1.),(1.,
1.),(1.,1.),(1.,1.),(1.,1.),(1.,1.),(1.,1.),(1.,1.),(1.,1.),(1.,1.),(1.,
1.),(1.,1.),(1.,1.),(1.,1.),(1.,1.),(1.,1.),(1.,1.),(1.,1.),(1.,1.),(1.,
1.),(1.,1.),(1.,1.),(1.,1.),(1.,1.),(1.,1.),(1.,1.),(1.,1.),(1.,1.),(1.,
1.),(1.,1.),(1.,1.),(1.,1.),(1.,1.),(1.,1.),(1.,1.),(1.,1.),(1.,1.),(1.,
1.),(1.,1.),(1.,1.),(1.,1.),(1.,1.),(1.,1.),(1.,1.),(1.,1.),(1.,1.),(1.,
1.),(1.,1.),(1.,1.),(1.,1.),(1.,1.),(1.,1.),(1.,1.),(1.,1.),(1.,1.),(1.,
1.),(1.,1.),(1.,1.),(1.,1.),(1.,1.),(1.,1.),(1.,1.),(1.,1.),(1.,1.),(1.,
1.),(1.,1.),(1.,1.),(1.,1.),(1.,1.),(1.,1.),(1.,1.),(1.,1.),(1.,1.),(1.,
1.),(1.,1.),(1.,1.),(1.,1.),(1.,1.),(1.,1.),(1.,1.),(1.,1.),(1.,1.),(1.,
1.),(1.,1.),(1.,1.),(1.,1.),(1.,1.),(1.,1.),(1.,1.),(1.,1.),(1.,1.),(1.,
1.),(1.,1.),(1.,1.),(1.,1.),(1.,1.),(1.,1.),(1.,1.),(1.,1.),(1.,1.),(1.,
1.),(1.,1.),(1.,1.),(1.,1.),(1.,1.),(1.,1.),(1.,1.),(1.,1.),(1.,1.),(1.,
1.),(1.,1.),(1.,1.),(1.,1.),(1.,1.),(1.,1.),(1.,1.),(1.,1.),(1.,1.),(1.,
1.),(1.,1.),(1.,1.),(1.,1.),(1.,1.),(1.,1.),(1.,1.),(1.,1.),(1.,1.),(1.,
1.),(1.,1.),(1.,1.),(1.,1.),(1.,1.),(1.,1.),(1.,1.),(1.,1.),(1.,1.),(1.,
1.),(1.,1.)))
REPRESENTATION_ITEM('')
SURFACE()
);
#901=(
BOUNDED_SURFACE()
B_SPLINE_SURFACE(5,1,((#68750,#68751),(#68752,#68753),(#68754,#68755),(#68756,
#68757),(#68758,#68759),(#68760,#68761),(#68762,#68763),(#68764,#68765),
(#68766,#68767),(#68768,#68769),(#68770,#68771),(#68772,#68773),(#68774,
#68775),(#68776,#68777),(#68778,#68779),(#68780,#68781),(#68782,#68783),
(#68784,#68785),(#68786,#68787),(#68788,#68789),(#68790,#68791),(#68792,
#68793),(#68794,#68795),(#68796,#68797),(#68798,#68799),(#68800,#68801),
(#68802,#68803),(#68804,#68805),(#68806,#68807),(#68808,#68809),(#68810,
#68811),(#68812,#68813),(#68814,#68815),(#68816,#68817),(#68818,#68819),
(#68820,#68821),(#68822,#68823),(#68824,#68825),(#68826,#68827),(#68828,
#68829),(#68830,#68831),(#68832,#68833),(#68834,#68835),(#68836,#68837),
(#68838,#68839),(#68840,#68841),(#68842,#68843),(#68844,#68845),(#68846,
#68847),(#68848,#68849),(#68850,#68851),(#68852,#68853),(#68854,#68855),
(#68856,#68857),(#68858,#68859),(#68860,#68861),(#68862,#68863),(#68864,
#68865),(#68866,#68867),(#68868,#68869),(#68870,#68871),(#68872,#68873),
(#68874,#68875),(#68876,#68877),(#68878,#68879),(#68880,#68881),(#68882,
#68883),(#68884,#68885),(#68886,#68887),(#68888,#68889),(#68890,#68891),
(#68892,#68893),(#68894,#68895),(#68896,#68897),(#68898,#68899),(#68900,
#68901),(#68902,#68903),(#68904,#68905),(#68906,#68907),(#68908,#68909),
(#68910,#68911),(#68912,#68913),(#68914,#68915),(#68916,#68917),(#68918,
#68919),(#68920,#68921),(#68922,#68923),(#68924,#68925),(#68926,#68927),
(#68928,#68929),(#68930,#68931),(#68932,#68933),(#68934,#68935),(#68936,
#68937),(#68938,#68939),(#68940,#68941),(#68942,#68943),(#68944,#68945),
(#68946,#68947),(#68948,#68949),(#68950,#68951),(#68952,#68953),(#68954,
#68955),(#68956,#68957),(#68958,#68959),(#68960,#68961),(#68962,#68963),
(#68964,#68965),(#68966,#68967),(#68968,#68969),(#68970,#68971),(#68972,
#68973),(#68974,#68975),(#68976,#68977),(#68978,#68979),(#68980,#68981),
(#68982,#68983),(#68984,#68985),(#68986,#68987),(#68988,#68989),(#68990,
#68991),(#68992,#68993),(#68994,#68995),(#68996,#68997),(#68998,#68999),
(#69000,#69001),(#69002,#69003),(#69004,#69005),(#69006,#69007),(#69008,
#69009),(#69010,#69011),(#69012,#69013),(#69014,#69015),(#69016,#69017),
(#69018,#69019),(#69020,#69021),(#69022,#69023),(#69024,#69025),(#69026,
#69027),(#69028,#69029),(#69030,#69031),(#69032,#69033),(#69034,#69035),
(#69036,#69037),(#69038,#69039),(#69040,#69041),(#69042,#69043),(#69044,
#69045),(#69046,#69047),(#69048,#69049),(#69050,#69051),(#69052,#69053),
(#69054,#69055),(#69056,#69057),(#69058,#69059),(#69060,#69061),(#69062,
#69063),(#69064,#69065),(#69066,#69067),(#69068,#69069),(#69070,#69071),
(#69072,#69073),(#69074,#69075),(#69076,#69077),(#69078,#69079),(#69080,
#69081),(#69082,#69083),(#69084,#69085),(#69086,#69087),(#69088,#69089),
(#69090,#69091),(#69092,#69093),(#69094,#69095),(#69096,#69097),(#69098,
#69099),(#69100,#69101),(#69102,#69103),(#69104,#69105),(#69106,#69107),
(#69108,#69109),(#69110,#69111),(#69112,#69113),(#69114,#69115),(#69116,
#69117),(#69118,#69119),(#69120,#69121),(#69122,#69123),(#69124,#69125),
(#69126,#69127),(#69128,#69129),(#69130,#69131),(#69132,#69133),(#69134,
#69135),(#69136,#69137),(#69138,#69139),(#69140,#69141),(#69142,#69143),
(#69144,#69145),(#69146,#69147),(#69148,#69149),(#69150,#69151),(#69152,
#69153),(#69154,#69155),(#69156,#69157),(#69158,#69159)),.UNSPECIFIED.,
 .F.,.F.,.F.)
B_SPLINE_SURFACE_WITH_KNOTS((6,1,1,1,1,1,1,1,1,1,1,1,1,1,1,1,1,1,1,1,1,
1,1,1,1,1,1,1,1,1,1,1,1,1,1,1,1,1,1,1,1,1,1,1,1,1,1,1,1,1,1,1,1,1,1,1,1,
1,1,1,1,1,1,1,1,1,1,1,1,1,1,1,1,1,1,1,1,1,1,1,1,1,1,1,1,1,1,1,1,1,1,1,1,
1,1,1,1,1,1,1,1,1,1,1,1,1,1,1,1,1,1,1,1,1,1,1,1,1,1,1,1,1,1,1,1,1,1,1,1,
1,1,1,1,1,1,1,1,1,1,1,1,1,1,1,1,1,1,1,1,1,1,1,1,1,1,1,1,1,1,1,1,1,1,1,1,
1,1,1,1,1,1,1,1,1,1,1,1,1,1,1,1,1,1,1,1,1,1,1,1,1,1,1,1,1,1,1,1,1,1,1,6),
(2,2),(0.,0.005,0.01,0.015,0.02,0.025,0.03,0.035,0.04,0.045,0.05,0.055,
0.06,0.065,0.07,0.075,0.08,0.085,0.09,0.095,0.1,0.105,0.11,0.115,0.12,0.125,
0.13,0.135,0.14,0.145,0.15,0.155,0.16,0.165,0.17,0.175,0.18,0.185,0.19,
0.195,0.2,0.205,0.21,0.215,0.22,0.225,0.23,0.235,0.24,0.245,0.25,0.255,
0.26,0.265,0.27,0.275,0.28,0.285,0.29,0.295,0.3,0.305,0.31,0.315,0.32,0.325,
0.33,0.335,0.34,0.345,0.35,0.355,0.36,0.365,0.37,0.375,0.38,0.385,0.39,
0.395,0.4,0.405,0.41,0.415,0.42,0.425,0.43,0.435,0.44,0.445,0.45,0.455,
0.46,0.465,0.47,0.475,0.48,0.485,0.49,0.495,0.5,0.505,0.51,0.515,0.52,0.525,
0.53,0.535,0.54,0.545,0.55,0.555,0.56,0.565,0.57,0.575,0.58,0.585,0.59,
0.595,0.6,0.605,0.61,0.615,0.62,0.625,0.63,0.635,0.64,0.645,0.65,0.655,
0.66,0.665,0.67,0.675,0.68,0.685,0.690000000000001,0.695000000000001,0.700000000000001,
0.705000000000001,0.710000000000001,0.715000000000001,0.720000000000001,
0.725000000000001,0.730000000000001,0.735000000000001,0.740000000000001,
0.745000000000001,0.750000000000001,0.755000000000001,0.760000000000001,
0.765000000000001,0.770000000000001,0.775000000000001,0.780000000000001,
0.785000000000001,0.790000000000001,0.795000000000001,0.800000000000001,
0.805000000000001,0.810000000000001,0.815000000000001,0.820000000000001,
0.825000000000001,0.830000000000001,0.835000000000001,0.840000000000001,
0.845000000000001,0.850000000000001,0.855000000000001,0.860000000000001,
0.865000000000001,0.870000000000001,0.875000000000001,0.880000000000001,
0.885000000000001,0.890000000000001,0.895000000000001,0.900000000000001,
0.905000000000001,0.910000000000001,0.915000000000001,0.920000000000001,
0.925000000000001,0.930000000000001,0.935000000000001,0.940000000000001,
0.945000000000001,0.950000000000001,0.955000000000001,0.960000000000001,
0.965000000000001,0.970000000000001,0.975000000000001,0.980000000000001,
0.985000000000001,0.990000000000001,0.995000000000001,1.),(0.,1.2),
 .UNSPECIFIED.)
GEOMETRIC_REPRESENTATION_ITEM()
RATIONAL_B_SPLINE_SURFACE(((1.,1.),(1.,1.),(1.,1.),(1.,1.),(1.,1.),(1.,
1.),(1.,1.),(1.,1.),(1.,1.),(1.,1.),(1.,1.),(1.,1.),(1.,1.),(1.,1.),(1.,
1.),(1.,1.),(1.,1.),(1.,1.),(1.,1.),(1.,1.),(1.,1.),(1.,1.),(1.,1.),(1.,
1.),(1.,1.),(1.,1.),(1.,1.),(1.,1.),(1.,1.),(1.,1.),(1.,1.),(1.,1.),(1.,
1.),(1.,1.),(1.,1.),(1.,1.),(1.,1.),(1.,1.),(1.,1.),(1.,1.),(1.,1.),(1.,
1.),(1.,1.),(1.,1.),(1.,1.),(1.,1.),(1.,1.),(1.,1.),(1.,1.),(1.,1.),(1.,
1.),(1.,1.),(1.,1.),(1.,1.),(1.,1.),(1.,1.),(1.,1.),(1.,1.),(1.,1.),(1.,
1.),(1.,1.),(1.,1.),(1.,1.),(1.,1.),(1.,1.),(1.,1.),(1.,1.),(1.,1.),(1.,
1.),(1.,1.),(1.,1.),(1.,1.),(1.,1.),(1.,1.),(1.,1.),(1.,1.),(1.,1.),(1.,
1.),(1.,1.),(1.,1.),(1.,1.),(1.,1.),(1.,1.),(1.,1.),(1.,1.),(1.,1.),(1.,
1.),(1.,1.),(1.,1.),(1.,1.),(1.,1.),(1.,1.),(1.,1.),(1.,1.),(1.,1.),(1.,
1.),(1.,1.),(1.,1.),(1.,1.),(1.,1.),(1.,1.),(1.,1.),(1.,1.),(1.,1.),(1.,
1.),(1.,1.),(1.,1.),(1.,1.),(1.,1.),(1.,1.),(1.,1.),(1.,1.),(1.,1.),(1.,
1.),(1.,1.),(1.,1.),(1.,1.),(1.,1.),(1.,1.),(1.,1.),(1.,1.),(1.,1.),(1.,
1.),(1.,1.),(1.,1.),(1.,1.),(1.,1.),(1.,1.),(1.,1.),(1.,1.),(1.,1.),(1.,
1.),(1.,1.),(1.,1.),(1.,1.),(1.,1.),(1.,1.),(1.,1.),(1.,1.),(1.,1.),(1.,
1.),(1.,1.),(1.,1.),(1.,1.),(1.,1.),(1.,1.),(1.,1.),(1.,1.),(1.,1.),(1.,
1.),(1.,1.),(1.,1.),(1.,1.),(1.,1.),(1.,1.),(1.,1.),(1.,1.),(1.,1.),(1.,
1.),(1.,1.),(1.,1.),(1.,1.),(1.,1.),(1.,1.),(1.,1.),(1.,1.),(1.,1.),(1.,
1.),(1.,1.),(1.,1.),(1.,1.),(1.,1.),(1.,1.),(1.,1.),(1.,1.),(1.,1.),(1.,
1.),(1.,1.),(1.,1.),(1.,1.),(1.,1.),(1.,1.),(1.,1.),(1.,1.),(1.,1.),(1.,
1.),(1.,1.),(1.,1.),(1.,1.),(1.,1.),(1.,1.),(1.,1.),(1.,1.),(1.,1.),(1.,
1.),(1.,1.),(1.,1.),(1.,1.),(1.,1.),(1.,1.),(1.,1.),(1.,1.),(1.,1.),(1.,
1.),(1.,1.)))
REPRESENTATION_ITEM('')
SURFACE()
);
#902=(
BOUNDED_SURFACE()
B_SPLINE_SURFACE(5,1,((#69646,#69647),(#69648,#69649),(#69650,#69651),(#69652,
#69653),(#69654,#69655),(#69656,#69657),(#69658,#69659),(#69660,#69661),
(#69662,#69663),(#69664,#69665),(#69666,#69667),(#69668,#69669),(#69670,
#69671),(#69672,#69673),(#69674,#69675),(#69676,#69677),(#69678,#69679),
(#69680,#69681),(#69682,#69683),(#69684,#69685),(#69686,#69687),(#69688,
#69689),(#69690,#69691),(#69692,#69693),(#69694,#69695),(#69696,#69697),
(#69698,#69699),(#69700,#69701),(#69702,#69703),(#69704,#69705),(#69706,
#69707),(#69708,#69709),(#69710,#69711),(#69712,#69713),(#69714,#69715),
(#69716,#69717),(#69718,#69719),(#69720,#69721),(#69722,#69723),(#69724,
#69725),(#69726,#69727),(#69728,#69729),(#69730,#69731),(#69732,#69733),
(#69734,#69735),(#69736,#69737),(#69738,#69739),(#69740,#69741),(#69742,
#69743),(#69744,#69745),(#69746,#69747),(#69748,#69749),(#69750,#69751),
(#69752,#69753),(#69754,#69755),(#69756,#69757),(#69758,#69759),(#69760,
#69761),(#69762,#69763),(#69764,#69765),(#69766,#69767),(#69768,#69769),
(#69770,#69771),(#69772,#69773),(#69774,#69775),(#69776,#69777),(#69778,
#69779),(#69780,#69781),(#69782,#69783),(#69784,#69785),(#69786,#69787),
(#69788,#69789),(#69790,#69791),(#69792,#69793),(#69794,#69795),(#69796,
#69797),(#69798,#69799),(#69800,#69801),(#69802,#69803),(#69804,#69805),
(#69806,#69807),(#69808,#69809),(#69810,#69811),(#69812,#69813),(#69814,
#69815),(#69816,#69817),(#69818,#69819),(#69820,#69821),(#69822,#69823),
(#69824,#69825),(#69826,#69827),(#69828,#69829),(#69830,#69831),(#69832,
#69833),(#69834,#69835),(#69836,#69837),(#69838,#69839),(#69840,#69841),
(#69842,#69843),(#69844,#69845),(#69846,#69847),(#69848,#69849),(#69850,
#69851),(#69852,#69853),(#69854,#69855),(#69856,#69857),(#69858,#69859),
(#69860,#69861),(#69862,#69863),(#69864,#69865),(#69866,#69867),(#69868,
#69869),(#69870,#69871),(#69872,#69873),(#69874,#69875),(#69876,#69877),
(#69878,#69879),(#69880,#69881),(#69882,#69883),(#69884,#69885),(#69886,
#69887),(#69888,#69889),(#69890,#69891),(#69892,#69893),(#69894,#69895),
(#69896,#69897),(#69898,#69899),(#69900,#69901),(#69902,#69903),(#69904,
#69905),(#69906,#69907),(#69908,#69909),(#69910,#69911),(#69912,#69913),
(#69914,#69915),(#69916,#69917),(#69918,#69919),(#69920,#69921),(#69922,
#69923),(#69924,#69925),(#69926,#69927),(#69928,#69929),(#69930,#69931),
(#69932,#69933),(#69934,#69935),(#69936,#69937),(#69938,#69939),(#69940,
#69941),(#69942,#69943),(#69944,#69945),(#69946,#69947),(#69948,#69949),
(#69950,#69951),(#69952,#69953),(#69954,#69955),(#69956,#69957),(#69958,
#69959),(#69960,#69961),(#69962,#69963),(#69964,#69965),(#69966,#69967),
(#69968,#69969),(#69970,#69971),(#69972,#69973),(#69974,#69975),(#69976,
#69977),(#69978,#69979),(#69980,#69981),(#69982,#69983),(#69984,#69985),
(#69986,#69987),(#69988,#69989),(#69990,#69991),(#69992,#69993),(#69994,
#69995),(#69996,#69997),(#69998,#69999),(#70000,#70001),(#70002,#70003),
(#70004,#70005),(#70006,#70007),(#70008,#70009),(#70010,#70011),(#70012,
#70013),(#70014,#70015),(#70016,#70017),(#70018,#70019),(#70020,#70021),
(#70022,#70023),(#70024,#70025),(#70026,#70027),(#70028,#70029),(#70030,
#70031),(#70032,#70033),(#70034,#70035),(#70036,#70037),(#70038,#70039),
(#70040,#70041),(#70042,#70043),(#70044,#70045),(#70046,#70047),(#70048,
#70049),(#70050,#70051),(#70052,#70053),(#70054,#70055)),.UNSPECIFIED.,
 .F.,.F.,.F.)
B_SPLINE_SURFACE_WITH_KNOTS((6,1,1,1,1,1,1,1,1,1,1,1,1,1,1,1,1,1,1,1,1,
1,1,1,1,1,1,1,1,1,1,1,1,1,1,1,1,1,1,1,1,1,1,1,1,1,1,1,1,1,1,1,1,1,1,1,1,
1,1,1,1,1,1,1,1,1,1,1,1,1,1,1,1,1,1,1,1,1,1,1,1,1,1,1,1,1,1,1,1,1,1,1,1,
1,1,1,1,1,1,1,1,1,1,1,1,1,1,1,1,1,1,1,1,1,1,1,1,1,1,1,1,1,1,1,1,1,1,1,1,
1,1,1,1,1,1,1,1,1,1,1,1,1,1,1,1,1,1,1,1,1,1,1,1,1,1,1,1,1,1,1,1,1,1,1,1,
1,1,1,1,1,1,1,1,1,1,1,1,1,1,1,1,1,1,1,1,1,1,1,1,1,1,1,1,1,1,1,1,1,1,1,6),
(2,2),(0.,0.005,0.01,0.015,0.02,0.025,0.03,0.035,0.04,0.045,0.05,0.055,
0.06,0.065,0.07,0.075,0.08,0.085,0.09,0.095,0.1,0.105,0.11,0.115,0.12,0.125,
0.13,0.135,0.14,0.145,0.15,0.155,0.16,0.165,0.17,0.175,0.18,0.185,0.19,
0.195,0.2,0.205,0.21,0.215,0.22,0.225,0.23,0.235,0.24,0.245,0.25,0.255,
0.26,0.265,0.27,0.275,0.28,0.285,0.29,0.295,0.3,0.305,0.31,0.315,0.32,0.325,
0.33,0.335,0.34,0.345,0.35,0.355,0.36,0.365,0.37,0.375,0.38,0.385,0.39,
0.395,0.4,0.405,0.41,0.415,0.42,0.425,0.43,0.435,0.44,0.445,0.45,0.455,
0.46,0.465,0.47,0.475,0.48,0.485,0.49,0.495,0.5,0.505,0.51,0.515,0.52,0.525,
0.53,0.535,0.54,0.545,0.55,0.555,0.56,0.565,0.57,0.575,0.58,0.585,0.59,
0.595,0.6,0.605,0.61,0.615,0.62,0.625,0.63,0.635,0.64,0.645,0.65,0.655,
0.66,0.665,0.67,0.675,0.68,0.685,0.690000000000001,0.695000000000001,0.700000000000001,
0.705000000000001,0.710000000000001,0.715000000000001,0.720000000000001,
0.725000000000001,0.730000000000001,0.735000000000001,0.740000000000001,
0.745000000000001,0.750000000000001,0.755000000000001,0.760000000000001,
0.765000000000001,0.770000000000001,0.775000000000001,0.780000000000001,
0.785000000000001,0.790000000000001,0.795000000000001,0.800000000000001,
0.805000000000001,0.810000000000001,0.815000000000001,0.820000000000001,
0.825000000000001,0.830000000000001,0.835000000000001,0.840000000000001,
0.845000000000001,0.850000000000001,0.855000000000001,0.860000000000001,
0.865000000000001,0.870000000000001,0.875000000000001,0.880000000000001,
0.885000000000001,0.890000000000001,0.895000000000001,0.900000000000001,
0.905000000000001,0.910000000000001,0.915000000000001,0.920000000000001,
0.925000000000001,0.930000000000001,0.935000000000001,0.940000000000001,
0.945000000000001,0.950000000000001,0.955000000000001,0.960000000000001,
0.965000000000001,0.970000000000001,0.975000000000001,0.980000000000001,
0.985000000000001,0.990000000000001,0.995000000000001,1.),(0.,1.2),
 .UNSPECIFIED.)
GEOMETRIC_REPRESENTATION_ITEM()
RATIONAL_B_SPLINE_SURFACE(((1.,1.),(1.,1.),(1.,1.),(1.,1.),(1.,1.),(1.,
1.),(1.,1.),(1.,1.),(1.,1.),(1.,1.),(1.,1.),(1.,1.),(1.,1.),(1.,1.),(1.,
1.),(1.,1.),(1.,1.),(1.,1.),(1.,1.),(1.,1.),(1.,1.),(1.,1.),(1.,1.),(1.,
1.),(1.,1.),(1.,1.),(1.,1.),(1.,1.),(1.,1.),(1.,1.),(1.,1.),(1.,1.),(1.,
1.),(1.,1.),(1.,1.),(1.,1.),(1.,1.),(1.,1.),(1.,1.),(1.,1.),(1.,1.),(1.,
1.),(1.,1.),(1.,1.),(1.,1.),(1.,1.),(1.,1.),(1.,1.),(1.,1.),(1.,1.),(1.,
1.),(1.,1.),(1.,1.),(1.,1.),(1.,1.),(1.,1.),(1.,1.),(1.,1.),(1.,1.),(1.,
1.),(1.,1.),(1.,1.),(1.,1.),(1.,1.),(1.,1.),(1.,1.),(1.,1.),(1.,1.),(1.,
1.),(1.,1.),(1.,1.),(1.,1.),(1.,1.),(1.,1.),(1.,1.),(1.,1.),(1.,1.),(1.,
1.),(1.,1.),(1.,1.),(1.,1.),(1.,1.),(1.,1.),(1.,1.),(1.,1.),(1.,1.),(1.,
1.),(1.,1.),(1.,1.),(1.,1.),(1.,1.),(1.,1.),(1.,1.),(1.,1.),(1.,1.),(1.,
1.),(1.,1.),(1.,1.),(1.,1.),(1.,1.),(1.,1.),(1.,1.),(1.,1.),(1.,1.),(1.,
1.),(1.,1.),(1.,1.),(1.,1.),(1.,1.),(1.,1.),(1.,1.),(1.,1.),(1.,1.),(1.,
1.),(1.,1.),(1.,1.),(1.,1.),(1.,1.),(1.,1.),(1.,1.),(1.,1.),(1.,1.),(1.,
1.),(1.,1.),(1.,1.),(1.,1.),(1.,1.),(1.,1.),(1.,1.),(1.,1.),(1.,1.),(1.,
1.),(1.,1.),(1.,1.),(1.,1.),(1.,1.),(1.,1.),(1.,1.),(1.,1.),(1.,1.),(1.,
1.),(1.,1.),(1.,1.),(1.,1.),(1.,1.),(1.,1.),(1.,1.),(1.,1.),(1.,1.),(1.,
1.),(1.,1.),(1.,1.),(1.,1.),(1.,1.),(1.,1.),(1.,1.),(1.,1.),(1.,1.),(1.,
1.),(1.,1.),(1.,1.),(1.,1.),(1.,1.),(1.,1.),(1.,1.),(1.,1.),(1.,1.),(1.,
1.),(1.,1.),(1.,1.),(1.,1.),(1.,1.),(1.,1.),(1.,1.),(1.,1.),(1.,1.),(1.,
1.),(1.,1.),(1.,1.),(1.,1.),(1.,1.),(1.,1.),(1.,1.),(1.,1.),(1.,1.),(1.,
1.),(1.,1.),(1.,1.),(1.,1.),(1.,1.),(1.,1.),(1.,1.),(1.,1.),(1.,1.),(1.,
1.),(1.,1.),(1.,1.),(1.,1.),(1.,1.),(1.,1.),(1.,1.),(1.,1.),(1.,1.),(1.,
1.),(1.,1.)))
REPRESENTATION_ITEM('')
SURFACE()
);
#903=(
BOUNDED_SURFACE()
B_SPLINE_SURFACE(5,1,((#70542,#70543),(#70544,#70545),(#70546,#70547),(#70548,
#70549),(#70550,#70551),(#70552,#70553),(#70554,#70555),(#70556,#70557),
(#70558,#70559),(#70560,#70561),(#70562,#70563),(#70564,#70565),(#70566,
#70567),(#70568,#70569),(#70570,#70571),(#70572,#70573),(#70574,#70575),
(#70576,#70577),(#70578,#70579),(#70580,#70581),(#70582,#70583),(#70584,
#70585),(#70586,#70587),(#70588,#70589),(#70590,#70591),(#70592,#70593),
(#70594,#70595),(#70596,#70597),(#70598,#70599),(#70600,#70601),(#70602,
#70603),(#70604,#70605),(#70606,#70607),(#70608,#70609),(#70610,#70611),
(#70612,#70613),(#70614,#70615),(#70616,#70617),(#70618,#70619),(#70620,
#70621),(#70622,#70623),(#70624,#70625),(#70626,#70627),(#70628,#70629),
(#70630,#70631),(#70632,#70633),(#70634,#70635),(#70636,#70637),(#70638,
#70639),(#70640,#70641),(#70642,#70643),(#70644,#70645),(#70646,#70647),
(#70648,#70649),(#70650,#70651),(#70652,#70653),(#70654,#70655),(#70656,
#70657),(#70658,#70659),(#70660,#70661),(#70662,#70663),(#70664,#70665),
(#70666,#70667),(#70668,#70669),(#70670,#70671),(#70672,#70673),(#70674,
#70675),(#70676,#70677),(#70678,#70679),(#70680,#70681),(#70682,#70683),
(#70684,#70685),(#70686,#70687),(#70688,#70689),(#70690,#70691),(#70692,
#70693),(#70694,#70695),(#70696,#70697),(#70698,#70699),(#70700,#70701),
(#70702,#70703),(#70704,#70705),(#70706,#70707),(#70708,#70709),(#70710,
#70711),(#70712,#70713),(#70714,#70715),(#70716,#70717),(#70718,#70719),
(#70720,#70721),(#70722,#70723),(#70724,#70725),(#70726,#70727),(#70728,
#70729),(#70730,#70731),(#70732,#70733),(#70734,#70735),(#70736,#70737),
(#70738,#70739),(#70740,#70741),(#70742,#70743),(#70744,#70745),(#70746,
#70747),(#70748,#70749),(#70750,#70751),(#70752,#70753),(#70754,#70755),
(#70756,#70757),(#70758,#70759),(#70760,#70761),(#70762,#70763),(#70764,
#70765),(#70766,#70767),(#70768,#70769),(#70770,#70771),(#70772,#70773),
(#70774,#70775),(#70776,#70777),(#70778,#70779),(#70780,#70781),(#70782,
#70783),(#70784,#70785),(#70786,#70787),(#70788,#70789),(#70790,#70791),
(#70792,#70793),(#70794,#70795),(#70796,#70797),(#70798,#70799),(#70800,
#70801),(#70802,#70803),(#70804,#70805),(#70806,#70807),(#70808,#70809),
(#70810,#70811),(#70812,#70813),(#70814,#70815),(#70816,#70817),(#70818,
#70819),(#70820,#70821),(#70822,#70823),(#70824,#70825),(#70826,#70827),
(#70828,#70829),(#70830,#70831),(#70832,#70833),(#70834,#70835),(#70836,
#70837),(#70838,#70839),(#70840,#70841),(#70842,#70843),(#70844,#70845),
(#70846,#70847),(#70848,#70849),(#70850,#70851),(#70852,#70853),(#70854,
#70855),(#70856,#70857),(#70858,#70859),(#70860,#70861),(#70862,#70863),
(#70864,#70865),(#70866,#70867),(#70868,#70869),(#70870,#70871),(#70872,
#70873),(#70874,#70875),(#70876,#70877),(#70878,#70879),(#70880,#70881),
(#70882,#70883),(#70884,#70885),(#70886,#70887),(#70888,#70889),(#70890,
#70891),(#70892,#70893),(#70894,#70895),(#70896,#70897),(#70898,#70899),
(#70900,#70901),(#70902,#70903),(#70904,#70905),(#70906,#70907),(#70908,
#70909),(#70910,#70911),(#70912,#70913),(#70914,#70915),(#70916,#70917),
(#70918,#70919),(#70920,#70921),(#70922,#70923),(#70924,#70925),(#70926,
#70927),(#70928,#70929),(#70930,#70931),(#70932,#70933),(#70934,#70935),
(#70936,#70937),(#70938,#70939),(#70940,#70941),(#70942,#70943),(#70944,
#70945),(#70946,#70947),(#70948,#70949),(#70950,#70951)),.UNSPECIFIED.,
 .F.,.F.,.F.)
B_SPLINE_SURFACE_WITH_KNOTS((6,1,1,1,1,1,1,1,1,1,1,1,1,1,1,1,1,1,1,1,1,
1,1,1,1,1,1,1,1,1,1,1,1,1,1,1,1,1,1,1,1,1,1,1,1,1,1,1,1,1,1,1,1,1,1,1,1,
1,1,1,1,1,1,1,1,1,1,1,1,1,1,1,1,1,1,1,1,1,1,1,1,1,1,1,1,1,1,1,1,1,1,1,1,
1,1,1,1,1,1,1,1,1,1,1,1,1,1,1,1,1,1,1,1,1,1,1,1,1,1,1,1,1,1,1,1,1,1,1,1,
1,1,1,1,1,1,1,1,1,1,1,1,1,1,1,1,1,1,1,1,1,1,1,1,1,1,1,1,1,1,1,1,1,1,1,1,
1,1,1,1,1,1,1,1,1,1,1,1,1,1,1,1,1,1,1,1,1,1,1,1,1,1,1,1,1,1,1,1,1,1,1,6),
(2,2),(0.,0.005,0.01,0.015,0.02,0.025,0.03,0.035,0.04,0.045,0.05,0.055,
0.06,0.065,0.07,0.075,0.08,0.085,0.09,0.095,0.1,0.105,0.11,0.115,0.12,0.125,
0.13,0.135,0.14,0.145,0.15,0.155,0.16,0.165,0.17,0.175,0.18,0.185,0.19,
0.195,0.2,0.205,0.21,0.215,0.22,0.225,0.23,0.235,0.24,0.245,0.25,0.255,
0.26,0.265,0.27,0.275,0.28,0.285,0.29,0.295,0.3,0.305,0.31,0.315,0.32,0.325,
0.33,0.335,0.34,0.345,0.35,0.355,0.36,0.365,0.37,0.375,0.38,0.385,0.39,
0.395,0.4,0.405,0.41,0.415,0.42,0.425,0.43,0.435,0.44,0.445,0.45,0.455,
0.46,0.465,0.47,0.475,0.48,0.485,0.49,0.495,0.5,0.505,0.51,0.515,0.52,0.525,
0.53,0.535,0.54,0.545,0.55,0.555,0.56,0.565,0.57,0.575,0.58,0.585,0.59,
0.595,0.6,0.605,0.61,0.615,0.62,0.625,0.63,0.635,0.64,0.645,0.65,0.655,
0.66,0.665,0.67,0.675,0.68,0.685,0.690000000000001,0.695000000000001,0.700000000000001,
0.705000000000001,0.710000000000001,0.715000000000001,0.720000000000001,
0.725000000000001,0.730000000000001,0.735000000000001,0.740000000000001,
0.745000000000001,0.750000000000001,0.755000000000001,0.760000000000001,
0.765000000000001,0.770000000000001,0.775000000000001,0.780000000000001,
0.785000000000001,0.790000000000001,0.795000000000001,0.800000000000001,
0.805000000000001,0.810000000000001,0.815000000000001,0.820000000000001,
0.825000000000001,0.830000000000001,0.835000000000001,0.840000000000001,
0.845000000000001,0.850000000000001,0.855000000000001,0.860000000000001,
0.865000000000001,0.870000000000001,0.875000000000001,0.880000000000001,
0.885000000000001,0.890000000000001,0.895000000000001,0.900000000000001,
0.905000000000001,0.910000000000001,0.915000000000001,0.920000000000001,
0.925000000000001,0.930000000000001,0.935000000000001,0.940000000000001,
0.945000000000001,0.950000000000001,0.955000000000001,0.960000000000001,
0.965000000000001,0.970000000000001,0.975000000000001,0.980000000000001,
0.985000000000001,0.990000000000001,0.995000000000001,1.),(0.,1.2),
 .UNSPECIFIED.)
GEOMETRIC_REPRESENTATION_ITEM()
RATIONAL_B_SPLINE_SURFACE(((1.,1.),(1.,1.),(1.,1.),(1.,1.),(1.,1.),(1.,
1.),(1.,1.),(1.,1.),(1.,1.),(1.,1.),(1.,1.),(1.,1.),(1.,1.),(1.,1.),(1.,
1.),(1.,1.),(1.,1.),(1.,1.),(1.,1.),(1.,1.),(1.,1.),(1.,1.),(1.,1.),(1.,
1.),(1.,1.),(1.,1.),(1.,1.),(1.,1.),(1.,1.),(1.,1.),(1.,1.),(1.,1.),(1.,
1.),(1.,1.),(1.,1.),(1.,1.),(1.,1.),(1.,1.),(1.,1.),(1.,1.),(1.,1.),(1.,
1.),(1.,1.),(1.,1.),(1.,1.),(1.,1.),(1.,1.),(1.,1.),(1.,1.),(1.,1.),(1.,
1.),(1.,1.),(1.,1.),(1.,1.),(1.,1.),(1.,1.),(1.,1.),(1.,1.),(1.,1.),(1.,
1.),(1.,1.),(1.,1.),(1.,1.),(1.,1.),(1.,1.),(1.,1.),(1.,1.),(1.,1.),(1.,
1.),(1.,1.),(1.,1.),(1.,1.),(1.,1.),(1.,1.),(1.,1.),(1.,1.),(1.,1.),(1.,
1.),(1.,1.),(1.,1.),(1.,1.),(1.,1.),(1.,1.),(1.,1.),(1.,1.),(1.,1.),(1.,
1.),(1.,1.),(1.,1.),(1.,1.),(1.,1.),(1.,1.),(1.,1.),(1.,1.),(1.,1.),(1.,
1.),(1.,1.),(1.,1.),(1.,1.),(1.,1.),(1.,1.),(1.,1.),(1.,1.),(1.,1.),(1.,
1.),(1.,1.),(1.,1.),(1.,1.),(1.,1.),(1.,1.),(1.,1.),(1.,1.),(1.,1.),(1.,
1.),(1.,1.),(1.,1.),(1.,1.),(1.,1.),(1.,1.),(1.,1.),(1.,1.),(1.,1.),(1.,
1.),(1.,1.),(1.,1.),(1.,1.),(1.,1.),(1.,1.),(1.,1.),(1.,1.),(1.,1.),(1.,
1.),(1.,1.),(1.,1.),(1.,1.),(1.,1.),(1.,1.),(1.,1.),(1.,1.),(1.,1.),(1.,
1.),(1.,1.),(1.,1.),(1.,1.),(1.,1.),(1.,1.),(1.,1.),(1.,1.),(1.,1.),(1.,
1.),(1.,1.),(1.,1.),(1.,1.),(1.,1.),(1.,1.),(1.,1.),(1.,1.),(1.,1.),(1.,
1.),(1.,1.),(1.,1.),(1.,1.),(1.,1.),(1.,1.),(1.,1.),(1.,1.),(1.,1.),(1.,
1.),(1.,1.),(1.,1.),(1.,1.),(1.,1.),(1.,1.),(1.,1.),(1.,1.),(1.,1.),(1.,
1.),(1.,1.),(1.,1.),(1.,1.),(1.,1.),(1.,1.),(1.,1.),(1.,1.),(1.,1.),(1.,
1.),(1.,1.),(1.,1.),(1.,1.),(1.,1.),(1.,1.),(1.,1.),(1.,1.),(1.,1.),(1.,
1.),(1.,1.),(1.,1.),(1.,1.),(1.,1.),(1.,1.),(1.,1.),(1.,1.),(1.,1.),(1.,
1.),(1.,1.)))
REPRESENTATION_ITEM('')
SURFACE()
);
#904=(
BOUNDED_SURFACE()
B_SPLINE_SURFACE(5,1,((#71438,#71439),(#71440,#71441),(#71442,#71443),(#71444,
#71445),(#71446,#71447),(#71448,#71449),(#71450,#71451),(#71452,#71453),
(#71454,#71455),(#71456,#71457),(#71458,#71459),(#71460,#71461),(#71462,
#71463),(#71464,#71465),(#71466,#71467),(#71468,#71469),(#71470,#71471),
(#71472,#71473),(#71474,#71475),(#71476,#71477),(#71478,#71479),(#71480,
#71481),(#71482,#71483),(#71484,#71485),(#71486,#71487),(#71488,#71489),
(#71490,#71491),(#71492,#71493),(#71494,#71495),(#71496,#71497),(#71498,
#71499),(#71500,#71501),(#71502,#71503),(#71504,#71505),(#71506,#71507),
(#71508,#71509),(#71510,#71511),(#71512,#71513),(#71514,#71515),(#71516,
#71517),(#71518,#71519),(#71520,#71521),(#71522,#71523),(#71524,#71525),
(#71526,#71527),(#71528,#71529),(#71530,#71531),(#71532,#71533),(#71534,
#71535),(#71536,#71537),(#71538,#71539),(#71540,#71541),(#71542,#71543),
(#71544,#71545),(#71546,#71547),(#71548,#71549),(#71550,#71551),(#71552,
#71553),(#71554,#71555),(#71556,#71557),(#71558,#71559),(#71560,#71561),
(#71562,#71563),(#71564,#71565),(#71566,#71567),(#71568,#71569),(#71570,
#71571),(#71572,#71573),(#71574,#71575),(#71576,#71577),(#71578,#71579),
(#71580,#71581),(#71582,#71583),(#71584,#71585),(#71586,#71587),(#71588,
#71589),(#71590,#71591),(#71592,#71593),(#71594,#71595),(#71596,#71597),
(#71598,#71599),(#71600,#71601),(#71602,#71603),(#71604,#71605),(#71606,
#71607),(#71608,#71609),(#71610,#71611),(#71612,#71613),(#71614,#71615),
(#71616,#71617),(#71618,#71619),(#71620,#71621),(#71622,#71623),(#71624,
#71625),(#71626,#71627),(#71628,#71629),(#71630,#71631),(#71632,#71633),
(#71634,#71635),(#71636,#71637),(#71638,#71639),(#71640,#71641),(#71642,
#71643),(#71644,#71645),(#71646,#71647),(#71648,#71649),(#71650,#71651),
(#71652,#71653),(#71654,#71655),(#71656,#71657),(#71658,#71659),(#71660,
#71661),(#71662,#71663),(#71664,#71665),(#71666,#71667),(#71668,#71669),
(#71670,#71671),(#71672,#71673),(#71674,#71675),(#71676,#71677),(#71678,
#71679),(#71680,#71681),(#71682,#71683),(#71684,#71685),(#71686,#71687),
(#71688,#71689),(#71690,#71691),(#71692,#71693),(#71694,#71695),(#71696,
#71697),(#71698,#71699),(#71700,#71701),(#71702,#71703),(#71704,#71705),
(#71706,#71707),(#71708,#71709),(#71710,#71711),(#71712,#71713),(#71714,
#71715),(#71716,#71717),(#71718,#71719),(#71720,#71721),(#71722,#71723),
(#71724,#71725),(#71726,#71727),(#71728,#71729),(#71730,#71731),(#71732,
#71733),(#71734,#71735),(#71736,#71737),(#71738,#71739),(#71740,#71741),
(#71742,#71743),(#71744,#71745),(#71746,#71747),(#71748,#71749),(#71750,
#71751),(#71752,#71753),(#71754,#71755),(#71756,#71757),(#71758,#71759),
(#71760,#71761),(#71762,#71763),(#71764,#71765),(#71766,#71767),(#71768,
#71769),(#71770,#71771),(#71772,#71773),(#71774,#71775),(#71776,#71777),
(#71778,#71779),(#71780,#71781),(#71782,#71783),(#71784,#71785),(#71786,
#71787),(#71788,#71789),(#71790,#71791),(#71792,#71793),(#71794,#71795),
(#71796,#71797),(#71798,#71799),(#71800,#71801),(#71802,#71803),(#71804,
#71805),(#71806,#71807),(#71808,#71809),(#71810,#71811),(#71812,#71813),
(#71814,#71815),(#71816,#71817),(#71818,#71819),(#71820,#71821),(#71822,
#71823),(#71824,#71825),(#71826,#71827),(#71828,#71829),(#71830,#71831),
(#71832,#71833),(#71834,#71835),(#71836,#71837),(#71838,#71839),(#71840,
#71841),(#71842,#71843),(#71844,#71845),(#71846,#71847)),.UNSPECIFIED.,
 .F.,.F.,.F.)
B_SPLINE_SURFACE_WITH_KNOTS((6,1,1,1,1,1,1,1,1,1,1,1,1,1,1,1,1,1,1,1,1,
1,1,1,1,1,1,1,1,1,1,1,1,1,1,1,1,1,1,1,1,1,1,1,1,1,1,1,1,1,1,1,1,1,1,1,1,
1,1,1,1,1,1,1,1,1,1,1,1,1,1,1,1,1,1,1,1,1,1,1,1,1,1,1,1,1,1,1,1,1,1,1,1,
1,1,1,1,1,1,1,1,1,1,1,1,1,1,1,1,1,1,1,1,1,1,1,1,1,1,1,1,1,1,1,1,1,1,1,1,
1,1,1,1,1,1,1,1,1,1,1,1,1,1,1,1,1,1,1,1,1,1,1,1,1,1,1,1,1,1,1,1,1,1,1,1,
1,1,1,1,1,1,1,1,1,1,1,1,1,1,1,1,1,1,1,1,1,1,1,1,1,1,1,1,1,1,1,1,1,1,1,6),
(2,2),(0.,0.005,0.01,0.015,0.02,0.025,0.03,0.035,0.04,0.045,0.05,0.055,
0.06,0.065,0.07,0.075,0.08,0.085,0.09,0.095,0.1,0.105,0.11,0.115,0.12,0.125,
0.13,0.135,0.14,0.145,0.15,0.155,0.16,0.165,0.17,0.175,0.18,0.185,0.19,
0.195,0.2,0.205,0.21,0.215,0.22,0.225,0.23,0.235,0.24,0.245,0.25,0.255,
0.26,0.265,0.27,0.275,0.28,0.285,0.29,0.295,0.3,0.305,0.31,0.315,0.32,0.325,
0.33,0.335,0.34,0.345,0.35,0.355,0.36,0.365,0.37,0.375,0.38,0.385,0.39,
0.395,0.4,0.405,0.41,0.415,0.42,0.425,0.43,0.435,0.44,0.445,0.45,0.455,
0.46,0.465,0.47,0.475,0.48,0.485,0.49,0.495,0.5,0.505,0.51,0.515,0.52,0.525,
0.53,0.535,0.54,0.545,0.55,0.555,0.56,0.565,0.57,0.575,0.58,0.585,0.59,
0.595,0.6,0.605,0.61,0.615,0.62,0.625,0.63,0.635,0.64,0.645,0.65,0.655,
0.66,0.665,0.67,0.675,0.68,0.685,0.690000000000001,0.695000000000001,0.700000000000001,
0.705000000000001,0.710000000000001,0.715000000000001,0.720000000000001,
0.725000000000001,0.730000000000001,0.735000000000001,0.740000000000001,
0.745000000000001,0.750000000000001,0.755000000000001,0.760000000000001,
0.765000000000001,0.770000000000001,0.775000000000001,0.780000000000001,
0.785000000000001,0.790000000000001,0.795000000000001,0.800000000000001,
0.805000000000001,0.810000000000001,0.815000000000001,0.820000000000001,
0.825000000000001,0.830000000000001,0.835000000000001,0.840000000000001,
0.845000000000001,0.850000000000001,0.855000000000001,0.860000000000001,
0.865000000000001,0.870000000000001,0.875000000000001,0.880000000000001,
0.885000000000001,0.890000000000001,0.895000000000001,0.900000000000001,
0.905000000000001,0.910000000000001,0.915000000000001,0.920000000000001,
0.925000000000001,0.930000000000001,0.935000000000001,0.940000000000001,
0.945000000000001,0.950000000000001,0.955000000000001,0.960000000000001,
0.965000000000001,0.970000000000001,0.975000000000001,0.980000000000001,
0.985000000000001,0.990000000000001,0.995000000000001,1.),(0.,1.2),
 .UNSPECIFIED.)
GEOMETRIC_REPRESENTATION_ITEM()
RATIONAL_B_SPLINE_SURFACE(((1.,1.),(1.,1.),(1.,1.),(1.,1.),(1.,1.),(1.,
1.),(1.,1.),(1.,1.),(1.,1.),(1.,1.),(1.,1.),(1.,1.),(1.,1.),(1.,1.),(1.,
1.),(1.,1.),(1.,1.),(1.,1.),(1.,1.),(1.,1.),(1.,1.),(1.,1.),(1.,1.),(1.,
1.),(1.,1.),(1.,1.),(1.,1.),(1.,1.),(1.,1.),(1.,1.),(1.,1.),(1.,1.),(1.,
1.),(1.,1.),(1.,1.),(1.,1.),(1.,1.),(1.,1.),(1.,1.),(1.,1.),(1.,1.),(1.,
1.),(1.,1.),(1.,1.),(1.,1.),(1.,1.),(1.,1.),(1.,1.),(1.,1.),(1.,1.),(1.,
1.),(1.,1.),(1.,1.),(1.,1.),(1.,1.),(1.,1.),(1.,1.),(1.,1.),(1.,1.),(1.,
1.),(1.,1.),(1.,1.),(1.,1.),(1.,1.),(1.,1.),(1.,1.),(1.,1.),(1.,1.),(1.,
1.),(1.,1.),(1.,1.),(1.,1.),(1.,1.),(1.,1.),(1.,1.),(1.,1.),(1.,1.),(1.,
1.),(1.,1.),(1.,1.),(1.,1.),(1.,1.),(1.,1.),(1.,1.),(1.,1.),(1.,1.),(1.,
1.),(1.,1.),(1.,1.),(1.,1.),(1.,1.),(1.,1.),(1.,1.),(1.,1.),(1.,1.),(1.,
1.),(1.,1.),(1.,1.),(1.,1.),(1.,1.),(1.,1.),(1.,1.),(1.,1.),(1.,1.),(1.,
1.),(1.,1.),(1.,1.),(1.,1.),(1.,1.),(1.,1.),(1.,1.),(1.,1.),(1.,1.),(1.,
1.),(1.,1.),(1.,1.),(1.,1.),(1.,1.),(1.,1.),(1.,1.),(1.,1.),(1.,1.),(1.,
1.),(1.,1.),(1.,1.),(1.,1.),(1.,1.),(1.,1.),(1.,1.),(1.,1.),(1.,1.),(1.,
1.),(1.,1.),(1.,1.),(1.,1.),(1.,1.),(1.,1.),(1.,1.),(1.,1.),(1.,1.),(1.,
1.),(1.,1.),(1.,1.),(1.,1.),(1.,1.),(1.,1.),(1.,1.),(1.,1.),(1.,1.),(1.,
1.),(1.,1.),(1.,1.),(1.,1.),(1.,1.),(1.,1.),(1.,1.),(1.,1.),(1.,1.),(1.,
1.),(1.,1.),(1.,1.),(1.,1.),(1.,1.),(1.,1.),(1.,1.),(1.,1.),(1.,1.),(1.,
1.),(1.,1.),(1.,1.),(1.,1.),(1.,1.),(1.,1.),(1.,1.),(1.,1.),(1.,1.),(1.,
1.),(1.,1.),(1.,1.),(1.,1.),(1.,1.),(1.,1.),(1.,1.),(1.,1.),(1.,1.),(1.,
1.),(1.,1.),(1.,1.),(1.,1.),(1.,1.),(1.,1.),(1.,1.),(1.,1.),(1.,1.),(1.,
1.),(1.,1.),(1.,1.),(1.,1.),(1.,1.),(1.,1.),(1.,1.),(1.,1.),(1.,1.),(1.,
1.),(1.,1.)))
REPRESENTATION_ITEM('')
SURFACE()
);
#905=(
BOUNDED_SURFACE()
B_SPLINE_SURFACE(5,1,((#72334,#72335),(#72336,#72337),(#72338,#72339),(#72340,
#72341),(#72342,#72343),(#72344,#72345),(#72346,#72347),(#72348,#72349),
(#72350,#72351),(#72352,#72353),(#72354,#72355),(#72356,#72357),(#72358,
#72359),(#72360,#72361),(#72362,#72363),(#72364,#72365),(#72366,#72367),
(#72368,#72369),(#72370,#72371),(#72372,#72373),(#72374,#72375),(#72376,
#72377),(#72378,#72379),(#72380,#72381),(#72382,#72383),(#72384,#72385),
(#72386,#72387),(#72388,#72389),(#72390,#72391),(#72392,#72393),(#72394,
#72395),(#72396,#72397),(#72398,#72399),(#72400,#72401),(#72402,#72403),
(#72404,#72405),(#72406,#72407),(#72408,#72409),(#72410,#72411),(#72412,
#72413),(#72414,#72415),(#72416,#72417),(#72418,#72419),(#72420,#72421),
(#72422,#72423),(#72424,#72425),(#72426,#72427),(#72428,#72429),(#72430,
#72431),(#72432,#72433),(#72434,#72435),(#72436,#72437),(#72438,#72439),
(#72440,#72441),(#72442,#72443),(#72444,#72445),(#72446,#72447),(#72448,
#72449),(#72450,#72451),(#72452,#72453),(#72454,#72455),(#72456,#72457),
(#72458,#72459),(#72460,#72461),(#72462,#72463),(#72464,#72465),(#72466,
#72467),(#72468,#72469),(#72470,#72471),(#72472,#72473),(#72474,#72475),
(#72476,#72477),(#72478,#72479),(#72480,#72481),(#72482,#72483),(#72484,
#72485),(#72486,#72487),(#72488,#72489),(#72490,#72491),(#72492,#72493),
(#72494,#72495),(#72496,#72497),(#72498,#72499),(#72500,#72501),(#72502,
#72503),(#72504,#72505),(#72506,#72507),(#72508,#72509),(#72510,#72511),
(#72512,#72513),(#72514,#72515),(#72516,#72517),(#72518,#72519),(#72520,
#72521),(#72522,#72523),(#72524,#72525),(#72526,#72527),(#72528,#72529),
(#72530,#72531),(#72532,#72533),(#72534,#72535),(#72536,#72537),(#72538,
#72539),(#72540,#72541),(#72542,#72543),(#72544,#72545),(#72546,#72547),
(#72548,#72549),(#72550,#72551),(#72552,#72553),(#72554,#72555),(#72556,
#72557),(#72558,#72559),(#72560,#72561),(#72562,#72563),(#72564,#72565),
(#72566,#72567),(#72568,#72569),(#72570,#72571),(#72572,#72573),(#72574,
#72575),(#72576,#72577),(#72578,#72579),(#72580,#72581),(#72582,#72583),
(#72584,#72585),(#72586,#72587),(#72588,#72589),(#72590,#72591),(#72592,
#72593),(#72594,#72595),(#72596,#72597),(#72598,#72599),(#72600,#72601),
(#72602,#72603),(#72604,#72605),(#72606,#72607),(#72608,#72609),(#72610,
#72611),(#72612,#72613),(#72614,#72615),(#72616,#72617),(#72618,#72619),
(#72620,#72621),(#72622,#72623),(#72624,#72625),(#72626,#72627),(#72628,
#72629),(#72630,#72631),(#72632,#72633),(#72634,#72635),(#72636,#72637),
(#72638,#72639),(#72640,#72641),(#72642,#72643),(#72644,#72645),(#72646,
#72647),(#72648,#72649),(#72650,#72651),(#72652,#72653),(#72654,#72655),
(#72656,#72657),(#72658,#72659),(#72660,#72661),(#72662,#72663),(#72664,
#72665),(#72666,#72667),(#72668,#72669),(#72670,#72671),(#72672,#72673),
(#72674,#72675),(#72676,#72677),(#72678,#72679),(#72680,#72681),(#72682,
#72683),(#72684,#72685),(#72686,#72687),(#72688,#72689),(#72690,#72691),
(#72692,#72693),(#72694,#72695),(#72696,#72697),(#72698,#72699),(#72700,
#72701),(#72702,#72703),(#72704,#72705),(#72706,#72707),(#72708,#72709),
(#72710,#72711),(#72712,#72713),(#72714,#72715),(#72716,#72717),(#72718,
#72719),(#72720,#72721),(#72722,#72723),(#72724,#72725),(#72726,#72727),
(#72728,#72729),(#72730,#72731),(#72732,#72733),(#72734,#72735),(#72736,
#72737),(#72738,#72739),(#72740,#72741),(#72742,#72743)),.UNSPECIFIED.,
 .F.,.F.,.F.)
B_SPLINE_SURFACE_WITH_KNOTS((6,1,1,1,1,1,1,1,1,1,1,1,1,1,1,1,1,1,1,1,1,
1,1,1,1,1,1,1,1,1,1,1,1,1,1,1,1,1,1,1,1,1,1,1,1,1,1,1,1,1,1,1,1,1,1,1,1,
1,1,1,1,1,1,1,1,1,1,1,1,1,1,1,1,1,1,1,1,1,1,1,1,1,1,1,1,1,1,1,1,1,1,1,1,
1,1,1,1,1,1,1,1,1,1,1,1,1,1,1,1,1,1,1,1,1,1,1,1,1,1,1,1,1,1,1,1,1,1,1,1,
1,1,1,1,1,1,1,1,1,1,1,1,1,1,1,1,1,1,1,1,1,1,1,1,1,1,1,1,1,1,1,1,1,1,1,1,
1,1,1,1,1,1,1,1,1,1,1,1,1,1,1,1,1,1,1,1,1,1,1,1,1,1,1,1,1,1,1,1,1,1,1,6),
(2,2),(0.,0.005,0.01,0.015,0.02,0.025,0.03,0.035,0.04,0.045,0.05,0.055,
0.06,0.065,0.07,0.075,0.08,0.085,0.09,0.095,0.1,0.105,0.11,0.115,0.12,0.125,
0.13,0.135,0.14,0.145,0.15,0.155,0.16,0.165,0.17,0.175,0.18,0.185,0.19,
0.195,0.2,0.205,0.21,0.215,0.22,0.225,0.23,0.235,0.24,0.245,0.25,0.255,
0.26,0.265,0.27,0.275,0.28,0.285,0.29,0.295,0.3,0.305,0.31,0.315,0.32,0.325,
0.33,0.335,0.34,0.345,0.35,0.355,0.36,0.365,0.37,0.375,0.38,0.385,0.39,
0.395,0.4,0.405,0.41,0.415,0.42,0.425,0.43,0.435,0.44,0.445,0.45,0.455,
0.46,0.465,0.47,0.475,0.48,0.485,0.49,0.495,0.5,0.505,0.51,0.515,0.52,0.525,
0.53,0.535,0.54,0.545,0.55,0.555,0.56,0.565,0.57,0.575,0.58,0.585,0.59,
0.595,0.6,0.605,0.61,0.615,0.62,0.625,0.63,0.635,0.64,0.645,0.65,0.655,
0.66,0.665,0.67,0.675,0.68,0.685,0.690000000000001,0.695000000000001,0.700000000000001,
0.705000000000001,0.710000000000001,0.715000000000001,0.720000000000001,
0.725000000000001,0.730000000000001,0.735000000000001,0.740000000000001,
0.745000000000001,0.750000000000001,0.755000000000001,0.760000000000001,
0.765000000000001,0.770000000000001,0.775000000000001,0.780000000000001,
0.785000000000001,0.790000000000001,0.795000000000001,0.800000000000001,
0.805000000000001,0.810000000000001,0.815000000000001,0.820000000000001,
0.825000000000001,0.830000000000001,0.835000000000001,0.840000000000001,
0.845000000000001,0.850000000000001,0.855000000000001,0.860000000000001,
0.865000000000001,0.870000000000001,0.875000000000001,0.880000000000001,
0.885000000000001,0.890000000000001,0.895000000000001,0.900000000000001,
0.905000000000001,0.910000000000001,0.915000000000001,0.920000000000001,
0.925000000000001,0.930000000000001,0.935000000000001,0.940000000000001,
0.945000000000001,0.950000000000001,0.955000000000001,0.960000000000001,
0.965000000000001,0.970000000000001,0.975000000000001,0.980000000000001,
0.985000000000001,0.990000000000001,0.995000000000001,1.),(0.,1.2),
 .UNSPECIFIED.)
GEOMETRIC_REPRESENTATION_ITEM()
RATIONAL_B_SPLINE_SURFACE(((1.,1.),(1.,1.),(1.,1.),(1.,1.),(1.,1.),(1.,
1.),(1.,1.),(1.,1.),(1.,1.),(1.,1.),(1.,1.),(1.,1.),(1.,1.),(1.,1.),(1.,
1.),(1.,1.),(1.,1.),(1.,1.),(1.,1.),(1.,1.),(1.,1.),(1.,1.),(1.,1.),(1.,
1.),(1.,1.),(1.,1.),(1.,1.),(1.,1.),(1.,1.),(1.,1.),(1.,1.),(1.,1.),(1.,
1.),(1.,1.),(1.,1.),(1.,1.),(1.,1.),(1.,1.),(1.,1.),(1.,1.),(1.,1.),(1.,
1.),(1.,1.),(1.,1.),(1.,1.),(1.,1.),(1.,1.),(1.,1.),(1.,1.),(1.,1.),(1.,
1.),(1.,1.),(1.,1.),(1.,1.),(1.,1.),(1.,1.),(1.,1.),(1.,1.),(1.,1.),(1.,
1.),(1.,1.),(1.,1.),(1.,1.),(1.,1.),(1.,1.),(1.,1.),(1.,1.),(1.,1.),(1.,
1.),(1.,1.),(1.,1.),(1.,1.),(1.,1.),(1.,1.),(1.,1.),(1.,1.),(1.,1.),(1.,
1.),(1.,1.),(1.,1.),(1.,1.),(1.,1.),(1.,1.),(1.,1.),(1.,1.),(1.,1.),(1.,
1.),(1.,1.),(1.,1.),(1.,1.),(1.,1.),(1.,1.),(1.,1.),(1.,1.),(1.,1.),(1.,
1.),(1.,1.),(1.,1.),(1.,1.),(1.,1.),(1.,1.),(1.,1.),(1.,1.),(1.,1.),(1.,
1.),(1.,1.),(1.,1.),(1.,1.),(1.,1.),(1.,1.),(1.,1.),(1.,1.),(1.,1.),(1.,
1.),(1.,1.),(1.,1.),(1.,1.),(1.,1.),(1.,1.),(1.,1.),(1.,1.),(1.,1.),(1.,
1.),(1.,1.),(1.,1.),(1.,1.),(1.,1.),(1.,1.),(1.,1.),(1.,1.),(1.,1.),(1.,
1.),(1.,1.),(1.,1.),(1.,1.),(1.,1.),(1.,1.),(1.,1.),(1.,1.),(1.,1.),(1.,
1.),(1.,1.),(1.,1.),(1.,1.),(1.,1.),(1.,1.),(1.,1.),(1.,1.),(1.,1.),(1.,
1.),(1.,1.),(1.,1.),(1.,1.),(1.,1.),(1.,1.),(1.,1.),(1.,1.),(1.,1.),(1.,
1.),(1.,1.),(1.,1.),(1.,1.),(1.,1.),(1.,1.),(1.,1.),(1.,1.),(1.,1.),(1.,
1.),(1.,1.),(1.,1.),(1.,1.),(1.,1.),(1.,1.),(1.,1.),(1.,1.),(1.,1.),(1.,
1.),(1.,1.),(1.,1.),(1.,1.),(1.,1.),(1.,1.),(1.,1.),(1.,1.),(1.,1.),(1.,
1.),(1.,1.),(1.,1.),(1.,1.),(1.,1.),(1.,1.),(1.,1.),(1.,1.),(1.,1.),(1.,
1.),(1.,1.),(1.,1.),(1.,1.),(1.,1.),(1.,1.),(1.,1.),(1.,1.),(1.,1.),(1.,
1.),(1.,1.)))
REPRESENTATION_ITEM('')
SURFACE()
);
#906=(
BOUNDED_SURFACE()
B_SPLINE_SURFACE(5,1,((#73230,#73231),(#73232,#73233),(#73234,#73235),(#73236,
#73237),(#73238,#73239),(#73240,#73241),(#73242,#73243),(#73244,#73245),
(#73246,#73247),(#73248,#73249),(#73250,#73251),(#73252,#73253),(#73254,
#73255),(#73256,#73257),(#73258,#73259),(#73260,#73261),(#73262,#73263),
(#73264,#73265),(#73266,#73267),(#73268,#73269),(#73270,#73271),(#73272,
#73273),(#73274,#73275),(#73276,#73277),(#73278,#73279),(#73280,#73281),
(#73282,#73283),(#73284,#73285),(#73286,#73287),(#73288,#73289),(#73290,
#73291),(#73292,#73293),(#73294,#73295),(#73296,#73297),(#73298,#73299),
(#73300,#73301),(#73302,#73303),(#73304,#73305),(#73306,#73307),(#73308,
#73309),(#73310,#73311),(#73312,#73313),(#73314,#73315),(#73316,#73317),
(#73318,#73319),(#73320,#73321),(#73322,#73323),(#73324,#73325),(#73326,
#73327),(#73328,#73329),(#73330,#73331),(#73332,#73333),(#73334,#73335),
(#73336,#73337),(#73338,#73339),(#73340,#73341),(#73342,#73343),(#73344,
#73345),(#73346,#73347),(#73348,#73349),(#73350,#73351),(#73352,#73353),
(#73354,#73355),(#73356,#73357),(#73358,#73359),(#73360,#73361),(#73362,
#73363),(#73364,#73365),(#73366,#73367),(#73368,#73369),(#73370,#73371),
(#73372,#73373),(#73374,#73375),(#73376,#73377),(#73378,#73379),(#73380,
#73381),(#73382,#73383),(#73384,#73385),(#73386,#73387),(#73388,#73389),
(#73390,#73391),(#73392,#73393),(#73394,#73395),(#73396,#73397),(#73398,
#73399),(#73400,#73401),(#73402,#73403),(#73404,#73405),(#73406,#73407),
(#73408,#73409),(#73410,#73411),(#73412,#73413),(#73414,#73415),(#73416,
#73417),(#73418,#73419),(#73420,#73421),(#73422,#73423),(#73424,#73425),
(#73426,#73427),(#73428,#73429),(#73430,#73431),(#73432,#73433),(#73434,
#73435),(#73436,#73437),(#73438,#73439),(#73440,#73441),(#73442,#73443),
(#73444,#73445),(#73446,#73447),(#73448,#73449),(#73450,#73451),(#73452,
#73453),(#73454,#73455),(#73456,#73457),(#73458,#73459),(#73460,#73461),
(#73462,#73463),(#73464,#73465),(#73466,#73467),(#73468,#73469),(#73470,
#73471),(#73472,#73473),(#73474,#73475),(#73476,#73477),(#73478,#73479),
(#73480,#73481),(#73482,#73483),(#73484,#73485),(#73486,#73487),(#73488,
#73489),(#73490,#73491),(#73492,#73493),(#73494,#73495),(#73496,#73497),
(#73498,#73499),(#73500,#73501),(#73502,#73503),(#73504,#73505),(#73506,
#73507),(#73508,#73509),(#73510,#73511),(#73512,#73513),(#73514,#73515),
(#73516,#73517),(#73518,#73519),(#73520,#73521),(#73522,#73523),(#73524,
#73525),(#73526,#73527),(#73528,#73529),(#73530,#73531),(#73532,#73533),
(#73534,#73535),(#73536,#73537),(#73538,#73539),(#73540,#73541),(#73542,
#73543),(#73544,#73545),(#73546,#73547),(#73548,#73549),(#73550,#73551),
(#73552,#73553),(#73554,#73555),(#73556,#73557),(#73558,#73559),(#73560,
#73561),(#73562,#73563),(#73564,#73565),(#73566,#73567),(#73568,#73569),
(#73570,#73571),(#73572,#73573),(#73574,#73575),(#73576,#73577),(#73578,
#73579),(#73580,#73581),(#73582,#73583),(#73584,#73585),(#73586,#73587),
(#73588,#73589),(#73590,#73591),(#73592,#73593),(#73594,#73595),(#73596,
#73597),(#73598,#73599),(#73600,#73601),(#73602,#73603),(#73604,#73605),
(#73606,#73607),(#73608,#73609),(#73610,#73611),(#73612,#73613),(#73614,
#73615),(#73616,#73617),(#73618,#73619),(#73620,#73621),(#73622,#73623),
(#73624,#73625),(#73626,#73627),(#73628,#73629),(#73630,#73631),(#73632,
#73633),(#73634,#73635),(#73636,#73637),(#73638,#73639)),.UNSPECIFIED.,
 .F.,.F.,.F.)
B_SPLINE_SURFACE_WITH_KNOTS((6,1,1,1,1,1,1,1,1,1,1,1,1,1,1,1,1,1,1,1,1,
1,1,1,1,1,1,1,1,1,1,1,1,1,1,1,1,1,1,1,1,1,1,1,1,1,1,1,1,1,1,1,1,1,1,1,1,
1,1,1,1,1,1,1,1,1,1,1,1,1,1,1,1,1,1,1,1,1,1,1,1,1,1,1,1,1,1,1,1,1,1,1,1,
1,1,1,1,1,1,1,1,1,1,1,1,1,1,1,1,1,1,1,1,1,1,1,1,1,1,1,1,1,1,1,1,1,1,1,1,
1,1,1,1,1,1,1,1,1,1,1,1,1,1,1,1,1,1,1,1,1,1,1,1,1,1,1,1,1,1,1,1,1,1,1,1,
1,1,1,1,1,1,1,1,1,1,1,1,1,1,1,1,1,1,1,1,1,1,1,1,1,1,1,1,1,1,1,1,1,1,1,6),
(2,2),(0.,0.005,0.01,0.015,0.02,0.025,0.03,0.035,0.04,0.045,0.05,0.055,
0.06,0.065,0.07,0.075,0.08,0.085,0.09,0.095,0.1,0.105,0.11,0.115,0.12,0.125,
0.13,0.135,0.14,0.145,0.15,0.155,0.16,0.165,0.17,0.175,0.18,0.185,0.19,
0.195,0.2,0.205,0.21,0.215,0.22,0.225,0.23,0.235,0.24,0.245,0.25,0.255,
0.26,0.265,0.27,0.275,0.28,0.285,0.29,0.295,0.3,0.305,0.31,0.315,0.32,0.325,
0.33,0.335,0.34,0.345,0.35,0.355,0.36,0.365,0.37,0.375,0.38,0.385,0.39,
0.395,0.4,0.405,0.41,0.415,0.42,0.425,0.43,0.435,0.44,0.445,0.45,0.455,
0.46,0.465,0.47,0.475,0.48,0.485,0.49,0.495,0.5,0.505,0.51,0.515,0.52,0.525,
0.53,0.535,0.54,0.545,0.55,0.555,0.56,0.565,0.57,0.575,0.58,0.585,0.59,
0.595,0.6,0.605,0.61,0.615,0.62,0.625,0.63,0.635,0.64,0.645,0.65,0.655,
0.66,0.665,0.67,0.675,0.68,0.685,0.690000000000001,0.695000000000001,0.700000000000001,
0.705000000000001,0.710000000000001,0.715000000000001,0.720000000000001,
0.725000000000001,0.730000000000001,0.735000000000001,0.740000000000001,
0.745000000000001,0.750000000000001,0.755000000000001,0.760000000000001,
0.765000000000001,0.770000000000001,0.775000000000001,0.780000000000001,
0.785000000000001,0.790000000000001,0.795000000000001,0.800000000000001,
0.805000000000001,0.810000000000001,0.815000000000001,0.820000000000001,
0.825000000000001,0.830000000000001,0.835000000000001,0.840000000000001,
0.845000000000001,0.850000000000001,0.855000000000001,0.860000000000001,
0.865000000000001,0.870000000000001,0.875000000000001,0.880000000000001,
0.885000000000001,0.890000000000001,0.895000000000001,0.900000000000001,
0.905000000000001,0.910000000000001,0.915000000000001,0.920000000000001,
0.925000000000001,0.930000000000001,0.935000000000001,0.940000000000001,
0.945000000000001,0.950000000000001,0.955000000000001,0.960000000000001,
0.965000000000001,0.970000000000001,0.975000000000001,0.980000000000001,
0.985000000000001,0.990000000000001,0.995000000000001,1.),(0.,1.2),
 .UNSPECIFIED.)
GEOMETRIC_REPRESENTATION_ITEM()
RATIONAL_B_SPLINE_SURFACE(((1.,1.),(1.,1.),(1.,1.),(1.,1.),(1.,1.),(1.,
1.),(1.,1.),(1.,1.),(1.,1.),(1.,1.),(1.,1.),(1.,1.),(1.,1.),(1.,1.),(1.,
1.),(1.,1.),(1.,1.),(1.,1.),(1.,1.),(1.,1.),(1.,1.),(1.,1.),(1.,1.),(1.,
1.),(1.,1.),(1.,1.),(1.,1.),(1.,1.),(1.,1.),(1.,1.),(1.,1.),(1.,1.),(1.,
1.),(1.,1.),(1.,1.),(1.,1.),(1.,1.),(1.,1.),(1.,1.),(1.,1.),(1.,1.),(1.,
1.),(1.,1.),(1.,1.),(1.,1.),(1.,1.),(1.,1.),(1.,1.),(1.,1.),(1.,1.),(1.,
1.),(1.,1.),(1.,1.),(1.,1.),(1.,1.),(1.,1.),(1.,1.),(1.,1.),(1.,1.),(1.,
1.),(1.,1.),(1.,1.),(1.,1.),(1.,1.),(1.,1.),(1.,1.),(1.,1.),(1.,1.),(1.,
1.),(1.,1.),(1.,1.),(1.,1.),(1.,1.),(1.,1.),(1.,1.),(1.,1.),(1.,1.),(1.,
1.),(1.,1.),(1.,1.),(1.,1.),(1.,1.),(1.,1.),(1.,1.),(1.,1.),(1.,1.),(1.,
1.),(1.,1.),(1.,1.),(1.,1.),(1.,1.),(1.,1.),(1.,1.),(1.,1.),(1.,1.),(1.,
1.),(1.,1.),(1.,1.),(1.,1.),(1.,1.),(1.,1.),(1.,1.),(1.,1.),(1.,1.),(1.,
1.),(1.,1.),(1.,1.),(1.,1.),(1.,1.),(1.,1.),(1.,1.),(1.,1.),(1.,1.),(1.,
1.),(1.,1.),(1.,1.),(1.,1.),(1.,1.),(1.,1.),(1.,1.),(1.,1.),(1.,1.),(1.,
1.),(1.,1.),(1.,1.),(1.,1.),(1.,1.),(1.,1.),(1.,1.),(1.,1.),(1.,1.),(1.,
1.),(1.,1.),(1.,1.),(1.,1.),(1.,1.),(1.,1.),(1.,1.),(1.,1.),(1.,1.),(1.,
1.),(1.,1.),(1.,1.),(1.,1.),(1.,1.),(1.,1.),(1.,1.),(1.,1.),(1.,1.),(1.,
1.),(1.,1.),(1.,1.),(1.,1.),(1.,1.),(1.,1.),(1.,1.),(1.,1.),(1.,1.),(1.,
1.),(1.,1.),(1.,1.),(1.,1.),(1.,1.),(1.,1.),(1.,1.),(1.,1.),(1.,1.),(1.,
1.),(1.,1.),(1.,1.),(1.,1.),(1.,1.),(1.,1.),(1.,1.),(1.,1.),(1.,1.),(1.,
1.),(1.,1.),(1.,1.),(1.,1.),(1.,1.),(1.,1.),(1.,1.),(1.,1.),(1.,1.),(1.,
1.),(1.,1.),(1.,1.),(1.,1.),(1.,1.),(1.,1.),(1.,1.),(1.,1.),(1.,1.),(1.,
1.),(1.,1.),(1.,1.),(1.,1.),(1.,1.),(1.,1.),(1.,1.),(1.,1.),(1.,1.),(1.,
1.),(1.,1.)))
REPRESENTATION_ITEM('')
SURFACE()
);
#907=(
BOUNDED_SURFACE()
B_SPLINE_SURFACE(5,1,((#74126,#74127),(#74128,#74129),(#74130,#74131),(#74132,
#74133),(#74134,#74135),(#74136,#74137),(#74138,#74139),(#74140,#74141),
(#74142,#74143),(#74144,#74145),(#74146,#74147),(#74148,#74149),(#74150,
#74151),(#74152,#74153),(#74154,#74155),(#74156,#74157),(#74158,#74159),
(#74160,#74161),(#74162,#74163),(#74164,#74165),(#74166,#74167),(#74168,
#74169),(#74170,#74171),(#74172,#74173),(#74174,#74175),(#74176,#74177),
(#74178,#74179),(#74180,#74181),(#74182,#74183),(#74184,#74185),(#74186,
#74187),(#74188,#74189),(#74190,#74191),(#74192,#74193),(#74194,#74195),
(#74196,#74197),(#74198,#74199),(#74200,#74201),(#74202,#74203),(#74204,
#74205),(#74206,#74207),(#74208,#74209),(#74210,#74211),(#74212,#74213),
(#74214,#74215),(#74216,#74217),(#74218,#74219),(#74220,#74221),(#74222,
#74223),(#74224,#74225),(#74226,#74227),(#74228,#74229),(#74230,#74231),
(#74232,#74233),(#74234,#74235),(#74236,#74237),(#74238,#74239),(#74240,
#74241),(#74242,#74243),(#74244,#74245),(#74246,#74247),(#74248,#74249),
(#74250,#74251),(#74252,#74253),(#74254,#74255),(#74256,#74257),(#74258,
#74259),(#74260,#74261),(#74262,#74263),(#74264,#74265),(#74266,#74267),
(#74268,#74269),(#74270,#74271),(#74272,#74273),(#74274,#74275),(#74276,
#74277),(#74278,#74279),(#74280,#74281),(#74282,#74283),(#74284,#74285),
(#74286,#74287),(#74288,#74289),(#74290,#74291),(#74292,#74293),(#74294,
#74295),(#74296,#74297),(#74298,#74299),(#74300,#74301),(#74302,#74303),
(#74304,#74305),(#74306,#74307),(#74308,#74309),(#74310,#74311),(#74312,
#74313),(#74314,#74315),(#74316,#74317),(#74318,#74319),(#74320,#74321),
(#74322,#74323),(#74324,#74325),(#74326,#74327),(#74328,#74329),(#74330,
#74331),(#74332,#74333),(#74334,#74335),(#74336,#74337),(#74338,#74339),
(#74340,#74341),(#74342,#74343),(#74344,#74345),(#74346,#74347),(#74348,
#74349),(#74350,#74351),(#74352,#74353),(#74354,#74355),(#74356,#74357),
(#74358,#74359),(#74360,#74361),(#74362,#74363),(#74364,#74365),(#74366,
#74367),(#74368,#74369),(#74370,#74371),(#74372,#74373),(#74374,#74375),
(#74376,#74377),(#74378,#74379),(#74380,#74381),(#74382,#74383),(#74384,
#74385),(#74386,#74387),(#74388,#74389),(#74390,#74391),(#74392,#74393),
(#74394,#74395),(#74396,#74397),(#74398,#74399),(#74400,#74401),(#74402,
#74403),(#74404,#74405),(#74406,#74407),(#74408,#74409),(#74410,#74411),
(#74412,#74413),(#74414,#74415),(#74416,#74417),(#74418,#74419),(#74420,
#74421),(#74422,#74423),(#74424,#74425),(#74426,#74427),(#74428,#74429),
(#74430,#74431),(#74432,#74433),(#74434,#74435),(#74436,#74437),(#74438,
#74439),(#74440,#74441),(#74442,#74443),(#74444,#74445),(#74446,#74447),
(#74448,#74449),(#74450,#74451),(#74452,#74453),(#74454,#74455),(#74456,
#74457),(#74458,#74459),(#74460,#74461),(#74462,#74463),(#74464,#74465),
(#74466,#74467),(#74468,#74469),(#74470,#74471),(#74472,#74473),(#74474,
#74475),(#74476,#74477),(#74478,#74479),(#74480,#74481),(#74482,#74483),
(#74484,#74485),(#74486,#74487),(#74488,#74489),(#74490,#74491),(#74492,
#74493),(#74494,#74495),(#74496,#74497),(#74498,#74499),(#74500,#74501),
(#74502,#74503),(#74504,#74505),(#74506,#74507),(#74508,#74509),(#74510,
#74511),(#74512,#74513),(#74514,#74515),(#74516,#74517),(#74518,#74519),
(#74520,#74521),(#74522,#74523),(#74524,#74525),(#74526,#74527),(#74528,
#74529),(#74530,#74531),(#74532,#74533),(#74534,#74535)),.UNSPECIFIED.,
 .F.,.F.,.F.)
B_SPLINE_SURFACE_WITH_KNOTS((6,1,1,1,1,1,1,1,1,1,1,1,1,1,1,1,1,1,1,1,1,
1,1,1,1,1,1,1,1,1,1,1,1,1,1,1,1,1,1,1,1,1,1,1,1,1,1,1,1,1,1,1,1,1,1,1,1,
1,1,1,1,1,1,1,1,1,1,1,1,1,1,1,1,1,1,1,1,1,1,1,1,1,1,1,1,1,1,1,1,1,1,1,1,
1,1,1,1,1,1,1,1,1,1,1,1,1,1,1,1,1,1,1,1,1,1,1,1,1,1,1,1,1,1,1,1,1,1,1,1,
1,1,1,1,1,1,1,1,1,1,1,1,1,1,1,1,1,1,1,1,1,1,1,1,1,1,1,1,1,1,1,1,1,1,1,1,
1,1,1,1,1,1,1,1,1,1,1,1,1,1,1,1,1,1,1,1,1,1,1,1,1,1,1,1,1,1,1,1,1,1,1,6),
(2,2),(0.,0.005,0.01,0.015,0.02,0.025,0.03,0.035,0.04,0.045,0.05,0.055,
0.06,0.065,0.07,0.075,0.08,0.085,0.09,0.095,0.1,0.105,0.11,0.115,0.12,0.125,
0.13,0.135,0.14,0.145,0.15,0.155,0.16,0.165,0.17,0.175,0.18,0.185,0.19,
0.195,0.2,0.205,0.21,0.215,0.22,0.225,0.23,0.235,0.24,0.245,0.25,0.255,
0.26,0.265,0.27,0.275,0.28,0.285,0.29,0.295,0.3,0.305,0.31,0.315,0.32,0.325,
0.33,0.335,0.34,0.345,0.35,0.355,0.36,0.365,0.37,0.375,0.38,0.385,0.39,
0.395,0.4,0.405,0.41,0.415,0.42,0.425,0.43,0.435,0.44,0.445,0.45,0.455,
0.46,0.465,0.47,0.475,0.48,0.485,0.49,0.495,0.5,0.505,0.51,0.515,0.52,0.525,
0.53,0.535,0.54,0.545,0.55,0.555,0.56,0.565,0.57,0.575,0.58,0.585,0.59,
0.595,0.6,0.605,0.61,0.615,0.62,0.625,0.63,0.635,0.64,0.645,0.65,0.655,
0.66,0.665,0.67,0.675,0.68,0.685,0.690000000000001,0.695000000000001,0.700000000000001,
0.705000000000001,0.710000000000001,0.715000000000001,0.720000000000001,
0.725000000000001,0.730000000000001,0.735000000000001,0.740000000000001,
0.745000000000001,0.750000000000001,0.755000000000001,0.760000000000001,
0.765000000000001,0.770000000000001,0.775000000000001,0.780000000000001,
0.785000000000001,0.790000000000001,0.795000000000001,0.800000000000001,
0.805000000000001,0.810000000000001,0.815000000000001,0.820000000000001,
0.825000000000001,0.830000000000001,0.835000000000001,0.840000000000001,
0.845000000000001,0.850000000000001,0.855000000000001,0.860000000000001,
0.865000000000001,0.870000000000001,0.875000000000001,0.880000000000001,
0.885000000000001,0.890000000000001,0.895000000000001,0.900000000000001,
0.905000000000001,0.910000000000001,0.915000000000001,0.920000000000001,
0.925000000000001,0.930000000000001,0.935000000000001,0.940000000000001,
0.945000000000001,0.950000000000001,0.955000000000001,0.960000000000001,
0.965000000000001,0.970000000000001,0.975000000000001,0.980000000000001,
0.985000000000001,0.990000000000001,0.995000000000001,1.),(0.,1.2),
 .UNSPECIFIED.)
GEOMETRIC_REPRESENTATION_ITEM()
RATIONAL_B_SPLINE_SURFACE(((1.,1.),(1.,1.),(1.,1.),(1.,1.),(1.,1.),(1.,
1.),(1.,1.),(1.,1.),(1.,1.),(1.,1.),(1.,1.),(1.,1.),(1.,1.),(1.,1.),(1.,
1.),(1.,1.),(1.,1.),(1.,1.),(1.,1.),(1.,1.),(1.,1.),(1.,1.),(1.,1.),(1.,
1.),(1.,1.),(1.,1.),(1.,1.),(1.,1.),(1.,1.),(1.,1.),(1.,1.),(1.,1.),(1.,
1.),(1.,1.),(1.,1.),(1.,1.),(1.,1.),(1.,1.),(1.,1.),(1.,1.),(1.,1.),(1.,
1.),(1.,1.),(1.,1.),(1.,1.),(1.,1.),(1.,1.),(1.,1.),(1.,1.),(1.,1.),(1.,
1.),(1.,1.),(1.,1.),(1.,1.),(1.,1.),(1.,1.),(1.,1.),(1.,1.),(1.,1.),(1.,
1.),(1.,1.),(1.,1.),(1.,1.),(1.,1.),(1.,1.),(1.,1.),(1.,1.),(1.,1.),(1.,
1.),(1.,1.),(1.,1.),(1.,1.),(1.,1.),(1.,1.),(1.,1.),(1.,1.),(1.,1.),(1.,
1.),(1.,1.),(1.,1.),(1.,1.),(1.,1.),(1.,1.),(1.,1.),(1.,1.),(1.,1.),(1.,
1.),(1.,1.),(1.,1.),(1.,1.),(1.,1.),(1.,1.),(1.,1.),(1.,1.),(1.,1.),(1.,
1.),(1.,1.),(1.,1.),(1.,1.),(1.,1.),(1.,1.),(1.,1.),(1.,1.),(1.,1.),(1.,
1.),(1.,1.),(1.,1.),(1.,1.),(1.,1.),(1.,1.),(1.,1.),(1.,1.),(1.,1.),(1.,
1.),(1.,1.),(1.,1.),(1.,1.),(1.,1.),(1.,1.),(1.,1.),(1.,1.),(1.,1.),(1.,
1.),(1.,1.),(1.,1.),(1.,1.),(1.,1.),(1.,1.),(1.,1.),(1.,1.),(1.,1.),(1.,
1.),(1.,1.),(1.,1.),(1.,1.),(1.,1.),(1.,1.),(1.,1.),(1.,1.),(1.,1.),(1.,
1.),(1.,1.),(1.,1.),(1.,1.),(1.,1.),(1.,1.),(1.,1.),(1.,1.),(1.,1.),(1.,
1.),(1.,1.),(1.,1.),(1.,1.),(1.,1.),(1.,1.),(1.,1.),(1.,1.),(1.,1.),(1.,
1.),(1.,1.),(1.,1.),(1.,1.),(1.,1.),(1.,1.),(1.,1.),(1.,1.),(1.,1.),(1.,
1.),(1.,1.),(1.,1.),(1.,1.),(1.,1.),(1.,1.),(1.,1.),(1.,1.),(1.,1.),(1.,
1.),(1.,1.),(1.,1.),(1.,1.),(1.,1.),(1.,1.),(1.,1.),(1.,1.),(1.,1.),(1.,
1.),(1.,1.),(1.,1.),(1.,1.),(1.,1.),(1.,1.),(1.,1.),(1.,1.),(1.,1.),(1.,
1.),(1.,1.),(1.,1.),(1.,1.),(1.,1.),(1.,1.),(1.,1.),(1.,1.),(1.,1.),(1.,
1.),(1.,1.)))
REPRESENTATION_ITEM('')
SURFACE()
);
#908=(
BOUNDED_SURFACE()
B_SPLINE_SURFACE(5,1,((#75022,#75023),(#75024,#75025),(#75026,#75027),(#75028,
#75029),(#75030,#75031),(#75032,#75033),(#75034,#75035),(#75036,#75037),
(#75038,#75039),(#75040,#75041),(#75042,#75043),(#75044,#75045),(#75046,
#75047),(#75048,#75049),(#75050,#75051),(#75052,#75053),(#75054,#75055),
(#75056,#75057),(#75058,#75059),(#75060,#75061),(#75062,#75063),(#75064,
#75065),(#75066,#75067),(#75068,#75069),(#75070,#75071),(#75072,#75073),
(#75074,#75075),(#75076,#75077),(#75078,#75079),(#75080,#75081),(#75082,
#75083),(#75084,#75085),(#75086,#75087),(#75088,#75089),(#75090,#75091),
(#75092,#75093),(#75094,#75095),(#75096,#75097),(#75098,#75099),(#75100,
#75101),(#75102,#75103),(#75104,#75105),(#75106,#75107),(#75108,#75109),
(#75110,#75111),(#75112,#75113),(#75114,#75115),(#75116,#75117),(#75118,
#75119),(#75120,#75121),(#75122,#75123),(#75124,#75125),(#75126,#75127),
(#75128,#75129),(#75130,#75131),(#75132,#75133),(#75134,#75135),(#75136,
#75137),(#75138,#75139),(#75140,#75141),(#75142,#75143),(#75144,#75145),
(#75146,#75147),(#75148,#75149),(#75150,#75151),(#75152,#75153),(#75154,
#75155),(#75156,#75157),(#75158,#75159),(#75160,#75161),(#75162,#75163),
(#75164,#75165),(#75166,#75167),(#75168,#75169),(#75170,#75171),(#75172,
#75173),(#75174,#75175),(#75176,#75177),(#75178,#75179),(#75180,#75181),
(#75182,#75183),(#75184,#75185),(#75186,#75187),(#75188,#75189),(#75190,
#75191),(#75192,#75193),(#75194,#75195),(#75196,#75197),(#75198,#75199),
(#75200,#75201),(#75202,#75203),(#75204,#75205),(#75206,#75207),(#75208,
#75209),(#75210,#75211),(#75212,#75213),(#75214,#75215),(#75216,#75217),
(#75218,#75219),(#75220,#75221),(#75222,#75223),(#75224,#75225),(#75226,
#75227),(#75228,#75229),(#75230,#75231),(#75232,#75233),(#75234,#75235),
(#75236,#75237),(#75238,#75239),(#75240,#75241),(#75242,#75243),(#75244,
#75245),(#75246,#75247),(#75248,#75249),(#75250,#75251),(#75252,#75253),
(#75254,#75255),(#75256,#75257),(#75258,#75259),(#75260,#75261),(#75262,
#75263),(#75264,#75265),(#75266,#75267),(#75268,#75269),(#75270,#75271),
(#75272,#75273),(#75274,#75275),(#75276,#75277),(#75278,#75279),(#75280,
#75281),(#75282,#75283),(#75284,#75285),(#75286,#75287),(#75288,#75289),
(#75290,#75291),(#75292,#75293),(#75294,#75295),(#75296,#75297),(#75298,
#75299),(#75300,#75301),(#75302,#75303),(#75304,#75305),(#75306,#75307),
(#75308,#75309),(#75310,#75311),(#75312,#75313),(#75314,#75315),(#75316,
#75317),(#75318,#75319),(#75320,#75321),(#75322,#75323),(#75324,#75325),
(#75326,#75327),(#75328,#75329),(#75330,#75331),(#75332,#75333),(#75334,
#75335),(#75336,#75337),(#75338,#75339),(#75340,#75341),(#75342,#75343),
(#75344,#75345),(#75346,#75347),(#75348,#75349),(#75350,#75351),(#75352,
#75353),(#75354,#75355),(#75356,#75357),(#75358,#75359),(#75360,#75361),
(#75362,#75363),(#75364,#75365),(#75366,#75367),(#75368,#75369),(#75370,
#75371),(#75372,#75373),(#75374,#75375),(#75376,#75377),(#75378,#75379),
(#75380,#75381),(#75382,#75383),(#75384,#75385),(#75386,#75387),(#75388,
#75389),(#75390,#75391),(#75392,#75393),(#75394,#75395),(#75396,#75397),
(#75398,#75399),(#75400,#75401),(#75402,#75403),(#75404,#75405),(#75406,
#75407),(#75408,#75409),(#75410,#75411),(#75412,#75413),(#75414,#75415),
(#75416,#75417),(#75418,#75419),(#75420,#75421),(#75422,#75423),(#75424,
#75425),(#75426,#75427),(#75428,#75429),(#75430,#75431)),.UNSPECIFIED.,
 .F.,.F.,.F.)
B_SPLINE_SURFACE_WITH_KNOTS((6,1,1,1,1,1,1,1,1,1,1,1,1,1,1,1,1,1,1,1,1,
1,1,1,1,1,1,1,1,1,1,1,1,1,1,1,1,1,1,1,1,1,1,1,1,1,1,1,1,1,1,1,1,1,1,1,1,
1,1,1,1,1,1,1,1,1,1,1,1,1,1,1,1,1,1,1,1,1,1,1,1,1,1,1,1,1,1,1,1,1,1,1,1,
1,1,1,1,1,1,1,1,1,1,1,1,1,1,1,1,1,1,1,1,1,1,1,1,1,1,1,1,1,1,1,1,1,1,1,1,
1,1,1,1,1,1,1,1,1,1,1,1,1,1,1,1,1,1,1,1,1,1,1,1,1,1,1,1,1,1,1,1,1,1,1,1,
1,1,1,1,1,1,1,1,1,1,1,1,1,1,1,1,1,1,1,1,1,1,1,1,1,1,1,1,1,1,1,1,1,1,1,6),
(2,2),(0.,0.005,0.01,0.015,0.02,0.025,0.03,0.035,0.04,0.045,0.05,0.055,
0.06,0.065,0.07,0.075,0.08,0.085,0.09,0.095,0.1,0.105,0.11,0.115,0.12,0.125,
0.13,0.135,0.14,0.145,0.15,0.155,0.16,0.165,0.17,0.175,0.18,0.185,0.19,
0.195,0.2,0.205,0.21,0.215,0.22,0.225,0.23,0.235,0.24,0.245,0.25,0.255,
0.26,0.265,0.27,0.275,0.28,0.285,0.29,0.295,0.3,0.305,0.31,0.315,0.32,0.325,
0.33,0.335,0.34,0.345,0.35,0.355,0.36,0.365,0.37,0.375,0.38,0.385,0.39,
0.395,0.4,0.405,0.41,0.415,0.42,0.425,0.43,0.435,0.44,0.445,0.45,0.455,
0.46,0.465,0.47,0.475,0.48,0.485,0.49,0.495,0.5,0.505,0.51,0.515,0.52,0.525,
0.53,0.535,0.54,0.545,0.55,0.555,0.56,0.565,0.57,0.575,0.58,0.585,0.59,
0.595,0.6,0.605,0.61,0.615,0.62,0.625,0.63,0.635,0.64,0.645,0.65,0.655,
0.66,0.665,0.67,0.675,0.68,0.685,0.690000000000001,0.695000000000001,0.700000000000001,
0.705000000000001,0.710000000000001,0.715000000000001,0.720000000000001,
0.725000000000001,0.730000000000001,0.735000000000001,0.740000000000001,
0.745000000000001,0.750000000000001,0.755000000000001,0.760000000000001,
0.765000000000001,0.770000000000001,0.775000000000001,0.780000000000001,
0.785000000000001,0.790000000000001,0.795000000000001,0.800000000000001,
0.805000000000001,0.810000000000001,0.815000000000001,0.820000000000001,
0.825000000000001,0.830000000000001,0.835000000000001,0.840000000000001,
0.845000000000001,0.850000000000001,0.855000000000001,0.860000000000001,
0.865000000000001,0.870000000000001,0.875000000000001,0.880000000000001,
0.885000000000001,0.890000000000001,0.895000000000001,0.900000000000001,
0.905000000000001,0.910000000000001,0.915000000000001,0.920000000000001,
0.925000000000001,0.930000000000001,0.935000000000001,0.940000000000001,
0.945000000000001,0.950000000000001,0.955000000000001,0.960000000000001,
0.965000000000001,0.970000000000001,0.975000000000001,0.980000000000001,
0.985000000000001,0.990000000000001,0.995000000000001,1.),(0.,1.2),
 .UNSPECIFIED.)
GEOMETRIC_REPRESENTATION_ITEM()
RATIONAL_B_SPLINE_SURFACE(((1.,1.),(1.,1.),(1.,1.),(1.,1.),(1.,1.),(1.,
1.),(1.,1.),(1.,1.),(1.,1.),(1.,1.),(1.,1.),(1.,1.),(1.,1.),(1.,1.),(1.,
1.),(1.,1.),(1.,1.),(1.,1.),(1.,1.),(1.,1.),(1.,1.),(1.,1.),(1.,1.),(1.,
1.),(1.,1.),(1.,1.),(1.,1.),(1.,1.),(1.,1.),(1.,1.),(1.,1.),(1.,1.),(1.,
1.),(1.,1.),(1.,1.),(1.,1.),(1.,1.),(1.,1.),(1.,1.),(1.,1.),(1.,1.),(1.,
1.),(1.,1.),(1.,1.),(1.,1.),(1.,1.),(1.,1.),(1.,1.),(1.,1.),(1.,1.),(1.,
1.),(1.,1.),(1.,1.),(1.,1.),(1.,1.),(1.,1.),(1.,1.),(1.,1.),(1.,1.),(1.,
1.),(1.,1.),(1.,1.),(1.,1.),(1.,1.),(1.,1.),(1.,1.),(1.,1.),(1.,1.),(1.,
1.),(1.,1.),(1.,1.),(1.,1.),(1.,1.),(1.,1.),(1.,1.),(1.,1.),(1.,1.),(1.,
1.),(1.,1.),(1.,1.),(1.,1.),(1.,1.),(1.,1.),(1.,1.),(1.,1.),(1.,1.),(1.,
1.),(1.,1.),(1.,1.),(1.,1.),(1.,1.),(1.,1.),(1.,1.),(1.,1.),(1.,1.),(1.,
1.),(1.,1.),(1.,1.),(1.,1.),(1.,1.),(1.,1.),(1.,1.),(1.,1.),(1.,1.),(1.,
1.),(1.,1.),(1.,1.),(1.,1.),(1.,1.),(1.,1.),(1.,1.),(1.,1.),(1.,1.),(1.,
1.),(1.,1.),(1.,1.),(1.,1.),(1.,1.),(1.,1.),(1.,1.),(1.,1.),(1.,1.),(1.,
1.),(1.,1.),(1.,1.),(1.,1.),(1.,1.),(1.,1.),(1.,1.),(1.,1.),(1.,1.),(1.,
1.),(1.,1.),(1.,1.),(1.,1.),(1.,1.),(1.,1.),(1.,1.),(1.,1.),(1.,1.),(1.,
1.),(1.,1.),(1.,1.),(1.,1.),(1.,1.),(1.,1.),(1.,1.),(1.,1.),(1.,1.),(1.,
1.),(1.,1.),(1.,1.),(1.,1.),(1.,1.),(1.,1.),(1.,1.),(1.,1.),(1.,1.),(1.,
1.),(1.,1.),(1.,1.),(1.,1.),(1.,1.),(1.,1.),(1.,1.),(1.,1.),(1.,1.),(1.,
1.),(1.,1.),(1.,1.),(1.,1.),(1.,1.),(1.,1.),(1.,1.),(1.,1.),(1.,1.),(1.,
1.),(1.,1.),(1.,1.),(1.,1.),(1.,1.),(1.,1.),(1.,1.),(1.,1.),(1.,1.),(1.,
1.),(1.,1.),(1.,1.),(1.,1.),(1.,1.),(1.,1.),(1.,1.),(1.,1.),(1.,1.),(1.,
1.),(1.,1.),(1.,1.),(1.,1.),(1.,1.),(1.,1.),(1.,1.),(1.,1.),(1.,1.),(1.,
1.),(1.,1.)))
REPRESENTATION_ITEM('')
SURFACE()
);
#909=(
BOUNDED_SURFACE()
B_SPLINE_SURFACE(5,1,((#75918,#75919),(#75920,#75921),(#75922,#75923),(#75924,
#75925),(#75926,#75927),(#75928,#75929),(#75930,#75931),(#75932,#75933),
(#75934,#75935),(#75936,#75937),(#75938,#75939),(#75940,#75941),(#75942,
#75943),(#75944,#75945),(#75946,#75947),(#75948,#75949),(#75950,#75951),
(#75952,#75953),(#75954,#75955),(#75956,#75957),(#75958,#75959),(#75960,
#75961),(#75962,#75963),(#75964,#75965),(#75966,#75967),(#75968,#75969),
(#75970,#75971),(#75972,#75973),(#75974,#75975),(#75976,#75977),(#75978,
#75979),(#75980,#75981),(#75982,#75983),(#75984,#75985),(#75986,#75987),
(#75988,#75989),(#75990,#75991),(#75992,#75993),(#75994,#75995),(#75996,
#75997),(#75998,#75999),(#76000,#76001),(#76002,#76003),(#76004,#76005),
(#76006,#76007),(#76008,#76009),(#76010,#76011),(#76012,#76013),(#76014,
#76015),(#76016,#76017),(#76018,#76019),(#76020,#76021),(#76022,#76023),
(#76024,#76025),(#76026,#76027),(#76028,#76029),(#76030,#76031),(#76032,
#76033),(#76034,#76035),(#76036,#76037),(#76038,#76039),(#76040,#76041),
(#76042,#76043),(#76044,#76045),(#76046,#76047),(#76048,#76049),(#76050,
#76051),(#76052,#76053),(#76054,#76055),(#76056,#76057),(#76058,#76059),
(#76060,#76061),(#76062,#76063),(#76064,#76065),(#76066,#76067),(#76068,
#76069),(#76070,#76071),(#76072,#76073),(#76074,#76075),(#76076,#76077),
(#76078,#76079),(#76080,#76081),(#76082,#76083),(#76084,#76085),(#76086,
#76087),(#76088,#76089),(#76090,#76091),(#76092,#76093),(#76094,#76095),
(#76096,#76097),(#76098,#76099),(#76100,#76101),(#76102,#76103),(#76104,
#76105),(#76106,#76107),(#76108,#76109),(#76110,#76111),(#76112,#76113),
(#76114,#76115),(#76116,#76117),(#76118,#76119),(#76120,#76121),(#76122,
#76123),(#76124,#76125),(#76126,#76127),(#76128,#76129),(#76130,#76131),
(#76132,#76133),(#76134,#76135),(#76136,#76137),(#76138,#76139),(#76140,
#76141),(#76142,#76143),(#76144,#76145),(#76146,#76147),(#76148,#76149),
(#76150,#76151),(#76152,#76153),(#76154,#76155),(#76156,#76157),(#76158,
#76159),(#76160,#76161),(#76162,#76163),(#76164,#76165),(#76166,#76167),
(#76168,#76169),(#76170,#76171),(#76172,#76173),(#76174,#76175),(#76176,
#76177),(#76178,#76179),(#76180,#76181),(#76182,#76183),(#76184,#76185),
(#76186,#76187),(#76188,#76189),(#76190,#76191),(#76192,#76193),(#76194,
#76195),(#76196,#76197),(#76198,#76199),(#76200,#76201),(#76202,#76203),
(#76204,#76205),(#76206,#76207),(#76208,#76209),(#76210,#76211),(#76212,
#76213),(#76214,#76215),(#76216,#76217),(#76218,#76219),(#76220,#76221),
(#76222,#76223),(#76224,#76225),(#76226,#76227),(#76228,#76229),(#76230,
#76231),(#76232,#76233),(#76234,#76235),(#76236,#76237),(#76238,#76239),
(#76240,#76241),(#76242,#76243),(#76244,#76245),(#76246,#76247),(#76248,
#76249),(#76250,#76251),(#76252,#76253),(#76254,#76255),(#76256,#76257),
(#76258,#76259),(#76260,#76261),(#76262,#76263),(#76264,#76265),(#76266,
#76267),(#76268,#76269),(#76270,#76271),(#76272,#76273),(#76274,#76275),
(#76276,#76277),(#76278,#76279),(#76280,#76281),(#76282,#76283),(#76284,
#76285),(#76286,#76287),(#76288,#76289),(#76290,#76291),(#76292,#76293),
(#76294,#76295),(#76296,#76297),(#76298,#76299),(#76300,#76301),(#76302,
#76303),(#76304,#76305),(#76306,#76307),(#76308,#76309),(#76310,#76311),
(#76312,#76313),(#76314,#76315),(#76316,#76317),(#76318,#76319),(#76320,
#76321),(#76322,#76323),(#76324,#76325),(#76326,#76327)),.UNSPECIFIED.,
 .F.,.F.,.F.)
B_SPLINE_SURFACE_WITH_KNOTS((6,1,1,1,1,1,1,1,1,1,1,1,1,1,1,1,1,1,1,1,1,
1,1,1,1,1,1,1,1,1,1,1,1,1,1,1,1,1,1,1,1,1,1,1,1,1,1,1,1,1,1,1,1,1,1,1,1,
1,1,1,1,1,1,1,1,1,1,1,1,1,1,1,1,1,1,1,1,1,1,1,1,1,1,1,1,1,1,1,1,1,1,1,1,
1,1,1,1,1,1,1,1,1,1,1,1,1,1,1,1,1,1,1,1,1,1,1,1,1,1,1,1,1,1,1,1,1,1,1,1,
1,1,1,1,1,1,1,1,1,1,1,1,1,1,1,1,1,1,1,1,1,1,1,1,1,1,1,1,1,1,1,1,1,1,1,1,
1,1,1,1,1,1,1,1,1,1,1,1,1,1,1,1,1,1,1,1,1,1,1,1,1,1,1,1,1,1,1,1,1,1,1,6),
(2,2),(0.,0.005,0.01,0.015,0.02,0.025,0.03,0.035,0.04,0.045,0.05,0.055,
0.06,0.065,0.07,0.075,0.08,0.085,0.09,0.095,0.1,0.105,0.11,0.115,0.12,0.125,
0.13,0.135,0.14,0.145,0.15,0.155,0.16,0.165,0.17,0.175,0.18,0.185,0.19,
0.195,0.2,0.205,0.21,0.215,0.22,0.225,0.23,0.235,0.24,0.245,0.25,0.255,
0.26,0.265,0.27,0.275,0.28,0.285,0.29,0.295,0.3,0.305,0.31,0.315,0.32,0.325,
0.33,0.335,0.34,0.345,0.35,0.355,0.36,0.365,0.37,0.375,0.38,0.385,0.39,
0.395,0.4,0.405,0.41,0.415,0.42,0.425,0.43,0.435,0.44,0.445,0.45,0.455,
0.46,0.465,0.47,0.475,0.48,0.485,0.49,0.495,0.5,0.505,0.51,0.515,0.52,0.525,
0.53,0.535,0.54,0.545,0.55,0.555,0.56,0.565,0.57,0.575,0.58,0.585,0.59,
0.595,0.6,0.605,0.61,0.615,0.62,0.625,0.63,0.635,0.64,0.645,0.65,0.655,
0.66,0.665,0.67,0.675,0.68,0.685,0.690000000000001,0.695000000000001,0.700000000000001,
0.705000000000001,0.710000000000001,0.715000000000001,0.720000000000001,
0.725000000000001,0.730000000000001,0.735000000000001,0.740000000000001,
0.745000000000001,0.750000000000001,0.755000000000001,0.760000000000001,
0.765000000000001,0.770000000000001,0.775000000000001,0.780000000000001,
0.785000000000001,0.790000000000001,0.795000000000001,0.800000000000001,
0.805000000000001,0.810000000000001,0.815000000000001,0.820000000000001,
0.825000000000001,0.830000000000001,0.835000000000001,0.840000000000001,
0.845000000000001,0.850000000000001,0.855000000000001,0.860000000000001,
0.865000000000001,0.870000000000001,0.875000000000001,0.880000000000001,
0.885000000000001,0.890000000000001,0.895000000000001,0.900000000000001,
0.905000000000001,0.910000000000001,0.915000000000001,0.920000000000001,
0.925000000000001,0.930000000000001,0.935000000000001,0.940000000000001,
0.945000000000001,0.950000000000001,0.955000000000001,0.960000000000001,
0.965000000000001,0.970000000000001,0.975000000000001,0.980000000000001,
0.985000000000001,0.990000000000001,0.995000000000001,1.),(0.,1.2),
 .UNSPECIFIED.)
GEOMETRIC_REPRESENTATION_ITEM()
RATIONAL_B_SPLINE_SURFACE(((1.,1.),(1.,1.),(1.,1.),(1.,1.),(1.,1.),(1.,
1.),(1.,1.),(1.,1.),(1.,1.),(1.,1.),(1.,1.),(1.,1.),(1.,1.),(1.,1.),(1.,
1.),(1.,1.),(1.,1.),(1.,1.),(1.,1.),(1.,1.),(1.,1.),(1.,1.),(1.,1.),(1.,
1.),(1.,1.),(1.,1.),(1.,1.),(1.,1.),(1.,1.),(1.,1.),(1.,1.),(1.,1.),(1.,
1.),(1.,1.),(1.,1.),(1.,1.),(1.,1.),(1.,1.),(1.,1.),(1.,1.),(1.,1.),(1.,
1.),(1.,1.),(1.,1.),(1.,1.),(1.,1.),(1.,1.),(1.,1.),(1.,1.),(1.,1.),(1.,
1.),(1.,1.),(1.,1.),(1.,1.),(1.,1.),(1.,1.),(1.,1.),(1.,1.),(1.,1.),(1.,
1.),(1.,1.),(1.,1.),(1.,1.),(1.,1.),(1.,1.),(1.,1.),(1.,1.),(1.,1.),(1.,
1.),(1.,1.),(1.,1.),(1.,1.),(1.,1.),(1.,1.),(1.,1.),(1.,1.),(1.,1.),(1.,
1.),(1.,1.),(1.,1.),(1.,1.),(1.,1.),(1.,1.),(1.,1.),(1.,1.),(1.,1.),(1.,
1.),(1.,1.),(1.,1.),(1.,1.),(1.,1.),(1.,1.),(1.,1.),(1.,1.),(1.,1.),(1.,
1.),(1.,1.),(1.,1.),(1.,1.),(1.,1.),(1.,1.),(1.,1.),(1.,1.),(1.,1.),(1.,
1.),(1.,1.),(1.,1.),(1.,1.),(1.,1.),(1.,1.),(1.,1.),(1.,1.),(1.,1.),(1.,
1.),(1.,1.),(1.,1.),(1.,1.),(1.,1.),(1.,1.),(1.,1.),(1.,1.),(1.,1.),(1.,
1.),(1.,1.),(1.,1.),(1.,1.),(1.,1.),(1.,1.),(1.,1.),(1.,1.),(1.,1.),(1.,
1.),(1.,1.),(1.,1.),(1.,1.),(1.,1.),(1.,1.),(1.,1.),(1.,1.),(1.,1.),(1.,
1.),(1.,1.),(1.,1.),(1.,1.),(1.,1.),(1.,1.),(1.,1.),(1.,1.),(1.,1.),(1.,
1.),(1.,1.),(1.,1.),(1.,1.),(1.,1.),(1.,1.),(1.,1.),(1.,1.),(1.,1.),(1.,
1.),(1.,1.),(1.,1.),(1.,1.),(1.,1.),(1.,1.),(1.,1.),(1.,1.),(1.,1.),(1.,
1.),(1.,1.),(1.,1.),(1.,1.),(1.,1.),(1.,1.),(1.,1.),(1.,1.),(1.,1.),(1.,
1.),(1.,1.),(1.,1.),(1.,1.),(1.,1.),(1.,1.),(1.,1.),(1.,1.),(1.,1.),(1.,
1.),(1.,1.),(1.,1.),(1.,1.),(1.,1.),(1.,1.),(1.,1.),(1.,1.),(1.,1.),(1.,
1.),(1.,1.),(1.,1.),(1.,1.),(1.,1.),(1.,1.),(1.,1.),(1.,1.),(1.,1.),(1.,
1.),(1.,1.)))
REPRESENTATION_ITEM('')
SURFACE()
);
#910=(
BOUNDED_SURFACE()
B_SPLINE_SURFACE(5,1,((#76814,#76815),(#76816,#76817),(#76818,#76819),(#76820,
#76821),(#76822,#76823),(#76824,#76825),(#76826,#76827),(#76828,#76829),
(#76830,#76831),(#76832,#76833),(#76834,#76835),(#76836,#76837),(#76838,
#76839),(#76840,#76841),(#76842,#76843),(#76844,#76845),(#76846,#76847),
(#76848,#76849),(#76850,#76851),(#76852,#76853),(#76854,#76855),(#76856,
#76857),(#76858,#76859),(#76860,#76861),(#76862,#76863),(#76864,#76865),
(#76866,#76867),(#76868,#76869),(#76870,#76871),(#76872,#76873),(#76874,
#76875),(#76876,#76877),(#76878,#76879),(#76880,#76881),(#76882,#76883),
(#76884,#76885),(#76886,#76887),(#76888,#76889),(#76890,#76891),(#76892,
#76893),(#76894,#76895),(#76896,#76897),(#76898,#76899),(#76900,#76901),
(#76902,#76903),(#76904,#76905),(#76906,#76907),(#76908,#76909),(#76910,
#76911),(#76912,#76913),(#76914,#76915),(#76916,#76917),(#76918,#76919),
(#76920,#76921),(#76922,#76923),(#76924,#76925),(#76926,#76927),(#76928,
#76929),(#76930,#76931),(#76932,#76933),(#76934,#76935),(#76936,#76937),
(#76938,#76939),(#76940,#76941),(#76942,#76943),(#76944,#76945),(#76946,
#76947),(#76948,#76949),(#76950,#76951),(#76952,#76953),(#76954,#76955),
(#76956,#76957),(#76958,#76959),(#76960,#76961),(#76962,#76963),(#76964,
#76965),(#76966,#76967),(#76968,#76969),(#76970,#76971),(#76972,#76973),
(#76974,#76975),(#76976,#76977),(#76978,#76979),(#76980,#76981),(#76982,
#76983),(#76984,#76985),(#76986,#76987),(#76988,#76989),(#76990,#76991),
(#76992,#76993),(#76994,#76995),(#76996,#76997),(#76998,#76999),(#77000,
#77001),(#77002,#77003),(#77004,#77005),(#77006,#77007),(#77008,#77009),
(#77010,#77011),(#77012,#77013),(#77014,#77015),(#77016,#77017),(#77018,
#77019),(#77020,#77021),(#77022,#77023),(#77024,#77025),(#77026,#77027),
(#77028,#77029),(#77030,#77031),(#77032,#77033),(#77034,#77035),(#77036,
#77037),(#77038,#77039),(#77040,#77041),(#77042,#77043),(#77044,#77045),
(#77046,#77047),(#77048,#77049),(#77050,#77051),(#77052,#77053),(#77054,
#77055),(#77056,#77057),(#77058,#77059),(#77060,#77061),(#77062,#77063),
(#77064,#77065),(#77066,#77067),(#77068,#77069),(#77070,#77071),(#77072,
#77073),(#77074,#77075),(#77076,#77077),(#77078,#77079),(#77080,#77081),
(#77082,#77083),(#77084,#77085),(#77086,#77087),(#77088,#77089),(#77090,
#77091),(#77092,#77093),(#77094,#77095),(#77096,#77097),(#77098,#77099),
(#77100,#77101),(#77102,#77103),(#77104,#77105),(#77106,#77107),(#77108,
#77109),(#77110,#77111),(#77112,#77113),(#77114,#77115),(#77116,#77117),
(#77118,#77119),(#77120,#77121),(#77122,#77123),(#77124,#77125),(#77126,
#77127),(#77128,#77129),(#77130,#77131),(#77132,#77133),(#77134,#77135),
(#77136,#77137),(#77138,#77139),(#77140,#77141),(#77142,#77143),(#77144,
#77145),(#77146,#77147),(#77148,#77149),(#77150,#77151),(#77152,#77153),
(#77154,#77155),(#77156,#77157),(#77158,#77159),(#77160,#77161),(#77162,
#77163),(#77164,#77165),(#77166,#77167),(#77168,#77169),(#77170,#77171),
(#77172,#77173),(#77174,#77175),(#77176,#77177),(#77178,#77179),(#77180,
#77181),(#77182,#77183),(#77184,#77185),(#77186,#77187),(#77188,#77189),
(#77190,#77191),(#77192,#77193),(#77194,#77195),(#77196,#77197),(#77198,
#77199),(#77200,#77201),(#77202,#77203),(#77204,#77205),(#77206,#77207),
(#77208,#77209),(#77210,#77211),(#77212,#77213),(#77214,#77215),(#77216,
#77217),(#77218,#77219),(#77220,#77221),(#77222,#77223)),.UNSPECIFIED.,
 .F.,.F.,.F.)
B_SPLINE_SURFACE_WITH_KNOTS((6,1,1,1,1,1,1,1,1,1,1,1,1,1,1,1,1,1,1,1,1,
1,1,1,1,1,1,1,1,1,1,1,1,1,1,1,1,1,1,1,1,1,1,1,1,1,1,1,1,1,1,1,1,1,1,1,1,
1,1,1,1,1,1,1,1,1,1,1,1,1,1,1,1,1,1,1,1,1,1,1,1,1,1,1,1,1,1,1,1,1,1,1,1,
1,1,1,1,1,1,1,1,1,1,1,1,1,1,1,1,1,1,1,1,1,1,1,1,1,1,1,1,1,1,1,1,1,1,1,1,
1,1,1,1,1,1,1,1,1,1,1,1,1,1,1,1,1,1,1,1,1,1,1,1,1,1,1,1,1,1,1,1,1,1,1,1,
1,1,1,1,1,1,1,1,1,1,1,1,1,1,1,1,1,1,1,1,1,1,1,1,1,1,1,1,1,1,1,1,1,1,1,6),
(2,2),(0.,0.005,0.01,0.015,0.02,0.025,0.03,0.035,0.04,0.045,0.05,0.055,
0.06,0.065,0.07,0.075,0.08,0.085,0.09,0.095,0.1,0.105,0.11,0.115,0.12,0.125,
0.13,0.135,0.14,0.145,0.15,0.155,0.16,0.165,0.17,0.175,0.18,0.185,0.19,
0.195,0.2,0.205,0.21,0.215,0.22,0.225,0.23,0.235,0.24,0.245,0.25,0.255,
0.26,0.265,0.27,0.275,0.28,0.285,0.29,0.295,0.3,0.305,0.31,0.315,0.32,0.325,
0.33,0.335,0.34,0.345,0.35,0.355,0.36,0.365,0.37,0.375,0.38,0.385,0.39,
0.395,0.4,0.405,0.41,0.415,0.42,0.425,0.43,0.435,0.44,0.445,0.45,0.455,
0.46,0.465,0.47,0.475,0.48,0.485,0.49,0.495,0.5,0.505,0.51,0.515,0.52,0.525,
0.53,0.535,0.54,0.545,0.55,0.555,0.56,0.565,0.57,0.575,0.58,0.585,0.59,
0.595,0.6,0.605,0.61,0.615,0.62,0.625,0.63,0.635,0.64,0.645,0.65,0.655,
0.66,0.665,0.67,0.675,0.68,0.685,0.690000000000001,0.695000000000001,0.700000000000001,
0.705000000000001,0.710000000000001,0.715000000000001,0.720000000000001,
0.725000000000001,0.730000000000001,0.735000000000001,0.740000000000001,
0.745000000000001,0.750000000000001,0.755000000000001,0.760000000000001,
0.765000000000001,0.770000000000001,0.775000000000001,0.780000000000001,
0.785000000000001,0.790000000000001,0.795000000000001,0.800000000000001,
0.805000000000001,0.810000000000001,0.815000000000001,0.820000000000001,
0.825000000000001,0.830000000000001,0.835000000000001,0.840000000000001,
0.845000000000001,0.850000000000001,0.855000000000001,0.860000000000001,
0.865000000000001,0.870000000000001,0.875000000000001,0.880000000000001,
0.885000000000001,0.890000000000001,0.895000000000001,0.900000000000001,
0.905000000000001,0.910000000000001,0.915000000000001,0.920000000000001,
0.925000000000001,0.930000000000001,0.935000000000001,0.940000000000001,
0.945000000000001,0.950000000000001,0.955000000000001,0.960000000000001,
0.965000000000001,0.970000000000001,0.975000000000001,0.980000000000001,
0.985000000000001,0.990000000000001,0.995000000000001,1.),(0.,1.2),
 .UNSPECIFIED.)
GEOMETRIC_REPRESENTATION_ITEM()
RATIONAL_B_SPLINE_SURFACE(((1.,1.),(1.,1.),(1.,1.),(1.,1.),(1.,1.),(1.,
1.),(1.,1.),(1.,1.),(1.,1.),(1.,1.),(1.,1.),(1.,1.),(1.,1.),(1.,1.),(1.,
1.),(1.,1.),(1.,1.),(1.,1.),(1.,1.),(1.,1.),(1.,1.),(1.,1.),(1.,1.),(1.,
1.),(1.,1.),(1.,1.),(1.,1.),(1.,1.),(1.,1.),(1.,1.),(1.,1.),(1.,1.),(1.,
1.),(1.,1.),(1.,1.),(1.,1.),(1.,1.),(1.,1.),(1.,1.),(1.,1.),(1.,1.),(1.,
1.),(1.,1.),(1.,1.),(1.,1.),(1.,1.),(1.,1.),(1.,1.),(1.,1.),(1.,1.),(1.,
1.),(1.,1.),(1.,1.),(1.,1.),(1.,1.),(1.,1.),(1.,1.),(1.,1.),(1.,1.),(1.,
1.),(1.,1.),(1.,1.),(1.,1.),(1.,1.),(1.,1.),(1.,1.),(1.,1.),(1.,1.),(1.,
1.),(1.,1.),(1.,1.),(1.,1.),(1.,1.),(1.,1.),(1.,1.),(1.,1.),(1.,1.),(1.,
1.),(1.,1.),(1.,1.),(1.,1.),(1.,1.),(1.,1.),(1.,1.),(1.,1.),(1.,1.),(1.,
1.),(1.,1.),(1.,1.),(1.,1.),(1.,1.),(1.,1.),(1.,1.),(1.,1.),(1.,1.),(1.,
1.),(1.,1.),(1.,1.),(1.,1.),(1.,1.),(1.,1.),(1.,1.),(1.,1.),(1.,1.),(1.,
1.),(1.,1.),(1.,1.),(1.,1.),(1.,1.),(1.,1.),(1.,1.),(1.,1.),(1.,1.),(1.,
1.),(1.,1.),(1.,1.),(1.,1.),(1.,1.),(1.,1.),(1.,1.),(1.,1.),(1.,1.),(1.,
1.),(1.,1.),(1.,1.),(1.,1.),(1.,1.),(1.,1.),(1.,1.),(1.,1.),(1.,1.),(1.,
1.),(1.,1.),(1.,1.),(1.,1.),(1.,1.),(1.,1.),(1.,1.),(1.,1.),(1.,1.),(1.,
1.),(1.,1.),(1.,1.),(1.,1.),(1.,1.),(1.,1.),(1.,1.),(1.,1.),(1.,1.),(1.,
1.),(1.,1.),(1.,1.),(1.,1.),(1.,1.),(1.,1.),(1.,1.),(1.,1.),(1.,1.),(1.,
1.),(1.,1.),(1.,1.),(1.,1.),(1.,1.),(1.,1.),(1.,1.),(1.,1.),(1.,1.),(1.,
1.),(1.,1.),(1.,1.),(1.,1.),(1.,1.),(1.,1.),(1.,1.),(1.,1.),(1.,1.),(1.,
1.),(1.,1.),(1.,1.),(1.,1.),(1.,1.),(1.,1.),(1.,1.),(1.,1.),(1.,1.),(1.,
1.),(1.,1.),(1.,1.),(1.,1.),(1.,1.),(1.,1.),(1.,1.),(1.,1.),(1.,1.),(1.,
1.),(1.,1.),(1.,1.),(1.,1.),(1.,1.),(1.,1.),(1.,1.),(1.,1.),(1.,1.),(1.,
1.),(1.,1.)))
REPRESENTATION_ITEM('')
SURFACE()
);
#911=(
BOUNDED_SURFACE()
B_SPLINE_SURFACE(5,1,((#77710,#77711),(#77712,#77713),(#77714,#77715),(#77716,
#77717),(#77718,#77719),(#77720,#77721),(#77722,#77723),(#77724,#77725),
(#77726,#77727),(#77728,#77729),(#77730,#77731),(#77732,#77733),(#77734,
#77735),(#77736,#77737),(#77738,#77739),(#77740,#77741),(#77742,#77743),
(#77744,#77745),(#77746,#77747),(#77748,#77749),(#77750,#77751),(#77752,
#77753),(#77754,#77755),(#77756,#77757),(#77758,#77759),(#77760,#77761),
(#77762,#77763),(#77764,#77765),(#77766,#77767),(#77768,#77769),(#77770,
#77771),(#77772,#77773),(#77774,#77775),(#77776,#77777),(#77778,#77779),
(#77780,#77781),(#77782,#77783),(#77784,#77785),(#77786,#77787),(#77788,
#77789),(#77790,#77791),(#77792,#77793),(#77794,#77795),(#77796,#77797),
(#77798,#77799),(#77800,#77801),(#77802,#77803),(#77804,#77805),(#77806,
#77807),(#77808,#77809),(#77810,#77811),(#77812,#77813),(#77814,#77815),
(#77816,#77817),(#77818,#77819),(#77820,#77821),(#77822,#77823),(#77824,
#77825),(#77826,#77827),(#77828,#77829),(#77830,#77831),(#77832,#77833),
(#77834,#77835),(#77836,#77837),(#77838,#77839),(#77840,#77841),(#77842,
#77843),(#77844,#77845),(#77846,#77847),(#77848,#77849),(#77850,#77851),
(#77852,#77853),(#77854,#77855),(#77856,#77857),(#77858,#77859),(#77860,
#77861),(#77862,#77863),(#77864,#77865),(#77866,#77867),(#77868,#77869),
(#77870,#77871),(#77872,#77873),(#77874,#77875),(#77876,#77877),(#77878,
#77879),(#77880,#77881),(#77882,#77883),(#77884,#77885),(#77886,#77887),
(#77888,#77889),(#77890,#77891),(#77892,#77893),(#77894,#77895),(#77896,
#77897),(#77898,#77899),(#77900,#77901),(#77902,#77903),(#77904,#77905),
(#77906,#77907),(#77908,#77909),(#77910,#77911),(#77912,#77913),(#77914,
#77915),(#77916,#77917),(#77918,#77919),(#77920,#77921),(#77922,#77923),
(#77924,#77925),(#77926,#77927),(#77928,#77929),(#77930,#77931),(#77932,
#77933),(#77934,#77935),(#77936,#77937),(#77938,#77939),(#77940,#77941),
(#77942,#77943),(#77944,#77945),(#77946,#77947),(#77948,#77949),(#77950,
#77951),(#77952,#77953),(#77954,#77955),(#77956,#77957),(#77958,#77959),
(#77960,#77961),(#77962,#77963),(#77964,#77965),(#77966,#77967),(#77968,
#77969),(#77970,#77971),(#77972,#77973),(#77974,#77975),(#77976,#77977),
(#77978,#77979),(#77980,#77981),(#77982,#77983),(#77984,#77985),(#77986,
#77987),(#77988,#77989),(#77990,#77991),(#77992,#77993),(#77994,#77995),
(#77996,#77997),(#77998,#77999),(#78000,#78001),(#78002,#78003),(#78004,
#78005),(#78006,#78007),(#78008,#78009),(#78010,#78011),(#78012,#78013),
(#78014,#78015),(#78016,#78017),(#78018,#78019),(#78020,#78021),(#78022,
#78023),(#78024,#78025),(#78026,#78027),(#78028,#78029),(#78030,#78031),
(#78032,#78033),(#78034,#78035),(#78036,#78037),(#78038,#78039),(#78040,
#78041),(#78042,#78043),(#78044,#78045),(#78046,#78047),(#78048,#78049),
(#78050,#78051),(#78052,#78053),(#78054,#78055),(#78056,#78057),(#78058,
#78059),(#78060,#78061),(#78062,#78063),(#78064,#78065),(#78066,#78067),
(#78068,#78069),(#78070,#78071),(#78072,#78073),(#78074,#78075),(#78076,
#78077),(#78078,#78079),(#78080,#78081),(#78082,#78083),(#78084,#78085),
(#78086,#78087),(#78088,#78089),(#78090,#78091),(#78092,#78093),(#78094,
#78095),(#78096,#78097),(#78098,#78099),(#78100,#78101),(#78102,#78103),
(#78104,#78105),(#78106,#78107),(#78108,#78109),(#78110,#78111),(#78112,
#78113),(#78114,#78115),(#78116,#78117),(#78118,#78119)),.UNSPECIFIED.,
 .F.,.F.,.F.)
B_SPLINE_SURFACE_WITH_KNOTS((6,1,1,1,1,1,1,1,1,1,1,1,1,1,1,1,1,1,1,1,1,
1,1,1,1,1,1,1,1,1,1,1,1,1,1,1,1,1,1,1,1,1,1,1,1,1,1,1,1,1,1,1,1,1,1,1,1,
1,1,1,1,1,1,1,1,1,1,1,1,1,1,1,1,1,1,1,1,1,1,1,1,1,1,1,1,1,1,1,1,1,1,1,1,
1,1,1,1,1,1,1,1,1,1,1,1,1,1,1,1,1,1,1,1,1,1,1,1,1,1,1,1,1,1,1,1,1,1,1,1,
1,1,1,1,1,1,1,1,1,1,1,1,1,1,1,1,1,1,1,1,1,1,1,1,1,1,1,1,1,1,1,1,1,1,1,1,
1,1,1,1,1,1,1,1,1,1,1,1,1,1,1,1,1,1,1,1,1,1,1,1,1,1,1,1,1,1,1,1,1,1,1,6),
(2,2),(0.,0.005,0.01,0.015,0.02,0.025,0.03,0.035,0.04,0.045,0.05,0.055,
0.06,0.065,0.07,0.075,0.08,0.085,0.09,0.095,0.1,0.105,0.11,0.115,0.12,0.125,
0.13,0.135,0.14,0.145,0.15,0.155,0.16,0.165,0.17,0.175,0.18,0.185,0.19,
0.195,0.2,0.205,0.21,0.215,0.22,0.225,0.23,0.235,0.24,0.245,0.25,0.255,
0.26,0.265,0.27,0.275,0.28,0.285,0.29,0.295,0.3,0.305,0.31,0.315,0.32,0.325,
0.33,0.335,0.34,0.345,0.35,0.355,0.36,0.365,0.37,0.375,0.38,0.385,0.39,
0.395,0.4,0.405,0.41,0.415,0.42,0.425,0.43,0.435,0.44,0.445,0.45,0.455,
0.46,0.465,0.47,0.475,0.48,0.485,0.49,0.495,0.5,0.505,0.51,0.515,0.52,0.525,
0.53,0.535,0.54,0.545,0.55,0.555,0.56,0.565,0.57,0.575,0.58,0.585,0.59,
0.595,0.6,0.605,0.61,0.615,0.62,0.625,0.63,0.635,0.64,0.645,0.65,0.655,
0.66,0.665,0.67,0.675,0.68,0.685,0.690000000000001,0.695000000000001,0.700000000000001,
0.705000000000001,0.710000000000001,0.715000000000001,0.720000000000001,
0.725000000000001,0.730000000000001,0.735000000000001,0.740000000000001,
0.745000000000001,0.750000000000001,0.755000000000001,0.760000000000001,
0.765000000000001,0.770000000000001,0.775000000000001,0.780000000000001,
0.785000000000001,0.790000000000001,0.795000000000001,0.800000000000001,
0.805000000000001,0.810000000000001,0.815000000000001,0.820000000000001,
0.825000000000001,0.830000000000001,0.835000000000001,0.840000000000001,
0.845000000000001,0.850000000000001,0.855000000000001,0.860000000000001,
0.865000000000001,0.870000000000001,0.875000000000001,0.880000000000001,
0.885000000000001,0.890000000000001,0.895000000000001,0.900000000000001,
0.905000000000001,0.910000000000001,0.915000000000001,0.920000000000001,
0.925000000000001,0.930000000000001,0.935000000000001,0.940000000000001,
0.945000000000001,0.950000000000001,0.955000000000001,0.960000000000001,
0.965000000000001,0.970000000000001,0.975000000000001,0.980000000000001,
0.985000000000001,0.990000000000001,0.995000000000001,1.),(0.,1.2),
 .UNSPECIFIED.)
GEOMETRIC_REPRESENTATION_ITEM()
RATIONAL_B_SPLINE_SURFACE(((1.,1.),(1.,1.),(1.,1.),(1.,1.),(1.,1.),(1.,
1.),(1.,1.),(1.,1.),(1.,1.),(1.,1.),(1.,1.),(1.,1.),(1.,1.),(1.,1.),(1.,
1.),(1.,1.),(1.,1.),(1.,1.),(1.,1.),(1.,1.),(1.,1.),(1.,1.),(1.,1.),(1.,
1.),(1.,1.),(1.,1.),(1.,1.),(1.,1.),(1.,1.),(1.,1.),(1.,1.),(1.,1.),(1.,
1.),(1.,1.),(1.,1.),(1.,1.),(1.,1.),(1.,1.),(1.,1.),(1.,1.),(1.,1.),(1.,
1.),(1.,1.),(1.,1.),(1.,1.),(1.,1.),(1.,1.),(1.,1.),(1.,1.),(1.,1.),(1.,
1.),(1.,1.),(1.,1.),(1.,1.),(1.,1.),(1.,1.),(1.,1.),(1.,1.),(1.,1.),(1.,
1.),(1.,1.),(1.,1.),(1.,1.),(1.,1.),(1.,1.),(1.,1.),(1.,1.),(1.,1.),(1.,
1.),(1.,1.),(1.,1.),(1.,1.),(1.,1.),(1.,1.),(1.,1.),(1.,1.),(1.,1.),(1.,
1.),(1.,1.),(1.,1.),(1.,1.),(1.,1.),(1.,1.),(1.,1.),(1.,1.),(1.,1.),(1.,
1.),(1.,1.),(1.,1.),(1.,1.),(1.,1.),(1.,1.),(1.,1.),(1.,1.),(1.,1.),(1.,
1.),(1.,1.),(1.,1.),(1.,1.),(1.,1.),(1.,1.),(1.,1.),(1.,1.),(1.,1.),(1.,
1.),(1.,1.),(1.,1.),(1.,1.),(1.,1.),(1.,1.),(1.,1.),(1.,1.),(1.,1.),(1.,
1.),(1.,1.),(1.,1.),(1.,1.),(1.,1.),(1.,1.),(1.,1.),(1.,1.),(1.,1.),(1.,
1.),(1.,1.),(1.,1.),(1.,1.),(1.,1.),(1.,1.),(1.,1.),(1.,1.),(1.,1.),(1.,
1.),(1.,1.),(1.,1.),(1.,1.),(1.,1.),(1.,1.),(1.,1.),(1.,1.),(1.,1.),(1.,
1.),(1.,1.),(1.,1.),(1.,1.),(1.,1.),(1.,1.),(1.,1.),(1.,1.),(1.,1.),(1.,
1.),(1.,1.),(1.,1.),(1.,1.),(1.,1.),(1.,1.),(1.,1.),(1.,1.),(1.,1.),(1.,
1.),(1.,1.),(1.,1.),(1.,1.),(1.,1.),(1.,1.),(1.,1.),(1.,1.),(1.,1.),(1.,
1.),(1.,1.),(1.,1.),(1.,1.),(1.,1.),(1.,1.),(1.,1.),(1.,1.),(1.,1.),(1.,
1.),(1.,1.),(1.,1.),(1.,1.),(1.,1.),(1.,1.),(1.,1.),(1.,1.),(1.,1.),(1.,
1.),(1.,1.),(1.,1.),(1.,1.),(1.,1.),(1.,1.),(1.,1.),(1.,1.),(1.,1.),(1.,
1.),(1.,1.),(1.,1.),(1.,1.),(1.,1.),(1.,1.),(1.,1.),(1.,1.),(1.,1.),(1.,
1.),(1.,1.)))
REPRESENTATION_ITEM('')
SURFACE()
);
#912=(
BOUNDED_SURFACE()
B_SPLINE_SURFACE(5,1,((#78606,#78607),(#78608,#78609),(#78610,#78611),(#78612,
#78613),(#78614,#78615),(#78616,#78617),(#78618,#78619),(#78620,#78621),
(#78622,#78623),(#78624,#78625),(#78626,#78627),(#78628,#78629),(#78630,
#78631),(#78632,#78633),(#78634,#78635),(#78636,#78637),(#78638,#78639),
(#78640,#78641),(#78642,#78643),(#78644,#78645),(#78646,#78647),(#78648,
#78649),(#78650,#78651),(#78652,#78653),(#78654,#78655),(#78656,#78657),
(#78658,#78659),(#78660,#78661),(#78662,#78663),(#78664,#78665),(#78666,
#78667),(#78668,#78669),(#78670,#78671),(#78672,#78673),(#78674,#78675),
(#78676,#78677),(#78678,#78679),(#78680,#78681),(#78682,#78683),(#78684,
#78685),(#78686,#78687),(#78688,#78689),(#78690,#78691),(#78692,#78693),
(#78694,#78695),(#78696,#78697),(#78698,#78699),(#78700,#78701),(#78702,
#78703),(#78704,#78705),(#78706,#78707),(#78708,#78709),(#78710,#78711),
(#78712,#78713),(#78714,#78715),(#78716,#78717),(#78718,#78719),(#78720,
#78721),(#78722,#78723),(#78724,#78725),(#78726,#78727),(#78728,#78729),
(#78730,#78731),(#78732,#78733),(#78734,#78735),(#78736,#78737),(#78738,
#78739),(#78740,#78741),(#78742,#78743),(#78744,#78745),(#78746,#78747),
(#78748,#78749),(#78750,#78751),(#78752,#78753),(#78754,#78755),(#78756,
#78757),(#78758,#78759),(#78760,#78761),(#78762,#78763),(#78764,#78765),
(#78766,#78767),(#78768,#78769),(#78770,#78771),(#78772,#78773),(#78774,
#78775),(#78776,#78777),(#78778,#78779),(#78780,#78781),(#78782,#78783),
(#78784,#78785),(#78786,#78787),(#78788,#78789),(#78790,#78791),(#78792,
#78793),(#78794,#78795),(#78796,#78797),(#78798,#78799),(#78800,#78801),
(#78802,#78803),(#78804,#78805),(#78806,#78807),(#78808,#78809),(#78810,
#78811),(#78812,#78813),(#78814,#78815),(#78816,#78817),(#78818,#78819),
(#78820,#78821),(#78822,#78823),(#78824,#78825),(#78826,#78827),(#78828,
#78829),(#78830,#78831),(#78832,#78833),(#78834,#78835),(#78836,#78837),
(#78838,#78839),(#78840,#78841),(#78842,#78843),(#78844,#78845),(#78846,
#78847),(#78848,#78849),(#78850,#78851),(#78852,#78853),(#78854,#78855),
(#78856,#78857),(#78858,#78859),(#78860,#78861),(#78862,#78863),(#78864,
#78865),(#78866,#78867),(#78868,#78869),(#78870,#78871),(#78872,#78873),
(#78874,#78875),(#78876,#78877),(#78878,#78879),(#78880,#78881),(#78882,
#78883),(#78884,#78885),(#78886,#78887),(#78888,#78889),(#78890,#78891),
(#78892,#78893),(#78894,#78895),(#78896,#78897),(#78898,#78899),(#78900,
#78901),(#78902,#78903),(#78904,#78905),(#78906,#78907),(#78908,#78909),
(#78910,#78911),(#78912,#78913),(#78914,#78915),(#78916,#78917),(#78918,
#78919),(#78920,#78921),(#78922,#78923),(#78924,#78925),(#78926,#78927),
(#78928,#78929),(#78930,#78931),(#78932,#78933),(#78934,#78935),(#78936,
#78937),(#78938,#78939),(#78940,#78941),(#78942,#78943),(#78944,#78945),
(#78946,#78947),(#78948,#78949),(#78950,#78951),(#78952,#78953),(#78954,
#78955),(#78956,#78957),(#78958,#78959),(#78960,#78961),(#78962,#78963),
(#78964,#78965),(#78966,#78967),(#78968,#78969),(#78970,#78971),(#78972,
#78973),(#78974,#78975),(#78976,#78977),(#78978,#78979),(#78980,#78981),
(#78982,#78983),(#78984,#78985),(#78986,#78987),(#78988,#78989),(#78990,
#78991),(#78992,#78993),(#78994,#78995),(#78996,#78997),(#78998,#78999),
(#79000,#79001),(#79002,#79003),(#79004,#79005),(#79006,#79007),(#79008,
#79009),(#79010,#79011),(#79012,#79013),(#79014,#79015)),.UNSPECIFIED.,
 .F.,.F.,.F.)
B_SPLINE_SURFACE_WITH_KNOTS((6,1,1,1,1,1,1,1,1,1,1,1,1,1,1,1,1,1,1,1,1,
1,1,1,1,1,1,1,1,1,1,1,1,1,1,1,1,1,1,1,1,1,1,1,1,1,1,1,1,1,1,1,1,1,1,1,1,
1,1,1,1,1,1,1,1,1,1,1,1,1,1,1,1,1,1,1,1,1,1,1,1,1,1,1,1,1,1,1,1,1,1,1,1,
1,1,1,1,1,1,1,1,1,1,1,1,1,1,1,1,1,1,1,1,1,1,1,1,1,1,1,1,1,1,1,1,1,1,1,1,
1,1,1,1,1,1,1,1,1,1,1,1,1,1,1,1,1,1,1,1,1,1,1,1,1,1,1,1,1,1,1,1,1,1,1,1,
1,1,1,1,1,1,1,1,1,1,1,1,1,1,1,1,1,1,1,1,1,1,1,1,1,1,1,1,1,1,1,1,1,1,1,6),
(2,2),(0.,0.005,0.01,0.015,0.02,0.025,0.03,0.035,0.04,0.045,0.05,0.055,
0.06,0.065,0.07,0.075,0.08,0.085,0.09,0.095,0.1,0.105,0.11,0.115,0.12,0.125,
0.13,0.135,0.14,0.145,0.15,0.155,0.16,0.165,0.17,0.175,0.18,0.185,0.19,
0.195,0.2,0.205,0.21,0.215,0.22,0.225,0.23,0.235,0.24,0.245,0.25,0.255,
0.26,0.265,0.27,0.275,0.28,0.285,0.29,0.295,0.3,0.305,0.31,0.315,0.32,0.325,
0.33,0.335,0.34,0.345,0.35,0.355,0.36,0.365,0.37,0.375,0.38,0.385,0.39,
0.395,0.4,0.405,0.41,0.415,0.42,0.425,0.43,0.435,0.44,0.445,0.45,0.455,
0.46,0.465,0.47,0.475,0.48,0.485,0.49,0.495,0.5,0.505,0.51,0.515,0.52,0.525,
0.53,0.535,0.54,0.545,0.55,0.555,0.56,0.565,0.57,0.575,0.58,0.585,0.59,
0.595,0.6,0.605,0.61,0.615,0.62,0.625,0.63,0.635,0.64,0.645,0.65,0.655,
0.66,0.665,0.67,0.675,0.68,0.685,0.690000000000001,0.695000000000001,0.700000000000001,
0.705000000000001,0.710000000000001,0.715000000000001,0.720000000000001,
0.725000000000001,0.730000000000001,0.735000000000001,0.740000000000001,
0.745000000000001,0.750000000000001,0.755000000000001,0.760000000000001,
0.765000000000001,0.770000000000001,0.775000000000001,0.780000000000001,
0.785000000000001,0.790000000000001,0.795000000000001,0.800000000000001,
0.805000000000001,0.810000000000001,0.815000000000001,0.820000000000001,
0.825000000000001,0.830000000000001,0.835000000000001,0.840000000000001,
0.845000000000001,0.850000000000001,0.855000000000001,0.860000000000001,
0.865000000000001,0.870000000000001,0.875000000000001,0.880000000000001,
0.885000000000001,0.890000000000001,0.895000000000001,0.900000000000001,
0.905000000000001,0.910000000000001,0.915000000000001,0.920000000000001,
0.925000000000001,0.930000000000001,0.935000000000001,0.940000000000001,
0.945000000000001,0.950000000000001,0.955000000000001,0.960000000000001,
0.965000000000001,0.970000000000001,0.975000000000001,0.980000000000001,
0.985000000000001,0.990000000000001,0.995000000000001,1.),(0.,1.2),
 .UNSPECIFIED.)
GEOMETRIC_REPRESENTATION_ITEM()
RATIONAL_B_SPLINE_SURFACE(((1.,1.),(1.,1.),(1.,1.),(1.,1.),(1.,1.),(1.,
1.),(1.,1.),(1.,1.),(1.,1.),(1.,1.),(1.,1.),(1.,1.),(1.,1.),(1.,1.),(1.,
1.),(1.,1.),(1.,1.),(1.,1.),(1.,1.),(1.,1.),(1.,1.),(1.,1.),(1.,1.),(1.,
1.),(1.,1.),(1.,1.),(1.,1.),(1.,1.),(1.,1.),(1.,1.),(1.,1.),(1.,1.),(1.,
1.),(1.,1.),(1.,1.),(1.,1.),(1.,1.),(1.,1.),(1.,1.),(1.,1.),(1.,1.),(1.,
1.),(1.,1.),(1.,1.),(1.,1.),(1.,1.),(1.,1.),(1.,1.),(1.,1.),(1.,1.),(1.,
1.),(1.,1.),(1.,1.),(1.,1.),(1.,1.),(1.,1.),(1.,1.),(1.,1.),(1.,1.),(1.,
1.),(1.,1.),(1.,1.),(1.,1.),(1.,1.),(1.,1.),(1.,1.),(1.,1.),(1.,1.),(1.,
1.),(1.,1.),(1.,1.),(1.,1.),(1.,1.),(1.,1.),(1.,1.),(1.,1.),(1.,1.),(1.,
1.),(1.,1.),(1.,1.),(1.,1.),(1.,1.),(1.,1.),(1.,1.),(1.,1.),(1.,1.),(1.,
1.),(1.,1.),(1.,1.),(1.,1.),(1.,1.),(1.,1.),(1.,1.),(1.,1.),(1.,1.),(1.,
1.),(1.,1.),(1.,1.),(1.,1.),(1.,1.),(1.,1.),(1.,1.),(1.,1.),(1.,1.),(1.,
1.),(1.,1.),(1.,1.),(1.,1.),(1.,1.),(1.,1.),(1.,1.),(1.,1.),(1.,1.),(1.,
1.),(1.,1.),(1.,1.),(1.,1.),(1.,1.),(1.,1.),(1.,1.),(1.,1.),(1.,1.),(1.,
1.),(1.,1.),(1.,1.),(1.,1.),(1.,1.),(1.,1.),(1.,1.),(1.,1.),(1.,1.),(1.,
1.),(1.,1.),(1.,1.),(1.,1.),(1.,1.),(1.,1.),(1.,1.),(1.,1.),(1.,1.),(1.,
1.),(1.,1.),(1.,1.),(1.,1.),(1.,1.),(1.,1.),(1.,1.),(1.,1.),(1.,1.),(1.,
1.),(1.,1.),(1.,1.),(1.,1.),(1.,1.),(1.,1.),(1.,1.),(1.,1.),(1.,1.),(1.,
1.),(1.,1.),(1.,1.),(1.,1.),(1.,1.),(1.,1.),(1.,1.),(1.,1.),(1.,1.),(1.,
1.),(1.,1.),(1.,1.),(1.,1.),(1.,1.),(1.,1.),(1.,1.),(1.,1.),(1.,1.),(1.,
1.),(1.,1.),(1.,1.),(1.,1.),(1.,1.),(1.,1.),(1.,1.),(1.,1.),(1.,1.),(1.,
1.),(1.,1.),(1.,1.),(1.,1.),(1.,1.),(1.,1.),(1.,1.),(1.,1.),(1.,1.),(1.,
1.),(1.,1.),(1.,1.),(1.,1.),(1.,1.),(1.,1.),(1.,1.),(1.,1.),(1.,1.),(1.,
1.),(1.,1.)))
REPRESENTATION_ITEM('')
SURFACE()
);
#913=(
BOUNDED_SURFACE()
B_SPLINE_SURFACE(5,1,((#79502,#79503),(#79504,#79505),(#79506,#79507),(#79508,
#79509),(#79510,#79511),(#79512,#79513),(#79514,#79515),(#79516,#79517),
(#79518,#79519),(#79520,#79521),(#79522,#79523),(#79524,#79525),(#79526,
#79527),(#79528,#79529),(#79530,#79531),(#79532,#79533),(#79534,#79535),
(#79536,#79537),(#79538,#79539),(#79540,#79541),(#79542,#79543),(#79544,
#79545),(#79546,#79547),(#79548,#79549),(#79550,#79551),(#79552,#79553),
(#79554,#79555),(#79556,#79557),(#79558,#79559),(#79560,#79561),(#79562,
#79563),(#79564,#79565),(#79566,#79567),(#79568,#79569),(#79570,#79571),
(#79572,#79573),(#79574,#79575),(#79576,#79577),(#79578,#79579),(#79580,
#79581),(#79582,#79583),(#79584,#79585),(#79586,#79587),(#79588,#79589),
(#79590,#79591),(#79592,#79593),(#79594,#79595),(#79596,#79597),(#79598,
#79599),(#79600,#79601),(#79602,#79603),(#79604,#79605),(#79606,#79607),
(#79608,#79609),(#79610,#79611),(#79612,#79613),(#79614,#79615),(#79616,
#79617),(#79618,#79619),(#79620,#79621),(#79622,#79623),(#79624,#79625),
(#79626,#79627),(#79628,#79629),(#79630,#79631),(#79632,#79633),(#79634,
#79635),(#79636,#79637),(#79638,#79639),(#79640,#79641),(#79642,#79643),
(#79644,#79645),(#79646,#79647),(#79648,#79649),(#79650,#79651),(#79652,
#79653),(#79654,#79655),(#79656,#79657),(#79658,#79659),(#79660,#79661),
(#79662,#79663),(#79664,#79665),(#79666,#79667),(#79668,#79669),(#79670,
#79671),(#79672,#79673),(#79674,#79675),(#79676,#79677),(#79678,#79679),
(#79680,#79681),(#79682,#79683),(#79684,#79685),(#79686,#79687),(#79688,
#79689),(#79690,#79691),(#79692,#79693),(#79694,#79695),(#79696,#79697),
(#79698,#79699),(#79700,#79701),(#79702,#79703),(#79704,#79705),(#79706,
#79707),(#79708,#79709),(#79710,#79711),(#79712,#79713),(#79714,#79715),
(#79716,#79717),(#79718,#79719),(#79720,#79721),(#79722,#79723),(#79724,
#79725),(#79726,#79727),(#79728,#79729),(#79730,#79731),(#79732,#79733),
(#79734,#79735),(#79736,#79737),(#79738,#79739),(#79740,#79741),(#79742,
#79743),(#79744,#79745),(#79746,#79747),(#79748,#79749),(#79750,#79751),
(#79752,#79753),(#79754,#79755),(#79756,#79757),(#79758,#79759),(#79760,
#79761),(#79762,#79763),(#79764,#79765),(#79766,#79767),(#79768,#79769),
(#79770,#79771),(#79772,#79773),(#79774,#79775),(#79776,#79777),(#79778,
#79779),(#79780,#79781),(#79782,#79783),(#79784,#79785),(#79786,#79787),
(#79788,#79789),(#79790,#79791),(#79792,#79793),(#79794,#79795),(#79796,
#79797),(#79798,#79799),(#79800,#79801),(#79802,#79803),(#79804,#79805),
(#79806,#79807),(#79808,#79809),(#79810,#79811),(#79812,#79813),(#79814,
#79815),(#79816,#79817),(#79818,#79819),(#79820,#79821),(#79822,#79823),
(#79824,#79825),(#79826,#79827),(#79828,#79829),(#79830,#79831),(#79832,
#79833),(#79834,#79835),(#79836,#79837),(#79838,#79839),(#79840,#79841),
(#79842,#79843),(#79844,#79845),(#79846,#79847),(#79848,#79849),(#79850,
#79851),(#79852,#79853),(#79854,#79855),(#79856,#79857),(#79858,#79859),
(#79860,#79861),(#79862,#79863),(#79864,#79865),(#79866,#79867),(#79868,
#79869),(#79870,#79871),(#79872,#79873),(#79874,#79875),(#79876,#79877),
(#79878,#79879),(#79880,#79881),(#79882,#79883),(#79884,#79885),(#79886,
#79887),(#79888,#79889),(#79890,#79891),(#79892,#79893),(#79894,#79895),
(#79896,#79897),(#79898,#79899),(#79900,#79901),(#79902,#79903),(#79904,
#79905),(#79906,#79907),(#79908,#79909),(#79910,#79911)),.UNSPECIFIED.,
 .F.,.F.,.F.)
B_SPLINE_SURFACE_WITH_KNOTS((6,1,1,1,1,1,1,1,1,1,1,1,1,1,1,1,1,1,1,1,1,
1,1,1,1,1,1,1,1,1,1,1,1,1,1,1,1,1,1,1,1,1,1,1,1,1,1,1,1,1,1,1,1,1,1,1,1,
1,1,1,1,1,1,1,1,1,1,1,1,1,1,1,1,1,1,1,1,1,1,1,1,1,1,1,1,1,1,1,1,1,1,1,1,
1,1,1,1,1,1,1,1,1,1,1,1,1,1,1,1,1,1,1,1,1,1,1,1,1,1,1,1,1,1,1,1,1,1,1,1,
1,1,1,1,1,1,1,1,1,1,1,1,1,1,1,1,1,1,1,1,1,1,1,1,1,1,1,1,1,1,1,1,1,1,1,1,
1,1,1,1,1,1,1,1,1,1,1,1,1,1,1,1,1,1,1,1,1,1,1,1,1,1,1,1,1,1,1,1,1,1,1,6),
(2,2),(0.,0.005,0.01,0.015,0.02,0.025,0.03,0.035,0.04,0.045,0.05,0.055,
0.06,0.065,0.07,0.075,0.08,0.085,0.09,0.095,0.1,0.105,0.11,0.115,0.12,0.125,
0.13,0.135,0.14,0.145,0.15,0.155,0.16,0.165,0.17,0.175,0.18,0.185,0.19,
0.195,0.2,0.205,0.21,0.215,0.22,0.225,0.23,0.235,0.24,0.245,0.25,0.255,
0.26,0.265,0.27,0.275,0.28,0.285,0.29,0.295,0.3,0.305,0.31,0.315,0.32,0.325,
0.33,0.335,0.34,0.345,0.35,0.355,0.36,0.365,0.37,0.375,0.38,0.385,0.39,
0.395,0.4,0.405,0.41,0.415,0.42,0.425,0.43,0.435,0.44,0.445,0.45,0.455,
0.46,0.465,0.47,0.475,0.48,0.485,0.49,0.495,0.5,0.505,0.51,0.515,0.52,0.525,
0.53,0.535,0.54,0.545,0.55,0.555,0.56,0.565,0.57,0.575,0.58,0.585,0.59,
0.595,0.6,0.605,0.61,0.615,0.62,0.625,0.63,0.635,0.64,0.645,0.65,0.655,
0.66,0.665,0.67,0.675,0.68,0.685,0.690000000000001,0.695000000000001,0.700000000000001,
0.705000000000001,0.710000000000001,0.715000000000001,0.720000000000001,
0.725000000000001,0.730000000000001,0.735000000000001,0.740000000000001,
0.745000000000001,0.750000000000001,0.755000000000001,0.760000000000001,
0.765000000000001,0.770000000000001,0.775000000000001,0.780000000000001,
0.785000000000001,0.790000000000001,0.795000000000001,0.800000000000001,
0.805000000000001,0.810000000000001,0.815000000000001,0.820000000000001,
0.825000000000001,0.830000000000001,0.835000000000001,0.840000000000001,
0.845000000000001,0.850000000000001,0.855000000000001,0.860000000000001,
0.865000000000001,0.870000000000001,0.875000000000001,0.880000000000001,
0.885000000000001,0.890000000000001,0.895000000000001,0.900000000000001,
0.905000000000001,0.910000000000001,0.915000000000001,0.920000000000001,
0.925000000000001,0.930000000000001,0.935000000000001,0.940000000000001,
0.945000000000001,0.950000000000001,0.955000000000001,0.960000000000001,
0.965000000000001,0.970000000000001,0.975000000000001,0.980000000000001,
0.985000000000001,0.990000000000001,0.995000000000001,1.),(0.,1.2),
 .UNSPECIFIED.)
GEOMETRIC_REPRESENTATION_ITEM()
RATIONAL_B_SPLINE_SURFACE(((1.,1.),(1.,1.),(1.,1.),(1.,1.),(1.,1.),(1.,
1.),(1.,1.),(1.,1.),(1.,1.),(1.,1.),(1.,1.),(1.,1.),(1.,1.),(1.,1.),(1.,
1.),(1.,1.),(1.,1.),(1.,1.),(1.,1.),(1.,1.),(1.,1.),(1.,1.),(1.,1.),(1.,
1.),(1.,1.),(1.,1.),(1.,1.),(1.,1.),(1.,1.),(1.,1.),(1.,1.),(1.,1.),(1.,
1.),(1.,1.),(1.,1.),(1.,1.),(1.,1.),(1.,1.),(1.,1.),(1.,1.),(1.,1.),(1.,
1.),(1.,1.),(1.,1.),(1.,1.),(1.,1.),(1.,1.),(1.,1.),(1.,1.),(1.,1.),(1.,
1.),(1.,1.),(1.,1.),(1.,1.),(1.,1.),(1.,1.),(1.,1.),(1.,1.),(1.,1.),(1.,
1.),(1.,1.),(1.,1.),(1.,1.),(1.,1.),(1.,1.),(1.,1.),(1.,1.),(1.,1.),(1.,
1.),(1.,1.),(1.,1.),(1.,1.),(1.,1.),(1.,1.),(1.,1.),(1.,1.),(1.,1.),(1.,
1.),(1.,1.),(1.,1.),(1.,1.),(1.,1.),(1.,1.),(1.,1.),(1.,1.),(1.,1.),(1.,
1.),(1.,1.),(1.,1.),(1.,1.),(1.,1.),(1.,1.),(1.,1.),(1.,1.),(1.,1.),(1.,
1.),(1.,1.),(1.,1.),(1.,1.),(1.,1.),(1.,1.),(1.,1.),(1.,1.),(1.,1.),(1.,
1.),(1.,1.),(1.,1.),(1.,1.),(1.,1.),(1.,1.),(1.,1.),(1.,1.),(1.,1.),(1.,
1.),(1.,1.),(1.,1.),(1.,1.),(1.,1.),(1.,1.),(1.,1.),(1.,1.),(1.,1.),(1.,
1.),(1.,1.),(1.,1.),(1.,1.),(1.,1.),(1.,1.),(1.,1.),(1.,1.),(1.,1.),(1.,
1.),(1.,1.),(1.,1.),(1.,1.),(1.,1.),(1.,1.),(1.,1.),(1.,1.),(1.,1.),(1.,
1.),(1.,1.),(1.,1.),(1.,1.),(1.,1.),(1.,1.),(1.,1.),(1.,1.),(1.,1.),(1.,
1.),(1.,1.),(1.,1.),(1.,1.),(1.,1.),(1.,1.),(1.,1.),(1.,1.),(1.,1.),(1.,
1.),(1.,1.),(1.,1.),(1.,1.),(1.,1.),(1.,1.),(1.,1.),(1.,1.),(1.,1.),(1.,
1.),(1.,1.),(1.,1.),(1.,1.),(1.,1.),(1.,1.),(1.,1.),(1.,1.),(1.,1.),(1.,
1.),(1.,1.),(1.,1.),(1.,1.),(1.,1.),(1.,1.),(1.,1.),(1.,1.),(1.,1.),(1.,
1.),(1.,1.),(1.,1.),(1.,1.),(1.,1.),(1.,1.),(1.,1.),(1.,1.),(1.,1.),(1.,
1.),(1.,1.),(1.,1.),(1.,1.),(1.,1.),(1.,1.),(1.,1.),(1.,1.),(1.,1.),(1.,
1.),(1.,1.)))
REPRESENTATION_ITEM('')
SURFACE()
);
#914=(
BOUNDED_SURFACE()
B_SPLINE_SURFACE(5,1,((#80398,#80399),(#80400,#80401),(#80402,#80403),(#80404,
#80405),(#80406,#80407),(#80408,#80409),(#80410,#80411),(#80412,#80413),
(#80414,#80415),(#80416,#80417),(#80418,#80419),(#80420,#80421),(#80422,
#80423),(#80424,#80425),(#80426,#80427),(#80428,#80429),(#80430,#80431),
(#80432,#80433),(#80434,#80435),(#80436,#80437),(#80438,#80439),(#80440,
#80441),(#80442,#80443),(#80444,#80445),(#80446,#80447),(#80448,#80449),
(#80450,#80451),(#80452,#80453),(#80454,#80455),(#80456,#80457),(#80458,
#80459),(#80460,#80461),(#80462,#80463),(#80464,#80465),(#80466,#80467),
(#80468,#80469),(#80470,#80471),(#80472,#80473),(#80474,#80475),(#80476,
#80477),(#80478,#80479),(#80480,#80481),(#80482,#80483),(#80484,#80485),
(#80486,#80487),(#80488,#80489),(#80490,#80491),(#80492,#80493),(#80494,
#80495),(#80496,#80497),(#80498,#80499),(#80500,#80501),(#80502,#80503),
(#80504,#80505),(#80506,#80507),(#80508,#80509),(#80510,#80511),(#80512,
#80513),(#80514,#80515),(#80516,#80517),(#80518,#80519),(#80520,#80521),
(#80522,#80523),(#80524,#80525),(#80526,#80527),(#80528,#80529),(#80530,
#80531),(#80532,#80533),(#80534,#80535),(#80536,#80537),(#80538,#80539),
(#80540,#80541),(#80542,#80543),(#80544,#80545),(#80546,#80547),(#80548,
#80549),(#80550,#80551),(#80552,#80553),(#80554,#80555),(#80556,#80557),
(#80558,#80559),(#80560,#80561),(#80562,#80563),(#80564,#80565),(#80566,
#80567),(#80568,#80569),(#80570,#80571),(#80572,#80573),(#80574,#80575),
(#80576,#80577),(#80578,#80579),(#80580,#80581),(#80582,#80583),(#80584,
#80585),(#80586,#80587),(#80588,#80589),(#80590,#80591),(#80592,#80593),
(#80594,#80595),(#80596,#80597),(#80598,#80599),(#80600,#80601),(#80602,
#80603),(#80604,#80605),(#80606,#80607),(#80608,#80609),(#80610,#80611),
(#80612,#80613),(#80614,#80615),(#80616,#80617),(#80618,#80619),(#80620,
#80621),(#80622,#80623),(#80624,#80625),(#80626,#80627),(#80628,#80629),
(#80630,#80631),(#80632,#80633),(#80634,#80635),(#80636,#80637),(#80638,
#80639),(#80640,#80641),(#80642,#80643),(#80644,#80645),(#80646,#80647),
(#80648,#80649),(#80650,#80651),(#80652,#80653),(#80654,#80655),(#80656,
#80657),(#80658,#80659),(#80660,#80661),(#80662,#80663),(#80664,#80665),
(#80666,#80667),(#80668,#80669),(#80670,#80671),(#80672,#80673),(#80674,
#80675),(#80676,#80677),(#80678,#80679),(#80680,#80681),(#80682,#80683),
(#80684,#80685),(#80686,#80687),(#80688,#80689),(#80690,#80691),(#80692,
#80693),(#80694,#80695),(#80696,#80697),(#80698,#80699),(#80700,#80701),
(#80702,#80703),(#80704,#80705),(#80706,#80707),(#80708,#80709),(#80710,
#80711),(#80712,#80713),(#80714,#80715),(#80716,#80717),(#80718,#80719),
(#80720,#80721),(#80722,#80723),(#80724,#80725),(#80726,#80727),(#80728,
#80729),(#80730,#80731),(#80732,#80733),(#80734,#80735),(#80736,#80737),
(#80738,#80739),(#80740,#80741),(#80742,#80743),(#80744,#80745),(#80746,
#80747),(#80748,#80749),(#80750,#80751),(#80752,#80753),(#80754,#80755),
(#80756,#80757),(#80758,#80759),(#80760,#80761),(#80762,#80763),(#80764,
#80765),(#80766,#80767),(#80768,#80769),(#80770,#80771),(#80772,#80773),
(#80774,#80775),(#80776,#80777),(#80778,#80779),(#80780,#80781),(#80782,
#80783),(#80784,#80785),(#80786,#80787),(#80788,#80789),(#80790,#80791),
(#80792,#80793),(#80794,#80795),(#80796,#80797),(#80798,#80799),(#80800,
#80801),(#80802,#80803),(#80804,#80805),(#80806,#80807)),.UNSPECIFIED.,
 .F.,.F.,.F.)
B_SPLINE_SURFACE_WITH_KNOTS((6,1,1,1,1,1,1,1,1,1,1,1,1,1,1,1,1,1,1,1,1,
1,1,1,1,1,1,1,1,1,1,1,1,1,1,1,1,1,1,1,1,1,1,1,1,1,1,1,1,1,1,1,1,1,1,1,1,
1,1,1,1,1,1,1,1,1,1,1,1,1,1,1,1,1,1,1,1,1,1,1,1,1,1,1,1,1,1,1,1,1,1,1,1,
1,1,1,1,1,1,1,1,1,1,1,1,1,1,1,1,1,1,1,1,1,1,1,1,1,1,1,1,1,1,1,1,1,1,1,1,
1,1,1,1,1,1,1,1,1,1,1,1,1,1,1,1,1,1,1,1,1,1,1,1,1,1,1,1,1,1,1,1,1,1,1,1,
1,1,1,1,1,1,1,1,1,1,1,1,1,1,1,1,1,1,1,1,1,1,1,1,1,1,1,1,1,1,1,1,1,1,1,6),
(2,2),(0.,0.005,0.01,0.015,0.02,0.025,0.03,0.035,0.04,0.045,0.05,0.055,
0.06,0.065,0.07,0.075,0.08,0.085,0.09,0.095,0.1,0.105,0.11,0.115,0.12,0.125,
0.13,0.135,0.14,0.145,0.15,0.155,0.16,0.165,0.17,0.175,0.18,0.185,0.19,
0.195,0.2,0.205,0.21,0.215,0.22,0.225,0.23,0.235,0.24,0.245,0.25,0.255,
0.26,0.265,0.27,0.275,0.28,0.285,0.29,0.295,0.3,0.305,0.31,0.315,0.32,0.325,
0.33,0.335,0.34,0.345,0.35,0.355,0.36,0.365,0.37,0.375,0.38,0.385,0.39,
0.395,0.4,0.405,0.41,0.415,0.42,0.425,0.43,0.435,0.44,0.445,0.45,0.455,
0.46,0.465,0.47,0.475,0.48,0.485,0.49,0.495,0.5,0.505,0.51,0.515,0.52,0.525,
0.53,0.535,0.54,0.545,0.55,0.555,0.56,0.565,0.57,0.575,0.58,0.585,0.59,
0.595,0.6,0.605,0.61,0.615,0.62,0.625,0.63,0.635,0.64,0.645,0.65,0.655,
0.66,0.665,0.67,0.675,0.68,0.685,0.690000000000001,0.695000000000001,0.700000000000001,
0.705000000000001,0.710000000000001,0.715000000000001,0.720000000000001,
0.725000000000001,0.730000000000001,0.735000000000001,0.740000000000001,
0.745000000000001,0.750000000000001,0.755000000000001,0.760000000000001,
0.765000000000001,0.770000000000001,0.775000000000001,0.780000000000001,
0.785000000000001,0.790000000000001,0.795000000000001,0.800000000000001,
0.805000000000001,0.810000000000001,0.815000000000001,0.820000000000001,
0.825000000000001,0.830000000000001,0.835000000000001,0.840000000000001,
0.845000000000001,0.850000000000001,0.855000000000001,0.860000000000001,
0.865000000000001,0.870000000000001,0.875000000000001,0.880000000000001,
0.885000000000001,0.890000000000001,0.895000000000001,0.900000000000001,
0.905000000000001,0.910000000000001,0.915000000000001,0.920000000000001,
0.925000000000001,0.930000000000001,0.935000000000001,0.940000000000001,
0.945000000000001,0.950000000000001,0.955000000000001,0.960000000000001,
0.965000000000001,0.970000000000001,0.975000000000001,0.980000000000001,
0.985000000000001,0.990000000000001,0.995000000000001,1.),(0.,1.2),
 .UNSPECIFIED.)
GEOMETRIC_REPRESENTATION_ITEM()
RATIONAL_B_SPLINE_SURFACE(((1.,1.),(1.,1.),(1.,1.),(1.,1.),(1.,1.),(1.,
1.),(1.,1.),(1.,1.),(1.,1.),(1.,1.),(1.,1.),(1.,1.),(1.,1.),(1.,1.),(1.,
1.),(1.,1.),(1.,1.),(1.,1.),(1.,1.),(1.,1.),(1.,1.),(1.,1.),(1.,1.),(1.,
1.),(1.,1.),(1.,1.),(1.,1.),(1.,1.),(1.,1.),(1.,1.),(1.,1.),(1.,1.),(1.,
1.),(1.,1.),(1.,1.),(1.,1.),(1.,1.),(1.,1.),(1.,1.),(1.,1.),(1.,1.),(1.,
1.),(1.,1.),(1.,1.),(1.,1.),(1.,1.),(1.,1.),(1.,1.),(1.,1.),(1.,1.),(1.,
1.),(1.,1.),(1.,1.),(1.,1.),(1.,1.),(1.,1.),(1.,1.),(1.,1.),(1.,1.),(1.,
1.),(1.,1.),(1.,1.),(1.,1.),(1.,1.),(1.,1.),(1.,1.),(1.,1.),(1.,1.),(1.,
1.),(1.,1.),(1.,1.),(1.,1.),(1.,1.),(1.,1.),(1.,1.),(1.,1.),(1.,1.),(1.,
1.),(1.,1.),(1.,1.),(1.,1.),(1.,1.),(1.,1.),(1.,1.),(1.,1.),(1.,1.),(1.,
1.),(1.,1.),(1.,1.),(1.,1.),(1.,1.),(1.,1.),(1.,1.),(1.,1.),(1.,1.),(1.,
1.),(1.,1.),(1.,1.),(1.,1.),(1.,1.),(1.,1.),(1.,1.),(1.,1.),(1.,1.),(1.,
1.),(1.,1.),(1.,1.),(1.,1.),(1.,1.),(1.,1.),(1.,1.),(1.,1.),(1.,1.),(1.,
1.),(1.,1.),(1.,1.),(1.,1.),(1.,1.),(1.,1.),(1.,1.),(1.,1.),(1.,1.),(1.,
1.),(1.,1.),(1.,1.),(1.,1.),(1.,1.),(1.,1.),(1.,1.),(1.,1.),(1.,1.),(1.,
1.),(1.,1.),(1.,1.),(1.,1.),(1.,1.),(1.,1.),(1.,1.),(1.,1.),(1.,1.),(1.,
1.),(1.,1.),(1.,1.),(1.,1.),(1.,1.),(1.,1.),(1.,1.),(1.,1.),(1.,1.),(1.,
1.),(1.,1.),(1.,1.),(1.,1.),(1.,1.),(1.,1.),(1.,1.),(1.,1.),(1.,1.),(1.,
1.),(1.,1.),(1.,1.),(1.,1.),(1.,1.),(1.,1.),(1.,1.),(1.,1.),(1.,1.),(1.,
1.),(1.,1.),(1.,1.),(1.,1.),(1.,1.),(1.,1.),(1.,1.),(1.,1.),(1.,1.),(1.,
1.),(1.,1.),(1.,1.),(1.,1.),(1.,1.),(1.,1.),(1.,1.),(1.,1.),(1.,1.),(1.,
1.),(1.,1.),(1.,1.),(1.,1.),(1.,1.),(1.,1.),(1.,1.),(1.,1.),(1.,1.),(1.,
1.),(1.,1.),(1.,1.),(1.,1.),(1.,1.),(1.,1.),(1.,1.),(1.,1.),(1.,1.),(1.,
1.),(1.,1.)))
REPRESENTATION_ITEM('')
SURFACE()
);
#915=(
BOUNDED_SURFACE()
B_SPLINE_SURFACE(5,1,((#81294,#81295),(#81296,#81297),(#81298,#81299),(#81300,
#81301),(#81302,#81303),(#81304,#81305),(#81306,#81307),(#81308,#81309),
(#81310,#81311),(#81312,#81313),(#81314,#81315),(#81316,#81317),(#81318,
#81319),(#81320,#81321),(#81322,#81323),(#81324,#81325),(#81326,#81327),
(#81328,#81329),(#81330,#81331),(#81332,#81333),(#81334,#81335),(#81336,
#81337),(#81338,#81339),(#81340,#81341),(#81342,#81343),(#81344,#81345),
(#81346,#81347),(#81348,#81349),(#81350,#81351),(#81352,#81353),(#81354,
#81355),(#81356,#81357),(#81358,#81359),(#81360,#81361),(#81362,#81363),
(#81364,#81365),(#81366,#81367),(#81368,#81369),(#81370,#81371),(#81372,
#81373),(#81374,#81375),(#81376,#81377),(#81378,#81379),(#81380,#81381),
(#81382,#81383),(#81384,#81385),(#81386,#81387),(#81388,#81389),(#81390,
#81391),(#81392,#81393),(#81394,#81395),(#81396,#81397),(#81398,#81399),
(#81400,#81401),(#81402,#81403),(#81404,#81405),(#81406,#81407),(#81408,
#81409),(#81410,#81411),(#81412,#81413),(#81414,#81415),(#81416,#81417),
(#81418,#81419),(#81420,#81421),(#81422,#81423),(#81424,#81425),(#81426,
#81427),(#81428,#81429),(#81430,#81431),(#81432,#81433),(#81434,#81435),
(#81436,#81437),(#81438,#81439),(#81440,#81441),(#81442,#81443),(#81444,
#81445),(#81446,#81447),(#81448,#81449),(#81450,#81451),(#81452,#81453),
(#81454,#81455),(#81456,#81457),(#81458,#81459),(#81460,#81461),(#81462,
#81463),(#81464,#81465),(#81466,#81467),(#81468,#81469),(#81470,#81471),
(#81472,#81473),(#81474,#81475),(#81476,#81477),(#81478,#81479),(#81480,
#81481),(#81482,#81483),(#81484,#81485),(#81486,#81487),(#81488,#81489),
(#81490,#81491),(#81492,#81493),(#81494,#81495),(#81496,#81497),(#81498,
#81499),(#81500,#81501),(#81502,#81503),(#81504,#81505),(#81506,#81507),
(#81508,#81509),(#81510,#81511),(#81512,#81513),(#81514,#81515),(#81516,
#81517),(#81518,#81519),(#81520,#81521),(#81522,#81523),(#81524,#81525),
(#81526,#81527),(#81528,#81529),(#81530,#81531),(#81532,#81533),(#81534,
#81535),(#81536,#81537),(#81538,#81539),(#81540,#81541),(#81542,#81543),
(#81544,#81545),(#81546,#81547),(#81548,#81549),(#81550,#81551),(#81552,
#81553),(#81554,#81555),(#81556,#81557),(#81558,#81559),(#81560,#81561),
(#81562,#81563),(#81564,#81565),(#81566,#81567),(#81568,#81569),(#81570,
#81571),(#81572,#81573),(#81574,#81575),(#81576,#81577),(#81578,#81579),
(#81580,#81581),(#81582,#81583),(#81584,#81585),(#81586,#81587),(#81588,
#81589),(#81590,#81591),(#81592,#81593),(#81594,#81595),(#81596,#81597),
(#81598,#81599),(#81600,#81601),(#81602,#81603),(#81604,#81605),(#81606,
#81607),(#81608,#81609),(#81610,#81611),(#81612,#81613),(#81614,#81615),
(#81616,#81617),(#81618,#81619),(#81620,#81621),(#81622,#81623),(#81624,
#81625),(#81626,#81627),(#81628,#81629),(#81630,#81631),(#81632,#81633),
(#81634,#81635),(#81636,#81637),(#81638,#81639),(#81640,#81641),(#81642,
#81643),(#81644,#81645),(#81646,#81647),(#81648,#81649),(#81650,#81651),
(#81652,#81653),(#81654,#81655),(#81656,#81657),(#81658,#81659),(#81660,
#81661),(#81662,#81663),(#81664,#81665),(#81666,#81667),(#81668,#81669),
(#81670,#81671),(#81672,#81673),(#81674,#81675),(#81676,#81677),(#81678,
#81679),(#81680,#81681),(#81682,#81683),(#81684,#81685),(#81686,#81687),
(#81688,#81689),(#81690,#81691),(#81692,#81693),(#81694,#81695),(#81696,
#81697),(#81698,#81699),(#81700,#81701),(#81702,#81703)),.UNSPECIFIED.,
 .F.,.F.,.F.)
B_SPLINE_SURFACE_WITH_KNOTS((6,1,1,1,1,1,1,1,1,1,1,1,1,1,1,1,1,1,1,1,1,
1,1,1,1,1,1,1,1,1,1,1,1,1,1,1,1,1,1,1,1,1,1,1,1,1,1,1,1,1,1,1,1,1,1,1,1,
1,1,1,1,1,1,1,1,1,1,1,1,1,1,1,1,1,1,1,1,1,1,1,1,1,1,1,1,1,1,1,1,1,1,1,1,
1,1,1,1,1,1,1,1,1,1,1,1,1,1,1,1,1,1,1,1,1,1,1,1,1,1,1,1,1,1,1,1,1,1,1,1,
1,1,1,1,1,1,1,1,1,1,1,1,1,1,1,1,1,1,1,1,1,1,1,1,1,1,1,1,1,1,1,1,1,1,1,1,
1,1,1,1,1,1,1,1,1,1,1,1,1,1,1,1,1,1,1,1,1,1,1,1,1,1,1,1,1,1,1,1,1,1,1,6),
(2,2),(0.,0.005,0.01,0.015,0.02,0.025,0.03,0.035,0.04,0.045,0.05,0.055,
0.06,0.065,0.07,0.075,0.08,0.085,0.09,0.095,0.1,0.105,0.11,0.115,0.12,0.125,
0.13,0.135,0.14,0.145,0.15,0.155,0.16,0.165,0.17,0.175,0.18,0.185,0.19,
0.195,0.2,0.205,0.21,0.215,0.22,0.225,0.23,0.235,0.24,0.245,0.25,0.255,
0.26,0.265,0.27,0.275,0.28,0.285,0.29,0.295,0.3,0.305,0.31,0.315,0.32,0.325,
0.33,0.335,0.34,0.345,0.35,0.355,0.36,0.365,0.37,0.375,0.38,0.385,0.39,
0.395,0.4,0.405,0.41,0.415,0.42,0.425,0.43,0.435,0.44,0.445,0.45,0.455,
0.46,0.465,0.47,0.475,0.48,0.485,0.49,0.495,0.5,0.505,0.51,0.515,0.52,0.525,
0.53,0.535,0.54,0.545,0.55,0.555,0.56,0.565,0.57,0.575,0.58,0.585,0.59,
0.595,0.6,0.605,0.61,0.615,0.62,0.625,0.63,0.635,0.64,0.645,0.65,0.655,
0.66,0.665,0.67,0.675,0.68,0.685,0.690000000000001,0.695000000000001,0.700000000000001,
0.705000000000001,0.710000000000001,0.715000000000001,0.720000000000001,
0.725000000000001,0.730000000000001,0.735000000000001,0.740000000000001,
0.745000000000001,0.750000000000001,0.755000000000001,0.760000000000001,
0.765000000000001,0.770000000000001,0.775000000000001,0.780000000000001,
0.785000000000001,0.790000000000001,0.795000000000001,0.800000000000001,
0.805000000000001,0.810000000000001,0.815000000000001,0.820000000000001,
0.825000000000001,0.830000000000001,0.835000000000001,0.840000000000001,
0.845000000000001,0.850000000000001,0.855000000000001,0.860000000000001,
0.865000000000001,0.870000000000001,0.875000000000001,0.880000000000001,
0.885000000000001,0.890000000000001,0.895000000000001,0.900000000000001,
0.905000000000001,0.910000000000001,0.915000000000001,0.920000000000001,
0.925000000000001,0.930000000000001,0.935000000000001,0.940000000000001,
0.945000000000001,0.950000000000001,0.955000000000001,0.960000000000001,
0.965000000000001,0.970000000000001,0.975000000000001,0.980000000000001,
0.985000000000001,0.990000000000001,0.995000000000001,1.),(0.,1.2),
 .UNSPECIFIED.)
GEOMETRIC_REPRESENTATION_ITEM()
RATIONAL_B_SPLINE_SURFACE(((1.,1.),(1.,1.),(1.,1.),(1.,1.),(1.,1.),(1.,
1.),(1.,1.),(1.,1.),(1.,1.),(1.,1.),(1.,1.),(1.,1.),(1.,1.),(1.,1.),(1.,
1.),(1.,1.),(1.,1.),(1.,1.),(1.,1.),(1.,1.),(1.,1.),(1.,1.),(1.,1.),(1.,
1.),(1.,1.),(1.,1.),(1.,1.),(1.,1.),(1.,1.),(1.,1.),(1.,1.),(1.,1.),(1.,
1.),(1.,1.),(1.,1.),(1.,1.),(1.,1.),(1.,1.),(1.,1.),(1.,1.),(1.,1.),(1.,
1.),(1.,1.),(1.,1.),(1.,1.),(1.,1.),(1.,1.),(1.,1.),(1.,1.),(1.,1.),(1.,
1.),(1.,1.),(1.,1.),(1.,1.),(1.,1.),(1.,1.),(1.,1.),(1.,1.),(1.,1.),(1.,
1.),(1.,1.),(1.,1.),(1.,1.),(1.,1.),(1.,1.),(1.,1.),(1.,1.),(1.,1.),(1.,
1.),(1.,1.),(1.,1.),(1.,1.),(1.,1.),(1.,1.),(1.,1.),(1.,1.),(1.,1.),(1.,
1.),(1.,1.),(1.,1.),(1.,1.),(1.,1.),(1.,1.),(1.,1.),(1.,1.),(1.,1.),(1.,
1.),(1.,1.),(1.,1.),(1.,1.),(1.,1.),(1.,1.),(1.,1.),(1.,1.),(1.,1.),(1.,
1.),(1.,1.),(1.,1.),(1.,1.),(1.,1.),(1.,1.),(1.,1.),(1.,1.),(1.,1.),(1.,
1.),(1.,1.),(1.,1.),(1.,1.),(1.,1.),(1.,1.),(1.,1.),(1.,1.),(1.,1.),(1.,
1.),(1.,1.),(1.,1.),(1.,1.),(1.,1.),(1.,1.),(1.,1.),(1.,1.),(1.,1.),(1.,
1.),(1.,1.),(1.,1.),(1.,1.),(1.,1.),(1.,1.),(1.,1.),(1.,1.),(1.,1.),(1.,
1.),(1.,1.),(1.,1.),(1.,1.),(1.,1.),(1.,1.),(1.,1.),(1.,1.),(1.,1.),(1.,
1.),(1.,1.),(1.,1.),(1.,1.),(1.,1.),(1.,1.),(1.,1.),(1.,1.),(1.,1.),(1.,
1.),(1.,1.),(1.,1.),(1.,1.),(1.,1.),(1.,1.),(1.,1.),(1.,1.),(1.,1.),(1.,
1.),(1.,1.),(1.,1.),(1.,1.),(1.,1.),(1.,1.),(1.,1.),(1.,1.),(1.,1.),(1.,
1.),(1.,1.),(1.,1.),(1.,1.),(1.,1.),(1.,1.),(1.,1.),(1.,1.),(1.,1.),(1.,
1.),(1.,1.),(1.,1.),(1.,1.),(1.,1.),(1.,1.),(1.,1.),(1.,1.),(1.,1.),(1.,
1.),(1.,1.),(1.,1.),(1.,1.),(1.,1.),(1.,1.),(1.,1.),(1.,1.),(1.,1.),(1.,
1.),(1.,1.),(1.,1.),(1.,1.),(1.,1.),(1.,1.),(1.,1.),(1.,1.),(1.,1.),(1.,
1.),(1.,1.)))
REPRESENTATION_ITEM('')
SURFACE()
);
#916=(
BOUNDED_SURFACE()
B_SPLINE_SURFACE(5,1,((#82190,#82191),(#82192,#82193),(#82194,#82195),(#82196,
#82197),(#82198,#82199),(#82200,#82201),(#82202,#82203),(#82204,#82205),
(#82206,#82207),(#82208,#82209),(#82210,#82211),(#82212,#82213),(#82214,
#82215),(#82216,#82217),(#82218,#82219),(#82220,#82221),(#82222,#82223),
(#82224,#82225),(#82226,#82227),(#82228,#82229),(#82230,#82231),(#82232,
#82233),(#82234,#82235),(#82236,#82237),(#82238,#82239),(#82240,#82241),
(#82242,#82243),(#82244,#82245),(#82246,#82247),(#82248,#82249),(#82250,
#82251),(#82252,#82253),(#82254,#82255),(#82256,#82257),(#82258,#82259),
(#82260,#82261),(#82262,#82263),(#82264,#82265),(#82266,#82267),(#82268,
#82269),(#82270,#82271),(#82272,#82273),(#82274,#82275),(#82276,#82277),
(#82278,#82279),(#82280,#82281),(#82282,#82283),(#82284,#82285),(#82286,
#82287),(#82288,#82289),(#82290,#82291),(#82292,#82293),(#82294,#82295),
(#82296,#82297),(#82298,#82299),(#82300,#82301),(#82302,#82303),(#82304,
#82305),(#82306,#82307),(#82308,#82309),(#82310,#82311),(#82312,#82313),
(#82314,#82315),(#82316,#82317),(#82318,#82319),(#82320,#82321),(#82322,
#82323),(#82324,#82325),(#82326,#82327),(#82328,#82329),(#82330,#82331),
(#82332,#82333),(#82334,#82335),(#82336,#82337),(#82338,#82339),(#82340,
#82341),(#82342,#82343),(#82344,#82345),(#82346,#82347),(#82348,#82349),
(#82350,#82351),(#82352,#82353),(#82354,#82355),(#82356,#82357),(#82358,
#82359),(#82360,#82361),(#82362,#82363),(#82364,#82365),(#82366,#82367),
(#82368,#82369),(#82370,#82371),(#82372,#82373),(#82374,#82375),(#82376,
#82377),(#82378,#82379),(#82380,#82381),(#82382,#82383),(#82384,#82385),
(#82386,#82387),(#82388,#82389),(#82390,#82391),(#82392,#82393),(#82394,
#82395),(#82396,#82397),(#82398,#82399),(#82400,#82401),(#82402,#82403),
(#82404,#82405),(#82406,#82407),(#82408,#82409),(#82410,#82411),(#82412,
#82413),(#82414,#82415),(#82416,#82417),(#82418,#82419),(#82420,#82421),
(#82422,#82423),(#82424,#82425),(#82426,#82427),(#82428,#82429),(#82430,
#82431),(#82432,#82433),(#82434,#82435),(#82436,#82437),(#82438,#82439),
(#82440,#82441),(#82442,#82443),(#82444,#82445),(#82446,#82447),(#82448,
#82449),(#82450,#82451),(#82452,#82453),(#82454,#82455),(#82456,#82457),
(#82458,#82459),(#82460,#82461),(#82462,#82463),(#82464,#82465),(#82466,
#82467),(#82468,#82469),(#82470,#82471),(#82472,#82473),(#82474,#82475),
(#82476,#82477),(#82478,#82479),(#82480,#82481),(#82482,#82483),(#82484,
#82485),(#82486,#82487),(#82488,#82489),(#82490,#82491),(#82492,#82493),
(#82494,#82495),(#82496,#82497),(#82498,#82499),(#82500,#82501),(#82502,
#82503),(#82504,#82505),(#82506,#82507),(#82508,#82509),(#82510,#82511),
(#82512,#82513),(#82514,#82515),(#82516,#82517),(#82518,#82519),(#82520,
#82521),(#82522,#82523),(#82524,#82525),(#82526,#82527),(#82528,#82529),
(#82530,#82531),(#82532,#82533),(#82534,#82535),(#82536,#82537),(#82538,
#82539),(#82540,#82541),(#82542,#82543),(#82544,#82545),(#82546,#82547),
(#82548,#82549),(#82550,#82551),(#82552,#82553),(#82554,#82555),(#82556,
#82557),(#82558,#82559),(#82560,#82561),(#82562,#82563),(#82564,#82565),
(#82566,#82567),(#82568,#82569),(#82570,#82571),(#82572,#82573),(#82574,
#82575),(#82576,#82577),(#82578,#82579),(#82580,#82581),(#82582,#82583),
(#82584,#82585),(#82586,#82587),(#82588,#82589),(#82590,#82591),(#82592,
#82593),(#82594,#82595),(#82596,#82597),(#82598,#82599)),.UNSPECIFIED.,
 .F.,.F.,.F.)
B_SPLINE_SURFACE_WITH_KNOTS((6,1,1,1,1,1,1,1,1,1,1,1,1,1,1,1,1,1,1,1,1,
1,1,1,1,1,1,1,1,1,1,1,1,1,1,1,1,1,1,1,1,1,1,1,1,1,1,1,1,1,1,1,1,1,1,1,1,
1,1,1,1,1,1,1,1,1,1,1,1,1,1,1,1,1,1,1,1,1,1,1,1,1,1,1,1,1,1,1,1,1,1,1,1,
1,1,1,1,1,1,1,1,1,1,1,1,1,1,1,1,1,1,1,1,1,1,1,1,1,1,1,1,1,1,1,1,1,1,1,1,
1,1,1,1,1,1,1,1,1,1,1,1,1,1,1,1,1,1,1,1,1,1,1,1,1,1,1,1,1,1,1,1,1,1,1,1,
1,1,1,1,1,1,1,1,1,1,1,1,1,1,1,1,1,1,1,1,1,1,1,1,1,1,1,1,1,1,1,1,1,1,1,6),
(2,2),(0.,0.005,0.01,0.015,0.02,0.025,0.03,0.035,0.04,0.045,0.05,0.055,
0.06,0.065,0.07,0.075,0.08,0.085,0.09,0.095,0.1,0.105,0.11,0.115,0.12,0.125,
0.13,0.135,0.14,0.145,0.15,0.155,0.16,0.165,0.17,0.175,0.18,0.185,0.19,
0.195,0.2,0.205,0.21,0.215,0.22,0.225,0.23,0.235,0.24,0.245,0.25,0.255,
0.26,0.265,0.27,0.275,0.28,0.285,0.29,0.295,0.3,0.305,0.31,0.315,0.32,0.325,
0.33,0.335,0.34,0.345,0.35,0.355,0.36,0.365,0.37,0.375,0.38,0.385,0.39,
0.395,0.4,0.405,0.41,0.415,0.42,0.425,0.43,0.435,0.44,0.445,0.45,0.455,
0.46,0.465,0.47,0.475,0.48,0.485,0.49,0.495,0.5,0.505,0.51,0.515,0.52,0.525,
0.53,0.535,0.54,0.545,0.55,0.555,0.56,0.565,0.57,0.575,0.58,0.585,0.59,
0.595,0.6,0.605,0.61,0.615,0.62,0.625,0.63,0.635,0.64,0.645,0.65,0.655,
0.66,0.665,0.67,0.675,0.68,0.685,0.690000000000001,0.695000000000001,0.700000000000001,
0.705000000000001,0.710000000000001,0.715000000000001,0.720000000000001,
0.725000000000001,0.730000000000001,0.735000000000001,0.740000000000001,
0.745000000000001,0.750000000000001,0.755000000000001,0.760000000000001,
0.765000000000001,0.770000000000001,0.775000000000001,0.780000000000001,
0.785000000000001,0.790000000000001,0.795000000000001,0.800000000000001,
0.805000000000001,0.810000000000001,0.815000000000001,0.820000000000001,
0.825000000000001,0.830000000000001,0.835000000000001,0.840000000000001,
0.845000000000001,0.850000000000001,0.855000000000001,0.860000000000001,
0.865000000000001,0.870000000000001,0.875000000000001,0.880000000000001,
0.885000000000001,0.890000000000001,0.895000000000001,0.900000000000001,
0.905000000000001,0.910000000000001,0.915000000000001,0.920000000000001,
0.925000000000001,0.930000000000001,0.935000000000001,0.940000000000001,
0.945000000000001,0.950000000000001,0.955000000000001,0.960000000000001,
0.965000000000001,0.970000000000001,0.975000000000001,0.980000000000001,
0.985000000000001,0.990000000000001,0.995000000000001,1.),(0.,1.2),
 .UNSPECIFIED.)
GEOMETRIC_REPRESENTATION_ITEM()
RATIONAL_B_SPLINE_SURFACE(((1.,1.),(1.,1.),(1.,1.),(1.,1.),(1.,1.),(1.,
1.),(1.,1.),(1.,1.),(1.,1.),(1.,1.),(1.,1.),(1.,1.),(1.,1.),(1.,1.),(1.,
1.),(1.,1.),(1.,1.),(1.,1.),(1.,1.),(1.,1.),(1.,1.),(1.,1.),(1.,1.),(1.,
1.),(1.,1.),(1.,1.),(1.,1.),(1.,1.),(1.,1.),(1.,1.),(1.,1.),(1.,1.),(1.,
1.),(1.,1.),(1.,1.),(1.,1.),(1.,1.),(1.,1.),(1.,1.),(1.,1.),(1.,1.),(1.,
1.),(1.,1.),(1.,1.),(1.,1.),(1.,1.),(1.,1.),(1.,1.),(1.,1.),(1.,1.),(1.,
1.),(1.,1.),(1.,1.),(1.,1.),(1.,1.),(1.,1.),(1.,1.),(1.,1.),(1.,1.),(1.,
1.),(1.,1.),(1.,1.),(1.,1.),(1.,1.),(1.,1.),(1.,1.),(1.,1.),(1.,1.),(1.,
1.),(1.,1.),(1.,1.),(1.,1.),(1.,1.),(1.,1.),(1.,1.),(1.,1.),(1.,1.),(1.,
1.),(1.,1.),(1.,1.),(1.,1.),(1.,1.),(1.,1.),(1.,1.),(1.,1.),(1.,1.),(1.,
1.),(1.,1.),(1.,1.),(1.,1.),(1.,1.),(1.,1.),(1.,1.),(1.,1.),(1.,1.),(1.,
1.),(1.,1.),(1.,1.),(1.,1.),(1.,1.),(1.,1.),(1.,1.),(1.,1.),(1.,1.),(1.,
1.),(1.,1.),(1.,1.),(1.,1.),(1.,1.),(1.,1.),(1.,1.),(1.,1.),(1.,1.),(1.,
1.),(1.,1.),(1.,1.),(1.,1.),(1.,1.),(1.,1.),(1.,1.),(1.,1.),(1.,1.),(1.,
1.),(1.,1.),(1.,1.),(1.,1.),(1.,1.),(1.,1.),(1.,1.),(1.,1.),(1.,1.),(1.,
1.),(1.,1.),(1.,1.),(1.,1.),(1.,1.),(1.,1.),(1.,1.),(1.,1.),(1.,1.),(1.,
1.),(1.,1.),(1.,1.),(1.,1.),(1.,1.),(1.,1.),(1.,1.),(1.,1.),(1.,1.),(1.,
1.),(1.,1.),(1.,1.),(1.,1.),(1.,1.),(1.,1.),(1.,1.),(1.,1.),(1.,1.),(1.,
1.),(1.,1.),(1.,1.),(1.,1.),(1.,1.),(1.,1.),(1.,1.),(1.,1.),(1.,1.),(1.,
1.),(1.,1.),(1.,1.),(1.,1.),(1.,1.),(1.,1.),(1.,1.),(1.,1.),(1.,1.),(1.,
1.),(1.,1.),(1.,1.),(1.,1.),(1.,1.),(1.,1.),(1.,1.),(1.,1.),(1.,1.),(1.,
1.),(1.,1.),(1.,1.),(1.,1.),(1.,1.),(1.,1.),(1.,1.),(1.,1.),(1.,1.),(1.,
1.),(1.,1.),(1.,1.),(1.,1.),(1.,1.),(1.,1.),(1.,1.),(1.,1.),(1.,1.),(1.,
1.),(1.,1.)))
REPRESENTATION_ITEM('')
SURFACE()
);
#917=(
BOUNDED_SURFACE()
B_SPLINE_SURFACE(5,1,((#83086,#83087),(#83088,#83089),(#83090,#83091),(#83092,
#83093),(#83094,#83095),(#83096,#83097),(#83098,#83099),(#83100,#83101),
(#83102,#83103),(#83104,#83105),(#83106,#83107),(#83108,#83109),(#83110,
#83111),(#83112,#83113),(#83114,#83115),(#83116,#83117),(#83118,#83119),
(#83120,#83121),(#83122,#83123),(#83124,#83125),(#83126,#83127),(#83128,
#83129),(#83130,#83131),(#83132,#83133),(#83134,#83135),(#83136,#83137),
(#83138,#83139),(#83140,#83141),(#83142,#83143),(#83144,#83145),(#83146,
#83147),(#83148,#83149),(#83150,#83151),(#83152,#83153),(#83154,#83155),
(#83156,#83157),(#83158,#83159),(#83160,#83161),(#83162,#83163),(#83164,
#83165),(#83166,#83167),(#83168,#83169),(#83170,#83171),(#83172,#83173),
(#83174,#83175),(#83176,#83177),(#83178,#83179),(#83180,#83181),(#83182,
#83183),(#83184,#83185),(#83186,#83187),(#83188,#83189),(#83190,#83191),
(#83192,#83193),(#83194,#83195),(#83196,#83197),(#83198,#83199),(#83200,
#83201),(#83202,#83203),(#83204,#83205),(#83206,#83207),(#83208,#83209),
(#83210,#83211),(#83212,#83213),(#83214,#83215),(#83216,#83217),(#83218,
#83219),(#83220,#83221),(#83222,#83223),(#83224,#83225),(#83226,#83227),
(#83228,#83229),(#83230,#83231),(#83232,#83233),(#83234,#83235),(#83236,
#83237),(#83238,#83239),(#83240,#83241),(#83242,#83243),(#83244,#83245),
(#83246,#83247),(#83248,#83249),(#83250,#83251),(#83252,#83253),(#83254,
#83255),(#83256,#83257),(#83258,#83259),(#83260,#83261),(#83262,#83263),
(#83264,#83265),(#83266,#83267),(#83268,#83269),(#83270,#83271),(#83272,
#83273),(#83274,#83275),(#83276,#83277),(#83278,#83279),(#83280,#83281),
(#83282,#83283),(#83284,#83285),(#83286,#83287),(#83288,#83289),(#83290,
#83291),(#83292,#83293),(#83294,#83295),(#83296,#83297),(#83298,#83299),
(#83300,#83301),(#83302,#83303),(#83304,#83305),(#83306,#83307),(#83308,
#83309),(#83310,#83311),(#83312,#83313),(#83314,#83315),(#83316,#83317),
(#83318,#83319),(#83320,#83321),(#83322,#83323),(#83324,#83325),(#83326,
#83327),(#83328,#83329),(#83330,#83331),(#83332,#83333),(#83334,#83335),
(#83336,#83337),(#83338,#83339),(#83340,#83341),(#83342,#83343),(#83344,
#83345),(#83346,#83347),(#83348,#83349),(#83350,#83351),(#83352,#83353),
(#83354,#83355),(#83356,#83357),(#83358,#83359),(#83360,#83361),(#83362,
#83363),(#83364,#83365),(#83366,#83367),(#83368,#83369),(#83370,#83371),
(#83372,#83373),(#83374,#83375),(#83376,#83377),(#83378,#83379),(#83380,
#83381),(#83382,#83383),(#83384,#83385),(#83386,#83387),(#83388,#83389),
(#83390,#83391),(#83392,#83393),(#83394,#83395),(#83396,#83397),(#83398,
#83399),(#83400,#83401),(#83402,#83403),(#83404,#83405),(#83406,#83407),
(#83408,#83409),(#83410,#83411),(#83412,#83413),(#83414,#83415),(#83416,
#83417),(#83418,#83419),(#83420,#83421),(#83422,#83423),(#83424,#83425),
(#83426,#83427),(#83428,#83429),(#83430,#83431),(#83432,#83433),(#83434,
#83435),(#83436,#83437),(#83438,#83439),(#83440,#83441),(#83442,#83443),
(#83444,#83445),(#83446,#83447),(#83448,#83449),(#83450,#83451),(#83452,
#83453),(#83454,#83455),(#83456,#83457),(#83458,#83459),(#83460,#83461),
(#83462,#83463),(#83464,#83465),(#83466,#83467),(#83468,#83469),(#83470,
#83471),(#83472,#83473),(#83474,#83475),(#83476,#83477),(#83478,#83479),
(#83480,#83481),(#83482,#83483),(#83484,#83485),(#83486,#83487),(#83488,
#83489),(#83490,#83491),(#83492,#83493),(#83494,#83495)),.UNSPECIFIED.,
 .F.,.F.,.F.)
B_SPLINE_SURFACE_WITH_KNOTS((6,1,1,1,1,1,1,1,1,1,1,1,1,1,1,1,1,1,1,1,1,
1,1,1,1,1,1,1,1,1,1,1,1,1,1,1,1,1,1,1,1,1,1,1,1,1,1,1,1,1,1,1,1,1,1,1,1,
1,1,1,1,1,1,1,1,1,1,1,1,1,1,1,1,1,1,1,1,1,1,1,1,1,1,1,1,1,1,1,1,1,1,1,1,
1,1,1,1,1,1,1,1,1,1,1,1,1,1,1,1,1,1,1,1,1,1,1,1,1,1,1,1,1,1,1,1,1,1,1,1,
1,1,1,1,1,1,1,1,1,1,1,1,1,1,1,1,1,1,1,1,1,1,1,1,1,1,1,1,1,1,1,1,1,1,1,1,
1,1,1,1,1,1,1,1,1,1,1,1,1,1,1,1,1,1,1,1,1,1,1,1,1,1,1,1,1,1,1,1,1,1,1,6),
(2,2),(0.,0.005,0.01,0.015,0.02,0.025,0.03,0.035,0.04,0.045,0.05,0.055,
0.06,0.065,0.07,0.075,0.08,0.085,0.09,0.095,0.1,0.105,0.11,0.115,0.12,0.125,
0.13,0.135,0.14,0.145,0.15,0.155,0.16,0.165,0.17,0.175,0.18,0.185,0.19,
0.195,0.2,0.205,0.21,0.215,0.22,0.225,0.23,0.235,0.24,0.245,0.25,0.255,
0.26,0.265,0.27,0.275,0.28,0.285,0.29,0.295,0.3,0.305,0.31,0.315,0.32,0.325,
0.33,0.335,0.34,0.345,0.35,0.355,0.36,0.365,0.37,0.375,0.38,0.385,0.39,
0.395,0.4,0.405,0.41,0.415,0.42,0.425,0.43,0.435,0.44,0.445,0.45,0.455,
0.46,0.465,0.47,0.475,0.48,0.485,0.49,0.495,0.5,0.505,0.51,0.515,0.52,0.525,
0.53,0.535,0.54,0.545,0.55,0.555,0.56,0.565,0.57,0.575,0.58,0.585,0.59,
0.595,0.6,0.605,0.61,0.615,0.62,0.625,0.63,0.635,0.64,0.645,0.65,0.655,
0.66,0.665,0.67,0.675,0.68,0.685,0.690000000000001,0.695000000000001,0.700000000000001,
0.705000000000001,0.710000000000001,0.715000000000001,0.720000000000001,
0.725000000000001,0.730000000000001,0.735000000000001,0.740000000000001,
0.745000000000001,0.750000000000001,0.755000000000001,0.760000000000001,
0.765000000000001,0.770000000000001,0.775000000000001,0.780000000000001,
0.785000000000001,0.790000000000001,0.795000000000001,0.800000000000001,
0.805000000000001,0.810000000000001,0.815000000000001,0.820000000000001,
0.825000000000001,0.830000000000001,0.835000000000001,0.840000000000001,
0.845000000000001,0.850000000000001,0.855000000000001,0.860000000000001,
0.865000000000001,0.870000000000001,0.875000000000001,0.880000000000001,
0.885000000000001,0.890000000000001,0.895000000000001,0.900000000000001,
0.905000000000001,0.910000000000001,0.915000000000001,0.920000000000001,
0.925000000000001,0.930000000000001,0.935000000000001,0.940000000000001,
0.945000000000001,0.950000000000001,0.955000000000001,0.960000000000001,
0.965000000000001,0.970000000000001,0.975000000000001,0.980000000000001,
0.985000000000001,0.990000000000001,0.995000000000001,1.),(0.,1.2),
 .UNSPECIFIED.)
GEOMETRIC_REPRESENTATION_ITEM()
RATIONAL_B_SPLINE_SURFACE(((1.,1.),(1.,1.),(1.,1.),(1.,1.),(1.,1.),(1.,
1.),(1.,1.),(1.,1.),(1.,1.),(1.,1.),(1.,1.),(1.,1.),(1.,1.),(1.,1.),(1.,
1.),(1.,1.),(1.,1.),(1.,1.),(1.,1.),(1.,1.),(1.,1.),(1.,1.),(1.,1.),(1.,
1.),(1.,1.),(1.,1.),(1.,1.),(1.,1.),(1.,1.),(1.,1.),(1.,1.),(1.,1.),(1.,
1.),(1.,1.),(1.,1.),(1.,1.),(1.,1.),(1.,1.),(1.,1.),(1.,1.),(1.,1.),(1.,
1.),(1.,1.),(1.,1.),(1.,1.),(1.,1.),(1.,1.),(1.,1.),(1.,1.),(1.,1.),(1.,
1.),(1.,1.),(1.,1.),(1.,1.),(1.,1.),(1.,1.),(1.,1.),(1.,1.),(1.,1.),(1.,
1.),(1.,1.),(1.,1.),(1.,1.),(1.,1.),(1.,1.),(1.,1.),(1.,1.),(1.,1.),(1.,
1.),(1.,1.),(1.,1.),(1.,1.),(1.,1.),(1.,1.),(1.,1.),(1.,1.),(1.,1.),(1.,
1.),(1.,1.),(1.,1.),(1.,1.),(1.,1.),(1.,1.),(1.,1.),(1.,1.),(1.,1.),(1.,
1.),(1.,1.),(1.,1.),(1.,1.),(1.,1.),(1.,1.),(1.,1.),(1.,1.),(1.,1.),(1.,
1.),(1.,1.),(1.,1.),(1.,1.),(1.,1.),(1.,1.),(1.,1.),(1.,1.),(1.,1.),(1.,
1.),(1.,1.),(1.,1.),(1.,1.),(1.,1.),(1.,1.),(1.,1.),(1.,1.),(1.,1.),(1.,
1.),(1.,1.),(1.,1.),(1.,1.),(1.,1.),(1.,1.),(1.,1.),(1.,1.),(1.,1.),(1.,
1.),(1.,1.),(1.,1.),(1.,1.),(1.,1.),(1.,1.),(1.,1.),(1.,1.),(1.,1.),(1.,
1.),(1.,1.),(1.,1.),(1.,1.),(1.,1.),(1.,1.),(1.,1.),(1.,1.),(1.,1.),(1.,
1.),(1.,1.),(1.,1.),(1.,1.),(1.,1.),(1.,1.),(1.,1.),(1.,1.),(1.,1.),(1.,
1.),(1.,1.),(1.,1.),(1.,1.),(1.,1.),(1.,1.),(1.,1.),(1.,1.),(1.,1.),(1.,
1.),(1.,1.),(1.,1.),(1.,1.),(1.,1.),(1.,1.),(1.,1.),(1.,1.),(1.,1.),(1.,
1.),(1.,1.),(1.,1.),(1.,1.),(1.,1.),(1.,1.),(1.,1.),(1.,1.),(1.,1.),(1.,
1.),(1.,1.),(1.,1.),(1.,1.),(1.,1.),(1.,1.),(1.,1.),(1.,1.),(1.,1.),(1.,
1.),(1.,1.),(1.,1.),(1.,1.),(1.,1.),(1.,1.),(1.,1.),(1.,1.),(1.,1.),(1.,
1.),(1.,1.),(1.,1.),(1.,1.),(1.,1.),(1.,1.),(1.,1.),(1.,1.),(1.,1.),(1.,
1.),(1.,1.)))
REPRESENTATION_ITEM('')
SURFACE()
);
#918=(
BOUNDED_SURFACE()
B_SPLINE_SURFACE(5,1,((#83982,#83983),(#83984,#83985),(#83986,#83987),(#83988,
#83989),(#83990,#83991),(#83992,#83993),(#83994,#83995),(#83996,#83997),
(#83998,#83999),(#84000,#84001),(#84002,#84003),(#84004,#84005),(#84006,
#84007),(#84008,#84009),(#84010,#84011),(#84012,#84013),(#84014,#84015),
(#84016,#84017),(#84018,#84019),(#84020,#84021),(#84022,#84023),(#84024,
#84025),(#84026,#84027),(#84028,#84029),(#84030,#84031),(#84032,#84033),
(#84034,#84035),(#84036,#84037),(#84038,#84039),(#84040,#84041),(#84042,
#84043),(#84044,#84045),(#84046,#84047),(#84048,#84049),(#84050,#84051),
(#84052,#84053),(#84054,#84055),(#84056,#84057),(#84058,#84059),(#84060,
#84061),(#84062,#84063),(#84064,#84065),(#84066,#84067),(#84068,#84069),
(#84070,#84071),(#84072,#84073),(#84074,#84075),(#84076,#84077),(#84078,
#84079),(#84080,#84081),(#84082,#84083),(#84084,#84085),(#84086,#84087),
(#84088,#84089),(#84090,#84091),(#84092,#84093),(#84094,#84095),(#84096,
#84097),(#84098,#84099),(#84100,#84101),(#84102,#84103),(#84104,#84105),
(#84106,#84107),(#84108,#84109),(#84110,#84111),(#84112,#84113),(#84114,
#84115),(#84116,#84117),(#84118,#84119),(#84120,#84121),(#84122,#84123),
(#84124,#84125),(#84126,#84127),(#84128,#84129),(#84130,#84131),(#84132,
#84133),(#84134,#84135),(#84136,#84137),(#84138,#84139),(#84140,#84141),
(#84142,#84143),(#84144,#84145),(#84146,#84147),(#84148,#84149),(#84150,
#84151),(#84152,#84153),(#84154,#84155),(#84156,#84157),(#84158,#84159),
(#84160,#84161),(#84162,#84163),(#84164,#84165),(#84166,#84167),(#84168,
#84169),(#84170,#84171),(#84172,#84173),(#84174,#84175),(#84176,#84177),
(#84178,#84179),(#84180,#84181),(#84182,#84183),(#84184,#84185),(#84186,
#84187),(#84188,#84189),(#84190,#84191),(#84192,#84193),(#84194,#84195),
(#84196,#84197),(#84198,#84199),(#84200,#84201),(#84202,#84203),(#84204,
#84205),(#84206,#84207),(#84208,#84209),(#84210,#84211),(#84212,#84213),
(#84214,#84215),(#84216,#84217),(#84218,#84219),(#84220,#84221),(#84222,
#84223),(#84224,#84225),(#84226,#84227),(#84228,#84229),(#84230,#84231),
(#84232,#84233),(#84234,#84235),(#84236,#84237),(#84238,#84239),(#84240,
#84241),(#84242,#84243),(#84244,#84245),(#84246,#84247),(#84248,#84249),
(#84250,#84251),(#84252,#84253),(#84254,#84255),(#84256,#84257),(#84258,
#84259),(#84260,#84261),(#84262,#84263),(#84264,#84265),(#84266,#84267),
(#84268,#84269),(#84270,#84271),(#84272,#84273),(#84274,#84275),(#84276,
#84277),(#84278,#84279),(#84280,#84281),(#84282,#84283),(#84284,#84285),
(#84286,#84287),(#84288,#84289),(#84290,#84291),(#84292,#84293),(#84294,
#84295),(#84296,#84297),(#84298,#84299),(#84300,#84301),(#84302,#84303),
(#84304,#84305),(#84306,#84307),(#84308,#84309),(#84310,#84311),(#84312,
#84313),(#84314,#84315),(#84316,#84317),(#84318,#84319),(#84320,#84321),
(#84322,#84323),(#84324,#84325),(#84326,#84327),(#84328,#84329),(#84330,
#84331),(#84332,#84333),(#84334,#84335),(#84336,#84337),(#84338,#84339),
(#84340,#84341),(#84342,#84343),(#84344,#84345),(#84346,#84347),(#84348,
#84349),(#84350,#84351),(#84352,#84353),(#84354,#84355),(#84356,#84357),
(#84358,#84359),(#84360,#84361),(#84362,#84363),(#84364,#84365),(#84366,
#84367),(#84368,#84369),(#84370,#84371),(#84372,#84373),(#84374,#84375),
(#84376,#84377),(#84378,#84379),(#84380,#84381),(#84382,#84383),(#84384,
#84385),(#84386,#84387),(#84388,#84389),(#84390,#84391)),.UNSPECIFIED.,
 .F.,.F.,.F.)
B_SPLINE_SURFACE_WITH_KNOTS((6,1,1,1,1,1,1,1,1,1,1,1,1,1,1,1,1,1,1,1,1,
1,1,1,1,1,1,1,1,1,1,1,1,1,1,1,1,1,1,1,1,1,1,1,1,1,1,1,1,1,1,1,1,1,1,1,1,
1,1,1,1,1,1,1,1,1,1,1,1,1,1,1,1,1,1,1,1,1,1,1,1,1,1,1,1,1,1,1,1,1,1,1,1,
1,1,1,1,1,1,1,1,1,1,1,1,1,1,1,1,1,1,1,1,1,1,1,1,1,1,1,1,1,1,1,1,1,1,1,1,
1,1,1,1,1,1,1,1,1,1,1,1,1,1,1,1,1,1,1,1,1,1,1,1,1,1,1,1,1,1,1,1,1,1,1,1,
1,1,1,1,1,1,1,1,1,1,1,1,1,1,1,1,1,1,1,1,1,1,1,1,1,1,1,1,1,1,1,1,1,1,1,6),
(2,2),(0.,0.005,0.01,0.015,0.02,0.025,0.03,0.035,0.04,0.045,0.05,0.055,
0.06,0.065,0.07,0.075,0.08,0.085,0.09,0.095,0.1,0.105,0.11,0.115,0.12,0.125,
0.13,0.135,0.14,0.145,0.15,0.155,0.16,0.165,0.17,0.175,0.18,0.185,0.19,
0.195,0.2,0.205,0.21,0.215,0.22,0.225,0.23,0.235,0.24,0.245,0.25,0.255,
0.26,0.265,0.27,0.275,0.28,0.285,0.29,0.295,0.3,0.305,0.31,0.315,0.32,0.325,
0.33,0.335,0.34,0.345,0.35,0.355,0.36,0.365,0.37,0.375,0.38,0.385,0.39,
0.395,0.4,0.405,0.41,0.415,0.42,0.425,0.43,0.435,0.44,0.445,0.45,0.455,
0.46,0.465,0.47,0.475,0.48,0.485,0.49,0.495,0.5,0.505,0.51,0.515,0.52,0.525,
0.53,0.535,0.54,0.545,0.55,0.555,0.56,0.565,0.57,0.575,0.58,0.585,0.59,
0.595,0.6,0.605,0.61,0.615,0.62,0.625,0.63,0.635,0.64,0.645,0.65,0.655,
0.66,0.665,0.67,0.675,0.68,0.685,0.690000000000001,0.695000000000001,0.700000000000001,
0.705000000000001,0.710000000000001,0.715000000000001,0.720000000000001,
0.725000000000001,0.730000000000001,0.735000000000001,0.740000000000001,
0.745000000000001,0.750000000000001,0.755000000000001,0.760000000000001,
0.765000000000001,0.770000000000001,0.775000000000001,0.780000000000001,
0.785000000000001,0.790000000000001,0.795000000000001,0.800000000000001,
0.805000000000001,0.810000000000001,0.815000000000001,0.820000000000001,
0.825000000000001,0.830000000000001,0.835000000000001,0.840000000000001,
0.845000000000001,0.850000000000001,0.855000000000001,0.860000000000001,
0.865000000000001,0.870000000000001,0.875000000000001,0.880000000000001,
0.885000000000001,0.890000000000001,0.895000000000001,0.900000000000001,
0.905000000000001,0.910000000000001,0.915000000000001,0.920000000000001,
0.925000000000001,0.930000000000001,0.935000000000001,0.940000000000001,
0.945000000000001,0.950000000000001,0.955000000000001,0.960000000000001,
0.965000000000001,0.970000000000001,0.975000000000001,0.980000000000001,
0.985000000000001,0.990000000000001,0.995000000000001,1.),(0.,1.2),
 .UNSPECIFIED.)
GEOMETRIC_REPRESENTATION_ITEM()
RATIONAL_B_SPLINE_SURFACE(((1.,1.),(1.,1.),(1.,1.),(1.,1.),(1.,1.),(1.,
1.),(1.,1.),(1.,1.),(1.,1.),(1.,1.),(1.,1.),(1.,1.),(1.,1.),(1.,1.),(1.,
1.),(1.,1.),(1.,1.),(1.,1.),(1.,1.),(1.,1.),(1.,1.),(1.,1.),(1.,1.),(1.,
1.),(1.,1.),(1.,1.),(1.,1.),(1.,1.),(1.,1.),(1.,1.),(1.,1.),(1.,1.),(1.,
1.),(1.,1.),(1.,1.),(1.,1.),(1.,1.),(1.,1.),(1.,1.),(1.,1.),(1.,1.),(1.,
1.),(1.,1.),(1.,1.),(1.,1.),(1.,1.),(1.,1.),(1.,1.),(1.,1.),(1.,1.),(1.,
1.),(1.,1.),(1.,1.),(1.,1.),(1.,1.),(1.,1.),(1.,1.),(1.,1.),(1.,1.),(1.,
1.),(1.,1.),(1.,1.),(1.,1.),(1.,1.),(1.,1.),(1.,1.),(1.,1.),(1.,1.),(1.,
1.),(1.,1.),(1.,1.),(1.,1.),(1.,1.),(1.,1.),(1.,1.),(1.,1.),(1.,1.),(1.,
1.),(1.,1.),(1.,1.),(1.,1.),(1.,1.),(1.,1.),(1.,1.),(1.,1.),(1.,1.),(1.,
1.),(1.,1.),(1.,1.),(1.,1.),(1.,1.),(1.,1.),(1.,1.),(1.,1.),(1.,1.),(1.,
1.),(1.,1.),(1.,1.),(1.,1.),(1.,1.),(1.,1.),(1.,1.),(1.,1.),(1.,1.),(1.,
1.),(1.,1.),(1.,1.),(1.,1.),(1.,1.),(1.,1.),(1.,1.),(1.,1.),(1.,1.),(1.,
1.),(1.,1.),(1.,1.),(1.,1.),(1.,1.),(1.,1.),(1.,1.),(1.,1.),(1.,1.),(1.,
1.),(1.,1.),(1.,1.),(1.,1.),(1.,1.),(1.,1.),(1.,1.),(1.,1.),(1.,1.),(1.,
1.),(1.,1.),(1.,1.),(1.,1.),(1.,1.),(1.,1.),(1.,1.),(1.,1.),(1.,1.),(1.,
1.),(1.,1.),(1.,1.),(1.,1.),(1.,1.),(1.,1.),(1.,1.),(1.,1.),(1.,1.),(1.,
1.),(1.,1.),(1.,1.),(1.,1.),(1.,1.),(1.,1.),(1.,1.),(1.,1.),(1.,1.),(1.,
1.),(1.,1.),(1.,1.),(1.,1.),(1.,1.),(1.,1.),(1.,1.),(1.,1.),(1.,1.),(1.,
1.),(1.,1.),(1.,1.),(1.,1.),(1.,1.),(1.,1.),(1.,1.),(1.,1.),(1.,1.),(1.,
1.),(1.,1.),(1.,1.),(1.,1.),(1.,1.),(1.,1.),(1.,1.),(1.,1.),(1.,1.),(1.,
1.),(1.,1.),(1.,1.),(1.,1.),(1.,1.),(1.,1.),(1.,1.),(1.,1.),(1.,1.),(1.,
1.),(1.,1.),(1.,1.),(1.,1.),(1.,1.),(1.,1.),(1.,1.),(1.,1.),(1.,1.),(1.,
1.),(1.,1.)))
REPRESENTATION_ITEM('')
SURFACE()
);
#919=(
BOUNDED_SURFACE()
B_SPLINE_SURFACE(5,1,((#84878,#84879),(#84880,#84881),(#84882,#84883),(#84884,
#84885),(#84886,#84887),(#84888,#84889),(#84890,#84891),(#84892,#84893),
(#84894,#84895),(#84896,#84897),(#84898,#84899),(#84900,#84901),(#84902,
#84903),(#84904,#84905),(#84906,#84907),(#84908,#84909),(#84910,#84911),
(#84912,#84913),(#84914,#84915),(#84916,#84917),(#84918,#84919),(#84920,
#84921),(#84922,#84923),(#84924,#84925),(#84926,#84927),(#84928,#84929),
(#84930,#84931),(#84932,#84933),(#84934,#84935),(#84936,#84937),(#84938,
#84939),(#84940,#84941),(#84942,#84943),(#84944,#84945),(#84946,#84947),
(#84948,#84949),(#84950,#84951),(#84952,#84953),(#84954,#84955),(#84956,
#84957),(#84958,#84959),(#84960,#84961),(#84962,#84963),(#84964,#84965),
(#84966,#84967),(#84968,#84969),(#84970,#84971),(#84972,#84973),(#84974,
#84975),(#84976,#84977),(#84978,#84979),(#84980,#84981),(#84982,#84983),
(#84984,#84985),(#84986,#84987),(#84988,#84989),(#84990,#84991),(#84992,
#84993),(#84994,#84995),(#84996,#84997),(#84998,#84999),(#85000,#85001),
(#85002,#85003),(#85004,#85005),(#85006,#85007),(#85008,#85009),(#85010,
#85011),(#85012,#85013),(#85014,#85015),(#85016,#85017),(#85018,#85019),
(#85020,#85021),(#85022,#85023),(#85024,#85025),(#85026,#85027),(#85028,
#85029),(#85030,#85031),(#85032,#85033),(#85034,#85035),(#85036,#85037),
(#85038,#85039),(#85040,#85041),(#85042,#85043),(#85044,#85045),(#85046,
#85047),(#85048,#85049),(#85050,#85051),(#85052,#85053),(#85054,#85055),
(#85056,#85057),(#85058,#85059),(#85060,#85061),(#85062,#85063),(#85064,
#85065),(#85066,#85067),(#85068,#85069),(#85070,#85071),(#85072,#85073),
(#85074,#85075),(#85076,#85077),(#85078,#85079),(#85080,#85081),(#85082,
#85083),(#85084,#85085),(#85086,#85087),(#85088,#85089),(#85090,#85091),
(#85092,#85093),(#85094,#85095),(#85096,#85097),(#85098,#85099),(#85100,
#85101),(#85102,#85103),(#85104,#85105),(#85106,#85107),(#85108,#85109),
(#85110,#85111),(#85112,#85113),(#85114,#85115),(#85116,#85117),(#85118,
#85119),(#85120,#85121),(#85122,#85123),(#85124,#85125),(#85126,#85127),
(#85128,#85129),(#85130,#85131),(#85132,#85133),(#85134,#85135),(#85136,
#85137),(#85138,#85139),(#85140,#85141),(#85142,#85143),(#85144,#85145),
(#85146,#85147),(#85148,#85149),(#85150,#85151),(#85152,#85153),(#85154,
#85155),(#85156,#85157),(#85158,#85159),(#85160,#85161),(#85162,#85163),
(#85164,#85165),(#85166,#85167),(#85168,#85169),(#85170,#85171),(#85172,
#85173),(#85174,#85175),(#85176,#85177),(#85178,#85179),(#85180,#85181),
(#85182,#85183),(#85184,#85185),(#85186,#85187),(#85188,#85189),(#85190,
#85191),(#85192,#85193),(#85194,#85195),(#85196,#85197),(#85198,#85199),
(#85200,#85201),(#85202,#85203),(#85204,#85205),(#85206,#85207),(#85208,
#85209),(#85210,#85211),(#85212,#85213),(#85214,#85215),(#85216,#85217),
(#85218,#85219),(#85220,#85221),(#85222,#85223),(#85224,#85225),(#85226,
#85227),(#85228,#85229),(#85230,#85231),(#85232,#85233),(#85234,#85235),
(#85236,#85237),(#85238,#85239),(#85240,#85241),(#85242,#85243),(#85244,
#85245),(#85246,#85247),(#85248,#85249),(#85250,#85251),(#85252,#85253),
(#85254,#85255),(#85256,#85257),(#85258,#85259),(#85260,#85261),(#85262,
#85263),(#85264,#85265),(#85266,#85267),(#85268,#85269),(#85270,#85271),
(#85272,#85273),(#85274,#85275),(#85276,#85277),(#85278,#85279),(#85280,
#85281),(#85282,#85283),(#85284,#85285),(#85286,#85287)),.UNSPECIFIED.,
 .F.,.F.,.F.)
B_SPLINE_SURFACE_WITH_KNOTS((6,1,1,1,1,1,1,1,1,1,1,1,1,1,1,1,1,1,1,1,1,
1,1,1,1,1,1,1,1,1,1,1,1,1,1,1,1,1,1,1,1,1,1,1,1,1,1,1,1,1,1,1,1,1,1,1,1,
1,1,1,1,1,1,1,1,1,1,1,1,1,1,1,1,1,1,1,1,1,1,1,1,1,1,1,1,1,1,1,1,1,1,1,1,
1,1,1,1,1,1,1,1,1,1,1,1,1,1,1,1,1,1,1,1,1,1,1,1,1,1,1,1,1,1,1,1,1,1,1,1,
1,1,1,1,1,1,1,1,1,1,1,1,1,1,1,1,1,1,1,1,1,1,1,1,1,1,1,1,1,1,1,1,1,1,1,1,
1,1,1,1,1,1,1,1,1,1,1,1,1,1,1,1,1,1,1,1,1,1,1,1,1,1,1,1,1,1,1,1,1,1,1,6),
(2,2),(0.,0.005,0.01,0.015,0.02,0.025,0.03,0.035,0.04,0.045,0.05,0.055,
0.06,0.065,0.07,0.075,0.08,0.085,0.09,0.095,0.1,0.105,0.11,0.115,0.12,0.125,
0.13,0.135,0.14,0.145,0.15,0.155,0.16,0.165,0.17,0.175,0.18,0.185,0.19,
0.195,0.2,0.205,0.21,0.215,0.22,0.225,0.23,0.235,0.24,0.245,0.25,0.255,
0.26,0.265,0.27,0.275,0.28,0.285,0.29,0.295,0.3,0.305,0.31,0.315,0.32,0.325,
0.33,0.335,0.34,0.345,0.35,0.355,0.36,0.365,0.37,0.375,0.38,0.385,0.39,
0.395,0.4,0.405,0.41,0.415,0.42,0.425,0.43,0.435,0.44,0.445,0.45,0.455,
0.46,0.465,0.47,0.475,0.48,0.485,0.49,0.495,0.5,0.505,0.51,0.515,0.52,0.525,
0.53,0.535,0.54,0.545,0.55,0.555,0.56,0.565,0.57,0.575,0.58,0.585,0.59,
0.595,0.6,0.605,0.61,0.615,0.62,0.625,0.63,0.635,0.64,0.645,0.65,0.655,
0.66,0.665,0.67,0.675,0.68,0.685,0.690000000000001,0.695000000000001,0.700000000000001,
0.705000000000001,0.710000000000001,0.715000000000001,0.720000000000001,
0.725000000000001,0.730000000000001,0.735000000000001,0.740000000000001,
0.745000000000001,0.750000000000001,0.755000000000001,0.760000000000001,
0.765000000000001,0.770000000000001,0.775000000000001,0.780000000000001,
0.785000000000001,0.790000000000001,0.795000000000001,0.800000000000001,
0.805000000000001,0.810000000000001,0.815000000000001,0.820000000000001,
0.825000000000001,0.830000000000001,0.835000000000001,0.840000000000001,
0.845000000000001,0.850000000000001,0.855000000000001,0.860000000000001,
0.865000000000001,0.870000000000001,0.875000000000001,0.880000000000001,
0.885000000000001,0.890000000000001,0.895000000000001,0.900000000000001,
0.905000000000001,0.910000000000001,0.915000000000001,0.920000000000001,
0.925000000000001,0.930000000000001,0.935000000000001,0.940000000000001,
0.945000000000001,0.950000000000001,0.955000000000001,0.960000000000001,
0.965000000000001,0.970000000000001,0.975000000000001,0.980000000000001,
0.985000000000001,0.990000000000001,0.995000000000001,1.),(0.,1.2),
 .UNSPECIFIED.)
GEOMETRIC_REPRESENTATION_ITEM()
RATIONAL_B_SPLINE_SURFACE(((1.,1.),(1.,1.),(1.,1.),(1.,1.),(1.,1.),(1.,
1.),(1.,1.),(1.,1.),(1.,1.),(1.,1.),(1.,1.),(1.,1.),(1.,1.),(1.,1.),(1.,
1.),(1.,1.),(1.,1.),(1.,1.),(1.,1.),(1.,1.),(1.,1.),(1.,1.),(1.,1.),(1.,
1.),(1.,1.),(1.,1.),(1.,1.),(1.,1.),(1.,1.),(1.,1.),(1.,1.),(1.,1.),(1.,
1.),(1.,1.),(1.,1.),(1.,1.),(1.,1.),(1.,1.),(1.,1.),(1.,1.),(1.,1.),(1.,
1.),(1.,1.),(1.,1.),(1.,1.),(1.,1.),(1.,1.),(1.,1.),(1.,1.),(1.,1.),(1.,
1.),(1.,1.),(1.,1.),(1.,1.),(1.,1.),(1.,1.),(1.,1.),(1.,1.),(1.,1.),(1.,
1.),(1.,1.),(1.,1.),(1.,1.),(1.,1.),(1.,1.),(1.,1.),(1.,1.),(1.,1.),(1.,
1.),(1.,1.),(1.,1.),(1.,1.),(1.,1.),(1.,1.),(1.,1.),(1.,1.),(1.,1.),(1.,
1.),(1.,1.),(1.,1.),(1.,1.),(1.,1.),(1.,1.),(1.,1.),(1.,1.),(1.,1.),(1.,
1.),(1.,1.),(1.,1.),(1.,1.),(1.,1.),(1.,1.),(1.,1.),(1.,1.),(1.,1.),(1.,
1.),(1.,1.),(1.,1.),(1.,1.),(1.,1.),(1.,1.),(1.,1.),(1.,1.),(1.,1.),(1.,
1.),(1.,1.),(1.,1.),(1.,1.),(1.,1.),(1.,1.),(1.,1.),(1.,1.),(1.,1.),(1.,
1.),(1.,1.),(1.,1.),(1.,1.),(1.,1.),(1.,1.),(1.,1.),(1.,1.),(1.,1.),(1.,
1.),(1.,1.),(1.,1.),(1.,1.),(1.,1.),(1.,1.),(1.,1.),(1.,1.),(1.,1.),(1.,
1.),(1.,1.),(1.,1.),(1.,1.),(1.,1.),(1.,1.),(1.,1.),(1.,1.),(1.,1.),(1.,
1.),(1.,1.),(1.,1.),(1.,1.),(1.,1.),(1.,1.),(1.,1.),(1.,1.),(1.,1.),(1.,
1.),(1.,1.),(1.,1.),(1.,1.),(1.,1.),(1.,1.),(1.,1.),(1.,1.),(1.,1.),(1.,
1.),(1.,1.),(1.,1.),(1.,1.),(1.,1.),(1.,1.),(1.,1.),(1.,1.),(1.,1.),(1.,
1.),(1.,1.),(1.,1.),(1.,1.),(1.,1.),(1.,1.),(1.,1.),(1.,1.),(1.,1.),(1.,
1.),(1.,1.),(1.,1.),(1.,1.),(1.,1.),(1.,1.),(1.,1.),(1.,1.),(1.,1.),(1.,
1.),(1.,1.),(1.,1.),(1.,1.),(1.,1.),(1.,1.),(1.,1.),(1.,1.),(1.,1.),(1.,
1.),(1.,1.),(1.,1.),(1.,1.),(1.,1.),(1.,1.),(1.,1.),(1.,1.),(1.,1.),(1.,
1.),(1.,1.)))
REPRESENTATION_ITEM('')
SURFACE()
);
#920=(
BOUNDED_SURFACE()
B_SPLINE_SURFACE(5,1,((#85774,#85775),(#85776,#85777),(#85778,#85779),(#85780,
#85781),(#85782,#85783),(#85784,#85785),(#85786,#85787),(#85788,#85789),
(#85790,#85791),(#85792,#85793),(#85794,#85795),(#85796,#85797),(#85798,
#85799),(#85800,#85801),(#85802,#85803),(#85804,#85805),(#85806,#85807),
(#85808,#85809),(#85810,#85811),(#85812,#85813),(#85814,#85815),(#85816,
#85817),(#85818,#85819),(#85820,#85821),(#85822,#85823),(#85824,#85825),
(#85826,#85827),(#85828,#85829),(#85830,#85831),(#85832,#85833),(#85834,
#85835),(#85836,#85837),(#85838,#85839),(#85840,#85841),(#85842,#85843),
(#85844,#85845),(#85846,#85847),(#85848,#85849),(#85850,#85851),(#85852,
#85853),(#85854,#85855),(#85856,#85857),(#85858,#85859),(#85860,#85861),
(#85862,#85863),(#85864,#85865),(#85866,#85867),(#85868,#85869),(#85870,
#85871),(#85872,#85873),(#85874,#85875),(#85876,#85877),(#85878,#85879),
(#85880,#85881),(#85882,#85883),(#85884,#85885),(#85886,#85887),(#85888,
#85889),(#85890,#85891),(#85892,#85893),(#85894,#85895),(#85896,#85897),
(#85898,#85899),(#85900,#85901),(#85902,#85903),(#85904,#85905),(#85906,
#85907),(#85908,#85909),(#85910,#85911),(#85912,#85913),(#85914,#85915),
(#85916,#85917),(#85918,#85919),(#85920,#85921),(#85922,#85923),(#85924,
#85925),(#85926,#85927),(#85928,#85929),(#85930,#85931),(#85932,#85933),
(#85934,#85935),(#85936,#85937),(#85938,#85939),(#85940,#85941),(#85942,
#85943),(#85944,#85945),(#85946,#85947),(#85948,#85949),(#85950,#85951),
(#85952,#85953),(#85954,#85955),(#85956,#85957),(#85958,#85959),(#85960,
#85961),(#85962,#85963),(#85964,#85965),(#85966,#85967),(#85968,#85969),
(#85970,#85971),(#85972,#85973),(#85974,#85975),(#85976,#85977),(#85978,
#85979),(#85980,#85981),(#85982,#85983),(#85984,#85985),(#85986,#85987),
(#85988,#85989),(#85990,#85991),(#85992,#85993),(#85994,#85995),(#85996,
#85997),(#85998,#85999),(#86000,#86001),(#86002,#86003),(#86004,#86005),
(#86006,#86007),(#86008,#86009),(#86010,#86011),(#86012,#86013),(#86014,
#86015),(#86016,#86017),(#86018,#86019),(#86020,#86021),(#86022,#86023),
(#86024,#86025),(#86026,#86027),(#86028,#86029),(#86030,#86031),(#86032,
#86033),(#86034,#86035),(#86036,#86037),(#86038,#86039),(#86040,#86041),
(#86042,#86043),(#86044,#86045),(#86046,#86047),(#86048,#86049),(#86050,
#86051),(#86052,#86053),(#86054,#86055),(#86056,#86057),(#86058,#86059),
(#86060,#86061),(#86062,#86063),(#86064,#86065),(#86066,#86067),(#86068,
#86069),(#86070,#86071),(#86072,#86073),(#86074,#86075),(#86076,#86077),
(#86078,#86079),(#86080,#86081),(#86082,#86083),(#86084,#86085),(#86086,
#86087),(#86088,#86089),(#86090,#86091),(#86092,#86093),(#86094,#86095),
(#86096,#86097),(#86098,#86099),(#86100,#86101),(#86102,#86103),(#86104,
#86105),(#86106,#86107),(#86108,#86109),(#86110,#86111),(#86112,#86113),
(#86114,#86115),(#86116,#86117),(#86118,#86119),(#86120,#86121),(#86122,
#86123),(#86124,#86125),(#86126,#86127),(#86128,#86129),(#86130,#86131),
(#86132,#86133),(#86134,#86135),(#86136,#86137),(#86138,#86139),(#86140,
#86141),(#86142,#86143),(#86144,#86145),(#86146,#86147),(#86148,#86149),
(#86150,#86151),(#86152,#86153),(#86154,#86155),(#86156,#86157),(#86158,
#86159),(#86160,#86161),(#86162,#86163),(#86164,#86165),(#86166,#86167),
(#86168,#86169),(#86170,#86171),(#86172,#86173),(#86174,#86175),(#86176,
#86177),(#86178,#86179),(#86180,#86181),(#86182,#86183)),.UNSPECIFIED.,
 .F.,.F.,.F.)
B_SPLINE_SURFACE_WITH_KNOTS((6,1,1,1,1,1,1,1,1,1,1,1,1,1,1,1,1,1,1,1,1,
1,1,1,1,1,1,1,1,1,1,1,1,1,1,1,1,1,1,1,1,1,1,1,1,1,1,1,1,1,1,1,1,1,1,1,1,
1,1,1,1,1,1,1,1,1,1,1,1,1,1,1,1,1,1,1,1,1,1,1,1,1,1,1,1,1,1,1,1,1,1,1,1,
1,1,1,1,1,1,1,1,1,1,1,1,1,1,1,1,1,1,1,1,1,1,1,1,1,1,1,1,1,1,1,1,1,1,1,1,
1,1,1,1,1,1,1,1,1,1,1,1,1,1,1,1,1,1,1,1,1,1,1,1,1,1,1,1,1,1,1,1,1,1,1,1,
1,1,1,1,1,1,1,1,1,1,1,1,1,1,1,1,1,1,1,1,1,1,1,1,1,1,1,1,1,1,1,1,1,1,1,6),
(2,2),(0.,0.005,0.01,0.015,0.02,0.025,0.03,0.035,0.04,0.045,0.05,0.055,
0.06,0.065,0.07,0.075,0.08,0.085,0.09,0.095,0.1,0.105,0.11,0.115,0.12,0.125,
0.13,0.135,0.14,0.145,0.15,0.155,0.16,0.165,0.17,0.175,0.18,0.185,0.19,
0.195,0.2,0.205,0.21,0.215,0.22,0.225,0.23,0.235,0.24,0.245,0.25,0.255,
0.26,0.265,0.27,0.275,0.28,0.285,0.29,0.295,0.3,0.305,0.31,0.315,0.32,0.325,
0.33,0.335,0.34,0.345,0.35,0.355,0.36,0.365,0.37,0.375,0.38,0.385,0.39,
0.395,0.4,0.405,0.41,0.415,0.42,0.425,0.43,0.435,0.44,0.445,0.45,0.455,
0.46,0.465,0.47,0.475,0.48,0.485,0.49,0.495,0.5,0.505,0.51,0.515,0.52,0.525,
0.53,0.535,0.54,0.545,0.55,0.555,0.56,0.565,0.57,0.575,0.58,0.585,0.59,
0.595,0.6,0.605,0.61,0.615,0.62,0.625,0.63,0.635,0.64,0.645,0.65,0.655,
0.66,0.665,0.67,0.675,0.68,0.685,0.690000000000001,0.695000000000001,0.700000000000001,
0.705000000000001,0.710000000000001,0.715000000000001,0.720000000000001,
0.725000000000001,0.730000000000001,0.735000000000001,0.740000000000001,
0.745000000000001,0.750000000000001,0.755000000000001,0.760000000000001,
0.765000000000001,0.770000000000001,0.775000000000001,0.780000000000001,
0.785000000000001,0.790000000000001,0.795000000000001,0.800000000000001,
0.805000000000001,0.810000000000001,0.815000000000001,0.820000000000001,
0.825000000000001,0.830000000000001,0.835000000000001,0.840000000000001,
0.845000000000001,0.850000000000001,0.855000000000001,0.860000000000001,
0.865000000000001,0.870000000000001,0.875000000000001,0.880000000000001,
0.885000000000001,0.890000000000001,0.895000000000001,0.900000000000001,
0.905000000000001,0.910000000000001,0.915000000000001,0.920000000000001,
0.925000000000001,0.930000000000001,0.935000000000001,0.940000000000001,
0.945000000000001,0.950000000000001,0.955000000000001,0.960000000000001,
0.965000000000001,0.970000000000001,0.975000000000001,0.980000000000001,
0.985000000000001,0.990000000000001,0.995000000000001,1.),(0.,1.2),
 .UNSPECIFIED.)
GEOMETRIC_REPRESENTATION_ITEM()
RATIONAL_B_SPLINE_SURFACE(((1.,1.),(1.,1.),(1.,1.),(1.,1.),(1.,1.),(1.,
1.),(1.,1.),(1.,1.),(1.,1.),(1.,1.),(1.,1.),(1.,1.),(1.,1.),(1.,1.),(1.,
1.),(1.,1.),(1.,1.),(1.,1.),(1.,1.),(1.,1.),(1.,1.),(1.,1.),(1.,1.),(1.,
1.),(1.,1.),(1.,1.),(1.,1.),(1.,1.),(1.,1.),(1.,1.),(1.,1.),(1.,1.),(1.,
1.),(1.,1.),(1.,1.),(1.,1.),(1.,1.),(1.,1.),(1.,1.),(1.,1.),(1.,1.),(1.,
1.),(1.,1.),(1.,1.),(1.,1.),(1.,1.),(1.,1.),(1.,1.),(1.,1.),(1.,1.),(1.,
1.),(1.,1.),(1.,1.),(1.,1.),(1.,1.),(1.,1.),(1.,1.),(1.,1.),(1.,1.),(1.,
1.),(1.,1.),(1.,1.),(1.,1.),(1.,1.),(1.,1.),(1.,1.),(1.,1.),(1.,1.),(1.,
1.),(1.,1.),(1.,1.),(1.,1.),(1.,1.),(1.,1.),(1.,1.),(1.,1.),(1.,1.),(1.,
1.),(1.,1.),(1.,1.),(1.,1.),(1.,1.),(1.,1.),(1.,1.),(1.,1.),(1.,1.),(1.,
1.),(1.,1.),(1.,1.),(1.,1.),(1.,1.),(1.,1.),(1.,1.),(1.,1.),(1.,1.),(1.,
1.),(1.,1.),(1.,1.),(1.,1.),(1.,1.),(1.,1.),(1.,1.),(1.,1.),(1.,1.),(1.,
1.),(1.,1.),(1.,1.),(1.,1.),(1.,1.),(1.,1.),(1.,1.),(1.,1.),(1.,1.),(1.,
1.),(1.,1.),(1.,1.),(1.,1.),(1.,1.),(1.,1.),(1.,1.),(1.,1.),(1.,1.),(1.,
1.),(1.,1.),(1.,1.),(1.,1.),(1.,1.),(1.,1.),(1.,1.),(1.,1.),(1.,1.),(1.,
1.),(1.,1.),(1.,1.),(1.,1.),(1.,1.),(1.,1.),(1.,1.),(1.,1.),(1.,1.),(1.,
1.),(1.,1.),(1.,1.),(1.,1.),(1.,1.),(1.,1.),(1.,1.),(1.,1.),(1.,1.),(1.,
1.),(1.,1.),(1.,1.),(1.,1.),(1.,1.),(1.,1.),(1.,1.),(1.,1.),(1.,1.),(1.,
1.),(1.,1.),(1.,1.),(1.,1.),(1.,1.),(1.,1.),(1.,1.),(1.,1.),(1.,1.),(1.,
1.),(1.,1.),(1.,1.),(1.,1.),(1.,1.),(1.,1.),(1.,1.),(1.,1.),(1.,1.),(1.,
1.),(1.,1.),(1.,1.),(1.,1.),(1.,1.),(1.,1.),(1.,1.),(1.,1.),(1.,1.),(1.,
1.),(1.,1.),(1.,1.),(1.,1.),(1.,1.),(1.,1.),(1.,1.),(1.,1.),(1.,1.),(1.,
1.),(1.,1.),(1.,1.),(1.,1.),(1.,1.),(1.,1.),(1.,1.),(1.,1.),(1.,1.),(1.,
1.),(1.,1.)))
REPRESENTATION_ITEM('')
SURFACE()
);
#921=(
BOUNDED_SURFACE()
B_SPLINE_SURFACE(5,1,((#86670,#86671),(#86672,#86673),(#86674,#86675),(#86676,
#86677),(#86678,#86679),(#86680,#86681),(#86682,#86683),(#86684,#86685),
(#86686,#86687),(#86688,#86689),(#86690,#86691),(#86692,#86693),(#86694,
#86695),(#86696,#86697),(#86698,#86699),(#86700,#86701),(#86702,#86703),
(#86704,#86705),(#86706,#86707),(#86708,#86709),(#86710,#86711),(#86712,
#86713),(#86714,#86715),(#86716,#86717),(#86718,#86719),(#86720,#86721),
(#86722,#86723),(#86724,#86725),(#86726,#86727),(#86728,#86729),(#86730,
#86731),(#86732,#86733),(#86734,#86735),(#86736,#86737),(#86738,#86739),
(#86740,#86741),(#86742,#86743),(#86744,#86745),(#86746,#86747),(#86748,
#86749),(#86750,#86751),(#86752,#86753),(#86754,#86755),(#86756,#86757),
(#86758,#86759),(#86760,#86761),(#86762,#86763),(#86764,#86765),(#86766,
#86767),(#86768,#86769),(#86770,#86771),(#86772,#86773),(#86774,#86775),
(#86776,#86777),(#86778,#86779),(#86780,#86781),(#86782,#86783),(#86784,
#86785),(#86786,#86787),(#86788,#86789),(#86790,#86791),(#86792,#86793),
(#86794,#86795),(#86796,#86797),(#86798,#86799),(#86800,#86801),(#86802,
#86803),(#86804,#86805),(#86806,#86807),(#86808,#86809),(#86810,#86811),
(#86812,#86813),(#86814,#86815),(#86816,#86817),(#86818,#86819),(#86820,
#86821),(#86822,#86823),(#86824,#86825),(#86826,#86827),(#86828,#86829),
(#86830,#86831),(#86832,#86833),(#86834,#86835),(#86836,#86837),(#86838,
#86839),(#86840,#86841),(#86842,#86843),(#86844,#86845),(#86846,#86847),
(#86848,#86849),(#86850,#86851),(#86852,#86853),(#86854,#86855),(#86856,
#86857),(#86858,#86859),(#86860,#86861),(#86862,#86863),(#86864,#86865),
(#86866,#86867),(#86868,#86869),(#86870,#86871),(#86872,#86873),(#86874,
#86875),(#86876,#86877),(#86878,#86879),(#86880,#86881),(#86882,#86883),
(#86884,#86885),(#86886,#86887),(#86888,#86889),(#86890,#86891),(#86892,
#86893),(#86894,#86895),(#86896,#86897),(#86898,#86899),(#86900,#86901),
(#86902,#86903),(#86904,#86905),(#86906,#86907),(#86908,#86909),(#86910,
#86911),(#86912,#86913),(#86914,#86915),(#86916,#86917),(#86918,#86919),
(#86920,#86921),(#86922,#86923),(#86924,#86925),(#86926,#86927),(#86928,
#86929),(#86930,#86931),(#86932,#86933),(#86934,#86935),(#86936,#86937),
(#86938,#86939),(#86940,#86941),(#86942,#86943),(#86944,#86945),(#86946,
#86947),(#86948,#86949),(#86950,#86951),(#86952,#86953),(#86954,#86955),
(#86956,#86957),(#86958,#86959),(#86960,#86961),(#86962,#86963),(#86964,
#86965),(#86966,#86967),(#86968,#86969),(#86970,#86971),(#86972,#86973),
(#86974,#86975),(#86976,#86977),(#86978,#86979),(#86980,#86981),(#86982,
#86983),(#86984,#86985),(#86986,#86987),(#86988,#86989),(#86990,#86991),
(#86992,#86993),(#86994,#86995),(#86996,#86997),(#86998,#86999),(#87000,
#87001),(#87002,#87003),(#87004,#87005),(#87006,#87007),(#87008,#87009),
(#87010,#87011),(#87012,#87013),(#87014,#87015),(#87016,#87017),(#87018,
#87019),(#87020,#87021),(#87022,#87023),(#87024,#87025),(#87026,#87027),
(#87028,#87029),(#87030,#87031),(#87032,#87033),(#87034,#87035),(#87036,
#87037),(#87038,#87039),(#87040,#87041),(#87042,#87043),(#87044,#87045),
(#87046,#87047),(#87048,#87049),(#87050,#87051),(#87052,#87053),(#87054,
#87055),(#87056,#87057),(#87058,#87059),(#87060,#87061),(#87062,#87063),
(#87064,#87065),(#87066,#87067),(#87068,#87069),(#87070,#87071),(#87072,
#87073),(#87074,#87075),(#87076,#87077),(#87078,#87079)),.UNSPECIFIED.,
 .F.,.F.,.F.)
B_SPLINE_SURFACE_WITH_KNOTS((6,1,1,1,1,1,1,1,1,1,1,1,1,1,1,1,1,1,1,1,1,
1,1,1,1,1,1,1,1,1,1,1,1,1,1,1,1,1,1,1,1,1,1,1,1,1,1,1,1,1,1,1,1,1,1,1,1,
1,1,1,1,1,1,1,1,1,1,1,1,1,1,1,1,1,1,1,1,1,1,1,1,1,1,1,1,1,1,1,1,1,1,1,1,
1,1,1,1,1,1,1,1,1,1,1,1,1,1,1,1,1,1,1,1,1,1,1,1,1,1,1,1,1,1,1,1,1,1,1,1,
1,1,1,1,1,1,1,1,1,1,1,1,1,1,1,1,1,1,1,1,1,1,1,1,1,1,1,1,1,1,1,1,1,1,1,1,
1,1,1,1,1,1,1,1,1,1,1,1,1,1,1,1,1,1,1,1,1,1,1,1,1,1,1,1,1,1,1,1,1,1,1,6),
(2,2),(0.,0.005,0.01,0.015,0.02,0.025,0.03,0.035,0.04,0.045,0.05,0.055,
0.06,0.065,0.07,0.075,0.08,0.085,0.09,0.095,0.1,0.105,0.11,0.115,0.12,0.125,
0.13,0.135,0.14,0.145,0.15,0.155,0.16,0.165,0.17,0.175,0.18,0.185,0.19,
0.195,0.2,0.205,0.21,0.215,0.22,0.225,0.23,0.235,0.24,0.245,0.25,0.255,
0.26,0.265,0.27,0.275,0.28,0.285,0.29,0.295,0.3,0.305,0.31,0.315,0.32,0.325,
0.33,0.335,0.34,0.345,0.35,0.355,0.36,0.365,0.37,0.375,0.38,0.385,0.39,
0.395,0.4,0.405,0.41,0.415,0.42,0.425,0.43,0.435,0.44,0.445,0.45,0.455,
0.46,0.465,0.47,0.475,0.48,0.485,0.49,0.495,0.5,0.505,0.51,0.515,0.52,0.525,
0.53,0.535,0.54,0.545,0.55,0.555,0.56,0.565,0.57,0.575,0.58,0.585,0.59,
0.595,0.6,0.605,0.61,0.615,0.62,0.625,0.63,0.635,0.64,0.645,0.65,0.655,
0.66,0.665,0.67,0.675,0.68,0.685,0.690000000000001,0.695000000000001,0.700000000000001,
0.705000000000001,0.710000000000001,0.715000000000001,0.720000000000001,
0.725000000000001,0.730000000000001,0.735000000000001,0.740000000000001,
0.745000000000001,0.750000000000001,0.755000000000001,0.760000000000001,
0.765000000000001,0.770000000000001,0.775000000000001,0.780000000000001,
0.785000000000001,0.790000000000001,0.795000000000001,0.800000000000001,
0.805000000000001,0.810000000000001,0.815000000000001,0.820000000000001,
0.825000000000001,0.830000000000001,0.835000000000001,0.840000000000001,
0.845000000000001,0.850000000000001,0.855000000000001,0.860000000000001,
0.865000000000001,0.870000000000001,0.875000000000001,0.880000000000001,
0.885000000000001,0.890000000000001,0.895000000000001,0.900000000000001,
0.905000000000001,0.910000000000001,0.915000000000001,0.920000000000001,
0.925000000000001,0.930000000000001,0.935000000000001,0.940000000000001,
0.945000000000001,0.950000000000001,0.955000000000001,0.960000000000001,
0.965000000000001,0.970000000000001,0.975000000000001,0.980000000000001,
0.985000000000001,0.990000000000001,0.995000000000001,1.),(0.,1.2),
 .UNSPECIFIED.)
GEOMETRIC_REPRESENTATION_ITEM()
RATIONAL_B_SPLINE_SURFACE(((1.,1.),(1.,1.),(1.,1.),(1.,1.),(1.,1.),(1.,
1.),(1.,1.),(1.,1.),(1.,1.),(1.,1.),(1.,1.),(1.,1.),(1.,1.),(1.,1.),(1.,
1.),(1.,1.),(1.,1.),(1.,1.),(1.,1.),(1.,1.),(1.,1.),(1.,1.),(1.,1.),(1.,
1.),(1.,1.),(1.,1.),(1.,1.),(1.,1.),(1.,1.),(1.,1.),(1.,1.),(1.,1.),(1.,
1.),(1.,1.),(1.,1.),(1.,1.),(1.,1.),(1.,1.),(1.,1.),(1.,1.),(1.,1.),(1.,
1.),(1.,1.),(1.,1.),(1.,1.),(1.,1.),(1.,1.),(1.,1.),(1.,1.),(1.,1.),(1.,
1.),(1.,1.),(1.,1.),(1.,1.),(1.,1.),(1.,1.),(1.,1.),(1.,1.),(1.,1.),(1.,
1.),(1.,1.),(1.,1.),(1.,1.),(1.,1.),(1.,1.),(1.,1.),(1.,1.),(1.,1.),(1.,
1.),(1.,1.),(1.,1.),(1.,1.),(1.,1.),(1.,1.),(1.,1.),(1.,1.),(1.,1.),(1.,
1.),(1.,1.),(1.,1.),(1.,1.),(1.,1.),(1.,1.),(1.,1.),(1.,1.),(1.,1.),(1.,
1.),(1.,1.),(1.,1.),(1.,1.),(1.,1.),(1.,1.),(1.,1.),(1.,1.),(1.,1.),(1.,
1.),(1.,1.),(1.,1.),(1.,1.),(1.,1.),(1.,1.),(1.,1.),(1.,1.),(1.,1.),(1.,
1.),(1.,1.),(1.,1.),(1.,1.),(1.,1.),(1.,1.),(1.,1.),(1.,1.),(1.,1.),(1.,
1.),(1.,1.),(1.,1.),(1.,1.),(1.,1.),(1.,1.),(1.,1.),(1.,1.),(1.,1.),(1.,
1.),(1.,1.),(1.,1.),(1.,1.),(1.,1.),(1.,1.),(1.,1.),(1.,1.),(1.,1.),(1.,
1.),(1.,1.),(1.,1.),(1.,1.),(1.,1.),(1.,1.),(1.,1.),(1.,1.),(1.,1.),(1.,
1.),(1.,1.),(1.,1.),(1.,1.),(1.,1.),(1.,1.),(1.,1.),(1.,1.),(1.,1.),(1.,
1.),(1.,1.),(1.,1.),(1.,1.),(1.,1.),(1.,1.),(1.,1.),(1.,1.),(1.,1.),(1.,
1.),(1.,1.),(1.,1.),(1.,1.),(1.,1.),(1.,1.),(1.,1.),(1.,1.),(1.,1.),(1.,
1.),(1.,1.),(1.,1.),(1.,1.),(1.,1.),(1.,1.),(1.,1.),(1.,1.),(1.,1.),(1.,
1.),(1.,1.),(1.,1.),(1.,1.),(1.,1.),(1.,1.),(1.,1.),(1.,1.),(1.,1.),(1.,
1.),(1.,1.),(1.,1.),(1.,1.),(1.,1.),(1.,1.),(1.,1.),(1.,1.),(1.,1.),(1.,
1.),(1.,1.),(1.,1.),(1.,1.),(1.,1.),(1.,1.),(1.,1.),(1.,1.),(1.,1.),(1.,
1.),(1.,1.)))
REPRESENTATION_ITEM('')
SURFACE()
);
#922=(
BOUNDED_SURFACE()
B_SPLINE_SURFACE(5,1,((#87566,#87567),(#87568,#87569),(#87570,#87571),(#87572,
#87573),(#87574,#87575),(#87576,#87577),(#87578,#87579),(#87580,#87581),
(#87582,#87583),(#87584,#87585),(#87586,#87587),(#87588,#87589),(#87590,
#87591),(#87592,#87593),(#87594,#87595),(#87596,#87597),(#87598,#87599),
(#87600,#87601),(#87602,#87603),(#87604,#87605),(#87606,#87607),(#87608,
#87609),(#87610,#87611),(#87612,#87613),(#87614,#87615),(#87616,#87617),
(#87618,#87619),(#87620,#87621),(#87622,#87623),(#87624,#87625),(#87626,
#87627),(#87628,#87629),(#87630,#87631),(#87632,#87633),(#87634,#87635),
(#87636,#87637),(#87638,#87639),(#87640,#87641),(#87642,#87643),(#87644,
#87645),(#87646,#87647),(#87648,#87649),(#87650,#87651),(#87652,#87653),
(#87654,#87655),(#87656,#87657),(#87658,#87659),(#87660,#87661),(#87662,
#87663),(#87664,#87665),(#87666,#87667),(#87668,#87669),(#87670,#87671),
(#87672,#87673),(#87674,#87675),(#87676,#87677),(#87678,#87679),(#87680,
#87681),(#87682,#87683),(#87684,#87685),(#87686,#87687),(#87688,#87689),
(#87690,#87691),(#87692,#87693),(#87694,#87695),(#87696,#87697),(#87698,
#87699),(#87700,#87701),(#87702,#87703),(#87704,#87705),(#87706,#87707),
(#87708,#87709),(#87710,#87711),(#87712,#87713),(#87714,#87715),(#87716,
#87717),(#87718,#87719),(#87720,#87721),(#87722,#87723),(#87724,#87725),
(#87726,#87727),(#87728,#87729),(#87730,#87731),(#87732,#87733),(#87734,
#87735),(#87736,#87737),(#87738,#87739),(#87740,#87741),(#87742,#87743),
(#87744,#87745),(#87746,#87747),(#87748,#87749),(#87750,#87751),(#87752,
#87753),(#87754,#87755),(#87756,#87757),(#87758,#87759),(#87760,#87761),
(#87762,#87763),(#87764,#87765),(#87766,#87767),(#87768,#87769),(#87770,
#87771),(#87772,#87773),(#87774,#87775),(#87776,#87777),(#87778,#87779),
(#87780,#87781),(#87782,#87783),(#87784,#87785),(#87786,#87787),(#87788,
#87789),(#87790,#87791),(#87792,#87793),(#87794,#87795),(#87796,#87797),
(#87798,#87799),(#87800,#87801),(#87802,#87803),(#87804,#87805),(#87806,
#87807),(#87808,#87809),(#87810,#87811),(#87812,#87813),(#87814,#87815),
(#87816,#87817),(#87818,#87819),(#87820,#87821),(#87822,#87823),(#87824,
#87825),(#87826,#87827),(#87828,#87829),(#87830,#87831),(#87832,#87833),
(#87834,#87835),(#87836,#87837),(#87838,#87839),(#87840,#87841),(#87842,
#87843),(#87844,#87845),(#87846,#87847),(#87848,#87849),(#87850,#87851),
(#87852,#87853),(#87854,#87855),(#87856,#87857),(#87858,#87859),(#87860,
#87861),(#87862,#87863),(#87864,#87865),(#87866,#87867),(#87868,#87869),
(#87870,#87871),(#87872,#87873),(#87874,#87875),(#87876,#87877),(#87878,
#87879),(#87880,#87881),(#87882,#87883),(#87884,#87885),(#87886,#87887),
(#87888,#87889),(#87890,#87891),(#87892,#87893),(#87894,#87895),(#87896,
#87897),(#87898,#87899),(#87900,#87901),(#87902,#87903),(#87904,#87905),
(#87906,#87907),(#87908,#87909),(#87910,#87911),(#87912,#87913),(#87914,
#87915),(#87916,#87917),(#87918,#87919),(#87920,#87921),(#87922,#87923),
(#87924,#87925),(#87926,#87927),(#87928,#87929),(#87930,#87931),(#87932,
#87933),(#87934,#87935),(#87936,#87937),(#87938,#87939),(#87940,#87941),
(#87942,#87943),(#87944,#87945),(#87946,#87947),(#87948,#87949),(#87950,
#87951),(#87952,#87953),(#87954,#87955),(#87956,#87957),(#87958,#87959),
(#87960,#87961),(#87962,#87963),(#87964,#87965),(#87966,#87967),(#87968,
#87969),(#87970,#87971),(#87972,#87973),(#87974,#87975)),.UNSPECIFIED.,
 .F.,.F.,.F.)
B_SPLINE_SURFACE_WITH_KNOTS((6,1,1,1,1,1,1,1,1,1,1,1,1,1,1,1,1,1,1,1,1,
1,1,1,1,1,1,1,1,1,1,1,1,1,1,1,1,1,1,1,1,1,1,1,1,1,1,1,1,1,1,1,1,1,1,1,1,
1,1,1,1,1,1,1,1,1,1,1,1,1,1,1,1,1,1,1,1,1,1,1,1,1,1,1,1,1,1,1,1,1,1,1,1,
1,1,1,1,1,1,1,1,1,1,1,1,1,1,1,1,1,1,1,1,1,1,1,1,1,1,1,1,1,1,1,1,1,1,1,1,
1,1,1,1,1,1,1,1,1,1,1,1,1,1,1,1,1,1,1,1,1,1,1,1,1,1,1,1,1,1,1,1,1,1,1,1,
1,1,1,1,1,1,1,1,1,1,1,1,1,1,1,1,1,1,1,1,1,1,1,1,1,1,1,1,1,1,1,1,1,1,1,6),
(2,2),(0.,0.005,0.01,0.015,0.02,0.025,0.03,0.035,0.04,0.045,0.05,0.055,
0.06,0.065,0.07,0.075,0.08,0.085,0.09,0.095,0.1,0.105,0.11,0.115,0.12,0.125,
0.13,0.135,0.14,0.145,0.15,0.155,0.16,0.165,0.17,0.175,0.18,0.185,0.19,
0.195,0.2,0.205,0.21,0.215,0.22,0.225,0.23,0.235,0.24,0.245,0.25,0.255,
0.26,0.265,0.27,0.275,0.28,0.285,0.29,0.295,0.3,0.305,0.31,0.315,0.32,0.325,
0.33,0.335,0.34,0.345,0.35,0.355,0.36,0.365,0.37,0.375,0.38,0.385,0.39,
0.395,0.4,0.405,0.41,0.415,0.42,0.425,0.43,0.435,0.44,0.445,0.45,0.455,
0.46,0.465,0.47,0.475,0.48,0.485,0.49,0.495,0.5,0.505,0.51,0.515,0.52,0.525,
0.53,0.535,0.54,0.545,0.55,0.555,0.56,0.565,0.57,0.575,0.58,0.585,0.59,
0.595,0.6,0.605,0.61,0.615,0.62,0.625,0.63,0.635,0.64,0.645,0.65,0.655,
0.66,0.665,0.67,0.675,0.68,0.685,0.690000000000001,0.695000000000001,0.700000000000001,
0.705000000000001,0.710000000000001,0.715000000000001,0.720000000000001,
0.725000000000001,0.730000000000001,0.735000000000001,0.740000000000001,
0.745000000000001,0.750000000000001,0.755000000000001,0.760000000000001,
0.765000000000001,0.770000000000001,0.775000000000001,0.780000000000001,
0.785000000000001,0.790000000000001,0.795000000000001,0.800000000000001,
0.805000000000001,0.810000000000001,0.815000000000001,0.820000000000001,
0.825000000000001,0.830000000000001,0.835000000000001,0.840000000000001,
0.845000000000001,0.850000000000001,0.855000000000001,0.860000000000001,
0.865000000000001,0.870000000000001,0.875000000000001,0.880000000000001,
0.885000000000001,0.890000000000001,0.895000000000001,0.900000000000001,
0.905000000000001,0.910000000000001,0.915000000000001,0.920000000000001,
0.925000000000001,0.930000000000001,0.935000000000001,0.940000000000001,
0.945000000000001,0.950000000000001,0.955000000000001,0.960000000000001,
0.965000000000001,0.970000000000001,0.975000000000001,0.980000000000001,
0.985000000000001,0.990000000000001,0.995000000000001,1.),(0.,1.2),
 .UNSPECIFIED.)
GEOMETRIC_REPRESENTATION_ITEM()
RATIONAL_B_SPLINE_SURFACE(((1.,1.),(1.,1.),(1.,1.),(1.,1.),(1.,1.),(1.,
1.),(1.,1.),(1.,1.),(1.,1.),(1.,1.),(1.,1.),(1.,1.),(1.,1.),(1.,1.),(1.,
1.),(1.,1.),(1.,1.),(1.,1.),(1.,1.),(1.,1.),(1.,1.),(1.,1.),(1.,1.),(1.,
1.),(1.,1.),(1.,1.),(1.,1.),(1.,1.),(1.,1.),(1.,1.),(1.,1.),(1.,1.),(1.,
1.),(1.,1.),(1.,1.),(1.,1.),(1.,1.),(1.,1.),(1.,1.),(1.,1.),(1.,1.),(1.,
1.),(1.,1.),(1.,1.),(1.,1.),(1.,1.),(1.,1.),(1.,1.),(1.,1.),(1.,1.),(1.,
1.),(1.,1.),(1.,1.),(1.,1.),(1.,1.),(1.,1.),(1.,1.),(1.,1.),(1.,1.),(1.,
1.),(1.,1.),(1.,1.),(1.,1.),(1.,1.),(1.,1.),(1.,1.),(1.,1.),(1.,1.),(1.,
1.),(1.,1.),(1.,1.),(1.,1.),(1.,1.),(1.,1.),(1.,1.),(1.,1.),(1.,1.),(1.,
1.),(1.,1.),(1.,1.),(1.,1.),(1.,1.),(1.,1.),(1.,1.),(1.,1.),(1.,1.),(1.,
1.),(1.,1.),(1.,1.),(1.,1.),(1.,1.),(1.,1.),(1.,1.),(1.,1.),(1.,1.),(1.,
1.),(1.,1.),(1.,1.),(1.,1.),(1.,1.),(1.,1.),(1.,1.),(1.,1.),(1.,1.),(1.,
1.),(1.,1.),(1.,1.),(1.,1.),(1.,1.),(1.,1.),(1.,1.),(1.,1.),(1.,1.),(1.,
1.),(1.,1.),(1.,1.),(1.,1.),(1.,1.),(1.,1.),(1.,1.),(1.,1.),(1.,1.),(1.,
1.),(1.,1.),(1.,1.),(1.,1.),(1.,1.),(1.,1.),(1.,1.),(1.,1.),(1.,1.),(1.,
1.),(1.,1.),(1.,1.),(1.,1.),(1.,1.),(1.,1.),(1.,1.),(1.,1.),(1.,1.),(1.,
1.),(1.,1.),(1.,1.),(1.,1.),(1.,1.),(1.,1.),(1.,1.),(1.,1.),(1.,1.),(1.,
1.),(1.,1.),(1.,1.),(1.,1.),(1.,1.),(1.,1.),(1.,1.),(1.,1.),(1.,1.),(1.,
1.),(1.,1.),(1.,1.),(1.,1.),(1.,1.),(1.,1.),(1.,1.),(1.,1.),(1.,1.),(1.,
1.),(1.,1.),(1.,1.),(1.,1.),(1.,1.),(1.,1.),(1.,1.),(1.,1.),(1.,1.),(1.,
1.),(1.,1.),(1.,1.),(1.,1.),(1.,1.),(1.,1.),(1.,1.),(1.,1.),(1.,1.),(1.,
1.),(1.,1.),(1.,1.),(1.,1.),(1.,1.),(1.,1.),(1.,1.),(1.,1.),(1.,1.),(1.,
1.),(1.,1.),(1.,1.),(1.,1.),(1.,1.),(1.,1.),(1.,1.),(1.,1.),(1.,1.),(1.,
1.),(1.,1.)))
REPRESENTATION_ITEM('')
SURFACE()
);
#923=(
BOUNDED_SURFACE()
B_SPLINE_SURFACE(5,1,((#88462,#88463),(#88464,#88465),(#88466,#88467),(#88468,
#88469),(#88470,#88471),(#88472,#88473),(#88474,#88475),(#88476,#88477),
(#88478,#88479),(#88480,#88481),(#88482,#88483),(#88484,#88485),(#88486,
#88487),(#88488,#88489),(#88490,#88491),(#88492,#88493),(#88494,#88495),
(#88496,#88497),(#88498,#88499),(#88500,#88501),(#88502,#88503),(#88504,
#88505),(#88506,#88507),(#88508,#88509),(#88510,#88511),(#88512,#88513),
(#88514,#88515),(#88516,#88517),(#88518,#88519),(#88520,#88521),(#88522,
#88523),(#88524,#88525),(#88526,#88527),(#88528,#88529),(#88530,#88531),
(#88532,#88533),(#88534,#88535),(#88536,#88537),(#88538,#88539),(#88540,
#88541),(#88542,#88543),(#88544,#88545),(#88546,#88547),(#88548,#88549),
(#88550,#88551),(#88552,#88553),(#88554,#88555),(#88556,#88557),(#88558,
#88559),(#88560,#88561),(#88562,#88563),(#88564,#88565),(#88566,#88567),
(#88568,#88569),(#88570,#88571),(#88572,#88573),(#88574,#88575),(#88576,
#88577),(#88578,#88579),(#88580,#88581),(#88582,#88583),(#88584,#88585),
(#88586,#88587),(#88588,#88589),(#88590,#88591),(#88592,#88593),(#88594,
#88595),(#88596,#88597),(#88598,#88599),(#88600,#88601),(#88602,#88603),
(#88604,#88605),(#88606,#88607),(#88608,#88609),(#88610,#88611),(#88612,
#88613),(#88614,#88615),(#88616,#88617),(#88618,#88619),(#88620,#88621),
(#88622,#88623),(#88624,#88625),(#88626,#88627),(#88628,#88629),(#88630,
#88631),(#88632,#88633),(#88634,#88635),(#88636,#88637),(#88638,#88639),
(#88640,#88641),(#88642,#88643),(#88644,#88645),(#88646,#88647),(#88648,
#88649),(#88650,#88651),(#88652,#88653),(#88654,#88655),(#88656,#88657),
(#88658,#88659),(#88660,#88661),(#88662,#88663),(#88664,#88665),(#88666,
#88667),(#88668,#88669),(#88670,#88671),(#88672,#88673),(#88674,#88675),
(#88676,#88677),(#88678,#88679),(#88680,#88681),(#88682,#88683),(#88684,
#88685),(#88686,#88687),(#88688,#88689),(#88690,#88691),(#88692,#88693),
(#88694,#88695),(#88696,#88697),(#88698,#88699),(#88700,#88701),(#88702,
#88703),(#88704,#88705),(#88706,#88707),(#88708,#88709),(#88710,#88711),
(#88712,#88713),(#88714,#88715),(#88716,#88717),(#88718,#88719),(#88720,
#88721),(#88722,#88723),(#88724,#88725),(#88726,#88727),(#88728,#88729),
(#88730,#88731),(#88732,#88733),(#88734,#88735),(#88736,#88737),(#88738,
#88739),(#88740,#88741),(#88742,#88743),(#88744,#88745),(#88746,#88747),
(#88748,#88749),(#88750,#88751),(#88752,#88753),(#88754,#88755),(#88756,
#88757),(#88758,#88759),(#88760,#88761),(#88762,#88763),(#88764,#88765),
(#88766,#88767),(#88768,#88769),(#88770,#88771),(#88772,#88773),(#88774,
#88775),(#88776,#88777),(#88778,#88779),(#88780,#88781),(#88782,#88783),
(#88784,#88785),(#88786,#88787),(#88788,#88789),(#88790,#88791),(#88792,
#88793),(#88794,#88795),(#88796,#88797),(#88798,#88799),(#88800,#88801),
(#88802,#88803),(#88804,#88805),(#88806,#88807),(#88808,#88809),(#88810,
#88811),(#88812,#88813),(#88814,#88815),(#88816,#88817),(#88818,#88819),
(#88820,#88821),(#88822,#88823),(#88824,#88825),(#88826,#88827),(#88828,
#88829),(#88830,#88831),(#88832,#88833),(#88834,#88835),(#88836,#88837),
(#88838,#88839),(#88840,#88841),(#88842,#88843),(#88844,#88845),(#88846,
#88847),(#88848,#88849),(#88850,#88851),(#88852,#88853),(#88854,#88855),
(#88856,#88857),(#88858,#88859),(#88860,#88861),(#88862,#88863),(#88864,
#88865),(#88866,#88867),(#88868,#88869),(#88870,#88871)),.UNSPECIFIED.,
 .F.,.F.,.F.)
B_SPLINE_SURFACE_WITH_KNOTS((6,1,1,1,1,1,1,1,1,1,1,1,1,1,1,1,1,1,1,1,1,
1,1,1,1,1,1,1,1,1,1,1,1,1,1,1,1,1,1,1,1,1,1,1,1,1,1,1,1,1,1,1,1,1,1,1,1,
1,1,1,1,1,1,1,1,1,1,1,1,1,1,1,1,1,1,1,1,1,1,1,1,1,1,1,1,1,1,1,1,1,1,1,1,
1,1,1,1,1,1,1,1,1,1,1,1,1,1,1,1,1,1,1,1,1,1,1,1,1,1,1,1,1,1,1,1,1,1,1,1,
1,1,1,1,1,1,1,1,1,1,1,1,1,1,1,1,1,1,1,1,1,1,1,1,1,1,1,1,1,1,1,1,1,1,1,1,
1,1,1,1,1,1,1,1,1,1,1,1,1,1,1,1,1,1,1,1,1,1,1,1,1,1,1,1,1,1,1,1,1,1,1,6),
(2,2),(0.,0.005,0.01,0.015,0.02,0.025,0.03,0.035,0.04,0.045,0.05,0.055,
0.06,0.065,0.07,0.075,0.08,0.085,0.09,0.095,0.1,0.105,0.11,0.115,0.12,0.125,
0.13,0.135,0.14,0.145,0.15,0.155,0.16,0.165,0.17,0.175,0.18,0.185,0.19,
0.195,0.2,0.205,0.21,0.215,0.22,0.225,0.23,0.235,0.24,0.245,0.25,0.255,
0.26,0.265,0.27,0.275,0.28,0.285,0.29,0.295,0.3,0.305,0.31,0.315,0.32,0.325,
0.33,0.335,0.34,0.345,0.35,0.355,0.36,0.365,0.37,0.375,0.38,0.385,0.39,
0.395,0.4,0.405,0.41,0.415,0.42,0.425,0.43,0.435,0.44,0.445,0.45,0.455,
0.46,0.465,0.47,0.475,0.48,0.485,0.49,0.495,0.5,0.505,0.51,0.515,0.52,0.525,
0.53,0.535,0.54,0.545,0.55,0.555,0.56,0.565,0.57,0.575,0.58,0.585,0.59,
0.595,0.6,0.605,0.61,0.615,0.62,0.625,0.63,0.635,0.64,0.645,0.65,0.655,
0.66,0.665,0.67,0.675,0.68,0.685,0.690000000000001,0.695000000000001,0.700000000000001,
0.705000000000001,0.710000000000001,0.715000000000001,0.720000000000001,
0.725000000000001,0.730000000000001,0.735000000000001,0.740000000000001,
0.745000000000001,0.750000000000001,0.755000000000001,0.760000000000001,
0.765000000000001,0.770000000000001,0.775000000000001,0.780000000000001,
0.785000000000001,0.790000000000001,0.795000000000001,0.800000000000001,
0.805000000000001,0.810000000000001,0.815000000000001,0.820000000000001,
0.825000000000001,0.830000000000001,0.835000000000001,0.840000000000001,
0.845000000000001,0.850000000000001,0.855000000000001,0.860000000000001,
0.865000000000001,0.870000000000001,0.875000000000001,0.880000000000001,
0.885000000000001,0.890000000000001,0.895000000000001,0.900000000000001,
0.905000000000001,0.910000000000001,0.915000000000001,0.920000000000001,
0.925000000000001,0.930000000000001,0.935000000000001,0.940000000000001,
0.945000000000001,0.950000000000001,0.955000000000001,0.960000000000001,
0.965000000000001,0.970000000000001,0.975000000000001,0.980000000000001,
0.985000000000001,0.990000000000001,0.995000000000001,1.),(0.,1.2),
 .UNSPECIFIED.)
GEOMETRIC_REPRESENTATION_ITEM()
RATIONAL_B_SPLINE_SURFACE(((1.,1.),(1.,1.),(1.,1.),(1.,1.),(1.,1.),(1.,
1.),(1.,1.),(1.,1.),(1.,1.),(1.,1.),(1.,1.),(1.,1.),(1.,1.),(1.,1.),(1.,
1.),(1.,1.),(1.,1.),(1.,1.),(1.,1.),(1.,1.),(1.,1.),(1.,1.),(1.,1.),(1.,
1.),(1.,1.),(1.,1.),(1.,1.),(1.,1.),(1.,1.),(1.,1.),(1.,1.),(1.,1.),(1.,
1.),(1.,1.),(1.,1.),(1.,1.),(1.,1.),(1.,1.),(1.,1.),(1.,1.),(1.,1.),(1.,
1.),(1.,1.),(1.,1.),(1.,1.),(1.,1.),(1.,1.),(1.,1.),(1.,1.),(1.,1.),(1.,
1.),(1.,1.),(1.,1.),(1.,1.),(1.,1.),(1.,1.),(1.,1.),(1.,1.),(1.,1.),(1.,
1.),(1.,1.),(1.,1.),(1.,1.),(1.,1.),(1.,1.),(1.,1.),(1.,1.),(1.,1.),(1.,
1.),(1.,1.),(1.,1.),(1.,1.),(1.,1.),(1.,1.),(1.,1.),(1.,1.),(1.,1.),(1.,
1.),(1.,1.),(1.,1.),(1.,1.),(1.,1.),(1.,1.),(1.,1.),(1.,1.),(1.,1.),(1.,
1.),(1.,1.),(1.,1.),(1.,1.),(1.,1.),(1.,1.),(1.,1.),(1.,1.),(1.,1.),(1.,
1.),(1.,1.),(1.,1.),(1.,1.),(1.,1.),(1.,1.),(1.,1.),(1.,1.),(1.,1.),(1.,
1.),(1.,1.),(1.,1.),(1.,1.),(1.,1.),(1.,1.),(1.,1.),(1.,1.),(1.,1.),(1.,
1.),(1.,1.),(1.,1.),(1.,1.),(1.,1.),(1.,1.),(1.,1.),(1.,1.),(1.,1.),(1.,
1.),(1.,1.),(1.,1.),(1.,1.),(1.,1.),(1.,1.),(1.,1.),(1.,1.),(1.,1.),(1.,
1.),(1.,1.),(1.,1.),(1.,1.),(1.,1.),(1.,1.),(1.,1.),(1.,1.),(1.,1.),(1.,
1.),(1.,1.),(1.,1.),(1.,1.),(1.,1.),(1.,1.),(1.,1.),(1.,1.),(1.,1.),(1.,
1.),(1.,1.),(1.,1.),(1.,1.),(1.,1.),(1.,1.),(1.,1.),(1.,1.),(1.,1.),(1.,
1.),(1.,1.),(1.,1.),(1.,1.),(1.,1.),(1.,1.),(1.,1.),(1.,1.),(1.,1.),(1.,
1.),(1.,1.),(1.,1.),(1.,1.),(1.,1.),(1.,1.),(1.,1.),(1.,1.),(1.,1.),(1.,
1.),(1.,1.),(1.,1.),(1.,1.),(1.,1.),(1.,1.),(1.,1.),(1.,1.),(1.,1.),(1.,
1.),(1.,1.),(1.,1.),(1.,1.),(1.,1.),(1.,1.),(1.,1.),(1.,1.),(1.,1.),(1.,
1.),(1.,1.),(1.,1.),(1.,1.),(1.,1.),(1.,1.),(1.,1.),(1.,1.),(1.,1.),(1.,
1.),(1.,1.)))
REPRESENTATION_ITEM('')
SURFACE()
);
#924=(
BOUNDED_SURFACE()
B_SPLINE_SURFACE(5,1,((#89358,#89359),(#89360,#89361),(#89362,#89363),(#89364,
#89365),(#89366,#89367),(#89368,#89369),(#89370,#89371),(#89372,#89373),
(#89374,#89375),(#89376,#89377),(#89378,#89379),(#89380,#89381),(#89382,
#89383),(#89384,#89385),(#89386,#89387),(#89388,#89389),(#89390,#89391),
(#89392,#89393),(#89394,#89395),(#89396,#89397),(#89398,#89399),(#89400,
#89401),(#89402,#89403),(#89404,#89405),(#89406,#89407),(#89408,#89409),
(#89410,#89411),(#89412,#89413),(#89414,#89415),(#89416,#89417),(#89418,
#89419),(#89420,#89421),(#89422,#89423),(#89424,#89425),(#89426,#89427),
(#89428,#89429),(#89430,#89431),(#89432,#89433),(#89434,#89435),(#89436,
#89437),(#89438,#89439),(#89440,#89441),(#89442,#89443),(#89444,#89445),
(#89446,#89447),(#89448,#89449),(#89450,#89451),(#89452,#89453),(#89454,
#89455),(#89456,#89457),(#89458,#89459),(#89460,#89461),(#89462,#89463),
(#89464,#89465),(#89466,#89467),(#89468,#89469),(#89470,#89471),(#89472,
#89473),(#89474,#89475),(#89476,#89477),(#89478,#89479),(#89480,#89481),
(#89482,#89483),(#89484,#89485),(#89486,#89487),(#89488,#89489),(#89490,
#89491),(#89492,#89493),(#89494,#89495),(#89496,#89497),(#89498,#89499),
(#89500,#89501),(#89502,#89503),(#89504,#89505),(#89506,#89507),(#89508,
#89509),(#89510,#89511),(#89512,#89513),(#89514,#89515),(#89516,#89517),
(#89518,#89519),(#89520,#89521),(#89522,#89523),(#89524,#89525),(#89526,
#89527),(#89528,#89529),(#89530,#89531),(#89532,#89533),(#89534,#89535),
(#89536,#89537),(#89538,#89539),(#89540,#89541),(#89542,#89543),(#89544,
#89545),(#89546,#89547),(#89548,#89549),(#89550,#89551),(#89552,#89553),
(#89554,#89555),(#89556,#89557),(#89558,#89559),(#89560,#89561),(#89562,
#89563),(#89564,#89565),(#89566,#89567),(#89568,#89569),(#89570,#89571),
(#89572,#89573),(#89574,#89575),(#89576,#89577),(#89578,#89579),(#89580,
#89581),(#89582,#89583),(#89584,#89585),(#89586,#89587),(#89588,#89589),
(#89590,#89591),(#89592,#89593),(#89594,#89595),(#89596,#89597),(#89598,
#89599),(#89600,#89601),(#89602,#89603),(#89604,#89605),(#89606,#89607),
(#89608,#89609),(#89610,#89611),(#89612,#89613),(#89614,#89615),(#89616,
#89617),(#89618,#89619),(#89620,#89621),(#89622,#89623),(#89624,#89625),
(#89626,#89627),(#89628,#89629),(#89630,#89631),(#89632,#89633),(#89634,
#89635),(#89636,#89637),(#89638,#89639),(#89640,#89641),(#89642,#89643),
(#89644,#89645),(#89646,#89647),(#89648,#89649),(#89650,#89651),(#89652,
#89653),(#89654,#89655),(#89656,#89657),(#89658,#89659),(#89660,#89661),
(#89662,#89663),(#89664,#89665),(#89666,#89667),(#89668,#89669),(#89670,
#89671),(#89672,#89673),(#89674,#89675),(#89676,#89677),(#89678,#89679),
(#89680,#89681),(#89682,#89683),(#89684,#89685),(#89686,#89687),(#89688,
#89689),(#89690,#89691),(#89692,#89693),(#89694,#89695),(#89696,#89697),
(#89698,#89699),(#89700,#89701),(#89702,#89703),(#89704,#89705),(#89706,
#89707),(#89708,#89709),(#89710,#89711),(#89712,#89713),(#89714,#89715),
(#89716,#89717),(#89718,#89719),(#89720,#89721),(#89722,#89723),(#89724,
#89725),(#89726,#89727),(#89728,#89729),(#89730,#89731),(#89732,#89733),
(#89734,#89735),(#89736,#89737),(#89738,#89739),(#89740,#89741),(#89742,
#89743),(#89744,#89745),(#89746,#89747),(#89748,#89749),(#89750,#89751),
(#89752,#89753),(#89754,#89755),(#89756,#89757),(#89758,#89759),(#89760,
#89761),(#89762,#89763),(#89764,#89765),(#89766,#89767)),.UNSPECIFIED.,
 .F.,.F.,.F.)
B_SPLINE_SURFACE_WITH_KNOTS((6,1,1,1,1,1,1,1,1,1,1,1,1,1,1,1,1,1,1,1,1,
1,1,1,1,1,1,1,1,1,1,1,1,1,1,1,1,1,1,1,1,1,1,1,1,1,1,1,1,1,1,1,1,1,1,1,1,
1,1,1,1,1,1,1,1,1,1,1,1,1,1,1,1,1,1,1,1,1,1,1,1,1,1,1,1,1,1,1,1,1,1,1,1,
1,1,1,1,1,1,1,1,1,1,1,1,1,1,1,1,1,1,1,1,1,1,1,1,1,1,1,1,1,1,1,1,1,1,1,1,
1,1,1,1,1,1,1,1,1,1,1,1,1,1,1,1,1,1,1,1,1,1,1,1,1,1,1,1,1,1,1,1,1,1,1,1,
1,1,1,1,1,1,1,1,1,1,1,1,1,1,1,1,1,1,1,1,1,1,1,1,1,1,1,1,1,1,1,1,1,1,1,6),
(2,2),(0.,0.005,0.01,0.015,0.02,0.025,0.03,0.035,0.04,0.045,0.05,0.055,
0.06,0.065,0.07,0.075,0.08,0.085,0.09,0.095,0.1,0.105,0.11,0.115,0.12,0.125,
0.13,0.135,0.14,0.145,0.15,0.155,0.16,0.165,0.17,0.175,0.18,0.185,0.19,
0.195,0.2,0.205,0.21,0.215,0.22,0.225,0.23,0.235,0.24,0.245,0.25,0.255,
0.26,0.265,0.27,0.275,0.28,0.285,0.29,0.295,0.3,0.305,0.31,0.315,0.32,0.325,
0.33,0.335,0.34,0.345,0.35,0.355,0.36,0.365,0.37,0.375,0.38,0.385,0.39,
0.395,0.4,0.405,0.41,0.415,0.42,0.425,0.43,0.435,0.44,0.445,0.45,0.455,
0.46,0.465,0.47,0.475,0.48,0.485,0.49,0.495,0.5,0.505,0.51,0.515,0.52,0.525,
0.53,0.535,0.54,0.545,0.55,0.555,0.56,0.565,0.57,0.575,0.58,0.585,0.59,
0.595,0.6,0.605,0.61,0.615,0.62,0.625,0.63,0.635,0.64,0.645,0.65,0.655,
0.66,0.665,0.67,0.675,0.68,0.685,0.690000000000001,0.695000000000001,0.700000000000001,
0.705000000000001,0.710000000000001,0.715000000000001,0.720000000000001,
0.725000000000001,0.730000000000001,0.735000000000001,0.740000000000001,
0.745000000000001,0.750000000000001,0.755000000000001,0.760000000000001,
0.765000000000001,0.770000000000001,0.775000000000001,0.780000000000001,
0.785000000000001,0.790000000000001,0.795000000000001,0.800000000000001,
0.805000000000001,0.810000000000001,0.815000000000001,0.820000000000001,
0.825000000000001,0.830000000000001,0.835000000000001,0.840000000000001,
0.845000000000001,0.850000000000001,0.855000000000001,0.860000000000001,
0.865000000000001,0.870000000000001,0.875000000000001,0.880000000000001,
0.885000000000001,0.890000000000001,0.895000000000001,0.900000000000001,
0.905000000000001,0.910000000000001,0.915000000000001,0.920000000000001,
0.925000000000001,0.930000000000001,0.935000000000001,0.940000000000001,
0.945000000000001,0.950000000000001,0.955000000000001,0.960000000000001,
0.965000000000001,0.970000000000001,0.975000000000001,0.980000000000001,
0.985000000000001,0.990000000000001,0.995000000000001,1.),(0.,1.2),
 .UNSPECIFIED.)
GEOMETRIC_REPRESENTATION_ITEM()
RATIONAL_B_SPLINE_SURFACE(((1.,1.),(1.,1.),(1.,1.),(1.,1.),(1.,1.),(1.,
1.),(1.,1.),(1.,1.),(1.,1.),(1.,1.),(1.,1.),(1.,1.),(1.,1.),(1.,1.),(1.,
1.),(1.,1.),(1.,1.),(1.,1.),(1.,1.),(1.,1.),(1.,1.),(1.,1.),(1.,1.),(1.,
1.),(1.,1.),(1.,1.),(1.,1.),(1.,1.),(1.,1.),(1.,1.),(1.,1.),(1.,1.),(1.,
1.),(1.,1.),(1.,1.),(1.,1.),(1.,1.),(1.,1.),(1.,1.),(1.,1.),(1.,1.),(1.,
1.),(1.,1.),(1.,1.),(1.,1.),(1.,1.),(1.,1.),(1.,1.),(1.,1.),(1.,1.),(1.,
1.),(1.,1.),(1.,1.),(1.,1.),(1.,1.),(1.,1.),(1.,1.),(1.,1.),(1.,1.),(1.,
1.),(1.,1.),(1.,1.),(1.,1.),(1.,1.),(1.,1.),(1.,1.),(1.,1.),(1.,1.),(1.,
1.),(1.,1.),(1.,1.),(1.,1.),(1.,1.),(1.,1.),(1.,1.),(1.,1.),(1.,1.),(1.,
1.),(1.,1.),(1.,1.),(1.,1.),(1.,1.),(1.,1.),(1.,1.),(1.,1.),(1.,1.),(1.,
1.),(1.,1.),(1.,1.),(1.,1.),(1.,1.),(1.,1.),(1.,1.),(1.,1.),(1.,1.),(1.,
1.),(1.,1.),(1.,1.),(1.,1.),(1.,1.),(1.,1.),(1.,1.),(1.,1.),(1.,1.),(1.,
1.),(1.,1.),(1.,1.),(1.,1.),(1.,1.),(1.,1.),(1.,1.),(1.,1.),(1.,1.),(1.,
1.),(1.,1.),(1.,1.),(1.,1.),(1.,1.),(1.,1.),(1.,1.),(1.,1.),(1.,1.),(1.,
1.),(1.,1.),(1.,1.),(1.,1.),(1.,1.),(1.,1.),(1.,1.),(1.,1.),(1.,1.),(1.,
1.),(1.,1.),(1.,1.),(1.,1.),(1.,1.),(1.,1.),(1.,1.),(1.,1.),(1.,1.),(1.,
1.),(1.,1.),(1.,1.),(1.,1.),(1.,1.),(1.,1.),(1.,1.),(1.,1.),(1.,1.),(1.,
1.),(1.,1.),(1.,1.),(1.,1.),(1.,1.),(1.,1.),(1.,1.),(1.,1.),(1.,1.),(1.,
1.),(1.,1.),(1.,1.),(1.,1.),(1.,1.),(1.,1.),(1.,1.),(1.,1.),(1.,1.),(1.,
1.),(1.,1.),(1.,1.),(1.,1.),(1.,1.),(1.,1.),(1.,1.),(1.,1.),(1.,1.),(1.,
1.),(1.,1.),(1.,1.),(1.,1.),(1.,1.),(1.,1.),(1.,1.),(1.,1.),(1.,1.),(1.,
1.),(1.,1.),(1.,1.),(1.,1.),(1.,1.),(1.,1.),(1.,1.),(1.,1.),(1.,1.),(1.,
1.),(1.,1.),(1.,1.),(1.,1.),(1.,1.),(1.,1.),(1.,1.),(1.,1.),(1.,1.),(1.,
1.),(1.,1.)))
REPRESENTATION_ITEM('')
SURFACE()
);
#925=(
BOUNDED_SURFACE()
B_SPLINE_SURFACE(5,1,((#90254,#90255),(#90256,#90257),(#90258,#90259),(#90260,
#90261),(#90262,#90263),(#90264,#90265),(#90266,#90267),(#90268,#90269),
(#90270,#90271),(#90272,#90273),(#90274,#90275),(#90276,#90277),(#90278,
#90279),(#90280,#90281),(#90282,#90283),(#90284,#90285),(#90286,#90287),
(#90288,#90289),(#90290,#90291),(#90292,#90293),(#90294,#90295),(#90296,
#90297),(#90298,#90299),(#90300,#90301),(#90302,#90303),(#90304,#90305),
(#90306,#90307),(#90308,#90309),(#90310,#90311),(#90312,#90313),(#90314,
#90315),(#90316,#90317),(#90318,#90319),(#90320,#90321),(#90322,#90323),
(#90324,#90325),(#90326,#90327),(#90328,#90329),(#90330,#90331),(#90332,
#90333),(#90334,#90335),(#90336,#90337),(#90338,#90339),(#90340,#90341),
(#90342,#90343),(#90344,#90345),(#90346,#90347),(#90348,#90349),(#90350,
#90351),(#90352,#90353),(#90354,#90355),(#90356,#90357),(#90358,#90359),
(#90360,#90361),(#90362,#90363),(#90364,#90365),(#90366,#90367),(#90368,
#90369),(#90370,#90371),(#90372,#90373),(#90374,#90375),(#90376,#90377),
(#90378,#90379),(#90380,#90381),(#90382,#90383),(#90384,#90385),(#90386,
#90387),(#90388,#90389),(#90390,#90391),(#90392,#90393),(#90394,#90395),
(#90396,#90397),(#90398,#90399),(#90400,#90401),(#90402,#90403),(#90404,
#90405),(#90406,#90407),(#90408,#90409),(#90410,#90411),(#90412,#90413),
(#90414,#90415),(#90416,#90417),(#90418,#90419),(#90420,#90421),(#90422,
#90423),(#90424,#90425),(#90426,#90427),(#90428,#90429),(#90430,#90431),
(#90432,#90433),(#90434,#90435),(#90436,#90437),(#90438,#90439),(#90440,
#90441),(#90442,#90443),(#90444,#90445),(#90446,#90447),(#90448,#90449),
(#90450,#90451),(#90452,#90453),(#90454,#90455),(#90456,#90457),(#90458,
#90459),(#90460,#90461),(#90462,#90463),(#90464,#90465),(#90466,#90467),
(#90468,#90469),(#90470,#90471),(#90472,#90473),(#90474,#90475),(#90476,
#90477),(#90478,#90479),(#90480,#90481),(#90482,#90483),(#90484,#90485),
(#90486,#90487),(#90488,#90489),(#90490,#90491),(#90492,#90493),(#90494,
#90495),(#90496,#90497),(#90498,#90499),(#90500,#90501),(#90502,#90503),
(#90504,#90505),(#90506,#90507),(#90508,#90509),(#90510,#90511),(#90512,
#90513),(#90514,#90515),(#90516,#90517),(#90518,#90519),(#90520,#90521),
(#90522,#90523),(#90524,#90525),(#90526,#90527),(#90528,#90529),(#90530,
#90531),(#90532,#90533),(#90534,#90535),(#90536,#90537),(#90538,#90539),
(#90540,#90541),(#90542,#90543),(#90544,#90545),(#90546,#90547),(#90548,
#90549),(#90550,#90551),(#90552,#90553),(#90554,#90555),(#90556,#90557),
(#90558,#90559),(#90560,#90561),(#90562,#90563),(#90564,#90565),(#90566,
#90567),(#90568,#90569),(#90570,#90571),(#90572,#90573),(#90574,#90575),
(#90576,#90577),(#90578,#90579),(#90580,#90581),(#90582,#90583),(#90584,
#90585),(#90586,#90587),(#90588,#90589),(#90590,#90591),(#90592,#90593),
(#90594,#90595),(#90596,#90597),(#90598,#90599),(#90600,#90601),(#90602,
#90603),(#90604,#90605),(#90606,#90607),(#90608,#90609),(#90610,#90611),
(#90612,#90613),(#90614,#90615),(#90616,#90617),(#90618,#90619),(#90620,
#90621),(#90622,#90623),(#90624,#90625),(#90626,#90627),(#90628,#90629),
(#90630,#90631),(#90632,#90633),(#90634,#90635),(#90636,#90637),(#90638,
#90639),(#90640,#90641),(#90642,#90643),(#90644,#90645),(#90646,#90647),
(#90648,#90649),(#90650,#90651),(#90652,#90653),(#90654,#90655),(#90656,
#90657),(#90658,#90659),(#90660,#90661),(#90662,#90663)),.UNSPECIFIED.,
 .F.,.F.,.F.)
B_SPLINE_SURFACE_WITH_KNOTS((6,1,1,1,1,1,1,1,1,1,1,1,1,1,1,1,1,1,1,1,1,
1,1,1,1,1,1,1,1,1,1,1,1,1,1,1,1,1,1,1,1,1,1,1,1,1,1,1,1,1,1,1,1,1,1,1,1,
1,1,1,1,1,1,1,1,1,1,1,1,1,1,1,1,1,1,1,1,1,1,1,1,1,1,1,1,1,1,1,1,1,1,1,1,
1,1,1,1,1,1,1,1,1,1,1,1,1,1,1,1,1,1,1,1,1,1,1,1,1,1,1,1,1,1,1,1,1,1,1,1,
1,1,1,1,1,1,1,1,1,1,1,1,1,1,1,1,1,1,1,1,1,1,1,1,1,1,1,1,1,1,1,1,1,1,1,1,
1,1,1,1,1,1,1,1,1,1,1,1,1,1,1,1,1,1,1,1,1,1,1,1,1,1,1,1,1,1,1,1,1,1,1,6),
(2,2),(0.,0.005,0.01,0.015,0.02,0.025,0.03,0.035,0.04,0.045,0.05,0.055,
0.06,0.065,0.07,0.075,0.08,0.085,0.09,0.095,0.1,0.105,0.11,0.115,0.12,0.125,
0.13,0.135,0.14,0.145,0.15,0.155,0.16,0.165,0.17,0.175,0.18,0.185,0.19,
0.195,0.2,0.205,0.21,0.215,0.22,0.225,0.23,0.235,0.24,0.245,0.25,0.255,
0.26,0.265,0.27,0.275,0.28,0.285,0.29,0.295,0.3,0.305,0.31,0.315,0.32,0.325,
0.33,0.335,0.34,0.345,0.35,0.355,0.36,0.365,0.37,0.375,0.38,0.385,0.39,
0.395,0.4,0.405,0.41,0.415,0.42,0.425,0.43,0.435,0.44,0.445,0.45,0.455,
0.46,0.465,0.47,0.475,0.48,0.485,0.49,0.495,0.5,0.505,0.51,0.515,0.52,0.525,
0.53,0.535,0.54,0.545,0.55,0.555,0.56,0.565,0.57,0.575,0.58,0.585,0.59,
0.595,0.6,0.605,0.61,0.615,0.62,0.625,0.63,0.635,0.64,0.645,0.65,0.655,
0.66,0.665,0.67,0.675,0.68,0.685,0.690000000000001,0.695000000000001,0.700000000000001,
0.705000000000001,0.710000000000001,0.715000000000001,0.720000000000001,
0.725000000000001,0.730000000000001,0.735000000000001,0.740000000000001,
0.745000000000001,0.750000000000001,0.755000000000001,0.760000000000001,
0.765000000000001,0.770000000000001,0.775000000000001,0.780000000000001,
0.785000000000001,0.790000000000001,0.795000000000001,0.800000000000001,
0.805000000000001,0.810000000000001,0.815000000000001,0.820000000000001,
0.825000000000001,0.830000000000001,0.835000000000001,0.840000000000001,
0.845000000000001,0.850000000000001,0.855000000000001,0.860000000000001,
0.865000000000001,0.870000000000001,0.875000000000001,0.880000000000001,
0.885000000000001,0.890000000000001,0.895000000000001,0.900000000000001,
0.905000000000001,0.910000000000001,0.915000000000001,0.920000000000001,
0.925000000000001,0.930000000000001,0.935000000000001,0.940000000000001,
0.945000000000001,0.950000000000001,0.955000000000001,0.960000000000001,
0.965000000000001,0.970000000000001,0.975000000000001,0.980000000000001,
0.985000000000001,0.990000000000001,0.995000000000001,1.),(0.,1.2),
 .UNSPECIFIED.)
GEOMETRIC_REPRESENTATION_ITEM()
RATIONAL_B_SPLINE_SURFACE(((1.,1.),(1.,1.),(1.,1.),(1.,1.),(1.,1.),(1.,
1.),(1.,1.),(1.,1.),(1.,1.),(1.,1.),(1.,1.),(1.,1.),(1.,1.),(1.,1.),(1.,
1.),(1.,1.),(1.,1.),(1.,1.),(1.,1.),(1.,1.),(1.,1.),(1.,1.),(1.,1.),(1.,
1.),(1.,1.),(1.,1.),(1.,1.),(1.,1.),(1.,1.),(1.,1.),(1.,1.),(1.,1.),(1.,
1.),(1.,1.),(1.,1.),(1.,1.),(1.,1.),(1.,1.),(1.,1.),(1.,1.),(1.,1.),(1.,
1.),(1.,1.),(1.,1.),(1.,1.),(1.,1.),(1.,1.),(1.,1.),(1.,1.),(1.,1.),(1.,
1.),(1.,1.),(1.,1.),(1.,1.),(1.,1.),(1.,1.),(1.,1.),(1.,1.),(1.,1.),(1.,
1.),(1.,1.),(1.,1.),(1.,1.),(1.,1.),(1.,1.),(1.,1.),(1.,1.),(1.,1.),(1.,
1.),(1.,1.),(1.,1.),(1.,1.),(1.,1.),(1.,1.),(1.,1.),(1.,1.),(1.,1.),(1.,
1.),(1.,1.),(1.,1.),(1.,1.),(1.,1.),(1.,1.),(1.,1.),(1.,1.),(1.,1.),(1.,
1.),(1.,1.),(1.,1.),(1.,1.),(1.,1.),(1.,1.),(1.,1.),(1.,1.),(1.,1.),(1.,
1.),(1.,1.),(1.,1.),(1.,1.),(1.,1.),(1.,1.),(1.,1.),(1.,1.),(1.,1.),(1.,
1.),(1.,1.),(1.,1.),(1.,1.),(1.,1.),(1.,1.),(1.,1.),(1.,1.),(1.,1.),(1.,
1.),(1.,1.),(1.,1.),(1.,1.),(1.,1.),(1.,1.),(1.,1.),(1.,1.),(1.,1.),(1.,
1.),(1.,1.),(1.,1.),(1.,1.),(1.,1.),(1.,1.),(1.,1.),(1.,1.),(1.,1.),(1.,
1.),(1.,1.),(1.,1.),(1.,1.),(1.,1.),(1.,1.),(1.,1.),(1.,1.),(1.,1.),(1.,
1.),(1.,1.),(1.,1.),(1.,1.),(1.,1.),(1.,1.),(1.,1.),(1.,1.),(1.,1.),(1.,
1.),(1.,1.),(1.,1.),(1.,1.),(1.,1.),(1.,1.),(1.,1.),(1.,1.),(1.,1.),(1.,
1.),(1.,1.),(1.,1.),(1.,1.),(1.,1.),(1.,1.),(1.,1.),(1.,1.),(1.,1.),(1.,
1.),(1.,1.),(1.,1.),(1.,1.),(1.,1.),(1.,1.),(1.,1.),(1.,1.),(1.,1.),(1.,
1.),(1.,1.),(1.,1.),(1.,1.),(1.,1.),(1.,1.),(1.,1.),(1.,1.),(1.,1.),(1.,
1.),(1.,1.),(1.,1.),(1.,1.),(1.,1.),(1.,1.),(1.,1.),(1.,1.),(1.,1.),(1.,
1.),(1.,1.),(1.,1.),(1.,1.),(1.,1.),(1.,1.),(1.,1.),(1.,1.),(1.,1.),(1.,
1.),(1.,1.)))
REPRESENTATION_ITEM('')
SURFACE()
);
#926=(
BOUNDED_SURFACE()
B_SPLINE_SURFACE(5,1,((#91150,#91151),(#91152,#91153),(#91154,#91155),(#91156,
#91157),(#91158,#91159),(#91160,#91161),(#91162,#91163),(#91164,#91165),
(#91166,#91167),(#91168,#91169),(#91170,#91171),(#91172,#91173),(#91174,
#91175),(#91176,#91177),(#91178,#91179),(#91180,#91181),(#91182,#91183),
(#91184,#91185),(#91186,#91187),(#91188,#91189),(#91190,#91191),(#91192,
#91193),(#91194,#91195),(#91196,#91197),(#91198,#91199),(#91200,#91201),
(#91202,#91203),(#91204,#91205),(#91206,#91207),(#91208,#91209),(#91210,
#91211),(#91212,#91213),(#91214,#91215),(#91216,#91217),(#91218,#91219),
(#91220,#91221),(#91222,#91223),(#91224,#91225),(#91226,#91227),(#91228,
#91229),(#91230,#91231),(#91232,#91233),(#91234,#91235),(#91236,#91237),
(#91238,#91239),(#91240,#91241),(#91242,#91243),(#91244,#91245),(#91246,
#91247),(#91248,#91249),(#91250,#91251),(#91252,#91253),(#91254,#91255),
(#91256,#91257),(#91258,#91259),(#91260,#91261),(#91262,#91263),(#91264,
#91265),(#91266,#91267),(#91268,#91269),(#91270,#91271),(#91272,#91273),
(#91274,#91275),(#91276,#91277),(#91278,#91279),(#91280,#91281),(#91282,
#91283),(#91284,#91285),(#91286,#91287),(#91288,#91289),(#91290,#91291),
(#91292,#91293),(#91294,#91295),(#91296,#91297),(#91298,#91299),(#91300,
#91301),(#91302,#91303),(#91304,#91305),(#91306,#91307),(#91308,#91309),
(#91310,#91311),(#91312,#91313),(#91314,#91315),(#91316,#91317),(#91318,
#91319),(#91320,#91321),(#91322,#91323),(#91324,#91325),(#91326,#91327),
(#91328,#91329),(#91330,#91331),(#91332,#91333),(#91334,#91335),(#91336,
#91337),(#91338,#91339),(#91340,#91341),(#91342,#91343),(#91344,#91345),
(#91346,#91347),(#91348,#91349),(#91350,#91351),(#91352,#91353),(#91354,
#91355),(#91356,#91357),(#91358,#91359),(#91360,#91361),(#91362,#91363),
(#91364,#91365),(#91366,#91367),(#91368,#91369),(#91370,#91371),(#91372,
#91373),(#91374,#91375),(#91376,#91377),(#91378,#91379),(#91380,#91381),
(#91382,#91383),(#91384,#91385),(#91386,#91387),(#91388,#91389),(#91390,
#91391),(#91392,#91393),(#91394,#91395),(#91396,#91397),(#91398,#91399),
(#91400,#91401),(#91402,#91403),(#91404,#91405),(#91406,#91407),(#91408,
#91409),(#91410,#91411),(#91412,#91413),(#91414,#91415),(#91416,#91417),
(#91418,#91419),(#91420,#91421),(#91422,#91423),(#91424,#91425),(#91426,
#91427),(#91428,#91429),(#91430,#91431),(#91432,#91433),(#91434,#91435),
(#91436,#91437),(#91438,#91439),(#91440,#91441),(#91442,#91443),(#91444,
#91445),(#91446,#91447),(#91448,#91449),(#91450,#91451),(#91452,#91453),
(#91454,#91455),(#91456,#91457),(#91458,#91459),(#91460,#91461),(#91462,
#91463),(#91464,#91465),(#91466,#91467),(#91468,#91469),(#91470,#91471),
(#91472,#91473),(#91474,#91475),(#91476,#91477),(#91478,#91479),(#91480,
#91481),(#91482,#91483),(#91484,#91485),(#91486,#91487),(#91488,#91489),
(#91490,#91491),(#91492,#91493),(#91494,#91495),(#91496,#91497),(#91498,
#91499),(#91500,#91501),(#91502,#91503),(#91504,#91505),(#91506,#91507),
(#91508,#91509),(#91510,#91511),(#91512,#91513),(#91514,#91515),(#91516,
#91517),(#91518,#91519),(#91520,#91521),(#91522,#91523),(#91524,#91525),
(#91526,#91527),(#91528,#91529),(#91530,#91531),(#91532,#91533),(#91534,
#91535),(#91536,#91537),(#91538,#91539),(#91540,#91541),(#91542,#91543),
(#91544,#91545),(#91546,#91547),(#91548,#91549),(#91550,#91551),(#91552,
#91553),(#91554,#91555),(#91556,#91557),(#91558,#91559)),.UNSPECIFIED.,
 .F.,.F.,.F.)
B_SPLINE_SURFACE_WITH_KNOTS((6,1,1,1,1,1,1,1,1,1,1,1,1,1,1,1,1,1,1,1,1,
1,1,1,1,1,1,1,1,1,1,1,1,1,1,1,1,1,1,1,1,1,1,1,1,1,1,1,1,1,1,1,1,1,1,1,1,
1,1,1,1,1,1,1,1,1,1,1,1,1,1,1,1,1,1,1,1,1,1,1,1,1,1,1,1,1,1,1,1,1,1,1,1,
1,1,1,1,1,1,1,1,1,1,1,1,1,1,1,1,1,1,1,1,1,1,1,1,1,1,1,1,1,1,1,1,1,1,1,1,
1,1,1,1,1,1,1,1,1,1,1,1,1,1,1,1,1,1,1,1,1,1,1,1,1,1,1,1,1,1,1,1,1,1,1,1,
1,1,1,1,1,1,1,1,1,1,1,1,1,1,1,1,1,1,1,1,1,1,1,1,1,1,1,1,1,1,1,1,1,1,1,6),
(2,2),(0.,0.005,0.01,0.015,0.02,0.025,0.03,0.035,0.04,0.045,0.05,0.055,
0.06,0.065,0.07,0.075,0.08,0.085,0.09,0.095,0.1,0.105,0.11,0.115,0.12,0.125,
0.13,0.135,0.14,0.145,0.15,0.155,0.16,0.165,0.17,0.175,0.18,0.185,0.19,
0.195,0.2,0.205,0.21,0.215,0.22,0.225,0.23,0.235,0.24,0.245,0.25,0.255,
0.26,0.265,0.27,0.275,0.28,0.285,0.29,0.295,0.3,0.305,0.31,0.315,0.32,0.325,
0.33,0.335,0.34,0.345,0.35,0.355,0.36,0.365,0.37,0.375,0.38,0.385,0.39,
0.395,0.4,0.405,0.41,0.415,0.42,0.425,0.43,0.435,0.44,0.445,0.45,0.455,
0.46,0.465,0.47,0.475,0.48,0.485,0.49,0.495,0.5,0.505,0.51,0.515,0.52,0.525,
0.53,0.535,0.54,0.545,0.55,0.555,0.56,0.565,0.57,0.575,0.58,0.585,0.59,
0.595,0.6,0.605,0.61,0.615,0.62,0.625,0.63,0.635,0.64,0.645,0.65,0.655,
0.66,0.665,0.67,0.675,0.68,0.685,0.690000000000001,0.695000000000001,0.700000000000001,
0.705000000000001,0.710000000000001,0.715000000000001,0.720000000000001,
0.725000000000001,0.730000000000001,0.735000000000001,0.740000000000001,
0.745000000000001,0.750000000000001,0.755000000000001,0.760000000000001,
0.765000000000001,0.770000000000001,0.775000000000001,0.780000000000001,
0.785000000000001,0.790000000000001,0.795000000000001,0.800000000000001,
0.805000000000001,0.810000000000001,0.815000000000001,0.820000000000001,
0.825000000000001,0.830000000000001,0.835000000000001,0.840000000000001,
0.845000000000001,0.850000000000001,0.855000000000001,0.860000000000001,
0.865000000000001,0.870000000000001,0.875000000000001,0.880000000000001,
0.885000000000001,0.890000000000001,0.895000000000001,0.900000000000001,
0.905000000000001,0.910000000000001,0.915000000000001,0.920000000000001,
0.925000000000001,0.930000000000001,0.935000000000001,0.940000000000001,
0.945000000000001,0.950000000000001,0.955000000000001,0.960000000000001,
0.965000000000001,0.970000000000001,0.975000000000001,0.980000000000001,
0.985000000000001,0.990000000000001,0.995000000000001,1.),(0.,1.2),
 .UNSPECIFIED.)
GEOMETRIC_REPRESENTATION_ITEM()
RATIONAL_B_SPLINE_SURFACE(((1.,1.),(1.,1.),(1.,1.),(1.,1.),(1.,1.),(1.,
1.),(1.,1.),(1.,1.),(1.,1.),(1.,1.),(1.,1.),(1.,1.),(1.,1.),(1.,1.),(1.,
1.),(1.,1.),(1.,1.),(1.,1.),(1.,1.),(1.,1.),(1.,1.),(1.,1.),(1.,1.),(1.,
1.),(1.,1.),(1.,1.),(1.,1.),(1.,1.),(1.,1.),(1.,1.),(1.,1.),(1.,1.),(1.,
1.),(1.,1.),(1.,1.),(1.,1.),(1.,1.),(1.,1.),(1.,1.),(1.,1.),(1.,1.),(1.,
1.),(1.,1.),(1.,1.),(1.,1.),(1.,1.),(1.,1.),(1.,1.),(1.,1.),(1.,1.),(1.,
1.),(1.,1.),(1.,1.),(1.,1.),(1.,1.),(1.,1.),(1.,1.),(1.,1.),(1.,1.),(1.,
1.),(1.,1.),(1.,1.),(1.,1.),(1.,1.),(1.,1.),(1.,1.),(1.,1.),(1.,1.),(1.,
1.),(1.,1.),(1.,1.),(1.,1.),(1.,1.),(1.,1.),(1.,1.),(1.,1.),(1.,1.),(1.,
1.),(1.,1.),(1.,1.),(1.,1.),(1.,1.),(1.,1.),(1.,1.),(1.,1.),(1.,1.),(1.,
1.),(1.,1.),(1.,1.),(1.,1.),(1.,1.),(1.,1.),(1.,1.),(1.,1.),(1.,1.),(1.,
1.),(1.,1.),(1.,1.),(1.,1.),(1.,1.),(1.,1.),(1.,1.),(1.,1.),(1.,1.),(1.,
1.),(1.,1.),(1.,1.),(1.,1.),(1.,1.),(1.,1.),(1.,1.),(1.,1.),(1.,1.),(1.,
1.),(1.,1.),(1.,1.),(1.,1.),(1.,1.),(1.,1.),(1.,1.),(1.,1.),(1.,1.),(1.,
1.),(1.,1.),(1.,1.),(1.,1.),(1.,1.),(1.,1.),(1.,1.),(1.,1.),(1.,1.),(1.,
1.),(1.,1.),(1.,1.),(1.,1.),(1.,1.),(1.,1.),(1.,1.),(1.,1.),(1.,1.),(1.,
1.),(1.,1.),(1.,1.),(1.,1.),(1.,1.),(1.,1.),(1.,1.),(1.,1.),(1.,1.),(1.,
1.),(1.,1.),(1.,1.),(1.,1.),(1.,1.),(1.,1.),(1.,1.),(1.,1.),(1.,1.),(1.,
1.),(1.,1.),(1.,1.),(1.,1.),(1.,1.),(1.,1.),(1.,1.),(1.,1.),(1.,1.),(1.,
1.),(1.,1.),(1.,1.),(1.,1.),(1.,1.),(1.,1.),(1.,1.),(1.,1.),(1.,1.),(1.,
1.),(1.,1.),(1.,1.),(1.,1.),(1.,1.),(1.,1.),(1.,1.),(1.,1.),(1.,1.),(1.,
1.),(1.,1.),(1.,1.),(1.,1.),(1.,1.),(1.,1.),(1.,1.),(1.,1.),(1.,1.),(1.,
1.),(1.,1.),(1.,1.),(1.,1.),(1.,1.),(1.,1.),(1.,1.),(1.,1.),(1.,1.),(1.,
1.),(1.,1.)))
REPRESENTATION_ITEM('')
SURFACE()
);
#927=(
BOUNDED_SURFACE()
B_SPLINE_SURFACE(5,1,((#92046,#92047),(#92048,#92049),(#92050,#92051),(#92052,
#92053),(#92054,#92055),(#92056,#92057),(#92058,#92059),(#92060,#92061),
(#92062,#92063),(#92064,#92065),(#92066,#92067),(#92068,#92069),(#92070,
#92071),(#92072,#92073),(#92074,#92075),(#92076,#92077),(#92078,#92079),
(#92080,#92081),(#92082,#92083),(#92084,#92085),(#92086,#92087),(#92088,
#92089),(#92090,#92091),(#92092,#92093),(#92094,#92095),(#92096,#92097),
(#92098,#92099),(#92100,#92101),(#92102,#92103),(#92104,#92105),(#92106,
#92107),(#92108,#92109),(#92110,#92111),(#92112,#92113),(#92114,#92115),
(#92116,#92117),(#92118,#92119),(#92120,#92121),(#92122,#92123),(#92124,
#92125),(#92126,#92127),(#92128,#92129),(#92130,#92131),(#92132,#92133),
(#92134,#92135),(#92136,#92137),(#92138,#92139),(#92140,#92141),(#92142,
#92143),(#92144,#92145),(#92146,#92147),(#92148,#92149),(#92150,#92151),
(#92152,#92153),(#92154,#92155),(#92156,#92157),(#92158,#92159),(#92160,
#92161),(#92162,#92163),(#92164,#92165),(#92166,#92167),(#92168,#92169),
(#92170,#92171),(#92172,#92173),(#92174,#92175),(#92176,#92177),(#92178,
#92179),(#92180,#92181),(#92182,#92183),(#92184,#92185),(#92186,#92187),
(#92188,#92189),(#92190,#92191),(#92192,#92193),(#92194,#92195),(#92196,
#92197),(#92198,#92199),(#92200,#92201),(#92202,#92203),(#92204,#92205),
(#92206,#92207),(#92208,#92209),(#92210,#92211),(#92212,#92213),(#92214,
#92215),(#92216,#92217),(#92218,#92219),(#92220,#92221),(#92222,#92223),
(#92224,#92225),(#92226,#92227),(#92228,#92229),(#92230,#92231),(#92232,
#92233),(#92234,#92235),(#92236,#92237),(#92238,#92239),(#92240,#92241),
(#92242,#92243),(#92244,#92245),(#92246,#92247),(#92248,#92249),(#92250,
#92251),(#92252,#92253),(#92254,#92255),(#92256,#92257),(#92258,#92259),
(#92260,#92261),(#92262,#92263),(#92264,#92265),(#92266,#92267),(#92268,
#92269),(#92270,#92271),(#92272,#92273),(#92274,#92275),(#92276,#92277),
(#92278,#92279),(#92280,#92281),(#92282,#92283),(#92284,#92285),(#92286,
#92287),(#92288,#92289),(#92290,#92291),(#92292,#92293),(#92294,#92295),
(#92296,#92297),(#92298,#92299),(#92300,#92301),(#92302,#92303),(#92304,
#92305),(#92306,#92307),(#92308,#92309),(#92310,#92311),(#92312,#92313),
(#92314,#92315),(#92316,#92317),(#92318,#92319),(#92320,#92321),(#92322,
#92323),(#92324,#92325),(#92326,#92327),(#92328,#92329),(#92330,#92331),
(#92332,#92333),(#92334,#92335),(#92336,#92337),(#92338,#92339),(#92340,
#92341),(#92342,#92343),(#92344,#92345),(#92346,#92347),(#92348,#92349),
(#92350,#92351),(#92352,#92353),(#92354,#92355),(#92356,#92357),(#92358,
#92359),(#92360,#92361),(#92362,#92363),(#92364,#92365),(#92366,#92367),
(#92368,#92369),(#92370,#92371),(#92372,#92373),(#92374,#92375),(#92376,
#92377),(#92378,#92379),(#92380,#92381),(#92382,#92383),(#92384,#92385),
(#92386,#92387),(#92388,#92389),(#92390,#92391),(#92392,#92393),(#92394,
#92395),(#92396,#92397),(#92398,#92399),(#92400,#92401),(#92402,#92403),
(#92404,#92405),(#92406,#92407),(#92408,#92409),(#92410,#92411),(#92412,
#92413),(#92414,#92415),(#92416,#92417),(#92418,#92419),(#92420,#92421),
(#92422,#92423),(#92424,#92425),(#92426,#92427),(#92428,#92429),(#92430,
#92431),(#92432,#92433),(#92434,#92435),(#92436,#92437),(#92438,#92439),
(#92440,#92441),(#92442,#92443),(#92444,#92445),(#92446,#92447),(#92448,
#92449),(#92450,#92451),(#92452,#92453),(#92454,#92455)),.UNSPECIFIED.,
 .F.,.F.,.F.)
B_SPLINE_SURFACE_WITH_KNOTS((6,1,1,1,1,1,1,1,1,1,1,1,1,1,1,1,1,1,1,1,1,
1,1,1,1,1,1,1,1,1,1,1,1,1,1,1,1,1,1,1,1,1,1,1,1,1,1,1,1,1,1,1,1,1,1,1,1,
1,1,1,1,1,1,1,1,1,1,1,1,1,1,1,1,1,1,1,1,1,1,1,1,1,1,1,1,1,1,1,1,1,1,1,1,
1,1,1,1,1,1,1,1,1,1,1,1,1,1,1,1,1,1,1,1,1,1,1,1,1,1,1,1,1,1,1,1,1,1,1,1,
1,1,1,1,1,1,1,1,1,1,1,1,1,1,1,1,1,1,1,1,1,1,1,1,1,1,1,1,1,1,1,1,1,1,1,1,
1,1,1,1,1,1,1,1,1,1,1,1,1,1,1,1,1,1,1,1,1,1,1,1,1,1,1,1,1,1,1,1,1,1,1,6),
(2,2),(0.,0.005,0.01,0.015,0.02,0.025,0.03,0.035,0.04,0.045,0.05,0.055,
0.06,0.065,0.07,0.075,0.08,0.085,0.09,0.095,0.1,0.105,0.11,0.115,0.12,0.125,
0.13,0.135,0.14,0.145,0.15,0.155,0.16,0.165,0.17,0.175,0.18,0.185,0.19,
0.195,0.2,0.205,0.21,0.215,0.22,0.225,0.23,0.235,0.24,0.245,0.25,0.255,
0.26,0.265,0.27,0.275,0.28,0.285,0.29,0.295,0.3,0.305,0.31,0.315,0.32,0.325,
0.33,0.335,0.34,0.345,0.35,0.355,0.36,0.365,0.37,0.375,0.38,0.385,0.39,
0.395,0.4,0.405,0.41,0.415,0.42,0.425,0.43,0.435,0.44,0.445,0.45,0.455,
0.46,0.465,0.47,0.475,0.48,0.485,0.49,0.495,0.5,0.505,0.51,0.515,0.52,0.525,
0.53,0.535,0.54,0.545,0.55,0.555,0.56,0.565,0.57,0.575,0.58,0.585,0.59,
0.595,0.6,0.605,0.61,0.615,0.62,0.625,0.63,0.635,0.64,0.645,0.65,0.655,
0.66,0.665,0.67,0.675,0.68,0.685,0.690000000000001,0.695000000000001,0.700000000000001,
0.705000000000001,0.710000000000001,0.715000000000001,0.720000000000001,
0.725000000000001,0.730000000000001,0.735000000000001,0.740000000000001,
0.745000000000001,0.750000000000001,0.755000000000001,0.760000000000001,
0.765000000000001,0.770000000000001,0.775000000000001,0.780000000000001,
0.785000000000001,0.790000000000001,0.795000000000001,0.800000000000001,
0.805000000000001,0.810000000000001,0.815000000000001,0.820000000000001,
0.825000000000001,0.830000000000001,0.835000000000001,0.840000000000001,
0.845000000000001,0.850000000000001,0.855000000000001,0.860000000000001,
0.865000000000001,0.870000000000001,0.875000000000001,0.880000000000001,
0.885000000000001,0.890000000000001,0.895000000000001,0.900000000000001,
0.905000000000001,0.910000000000001,0.915000000000001,0.920000000000001,
0.925000000000001,0.930000000000001,0.935000000000001,0.940000000000001,
0.945000000000001,0.950000000000001,0.955000000000001,0.960000000000001,
0.965000000000001,0.970000000000001,0.975000000000001,0.980000000000001,
0.985000000000001,0.990000000000001,0.995000000000001,1.),(0.,1.2),
 .UNSPECIFIED.)
GEOMETRIC_REPRESENTATION_ITEM()
RATIONAL_B_SPLINE_SURFACE(((1.,1.),(1.,1.),(1.,1.),(1.,1.),(1.,1.),(1.,
1.),(1.,1.),(1.,1.),(1.,1.),(1.,1.),(1.,1.),(1.,1.),(1.,1.),(1.,1.),(1.,
1.),(1.,1.),(1.,1.),(1.,1.),(1.,1.),(1.,1.),(1.,1.),(1.,1.),(1.,1.),(1.,
1.),(1.,1.),(1.,1.),(1.,1.),(1.,1.),(1.,1.),(1.,1.),(1.,1.),(1.,1.),(1.,
1.),(1.,1.),(1.,1.),(1.,1.),(1.,1.),(1.,1.),(1.,1.),(1.,1.),(1.,1.),(1.,
1.),(1.,1.),(1.,1.),(1.,1.),(1.,1.),(1.,1.),(1.,1.),(1.,1.),(1.,1.),(1.,
1.),(1.,1.),(1.,1.),(1.,1.),(1.,1.),(1.,1.),(1.,1.),(1.,1.),(1.,1.),(1.,
1.),(1.,1.),(1.,1.),(1.,1.),(1.,1.),(1.,1.),(1.,1.),(1.,1.),(1.,1.),(1.,
1.),(1.,1.),(1.,1.),(1.,1.),(1.,1.),(1.,1.),(1.,1.),(1.,1.),(1.,1.),(1.,
1.),(1.,1.),(1.,1.),(1.,1.),(1.,1.),(1.,1.),(1.,1.),(1.,1.),(1.,1.),(1.,
1.),(1.,1.),(1.,1.),(1.,1.),(1.,1.),(1.,1.),(1.,1.),(1.,1.),(1.,1.),(1.,
1.),(1.,1.),(1.,1.),(1.,1.),(1.,1.),(1.,1.),(1.,1.),(1.,1.),(1.,1.),(1.,
1.),(1.,1.),(1.,1.),(1.,1.),(1.,1.),(1.,1.),(1.,1.),(1.,1.),(1.,1.),(1.,
1.),(1.,1.),(1.,1.),(1.,1.),(1.,1.),(1.,1.),(1.,1.),(1.,1.),(1.,1.),(1.,
1.),(1.,1.),(1.,1.),(1.,1.),(1.,1.),(1.,1.),(1.,1.),(1.,1.),(1.,1.),(1.,
1.),(1.,1.),(1.,1.),(1.,1.),(1.,1.),(1.,1.),(1.,1.),(1.,1.),(1.,1.),(1.,
1.),(1.,1.),(1.,1.),(1.,1.),(1.,1.),(1.,1.),(1.,1.),(1.,1.),(1.,1.),(1.,
1.),(1.,1.),(1.,1.),(1.,1.),(1.,1.),(1.,1.),(1.,1.),(1.,1.),(1.,1.),(1.,
1.),(1.,1.),(1.,1.),(1.,1.),(1.,1.),(1.,1.),(1.,1.),(1.,1.),(1.,1.),(1.,
1.),(1.,1.),(1.,1.),(1.,1.),(1.,1.),(1.,1.),(1.,1.),(1.,1.),(1.,1.),(1.,
1.),(1.,1.),(1.,1.),(1.,1.),(1.,1.),(1.,1.),(1.,1.),(1.,1.),(1.,1.),(1.,
1.),(1.,1.),(1.,1.),(1.,1.),(1.,1.),(1.,1.),(1.,1.),(1.,1.),(1.,1.),(1.,
1.),(1.,1.),(1.,1.),(1.,1.),(1.,1.),(1.,1.),(1.,1.),(1.,1.),(1.,1.),(1.,
1.),(1.,1.)))
REPRESENTATION_ITEM('')
SURFACE()
);
#928=(
BOUNDED_SURFACE()
B_SPLINE_SURFACE(5,1,((#92942,#92943),(#92944,#92945),(#92946,#92947),(#92948,
#92949),(#92950,#92951),(#92952,#92953),(#92954,#92955),(#92956,#92957),
(#92958,#92959),(#92960,#92961),(#92962,#92963),(#92964,#92965),(#92966,
#92967),(#92968,#92969),(#92970,#92971),(#92972,#92973),(#92974,#92975),
(#92976,#92977),(#92978,#92979),(#92980,#92981),(#92982,#92983),(#92984,
#92985),(#92986,#92987),(#92988,#92989),(#92990,#92991),(#92992,#92993),
(#92994,#92995),(#92996,#92997),(#92998,#92999),(#93000,#93001),(#93002,
#93003),(#93004,#93005),(#93006,#93007),(#93008,#93009),(#93010,#93011),
(#93012,#93013),(#93014,#93015),(#93016,#93017),(#93018,#93019),(#93020,
#93021),(#93022,#93023),(#93024,#93025),(#93026,#93027),(#93028,#93029),
(#93030,#93031),(#93032,#93033),(#93034,#93035),(#93036,#93037),(#93038,
#93039),(#93040,#93041),(#93042,#93043),(#93044,#93045),(#93046,#93047),
(#93048,#93049),(#93050,#93051),(#93052,#93053),(#93054,#93055),(#93056,
#93057),(#93058,#93059),(#93060,#93061),(#93062,#93063),(#93064,#93065),
(#93066,#93067),(#93068,#93069),(#93070,#93071),(#93072,#93073),(#93074,
#93075),(#93076,#93077),(#93078,#93079),(#93080,#93081),(#93082,#93083),
(#93084,#93085),(#93086,#93087),(#93088,#93089),(#93090,#93091),(#93092,
#93093),(#93094,#93095),(#93096,#93097),(#93098,#93099),(#93100,#93101),
(#93102,#93103),(#93104,#93105),(#93106,#93107),(#93108,#93109),(#93110,
#93111),(#93112,#93113),(#93114,#93115),(#93116,#93117),(#93118,#93119),
(#93120,#93121),(#93122,#93123),(#93124,#93125),(#93126,#93127),(#93128,
#93129),(#93130,#93131),(#93132,#93133),(#93134,#93135),(#93136,#93137),
(#93138,#93139),(#93140,#93141),(#93142,#93143),(#93144,#93145),(#93146,
#93147),(#93148,#93149),(#93150,#93151),(#93152,#93153),(#93154,#93155),
(#93156,#93157),(#93158,#93159),(#93160,#93161),(#93162,#93163),(#93164,
#93165),(#93166,#93167),(#93168,#93169),(#93170,#93171),(#93172,#93173),
(#93174,#93175),(#93176,#93177),(#93178,#93179),(#93180,#93181),(#93182,
#93183),(#93184,#93185),(#93186,#93187),(#93188,#93189),(#93190,#93191),
(#93192,#93193),(#93194,#93195),(#93196,#93197),(#93198,#93199),(#93200,
#93201),(#93202,#93203),(#93204,#93205),(#93206,#93207),(#93208,#93209),
(#93210,#93211),(#93212,#93213),(#93214,#93215),(#93216,#93217),(#93218,
#93219),(#93220,#93221),(#93222,#93223),(#93224,#93225),(#93226,#93227),
(#93228,#93229),(#93230,#93231),(#93232,#93233),(#93234,#93235),(#93236,
#93237),(#93238,#93239),(#93240,#93241),(#93242,#93243),(#93244,#93245),
(#93246,#93247),(#93248,#93249),(#93250,#93251),(#93252,#93253),(#93254,
#93255),(#93256,#93257),(#93258,#93259),(#93260,#93261),(#93262,#93263),
(#93264,#93265),(#93266,#93267),(#93268,#93269),(#93270,#93271),(#93272,
#93273),(#93274,#93275),(#93276,#93277),(#93278,#93279),(#93280,#93281),
(#93282,#93283),(#93284,#93285),(#93286,#93287),(#93288,#93289),(#93290,
#93291),(#93292,#93293),(#93294,#93295),(#93296,#93297),(#93298,#93299),
(#93300,#93301),(#93302,#93303),(#93304,#93305),(#93306,#93307),(#93308,
#93309),(#93310,#93311),(#93312,#93313),(#93314,#93315),(#93316,#93317),
(#93318,#93319),(#93320,#93321),(#93322,#93323),(#93324,#93325),(#93326,
#93327),(#93328,#93329),(#93330,#93331),(#93332,#93333),(#93334,#93335),
(#93336,#93337),(#93338,#93339),(#93340,#93341),(#93342,#93343),(#93344,
#93345),(#93346,#93347),(#93348,#93349),(#93350,#93351)),.UNSPECIFIED.,
 .F.,.F.,.F.)
B_SPLINE_SURFACE_WITH_KNOTS((6,1,1,1,1,1,1,1,1,1,1,1,1,1,1,1,1,1,1,1,1,
1,1,1,1,1,1,1,1,1,1,1,1,1,1,1,1,1,1,1,1,1,1,1,1,1,1,1,1,1,1,1,1,1,1,1,1,
1,1,1,1,1,1,1,1,1,1,1,1,1,1,1,1,1,1,1,1,1,1,1,1,1,1,1,1,1,1,1,1,1,1,1,1,
1,1,1,1,1,1,1,1,1,1,1,1,1,1,1,1,1,1,1,1,1,1,1,1,1,1,1,1,1,1,1,1,1,1,1,1,
1,1,1,1,1,1,1,1,1,1,1,1,1,1,1,1,1,1,1,1,1,1,1,1,1,1,1,1,1,1,1,1,1,1,1,1,
1,1,1,1,1,1,1,1,1,1,1,1,1,1,1,1,1,1,1,1,1,1,1,1,1,1,1,1,1,1,1,1,1,1,1,6),
(2,2),(0.,0.005,0.01,0.015,0.02,0.025,0.03,0.035,0.04,0.045,0.05,0.055,
0.06,0.065,0.07,0.075,0.08,0.085,0.09,0.095,0.1,0.105,0.11,0.115,0.12,0.125,
0.13,0.135,0.14,0.145,0.15,0.155,0.16,0.165,0.17,0.175,0.18,0.185,0.19,
0.195,0.2,0.205,0.21,0.215,0.22,0.225,0.23,0.235,0.24,0.245,0.25,0.255,
0.26,0.265,0.27,0.275,0.28,0.285,0.29,0.295,0.3,0.305,0.31,0.315,0.32,0.325,
0.33,0.335,0.34,0.345,0.35,0.355,0.36,0.365,0.37,0.375,0.38,0.385,0.39,
0.395,0.4,0.405,0.41,0.415,0.42,0.425,0.43,0.435,0.44,0.445,0.45,0.455,
0.46,0.465,0.47,0.475,0.48,0.485,0.49,0.495,0.5,0.505,0.51,0.515,0.52,0.525,
0.53,0.535,0.54,0.545,0.55,0.555,0.56,0.565,0.57,0.575,0.58,0.585,0.59,
0.595,0.6,0.605,0.61,0.615,0.62,0.625,0.63,0.635,0.64,0.645,0.65,0.655,
0.66,0.665,0.67,0.675,0.68,0.685,0.690000000000001,0.695000000000001,0.700000000000001,
0.705000000000001,0.710000000000001,0.715000000000001,0.720000000000001,
0.725000000000001,0.730000000000001,0.735000000000001,0.740000000000001,
0.745000000000001,0.750000000000001,0.755000000000001,0.760000000000001,
0.765000000000001,0.770000000000001,0.775000000000001,0.780000000000001,
0.785000000000001,0.790000000000001,0.795000000000001,0.800000000000001,
0.805000000000001,0.810000000000001,0.815000000000001,0.820000000000001,
0.825000000000001,0.830000000000001,0.835000000000001,0.840000000000001,
0.845000000000001,0.850000000000001,0.855000000000001,0.860000000000001,
0.865000000000001,0.870000000000001,0.875000000000001,0.880000000000001,
0.885000000000001,0.890000000000001,0.895000000000001,0.900000000000001,
0.905000000000001,0.910000000000001,0.915000000000001,0.920000000000001,
0.925000000000001,0.930000000000001,0.935000000000001,0.940000000000001,
0.945000000000001,0.950000000000001,0.955000000000001,0.960000000000001,
0.965000000000001,0.970000000000001,0.975000000000001,0.980000000000001,
0.985000000000001,0.990000000000001,0.995000000000001,1.),(0.,1.2),
 .UNSPECIFIED.)
GEOMETRIC_REPRESENTATION_ITEM()
RATIONAL_B_SPLINE_SURFACE(((1.,1.),(1.,1.),(1.,1.),(1.,1.),(1.,1.),(1.,
1.),(1.,1.),(1.,1.),(1.,1.),(1.,1.),(1.,1.),(1.,1.),(1.,1.),(1.,1.),(1.,
1.),(1.,1.),(1.,1.),(1.,1.),(1.,1.),(1.,1.),(1.,1.),(1.,1.),(1.,1.),(1.,
1.),(1.,1.),(1.,1.),(1.,1.),(1.,1.),(1.,1.),(1.,1.),(1.,1.),(1.,1.),(1.,
1.),(1.,1.),(1.,1.),(1.,1.),(1.,1.),(1.,1.),(1.,1.),(1.,1.),(1.,1.),(1.,
1.),(1.,1.),(1.,1.),(1.,1.),(1.,1.),(1.,1.),(1.,1.),(1.,1.),(1.,1.),(1.,
1.),(1.,1.),(1.,1.),(1.,1.),(1.,1.),(1.,1.),(1.,1.),(1.,1.),(1.,1.),(1.,
1.),(1.,1.),(1.,1.),(1.,1.),(1.,1.),(1.,1.),(1.,1.),(1.,1.),(1.,1.),(1.,
1.),(1.,1.),(1.,1.),(1.,1.),(1.,1.),(1.,1.),(1.,1.),(1.,1.),(1.,1.),(1.,
1.),(1.,1.),(1.,1.),(1.,1.),(1.,1.),(1.,1.),(1.,1.),(1.,1.),(1.,1.),(1.,
1.),(1.,1.),(1.,1.),(1.,1.),(1.,1.),(1.,1.),(1.,1.),(1.,1.),(1.,1.),(1.,
1.),(1.,1.),(1.,1.),(1.,1.),(1.,1.),(1.,1.),(1.,1.),(1.,1.),(1.,1.),(1.,
1.),(1.,1.),(1.,1.),(1.,1.),(1.,1.),(1.,1.),(1.,1.),(1.,1.),(1.,1.),(1.,
1.),(1.,1.),(1.,1.),(1.,1.),(1.,1.),(1.,1.),(1.,1.),(1.,1.),(1.,1.),(1.,
1.),(1.,1.),(1.,1.),(1.,1.),(1.,1.),(1.,1.),(1.,1.),(1.,1.),(1.,1.),(1.,
1.),(1.,1.),(1.,1.),(1.,1.),(1.,1.),(1.,1.),(1.,1.),(1.,1.),(1.,1.),(1.,
1.),(1.,1.),(1.,1.),(1.,1.),(1.,1.),(1.,1.),(1.,1.),(1.,1.),(1.,1.),(1.,
1.),(1.,1.),(1.,1.),(1.,1.),(1.,1.),(1.,1.),(1.,1.),(1.,1.),(1.,1.),(1.,
1.),(1.,1.),(1.,1.),(1.,1.),(1.,1.),(1.,1.),(1.,1.),(1.,1.),(1.,1.),(1.,
1.),(1.,1.),(1.,1.),(1.,1.),(1.,1.),(1.,1.),(1.,1.),(1.,1.),(1.,1.),(1.,
1.),(1.,1.),(1.,1.),(1.,1.),(1.,1.),(1.,1.),(1.,1.),(1.,1.),(1.,1.),(1.,
1.),(1.,1.),(1.,1.),(1.,1.),(1.,1.),(1.,1.),(1.,1.),(1.,1.),(1.,1.),(1.,
1.),(1.,1.),(1.,1.),(1.,1.),(1.,1.),(1.,1.),(1.,1.),(1.,1.),(1.,1.),(1.,
1.),(1.,1.)))
REPRESENTATION_ITEM('')
SURFACE()
);
#929=(
BOUNDED_SURFACE()
B_SPLINE_SURFACE(5,1,((#93838,#93839),(#93840,#93841),(#93842,#93843),(#93844,
#93845),(#93846,#93847),(#93848,#93849),(#93850,#93851),(#93852,#93853),
(#93854,#93855),(#93856,#93857),(#93858,#93859),(#93860,#93861),(#93862,
#93863),(#93864,#93865),(#93866,#93867),(#93868,#93869),(#93870,#93871),
(#93872,#93873),(#93874,#93875),(#93876,#93877),(#93878,#93879),(#93880,
#93881),(#93882,#93883),(#93884,#93885),(#93886,#93887),(#93888,#93889),
(#93890,#93891),(#93892,#93893),(#93894,#93895),(#93896,#93897),(#93898,
#93899),(#93900,#93901),(#93902,#93903),(#93904,#93905),(#93906,#93907),
(#93908,#93909),(#93910,#93911),(#93912,#93913),(#93914,#93915),(#93916,
#93917),(#93918,#93919),(#93920,#93921),(#93922,#93923),(#93924,#93925),
(#93926,#93927),(#93928,#93929),(#93930,#93931),(#93932,#93933),(#93934,
#93935),(#93936,#93937),(#93938,#93939),(#93940,#93941),(#93942,#93943),
(#93944,#93945),(#93946,#93947),(#93948,#93949),(#93950,#93951),(#93952,
#93953),(#93954,#93955),(#93956,#93957),(#93958,#93959),(#93960,#93961),
(#93962,#93963),(#93964,#93965),(#93966,#93967),(#93968,#93969),(#93970,
#93971),(#93972,#93973),(#93974,#93975),(#93976,#93977),(#93978,#93979),
(#93980,#93981),(#93982,#93983),(#93984,#93985),(#93986,#93987),(#93988,
#93989),(#93990,#93991),(#93992,#93993),(#93994,#93995),(#93996,#93997),
(#93998,#93999),(#94000,#94001),(#94002,#94003),(#94004,#94005),(#94006,
#94007),(#94008,#94009),(#94010,#94011),(#94012,#94013),(#94014,#94015),
(#94016,#94017),(#94018,#94019),(#94020,#94021),(#94022,#94023),(#94024,
#94025),(#94026,#94027),(#94028,#94029),(#94030,#94031),(#94032,#94033),
(#94034,#94035),(#94036,#94037),(#94038,#94039),(#94040,#94041),(#94042,
#94043),(#94044,#94045),(#94046,#94047),(#94048,#94049),(#94050,#94051),
(#94052,#94053),(#94054,#94055),(#94056,#94057),(#94058,#94059),(#94060,
#94061),(#94062,#94063),(#94064,#94065),(#94066,#94067),(#94068,#94069),
(#94070,#94071),(#94072,#94073),(#94074,#94075),(#94076,#94077),(#94078,
#94079),(#94080,#94081),(#94082,#94083),(#94084,#94085),(#94086,#94087),
(#94088,#94089),(#94090,#94091),(#94092,#94093),(#94094,#94095),(#94096,
#94097),(#94098,#94099),(#94100,#94101),(#94102,#94103),(#94104,#94105),
(#94106,#94107),(#94108,#94109),(#94110,#94111),(#94112,#94113),(#94114,
#94115),(#94116,#94117),(#94118,#94119),(#94120,#94121),(#94122,#94123),
(#94124,#94125),(#94126,#94127),(#94128,#94129),(#94130,#94131),(#94132,
#94133),(#94134,#94135),(#94136,#94137),(#94138,#94139),(#94140,#94141),
(#94142,#94143),(#94144,#94145),(#94146,#94147),(#94148,#94149),(#94150,
#94151),(#94152,#94153),(#94154,#94155),(#94156,#94157),(#94158,#94159),
(#94160,#94161),(#94162,#94163),(#94164,#94165),(#94166,#94167),(#94168,
#94169),(#94170,#94171),(#94172,#94173),(#94174,#94175),(#94176,#94177),
(#94178,#94179),(#94180,#94181),(#94182,#94183),(#94184,#94185),(#94186,
#94187),(#94188,#94189),(#94190,#94191),(#94192,#94193),(#94194,#94195),
(#94196,#94197),(#94198,#94199),(#94200,#94201),(#94202,#94203),(#94204,
#94205),(#94206,#94207),(#94208,#94209),(#94210,#94211),(#94212,#94213),
(#94214,#94215),(#94216,#94217),(#94218,#94219),(#94220,#94221),(#94222,
#94223),(#94224,#94225),(#94226,#94227),(#94228,#94229),(#94230,#94231),
(#94232,#94233),(#94234,#94235),(#94236,#94237),(#94238,#94239),(#94240,
#94241),(#94242,#94243),(#94244,#94245),(#94246,#94247)),.UNSPECIFIED.,
 .F.,.F.,.F.)
B_SPLINE_SURFACE_WITH_KNOTS((6,1,1,1,1,1,1,1,1,1,1,1,1,1,1,1,1,1,1,1,1,
1,1,1,1,1,1,1,1,1,1,1,1,1,1,1,1,1,1,1,1,1,1,1,1,1,1,1,1,1,1,1,1,1,1,1,1,
1,1,1,1,1,1,1,1,1,1,1,1,1,1,1,1,1,1,1,1,1,1,1,1,1,1,1,1,1,1,1,1,1,1,1,1,
1,1,1,1,1,1,1,1,1,1,1,1,1,1,1,1,1,1,1,1,1,1,1,1,1,1,1,1,1,1,1,1,1,1,1,1,
1,1,1,1,1,1,1,1,1,1,1,1,1,1,1,1,1,1,1,1,1,1,1,1,1,1,1,1,1,1,1,1,1,1,1,1,
1,1,1,1,1,1,1,1,1,1,1,1,1,1,1,1,1,1,1,1,1,1,1,1,1,1,1,1,1,1,1,1,1,1,1,6),
(2,2),(0.,0.005,0.01,0.015,0.02,0.025,0.03,0.035,0.04,0.045,0.05,0.055,
0.06,0.065,0.07,0.075,0.08,0.085,0.09,0.095,0.1,0.105,0.11,0.115,0.12,0.125,
0.13,0.135,0.14,0.145,0.15,0.155,0.16,0.165,0.17,0.175,0.18,0.185,0.19,
0.195,0.2,0.205,0.21,0.215,0.22,0.225,0.23,0.235,0.24,0.245,0.25,0.255,
0.26,0.265,0.27,0.275,0.28,0.285,0.29,0.295,0.3,0.305,0.31,0.315,0.32,0.325,
0.33,0.335,0.34,0.345,0.35,0.355,0.36,0.365,0.37,0.375,0.38,0.385,0.39,
0.395,0.4,0.405,0.41,0.415,0.42,0.425,0.43,0.435,0.44,0.445,0.45,0.455,
0.46,0.465,0.47,0.475,0.48,0.485,0.49,0.495,0.5,0.505,0.51,0.515,0.52,0.525,
0.53,0.535,0.54,0.545,0.55,0.555,0.56,0.565,0.57,0.575,0.58,0.585,0.59,
0.595,0.6,0.605,0.61,0.615,0.62,0.625,0.63,0.635,0.64,0.645,0.65,0.655,
0.66,0.665,0.67,0.675,0.68,0.685,0.690000000000001,0.695000000000001,0.700000000000001,
0.705000000000001,0.710000000000001,0.715000000000001,0.720000000000001,
0.725000000000001,0.730000000000001,0.735000000000001,0.740000000000001,
0.745000000000001,0.750000000000001,0.755000000000001,0.760000000000001,
0.765000000000001,0.770000000000001,0.775000000000001,0.780000000000001,
0.785000000000001,0.790000000000001,0.795000000000001,0.800000000000001,
0.805000000000001,0.810000000000001,0.815000000000001,0.820000000000001,
0.825000000000001,0.830000000000001,0.835000000000001,0.840000000000001,
0.845000000000001,0.850000000000001,0.855000000000001,0.860000000000001,
0.865000000000001,0.870000000000001,0.875000000000001,0.880000000000001,
0.885000000000001,0.890000000000001,0.895000000000001,0.900000000000001,
0.905000000000001,0.910000000000001,0.915000000000001,0.920000000000001,
0.925000000000001,0.930000000000001,0.935000000000001,0.940000000000001,
0.945000000000001,0.950000000000001,0.955000000000001,0.960000000000001,
0.965000000000001,0.970000000000001,0.975000000000001,0.980000000000001,
0.985000000000001,0.990000000000001,0.995000000000001,1.),(0.,1.2),
 .UNSPECIFIED.)
GEOMETRIC_REPRESENTATION_ITEM()
RATIONAL_B_SPLINE_SURFACE(((1.,1.),(1.,1.),(1.,1.),(1.,1.),(1.,1.),(1.,
1.),(1.,1.),(1.,1.),(1.,1.),(1.,1.),(1.,1.),(1.,1.),(1.,1.),(1.,1.),(1.,
1.),(1.,1.),(1.,1.),(1.,1.),(1.,1.),(1.,1.),(1.,1.),(1.,1.),(1.,1.),(1.,
1.),(1.,1.),(1.,1.),(1.,1.),(1.,1.),(1.,1.),(1.,1.),(1.,1.),(1.,1.),(1.,
1.),(1.,1.),(1.,1.),(1.,1.),(1.,1.),(1.,1.),(1.,1.),(1.,1.),(1.,1.),(1.,
1.),(1.,1.),(1.,1.),(1.,1.),(1.,1.),(1.,1.),(1.,1.),(1.,1.),(1.,1.),(1.,
1.),(1.,1.),(1.,1.),(1.,1.),(1.,1.),(1.,1.),(1.,1.),(1.,1.),(1.,1.),(1.,
1.),(1.,1.),(1.,1.),(1.,1.),(1.,1.),(1.,1.),(1.,1.),(1.,1.),(1.,1.),(1.,
1.),(1.,1.),(1.,1.),(1.,1.),(1.,1.),(1.,1.),(1.,1.),(1.,1.),(1.,1.),(1.,
1.),(1.,1.),(1.,1.),(1.,1.),(1.,1.),(1.,1.),(1.,1.),(1.,1.),(1.,1.),(1.,
1.),(1.,1.),(1.,1.),(1.,1.),(1.,1.),(1.,1.),(1.,1.),(1.,1.),(1.,1.),(1.,
1.),(1.,1.),(1.,1.),(1.,1.),(1.,1.),(1.,1.),(1.,1.),(1.,1.),(1.,1.),(1.,
1.),(1.,1.),(1.,1.),(1.,1.),(1.,1.),(1.,1.),(1.,1.),(1.,1.),(1.,1.),(1.,
1.),(1.,1.),(1.,1.),(1.,1.),(1.,1.),(1.,1.),(1.,1.),(1.,1.),(1.,1.),(1.,
1.),(1.,1.),(1.,1.),(1.,1.),(1.,1.),(1.,1.),(1.,1.),(1.,1.),(1.,1.),(1.,
1.),(1.,1.),(1.,1.),(1.,1.),(1.,1.),(1.,1.),(1.,1.),(1.,1.),(1.,1.),(1.,
1.),(1.,1.),(1.,1.),(1.,1.),(1.,1.),(1.,1.),(1.,1.),(1.,1.),(1.,1.),(1.,
1.),(1.,1.),(1.,1.),(1.,1.),(1.,1.),(1.,1.),(1.,1.),(1.,1.),(1.,1.),(1.,
1.),(1.,1.),(1.,1.),(1.,1.),(1.,1.),(1.,1.),(1.,1.),(1.,1.),(1.,1.),(1.,
1.),(1.,1.),(1.,1.),(1.,1.),(1.,1.),(1.,1.),(1.,1.),(1.,1.),(1.,1.),(1.,
1.),(1.,1.),(1.,1.),(1.,1.),(1.,1.),(1.,1.),(1.,1.),(1.,1.),(1.,1.),(1.,
1.),(1.,1.),(1.,1.),(1.,1.),(1.,1.),(1.,1.),(1.,1.),(1.,1.),(1.,1.),(1.,
1.),(1.,1.),(1.,1.),(1.,1.),(1.,1.),(1.,1.),(1.,1.),(1.,1.),(1.,1.),(1.,
1.),(1.,1.)))
REPRESENTATION_ITEM('')
SURFACE()
);
#930=(
BOUNDED_SURFACE()
B_SPLINE_SURFACE(5,1,((#94734,#94735),(#94736,#94737),(#94738,#94739),(#94740,
#94741),(#94742,#94743),(#94744,#94745),(#94746,#94747),(#94748,#94749),
(#94750,#94751),(#94752,#94753),(#94754,#94755),(#94756,#94757),(#94758,
#94759),(#94760,#94761),(#94762,#94763),(#94764,#94765),(#94766,#94767),
(#94768,#94769),(#94770,#94771),(#94772,#94773),(#94774,#94775),(#94776,
#94777),(#94778,#94779),(#94780,#94781),(#94782,#94783),(#94784,#94785),
(#94786,#94787),(#94788,#94789),(#94790,#94791),(#94792,#94793),(#94794,
#94795),(#94796,#94797),(#94798,#94799),(#94800,#94801),(#94802,#94803),
(#94804,#94805),(#94806,#94807),(#94808,#94809),(#94810,#94811),(#94812,
#94813),(#94814,#94815),(#94816,#94817),(#94818,#94819),(#94820,#94821),
(#94822,#94823),(#94824,#94825),(#94826,#94827),(#94828,#94829),(#94830,
#94831),(#94832,#94833),(#94834,#94835),(#94836,#94837),(#94838,#94839),
(#94840,#94841),(#94842,#94843),(#94844,#94845),(#94846,#94847),(#94848,
#94849),(#94850,#94851),(#94852,#94853),(#94854,#94855),(#94856,#94857),
(#94858,#94859),(#94860,#94861),(#94862,#94863),(#94864,#94865),(#94866,
#94867),(#94868,#94869),(#94870,#94871),(#94872,#94873),(#94874,#94875),
(#94876,#94877),(#94878,#94879),(#94880,#94881),(#94882,#94883),(#94884,
#94885),(#94886,#94887),(#94888,#94889),(#94890,#94891),(#94892,#94893),
(#94894,#94895),(#94896,#94897),(#94898,#94899),(#94900,#94901),(#94902,
#94903),(#94904,#94905),(#94906,#94907),(#94908,#94909),(#94910,#94911),
(#94912,#94913),(#94914,#94915),(#94916,#94917),(#94918,#94919),(#94920,
#94921),(#94922,#94923),(#94924,#94925),(#94926,#94927),(#94928,#94929),
(#94930,#94931),(#94932,#94933),(#94934,#94935),(#94936,#94937),(#94938,
#94939),(#94940,#94941),(#94942,#94943),(#94944,#94945),(#94946,#94947),
(#94948,#94949),(#94950,#94951),(#94952,#94953),(#94954,#94955),(#94956,
#94957),(#94958,#94959),(#94960,#94961),(#94962,#94963),(#94964,#94965),
(#94966,#94967),(#94968,#94969),(#94970,#94971),(#94972,#94973),(#94974,
#94975),(#94976,#94977),(#94978,#94979),(#94980,#94981),(#94982,#94983),
(#94984,#94985),(#94986,#94987),(#94988,#94989),(#94990,#94991),(#94992,
#94993),(#94994,#94995),(#94996,#94997),(#94998,#94999),(#95000,#95001),
(#95002,#95003),(#95004,#95005),(#95006,#95007),(#95008,#95009),(#95010,
#95011),(#95012,#95013),(#95014,#95015),(#95016,#95017),(#95018,#95019),
(#95020,#95021),(#95022,#95023),(#95024,#95025),(#95026,#95027),(#95028,
#95029),(#95030,#95031),(#95032,#95033),(#95034,#95035),(#95036,#95037),
(#95038,#95039),(#95040,#95041),(#95042,#95043),(#95044,#95045),(#95046,
#95047),(#95048,#95049),(#95050,#95051),(#95052,#95053),(#95054,#95055),
(#95056,#95057),(#95058,#95059),(#95060,#95061),(#95062,#95063),(#95064,
#95065),(#95066,#95067),(#95068,#95069),(#95070,#95071),(#95072,#95073),
(#95074,#95075),(#95076,#95077),(#95078,#95079),(#95080,#95081),(#95082,
#95083),(#95084,#95085),(#95086,#95087),(#95088,#95089),(#95090,#95091),
(#95092,#95093),(#95094,#95095),(#95096,#95097),(#95098,#95099),(#95100,
#95101),(#95102,#95103),(#95104,#95105),(#95106,#95107),(#95108,#95109),
(#95110,#95111),(#95112,#95113),(#95114,#95115),(#95116,#95117),(#95118,
#95119),(#95120,#95121),(#95122,#95123),(#95124,#95125),(#95126,#95127),
(#95128,#95129),(#95130,#95131),(#95132,#95133),(#95134,#95135),(#95136,
#95137),(#95138,#95139),(#95140,#95141),(#95142,#95143)),.UNSPECIFIED.,
 .F.,.F.,.F.)
B_SPLINE_SURFACE_WITH_KNOTS((6,1,1,1,1,1,1,1,1,1,1,1,1,1,1,1,1,1,1,1,1,
1,1,1,1,1,1,1,1,1,1,1,1,1,1,1,1,1,1,1,1,1,1,1,1,1,1,1,1,1,1,1,1,1,1,1,1,
1,1,1,1,1,1,1,1,1,1,1,1,1,1,1,1,1,1,1,1,1,1,1,1,1,1,1,1,1,1,1,1,1,1,1,1,
1,1,1,1,1,1,1,1,1,1,1,1,1,1,1,1,1,1,1,1,1,1,1,1,1,1,1,1,1,1,1,1,1,1,1,1,
1,1,1,1,1,1,1,1,1,1,1,1,1,1,1,1,1,1,1,1,1,1,1,1,1,1,1,1,1,1,1,1,1,1,1,1,
1,1,1,1,1,1,1,1,1,1,1,1,1,1,1,1,1,1,1,1,1,1,1,1,1,1,1,1,1,1,1,1,1,1,1,6),
(2,2),(0.,0.005,0.01,0.015,0.02,0.025,0.03,0.035,0.04,0.045,0.05,0.055,
0.06,0.065,0.07,0.075,0.08,0.085,0.09,0.095,0.1,0.105,0.11,0.115,0.12,0.125,
0.13,0.135,0.14,0.145,0.15,0.155,0.16,0.165,0.17,0.175,0.18,0.185,0.19,
0.195,0.2,0.205,0.21,0.215,0.22,0.225,0.23,0.235,0.24,0.245,0.25,0.255,
0.26,0.265,0.27,0.275,0.28,0.285,0.29,0.295,0.3,0.305,0.31,0.315,0.32,0.325,
0.33,0.335,0.34,0.345,0.35,0.355,0.36,0.365,0.37,0.375,0.38,0.385,0.39,
0.395,0.4,0.405,0.41,0.415,0.42,0.425,0.43,0.435,0.44,0.445,0.45,0.455,
0.46,0.465,0.47,0.475,0.48,0.485,0.49,0.495,0.5,0.505,0.51,0.515,0.52,0.525,
0.53,0.535,0.54,0.545,0.55,0.555,0.56,0.565,0.57,0.575,0.58,0.585,0.59,
0.595,0.6,0.605,0.61,0.615,0.62,0.625,0.63,0.635,0.64,0.645,0.65,0.655,
0.66,0.665,0.67,0.675,0.68,0.685,0.690000000000001,0.695000000000001,0.700000000000001,
0.705000000000001,0.710000000000001,0.715000000000001,0.720000000000001,
0.725000000000001,0.730000000000001,0.735000000000001,0.740000000000001,
0.745000000000001,0.750000000000001,0.755000000000001,0.760000000000001,
0.765000000000001,0.770000000000001,0.775000000000001,0.780000000000001,
0.785000000000001,0.790000000000001,0.795000000000001,0.800000000000001,
0.805000000000001,0.810000000000001,0.815000000000001,0.820000000000001,
0.825000000000001,0.830000000000001,0.835000000000001,0.840000000000001,
0.845000000000001,0.850000000000001,0.855000000000001,0.860000000000001,
0.865000000000001,0.870000000000001,0.875000000000001,0.880000000000001,
0.885000000000001,0.890000000000001,0.895000000000001,0.900000000000001,
0.905000000000001,0.910000000000001,0.915000000000001,0.920000000000001,
0.925000000000001,0.930000000000001,0.935000000000001,0.940000000000001,
0.945000000000001,0.950000000000001,0.955000000000001,0.960000000000001,
0.965000000000001,0.970000000000001,0.975000000000001,0.980000000000001,
0.985000000000001,0.990000000000001,0.995000000000001,1.),(0.,1.2),
 .UNSPECIFIED.)
GEOMETRIC_REPRESENTATION_ITEM()
RATIONAL_B_SPLINE_SURFACE(((1.,1.),(1.,1.),(1.,1.),(1.,1.),(1.,1.),(1.,
1.),(1.,1.),(1.,1.),(1.,1.),(1.,1.),(1.,1.),(1.,1.),(1.,1.),(1.,1.),(1.,
1.),(1.,1.),(1.,1.),(1.,1.),(1.,1.),(1.,1.),(1.,1.),(1.,1.),(1.,1.),(1.,
1.),(1.,1.),(1.,1.),(1.,1.),(1.,1.),(1.,1.),(1.,1.),(1.,1.),(1.,1.),(1.,
1.),(1.,1.),(1.,1.),(1.,1.),(1.,1.),(1.,1.),(1.,1.),(1.,1.),(1.,1.),(1.,
1.),(1.,1.),(1.,1.),(1.,1.),(1.,1.),(1.,1.),(1.,1.),(1.,1.),(1.,1.),(1.,
1.),(1.,1.),(1.,1.),(1.,1.),(1.,1.),(1.,1.),(1.,1.),(1.,1.),(1.,1.),(1.,
1.),(1.,1.),(1.,1.),(1.,1.),(1.,1.),(1.,1.),(1.,1.),(1.,1.),(1.,1.),(1.,
1.),(1.,1.),(1.,1.),(1.,1.),(1.,1.),(1.,1.),(1.,1.),(1.,1.),(1.,1.),(1.,
1.),(1.,1.),(1.,1.),(1.,1.),(1.,1.),(1.,1.),(1.,1.),(1.,1.),(1.,1.),(1.,
1.),(1.,1.),(1.,1.),(1.,1.),(1.,1.),(1.,1.),(1.,1.),(1.,1.),(1.,1.),(1.,
1.),(1.,1.),(1.,1.),(1.,1.),(1.,1.),(1.,1.),(1.,1.),(1.,1.),(1.,1.),(1.,
1.),(1.,1.),(1.,1.),(1.,1.),(1.,1.),(1.,1.),(1.,1.),(1.,1.),(1.,1.),(1.,
1.),(1.,1.),(1.,1.),(1.,1.),(1.,1.),(1.,1.),(1.,1.),(1.,1.),(1.,1.),(1.,
1.),(1.,1.),(1.,1.),(1.,1.),(1.,1.),(1.,1.),(1.,1.),(1.,1.),(1.,1.),(1.,
1.),(1.,1.),(1.,1.),(1.,1.),(1.,1.),(1.,1.),(1.,1.),(1.,1.),(1.,1.),(1.,
1.),(1.,1.),(1.,1.),(1.,1.),(1.,1.),(1.,1.),(1.,1.),(1.,1.),(1.,1.),(1.,
1.),(1.,1.),(1.,1.),(1.,1.),(1.,1.),(1.,1.),(1.,1.),(1.,1.),(1.,1.),(1.,
1.),(1.,1.),(1.,1.),(1.,1.),(1.,1.),(1.,1.),(1.,1.),(1.,1.),(1.,1.),(1.,
1.),(1.,1.),(1.,1.),(1.,1.),(1.,1.),(1.,1.),(1.,1.),(1.,1.),(1.,1.),(1.,
1.),(1.,1.),(1.,1.),(1.,1.),(1.,1.),(1.,1.),(1.,1.),(1.,1.),(1.,1.),(1.,
1.),(1.,1.),(1.,1.),(1.,1.),(1.,1.),(1.,1.),(1.,1.),(1.,1.),(1.,1.),(1.,
1.),(1.,1.),(1.,1.),(1.,1.),(1.,1.),(1.,1.),(1.,1.),(1.,1.),(1.,1.),(1.,
1.),(1.,1.)))
REPRESENTATION_ITEM('')
SURFACE()
);
#931=(
BOUNDED_SURFACE()
B_SPLINE_SURFACE(5,1,((#95630,#95631),(#95632,#95633),(#95634,#95635),(#95636,
#95637),(#95638,#95639),(#95640,#95641),(#95642,#95643),(#95644,#95645),
(#95646,#95647),(#95648,#95649),(#95650,#95651),(#95652,#95653),(#95654,
#95655),(#95656,#95657),(#95658,#95659),(#95660,#95661),(#95662,#95663),
(#95664,#95665),(#95666,#95667),(#95668,#95669),(#95670,#95671),(#95672,
#95673),(#95674,#95675),(#95676,#95677),(#95678,#95679),(#95680,#95681),
(#95682,#95683),(#95684,#95685),(#95686,#95687),(#95688,#95689),(#95690,
#95691),(#95692,#95693),(#95694,#95695),(#95696,#95697),(#95698,#95699),
(#95700,#95701),(#95702,#95703),(#95704,#95705),(#95706,#95707),(#95708,
#95709),(#95710,#95711),(#95712,#95713),(#95714,#95715),(#95716,#95717),
(#95718,#95719),(#95720,#95721),(#95722,#95723),(#95724,#95725),(#95726,
#95727),(#95728,#95729),(#95730,#95731),(#95732,#95733),(#95734,#95735),
(#95736,#95737),(#95738,#95739),(#95740,#95741),(#95742,#95743),(#95744,
#95745),(#95746,#95747),(#95748,#95749),(#95750,#95751),(#95752,#95753),
(#95754,#95755),(#95756,#95757),(#95758,#95759),(#95760,#95761),(#95762,
#95763),(#95764,#95765),(#95766,#95767),(#95768,#95769),(#95770,#95771),
(#95772,#95773),(#95774,#95775),(#95776,#95777),(#95778,#95779),(#95780,
#95781),(#95782,#95783),(#95784,#95785),(#95786,#95787),(#95788,#95789),
(#95790,#95791),(#95792,#95793),(#95794,#95795),(#95796,#95797),(#95798,
#95799),(#95800,#95801),(#95802,#95803),(#95804,#95805),(#95806,#95807),
(#95808,#95809),(#95810,#95811),(#95812,#95813),(#95814,#95815),(#95816,
#95817),(#95818,#95819),(#95820,#95821),(#95822,#95823),(#95824,#95825),
(#95826,#95827),(#95828,#95829),(#95830,#95831),(#95832,#95833),(#95834,
#95835),(#95836,#95837),(#95838,#95839),(#95840,#95841),(#95842,#95843),
(#95844,#95845),(#95846,#95847),(#95848,#95849),(#95850,#95851),(#95852,
#95853),(#95854,#95855),(#95856,#95857),(#95858,#95859),(#95860,#95861),
(#95862,#95863),(#95864,#95865),(#95866,#95867),(#95868,#95869),(#95870,
#95871),(#95872,#95873),(#95874,#95875),(#95876,#95877),(#95878,#95879),
(#95880,#95881),(#95882,#95883),(#95884,#95885),(#95886,#95887),(#95888,
#95889),(#95890,#95891),(#95892,#95893),(#95894,#95895),(#95896,#95897),
(#95898,#95899),(#95900,#95901),(#95902,#95903),(#95904,#95905),(#95906,
#95907),(#95908,#95909),(#95910,#95911),(#95912,#95913),(#95914,#95915),
(#95916,#95917),(#95918,#95919),(#95920,#95921),(#95922,#95923),(#95924,
#95925),(#95926,#95927),(#95928,#95929),(#95930,#95931),(#95932,#95933),
(#95934,#95935),(#95936,#95937),(#95938,#95939),(#95940,#95941),(#95942,
#95943),(#95944,#95945),(#95946,#95947),(#95948,#95949),(#95950,#95951),
(#95952,#95953),(#95954,#95955),(#95956,#95957),(#95958,#95959),(#95960,
#95961),(#95962,#95963),(#95964,#95965),(#95966,#95967),(#95968,#95969),
(#95970,#95971),(#95972,#95973),(#95974,#95975),(#95976,#95977),(#95978,
#95979),(#95980,#95981),(#95982,#95983),(#95984,#95985),(#95986,#95987),
(#95988,#95989),(#95990,#95991),(#95992,#95993),(#95994,#95995),(#95996,
#95997),(#95998,#95999),(#96000,#96001),(#96002,#96003),(#96004,#96005),
(#96006,#96007),(#96008,#96009),(#96010,#96011),(#96012,#96013),(#96014,
#96015),(#96016,#96017),(#96018,#96019),(#96020,#96021),(#96022,#96023),
(#96024,#96025),(#96026,#96027),(#96028,#96029),(#96030,#96031),(#96032,
#96033),(#96034,#96035),(#96036,#96037),(#96038,#96039)),.UNSPECIFIED.,
 .F.,.F.,.F.)
B_SPLINE_SURFACE_WITH_KNOTS((6,1,1,1,1,1,1,1,1,1,1,1,1,1,1,1,1,1,1,1,1,
1,1,1,1,1,1,1,1,1,1,1,1,1,1,1,1,1,1,1,1,1,1,1,1,1,1,1,1,1,1,1,1,1,1,1,1,
1,1,1,1,1,1,1,1,1,1,1,1,1,1,1,1,1,1,1,1,1,1,1,1,1,1,1,1,1,1,1,1,1,1,1,1,
1,1,1,1,1,1,1,1,1,1,1,1,1,1,1,1,1,1,1,1,1,1,1,1,1,1,1,1,1,1,1,1,1,1,1,1,
1,1,1,1,1,1,1,1,1,1,1,1,1,1,1,1,1,1,1,1,1,1,1,1,1,1,1,1,1,1,1,1,1,1,1,1,
1,1,1,1,1,1,1,1,1,1,1,1,1,1,1,1,1,1,1,1,1,1,1,1,1,1,1,1,1,1,1,1,1,1,1,6),
(2,2),(0.,0.005,0.01,0.015,0.02,0.025,0.03,0.035,0.04,0.045,0.05,0.055,
0.06,0.065,0.07,0.075,0.08,0.085,0.09,0.095,0.1,0.105,0.11,0.115,0.12,0.125,
0.13,0.135,0.14,0.145,0.15,0.155,0.16,0.165,0.17,0.175,0.18,0.185,0.19,
0.195,0.2,0.205,0.21,0.215,0.22,0.225,0.23,0.235,0.24,0.245,0.25,0.255,
0.26,0.265,0.27,0.275,0.28,0.285,0.29,0.295,0.3,0.305,0.31,0.315,0.32,0.325,
0.33,0.335,0.34,0.345,0.35,0.355,0.36,0.365,0.37,0.375,0.38,0.385,0.39,
0.395,0.4,0.405,0.41,0.415,0.42,0.425,0.43,0.435,0.44,0.445,0.45,0.455,
0.46,0.465,0.47,0.475,0.48,0.485,0.49,0.495,0.5,0.505,0.51,0.515,0.52,0.525,
0.53,0.535,0.54,0.545,0.55,0.555,0.56,0.565,0.57,0.575,0.58,0.585,0.59,
0.595,0.6,0.605,0.61,0.615,0.62,0.625,0.63,0.635,0.64,0.645,0.65,0.655,
0.66,0.665,0.67,0.675,0.68,0.685,0.690000000000001,0.695000000000001,0.700000000000001,
0.705000000000001,0.710000000000001,0.715000000000001,0.720000000000001,
0.725000000000001,0.730000000000001,0.735000000000001,0.740000000000001,
0.745000000000001,0.750000000000001,0.755000000000001,0.760000000000001,
0.765000000000001,0.770000000000001,0.775000000000001,0.780000000000001,
0.785000000000001,0.790000000000001,0.795000000000001,0.800000000000001,
0.805000000000001,0.810000000000001,0.815000000000001,0.820000000000001,
0.825000000000001,0.830000000000001,0.835000000000001,0.840000000000001,
0.845000000000001,0.850000000000001,0.855000000000001,0.860000000000001,
0.865000000000001,0.870000000000001,0.875000000000001,0.880000000000001,
0.885000000000001,0.890000000000001,0.895000000000001,0.900000000000001,
0.905000000000001,0.910000000000001,0.915000000000001,0.920000000000001,
0.925000000000001,0.930000000000001,0.935000000000001,0.940000000000001,
0.945000000000001,0.950000000000001,0.955000000000001,0.960000000000001,
0.965000000000001,0.970000000000001,0.975000000000001,0.980000000000001,
0.985000000000001,0.990000000000001,0.995000000000001,1.),(0.,1.2),
 .UNSPECIFIED.)
GEOMETRIC_REPRESENTATION_ITEM()
RATIONAL_B_SPLINE_SURFACE(((1.,1.),(1.,1.),(1.,1.),(1.,1.),(1.,1.),(1.,
1.),(1.,1.),(1.,1.),(1.,1.),(1.,1.),(1.,1.),(1.,1.),(1.,1.),(1.,1.),(1.,
1.),(1.,1.),(1.,1.),(1.,1.),(1.,1.),(1.,1.),(1.,1.),(1.,1.),(1.,1.),(1.,
1.),(1.,1.),(1.,1.),(1.,1.),(1.,1.),(1.,1.),(1.,1.),(1.,1.),(1.,1.),(1.,
1.),(1.,1.),(1.,1.),(1.,1.),(1.,1.),(1.,1.),(1.,1.),(1.,1.),(1.,1.),(1.,
1.),(1.,1.),(1.,1.),(1.,1.),(1.,1.),(1.,1.),(1.,1.),(1.,1.),(1.,1.),(1.,
1.),(1.,1.),(1.,1.),(1.,1.),(1.,1.),(1.,1.),(1.,1.),(1.,1.),(1.,1.),(1.,
1.),(1.,1.),(1.,1.),(1.,1.),(1.,1.),(1.,1.),(1.,1.),(1.,1.),(1.,1.),(1.,
1.),(1.,1.),(1.,1.),(1.,1.),(1.,1.),(1.,1.),(1.,1.),(1.,1.),(1.,1.),(1.,
1.),(1.,1.),(1.,1.),(1.,1.),(1.,1.),(1.,1.),(1.,1.),(1.,1.),(1.,1.),(1.,
1.),(1.,1.),(1.,1.),(1.,1.),(1.,1.),(1.,1.),(1.,1.),(1.,1.),(1.,1.),(1.,
1.),(1.,1.),(1.,1.),(1.,1.),(1.,1.),(1.,1.),(1.,1.),(1.,1.),(1.,1.),(1.,
1.),(1.,1.),(1.,1.),(1.,1.),(1.,1.),(1.,1.),(1.,1.),(1.,1.),(1.,1.),(1.,
1.),(1.,1.),(1.,1.),(1.,1.),(1.,1.),(1.,1.),(1.,1.),(1.,1.),(1.,1.),(1.,
1.),(1.,1.),(1.,1.),(1.,1.),(1.,1.),(1.,1.),(1.,1.),(1.,1.),(1.,1.),(1.,
1.),(1.,1.),(1.,1.),(1.,1.),(1.,1.),(1.,1.),(1.,1.),(1.,1.),(1.,1.),(1.,
1.),(1.,1.),(1.,1.),(1.,1.),(1.,1.),(1.,1.),(1.,1.),(1.,1.),(1.,1.),(1.,
1.),(1.,1.),(1.,1.),(1.,1.),(1.,1.),(1.,1.),(1.,1.),(1.,1.),(1.,1.),(1.,
1.),(1.,1.),(1.,1.),(1.,1.),(1.,1.),(1.,1.),(1.,1.),(1.,1.),(1.,1.),(1.,
1.),(1.,1.),(1.,1.),(1.,1.),(1.,1.),(1.,1.),(1.,1.),(1.,1.),(1.,1.),(1.,
1.),(1.,1.),(1.,1.),(1.,1.),(1.,1.),(1.,1.),(1.,1.),(1.,1.),(1.,1.),(1.,
1.),(1.,1.),(1.,1.),(1.,1.),(1.,1.),(1.,1.),(1.,1.),(1.,1.),(1.,1.),(1.,
1.),(1.,1.),(1.,1.),(1.,1.),(1.,1.),(1.,1.),(1.,1.),(1.,1.),(1.,1.),(1.,
1.),(1.,1.)))
REPRESENTATION_ITEM('')
SURFACE()
);
#932=(
BOUNDED_SURFACE()
B_SPLINE_SURFACE(5,1,((#96526,#96527),(#96528,#96529),(#96530,#96531),(#96532,
#96533),(#96534,#96535),(#96536,#96537),(#96538,#96539),(#96540,#96541),
(#96542,#96543),(#96544,#96545),(#96546,#96547),(#96548,#96549),(#96550,
#96551),(#96552,#96553),(#96554,#96555),(#96556,#96557),(#96558,#96559),
(#96560,#96561),(#96562,#96563),(#96564,#96565),(#96566,#96567),(#96568,
#96569),(#96570,#96571),(#96572,#96573),(#96574,#96575),(#96576,#96577),
(#96578,#96579),(#96580,#96581),(#96582,#96583),(#96584,#96585),(#96586,
#96587),(#96588,#96589),(#96590,#96591),(#96592,#96593),(#96594,#96595),
(#96596,#96597),(#96598,#96599),(#96600,#96601),(#96602,#96603),(#96604,
#96605),(#96606,#96607),(#96608,#96609),(#96610,#96611),(#96612,#96613),
(#96614,#96615),(#96616,#96617),(#96618,#96619),(#96620,#96621),(#96622,
#96623),(#96624,#96625),(#96626,#96627),(#96628,#96629),(#96630,#96631),
(#96632,#96633),(#96634,#96635),(#96636,#96637),(#96638,#96639),(#96640,
#96641),(#96642,#96643),(#96644,#96645),(#96646,#96647),(#96648,#96649),
(#96650,#96651),(#96652,#96653),(#96654,#96655),(#96656,#96657),(#96658,
#96659),(#96660,#96661),(#96662,#96663),(#96664,#96665),(#96666,#96667),
(#96668,#96669),(#96670,#96671),(#96672,#96673),(#96674,#96675),(#96676,
#96677),(#96678,#96679),(#96680,#96681),(#96682,#96683),(#96684,#96685),
(#96686,#96687),(#96688,#96689),(#96690,#96691),(#96692,#96693),(#96694,
#96695),(#96696,#96697),(#96698,#96699),(#96700,#96701),(#96702,#96703),
(#96704,#96705),(#96706,#96707),(#96708,#96709),(#96710,#96711),(#96712,
#96713),(#96714,#96715),(#96716,#96717),(#96718,#96719),(#96720,#96721),
(#96722,#96723),(#96724,#96725),(#96726,#96727),(#96728,#96729),(#96730,
#96731),(#96732,#96733),(#96734,#96735),(#96736,#96737),(#96738,#96739),
(#96740,#96741),(#96742,#96743),(#96744,#96745),(#96746,#96747),(#96748,
#96749),(#96750,#96751),(#96752,#96753),(#96754,#96755),(#96756,#96757),
(#96758,#96759),(#96760,#96761),(#96762,#96763),(#96764,#96765),(#96766,
#96767),(#96768,#96769),(#96770,#96771),(#96772,#96773),(#96774,#96775),
(#96776,#96777),(#96778,#96779),(#96780,#96781),(#96782,#96783),(#96784,
#96785),(#96786,#96787),(#96788,#96789),(#96790,#96791),(#96792,#96793),
(#96794,#96795),(#96796,#96797),(#96798,#96799),(#96800,#96801),(#96802,
#96803),(#96804,#96805),(#96806,#96807),(#96808,#96809),(#96810,#96811),
(#96812,#96813),(#96814,#96815),(#96816,#96817),(#96818,#96819),(#96820,
#96821),(#96822,#96823),(#96824,#96825),(#96826,#96827),(#96828,#96829),
(#96830,#96831),(#96832,#96833),(#96834,#96835),(#96836,#96837),(#96838,
#96839),(#96840,#96841),(#96842,#96843),(#96844,#96845),(#96846,#96847),
(#96848,#96849),(#96850,#96851),(#96852,#96853),(#96854,#96855),(#96856,
#96857),(#96858,#96859),(#96860,#96861),(#96862,#96863),(#96864,#96865),
(#96866,#96867),(#96868,#96869),(#96870,#96871),(#96872,#96873),(#96874,
#96875),(#96876,#96877),(#96878,#96879),(#96880,#96881),(#96882,#96883),
(#96884,#96885),(#96886,#96887),(#96888,#96889),(#96890,#96891),(#96892,
#96893),(#96894,#96895),(#96896,#96897),(#96898,#96899),(#96900,#96901),
(#96902,#96903),(#96904,#96905),(#96906,#96907),(#96908,#96909),(#96910,
#96911),(#96912,#96913),(#96914,#96915),(#96916,#96917),(#96918,#96919),
(#96920,#96921),(#96922,#96923),(#96924,#96925),(#96926,#96927),(#96928,
#96929),(#96930,#96931),(#96932,#96933),(#96934,#96935)),.UNSPECIFIED.,
 .F.,.F.,.F.)
B_SPLINE_SURFACE_WITH_KNOTS((6,1,1,1,1,1,1,1,1,1,1,1,1,1,1,1,1,1,1,1,1,
1,1,1,1,1,1,1,1,1,1,1,1,1,1,1,1,1,1,1,1,1,1,1,1,1,1,1,1,1,1,1,1,1,1,1,1,
1,1,1,1,1,1,1,1,1,1,1,1,1,1,1,1,1,1,1,1,1,1,1,1,1,1,1,1,1,1,1,1,1,1,1,1,
1,1,1,1,1,1,1,1,1,1,1,1,1,1,1,1,1,1,1,1,1,1,1,1,1,1,1,1,1,1,1,1,1,1,1,1,
1,1,1,1,1,1,1,1,1,1,1,1,1,1,1,1,1,1,1,1,1,1,1,1,1,1,1,1,1,1,1,1,1,1,1,1,
1,1,1,1,1,1,1,1,1,1,1,1,1,1,1,1,1,1,1,1,1,1,1,1,1,1,1,1,1,1,1,1,1,1,1,6),
(2,2),(0.,0.005,0.01,0.015,0.02,0.025,0.03,0.035,0.04,0.045,0.05,0.055,
0.06,0.065,0.07,0.075,0.08,0.085,0.09,0.095,0.1,0.105,0.11,0.115,0.12,0.125,
0.13,0.135,0.14,0.145,0.15,0.155,0.16,0.165,0.17,0.175,0.18,0.185,0.19,
0.195,0.2,0.205,0.21,0.215,0.22,0.225,0.23,0.235,0.24,0.245,0.25,0.255,
0.26,0.265,0.27,0.275,0.28,0.285,0.29,0.295,0.3,0.305,0.31,0.315,0.32,0.325,
0.33,0.335,0.34,0.345,0.35,0.355,0.36,0.365,0.37,0.375,0.38,0.385,0.39,
0.395,0.4,0.405,0.41,0.415,0.42,0.425,0.43,0.435,0.44,0.445,0.45,0.455,
0.46,0.465,0.47,0.475,0.48,0.485,0.49,0.495,0.5,0.505,0.51,0.515,0.52,0.525,
0.53,0.535,0.54,0.545,0.55,0.555,0.56,0.565,0.57,0.575,0.58,0.585,0.59,
0.595,0.6,0.605,0.61,0.615,0.62,0.625,0.63,0.635,0.64,0.645,0.65,0.655,
0.66,0.665,0.67,0.675,0.68,0.685,0.690000000000001,0.695000000000001,0.700000000000001,
0.705000000000001,0.710000000000001,0.715000000000001,0.720000000000001,
0.725000000000001,0.730000000000001,0.735000000000001,0.740000000000001,
0.745000000000001,0.750000000000001,0.755000000000001,0.760000000000001,
0.765000000000001,0.770000000000001,0.775000000000001,0.780000000000001,
0.785000000000001,0.790000000000001,0.795000000000001,0.800000000000001,
0.805000000000001,0.810000000000001,0.815000000000001,0.820000000000001,
0.825000000000001,0.830000000000001,0.835000000000001,0.840000000000001,
0.845000000000001,0.850000000000001,0.855000000000001,0.860000000000001,
0.865000000000001,0.870000000000001,0.875000000000001,0.880000000000001,
0.885000000000001,0.890000000000001,0.895000000000001,0.900000000000001,
0.905000000000001,0.910000000000001,0.915000000000001,0.920000000000001,
0.925000000000001,0.930000000000001,0.935000000000001,0.940000000000001,
0.945000000000001,0.950000000000001,0.955000000000001,0.960000000000001,
0.965000000000001,0.970000000000001,0.975000000000001,0.980000000000001,
0.985000000000001,0.990000000000001,0.995000000000001,1.),(0.,1.2),
 .UNSPECIFIED.)
GEOMETRIC_REPRESENTATION_ITEM()
RATIONAL_B_SPLINE_SURFACE(((1.,1.),(1.,1.),(1.,1.),(1.,1.),(1.,1.),(1.,
1.),(1.,1.),(1.,1.),(1.,1.),(1.,1.),(1.,1.),(1.,1.),(1.,1.),(1.,1.),(1.,
1.),(1.,1.),(1.,1.),(1.,1.),(1.,1.),(1.,1.),(1.,1.),(1.,1.),(1.,1.),(1.,
1.),(1.,1.),(1.,1.),(1.,1.),(1.,1.),(1.,1.),(1.,1.),(1.,1.),(1.,1.),(1.,
1.),(1.,1.),(1.,1.),(1.,1.),(1.,1.),(1.,1.),(1.,1.),(1.,1.),(1.,1.),(1.,
1.),(1.,1.),(1.,1.),(1.,1.),(1.,1.),(1.,1.),(1.,1.),(1.,1.),(1.,1.),(1.,
1.),(1.,1.),(1.,1.),(1.,1.),(1.,1.),(1.,1.),(1.,1.),(1.,1.),(1.,1.),(1.,
1.),(1.,1.),(1.,1.),(1.,1.),(1.,1.),(1.,1.),(1.,1.),(1.,1.),(1.,1.),(1.,
1.),(1.,1.),(1.,1.),(1.,1.),(1.,1.),(1.,1.),(1.,1.),(1.,1.),(1.,1.),(1.,
1.),(1.,1.),(1.,1.),(1.,1.),(1.,1.),(1.,1.),(1.,1.),(1.,1.),(1.,1.),(1.,
1.),(1.,1.),(1.,1.),(1.,1.),(1.,1.),(1.,1.),(1.,1.),(1.,1.),(1.,1.),(1.,
1.),(1.,1.),(1.,1.),(1.,1.),(1.,1.),(1.,1.),(1.,1.),(1.,1.),(1.,1.),(1.,
1.),(1.,1.),(1.,1.),(1.,1.),(1.,1.),(1.,1.),(1.,1.),(1.,1.),(1.,1.),(1.,
1.),(1.,1.),(1.,1.),(1.,1.),(1.,1.),(1.,1.),(1.,1.),(1.,1.),(1.,1.),(1.,
1.),(1.,1.),(1.,1.),(1.,1.),(1.,1.),(1.,1.),(1.,1.),(1.,1.),(1.,1.),(1.,
1.),(1.,1.),(1.,1.),(1.,1.),(1.,1.),(1.,1.),(1.,1.),(1.,1.),(1.,1.),(1.,
1.),(1.,1.),(1.,1.),(1.,1.),(1.,1.),(1.,1.),(1.,1.),(1.,1.),(1.,1.),(1.,
1.),(1.,1.),(1.,1.),(1.,1.),(1.,1.),(1.,1.),(1.,1.),(1.,1.),(1.,1.),(1.,
1.),(1.,1.),(1.,1.),(1.,1.),(1.,1.),(1.,1.),(1.,1.),(1.,1.),(1.,1.),(1.,
1.),(1.,1.),(1.,1.),(1.,1.),(1.,1.),(1.,1.),(1.,1.),(1.,1.),(1.,1.),(1.,
1.),(1.,1.),(1.,1.),(1.,1.),(1.,1.),(1.,1.),(1.,1.),(1.,1.),(1.,1.),(1.,
1.),(1.,1.),(1.,1.),(1.,1.),(1.,1.),(1.,1.),(1.,1.),(1.,1.),(1.,1.),(1.,
1.),(1.,1.),(1.,1.),(1.,1.),(1.,1.),(1.,1.),(1.,1.),(1.,1.),(1.,1.),(1.,
1.),(1.,1.)))
REPRESENTATION_ITEM('')
SURFACE()
);
#933=(
BOUNDED_SURFACE()
B_SPLINE_SURFACE(5,1,((#97422,#97423),(#97424,#97425),(#97426,#97427),(#97428,
#97429),(#97430,#97431),(#97432,#97433),(#97434,#97435),(#97436,#97437),
(#97438,#97439),(#97440,#97441),(#97442,#97443),(#97444,#97445),(#97446,
#97447),(#97448,#97449),(#97450,#97451),(#97452,#97453),(#97454,#97455),
(#97456,#97457),(#97458,#97459),(#97460,#97461),(#97462,#97463),(#97464,
#97465),(#97466,#97467),(#97468,#97469),(#97470,#97471),(#97472,#97473),
(#97474,#97475),(#97476,#97477),(#97478,#97479),(#97480,#97481),(#97482,
#97483),(#97484,#97485),(#97486,#97487),(#97488,#97489),(#97490,#97491),
(#97492,#97493),(#97494,#97495),(#97496,#97497),(#97498,#97499),(#97500,
#97501),(#97502,#97503),(#97504,#97505),(#97506,#97507),(#97508,#97509),
(#97510,#97511),(#97512,#97513),(#97514,#97515),(#97516,#97517),(#97518,
#97519),(#97520,#97521),(#97522,#97523),(#97524,#97525),(#97526,#97527),
(#97528,#97529),(#97530,#97531),(#97532,#97533),(#97534,#97535),(#97536,
#97537),(#97538,#97539),(#97540,#97541),(#97542,#97543),(#97544,#97545),
(#97546,#97547),(#97548,#97549),(#97550,#97551),(#97552,#97553),(#97554,
#97555),(#97556,#97557),(#97558,#97559),(#97560,#97561),(#97562,#97563),
(#97564,#97565),(#97566,#97567),(#97568,#97569),(#97570,#97571),(#97572,
#97573),(#97574,#97575),(#97576,#97577),(#97578,#97579),(#97580,#97581),
(#97582,#97583),(#97584,#97585),(#97586,#97587),(#97588,#97589),(#97590,
#97591),(#97592,#97593),(#97594,#97595),(#97596,#97597),(#97598,#97599),
(#97600,#97601),(#97602,#97603),(#97604,#97605),(#97606,#97607),(#97608,
#97609),(#97610,#97611),(#97612,#97613),(#97614,#97615),(#97616,#97617),
(#97618,#97619),(#97620,#97621),(#97622,#97623),(#97624,#97625),(#97626,
#97627),(#97628,#97629),(#97630,#97631),(#97632,#97633),(#97634,#97635),
(#97636,#97637),(#97638,#97639),(#97640,#97641),(#97642,#97643),(#97644,
#97645),(#97646,#97647),(#97648,#97649),(#97650,#97651),(#97652,#97653),
(#97654,#97655),(#97656,#97657),(#97658,#97659),(#97660,#97661),(#97662,
#97663),(#97664,#97665),(#97666,#97667),(#97668,#97669),(#97670,#97671),
(#97672,#97673),(#97674,#97675),(#97676,#97677),(#97678,#97679),(#97680,
#97681),(#97682,#97683),(#97684,#97685),(#97686,#97687),(#97688,#97689),
(#97690,#97691),(#97692,#97693),(#97694,#97695),(#97696,#97697),(#97698,
#97699),(#97700,#97701),(#97702,#97703),(#97704,#97705),(#97706,#97707),
(#97708,#97709),(#97710,#97711),(#97712,#97713),(#97714,#97715),(#97716,
#97717),(#97718,#97719),(#97720,#97721),(#97722,#97723),(#97724,#97725),
(#97726,#97727),(#97728,#97729),(#97730,#97731),(#97732,#97733),(#97734,
#97735),(#97736,#97737),(#97738,#97739),(#97740,#97741),(#97742,#97743),
(#97744,#97745),(#97746,#97747),(#97748,#97749),(#97750,#97751),(#97752,
#97753),(#97754,#97755),(#97756,#97757),(#97758,#97759),(#97760,#97761),
(#97762,#97763),(#97764,#97765),(#97766,#97767),(#97768,#97769),(#97770,
#97771),(#97772,#97773),(#97774,#97775),(#97776,#97777),(#97778,#97779),
(#97780,#97781),(#97782,#97783),(#97784,#97785),(#97786,#97787),(#97788,
#97789),(#97790,#97791),(#97792,#97793),(#97794,#97795),(#97796,#97797),
(#97798,#97799),(#97800,#97801),(#97802,#97803),(#97804,#97805),(#97806,
#97807),(#97808,#97809),(#97810,#97811),(#97812,#97813),(#97814,#97815),
(#97816,#97817),(#97818,#97819),(#97820,#97821),(#97822,#97823),(#97824,
#97825),(#97826,#97827),(#97828,#97829),(#97830,#97831)),.UNSPECIFIED.,
 .F.,.F.,.F.)
B_SPLINE_SURFACE_WITH_KNOTS((6,1,1,1,1,1,1,1,1,1,1,1,1,1,1,1,1,1,1,1,1,
1,1,1,1,1,1,1,1,1,1,1,1,1,1,1,1,1,1,1,1,1,1,1,1,1,1,1,1,1,1,1,1,1,1,1,1,
1,1,1,1,1,1,1,1,1,1,1,1,1,1,1,1,1,1,1,1,1,1,1,1,1,1,1,1,1,1,1,1,1,1,1,1,
1,1,1,1,1,1,1,1,1,1,1,1,1,1,1,1,1,1,1,1,1,1,1,1,1,1,1,1,1,1,1,1,1,1,1,1,
1,1,1,1,1,1,1,1,1,1,1,1,1,1,1,1,1,1,1,1,1,1,1,1,1,1,1,1,1,1,1,1,1,1,1,1,
1,1,1,1,1,1,1,1,1,1,1,1,1,1,1,1,1,1,1,1,1,1,1,1,1,1,1,1,1,1,1,1,1,1,1,6),
(2,2),(0.,0.005,0.01,0.015,0.02,0.025,0.03,0.035,0.04,0.045,0.05,0.055,
0.06,0.065,0.07,0.075,0.08,0.085,0.09,0.095,0.1,0.105,0.11,0.115,0.12,0.125,
0.13,0.135,0.14,0.145,0.15,0.155,0.16,0.165,0.17,0.175,0.18,0.185,0.19,
0.195,0.2,0.205,0.21,0.215,0.22,0.225,0.23,0.235,0.24,0.245,0.25,0.255,
0.26,0.265,0.27,0.275,0.28,0.285,0.29,0.295,0.3,0.305,0.31,0.315,0.32,0.325,
0.33,0.335,0.34,0.345,0.35,0.355,0.36,0.365,0.37,0.375,0.38,0.385,0.39,
0.395,0.4,0.405,0.41,0.415,0.42,0.425,0.43,0.435,0.44,0.445,0.45,0.455,
0.46,0.465,0.47,0.475,0.48,0.485,0.49,0.495,0.5,0.505,0.51,0.515,0.52,0.525,
0.53,0.535,0.54,0.545,0.55,0.555,0.56,0.565,0.57,0.575,0.58,0.585,0.59,
0.595,0.6,0.605,0.61,0.615,0.62,0.625,0.63,0.635,0.64,0.645,0.65,0.655,
0.66,0.665,0.67,0.675,0.68,0.685,0.690000000000001,0.695000000000001,0.700000000000001,
0.705000000000001,0.710000000000001,0.715000000000001,0.720000000000001,
0.725000000000001,0.730000000000001,0.735000000000001,0.740000000000001,
0.745000000000001,0.750000000000001,0.755000000000001,0.760000000000001,
0.765000000000001,0.770000000000001,0.775000000000001,0.780000000000001,
0.785000000000001,0.790000000000001,0.795000000000001,0.800000000000001,
0.805000000000001,0.810000000000001,0.815000000000001,0.820000000000001,
0.825000000000001,0.830000000000001,0.835000000000001,0.840000000000001,
0.845000000000001,0.850000000000001,0.855000000000001,0.860000000000001,
0.865000000000001,0.870000000000001,0.875000000000001,0.880000000000001,
0.885000000000001,0.890000000000001,0.895000000000001,0.900000000000001,
0.905000000000001,0.910000000000001,0.915000000000001,0.920000000000001,
0.925000000000001,0.930000000000001,0.935000000000001,0.940000000000001,
0.945000000000001,0.950000000000001,0.955000000000001,0.960000000000001,
0.965000000000001,0.970000000000001,0.975000000000001,0.980000000000001,
0.985000000000001,0.990000000000001,0.995000000000001,1.),(0.,1.2),
 .UNSPECIFIED.)
GEOMETRIC_REPRESENTATION_ITEM()
RATIONAL_B_SPLINE_SURFACE(((1.,1.),(1.,1.),(1.,1.),(1.,1.),(1.,1.),(1.,
1.),(1.,1.),(1.,1.),(1.,1.),(1.,1.),(1.,1.),(1.,1.),(1.,1.),(1.,1.),(1.,
1.),(1.,1.),(1.,1.),(1.,1.),(1.,1.),(1.,1.),(1.,1.),(1.,1.),(1.,1.),(1.,
1.),(1.,1.),(1.,1.),(1.,1.),(1.,1.),(1.,1.),(1.,1.),(1.,1.),(1.,1.),(1.,
1.),(1.,1.),(1.,1.),(1.,1.),(1.,1.),(1.,1.),(1.,1.),(1.,1.),(1.,1.),(1.,
1.),(1.,1.),(1.,1.),(1.,1.),(1.,1.),(1.,1.),(1.,1.),(1.,1.),(1.,1.),(1.,
1.),(1.,1.),(1.,1.),(1.,1.),(1.,1.),(1.,1.),(1.,1.),(1.,1.),(1.,1.),(1.,
1.),(1.,1.),(1.,1.),(1.,1.),(1.,1.),(1.,1.),(1.,1.),(1.,1.),(1.,1.),(1.,
1.),(1.,1.),(1.,1.),(1.,1.),(1.,1.),(1.,1.),(1.,1.),(1.,1.),(1.,1.),(1.,
1.),(1.,1.),(1.,1.),(1.,1.),(1.,1.),(1.,1.),(1.,1.),(1.,1.),(1.,1.),(1.,
1.),(1.,1.),(1.,1.),(1.,1.),(1.,1.),(1.,1.),(1.,1.),(1.,1.),(1.,1.),(1.,
1.),(1.,1.),(1.,1.),(1.,1.),(1.,1.),(1.,1.),(1.,1.),(1.,1.),(1.,1.),(1.,
1.),(1.,1.),(1.,1.),(1.,1.),(1.,1.),(1.,1.),(1.,1.),(1.,1.),(1.,1.),(1.,
1.),(1.,1.),(1.,1.),(1.,1.),(1.,1.),(1.,1.),(1.,1.),(1.,1.),(1.,1.),(1.,
1.),(1.,1.),(1.,1.),(1.,1.),(1.,1.),(1.,1.),(1.,1.),(1.,1.),(1.,1.),(1.,
1.),(1.,1.),(1.,1.),(1.,1.),(1.,1.),(1.,1.),(1.,1.),(1.,1.),(1.,1.),(1.,
1.),(1.,1.),(1.,1.),(1.,1.),(1.,1.),(1.,1.),(1.,1.),(1.,1.),(1.,1.),(1.,
1.),(1.,1.),(1.,1.),(1.,1.),(1.,1.),(1.,1.),(1.,1.),(1.,1.),(1.,1.),(1.,
1.),(1.,1.),(1.,1.),(1.,1.),(1.,1.),(1.,1.),(1.,1.),(1.,1.),(1.,1.),(1.,
1.),(1.,1.),(1.,1.),(1.,1.),(1.,1.),(1.,1.),(1.,1.),(1.,1.),(1.,1.),(1.,
1.),(1.,1.),(1.,1.),(1.,1.),(1.,1.),(1.,1.),(1.,1.),(1.,1.),(1.,1.),(1.,
1.),(1.,1.),(1.,1.),(1.,1.),(1.,1.),(1.,1.),(1.,1.),(1.,1.),(1.,1.),(1.,
1.),(1.,1.),(1.,1.),(1.,1.),(1.,1.),(1.,1.),(1.,1.),(1.,1.),(1.,1.),(1.,
1.),(1.,1.)))
REPRESENTATION_ITEM('')
SURFACE()
);
#934=(
BOUNDED_SURFACE()
B_SPLINE_SURFACE(5,1,((#98318,#98319),(#98320,#98321),(#98322,#98323),(#98324,
#98325),(#98326,#98327),(#98328,#98329),(#98330,#98331),(#98332,#98333),
(#98334,#98335),(#98336,#98337),(#98338,#98339),(#98340,#98341),(#98342,
#98343),(#98344,#98345),(#98346,#98347),(#98348,#98349),(#98350,#98351),
(#98352,#98353),(#98354,#98355),(#98356,#98357),(#98358,#98359),(#98360,
#98361),(#98362,#98363),(#98364,#98365),(#98366,#98367),(#98368,#98369),
(#98370,#98371),(#98372,#98373),(#98374,#98375),(#98376,#98377),(#98378,
#98379),(#98380,#98381),(#98382,#98383),(#98384,#98385),(#98386,#98387),
(#98388,#98389),(#98390,#98391),(#98392,#98393),(#98394,#98395),(#98396,
#98397),(#98398,#98399),(#98400,#98401),(#98402,#98403),(#98404,#98405),
(#98406,#98407),(#98408,#98409),(#98410,#98411),(#98412,#98413),(#98414,
#98415),(#98416,#98417),(#98418,#98419),(#98420,#98421),(#98422,#98423),
(#98424,#98425),(#98426,#98427),(#98428,#98429),(#98430,#98431),(#98432,
#98433),(#98434,#98435),(#98436,#98437),(#98438,#98439),(#98440,#98441),
(#98442,#98443),(#98444,#98445),(#98446,#98447),(#98448,#98449),(#98450,
#98451),(#98452,#98453),(#98454,#98455),(#98456,#98457),(#98458,#98459),
(#98460,#98461),(#98462,#98463),(#98464,#98465),(#98466,#98467),(#98468,
#98469),(#98470,#98471),(#98472,#98473),(#98474,#98475),(#98476,#98477),
(#98478,#98479),(#98480,#98481),(#98482,#98483),(#98484,#98485),(#98486,
#98487),(#98488,#98489),(#98490,#98491),(#98492,#98493),(#98494,#98495),
(#98496,#98497),(#98498,#98499),(#98500,#98501),(#98502,#98503),(#98504,
#98505),(#98506,#98507),(#98508,#98509),(#98510,#98511),(#98512,#98513),
(#98514,#98515),(#98516,#98517),(#98518,#98519),(#98520,#98521),(#98522,
#98523),(#98524,#98525),(#98526,#98527),(#98528,#98529),(#98530,#98531),
(#98532,#98533),(#98534,#98535),(#98536,#98537),(#98538,#98539),(#98540,
#98541),(#98542,#98543),(#98544,#98545),(#98546,#98547),(#98548,#98549),
(#98550,#98551),(#98552,#98553),(#98554,#98555),(#98556,#98557),(#98558,
#98559),(#98560,#98561),(#98562,#98563),(#98564,#98565),(#98566,#98567),
(#98568,#98569),(#98570,#98571),(#98572,#98573),(#98574,#98575),(#98576,
#98577),(#98578,#98579),(#98580,#98581),(#98582,#98583),(#98584,#98585),
(#98586,#98587),(#98588,#98589),(#98590,#98591),(#98592,#98593),(#98594,
#98595),(#98596,#98597),(#98598,#98599),(#98600,#98601),(#98602,#98603),
(#98604,#98605),(#98606,#98607),(#98608,#98609),(#98610,#98611),(#98612,
#98613),(#98614,#98615),(#98616,#98617),(#98618,#98619),(#98620,#98621),
(#98622,#98623),(#98624,#98625),(#98626,#98627),(#98628,#98629),(#98630,
#98631),(#98632,#98633),(#98634,#98635),(#98636,#98637),(#98638,#98639),
(#98640,#98641),(#98642,#98643),(#98644,#98645),(#98646,#98647),(#98648,
#98649),(#98650,#98651),(#98652,#98653),(#98654,#98655),(#98656,#98657),
(#98658,#98659),(#98660,#98661),(#98662,#98663),(#98664,#98665),(#98666,
#98667),(#98668,#98669),(#98670,#98671),(#98672,#98673),(#98674,#98675),
(#98676,#98677),(#98678,#98679),(#98680,#98681),(#98682,#98683),(#98684,
#98685),(#98686,#98687),(#98688,#98689),(#98690,#98691),(#98692,#98693),
(#98694,#98695),(#98696,#98697),(#98698,#98699),(#98700,#98701),(#98702,
#98703),(#98704,#98705),(#98706,#98707),(#98708,#98709),(#98710,#98711),
(#98712,#98713),(#98714,#98715),(#98716,#98717),(#98718,#98719),(#98720,
#98721),(#98722,#98723),(#98724,#98725),(#98726,#98727)),.UNSPECIFIED.,
 .F.,.F.,.F.)
B_SPLINE_SURFACE_WITH_KNOTS((6,1,1,1,1,1,1,1,1,1,1,1,1,1,1,1,1,1,1,1,1,
1,1,1,1,1,1,1,1,1,1,1,1,1,1,1,1,1,1,1,1,1,1,1,1,1,1,1,1,1,1,1,1,1,1,1,1,
1,1,1,1,1,1,1,1,1,1,1,1,1,1,1,1,1,1,1,1,1,1,1,1,1,1,1,1,1,1,1,1,1,1,1,1,
1,1,1,1,1,1,1,1,1,1,1,1,1,1,1,1,1,1,1,1,1,1,1,1,1,1,1,1,1,1,1,1,1,1,1,1,
1,1,1,1,1,1,1,1,1,1,1,1,1,1,1,1,1,1,1,1,1,1,1,1,1,1,1,1,1,1,1,1,1,1,1,1,
1,1,1,1,1,1,1,1,1,1,1,1,1,1,1,1,1,1,1,1,1,1,1,1,1,1,1,1,1,1,1,1,1,1,1,6),
(2,2),(0.,0.005,0.01,0.015,0.02,0.025,0.03,0.035,0.04,0.045,0.05,0.055,
0.06,0.065,0.07,0.075,0.08,0.085,0.09,0.095,0.1,0.105,0.11,0.115,0.12,0.125,
0.13,0.135,0.14,0.145,0.15,0.155,0.16,0.165,0.17,0.175,0.18,0.185,0.19,
0.195,0.2,0.205,0.21,0.215,0.22,0.225,0.23,0.235,0.24,0.245,0.25,0.255,
0.26,0.265,0.27,0.275,0.28,0.285,0.29,0.295,0.3,0.305,0.31,0.315,0.32,0.325,
0.33,0.335,0.34,0.345,0.35,0.355,0.36,0.365,0.37,0.375,0.38,0.385,0.39,
0.395,0.4,0.405,0.41,0.415,0.42,0.425,0.43,0.435,0.44,0.445,0.45,0.455,
0.46,0.465,0.47,0.475,0.48,0.485,0.49,0.495,0.5,0.505,0.51,0.515,0.52,0.525,
0.53,0.535,0.54,0.545,0.55,0.555,0.56,0.565,0.57,0.575,0.58,0.585,0.59,
0.595,0.6,0.605,0.61,0.615,0.62,0.625,0.63,0.635,0.64,0.645,0.65,0.655,
0.66,0.665,0.67,0.675,0.68,0.685,0.690000000000001,0.695000000000001,0.700000000000001,
0.705000000000001,0.710000000000001,0.715000000000001,0.720000000000001,
0.725000000000001,0.730000000000001,0.735000000000001,0.740000000000001,
0.745000000000001,0.750000000000001,0.755000000000001,0.760000000000001,
0.765000000000001,0.770000000000001,0.775000000000001,0.780000000000001,
0.785000000000001,0.790000000000001,0.795000000000001,0.800000000000001,
0.805000000000001,0.810000000000001,0.815000000000001,0.820000000000001,
0.825000000000001,0.830000000000001,0.835000000000001,0.840000000000001,
0.845000000000001,0.850000000000001,0.855000000000001,0.860000000000001,
0.865000000000001,0.870000000000001,0.875000000000001,0.880000000000001,
0.885000000000001,0.890000000000001,0.895000000000001,0.900000000000001,
0.905000000000001,0.910000000000001,0.915000000000001,0.920000000000001,
0.925000000000001,0.930000000000001,0.935000000000001,0.940000000000001,
0.945000000000001,0.950000000000001,0.955000000000001,0.960000000000001,
0.965000000000001,0.970000000000001,0.975000000000001,0.980000000000001,
0.985000000000001,0.990000000000001,0.995000000000001,1.),(0.,1.2),
 .UNSPECIFIED.)
GEOMETRIC_REPRESENTATION_ITEM()
RATIONAL_B_SPLINE_SURFACE(((1.,1.),(1.,1.),(1.,1.),(1.,1.),(1.,1.),(1.,
1.),(1.,1.),(1.,1.),(1.,1.),(1.,1.),(1.,1.),(1.,1.),(1.,1.),(1.,1.),(1.,
1.),(1.,1.),(1.,1.),(1.,1.),(1.,1.),(1.,1.),(1.,1.),(1.,1.),(1.,1.),(1.,
1.),(1.,1.),(1.,1.),(1.,1.),(1.,1.),(1.,1.),(1.,1.),(1.,1.),(1.,1.),(1.,
1.),(1.,1.),(1.,1.),(1.,1.),(1.,1.),(1.,1.),(1.,1.),(1.,1.),(1.,1.),(1.,
1.),(1.,1.),(1.,1.),(1.,1.),(1.,1.),(1.,1.),(1.,1.),(1.,1.),(1.,1.),(1.,
1.),(1.,1.),(1.,1.),(1.,1.),(1.,1.),(1.,1.),(1.,1.),(1.,1.),(1.,1.),(1.,
1.),(1.,1.),(1.,1.),(1.,1.),(1.,1.),(1.,1.),(1.,1.),(1.,1.),(1.,1.),(1.,
1.),(1.,1.),(1.,1.),(1.,1.),(1.,1.),(1.,1.),(1.,1.),(1.,1.),(1.,1.),(1.,
1.),(1.,1.),(1.,1.),(1.,1.),(1.,1.),(1.,1.),(1.,1.),(1.,1.),(1.,1.),(1.,
1.),(1.,1.),(1.,1.),(1.,1.),(1.,1.),(1.,1.),(1.,1.),(1.,1.),(1.,1.),(1.,
1.),(1.,1.),(1.,1.),(1.,1.),(1.,1.),(1.,1.),(1.,1.),(1.,1.),(1.,1.),(1.,
1.),(1.,1.),(1.,1.),(1.,1.),(1.,1.),(1.,1.),(1.,1.),(1.,1.),(1.,1.),(1.,
1.),(1.,1.),(1.,1.),(1.,1.),(1.,1.),(1.,1.),(1.,1.),(1.,1.),(1.,1.),(1.,
1.),(1.,1.),(1.,1.),(1.,1.),(1.,1.),(1.,1.),(1.,1.),(1.,1.),(1.,1.),(1.,
1.),(1.,1.),(1.,1.),(1.,1.),(1.,1.),(1.,1.),(1.,1.),(1.,1.),(1.,1.),(1.,
1.),(1.,1.),(1.,1.),(1.,1.),(1.,1.),(1.,1.),(1.,1.),(1.,1.),(1.,1.),(1.,
1.),(1.,1.),(1.,1.),(1.,1.),(1.,1.),(1.,1.),(1.,1.),(1.,1.),(1.,1.),(1.,
1.),(1.,1.),(1.,1.),(1.,1.),(1.,1.),(1.,1.),(1.,1.),(1.,1.),(1.,1.),(1.,
1.),(1.,1.),(1.,1.),(1.,1.),(1.,1.),(1.,1.),(1.,1.),(1.,1.),(1.,1.),(1.,
1.),(1.,1.),(1.,1.),(1.,1.),(1.,1.),(1.,1.),(1.,1.),(1.,1.),(1.,1.),(1.,
1.),(1.,1.),(1.,1.),(1.,1.),(1.,1.),(1.,1.),(1.,1.),(1.,1.),(1.,1.),(1.,
1.),(1.,1.),(1.,1.),(1.,1.),(1.,1.),(1.,1.),(1.,1.),(1.,1.),(1.,1.),(1.,
1.),(1.,1.)))
REPRESENTATION_ITEM('')
SURFACE()
);
#935=(
BOUNDED_SURFACE()
B_SPLINE_SURFACE(5,1,((#99214,#99215),(#99216,#99217),(#99218,#99219),(#99220,
#99221),(#99222,#99223),(#99224,#99225),(#99226,#99227),(#99228,#99229),
(#99230,#99231),(#99232,#99233),(#99234,#99235),(#99236,#99237),(#99238,
#99239),(#99240,#99241),(#99242,#99243),(#99244,#99245),(#99246,#99247),
(#99248,#99249),(#99250,#99251),(#99252,#99253),(#99254,#99255),(#99256,
#99257),(#99258,#99259),(#99260,#99261),(#99262,#99263),(#99264,#99265),
(#99266,#99267),(#99268,#99269),(#99270,#99271),(#99272,#99273),(#99274,
#99275),(#99276,#99277),(#99278,#99279),(#99280,#99281),(#99282,#99283),
(#99284,#99285),(#99286,#99287),(#99288,#99289),(#99290,#99291),(#99292,
#99293),(#99294,#99295),(#99296,#99297),(#99298,#99299),(#99300,#99301),
(#99302,#99303),(#99304,#99305),(#99306,#99307),(#99308,#99309),(#99310,
#99311),(#99312,#99313),(#99314,#99315),(#99316,#99317),(#99318,#99319),
(#99320,#99321),(#99322,#99323),(#99324,#99325),(#99326,#99327),(#99328,
#99329),(#99330,#99331),(#99332,#99333),(#99334,#99335),(#99336,#99337),
(#99338,#99339),(#99340,#99341),(#99342,#99343),(#99344,#99345),(#99346,
#99347),(#99348,#99349),(#99350,#99351),(#99352,#99353),(#99354,#99355),
(#99356,#99357),(#99358,#99359),(#99360,#99361),(#99362,#99363),(#99364,
#99365),(#99366,#99367),(#99368,#99369),(#99370,#99371),(#99372,#99373),
(#99374,#99375),(#99376,#99377),(#99378,#99379),(#99380,#99381),(#99382,
#99383),(#99384,#99385),(#99386,#99387),(#99388,#99389),(#99390,#99391),
(#99392,#99393),(#99394,#99395),(#99396,#99397),(#99398,#99399),(#99400,
#99401),(#99402,#99403),(#99404,#99405),(#99406,#99407),(#99408,#99409),
(#99410,#99411),(#99412,#99413),(#99414,#99415),(#99416,#99417),(#99418,
#99419),(#99420,#99421),(#99422,#99423),(#99424,#99425),(#99426,#99427),
(#99428,#99429),(#99430,#99431),(#99432,#99433),(#99434,#99435),(#99436,
#99437),(#99438,#99439),(#99440,#99441),(#99442,#99443),(#99444,#99445),
(#99446,#99447),(#99448,#99449),(#99450,#99451),(#99452,#99453),(#99454,
#99455),(#99456,#99457),(#99458,#99459),(#99460,#99461),(#99462,#99463),
(#99464,#99465),(#99466,#99467),(#99468,#99469),(#99470,#99471),(#99472,
#99473),(#99474,#99475),(#99476,#99477),(#99478,#99479),(#99480,#99481),
(#99482,#99483),(#99484,#99485),(#99486,#99487),(#99488,#99489),(#99490,
#99491),(#99492,#99493),(#99494,#99495),(#99496,#99497),(#99498,#99499),
(#99500,#99501),(#99502,#99503),(#99504,#99505),(#99506,#99507),(#99508,
#99509),(#99510,#99511),(#99512,#99513),(#99514,#99515),(#99516,#99517),
(#99518,#99519),(#99520,#99521),(#99522,#99523),(#99524,#99525),(#99526,
#99527),(#99528,#99529),(#99530,#99531),(#99532,#99533),(#99534,#99535),
(#99536,#99537),(#99538,#99539),(#99540,#99541),(#99542,#99543),(#99544,
#99545),(#99546,#99547),(#99548,#99549),(#99550,#99551),(#99552,#99553),
(#99554,#99555),(#99556,#99557),(#99558,#99559),(#99560,#99561),(#99562,
#99563),(#99564,#99565),(#99566,#99567),(#99568,#99569),(#99570,#99571),
(#99572,#99573),(#99574,#99575),(#99576,#99577),(#99578,#99579),(#99580,
#99581),(#99582,#99583),(#99584,#99585),(#99586,#99587),(#99588,#99589),
(#99590,#99591),(#99592,#99593),(#99594,#99595),(#99596,#99597),(#99598,
#99599),(#99600,#99601),(#99602,#99603),(#99604,#99605),(#99606,#99607),
(#99608,#99609),(#99610,#99611),(#99612,#99613),(#99614,#99615),(#99616,
#99617),(#99618,#99619),(#99620,#99621),(#99622,#99623)),.UNSPECIFIED.,
 .F.,.F.,.F.)
B_SPLINE_SURFACE_WITH_KNOTS((6,1,1,1,1,1,1,1,1,1,1,1,1,1,1,1,1,1,1,1,1,
1,1,1,1,1,1,1,1,1,1,1,1,1,1,1,1,1,1,1,1,1,1,1,1,1,1,1,1,1,1,1,1,1,1,1,1,
1,1,1,1,1,1,1,1,1,1,1,1,1,1,1,1,1,1,1,1,1,1,1,1,1,1,1,1,1,1,1,1,1,1,1,1,
1,1,1,1,1,1,1,1,1,1,1,1,1,1,1,1,1,1,1,1,1,1,1,1,1,1,1,1,1,1,1,1,1,1,1,1,
1,1,1,1,1,1,1,1,1,1,1,1,1,1,1,1,1,1,1,1,1,1,1,1,1,1,1,1,1,1,1,1,1,1,1,1,
1,1,1,1,1,1,1,1,1,1,1,1,1,1,1,1,1,1,1,1,1,1,1,1,1,1,1,1,1,1,1,1,1,1,1,6),
(2,2),(0.,0.005,0.01,0.015,0.02,0.025,0.03,0.035,0.04,0.045,0.05,0.055,
0.06,0.065,0.07,0.075,0.08,0.085,0.09,0.095,0.1,0.105,0.11,0.115,0.12,0.125,
0.13,0.135,0.14,0.145,0.15,0.155,0.16,0.165,0.17,0.175,0.18,0.185,0.19,
0.195,0.2,0.205,0.21,0.215,0.22,0.225,0.23,0.235,0.24,0.245,0.25,0.255,
0.26,0.265,0.27,0.275,0.28,0.285,0.29,0.295,0.3,0.305,0.31,0.315,0.32,0.325,
0.33,0.335,0.34,0.345,0.35,0.355,0.36,0.365,0.37,0.375,0.38,0.385,0.39,
0.395,0.4,0.405,0.41,0.415,0.42,0.425,0.43,0.435,0.44,0.445,0.45,0.455,
0.46,0.465,0.47,0.475,0.48,0.485,0.49,0.495,0.5,0.505,0.51,0.515,0.52,0.525,
0.53,0.535,0.54,0.545,0.55,0.555,0.56,0.565,0.57,0.575,0.58,0.585,0.59,
0.595,0.6,0.605,0.61,0.615,0.62,0.625,0.63,0.635,0.64,0.645,0.65,0.655,
0.66,0.665,0.67,0.675,0.68,0.685,0.690000000000001,0.695000000000001,0.700000000000001,
0.705000000000001,0.710000000000001,0.715000000000001,0.720000000000001,
0.725000000000001,0.730000000000001,0.735000000000001,0.740000000000001,
0.745000000000001,0.750000000000001,0.755000000000001,0.760000000000001,
0.765000000000001,0.770000000000001,0.775000000000001,0.780000000000001,
0.785000000000001,0.790000000000001,0.795000000000001,0.800000000000001,
0.805000000000001,0.810000000000001,0.815000000000001,0.820000000000001,
0.825000000000001,0.830000000000001,0.835000000000001,0.840000000000001,
0.845000000000001,0.850000000000001,0.855000000000001,0.860000000000001,
0.865000000000001,0.870000000000001,0.875000000000001,0.880000000000001,
0.885000000000001,0.890000000000001,0.895000000000001,0.900000000000001,
0.905000000000001,0.910000000000001,0.915000000000001,0.920000000000001,
0.925000000000001,0.930000000000001,0.935000000000001,0.940000000000001,
0.945000000000001,0.950000000000001,0.955000000000001,0.960000000000001,
0.965000000000001,0.970000000000001,0.975000000000001,0.980000000000001,
0.985000000000001,0.990000000000001,0.995000000000001,1.),(0.,1.2),
 .UNSPECIFIED.)
GEOMETRIC_REPRESENTATION_ITEM()
RATIONAL_B_SPLINE_SURFACE(((1.,1.),(1.,1.),(1.,1.),(1.,1.),(1.,1.),(1.,
1.),(1.,1.),(1.,1.),(1.,1.),(1.,1.),(1.,1.),(1.,1.),(1.,1.),(1.,1.),(1.,
1.),(1.,1.),(1.,1.),(1.,1.),(1.,1.),(1.,1.),(1.,1.),(1.,1.),(1.,1.),(1.,
1.),(1.,1.),(1.,1.),(1.,1.),(1.,1.),(1.,1.),(1.,1.),(1.,1.),(1.,1.),(1.,
1.),(1.,1.),(1.,1.),(1.,1.),(1.,1.),(1.,1.),(1.,1.),(1.,1.),(1.,1.),(1.,
1.),(1.,1.),(1.,1.),(1.,1.),(1.,1.),(1.,1.),(1.,1.),(1.,1.),(1.,1.),(1.,
1.),(1.,1.),(1.,1.),(1.,1.),(1.,1.),(1.,1.),(1.,1.),(1.,1.),(1.,1.),(1.,
1.),(1.,1.),(1.,1.),(1.,1.),(1.,1.),(1.,1.),(1.,1.),(1.,1.),(1.,1.),(1.,
1.),(1.,1.),(1.,1.),(1.,1.),(1.,1.),(1.,1.),(1.,1.),(1.,1.),(1.,1.),(1.,
1.),(1.,1.),(1.,1.),(1.,1.),(1.,1.),(1.,1.),(1.,1.),(1.,1.),(1.,1.),(1.,
1.),(1.,1.),(1.,1.),(1.,1.),(1.,1.),(1.,1.),(1.,1.),(1.,1.),(1.,1.),(1.,
1.),(1.,1.),(1.,1.),(1.,1.),(1.,1.),(1.,1.),(1.,1.),(1.,1.),(1.,1.),(1.,
1.),(1.,1.),(1.,1.),(1.,1.),(1.,1.),(1.,1.),(1.,1.),(1.,1.),(1.,1.),(1.,
1.),(1.,1.),(1.,1.),(1.,1.),(1.,1.),(1.,1.),(1.,1.),(1.,1.),(1.,1.),(1.,
1.),(1.,1.),(1.,1.),(1.,1.),(1.,1.),(1.,1.),(1.,1.),(1.,1.),(1.,1.),(1.,
1.),(1.,1.),(1.,1.),(1.,1.),(1.,1.),(1.,1.),(1.,1.),(1.,1.),(1.,1.),(1.,
1.),(1.,1.),(1.,1.),(1.,1.),(1.,1.),(1.,1.),(1.,1.),(1.,1.),(1.,1.),(1.,
1.),(1.,1.),(1.,1.),(1.,1.),(1.,1.),(1.,1.),(1.,1.),(1.,1.),(1.,1.),(1.,
1.),(1.,1.),(1.,1.),(1.,1.),(1.,1.),(1.,1.),(1.,1.),(1.,1.),(1.,1.),(1.,
1.),(1.,1.),(1.,1.),(1.,1.),(1.,1.),(1.,1.),(1.,1.),(1.,1.),(1.,1.),(1.,
1.),(1.,1.),(1.,1.),(1.,1.),(1.,1.),(1.,1.),(1.,1.),(1.,1.),(1.,1.),(1.,
1.),(1.,1.),(1.,1.),(1.,1.),(1.,1.),(1.,1.),(1.,1.),(1.,1.),(1.,1.),(1.,
1.),(1.,1.),(1.,1.),(1.,1.),(1.,1.),(1.,1.),(1.,1.),(1.,1.),(1.,1.),(1.,
1.),(1.,1.)))
REPRESENTATION_ITEM('')
SURFACE()
);
#936=(
BOUNDED_SURFACE()
B_SPLINE_SURFACE(5,1,((#100110,#100111),(#100112,#100113),(#100114,#100115),
(#100116,#100117),(#100118,#100119),(#100120,#100121),(#100122,#100123),
(#100124,#100125),(#100126,#100127),(#100128,#100129),(#100130,#100131),
(#100132,#100133),(#100134,#100135),(#100136,#100137),(#100138,#100139),
(#100140,#100141),(#100142,#100143),(#100144,#100145),(#100146,#100147),
(#100148,#100149),(#100150,#100151),(#100152,#100153),(#100154,#100155),
(#100156,#100157),(#100158,#100159),(#100160,#100161),(#100162,#100163),
(#100164,#100165),(#100166,#100167),(#100168,#100169),(#100170,#100171),
(#100172,#100173),(#100174,#100175),(#100176,#100177),(#100178,#100179),
(#100180,#100181),(#100182,#100183),(#100184,#100185),(#100186,#100187),
(#100188,#100189),(#100190,#100191),(#100192,#100193),(#100194,#100195),
(#100196,#100197),(#100198,#100199),(#100200,#100201),(#100202,#100203),
(#100204,#100205),(#100206,#100207),(#100208,#100209),(#100210,#100211),
(#100212,#100213),(#100214,#100215),(#100216,#100217),(#100218,#100219),
(#100220,#100221),(#100222,#100223),(#100224,#100225),(#100226,#100227),
(#100228,#100229),(#100230,#100231),(#100232,#100233),(#100234,#100235),
(#100236,#100237),(#100238,#100239),(#100240,#100241),(#100242,#100243),
(#100244,#100245),(#100246,#100247),(#100248,#100249),(#100250,#100251),
(#100252,#100253),(#100254,#100255),(#100256,#100257),(#100258,#100259),
(#100260,#100261),(#100262,#100263),(#100264,#100265),(#100266,#100267),
(#100268,#100269),(#100270,#100271),(#100272,#100273),(#100274,#100275),
(#100276,#100277),(#100278,#100279),(#100280,#100281),(#100282,#100283),
(#100284,#100285),(#100286,#100287),(#100288,#100289),(#100290,#100291),
(#100292,#100293),(#100294,#100295),(#100296,#100297),(#100298,#100299),
(#100300,#100301),(#100302,#100303),(#100304,#100305),(#100306,#100307),
(#100308,#100309),(#100310,#100311),(#100312,#100313),(#100314,#100315),
(#100316,#100317),(#100318,#100319),(#100320,#100321),(#100322,#100323),
(#100324,#100325),(#100326,#100327),(#100328,#100329),(#100330,#100331),
(#100332,#100333),(#100334,#100335),(#100336,#100337),(#100338,#100339),
(#100340,#100341),(#100342,#100343),(#100344,#100345),(#100346,#100347),
(#100348,#100349),(#100350,#100351),(#100352,#100353),(#100354,#100355),
(#100356,#100357),(#100358,#100359),(#100360,#100361),(#100362,#100363),
(#100364,#100365),(#100366,#100367),(#100368,#100369),(#100370,#100371),
(#100372,#100373),(#100374,#100375),(#100376,#100377),(#100378,#100379),
(#100380,#100381),(#100382,#100383),(#100384,#100385),(#100386,#100387),
(#100388,#100389),(#100390,#100391),(#100392,#100393),(#100394,#100395),
(#100396,#100397),(#100398,#100399),(#100400,#100401),(#100402,#100403),
(#100404,#100405),(#100406,#100407),(#100408,#100409),(#100410,#100411),
(#100412,#100413),(#100414,#100415),(#100416,#100417),(#100418,#100419),
(#100420,#100421),(#100422,#100423),(#100424,#100425),(#100426,#100427),
(#100428,#100429),(#100430,#100431),(#100432,#100433),(#100434,#100435),
(#100436,#100437),(#100438,#100439),(#100440,#100441),(#100442,#100443),
(#100444,#100445),(#100446,#100447),(#100448,#100449),(#100450,#100451),
(#100452,#100453),(#100454,#100455),(#100456,#100457),(#100458,#100459),
(#100460,#100461),(#100462,#100463),(#100464,#100465),(#100466,#100467),
(#100468,#100469),(#100470,#100471),(#100472,#100473),(#100474,#100475),
(#100476,#100477),(#100478,#100479),(#100480,#100481),(#100482,#100483),
(#100484,#100485),(#100486,#100487),(#100488,#100489),(#100490,#100491),
(#100492,#100493),(#100494,#100495),(#100496,#100497),(#100498,#100499),
(#100500,#100501),(#100502,#100503),(#100504,#100505),(#100506,#100507),
(#100508,#100509),(#100510,#100511),(#100512,#100513),(#100514,#100515),
(#100516,#100517),(#100518,#100519)),.UNSPECIFIED.,.F.,.F.,.F.)
B_SPLINE_SURFACE_WITH_KNOTS((6,1,1,1,1,1,1,1,1,1,1,1,1,1,1,1,1,1,1,1,1,
1,1,1,1,1,1,1,1,1,1,1,1,1,1,1,1,1,1,1,1,1,1,1,1,1,1,1,1,1,1,1,1,1,1,1,1,
1,1,1,1,1,1,1,1,1,1,1,1,1,1,1,1,1,1,1,1,1,1,1,1,1,1,1,1,1,1,1,1,1,1,1,1,
1,1,1,1,1,1,1,1,1,1,1,1,1,1,1,1,1,1,1,1,1,1,1,1,1,1,1,1,1,1,1,1,1,1,1,1,
1,1,1,1,1,1,1,1,1,1,1,1,1,1,1,1,1,1,1,1,1,1,1,1,1,1,1,1,1,1,1,1,1,1,1,1,
1,1,1,1,1,1,1,1,1,1,1,1,1,1,1,1,1,1,1,1,1,1,1,1,1,1,1,1,1,1,1,1,1,1,1,6),
(2,2),(0.,0.005,0.01,0.015,0.02,0.025,0.03,0.035,0.04,0.045,0.05,0.055,
0.06,0.065,0.07,0.075,0.08,0.085,0.09,0.095,0.1,0.105,0.11,0.115,0.12,0.125,
0.13,0.135,0.14,0.145,0.15,0.155,0.16,0.165,0.17,0.175,0.18,0.185,0.19,
0.195,0.2,0.205,0.21,0.215,0.22,0.225,0.23,0.235,0.24,0.245,0.25,0.255,
0.26,0.265,0.27,0.275,0.28,0.285,0.29,0.295,0.3,0.305,0.31,0.315,0.32,0.325,
0.33,0.335,0.34,0.345,0.35,0.355,0.36,0.365,0.37,0.375,0.38,0.385,0.39,
0.395,0.4,0.405,0.41,0.415,0.42,0.425,0.43,0.435,0.44,0.445,0.45,0.455,
0.46,0.465,0.47,0.475,0.48,0.485,0.49,0.495,0.5,0.505,0.51,0.515,0.52,0.525,
0.53,0.535,0.54,0.545,0.55,0.555,0.56,0.565,0.57,0.575,0.58,0.585,0.59,
0.595,0.6,0.605,0.61,0.615,0.62,0.625,0.63,0.635,0.64,0.645,0.65,0.655,
0.66,0.665,0.67,0.675,0.68,0.685,0.690000000000001,0.695000000000001,0.700000000000001,
0.705000000000001,0.710000000000001,0.715000000000001,0.720000000000001,
0.725000000000001,0.730000000000001,0.735000000000001,0.740000000000001,
0.745000000000001,0.750000000000001,0.755000000000001,0.760000000000001,
0.765000000000001,0.770000000000001,0.775000000000001,0.780000000000001,
0.785000000000001,0.790000000000001,0.795000000000001,0.800000000000001,
0.805000000000001,0.810000000000001,0.815000000000001,0.820000000000001,
0.825000000000001,0.830000000000001,0.835000000000001,0.840000000000001,
0.845000000000001,0.850000000000001,0.855000000000001,0.860000000000001,
0.865000000000001,0.870000000000001,0.875000000000001,0.880000000000001,
0.885000000000001,0.890000000000001,0.895000000000001,0.900000000000001,
0.905000000000001,0.910000000000001,0.915000000000001,0.920000000000001,
0.925000000000001,0.930000000000001,0.935000000000001,0.940000000000001,
0.945000000000001,0.950000000000001,0.955000000000001,0.960000000000001,
0.965000000000001,0.970000000000001,0.975000000000001,0.980000000000001,
0.985000000000001,0.990000000000001,0.995000000000001,1.),(0.,1.2),
 .UNSPECIFIED.)
GEOMETRIC_REPRESENTATION_ITEM()
RATIONAL_B_SPLINE_SURFACE(((1.,1.),(1.,1.),(1.,1.),(1.,1.),(1.,1.),(1.,
1.),(1.,1.),(1.,1.),(1.,1.),(1.,1.),(1.,1.),(1.,1.),(1.,1.),(1.,1.),(1.,
1.),(1.,1.),(1.,1.),(1.,1.),(1.,1.),(1.,1.),(1.,1.),(1.,1.),(1.,1.),(1.,
1.),(1.,1.),(1.,1.),(1.,1.),(1.,1.),(1.,1.),(1.,1.),(1.,1.),(1.,1.),(1.,
1.),(1.,1.),(1.,1.),(1.,1.),(1.,1.),(1.,1.),(1.,1.),(1.,1.),(1.,1.),(1.,
1.),(1.,1.),(1.,1.),(1.,1.),(1.,1.),(1.,1.),(1.,1.),(1.,1.),(1.,1.),(1.,
1.),(1.,1.),(1.,1.),(1.,1.),(1.,1.),(1.,1.),(1.,1.),(1.,1.),(1.,1.),(1.,
1.),(1.,1.),(1.,1.),(1.,1.),(1.,1.),(1.,1.),(1.,1.),(1.,1.),(1.,1.),(1.,
1.),(1.,1.),(1.,1.),(1.,1.),(1.,1.),(1.,1.),(1.,1.),(1.,1.),(1.,1.),(1.,
1.),(1.,1.),(1.,1.),(1.,1.),(1.,1.),(1.,1.),(1.,1.),(1.,1.),(1.,1.),(1.,
1.),(1.,1.),(1.,1.),(1.,1.),(1.,1.),(1.,1.),(1.,1.),(1.,1.),(1.,1.),(1.,
1.),(1.,1.),(1.,1.),(1.,1.),(1.,1.),(1.,1.),(1.,1.),(1.,1.),(1.,1.),(1.,
1.),(1.,1.),(1.,1.),(1.,1.),(1.,1.),(1.,1.),(1.,1.),(1.,1.),(1.,1.),(1.,
1.),(1.,1.),(1.,1.),(1.,1.),(1.,1.),(1.,1.),(1.,1.),(1.,1.),(1.,1.),(1.,
1.),(1.,1.),(1.,1.),(1.,1.),(1.,1.),(1.,1.),(1.,1.),(1.,1.),(1.,1.),(1.,
1.),(1.,1.),(1.,1.),(1.,1.),(1.,1.),(1.,1.),(1.,1.),(1.,1.),(1.,1.),(1.,
1.),(1.,1.),(1.,1.),(1.,1.),(1.,1.),(1.,1.),(1.,1.),(1.,1.),(1.,1.),(1.,
1.),(1.,1.),(1.,1.),(1.,1.),(1.,1.),(1.,1.),(1.,1.),(1.,1.),(1.,1.),(1.,
1.),(1.,1.),(1.,1.),(1.,1.),(1.,1.),(1.,1.),(1.,1.),(1.,1.),(1.,1.),(1.,
1.),(1.,1.),(1.,1.),(1.,1.),(1.,1.),(1.,1.),(1.,1.),(1.,1.),(1.,1.),(1.,
1.),(1.,1.),(1.,1.),(1.,1.),(1.,1.),(1.,1.),(1.,1.),(1.,1.),(1.,1.),(1.,
1.),(1.,1.),(1.,1.),(1.,1.),(1.,1.),(1.,1.),(1.,1.),(1.,1.),(1.,1.),(1.,
1.),(1.,1.),(1.,1.),(1.,1.),(1.,1.),(1.,1.),(1.,1.),(1.,1.),(1.,1.),(1.,
1.),(1.,1.)))
REPRESENTATION_ITEM('')
SURFACE()
);
#937=(
BOUNDED_SURFACE()
B_SPLINE_SURFACE(5,1,((#101006,#101007),(#101008,#101009),(#101010,#101011),
(#101012,#101013),(#101014,#101015),(#101016,#101017),(#101018,#101019),
(#101020,#101021),(#101022,#101023),(#101024,#101025),(#101026,#101027),
(#101028,#101029),(#101030,#101031),(#101032,#101033),(#101034,#101035),
(#101036,#101037),(#101038,#101039),(#101040,#101041),(#101042,#101043),
(#101044,#101045),(#101046,#101047),(#101048,#101049),(#101050,#101051),
(#101052,#101053),(#101054,#101055),(#101056,#101057),(#101058,#101059),
(#101060,#101061),(#101062,#101063),(#101064,#101065),(#101066,#101067),
(#101068,#101069),(#101070,#101071),(#101072,#101073),(#101074,#101075),
(#101076,#101077),(#101078,#101079),(#101080,#101081),(#101082,#101083),
(#101084,#101085),(#101086,#101087),(#101088,#101089),(#101090,#101091),
(#101092,#101093),(#101094,#101095),(#101096,#101097),(#101098,#101099),
(#101100,#101101),(#101102,#101103),(#101104,#101105),(#101106,#101107),
(#101108,#101109),(#101110,#101111),(#101112,#101113),(#101114,#101115),
(#101116,#101117),(#101118,#101119),(#101120,#101121),(#101122,#101123),
(#101124,#101125),(#101126,#101127),(#101128,#101129),(#101130,#101131),
(#101132,#101133),(#101134,#101135),(#101136,#101137),(#101138,#101139),
(#101140,#101141),(#101142,#101143),(#101144,#101145),(#101146,#101147),
(#101148,#101149),(#101150,#101151),(#101152,#101153),(#101154,#101155),
(#101156,#101157),(#101158,#101159),(#101160,#101161),(#101162,#101163),
(#101164,#101165),(#101166,#101167),(#101168,#101169),(#101170,#101171),
(#101172,#101173),(#101174,#101175),(#101176,#101177),(#101178,#101179),
(#101180,#101181),(#101182,#101183),(#101184,#101185),(#101186,#101187),
(#101188,#101189),(#101190,#101191),(#101192,#101193),(#101194,#101195),
(#101196,#101197),(#101198,#101199),(#101200,#101201),(#101202,#101203),
(#101204,#101205),(#101206,#101207),(#101208,#101209),(#101210,#101211),
(#101212,#101213),(#101214,#101215),(#101216,#101217),(#101218,#101219),
(#101220,#101221),(#101222,#101223),(#101224,#101225),(#101226,#101227),
(#101228,#101229),(#101230,#101231),(#101232,#101233),(#101234,#101235),
(#101236,#101237),(#101238,#101239),(#101240,#101241),(#101242,#101243),
(#101244,#101245),(#101246,#101247),(#101248,#101249),(#101250,#101251),
(#101252,#101253),(#101254,#101255),(#101256,#101257),(#101258,#101259),
(#101260,#101261),(#101262,#101263),(#101264,#101265),(#101266,#101267),
(#101268,#101269),(#101270,#101271),(#101272,#101273),(#101274,#101275),
(#101276,#101277),(#101278,#101279),(#101280,#101281),(#101282,#101283),
(#101284,#101285),(#101286,#101287),(#101288,#101289),(#101290,#101291),
(#101292,#101293),(#101294,#101295),(#101296,#101297),(#101298,#101299),
(#101300,#101301),(#101302,#101303),(#101304,#101305),(#101306,#101307),
(#101308,#101309),(#101310,#101311),(#101312,#101313),(#101314,#101315),
(#101316,#101317),(#101318,#101319),(#101320,#101321),(#101322,#101323),
(#101324,#101325),(#101326,#101327),(#101328,#101329),(#101330,#101331),
(#101332,#101333),(#101334,#101335),(#101336,#101337),(#101338,#101339),
(#101340,#101341),(#101342,#101343),(#101344,#101345),(#101346,#101347),
(#101348,#101349),(#101350,#101351),(#101352,#101353),(#101354,#101355),
(#101356,#101357),(#101358,#101359),(#101360,#101361),(#101362,#101363),
(#101364,#101365),(#101366,#101367),(#101368,#101369),(#101370,#101371),
(#101372,#101373),(#101374,#101375),(#101376,#101377),(#101378,#101379),
(#101380,#101381),(#101382,#101383),(#101384,#101385),(#101386,#101387),
(#101388,#101389),(#101390,#101391),(#101392,#101393),(#101394,#101395),
(#101396,#101397),(#101398,#101399),(#101400,#101401),(#101402,#101403),
(#101404,#101405),(#101406,#101407),(#101408,#101409),(#101410,#101411),
(#101412,#101413),(#101414,#101415)),.UNSPECIFIED.,.F.,.F.,.F.)
B_SPLINE_SURFACE_WITH_KNOTS((6,1,1,1,1,1,1,1,1,1,1,1,1,1,1,1,1,1,1,1,1,
1,1,1,1,1,1,1,1,1,1,1,1,1,1,1,1,1,1,1,1,1,1,1,1,1,1,1,1,1,1,1,1,1,1,1,1,
1,1,1,1,1,1,1,1,1,1,1,1,1,1,1,1,1,1,1,1,1,1,1,1,1,1,1,1,1,1,1,1,1,1,1,1,
1,1,1,1,1,1,1,1,1,1,1,1,1,1,1,1,1,1,1,1,1,1,1,1,1,1,1,1,1,1,1,1,1,1,1,1,
1,1,1,1,1,1,1,1,1,1,1,1,1,1,1,1,1,1,1,1,1,1,1,1,1,1,1,1,1,1,1,1,1,1,1,1,
1,1,1,1,1,1,1,1,1,1,1,1,1,1,1,1,1,1,1,1,1,1,1,1,1,1,1,1,1,1,1,1,1,1,1,6),
(2,2),(0.,0.005,0.01,0.015,0.02,0.025,0.03,0.035,0.04,0.045,0.05,0.055,
0.06,0.065,0.07,0.075,0.08,0.085,0.09,0.095,0.1,0.105,0.11,0.115,0.12,0.125,
0.13,0.135,0.14,0.145,0.15,0.155,0.16,0.165,0.17,0.175,0.18,0.185,0.19,
0.195,0.2,0.205,0.21,0.215,0.22,0.225,0.23,0.235,0.24,0.245,0.25,0.255,
0.26,0.265,0.27,0.275,0.28,0.285,0.29,0.295,0.3,0.305,0.31,0.315,0.32,0.325,
0.33,0.335,0.34,0.345,0.35,0.355,0.36,0.365,0.37,0.375,0.38,0.385,0.39,
0.395,0.4,0.405,0.41,0.415,0.42,0.425,0.43,0.435,0.44,0.445,0.45,0.455,
0.46,0.465,0.47,0.475,0.48,0.485,0.49,0.495,0.5,0.505,0.51,0.515,0.52,0.525,
0.53,0.535,0.54,0.545,0.55,0.555,0.56,0.565,0.57,0.575,0.58,0.585,0.59,
0.595,0.6,0.605,0.61,0.615,0.62,0.625,0.63,0.635,0.64,0.645,0.65,0.655,
0.66,0.665,0.67,0.675,0.68,0.685,0.690000000000001,0.695000000000001,0.700000000000001,
0.705000000000001,0.710000000000001,0.715000000000001,0.720000000000001,
0.725000000000001,0.730000000000001,0.735000000000001,0.740000000000001,
0.745000000000001,0.750000000000001,0.755000000000001,0.760000000000001,
0.765000000000001,0.770000000000001,0.775000000000001,0.780000000000001,
0.785000000000001,0.790000000000001,0.795000000000001,0.800000000000001,
0.805000000000001,0.810000000000001,0.815000000000001,0.820000000000001,
0.825000000000001,0.830000000000001,0.835000000000001,0.840000000000001,
0.845000000000001,0.850000000000001,0.855000000000001,0.860000000000001,
0.865000000000001,0.870000000000001,0.875000000000001,0.880000000000001,
0.885000000000001,0.890000000000001,0.895000000000001,0.900000000000001,
0.905000000000001,0.910000000000001,0.915000000000001,0.920000000000001,
0.925000000000001,0.930000000000001,0.935000000000001,0.940000000000001,
0.945000000000001,0.950000000000001,0.955000000000001,0.960000000000001,
0.965000000000001,0.970000000000001,0.975000000000001,0.980000000000001,
0.985000000000001,0.990000000000001,0.995000000000001,1.),(0.,1.2),
 .UNSPECIFIED.)
GEOMETRIC_REPRESENTATION_ITEM()
RATIONAL_B_SPLINE_SURFACE(((1.,1.),(1.,1.),(1.,1.),(1.,1.),(1.,1.),(1.,
1.),(1.,1.),(1.,1.),(1.,1.),(1.,1.),(1.,1.),(1.,1.),(1.,1.),(1.,1.),(1.,
1.),(1.,1.),(1.,1.),(1.,1.),(1.,1.),(1.,1.),(1.,1.),(1.,1.),(1.,1.),(1.,
1.),(1.,1.),(1.,1.),(1.,1.),(1.,1.),(1.,1.),(1.,1.),(1.,1.),(1.,1.),(1.,
1.),(1.,1.),(1.,1.),(1.,1.),(1.,1.),(1.,1.),(1.,1.),(1.,1.),(1.,1.),(1.,
1.),(1.,1.),(1.,1.),(1.,1.),(1.,1.),(1.,1.),(1.,1.),(1.,1.),(1.,1.),(1.,
1.),(1.,1.),(1.,1.),(1.,1.),(1.,1.),(1.,1.),(1.,1.),(1.,1.),(1.,1.),(1.,
1.),(1.,1.),(1.,1.),(1.,1.),(1.,1.),(1.,1.),(1.,1.),(1.,1.),(1.,1.),(1.,
1.),(1.,1.),(1.,1.),(1.,1.),(1.,1.),(1.,1.),(1.,1.),(1.,1.),(1.,1.),(1.,
1.),(1.,1.),(1.,1.),(1.,1.),(1.,1.),(1.,1.),(1.,1.),(1.,1.),(1.,1.),(1.,
1.),(1.,1.),(1.,1.),(1.,1.),(1.,1.),(1.,1.),(1.,1.),(1.,1.),(1.,1.),(1.,
1.),(1.,1.),(1.,1.),(1.,1.),(1.,1.),(1.,1.),(1.,1.),(1.,1.),(1.,1.),(1.,
1.),(1.,1.),(1.,1.),(1.,1.),(1.,1.),(1.,1.),(1.,1.),(1.,1.),(1.,1.),(1.,
1.),(1.,1.),(1.,1.),(1.,1.),(1.,1.),(1.,1.),(1.,1.),(1.,1.),(1.,1.),(1.,
1.),(1.,1.),(1.,1.),(1.,1.),(1.,1.),(1.,1.),(1.,1.),(1.,1.),(1.,1.),(1.,
1.),(1.,1.),(1.,1.),(1.,1.),(1.,1.),(1.,1.),(1.,1.),(1.,1.),(1.,1.),(1.,
1.),(1.,1.),(1.,1.),(1.,1.),(1.,1.),(1.,1.),(1.,1.),(1.,1.),(1.,1.),(1.,
1.),(1.,1.),(1.,1.),(1.,1.),(1.,1.),(1.,1.),(1.,1.),(1.,1.),(1.,1.),(1.,
1.),(1.,1.),(1.,1.),(1.,1.),(1.,1.),(1.,1.),(1.,1.),(1.,1.),(1.,1.),(1.,
1.),(1.,1.),(1.,1.),(1.,1.),(1.,1.),(1.,1.),(1.,1.),(1.,1.),(1.,1.),(1.,
1.),(1.,1.),(1.,1.),(1.,1.),(1.,1.),(1.,1.),(1.,1.),(1.,1.),(1.,1.),(1.,
1.),(1.,1.),(1.,1.),(1.,1.),(1.,1.),(1.,1.),(1.,1.),(1.,1.),(1.,1.),(1.,
1.),(1.,1.),(1.,1.),(1.,1.),(1.,1.),(1.,1.),(1.,1.),(1.,1.),(1.,1.),(1.,
1.),(1.,1.)))
REPRESENTATION_ITEM('')
SURFACE()
);
#938=(
BOUNDED_SURFACE()
B_SPLINE_SURFACE(5,1,((#101902,#101903),(#101904,#101905),(#101906,#101907),
(#101908,#101909),(#101910,#101911),(#101912,#101913),(#101914,#101915),
(#101916,#101917),(#101918,#101919),(#101920,#101921),(#101922,#101923),
(#101924,#101925),(#101926,#101927),(#101928,#101929),(#101930,#101931),
(#101932,#101933),(#101934,#101935),(#101936,#101937),(#101938,#101939),
(#101940,#101941),(#101942,#101943),(#101944,#101945),(#101946,#101947),
(#101948,#101949),(#101950,#101951),(#101952,#101953),(#101954,#101955),
(#101956,#101957),(#101958,#101959),(#101960,#101961),(#101962,#101963),
(#101964,#101965),(#101966,#101967),(#101968,#101969),(#101970,#101971),
(#101972,#101973),(#101974,#101975),(#101976,#101977),(#101978,#101979),
(#101980,#101981),(#101982,#101983),(#101984,#101985),(#101986,#101987),
(#101988,#101989),(#101990,#101991),(#101992,#101993),(#101994,#101995),
(#101996,#101997),(#101998,#101999),(#102000,#102001),(#102002,#102003),
(#102004,#102005),(#102006,#102007),(#102008,#102009),(#102010,#102011),
(#102012,#102013),(#102014,#102015),(#102016,#102017),(#102018,#102019),
(#102020,#102021),(#102022,#102023),(#102024,#102025),(#102026,#102027),
(#102028,#102029),(#102030,#102031),(#102032,#102033),(#102034,#102035),
(#102036,#102037),(#102038,#102039),(#102040,#102041),(#102042,#102043),
(#102044,#102045),(#102046,#102047),(#102048,#102049),(#102050,#102051),
(#102052,#102053),(#102054,#102055),(#102056,#102057),(#102058,#102059),
(#102060,#102061),(#102062,#102063),(#102064,#102065),(#102066,#102067),
(#102068,#102069),(#102070,#102071),(#102072,#102073),(#102074,#102075),
(#102076,#102077),(#102078,#102079),(#102080,#102081),(#102082,#102083),
(#102084,#102085),(#102086,#102087),(#102088,#102089),(#102090,#102091),
(#102092,#102093),(#102094,#102095),(#102096,#102097),(#102098,#102099),
(#102100,#102101),(#102102,#102103),(#102104,#102105),(#102106,#102107),
(#102108,#102109),(#102110,#102111),(#102112,#102113),(#102114,#102115),
(#102116,#102117),(#102118,#102119),(#102120,#102121),(#102122,#102123),
(#102124,#102125),(#102126,#102127),(#102128,#102129),(#102130,#102131),
(#102132,#102133),(#102134,#102135),(#102136,#102137),(#102138,#102139),
(#102140,#102141),(#102142,#102143),(#102144,#102145),(#102146,#102147),
(#102148,#102149),(#102150,#102151),(#102152,#102153),(#102154,#102155),
(#102156,#102157),(#102158,#102159),(#102160,#102161),(#102162,#102163),
(#102164,#102165),(#102166,#102167),(#102168,#102169),(#102170,#102171),
(#102172,#102173),(#102174,#102175),(#102176,#102177),(#102178,#102179),
(#102180,#102181),(#102182,#102183),(#102184,#102185),(#102186,#102187),
(#102188,#102189),(#102190,#102191),(#102192,#102193),(#102194,#102195),
(#102196,#102197),(#102198,#102199),(#102200,#102201),(#102202,#102203),
(#102204,#102205),(#102206,#102207),(#102208,#102209),(#102210,#102211),
(#102212,#102213),(#102214,#102215),(#102216,#102217),(#102218,#102219),
(#102220,#102221),(#102222,#102223),(#102224,#102225),(#102226,#102227),
(#102228,#102229),(#102230,#102231),(#102232,#102233),(#102234,#102235),
(#102236,#102237),(#102238,#102239),(#102240,#102241),(#102242,#102243),
(#102244,#102245),(#102246,#102247),(#102248,#102249),(#102250,#102251),
(#102252,#102253),(#102254,#102255),(#102256,#102257),(#102258,#102259),
(#102260,#102261),(#102262,#102263),(#102264,#102265),(#102266,#102267),
(#102268,#102269),(#102270,#102271),(#102272,#102273),(#102274,#102275),
(#102276,#102277),(#102278,#102279),(#102280,#102281),(#102282,#102283),
(#102284,#102285),(#102286,#102287),(#102288,#102289),(#102290,#102291),
(#102292,#102293),(#102294,#102295),(#102296,#102297),(#102298,#102299),
(#102300,#102301),(#102302,#102303),(#102304,#102305),(#102306,#102307),
(#102308,#102309),(#102310,#102311)),.UNSPECIFIED.,.F.,.F.,.F.)
B_SPLINE_SURFACE_WITH_KNOTS((6,1,1,1,1,1,1,1,1,1,1,1,1,1,1,1,1,1,1,1,1,
1,1,1,1,1,1,1,1,1,1,1,1,1,1,1,1,1,1,1,1,1,1,1,1,1,1,1,1,1,1,1,1,1,1,1,1,
1,1,1,1,1,1,1,1,1,1,1,1,1,1,1,1,1,1,1,1,1,1,1,1,1,1,1,1,1,1,1,1,1,1,1,1,
1,1,1,1,1,1,1,1,1,1,1,1,1,1,1,1,1,1,1,1,1,1,1,1,1,1,1,1,1,1,1,1,1,1,1,1,
1,1,1,1,1,1,1,1,1,1,1,1,1,1,1,1,1,1,1,1,1,1,1,1,1,1,1,1,1,1,1,1,1,1,1,1,
1,1,1,1,1,1,1,1,1,1,1,1,1,1,1,1,1,1,1,1,1,1,1,1,1,1,1,1,1,1,1,1,1,1,1,6),
(2,2),(0.,0.005,0.01,0.015,0.02,0.025,0.03,0.035,0.04,0.045,0.05,0.055,
0.06,0.065,0.07,0.075,0.08,0.085,0.09,0.095,0.1,0.105,0.11,0.115,0.12,0.125,
0.13,0.135,0.14,0.145,0.15,0.155,0.16,0.165,0.17,0.175,0.18,0.185,0.19,
0.195,0.2,0.205,0.21,0.215,0.22,0.225,0.23,0.235,0.24,0.245,0.25,0.255,
0.26,0.265,0.27,0.275,0.28,0.285,0.29,0.295,0.3,0.305,0.31,0.315,0.32,0.325,
0.33,0.335,0.34,0.345,0.35,0.355,0.36,0.365,0.37,0.375,0.38,0.385,0.39,
0.395,0.4,0.405,0.41,0.415,0.42,0.425,0.43,0.435,0.44,0.445,0.45,0.455,
0.46,0.465,0.47,0.475,0.48,0.485,0.49,0.495,0.5,0.505,0.51,0.515,0.52,0.525,
0.53,0.535,0.54,0.545,0.55,0.555,0.56,0.565,0.57,0.575,0.58,0.585,0.59,
0.595,0.6,0.605,0.61,0.615,0.62,0.625,0.63,0.635,0.64,0.645,0.65,0.655,
0.66,0.665,0.67,0.675,0.68,0.685,0.690000000000001,0.695000000000001,0.700000000000001,
0.705000000000001,0.710000000000001,0.715000000000001,0.720000000000001,
0.725000000000001,0.730000000000001,0.735000000000001,0.740000000000001,
0.745000000000001,0.750000000000001,0.755000000000001,0.760000000000001,
0.765000000000001,0.770000000000001,0.775000000000001,0.780000000000001,
0.785000000000001,0.790000000000001,0.795000000000001,0.800000000000001,
0.805000000000001,0.810000000000001,0.815000000000001,0.820000000000001,
0.825000000000001,0.830000000000001,0.835000000000001,0.840000000000001,
0.845000000000001,0.850000000000001,0.855000000000001,0.860000000000001,
0.865000000000001,0.870000000000001,0.875000000000001,0.880000000000001,
0.885000000000001,0.890000000000001,0.895000000000001,0.900000000000001,
0.905000000000001,0.910000000000001,0.915000000000001,0.920000000000001,
0.925000000000001,0.930000000000001,0.935000000000001,0.940000000000001,
0.945000000000001,0.950000000000001,0.955000000000001,0.960000000000001,
0.965000000000001,0.970000000000001,0.975000000000001,0.980000000000001,
0.985000000000001,0.990000000000001,0.995000000000001,1.),(0.,1.2),
 .UNSPECIFIED.)
GEOMETRIC_REPRESENTATION_ITEM()
RATIONAL_B_SPLINE_SURFACE(((1.,1.),(1.,1.),(1.,1.),(1.,1.),(1.,1.),(1.,
1.),(1.,1.),(1.,1.),(1.,1.),(1.,1.),(1.,1.),(1.,1.),(1.,1.),(1.,1.),(1.,
1.),(1.,1.),(1.,1.),(1.,1.),(1.,1.),(1.,1.),(1.,1.),(1.,1.),(1.,1.),(1.,
1.),(1.,1.),(1.,1.),(1.,1.),(1.,1.),(1.,1.),(1.,1.),(1.,1.),(1.,1.),(1.,
1.),(1.,1.),(1.,1.),(1.,1.),(1.,1.),(1.,1.),(1.,1.),(1.,1.),(1.,1.),(1.,
1.),(1.,1.),(1.,1.),(1.,1.),(1.,1.),(1.,1.),(1.,1.),(1.,1.),(1.,1.),(1.,
1.),(1.,1.),(1.,1.),(1.,1.),(1.,1.),(1.,1.),(1.,1.),(1.,1.),(1.,1.),(1.,
1.),(1.,1.),(1.,1.),(1.,1.),(1.,1.),(1.,1.),(1.,1.),(1.,1.),(1.,1.),(1.,
1.),(1.,1.),(1.,1.),(1.,1.),(1.,1.),(1.,1.),(1.,1.),(1.,1.),(1.,1.),(1.,
1.),(1.,1.),(1.,1.),(1.,1.),(1.,1.),(1.,1.),(1.,1.),(1.,1.),(1.,1.),(1.,
1.),(1.,1.),(1.,1.),(1.,1.),(1.,1.),(1.,1.),(1.,1.),(1.,1.),(1.,1.),(1.,
1.),(1.,1.),(1.,1.),(1.,1.),(1.,1.),(1.,1.),(1.,1.),(1.,1.),(1.,1.),(1.,
1.),(1.,1.),(1.,1.),(1.,1.),(1.,1.),(1.,1.),(1.,1.),(1.,1.),(1.,1.),(1.,
1.),(1.,1.),(1.,1.),(1.,1.),(1.,1.),(1.,1.),(1.,1.),(1.,1.),(1.,1.),(1.,
1.),(1.,1.),(1.,1.),(1.,1.),(1.,1.),(1.,1.),(1.,1.),(1.,1.),(1.,1.),(1.,
1.),(1.,1.),(1.,1.),(1.,1.),(1.,1.),(1.,1.),(1.,1.),(1.,1.),(1.,1.),(1.,
1.),(1.,1.),(1.,1.),(1.,1.),(1.,1.),(1.,1.),(1.,1.),(1.,1.),(1.,1.),(1.,
1.),(1.,1.),(1.,1.),(1.,1.),(1.,1.),(1.,1.),(1.,1.),(1.,1.),(1.,1.),(1.,
1.),(1.,1.),(1.,1.),(1.,1.),(1.,1.),(1.,1.),(1.,1.),(1.,1.),(1.,1.),(1.,
1.),(1.,1.),(1.,1.),(1.,1.),(1.,1.),(1.,1.),(1.,1.),(1.,1.),(1.,1.),(1.,
1.),(1.,1.),(1.,1.),(1.,1.),(1.,1.),(1.,1.),(1.,1.),(1.,1.),(1.,1.),(1.,
1.),(1.,1.),(1.,1.),(1.,1.),(1.,1.),(1.,1.),(1.,1.),(1.,1.),(1.,1.),(1.,
1.),(1.,1.),(1.,1.),(1.,1.),(1.,1.),(1.,1.),(1.,1.),(1.,1.),(1.,1.),(1.,
1.),(1.,1.)))
REPRESENTATION_ITEM('')
SURFACE()
);
#939=(
BOUNDED_SURFACE()
B_SPLINE_SURFACE(5,1,((#102798,#102799),(#102800,#102801),(#102802,#102803),
(#102804,#102805),(#102806,#102807),(#102808,#102809),(#102810,#102811),
(#102812,#102813),(#102814,#102815),(#102816,#102817),(#102818,#102819),
(#102820,#102821),(#102822,#102823),(#102824,#102825),(#102826,#102827),
(#102828,#102829),(#102830,#102831),(#102832,#102833),(#102834,#102835),
(#102836,#102837),(#102838,#102839),(#102840,#102841),(#102842,#102843),
(#102844,#102845),(#102846,#102847),(#102848,#102849),(#102850,#102851),
(#102852,#102853),(#102854,#102855),(#102856,#102857),(#102858,#102859),
(#102860,#102861),(#102862,#102863),(#102864,#102865),(#102866,#102867),
(#102868,#102869),(#102870,#102871),(#102872,#102873),(#102874,#102875),
(#102876,#102877),(#102878,#102879),(#102880,#102881),(#102882,#102883),
(#102884,#102885),(#102886,#102887),(#102888,#102889),(#102890,#102891),
(#102892,#102893),(#102894,#102895),(#102896,#102897),(#102898,#102899),
(#102900,#102901),(#102902,#102903),(#102904,#102905),(#102906,#102907),
(#102908,#102909),(#102910,#102911),(#102912,#102913),(#102914,#102915),
(#102916,#102917),(#102918,#102919),(#102920,#102921),(#102922,#102923),
(#102924,#102925),(#102926,#102927),(#102928,#102929),(#102930,#102931),
(#102932,#102933),(#102934,#102935),(#102936,#102937),(#102938,#102939),
(#102940,#102941),(#102942,#102943),(#102944,#102945),(#102946,#102947),
(#102948,#102949),(#102950,#102951),(#102952,#102953),(#102954,#102955),
(#102956,#102957),(#102958,#102959),(#102960,#102961),(#102962,#102963),
(#102964,#102965),(#102966,#102967),(#102968,#102969),(#102970,#102971),
(#102972,#102973),(#102974,#102975),(#102976,#102977),(#102978,#102979),
(#102980,#102981),(#102982,#102983),(#102984,#102985),(#102986,#102987),
(#102988,#102989),(#102990,#102991),(#102992,#102993),(#102994,#102995),
(#102996,#102997),(#102998,#102999),(#103000,#103001),(#103002,#103003),
(#103004,#103005),(#103006,#103007),(#103008,#103009),(#103010,#103011),
(#103012,#103013),(#103014,#103015),(#103016,#103017),(#103018,#103019),
(#103020,#103021),(#103022,#103023),(#103024,#103025),(#103026,#103027),
(#103028,#103029),(#103030,#103031),(#103032,#103033),(#103034,#103035),
(#103036,#103037),(#103038,#103039),(#103040,#103041),(#103042,#103043),
(#103044,#103045),(#103046,#103047),(#103048,#103049),(#103050,#103051),
(#103052,#103053),(#103054,#103055),(#103056,#103057),(#103058,#103059),
(#103060,#103061),(#103062,#103063),(#103064,#103065),(#103066,#103067),
(#103068,#103069),(#103070,#103071),(#103072,#103073),(#103074,#103075),
(#103076,#103077),(#103078,#103079),(#103080,#103081),(#103082,#103083),
(#103084,#103085),(#103086,#103087),(#103088,#103089),(#103090,#103091),
(#103092,#103093),(#103094,#103095),(#103096,#103097),(#103098,#103099),
(#103100,#103101),(#103102,#103103),(#103104,#103105),(#103106,#103107),
(#103108,#103109),(#103110,#103111),(#103112,#103113),(#103114,#103115),
(#103116,#103117),(#103118,#103119),(#103120,#103121),(#103122,#103123),
(#103124,#103125),(#103126,#103127),(#103128,#103129),(#103130,#103131),
(#103132,#103133),(#103134,#103135),(#103136,#103137),(#103138,#103139),
(#103140,#103141),(#103142,#103143),(#103144,#103145),(#103146,#103147),
(#103148,#103149),(#103150,#103151),(#103152,#103153),(#103154,#103155),
(#103156,#103157),(#103158,#103159),(#103160,#103161),(#103162,#103163),
(#103164,#103165),(#103166,#103167),(#103168,#103169),(#103170,#103171),
(#103172,#103173),(#103174,#103175),(#103176,#103177),(#103178,#103179),
(#103180,#103181),(#103182,#103183),(#103184,#103185),(#103186,#103187),
(#103188,#103189),(#103190,#103191),(#103192,#103193),(#103194,#103195),
(#103196,#103197),(#103198,#103199),(#103200,#103201),(#103202,#103203),
(#103204,#103205),(#103206,#103207)),.UNSPECIFIED.,.F.,.F.,.F.)
B_SPLINE_SURFACE_WITH_KNOTS((6,1,1,1,1,1,1,1,1,1,1,1,1,1,1,1,1,1,1,1,1,
1,1,1,1,1,1,1,1,1,1,1,1,1,1,1,1,1,1,1,1,1,1,1,1,1,1,1,1,1,1,1,1,1,1,1,1,
1,1,1,1,1,1,1,1,1,1,1,1,1,1,1,1,1,1,1,1,1,1,1,1,1,1,1,1,1,1,1,1,1,1,1,1,
1,1,1,1,1,1,1,1,1,1,1,1,1,1,1,1,1,1,1,1,1,1,1,1,1,1,1,1,1,1,1,1,1,1,1,1,
1,1,1,1,1,1,1,1,1,1,1,1,1,1,1,1,1,1,1,1,1,1,1,1,1,1,1,1,1,1,1,1,1,1,1,1,
1,1,1,1,1,1,1,1,1,1,1,1,1,1,1,1,1,1,1,1,1,1,1,1,1,1,1,1,1,1,1,1,1,1,1,6),
(2,2),(0.,0.005,0.01,0.015,0.02,0.025,0.03,0.035,0.04,0.045,0.05,0.055,
0.06,0.065,0.07,0.075,0.08,0.085,0.09,0.095,0.1,0.105,0.11,0.115,0.12,0.125,
0.13,0.135,0.14,0.145,0.15,0.155,0.16,0.165,0.17,0.175,0.18,0.185,0.19,
0.195,0.2,0.205,0.21,0.215,0.22,0.225,0.23,0.235,0.24,0.245,0.25,0.255,
0.26,0.265,0.27,0.275,0.28,0.285,0.29,0.295,0.3,0.305,0.31,0.315,0.32,0.325,
0.33,0.335,0.34,0.345,0.35,0.355,0.36,0.365,0.37,0.375,0.38,0.385,0.39,
0.395,0.4,0.405,0.41,0.415,0.42,0.425,0.43,0.435,0.44,0.445,0.45,0.455,
0.46,0.465,0.47,0.475,0.48,0.485,0.49,0.495,0.5,0.505,0.51,0.515,0.52,0.525,
0.53,0.535,0.54,0.545,0.55,0.555,0.56,0.565,0.57,0.575,0.58,0.585,0.59,
0.595,0.6,0.605,0.61,0.615,0.62,0.625,0.63,0.635,0.64,0.645,0.65,0.655,
0.66,0.665,0.67,0.675,0.68,0.685,0.690000000000001,0.695000000000001,0.700000000000001,
0.705000000000001,0.710000000000001,0.715000000000001,0.720000000000001,
0.725000000000001,0.730000000000001,0.735000000000001,0.740000000000001,
0.745000000000001,0.750000000000001,0.755000000000001,0.760000000000001,
0.765000000000001,0.770000000000001,0.775000000000001,0.780000000000001,
0.785000000000001,0.790000000000001,0.795000000000001,0.800000000000001,
0.805000000000001,0.810000000000001,0.815000000000001,0.820000000000001,
0.825000000000001,0.830000000000001,0.835000000000001,0.840000000000001,
0.845000000000001,0.850000000000001,0.855000000000001,0.860000000000001,
0.865000000000001,0.870000000000001,0.875000000000001,0.880000000000001,
0.885000000000001,0.890000000000001,0.895000000000001,0.900000000000001,
0.905000000000001,0.910000000000001,0.915000000000001,0.920000000000001,
0.925000000000001,0.930000000000001,0.935000000000001,0.940000000000001,
0.945000000000001,0.950000000000001,0.955000000000001,0.960000000000001,
0.965000000000001,0.970000000000001,0.975000000000001,0.980000000000001,
0.985000000000001,0.990000000000001,0.995000000000001,1.),(0.,1.2),
 .UNSPECIFIED.)
GEOMETRIC_REPRESENTATION_ITEM()
RATIONAL_B_SPLINE_SURFACE(((1.,1.),(1.,1.),(1.,1.),(1.,1.),(1.,1.),(1.,
1.),(1.,1.),(1.,1.),(1.,1.),(1.,1.),(1.,1.),(1.,1.),(1.,1.),(1.,1.),(1.,
1.),(1.,1.),(1.,1.),(1.,1.),(1.,1.),(1.,1.),(1.,1.),(1.,1.),(1.,1.),(1.,
1.),(1.,1.),(1.,1.),(1.,1.),(1.,1.),(1.,1.),(1.,1.),(1.,1.),(1.,1.),(1.,
1.),(1.,1.),(1.,1.),(1.,1.),(1.,1.),(1.,1.),(1.,1.),(1.,1.),(1.,1.),(1.,
1.),(1.,1.),(1.,1.),(1.,1.),(1.,1.),(1.,1.),(1.,1.),(1.,1.),(1.,1.),(1.,
1.),(1.,1.),(1.,1.),(1.,1.),(1.,1.),(1.,1.),(1.,1.),(1.,1.),(1.,1.),(1.,
1.),(1.,1.),(1.,1.),(1.,1.),(1.,1.),(1.,1.),(1.,1.),(1.,1.),(1.,1.),(1.,
1.),(1.,1.),(1.,1.),(1.,1.),(1.,1.),(1.,1.),(1.,1.),(1.,1.),(1.,1.),(1.,
1.),(1.,1.),(1.,1.),(1.,1.),(1.,1.),(1.,1.),(1.,1.),(1.,1.),(1.,1.),(1.,
1.),(1.,1.),(1.,1.),(1.,1.),(1.,1.),(1.,1.),(1.,1.),(1.,1.),(1.,1.),(1.,
1.),(1.,1.),(1.,1.),(1.,1.),(1.,1.),(1.,1.),(1.,1.),(1.,1.),(1.,1.),(1.,
1.),(1.,1.),(1.,1.),(1.,1.),(1.,1.),(1.,1.),(1.,1.),(1.,1.),(1.,1.),(1.,
1.),(1.,1.),(1.,1.),(1.,1.),(1.,1.),(1.,1.),(1.,1.),(1.,1.),(1.,1.),(1.,
1.),(1.,1.),(1.,1.),(1.,1.),(1.,1.),(1.,1.),(1.,1.),(1.,1.),(1.,1.),(1.,
1.),(1.,1.),(1.,1.),(1.,1.),(1.,1.),(1.,1.),(1.,1.),(1.,1.),(1.,1.),(1.,
1.),(1.,1.),(1.,1.),(1.,1.),(1.,1.),(1.,1.),(1.,1.),(1.,1.),(1.,1.),(1.,
1.),(1.,1.),(1.,1.),(1.,1.),(1.,1.),(1.,1.),(1.,1.),(1.,1.),(1.,1.),(1.,
1.),(1.,1.),(1.,1.),(1.,1.),(1.,1.),(1.,1.),(1.,1.),(1.,1.),(1.,1.),(1.,
1.),(1.,1.),(1.,1.),(1.,1.),(1.,1.),(1.,1.),(1.,1.),(1.,1.),(1.,1.),(1.,
1.),(1.,1.),(1.,1.),(1.,1.),(1.,1.),(1.,1.),(1.,1.),(1.,1.),(1.,1.),(1.,
1.),(1.,1.),(1.,1.),(1.,1.),(1.,1.),(1.,1.),(1.,1.),(1.,1.),(1.,1.),(1.,
1.),(1.,1.),(1.,1.),(1.,1.),(1.,1.),(1.,1.),(1.,1.),(1.,1.),(1.,1.),(1.,
1.),(1.,1.)))
REPRESENTATION_ITEM('')
SURFACE()
);
#940=(
BOUNDED_SURFACE()
B_SPLINE_SURFACE(5,1,((#103694,#103695),(#103696,#103697),(#103698,#103699),
(#103700,#103701),(#103702,#103703),(#103704,#103705),(#103706,#103707),
(#103708,#103709),(#103710,#103711),(#103712,#103713),(#103714,#103715),
(#103716,#103717),(#103718,#103719),(#103720,#103721),(#103722,#103723),
(#103724,#103725),(#103726,#103727),(#103728,#103729),(#103730,#103731),
(#103732,#103733),(#103734,#103735),(#103736,#103737),(#103738,#103739),
(#103740,#103741),(#103742,#103743),(#103744,#103745),(#103746,#103747),
(#103748,#103749),(#103750,#103751),(#103752,#103753),(#103754,#103755),
(#103756,#103757),(#103758,#103759),(#103760,#103761),(#103762,#103763),
(#103764,#103765),(#103766,#103767),(#103768,#103769),(#103770,#103771),
(#103772,#103773),(#103774,#103775),(#103776,#103777),(#103778,#103779),
(#103780,#103781),(#103782,#103783),(#103784,#103785),(#103786,#103787),
(#103788,#103789),(#103790,#103791),(#103792,#103793),(#103794,#103795),
(#103796,#103797),(#103798,#103799),(#103800,#103801),(#103802,#103803),
(#103804,#103805),(#103806,#103807),(#103808,#103809),(#103810,#103811),
(#103812,#103813),(#103814,#103815),(#103816,#103817),(#103818,#103819),
(#103820,#103821),(#103822,#103823),(#103824,#103825),(#103826,#103827),
(#103828,#103829),(#103830,#103831),(#103832,#103833),(#103834,#103835),
(#103836,#103837),(#103838,#103839),(#103840,#103841),(#103842,#103843),
(#103844,#103845),(#103846,#103847),(#103848,#103849),(#103850,#103851),
(#103852,#103853),(#103854,#103855),(#103856,#103857),(#103858,#103859),
(#103860,#103861),(#103862,#103863),(#103864,#103865),(#103866,#103867),
(#103868,#103869),(#103870,#103871),(#103872,#103873),(#103874,#103875),
(#103876,#103877),(#103878,#103879),(#103880,#103881),(#103882,#103883),
(#103884,#103885),(#103886,#103887),(#103888,#103889),(#103890,#103891),
(#103892,#103893),(#103894,#103895),(#103896,#103897),(#103898,#103899),
(#103900,#103901),(#103902,#103903),(#103904,#103905),(#103906,#103907),
(#103908,#103909),(#103910,#103911),(#103912,#103913),(#103914,#103915),
(#103916,#103917),(#103918,#103919),(#103920,#103921),(#103922,#103923),
(#103924,#103925),(#103926,#103927),(#103928,#103929),(#103930,#103931),
(#103932,#103933),(#103934,#103935),(#103936,#103937),(#103938,#103939),
(#103940,#103941),(#103942,#103943),(#103944,#103945),(#103946,#103947),
(#103948,#103949),(#103950,#103951),(#103952,#103953),(#103954,#103955),
(#103956,#103957),(#103958,#103959),(#103960,#103961),(#103962,#103963),
(#103964,#103965),(#103966,#103967),(#103968,#103969),(#103970,#103971),
(#103972,#103973),(#103974,#103975),(#103976,#103977),(#103978,#103979),
(#103980,#103981),(#103982,#103983),(#103984,#103985),(#103986,#103987),
(#103988,#103989),(#103990,#103991),(#103992,#103993),(#103994,#103995),
(#103996,#103997),(#103998,#103999),(#104000,#104001),(#104002,#104003),
(#104004,#104005),(#104006,#104007),(#104008,#104009),(#104010,#104011),
(#104012,#104013),(#104014,#104015),(#104016,#104017),(#104018,#104019),
(#104020,#104021),(#104022,#104023),(#104024,#104025),(#104026,#104027),
(#104028,#104029),(#104030,#104031),(#104032,#104033),(#104034,#104035),
(#104036,#104037),(#104038,#104039),(#104040,#104041),(#104042,#104043),
(#104044,#104045),(#104046,#104047),(#104048,#104049),(#104050,#104051),
(#104052,#104053),(#104054,#104055),(#104056,#104057),(#104058,#104059),
(#104060,#104061),(#104062,#104063),(#104064,#104065),(#104066,#104067),
(#104068,#104069),(#104070,#104071),(#104072,#104073),(#104074,#104075),
(#104076,#104077),(#104078,#104079),(#104080,#104081),(#104082,#104083),
(#104084,#104085),(#104086,#104087),(#104088,#104089),(#104090,#104091),
(#104092,#104093),(#104094,#104095),(#104096,#104097),(#104098,#104099),
(#104100,#104101),(#104102,#104103)),.UNSPECIFIED.,.F.,.F.,.F.)
B_SPLINE_SURFACE_WITH_KNOTS((6,1,1,1,1,1,1,1,1,1,1,1,1,1,1,1,1,1,1,1,1,
1,1,1,1,1,1,1,1,1,1,1,1,1,1,1,1,1,1,1,1,1,1,1,1,1,1,1,1,1,1,1,1,1,1,1,1,
1,1,1,1,1,1,1,1,1,1,1,1,1,1,1,1,1,1,1,1,1,1,1,1,1,1,1,1,1,1,1,1,1,1,1,1,
1,1,1,1,1,1,1,1,1,1,1,1,1,1,1,1,1,1,1,1,1,1,1,1,1,1,1,1,1,1,1,1,1,1,1,1,
1,1,1,1,1,1,1,1,1,1,1,1,1,1,1,1,1,1,1,1,1,1,1,1,1,1,1,1,1,1,1,1,1,1,1,1,
1,1,1,1,1,1,1,1,1,1,1,1,1,1,1,1,1,1,1,1,1,1,1,1,1,1,1,1,1,1,1,1,1,1,1,6),
(2,2),(0.,0.005,0.01,0.015,0.02,0.025,0.03,0.035,0.04,0.045,0.05,0.055,
0.06,0.065,0.07,0.075,0.08,0.085,0.09,0.095,0.1,0.105,0.11,0.115,0.12,0.125,
0.13,0.135,0.14,0.145,0.15,0.155,0.16,0.165,0.17,0.175,0.18,0.185,0.19,
0.195,0.2,0.205,0.21,0.215,0.22,0.225,0.23,0.235,0.24,0.245,0.25,0.255,
0.26,0.265,0.27,0.275,0.28,0.285,0.29,0.295,0.3,0.305,0.31,0.315,0.32,0.325,
0.33,0.335,0.34,0.345,0.35,0.355,0.36,0.365,0.37,0.375,0.38,0.385,0.39,
0.395,0.4,0.405,0.41,0.415,0.42,0.425,0.43,0.435,0.44,0.445,0.45,0.455,
0.46,0.465,0.47,0.475,0.48,0.485,0.49,0.495,0.5,0.505,0.51,0.515,0.52,0.525,
0.53,0.535,0.54,0.545,0.55,0.555,0.56,0.565,0.57,0.575,0.58,0.585,0.59,
0.595,0.6,0.605,0.61,0.615,0.62,0.625,0.63,0.635,0.64,0.645,0.65,0.655,
0.66,0.665,0.67,0.675,0.68,0.685,0.690000000000001,0.695000000000001,0.700000000000001,
0.705000000000001,0.710000000000001,0.715000000000001,0.720000000000001,
0.725000000000001,0.730000000000001,0.735000000000001,0.740000000000001,
0.745000000000001,0.750000000000001,0.755000000000001,0.760000000000001,
0.765000000000001,0.770000000000001,0.775000000000001,0.780000000000001,
0.785000000000001,0.790000000000001,0.795000000000001,0.800000000000001,
0.805000000000001,0.810000000000001,0.815000000000001,0.820000000000001,
0.825000000000001,0.830000000000001,0.835000000000001,0.840000000000001,
0.845000000000001,0.850000000000001,0.855000000000001,0.860000000000001,
0.865000000000001,0.870000000000001,0.875000000000001,0.880000000000001,
0.885000000000001,0.890000000000001,0.895000000000001,0.900000000000001,
0.905000000000001,0.910000000000001,0.915000000000001,0.920000000000001,
0.925000000000001,0.930000000000001,0.935000000000001,0.940000000000001,
0.945000000000001,0.950000000000001,0.955000000000001,0.960000000000001,
0.965000000000001,0.970000000000001,0.975000000000001,0.980000000000001,
0.985000000000001,0.990000000000001,0.995000000000001,1.),(0.,1.2),
 .UNSPECIFIED.)
GEOMETRIC_REPRESENTATION_ITEM()
RATIONAL_B_SPLINE_SURFACE(((1.,1.),(1.,1.),(1.,1.),(1.,1.),(1.,1.),(1.,
1.),(1.,1.),(1.,1.),(1.,1.),(1.,1.),(1.,1.),(1.,1.),(1.,1.),(1.,1.),(1.,
1.),(1.,1.),(1.,1.),(1.,1.),(1.,1.),(1.,1.),(1.,1.),(1.,1.),(1.,1.),(1.,
1.),(1.,1.),(1.,1.),(1.,1.),(1.,1.),(1.,1.),(1.,1.),(1.,1.),(1.,1.),(1.,
1.),(1.,1.),(1.,1.),(1.,1.),(1.,1.),(1.,1.),(1.,1.),(1.,1.),(1.,1.),(1.,
1.),(1.,1.),(1.,1.),(1.,1.),(1.,1.),(1.,1.),(1.,1.),(1.,1.),(1.,1.),(1.,
1.),(1.,1.),(1.,1.),(1.,1.),(1.,1.),(1.,1.),(1.,1.),(1.,1.),(1.,1.),(1.,
1.),(1.,1.),(1.,1.),(1.,1.),(1.,1.),(1.,1.),(1.,1.),(1.,1.),(1.,1.),(1.,
1.),(1.,1.),(1.,1.),(1.,1.),(1.,1.),(1.,1.),(1.,1.),(1.,1.),(1.,1.),(1.,
1.),(1.,1.),(1.,1.),(1.,1.),(1.,1.),(1.,1.),(1.,1.),(1.,1.),(1.,1.),(1.,
1.),(1.,1.),(1.,1.),(1.,1.),(1.,1.),(1.,1.),(1.,1.),(1.,1.),(1.,1.),(1.,
1.),(1.,1.),(1.,1.),(1.,1.),(1.,1.),(1.,1.),(1.,1.),(1.,1.),(1.,1.),(1.,
1.),(1.,1.),(1.,1.),(1.,1.),(1.,1.),(1.,1.),(1.,1.),(1.,1.),(1.,1.),(1.,
1.),(1.,1.),(1.,1.),(1.,1.),(1.,1.),(1.,1.),(1.,1.),(1.,1.),(1.,1.),(1.,
1.),(1.,1.),(1.,1.),(1.,1.),(1.,1.),(1.,1.),(1.,1.),(1.,1.),(1.,1.),(1.,
1.),(1.,1.),(1.,1.),(1.,1.),(1.,1.),(1.,1.),(1.,1.),(1.,1.),(1.,1.),(1.,
1.),(1.,1.),(1.,1.),(1.,1.),(1.,1.),(1.,1.),(1.,1.),(1.,1.),(1.,1.),(1.,
1.),(1.,1.),(1.,1.),(1.,1.),(1.,1.),(1.,1.),(1.,1.),(1.,1.),(1.,1.),(1.,
1.),(1.,1.),(1.,1.),(1.,1.),(1.,1.),(1.,1.),(1.,1.),(1.,1.),(1.,1.),(1.,
1.),(1.,1.),(1.,1.),(1.,1.),(1.,1.),(1.,1.),(1.,1.),(1.,1.),(1.,1.),(1.,
1.),(1.,1.),(1.,1.),(1.,1.),(1.,1.),(1.,1.),(1.,1.),(1.,1.),(1.,1.),(1.,
1.),(1.,1.),(1.,1.),(1.,1.),(1.,1.),(1.,1.),(1.,1.),(1.,1.),(1.,1.),(1.,
1.),(1.,1.),(1.,1.),(1.,1.),(1.,1.),(1.,1.),(1.,1.),(1.,1.),(1.,1.),(1.,
1.),(1.,1.)))
REPRESENTATION_ITEM('')
SURFACE()
);
#941=(
BOUNDED_SURFACE()
B_SPLINE_SURFACE(5,1,((#104590,#104591),(#104592,#104593),(#104594,#104595),
(#104596,#104597),(#104598,#104599),(#104600,#104601),(#104602,#104603),
(#104604,#104605),(#104606,#104607),(#104608,#104609),(#104610,#104611),
(#104612,#104613),(#104614,#104615),(#104616,#104617),(#104618,#104619),
(#104620,#104621),(#104622,#104623),(#104624,#104625),(#104626,#104627),
(#104628,#104629),(#104630,#104631),(#104632,#104633),(#104634,#104635),
(#104636,#104637),(#104638,#104639),(#104640,#104641),(#104642,#104643),
(#104644,#104645),(#104646,#104647),(#104648,#104649),(#104650,#104651),
(#104652,#104653),(#104654,#104655),(#104656,#104657),(#104658,#104659),
(#104660,#104661),(#104662,#104663),(#104664,#104665),(#104666,#104667),
(#104668,#104669),(#104670,#104671),(#104672,#104673),(#104674,#104675),
(#104676,#104677),(#104678,#104679),(#104680,#104681),(#104682,#104683),
(#104684,#104685),(#104686,#104687),(#104688,#104689),(#104690,#104691),
(#104692,#104693),(#104694,#104695),(#104696,#104697),(#104698,#104699),
(#104700,#104701),(#104702,#104703),(#104704,#104705),(#104706,#104707),
(#104708,#104709),(#104710,#104711),(#104712,#104713),(#104714,#104715),
(#104716,#104717),(#104718,#104719),(#104720,#104721),(#104722,#104723),
(#104724,#104725),(#104726,#104727),(#104728,#104729),(#104730,#104731),
(#104732,#104733),(#104734,#104735),(#104736,#104737),(#104738,#104739),
(#104740,#104741),(#104742,#104743),(#104744,#104745),(#104746,#104747),
(#104748,#104749),(#104750,#104751),(#104752,#104753),(#104754,#104755),
(#104756,#104757),(#104758,#104759),(#104760,#104761),(#104762,#104763),
(#104764,#104765),(#104766,#104767),(#104768,#104769),(#104770,#104771),
(#104772,#104773),(#104774,#104775),(#104776,#104777),(#104778,#104779),
(#104780,#104781),(#104782,#104783),(#104784,#104785),(#104786,#104787),
(#104788,#104789),(#104790,#104791),(#104792,#104793),(#104794,#104795),
(#104796,#104797),(#104798,#104799),(#104800,#104801),(#104802,#104803),
(#104804,#104805),(#104806,#104807),(#104808,#104809),(#104810,#104811),
(#104812,#104813),(#104814,#104815),(#104816,#104817),(#104818,#104819),
(#104820,#104821),(#104822,#104823),(#104824,#104825),(#104826,#104827),
(#104828,#104829),(#104830,#104831),(#104832,#104833),(#104834,#104835),
(#104836,#104837),(#104838,#104839),(#104840,#104841),(#104842,#104843),
(#104844,#104845),(#104846,#104847),(#104848,#104849),(#104850,#104851),
(#104852,#104853),(#104854,#104855),(#104856,#104857),(#104858,#104859),
(#104860,#104861),(#104862,#104863),(#104864,#104865),(#104866,#104867),
(#104868,#104869),(#104870,#104871),(#104872,#104873),(#104874,#104875),
(#104876,#104877),(#104878,#104879),(#104880,#104881),(#104882,#104883),
(#104884,#104885),(#104886,#104887),(#104888,#104889),(#104890,#104891),
(#104892,#104893),(#104894,#104895),(#104896,#104897),(#104898,#104899),
(#104900,#104901),(#104902,#104903),(#104904,#104905),(#104906,#104907),
(#104908,#104909),(#104910,#104911),(#104912,#104913),(#104914,#104915),
(#104916,#104917),(#104918,#104919),(#104920,#104921),(#104922,#104923),
(#104924,#104925),(#104926,#104927),(#104928,#104929),(#104930,#104931),
(#104932,#104933),(#104934,#104935),(#104936,#104937),(#104938,#104939),
(#104940,#104941),(#104942,#104943),(#104944,#104945),(#104946,#104947),
(#104948,#104949),(#104950,#104951),(#104952,#104953),(#104954,#104955),
(#104956,#104957),(#104958,#104959),(#104960,#104961),(#104962,#104963),
(#104964,#104965),(#104966,#104967),(#104968,#104969),(#104970,#104971),
(#104972,#104973),(#104974,#104975),(#104976,#104977),(#104978,#104979),
(#104980,#104981),(#104982,#104983),(#104984,#104985),(#104986,#104987),
(#104988,#104989),(#104990,#104991),(#104992,#104993),(#104994,#104995),
(#104996,#104997),(#104998,#104999)),.UNSPECIFIED.,.F.,.F.,.F.)
B_SPLINE_SURFACE_WITH_KNOTS((6,1,1,1,1,1,1,1,1,1,1,1,1,1,1,1,1,1,1,1,1,
1,1,1,1,1,1,1,1,1,1,1,1,1,1,1,1,1,1,1,1,1,1,1,1,1,1,1,1,1,1,1,1,1,1,1,1,
1,1,1,1,1,1,1,1,1,1,1,1,1,1,1,1,1,1,1,1,1,1,1,1,1,1,1,1,1,1,1,1,1,1,1,1,
1,1,1,1,1,1,1,1,1,1,1,1,1,1,1,1,1,1,1,1,1,1,1,1,1,1,1,1,1,1,1,1,1,1,1,1,
1,1,1,1,1,1,1,1,1,1,1,1,1,1,1,1,1,1,1,1,1,1,1,1,1,1,1,1,1,1,1,1,1,1,1,1,
1,1,1,1,1,1,1,1,1,1,1,1,1,1,1,1,1,1,1,1,1,1,1,1,1,1,1,1,1,1,1,1,1,1,1,6),
(2,2),(0.,0.005,0.01,0.015,0.02,0.025,0.03,0.035,0.04,0.045,0.05,0.055,
0.06,0.065,0.07,0.075,0.08,0.085,0.09,0.095,0.1,0.105,0.11,0.115,0.12,0.125,
0.13,0.135,0.14,0.145,0.15,0.155,0.16,0.165,0.17,0.175,0.18,0.185,0.19,
0.195,0.2,0.205,0.21,0.215,0.22,0.225,0.23,0.235,0.24,0.245,0.25,0.255,
0.26,0.265,0.27,0.275,0.28,0.285,0.29,0.295,0.3,0.305,0.31,0.315,0.32,0.325,
0.33,0.335,0.34,0.345,0.35,0.355,0.36,0.365,0.37,0.375,0.38,0.385,0.39,
0.395,0.4,0.405,0.41,0.415,0.42,0.425,0.43,0.435,0.44,0.445,0.45,0.455,
0.46,0.465,0.47,0.475,0.48,0.485,0.49,0.495,0.5,0.505,0.51,0.515,0.52,0.525,
0.53,0.535,0.54,0.545,0.55,0.555,0.56,0.565,0.57,0.575,0.58,0.585,0.59,
0.595,0.6,0.605,0.61,0.615,0.62,0.625,0.63,0.635,0.64,0.645,0.65,0.655,
0.66,0.665,0.67,0.675,0.68,0.685,0.690000000000001,0.695000000000001,0.700000000000001,
0.705000000000001,0.710000000000001,0.715000000000001,0.720000000000001,
0.725000000000001,0.730000000000001,0.735000000000001,0.740000000000001,
0.745000000000001,0.750000000000001,0.755000000000001,0.760000000000001,
0.765000000000001,0.770000000000001,0.775000000000001,0.780000000000001,
0.785000000000001,0.790000000000001,0.795000000000001,0.800000000000001,
0.805000000000001,0.810000000000001,0.815000000000001,0.820000000000001,
0.825000000000001,0.830000000000001,0.835000000000001,0.840000000000001,
0.845000000000001,0.850000000000001,0.855000000000001,0.860000000000001,
0.865000000000001,0.870000000000001,0.875000000000001,0.880000000000001,
0.885000000000001,0.890000000000001,0.895000000000001,0.900000000000001,
0.905000000000001,0.910000000000001,0.915000000000001,0.920000000000001,
0.925000000000001,0.930000000000001,0.935000000000001,0.940000000000001,
0.945000000000001,0.950000000000001,0.955000000000001,0.960000000000001,
0.965000000000001,0.970000000000001,0.975000000000001,0.980000000000001,
0.985000000000001,0.990000000000001,0.995000000000001,1.),(0.,1.2),
 .UNSPECIFIED.)
GEOMETRIC_REPRESENTATION_ITEM()
RATIONAL_B_SPLINE_SURFACE(((1.,1.),(1.,1.),(1.,1.),(1.,1.),(1.,1.),(1.,
1.),(1.,1.),(1.,1.),(1.,1.),(1.,1.),(1.,1.),(1.,1.),(1.,1.),(1.,1.),(1.,
1.),(1.,1.),(1.,1.),(1.,1.),(1.,1.),(1.,1.),(1.,1.),(1.,1.),(1.,1.),(1.,
1.),(1.,1.),(1.,1.),(1.,1.),(1.,1.),(1.,1.),(1.,1.),(1.,1.),(1.,1.),(1.,
1.),(1.,1.),(1.,1.),(1.,1.),(1.,1.),(1.,1.),(1.,1.),(1.,1.),(1.,1.),(1.,
1.),(1.,1.),(1.,1.),(1.,1.),(1.,1.),(1.,1.),(1.,1.),(1.,1.),(1.,1.),(1.,
1.),(1.,1.),(1.,1.),(1.,1.),(1.,1.),(1.,1.),(1.,1.),(1.,1.),(1.,1.),(1.,
1.),(1.,1.),(1.,1.),(1.,1.),(1.,1.),(1.,1.),(1.,1.),(1.,1.),(1.,1.),(1.,
1.),(1.,1.),(1.,1.),(1.,1.),(1.,1.),(1.,1.),(1.,1.),(1.,1.),(1.,1.),(1.,
1.),(1.,1.),(1.,1.),(1.,1.),(1.,1.),(1.,1.),(1.,1.),(1.,1.),(1.,1.),(1.,
1.),(1.,1.),(1.,1.),(1.,1.),(1.,1.),(1.,1.),(1.,1.),(1.,1.),(1.,1.),(1.,
1.),(1.,1.),(1.,1.),(1.,1.),(1.,1.),(1.,1.),(1.,1.),(1.,1.),(1.,1.),(1.,
1.),(1.,1.),(1.,1.),(1.,1.),(1.,1.),(1.,1.),(1.,1.),(1.,1.),(1.,1.),(1.,
1.),(1.,1.),(1.,1.),(1.,1.),(1.,1.),(1.,1.),(1.,1.),(1.,1.),(1.,1.),(1.,
1.),(1.,1.),(1.,1.),(1.,1.),(1.,1.),(1.,1.),(1.,1.),(1.,1.),(1.,1.),(1.,
1.),(1.,1.),(1.,1.),(1.,1.),(1.,1.),(1.,1.),(1.,1.),(1.,1.),(1.,1.),(1.,
1.),(1.,1.),(1.,1.),(1.,1.),(1.,1.),(1.,1.),(1.,1.),(1.,1.),(1.,1.),(1.,
1.),(1.,1.),(1.,1.),(1.,1.),(1.,1.),(1.,1.),(1.,1.),(1.,1.),(1.,1.),(1.,
1.),(1.,1.),(1.,1.),(1.,1.),(1.,1.),(1.,1.),(1.,1.),(1.,1.),(1.,1.),(1.,
1.),(1.,1.),(1.,1.),(1.,1.),(1.,1.),(1.,1.),(1.,1.),(1.,1.),(1.,1.),(1.,
1.),(1.,1.),(1.,1.),(1.,1.),(1.,1.),(1.,1.),(1.,1.),(1.,1.),(1.,1.),(1.,
1.),(1.,1.),(1.,1.),(1.,1.),(1.,1.),(1.,1.),(1.,1.),(1.,1.),(1.,1.),(1.,
1.),(1.,1.),(1.,1.),(1.,1.),(1.,1.),(1.,1.),(1.,1.),(1.,1.),(1.,1.),(1.,
1.),(1.,1.)))
REPRESENTATION_ITEM('')
SURFACE()
);
#942=(
BOUNDED_SURFACE()
B_SPLINE_SURFACE(5,1,((#105486,#105487),(#105488,#105489),(#105490,#105491),
(#105492,#105493),(#105494,#105495),(#105496,#105497),(#105498,#105499),
(#105500,#105501),(#105502,#105503),(#105504,#105505),(#105506,#105507),
(#105508,#105509),(#105510,#105511),(#105512,#105513),(#105514,#105515),
(#105516,#105517),(#105518,#105519),(#105520,#105521),(#105522,#105523),
(#105524,#105525),(#105526,#105527),(#105528,#105529),(#105530,#105531),
(#105532,#105533),(#105534,#105535),(#105536,#105537),(#105538,#105539),
(#105540,#105541),(#105542,#105543),(#105544,#105545),(#105546,#105547),
(#105548,#105549),(#105550,#105551),(#105552,#105553),(#105554,#105555),
(#105556,#105557),(#105558,#105559),(#105560,#105561),(#105562,#105563),
(#105564,#105565),(#105566,#105567),(#105568,#105569),(#105570,#105571),
(#105572,#105573),(#105574,#105575),(#105576,#105577),(#105578,#105579),
(#105580,#105581),(#105582,#105583),(#105584,#105585),(#105586,#105587),
(#105588,#105589),(#105590,#105591),(#105592,#105593),(#105594,#105595),
(#105596,#105597),(#105598,#105599),(#105600,#105601),(#105602,#105603),
(#105604,#105605),(#105606,#105607),(#105608,#105609),(#105610,#105611),
(#105612,#105613),(#105614,#105615),(#105616,#105617),(#105618,#105619),
(#105620,#105621),(#105622,#105623),(#105624,#105625),(#105626,#105627),
(#105628,#105629),(#105630,#105631),(#105632,#105633),(#105634,#105635),
(#105636,#105637),(#105638,#105639),(#105640,#105641),(#105642,#105643),
(#105644,#105645),(#105646,#105647),(#105648,#105649),(#105650,#105651),
(#105652,#105653),(#105654,#105655),(#105656,#105657),(#105658,#105659),
(#105660,#105661),(#105662,#105663),(#105664,#105665),(#105666,#105667),
(#105668,#105669),(#105670,#105671),(#105672,#105673),(#105674,#105675),
(#105676,#105677),(#105678,#105679),(#105680,#105681),(#105682,#105683),
(#105684,#105685),(#105686,#105687),(#105688,#105689),(#105690,#105691),
(#105692,#105693),(#105694,#105695),(#105696,#105697),(#105698,#105699),
(#105700,#105701),(#105702,#105703),(#105704,#105705),(#105706,#105707),
(#105708,#105709),(#105710,#105711),(#105712,#105713),(#105714,#105715),
(#105716,#105717),(#105718,#105719),(#105720,#105721),(#105722,#105723),
(#105724,#105725),(#105726,#105727),(#105728,#105729),(#105730,#105731),
(#105732,#105733),(#105734,#105735),(#105736,#105737),(#105738,#105739),
(#105740,#105741),(#105742,#105743),(#105744,#105745),(#105746,#105747),
(#105748,#105749),(#105750,#105751),(#105752,#105753),(#105754,#105755),
(#105756,#105757),(#105758,#105759),(#105760,#105761),(#105762,#105763),
(#105764,#105765),(#105766,#105767),(#105768,#105769),(#105770,#105771),
(#105772,#105773),(#105774,#105775),(#105776,#105777),(#105778,#105779),
(#105780,#105781),(#105782,#105783),(#105784,#105785),(#105786,#105787),
(#105788,#105789),(#105790,#105791),(#105792,#105793),(#105794,#105795),
(#105796,#105797),(#105798,#105799),(#105800,#105801),(#105802,#105803),
(#105804,#105805),(#105806,#105807),(#105808,#105809),(#105810,#105811),
(#105812,#105813),(#105814,#105815),(#105816,#105817),(#105818,#105819),
(#105820,#105821),(#105822,#105823),(#105824,#105825),(#105826,#105827),
(#105828,#105829),(#105830,#105831),(#105832,#105833),(#105834,#105835),
(#105836,#105837),(#105838,#105839),(#105840,#105841),(#105842,#105843),
(#105844,#105845),(#105846,#105847),(#105848,#105849),(#105850,#105851),
(#105852,#105853),(#105854,#105855),(#105856,#105857),(#105858,#105859),
(#105860,#105861),(#105862,#105863),(#105864,#105865),(#105866,#105867),
(#105868,#105869),(#105870,#105871),(#105872,#105873),(#105874,#105875),
(#105876,#105877),(#105878,#105879),(#105880,#105881),(#105882,#105883),
(#105884,#105885),(#105886,#105887),(#105888,#105889),(#105890,#105891),
(#105892,#105893),(#105894,#105895)),.UNSPECIFIED.,.F.,.F.,.F.)
B_SPLINE_SURFACE_WITH_KNOTS((6,1,1,1,1,1,1,1,1,1,1,1,1,1,1,1,1,1,1,1,1,
1,1,1,1,1,1,1,1,1,1,1,1,1,1,1,1,1,1,1,1,1,1,1,1,1,1,1,1,1,1,1,1,1,1,1,1,
1,1,1,1,1,1,1,1,1,1,1,1,1,1,1,1,1,1,1,1,1,1,1,1,1,1,1,1,1,1,1,1,1,1,1,1,
1,1,1,1,1,1,1,1,1,1,1,1,1,1,1,1,1,1,1,1,1,1,1,1,1,1,1,1,1,1,1,1,1,1,1,1,
1,1,1,1,1,1,1,1,1,1,1,1,1,1,1,1,1,1,1,1,1,1,1,1,1,1,1,1,1,1,1,1,1,1,1,1,
1,1,1,1,1,1,1,1,1,1,1,1,1,1,1,1,1,1,1,1,1,1,1,1,1,1,1,1,1,1,1,1,1,1,1,6),
(2,2),(0.,0.005,0.01,0.015,0.02,0.025,0.03,0.035,0.04,0.045,0.05,0.055,
0.06,0.065,0.07,0.075,0.08,0.085,0.09,0.095,0.1,0.105,0.11,0.115,0.12,0.125,
0.13,0.135,0.14,0.145,0.15,0.155,0.16,0.165,0.17,0.175,0.18,0.185,0.19,
0.195,0.2,0.205,0.21,0.215,0.22,0.225,0.23,0.235,0.24,0.245,0.25,0.255,
0.26,0.265,0.27,0.275,0.28,0.285,0.29,0.295,0.3,0.305,0.31,0.315,0.32,0.325,
0.33,0.335,0.34,0.345,0.35,0.355,0.36,0.365,0.37,0.375,0.38,0.385,0.39,
0.395,0.4,0.405,0.41,0.415,0.42,0.425,0.43,0.435,0.44,0.445,0.45,0.455,
0.46,0.465,0.47,0.475,0.48,0.485,0.49,0.495,0.5,0.505,0.51,0.515,0.52,0.525,
0.53,0.535,0.54,0.545,0.55,0.555,0.56,0.565,0.57,0.575,0.58,0.585,0.59,
0.595,0.6,0.605,0.61,0.615,0.62,0.625,0.63,0.635,0.64,0.645,0.65,0.655,
0.66,0.665,0.67,0.675,0.68,0.685,0.690000000000001,0.695000000000001,0.700000000000001,
0.705000000000001,0.710000000000001,0.715000000000001,0.720000000000001,
0.725000000000001,0.730000000000001,0.735000000000001,0.740000000000001,
0.745000000000001,0.750000000000001,0.755000000000001,0.760000000000001,
0.765000000000001,0.770000000000001,0.775000000000001,0.780000000000001,
0.785000000000001,0.790000000000001,0.795000000000001,0.800000000000001,
0.805000000000001,0.810000000000001,0.815000000000001,0.820000000000001,
0.825000000000001,0.830000000000001,0.835000000000001,0.840000000000001,
0.845000000000001,0.850000000000001,0.855000000000001,0.860000000000001,
0.865000000000001,0.870000000000001,0.875000000000001,0.880000000000001,
0.885000000000001,0.890000000000001,0.895000000000001,0.900000000000001,
0.905000000000001,0.910000000000001,0.915000000000001,0.920000000000001,
0.925000000000001,0.930000000000001,0.935000000000001,0.940000000000001,
0.945000000000001,0.950000000000001,0.955000000000001,0.960000000000001,
0.965000000000001,0.970000000000001,0.975000000000001,0.980000000000001,
0.985000000000001,0.990000000000001,0.995000000000001,1.),(0.,1.2),
 .UNSPECIFIED.)
GEOMETRIC_REPRESENTATION_ITEM()
RATIONAL_B_SPLINE_SURFACE(((1.,1.),(1.,1.),(1.,1.),(1.,1.),(1.,1.),(1.,
1.),(1.,1.),(1.,1.),(1.,1.),(1.,1.),(1.,1.),(1.,1.),(1.,1.),(1.,1.),(1.,
1.),(1.,1.),(1.,1.),(1.,1.),(1.,1.),(1.,1.),(1.,1.),(1.,1.),(1.,1.),(1.,
1.),(1.,1.),(1.,1.),(1.,1.),(1.,1.),(1.,1.),(1.,1.),(1.,1.),(1.,1.),(1.,
1.),(1.,1.),(1.,1.),(1.,1.),(1.,1.),(1.,1.),(1.,1.),(1.,1.),(1.,1.),(1.,
1.),(1.,1.),(1.,1.),(1.,1.),(1.,1.),(1.,1.),(1.,1.),(1.,1.),(1.,1.),(1.,
1.),(1.,1.),(1.,1.),(1.,1.),(1.,1.),(1.,1.),(1.,1.),(1.,1.),(1.,1.),(1.,
1.),(1.,1.),(1.,1.),(1.,1.),(1.,1.),(1.,1.),(1.,1.),(1.,1.),(1.,1.),(1.,
1.),(1.,1.),(1.,1.),(1.,1.),(1.,1.),(1.,1.),(1.,1.),(1.,1.),(1.,1.),(1.,
1.),(1.,1.),(1.,1.),(1.,1.),(1.,1.),(1.,1.),(1.,1.),(1.,1.),(1.,1.),(1.,
1.),(1.,1.),(1.,1.),(1.,1.),(1.,1.),(1.,1.),(1.,1.),(1.,1.),(1.,1.),(1.,
1.),(1.,1.),(1.,1.),(1.,1.),(1.,1.),(1.,1.),(1.,1.),(1.,1.),(1.,1.),(1.,
1.),(1.,1.),(1.,1.),(1.,1.),(1.,1.),(1.,1.),(1.,1.),(1.,1.),(1.,1.),(1.,
1.),(1.,1.),(1.,1.),(1.,1.),(1.,1.),(1.,1.),(1.,1.),(1.,1.),(1.,1.),(1.,
1.),(1.,1.),(1.,1.),(1.,1.),(1.,1.),(1.,1.),(1.,1.),(1.,1.),(1.,1.),(1.,
1.),(1.,1.),(1.,1.),(1.,1.),(1.,1.),(1.,1.),(1.,1.),(1.,1.),(1.,1.),(1.,
1.),(1.,1.),(1.,1.),(1.,1.),(1.,1.),(1.,1.),(1.,1.),(1.,1.),(1.,1.),(1.,
1.),(1.,1.),(1.,1.),(1.,1.),(1.,1.),(1.,1.),(1.,1.),(1.,1.),(1.,1.),(1.,
1.),(1.,1.),(1.,1.),(1.,1.),(1.,1.),(1.,1.),(1.,1.),(1.,1.),(1.,1.),(1.,
1.),(1.,1.),(1.,1.),(1.,1.),(1.,1.),(1.,1.),(1.,1.),(1.,1.),(1.,1.),(1.,
1.),(1.,1.),(1.,1.),(1.,1.),(1.,1.),(1.,1.),(1.,1.),(1.,1.),(1.,1.),(1.,
1.),(1.,1.),(1.,1.),(1.,1.),(1.,1.),(1.,1.),(1.,1.),(1.,1.),(1.,1.),(1.,
1.),(1.,1.),(1.,1.),(1.,1.),(1.,1.),(1.,1.),(1.,1.),(1.,1.),(1.,1.),(1.,
1.),(1.,1.)))
REPRESENTATION_ITEM('')
SURFACE()
);
#943=(
BOUNDED_SURFACE()
B_SPLINE_SURFACE(5,1,((#106382,#106383),(#106384,#106385),(#106386,#106387),
(#106388,#106389),(#106390,#106391),(#106392,#106393),(#106394,#106395),
(#106396,#106397),(#106398,#106399),(#106400,#106401),(#106402,#106403),
(#106404,#106405),(#106406,#106407),(#106408,#106409),(#106410,#106411),
(#106412,#106413),(#106414,#106415),(#106416,#106417),(#106418,#106419),
(#106420,#106421),(#106422,#106423),(#106424,#106425),(#106426,#106427),
(#106428,#106429),(#106430,#106431),(#106432,#106433),(#106434,#106435),
(#106436,#106437),(#106438,#106439),(#106440,#106441),(#106442,#106443),
(#106444,#106445),(#106446,#106447),(#106448,#106449),(#106450,#106451),
(#106452,#106453),(#106454,#106455),(#106456,#106457),(#106458,#106459),
(#106460,#106461),(#106462,#106463),(#106464,#106465),(#106466,#106467),
(#106468,#106469),(#106470,#106471),(#106472,#106473),(#106474,#106475),
(#106476,#106477),(#106478,#106479),(#106480,#106481),(#106482,#106483),
(#106484,#106485),(#106486,#106487),(#106488,#106489),(#106490,#106491),
(#106492,#106493),(#106494,#106495),(#106496,#106497),(#106498,#106499),
(#106500,#106501),(#106502,#106503),(#106504,#106505),(#106506,#106507),
(#106508,#106509),(#106510,#106511),(#106512,#106513),(#106514,#106515),
(#106516,#106517),(#106518,#106519),(#106520,#106521),(#106522,#106523),
(#106524,#106525),(#106526,#106527),(#106528,#106529),(#106530,#106531),
(#106532,#106533),(#106534,#106535),(#106536,#106537),(#106538,#106539),
(#106540,#106541),(#106542,#106543),(#106544,#106545),(#106546,#106547),
(#106548,#106549),(#106550,#106551),(#106552,#106553),(#106554,#106555),
(#106556,#106557),(#106558,#106559),(#106560,#106561),(#106562,#106563),
(#106564,#106565),(#106566,#106567),(#106568,#106569),(#106570,#106571),
(#106572,#106573),(#106574,#106575),(#106576,#106577),(#106578,#106579),
(#106580,#106581),(#106582,#106583),(#106584,#106585),(#106586,#106587),
(#106588,#106589),(#106590,#106591),(#106592,#106593),(#106594,#106595),
(#106596,#106597),(#106598,#106599),(#106600,#106601),(#106602,#106603),
(#106604,#106605),(#106606,#106607),(#106608,#106609),(#106610,#106611),
(#106612,#106613),(#106614,#106615),(#106616,#106617),(#106618,#106619),
(#106620,#106621),(#106622,#106623),(#106624,#106625),(#106626,#106627),
(#106628,#106629),(#106630,#106631),(#106632,#106633),(#106634,#106635),
(#106636,#106637),(#106638,#106639),(#106640,#106641),(#106642,#106643),
(#106644,#106645),(#106646,#106647),(#106648,#106649),(#106650,#106651),
(#106652,#106653),(#106654,#106655),(#106656,#106657),(#106658,#106659),
(#106660,#106661),(#106662,#106663),(#106664,#106665),(#106666,#106667),
(#106668,#106669),(#106670,#106671),(#106672,#106673),(#106674,#106675),
(#106676,#106677),(#106678,#106679),(#106680,#106681),(#106682,#106683),
(#106684,#106685),(#106686,#106687),(#106688,#106689),(#106690,#106691),
(#106692,#106693),(#106694,#106695),(#106696,#106697),(#106698,#106699),
(#106700,#106701),(#106702,#106703),(#106704,#106705),(#106706,#106707),
(#106708,#106709),(#106710,#106711),(#106712,#106713),(#106714,#106715),
(#106716,#106717),(#106718,#106719),(#106720,#106721),(#106722,#106723),
(#106724,#106725),(#106726,#106727),(#106728,#106729),(#106730,#106731),
(#106732,#106733),(#106734,#106735),(#106736,#106737),(#106738,#106739),
(#106740,#106741),(#106742,#106743),(#106744,#106745),(#106746,#106747),
(#106748,#106749),(#106750,#106751),(#106752,#106753),(#106754,#106755),
(#106756,#106757),(#106758,#106759),(#106760,#106761),(#106762,#106763),
(#106764,#106765),(#106766,#106767),(#106768,#106769),(#106770,#106771),
(#106772,#106773),(#106774,#106775),(#106776,#106777),(#106778,#106779),
(#106780,#106781),(#106782,#106783),(#106784,#106785),(#106786,#106787),
(#106788,#106789),(#106790,#106791)),.UNSPECIFIED.,.F.,.F.,.F.)
B_SPLINE_SURFACE_WITH_KNOTS((6,1,1,1,1,1,1,1,1,1,1,1,1,1,1,1,1,1,1,1,1,
1,1,1,1,1,1,1,1,1,1,1,1,1,1,1,1,1,1,1,1,1,1,1,1,1,1,1,1,1,1,1,1,1,1,1,1,
1,1,1,1,1,1,1,1,1,1,1,1,1,1,1,1,1,1,1,1,1,1,1,1,1,1,1,1,1,1,1,1,1,1,1,1,
1,1,1,1,1,1,1,1,1,1,1,1,1,1,1,1,1,1,1,1,1,1,1,1,1,1,1,1,1,1,1,1,1,1,1,1,
1,1,1,1,1,1,1,1,1,1,1,1,1,1,1,1,1,1,1,1,1,1,1,1,1,1,1,1,1,1,1,1,1,1,1,1,
1,1,1,1,1,1,1,1,1,1,1,1,1,1,1,1,1,1,1,1,1,1,1,1,1,1,1,1,1,1,1,1,1,1,1,6),
(2,2),(0.,0.005,0.01,0.015,0.02,0.025,0.03,0.035,0.04,0.045,0.05,0.055,
0.06,0.065,0.07,0.075,0.08,0.085,0.09,0.095,0.1,0.105,0.11,0.115,0.12,0.125,
0.13,0.135,0.14,0.145,0.15,0.155,0.16,0.165,0.17,0.175,0.18,0.185,0.19,
0.195,0.2,0.205,0.21,0.215,0.22,0.225,0.23,0.235,0.24,0.245,0.25,0.255,
0.26,0.265,0.27,0.275,0.28,0.285,0.29,0.295,0.3,0.305,0.31,0.315,0.32,0.325,
0.33,0.335,0.34,0.345,0.35,0.355,0.36,0.365,0.37,0.375,0.38,0.385,0.39,
0.395,0.4,0.405,0.41,0.415,0.42,0.425,0.43,0.435,0.44,0.445,0.45,0.455,
0.46,0.465,0.47,0.475,0.48,0.485,0.49,0.495,0.5,0.505,0.51,0.515,0.52,0.525,
0.53,0.535,0.54,0.545,0.55,0.555,0.56,0.565,0.57,0.575,0.58,0.585,0.59,
0.595,0.6,0.605,0.61,0.615,0.62,0.625,0.63,0.635,0.64,0.645,0.65,0.655,
0.66,0.665,0.67,0.675,0.68,0.685,0.690000000000001,0.695000000000001,0.700000000000001,
0.705000000000001,0.710000000000001,0.715000000000001,0.720000000000001,
0.725000000000001,0.730000000000001,0.735000000000001,0.740000000000001,
0.745000000000001,0.750000000000001,0.755000000000001,0.760000000000001,
0.765000000000001,0.770000000000001,0.775000000000001,0.780000000000001,
0.785000000000001,0.790000000000001,0.795000000000001,0.800000000000001,
0.805000000000001,0.810000000000001,0.815000000000001,0.820000000000001,
0.825000000000001,0.830000000000001,0.835000000000001,0.840000000000001,
0.845000000000001,0.850000000000001,0.855000000000001,0.860000000000001,
0.865000000000001,0.870000000000001,0.875000000000001,0.880000000000001,
0.885000000000001,0.890000000000001,0.895000000000001,0.900000000000001,
0.905000000000001,0.910000000000001,0.915000000000001,0.920000000000001,
0.925000000000001,0.930000000000001,0.935000000000001,0.940000000000001,
0.945000000000001,0.950000000000001,0.955000000000001,0.960000000000001,
0.965000000000001,0.970000000000001,0.975000000000001,0.980000000000001,
0.985000000000001,0.990000000000001,0.995000000000001,1.),(0.,1.2),
 .UNSPECIFIED.)
GEOMETRIC_REPRESENTATION_ITEM()
RATIONAL_B_SPLINE_SURFACE(((1.,1.),(1.,1.),(1.,1.),(1.,1.),(1.,1.),(1.,
1.),(1.,1.),(1.,1.),(1.,1.),(1.,1.),(1.,1.),(1.,1.),(1.,1.),(1.,1.),(1.,
1.),(1.,1.),(1.,1.),(1.,1.),(1.,1.),(1.,1.),(1.,1.),(1.,1.),(1.,1.),(1.,
1.),(1.,1.),(1.,1.),(1.,1.),(1.,1.),(1.,1.),(1.,1.),(1.,1.),(1.,1.),(1.,
1.),(1.,1.),(1.,1.),(1.,1.),(1.,1.),(1.,1.),(1.,1.),(1.,1.),(1.,1.),(1.,
1.),(1.,1.),(1.,1.),(1.,1.),(1.,1.),(1.,1.),(1.,1.),(1.,1.),(1.,1.),(1.,
1.),(1.,1.),(1.,1.),(1.,1.),(1.,1.),(1.,1.),(1.,1.),(1.,1.),(1.,1.),(1.,
1.),(1.,1.),(1.,1.),(1.,1.),(1.,1.),(1.,1.),(1.,1.),(1.,1.),(1.,1.),(1.,
1.),(1.,1.),(1.,1.),(1.,1.),(1.,1.),(1.,1.),(1.,1.),(1.,1.),(1.,1.),(1.,
1.),(1.,1.),(1.,1.),(1.,1.),(1.,1.),(1.,1.),(1.,1.),(1.,1.),(1.,1.),(1.,
1.),(1.,1.),(1.,1.),(1.,1.),(1.,1.),(1.,1.),(1.,1.),(1.,1.),(1.,1.),(1.,
1.),(1.,1.),(1.,1.),(1.,1.),(1.,1.),(1.,1.),(1.,1.),(1.,1.),(1.,1.),(1.,
1.),(1.,1.),(1.,1.),(1.,1.),(1.,1.),(1.,1.),(1.,1.),(1.,1.),(1.,1.),(1.,
1.),(1.,1.),(1.,1.),(1.,1.),(1.,1.),(1.,1.),(1.,1.),(1.,1.),(1.,1.),(1.,
1.),(1.,1.),(1.,1.),(1.,1.),(1.,1.),(1.,1.),(1.,1.),(1.,1.),(1.,1.),(1.,
1.),(1.,1.),(1.,1.),(1.,1.),(1.,1.),(1.,1.),(1.,1.),(1.,1.),(1.,1.),(1.,
1.),(1.,1.),(1.,1.),(1.,1.),(1.,1.),(1.,1.),(1.,1.),(1.,1.),(1.,1.),(1.,
1.),(1.,1.),(1.,1.),(1.,1.),(1.,1.),(1.,1.),(1.,1.),(1.,1.),(1.,1.),(1.,
1.),(1.,1.),(1.,1.),(1.,1.),(1.,1.),(1.,1.),(1.,1.),(1.,1.),(1.,1.),(1.,
1.),(1.,1.),(1.,1.),(1.,1.),(1.,1.),(1.,1.),(1.,1.),(1.,1.),(1.,1.),(1.,
1.),(1.,1.),(1.,1.),(1.,1.),(1.,1.),(1.,1.),(1.,1.),(1.,1.),(1.,1.),(1.,
1.),(1.,1.),(1.,1.),(1.,1.),(1.,1.),(1.,1.),(1.,1.),(1.,1.),(1.,1.),(1.,
1.),(1.,1.),(1.,1.),(1.,1.),(1.,1.),(1.,1.),(1.,1.),(1.,1.),(1.,1.),(1.,
1.),(1.,1.)))
REPRESENTATION_ITEM('')
SURFACE()
);
#944=(
BOUNDED_SURFACE()
B_SPLINE_SURFACE(5,1,((#107278,#107279),(#107280,#107281),(#107282,#107283),
(#107284,#107285),(#107286,#107287),(#107288,#107289),(#107290,#107291),
(#107292,#107293),(#107294,#107295),(#107296,#107297),(#107298,#107299),
(#107300,#107301),(#107302,#107303),(#107304,#107305),(#107306,#107307),
(#107308,#107309),(#107310,#107311),(#107312,#107313),(#107314,#107315),
(#107316,#107317),(#107318,#107319),(#107320,#107321),(#107322,#107323),
(#107324,#107325),(#107326,#107327),(#107328,#107329),(#107330,#107331),
(#107332,#107333),(#107334,#107335),(#107336,#107337),(#107338,#107339),
(#107340,#107341),(#107342,#107343),(#107344,#107345),(#107346,#107347),
(#107348,#107349),(#107350,#107351),(#107352,#107353),(#107354,#107355),
(#107356,#107357),(#107358,#107359),(#107360,#107361),(#107362,#107363),
(#107364,#107365),(#107366,#107367),(#107368,#107369),(#107370,#107371),
(#107372,#107373),(#107374,#107375),(#107376,#107377),(#107378,#107379),
(#107380,#107381),(#107382,#107383),(#107384,#107385),(#107386,#107387),
(#107388,#107389),(#107390,#107391),(#107392,#107393),(#107394,#107395),
(#107396,#107397),(#107398,#107399),(#107400,#107401),(#107402,#107403),
(#107404,#107405),(#107406,#107407),(#107408,#107409),(#107410,#107411),
(#107412,#107413),(#107414,#107415),(#107416,#107417),(#107418,#107419),
(#107420,#107421),(#107422,#107423),(#107424,#107425),(#107426,#107427),
(#107428,#107429),(#107430,#107431),(#107432,#107433),(#107434,#107435),
(#107436,#107437),(#107438,#107439),(#107440,#107441),(#107442,#107443),
(#107444,#107445),(#107446,#107447),(#107448,#107449),(#107450,#107451),
(#107452,#107453),(#107454,#107455),(#107456,#107457),(#107458,#107459),
(#107460,#107461),(#107462,#107463),(#107464,#107465),(#107466,#107467),
(#107468,#107469),(#107470,#107471),(#107472,#107473),(#107474,#107475),
(#107476,#107477),(#107478,#107479),(#107480,#107481),(#107482,#107483),
(#107484,#107485),(#107486,#107487),(#107488,#107489),(#107490,#107491),
(#107492,#107493),(#107494,#107495),(#107496,#107497),(#107498,#107499),
(#107500,#107501),(#107502,#107503),(#107504,#107505),(#107506,#107507),
(#107508,#107509),(#107510,#107511),(#107512,#107513),(#107514,#107515),
(#107516,#107517),(#107518,#107519),(#107520,#107521),(#107522,#107523),
(#107524,#107525),(#107526,#107527),(#107528,#107529),(#107530,#107531),
(#107532,#107533),(#107534,#107535),(#107536,#107537),(#107538,#107539),
(#107540,#107541),(#107542,#107543),(#107544,#107545),(#107546,#107547),
(#107548,#107549),(#107550,#107551),(#107552,#107553),(#107554,#107555),
(#107556,#107557),(#107558,#107559),(#107560,#107561),(#107562,#107563),
(#107564,#107565),(#107566,#107567),(#107568,#107569),(#107570,#107571),
(#107572,#107573),(#107574,#107575),(#107576,#107577),(#107578,#107579),
(#107580,#107581),(#107582,#107583),(#107584,#107585),(#107586,#107587),
(#107588,#107589),(#107590,#107591),(#107592,#107593),(#107594,#107595),
(#107596,#107597),(#107598,#107599),(#107600,#107601),(#107602,#107603),
(#107604,#107605),(#107606,#107607),(#107608,#107609),(#107610,#107611),
(#107612,#107613),(#107614,#107615),(#107616,#107617),(#107618,#107619),
(#107620,#107621),(#107622,#107623),(#107624,#107625),(#107626,#107627),
(#107628,#107629),(#107630,#107631),(#107632,#107633),(#107634,#107635),
(#107636,#107637),(#107638,#107639),(#107640,#107641),(#107642,#107643),
(#107644,#107645),(#107646,#107647),(#107648,#107649),(#107650,#107651),
(#107652,#107653),(#107654,#107655),(#107656,#107657),(#107658,#107659),
(#107660,#107661),(#107662,#107663),(#107664,#107665),(#107666,#107667),
(#107668,#107669),(#107670,#107671),(#107672,#107673),(#107674,#107675),
(#107676,#107677),(#107678,#107679),(#107680,#107681),(#107682,#107683),
(#107684,#107685),(#107686,#107687)),.UNSPECIFIED.,.F.,.F.,.F.)
B_SPLINE_SURFACE_WITH_KNOTS((6,1,1,1,1,1,1,1,1,1,1,1,1,1,1,1,1,1,1,1,1,
1,1,1,1,1,1,1,1,1,1,1,1,1,1,1,1,1,1,1,1,1,1,1,1,1,1,1,1,1,1,1,1,1,1,1,1,
1,1,1,1,1,1,1,1,1,1,1,1,1,1,1,1,1,1,1,1,1,1,1,1,1,1,1,1,1,1,1,1,1,1,1,1,
1,1,1,1,1,1,1,1,1,1,1,1,1,1,1,1,1,1,1,1,1,1,1,1,1,1,1,1,1,1,1,1,1,1,1,1,
1,1,1,1,1,1,1,1,1,1,1,1,1,1,1,1,1,1,1,1,1,1,1,1,1,1,1,1,1,1,1,1,1,1,1,1,
1,1,1,1,1,1,1,1,1,1,1,1,1,1,1,1,1,1,1,1,1,1,1,1,1,1,1,1,1,1,1,1,1,1,1,6),
(2,2),(0.,0.005,0.01,0.015,0.02,0.025,0.03,0.035,0.04,0.045,0.05,0.055,
0.06,0.065,0.07,0.075,0.08,0.085,0.09,0.095,0.1,0.105,0.11,0.115,0.12,0.125,
0.13,0.135,0.14,0.145,0.15,0.155,0.16,0.165,0.17,0.175,0.18,0.185,0.19,
0.195,0.2,0.205,0.21,0.215,0.22,0.225,0.23,0.235,0.24,0.245,0.25,0.255,
0.26,0.265,0.27,0.275,0.28,0.285,0.29,0.295,0.3,0.305,0.31,0.315,0.32,0.325,
0.33,0.335,0.34,0.345,0.35,0.355,0.36,0.365,0.37,0.375,0.38,0.385,0.39,
0.395,0.4,0.405,0.41,0.415,0.42,0.425,0.43,0.435,0.44,0.445,0.45,0.455,
0.46,0.465,0.47,0.475,0.48,0.485,0.49,0.495,0.5,0.505,0.51,0.515,0.52,0.525,
0.53,0.535,0.54,0.545,0.55,0.555,0.56,0.565,0.57,0.575,0.58,0.585,0.59,
0.595,0.6,0.605,0.61,0.615,0.62,0.625,0.63,0.635,0.64,0.645,0.65,0.655,
0.66,0.665,0.67,0.675,0.68,0.685,0.690000000000001,0.695000000000001,0.700000000000001,
0.705000000000001,0.710000000000001,0.715000000000001,0.720000000000001,
0.725000000000001,0.730000000000001,0.735000000000001,0.740000000000001,
0.745000000000001,0.750000000000001,0.755000000000001,0.760000000000001,
0.765000000000001,0.770000000000001,0.775000000000001,0.780000000000001,
0.785000000000001,0.790000000000001,0.795000000000001,0.800000000000001,
0.805000000000001,0.810000000000001,0.815000000000001,0.820000000000001,
0.825000000000001,0.830000000000001,0.835000000000001,0.840000000000001,
0.845000000000001,0.850000000000001,0.855000000000001,0.860000000000001,
0.865000000000001,0.870000000000001,0.875000000000001,0.880000000000001,
0.885000000000001,0.890000000000001,0.895000000000001,0.900000000000001,
0.905000000000001,0.910000000000001,0.915000000000001,0.920000000000001,
0.925000000000001,0.930000000000001,0.935000000000001,0.940000000000001,
0.945000000000001,0.950000000000001,0.955000000000001,0.960000000000001,
0.965000000000001,0.970000000000001,0.975000000000001,0.980000000000001,
0.985000000000001,0.990000000000001,0.995000000000001,1.),(0.,1.2),
 .UNSPECIFIED.)
GEOMETRIC_REPRESENTATION_ITEM()
RATIONAL_B_SPLINE_SURFACE(((1.,1.),(1.,1.),(1.,1.),(1.,1.),(1.,1.),(1.,
1.),(1.,1.),(1.,1.),(1.,1.),(1.,1.),(1.,1.),(1.,1.),(1.,1.),(1.,1.),(1.,
1.),(1.,1.),(1.,1.),(1.,1.),(1.,1.),(1.,1.),(1.,1.),(1.,1.),(1.,1.),(1.,
1.),(1.,1.),(1.,1.),(1.,1.),(1.,1.),(1.,1.),(1.,1.),(1.,1.),(1.,1.),(1.,
1.),(1.,1.),(1.,1.),(1.,1.),(1.,1.),(1.,1.),(1.,1.),(1.,1.),(1.,1.),(1.,
1.),(1.,1.),(1.,1.),(1.,1.),(1.,1.),(1.,1.),(1.,1.),(1.,1.),(1.,1.),(1.,
1.),(1.,1.),(1.,1.),(1.,1.),(1.,1.),(1.,1.),(1.,1.),(1.,1.),(1.,1.),(1.,
1.),(1.,1.),(1.,1.),(1.,1.),(1.,1.),(1.,1.),(1.,1.),(1.,1.),(1.,1.),(1.,
1.),(1.,1.),(1.,1.),(1.,1.),(1.,1.),(1.,1.),(1.,1.),(1.,1.),(1.,1.),(1.,
1.),(1.,1.),(1.,1.),(1.,1.),(1.,1.),(1.,1.),(1.,1.),(1.,1.),(1.,1.),(1.,
1.),(1.,1.),(1.,1.),(1.,1.),(1.,1.),(1.,1.),(1.,1.),(1.,1.),(1.,1.),(1.,
1.),(1.,1.),(1.,1.),(1.,1.),(1.,1.),(1.,1.),(1.,1.),(1.,1.),(1.,1.),(1.,
1.),(1.,1.),(1.,1.),(1.,1.),(1.,1.),(1.,1.),(1.,1.),(1.,1.),(1.,1.),(1.,
1.),(1.,1.),(1.,1.),(1.,1.),(1.,1.),(1.,1.),(1.,1.),(1.,1.),(1.,1.),(1.,
1.),(1.,1.),(1.,1.),(1.,1.),(1.,1.),(1.,1.),(1.,1.),(1.,1.),(1.,1.),(1.,
1.),(1.,1.),(1.,1.),(1.,1.),(1.,1.),(1.,1.),(1.,1.),(1.,1.),(1.,1.),(1.,
1.),(1.,1.),(1.,1.),(1.,1.),(1.,1.),(1.,1.),(1.,1.),(1.,1.),(1.,1.),(1.,
1.),(1.,1.),(1.,1.),(1.,1.),(1.,1.),(1.,1.),(1.,1.),(1.,1.),(1.,1.),(1.,
1.),(1.,1.),(1.,1.),(1.,1.),(1.,1.),(1.,1.),(1.,1.),(1.,1.),(1.,1.),(1.,
1.),(1.,1.),(1.,1.),(1.,1.),(1.,1.),(1.,1.),(1.,1.),(1.,1.),(1.,1.),(1.,
1.),(1.,1.),(1.,1.),(1.,1.),(1.,1.),(1.,1.),(1.,1.),(1.,1.),(1.,1.),(1.,
1.),(1.,1.),(1.,1.),(1.,1.),(1.,1.),(1.,1.),(1.,1.),(1.,1.),(1.,1.),(1.,
1.),(1.,1.),(1.,1.),(1.,1.),(1.,1.),(1.,1.),(1.,1.),(1.,1.),(1.,1.),(1.,
1.),(1.,1.)))
REPRESENTATION_ITEM('')
SURFACE()
);
#945=(
BOUNDED_SURFACE()
B_SPLINE_SURFACE(5,1,((#108174,#108175),(#108176,#108177),(#108178,#108179),
(#108180,#108181),(#108182,#108183),(#108184,#108185),(#108186,#108187),
(#108188,#108189),(#108190,#108191),(#108192,#108193),(#108194,#108195),
(#108196,#108197),(#108198,#108199),(#108200,#108201),(#108202,#108203),
(#108204,#108205),(#108206,#108207),(#108208,#108209),(#108210,#108211),
(#108212,#108213),(#108214,#108215),(#108216,#108217),(#108218,#108219),
(#108220,#108221),(#108222,#108223),(#108224,#108225),(#108226,#108227),
(#108228,#108229),(#108230,#108231),(#108232,#108233),(#108234,#108235),
(#108236,#108237),(#108238,#108239),(#108240,#108241),(#108242,#108243),
(#108244,#108245),(#108246,#108247),(#108248,#108249),(#108250,#108251),
(#108252,#108253),(#108254,#108255),(#108256,#108257),(#108258,#108259),
(#108260,#108261),(#108262,#108263),(#108264,#108265),(#108266,#108267),
(#108268,#108269),(#108270,#108271),(#108272,#108273),(#108274,#108275),
(#108276,#108277),(#108278,#108279),(#108280,#108281),(#108282,#108283),
(#108284,#108285),(#108286,#108287),(#108288,#108289),(#108290,#108291),
(#108292,#108293),(#108294,#108295),(#108296,#108297),(#108298,#108299),
(#108300,#108301),(#108302,#108303),(#108304,#108305),(#108306,#108307),
(#108308,#108309),(#108310,#108311),(#108312,#108313),(#108314,#108315),
(#108316,#108317),(#108318,#108319),(#108320,#108321),(#108322,#108323),
(#108324,#108325),(#108326,#108327),(#108328,#108329),(#108330,#108331),
(#108332,#108333),(#108334,#108335),(#108336,#108337),(#108338,#108339),
(#108340,#108341),(#108342,#108343),(#108344,#108345),(#108346,#108347),
(#108348,#108349),(#108350,#108351),(#108352,#108353),(#108354,#108355),
(#108356,#108357),(#108358,#108359),(#108360,#108361),(#108362,#108363),
(#108364,#108365),(#108366,#108367),(#108368,#108369),(#108370,#108371),
(#108372,#108373),(#108374,#108375),(#108376,#108377),(#108378,#108379),
(#108380,#108381),(#108382,#108383),(#108384,#108385),(#108386,#108387),
(#108388,#108389),(#108390,#108391),(#108392,#108393),(#108394,#108395),
(#108396,#108397),(#108398,#108399),(#108400,#108401),(#108402,#108403),
(#108404,#108405),(#108406,#108407),(#108408,#108409),(#108410,#108411),
(#108412,#108413),(#108414,#108415),(#108416,#108417),(#108418,#108419),
(#108420,#108421),(#108422,#108423),(#108424,#108425),(#108426,#108427),
(#108428,#108429),(#108430,#108431),(#108432,#108433),(#108434,#108435),
(#108436,#108437),(#108438,#108439),(#108440,#108441),(#108442,#108443),
(#108444,#108445),(#108446,#108447),(#108448,#108449),(#108450,#108451),
(#108452,#108453),(#108454,#108455),(#108456,#108457),(#108458,#108459),
(#108460,#108461),(#108462,#108463),(#108464,#108465),(#108466,#108467),
(#108468,#108469),(#108470,#108471),(#108472,#108473),(#108474,#108475),
(#108476,#108477),(#108478,#108479),(#108480,#108481),(#108482,#108483),
(#108484,#108485),(#108486,#108487),(#108488,#108489),(#108490,#108491),
(#108492,#108493),(#108494,#108495),(#108496,#108497),(#108498,#108499),
(#108500,#108501),(#108502,#108503),(#108504,#108505),(#108506,#108507),
(#108508,#108509),(#108510,#108511),(#108512,#108513),(#108514,#108515),
(#108516,#108517),(#108518,#108519),(#108520,#108521),(#108522,#108523),
(#108524,#108525),(#108526,#108527),(#108528,#108529),(#108530,#108531),
(#108532,#108533),(#108534,#108535),(#108536,#108537),(#108538,#108539),
(#108540,#108541),(#108542,#108543),(#108544,#108545),(#108546,#108547),
(#108548,#108549),(#108550,#108551),(#108552,#108553),(#108554,#108555),
(#108556,#108557),(#108558,#108559),(#108560,#108561),(#108562,#108563),
(#108564,#108565),(#108566,#108567),(#108568,#108569),(#108570,#108571),
(#108572,#108573),(#108574,#108575),(#108576,#108577),(#108578,#108579),
(#108580,#108581),(#108582,#108583)),.UNSPECIFIED.,.F.,.F.,.F.)
B_SPLINE_SURFACE_WITH_KNOTS((6,1,1,1,1,1,1,1,1,1,1,1,1,1,1,1,1,1,1,1,1,
1,1,1,1,1,1,1,1,1,1,1,1,1,1,1,1,1,1,1,1,1,1,1,1,1,1,1,1,1,1,1,1,1,1,1,1,
1,1,1,1,1,1,1,1,1,1,1,1,1,1,1,1,1,1,1,1,1,1,1,1,1,1,1,1,1,1,1,1,1,1,1,1,
1,1,1,1,1,1,1,1,1,1,1,1,1,1,1,1,1,1,1,1,1,1,1,1,1,1,1,1,1,1,1,1,1,1,1,1,
1,1,1,1,1,1,1,1,1,1,1,1,1,1,1,1,1,1,1,1,1,1,1,1,1,1,1,1,1,1,1,1,1,1,1,1,
1,1,1,1,1,1,1,1,1,1,1,1,1,1,1,1,1,1,1,1,1,1,1,1,1,1,1,1,1,1,1,1,1,1,1,6),
(2,2),(0.,0.005,0.01,0.015,0.02,0.025,0.03,0.035,0.04,0.045,0.05,0.055,
0.06,0.065,0.07,0.075,0.08,0.085,0.09,0.095,0.1,0.105,0.11,0.115,0.12,0.125,
0.13,0.135,0.14,0.145,0.15,0.155,0.16,0.165,0.17,0.175,0.18,0.185,0.19,
0.195,0.2,0.205,0.21,0.215,0.22,0.225,0.23,0.235,0.24,0.245,0.25,0.255,
0.26,0.265,0.27,0.275,0.28,0.285,0.29,0.295,0.3,0.305,0.31,0.315,0.32,0.325,
0.33,0.335,0.34,0.345,0.35,0.355,0.36,0.365,0.37,0.375,0.38,0.385,0.39,
0.395,0.4,0.405,0.41,0.415,0.42,0.425,0.43,0.435,0.44,0.445,0.45,0.455,
0.46,0.465,0.47,0.475,0.48,0.485,0.49,0.495,0.5,0.505,0.51,0.515,0.52,0.525,
0.53,0.535,0.54,0.545,0.55,0.555,0.56,0.565,0.57,0.575,0.58,0.585,0.59,
0.595,0.6,0.605,0.61,0.615,0.62,0.625,0.63,0.635,0.64,0.645,0.65,0.655,
0.66,0.665,0.67,0.675,0.68,0.685,0.690000000000001,0.695000000000001,0.700000000000001,
0.705000000000001,0.710000000000001,0.715000000000001,0.720000000000001,
0.725000000000001,0.730000000000001,0.735000000000001,0.740000000000001,
0.745000000000001,0.750000000000001,0.755000000000001,0.760000000000001,
0.765000000000001,0.770000000000001,0.775000000000001,0.780000000000001,
0.785000000000001,0.790000000000001,0.795000000000001,0.800000000000001,
0.805000000000001,0.810000000000001,0.815000000000001,0.820000000000001,
0.825000000000001,0.830000000000001,0.835000000000001,0.840000000000001,
0.845000000000001,0.850000000000001,0.855000000000001,0.860000000000001,
0.865000000000001,0.870000000000001,0.875000000000001,0.880000000000001,
0.885000000000001,0.890000000000001,0.895000000000001,0.900000000000001,
0.905000000000001,0.910000000000001,0.915000000000001,0.920000000000001,
0.925000000000001,0.930000000000001,0.935000000000001,0.940000000000001,
0.945000000000001,0.950000000000001,0.955000000000001,0.960000000000001,
0.965000000000001,0.970000000000001,0.975000000000001,0.980000000000001,
0.985000000000001,0.990000000000001,0.995000000000001,1.),(0.,1.2),
 .UNSPECIFIED.)
GEOMETRIC_REPRESENTATION_ITEM()
RATIONAL_B_SPLINE_SURFACE(((1.,1.),(1.,1.),(1.,1.),(1.,1.),(1.,1.),(1.,
1.),(1.,1.),(1.,1.),(1.,1.),(1.,1.),(1.,1.),(1.,1.),(1.,1.),(1.,1.),(1.,
1.),(1.,1.),(1.,1.),(1.,1.),(1.,1.),(1.,1.),(1.,1.),(1.,1.),(1.,1.),(1.,
1.),(1.,1.),(1.,1.),(1.,1.),(1.,1.),(1.,1.),(1.,1.),(1.,1.),(1.,1.),(1.,
1.),(1.,1.),(1.,1.),(1.,1.),(1.,1.),(1.,1.),(1.,1.),(1.,1.),(1.,1.),(1.,
1.),(1.,1.),(1.,1.),(1.,1.),(1.,1.),(1.,1.),(1.,1.),(1.,1.),(1.,1.),(1.,
1.),(1.,1.),(1.,1.),(1.,1.),(1.,1.),(1.,1.),(1.,1.),(1.,1.),(1.,1.),(1.,
1.),(1.,1.),(1.,1.),(1.,1.),(1.,1.),(1.,1.),(1.,1.),(1.,1.),(1.,1.),(1.,
1.),(1.,1.),(1.,1.),(1.,1.),(1.,1.),(1.,1.),(1.,1.),(1.,1.),(1.,1.),(1.,
1.),(1.,1.),(1.,1.),(1.,1.),(1.,1.),(1.,1.),(1.,1.),(1.,1.),(1.,1.),(1.,
1.),(1.,1.),(1.,1.),(1.,1.),(1.,1.),(1.,1.),(1.,1.),(1.,1.),(1.,1.),(1.,
1.),(1.,1.),(1.,1.),(1.,1.),(1.,1.),(1.,1.),(1.,1.),(1.,1.),(1.,1.),(1.,
1.),(1.,1.),(1.,1.),(1.,1.),(1.,1.),(1.,1.),(1.,1.),(1.,1.),(1.,1.),(1.,
1.),(1.,1.),(1.,1.),(1.,1.),(1.,1.),(1.,1.),(1.,1.),(1.,1.),(1.,1.),(1.,
1.),(1.,1.),(1.,1.),(1.,1.),(1.,1.),(1.,1.),(1.,1.),(1.,1.),(1.,1.),(1.,
1.),(1.,1.),(1.,1.),(1.,1.),(1.,1.),(1.,1.),(1.,1.),(1.,1.),(1.,1.),(1.,
1.),(1.,1.),(1.,1.),(1.,1.),(1.,1.),(1.,1.),(1.,1.),(1.,1.),(1.,1.),(1.,
1.),(1.,1.),(1.,1.),(1.,1.),(1.,1.),(1.,1.),(1.,1.),(1.,1.),(1.,1.),(1.,
1.),(1.,1.),(1.,1.),(1.,1.),(1.,1.),(1.,1.),(1.,1.),(1.,1.),(1.,1.),(1.,
1.),(1.,1.),(1.,1.),(1.,1.),(1.,1.),(1.,1.),(1.,1.),(1.,1.),(1.,1.),(1.,
1.),(1.,1.),(1.,1.),(1.,1.),(1.,1.),(1.,1.),(1.,1.),(1.,1.),(1.,1.),(1.,
1.),(1.,1.),(1.,1.),(1.,1.),(1.,1.),(1.,1.),(1.,1.),(1.,1.),(1.,1.),(1.,
1.),(1.,1.),(1.,1.),(1.,1.),(1.,1.),(1.,1.),(1.,1.),(1.,1.),(1.,1.),(1.,
1.),(1.,1.)))
REPRESENTATION_ITEM('')
SURFACE()
);
#946=(
BOUNDED_SURFACE()
B_SPLINE_SURFACE(5,1,((#109070,#109071),(#109072,#109073),(#109074,#109075),
(#109076,#109077),(#109078,#109079),(#109080,#109081),(#109082,#109083),
(#109084,#109085),(#109086,#109087),(#109088,#109089),(#109090,#109091),
(#109092,#109093),(#109094,#109095),(#109096,#109097),(#109098,#109099),
(#109100,#109101),(#109102,#109103),(#109104,#109105),(#109106,#109107),
(#109108,#109109),(#109110,#109111),(#109112,#109113),(#109114,#109115),
(#109116,#109117),(#109118,#109119),(#109120,#109121),(#109122,#109123),
(#109124,#109125),(#109126,#109127),(#109128,#109129),(#109130,#109131),
(#109132,#109133),(#109134,#109135),(#109136,#109137),(#109138,#109139),
(#109140,#109141),(#109142,#109143),(#109144,#109145),(#109146,#109147),
(#109148,#109149),(#109150,#109151),(#109152,#109153),(#109154,#109155),
(#109156,#109157),(#109158,#109159),(#109160,#109161),(#109162,#109163),
(#109164,#109165),(#109166,#109167),(#109168,#109169),(#109170,#109171),
(#109172,#109173),(#109174,#109175),(#109176,#109177),(#109178,#109179),
(#109180,#109181),(#109182,#109183),(#109184,#109185),(#109186,#109187),
(#109188,#109189),(#109190,#109191),(#109192,#109193),(#109194,#109195),
(#109196,#109197),(#109198,#109199),(#109200,#109201),(#109202,#109203),
(#109204,#109205),(#109206,#109207),(#109208,#109209),(#109210,#109211),
(#109212,#109213),(#109214,#109215),(#109216,#109217),(#109218,#109219),
(#109220,#109221),(#109222,#109223),(#109224,#109225),(#109226,#109227),
(#109228,#109229),(#109230,#109231),(#109232,#109233),(#109234,#109235),
(#109236,#109237),(#109238,#109239),(#109240,#109241),(#109242,#109243),
(#109244,#109245),(#109246,#109247),(#109248,#109249),(#109250,#109251),
(#109252,#109253),(#109254,#109255),(#109256,#109257),(#109258,#109259),
(#109260,#109261),(#109262,#109263),(#109264,#109265),(#109266,#109267),
(#109268,#109269),(#109270,#109271),(#109272,#109273),(#109274,#109275),
(#109276,#109277),(#109278,#109279),(#109280,#109281),(#109282,#109283),
(#109284,#109285),(#109286,#109287),(#109288,#109289),(#109290,#109291),
(#109292,#109293),(#109294,#109295),(#109296,#109297),(#109298,#109299),
(#109300,#109301),(#109302,#109303),(#109304,#109305),(#109306,#109307),
(#109308,#109309),(#109310,#109311),(#109312,#109313),(#109314,#109315),
(#109316,#109317),(#109318,#109319),(#109320,#109321),(#109322,#109323),
(#109324,#109325),(#109326,#109327),(#109328,#109329),(#109330,#109331),
(#109332,#109333),(#109334,#109335),(#109336,#109337),(#109338,#109339),
(#109340,#109341),(#109342,#109343),(#109344,#109345),(#109346,#109347),
(#109348,#109349),(#109350,#109351),(#109352,#109353),(#109354,#109355),
(#109356,#109357),(#109358,#109359),(#109360,#109361),(#109362,#109363),
(#109364,#109365),(#109366,#109367),(#109368,#109369),(#109370,#109371),
(#109372,#109373),(#109374,#109375),(#109376,#109377),(#109378,#109379),
(#109380,#109381),(#109382,#109383),(#109384,#109385),(#109386,#109387),
(#109388,#109389),(#109390,#109391),(#109392,#109393),(#109394,#109395),
(#109396,#109397),(#109398,#109399),(#109400,#109401),(#109402,#109403),
(#109404,#109405),(#109406,#109407),(#109408,#109409),(#109410,#109411),
(#109412,#109413),(#109414,#109415),(#109416,#109417),(#109418,#109419),
(#109420,#109421),(#109422,#109423),(#109424,#109425),(#109426,#109427),
(#109428,#109429),(#109430,#109431),(#109432,#109433),(#109434,#109435),
(#109436,#109437),(#109438,#109439),(#109440,#109441),(#109442,#109443),
(#109444,#109445),(#109446,#109447),(#109448,#109449),(#109450,#109451),
(#109452,#109453),(#109454,#109455),(#109456,#109457),(#109458,#109459),
(#109460,#109461),(#109462,#109463),(#109464,#109465),(#109466,#109467),
(#109468,#109469),(#109470,#109471),(#109472,#109473),(#109474,#109475),
(#109476,#109477),(#109478,#109479)),.UNSPECIFIED.,.F.,.F.,.F.)
B_SPLINE_SURFACE_WITH_KNOTS((6,1,1,1,1,1,1,1,1,1,1,1,1,1,1,1,1,1,1,1,1,
1,1,1,1,1,1,1,1,1,1,1,1,1,1,1,1,1,1,1,1,1,1,1,1,1,1,1,1,1,1,1,1,1,1,1,1,
1,1,1,1,1,1,1,1,1,1,1,1,1,1,1,1,1,1,1,1,1,1,1,1,1,1,1,1,1,1,1,1,1,1,1,1,
1,1,1,1,1,1,1,1,1,1,1,1,1,1,1,1,1,1,1,1,1,1,1,1,1,1,1,1,1,1,1,1,1,1,1,1,
1,1,1,1,1,1,1,1,1,1,1,1,1,1,1,1,1,1,1,1,1,1,1,1,1,1,1,1,1,1,1,1,1,1,1,1,
1,1,1,1,1,1,1,1,1,1,1,1,1,1,1,1,1,1,1,1,1,1,1,1,1,1,1,1,1,1,1,1,1,1,1,6),
(2,2),(0.,0.005,0.01,0.015,0.02,0.025,0.03,0.035,0.04,0.045,0.05,0.055,
0.06,0.065,0.07,0.075,0.08,0.085,0.09,0.095,0.1,0.105,0.11,0.115,0.12,0.125,
0.13,0.135,0.14,0.145,0.15,0.155,0.16,0.165,0.17,0.175,0.18,0.185,0.19,
0.195,0.2,0.205,0.21,0.215,0.22,0.225,0.23,0.235,0.24,0.245,0.25,0.255,
0.26,0.265,0.27,0.275,0.28,0.285,0.29,0.295,0.3,0.305,0.31,0.315,0.32,0.325,
0.33,0.335,0.34,0.345,0.35,0.355,0.36,0.365,0.37,0.375,0.38,0.385,0.39,
0.395,0.4,0.405,0.41,0.415,0.42,0.425,0.43,0.435,0.44,0.445,0.45,0.455,
0.46,0.465,0.47,0.475,0.48,0.485,0.49,0.495,0.5,0.505,0.51,0.515,0.52,0.525,
0.53,0.535,0.54,0.545,0.55,0.555,0.56,0.565,0.57,0.575,0.58,0.585,0.59,
0.595,0.6,0.605,0.61,0.615,0.62,0.625,0.63,0.635,0.64,0.645,0.65,0.655,
0.66,0.665,0.67,0.675,0.68,0.685,0.690000000000001,0.695000000000001,0.700000000000001,
0.705000000000001,0.710000000000001,0.715000000000001,0.720000000000001,
0.725000000000001,0.730000000000001,0.735000000000001,0.740000000000001,
0.745000000000001,0.750000000000001,0.755000000000001,0.760000000000001,
0.765000000000001,0.770000000000001,0.775000000000001,0.780000000000001,
0.785000000000001,0.790000000000001,0.795000000000001,0.800000000000001,
0.805000000000001,0.810000000000001,0.815000000000001,0.820000000000001,
0.825000000000001,0.830000000000001,0.835000000000001,0.840000000000001,
0.845000000000001,0.850000000000001,0.855000000000001,0.860000000000001,
0.865000000000001,0.870000000000001,0.875000000000001,0.880000000000001,
0.885000000000001,0.890000000000001,0.895000000000001,0.900000000000001,
0.905000000000001,0.910000000000001,0.915000000000001,0.920000000000001,
0.925000000000001,0.930000000000001,0.935000000000001,0.940000000000001,
0.945000000000001,0.950000000000001,0.955000000000001,0.960000000000001,
0.965000000000001,0.970000000000001,0.975000000000001,0.980000000000001,
0.985000000000001,0.990000000000001,0.995000000000001,1.),(0.,1.2),
 .UNSPECIFIED.)
GEOMETRIC_REPRESENTATION_ITEM()
RATIONAL_B_SPLINE_SURFACE(((1.,1.),(1.,1.),(1.,1.),(1.,1.),(1.,1.),(1.,
1.),(1.,1.),(1.,1.),(1.,1.),(1.,1.),(1.,1.),(1.,1.),(1.,1.),(1.,1.),(1.,
1.),(1.,1.),(1.,1.),(1.,1.),(1.,1.),(1.,1.),(1.,1.),(1.,1.),(1.,1.),(1.,
1.),(1.,1.),(1.,1.),(1.,1.),(1.,1.),(1.,1.),(1.,1.),(1.,1.),(1.,1.),(1.,
1.),(1.,1.),(1.,1.),(1.,1.),(1.,1.),(1.,1.),(1.,1.),(1.,1.),(1.,1.),(1.,
1.),(1.,1.),(1.,1.),(1.,1.),(1.,1.),(1.,1.),(1.,1.),(1.,1.),(1.,1.),(1.,
1.),(1.,1.),(1.,1.),(1.,1.),(1.,1.),(1.,1.),(1.,1.),(1.,1.),(1.,1.),(1.,
1.),(1.,1.),(1.,1.),(1.,1.),(1.,1.),(1.,1.),(1.,1.),(1.,1.),(1.,1.),(1.,
1.),(1.,1.),(1.,1.),(1.,1.),(1.,1.),(1.,1.),(1.,1.),(1.,1.),(1.,1.),(1.,
1.),(1.,1.),(1.,1.),(1.,1.),(1.,1.),(1.,1.),(1.,1.),(1.,1.),(1.,1.),(1.,
1.),(1.,1.),(1.,1.),(1.,1.),(1.,1.),(1.,1.),(1.,1.),(1.,1.),(1.,1.),(1.,
1.),(1.,1.),(1.,1.),(1.,1.),(1.,1.),(1.,1.),(1.,1.),(1.,1.),(1.,1.),(1.,
1.),(1.,1.),(1.,1.),(1.,1.),(1.,1.),(1.,1.),(1.,1.),(1.,1.),(1.,1.),(1.,
1.),(1.,1.),(1.,1.),(1.,1.),(1.,1.),(1.,1.),(1.,1.),(1.,1.),(1.,1.),(1.,
1.),(1.,1.),(1.,1.),(1.,1.),(1.,1.),(1.,1.),(1.,1.),(1.,1.),(1.,1.),(1.,
1.),(1.,1.),(1.,1.),(1.,1.),(1.,1.),(1.,1.),(1.,1.),(1.,1.),(1.,1.),(1.,
1.),(1.,1.),(1.,1.),(1.,1.),(1.,1.),(1.,1.),(1.,1.),(1.,1.),(1.,1.),(1.,
1.),(1.,1.),(1.,1.),(1.,1.),(1.,1.),(1.,1.),(1.,1.),(1.,1.),(1.,1.),(1.,
1.),(1.,1.),(1.,1.),(1.,1.),(1.,1.),(1.,1.),(1.,1.),(1.,1.),(1.,1.),(1.,
1.),(1.,1.),(1.,1.),(1.,1.),(1.,1.),(1.,1.),(1.,1.),(1.,1.),(1.,1.),(1.,
1.),(1.,1.),(1.,1.),(1.,1.),(1.,1.),(1.,1.),(1.,1.),(1.,1.),(1.,1.),(1.,
1.),(1.,1.),(1.,1.),(1.,1.),(1.,1.),(1.,1.),(1.,1.),(1.,1.),(1.,1.),(1.,
1.),(1.,1.),(1.,1.),(1.,1.),(1.,1.),(1.,1.),(1.,1.),(1.,1.),(1.,1.),(1.,
1.),(1.,1.)))
REPRESENTATION_ITEM('')
SURFACE()
);
#947=(
BOUNDED_SURFACE()
B_SPLINE_SURFACE(5,1,((#109966,#109967),(#109968,#109969),(#109970,#109971),
(#109972,#109973),(#109974,#109975),(#109976,#109977),(#109978,#109979),
(#109980,#109981),(#109982,#109983),(#109984,#109985),(#109986,#109987),
(#109988,#109989),(#109990,#109991),(#109992,#109993),(#109994,#109995),
(#109996,#109997),(#109998,#109999),(#110000,#110001),(#110002,#110003),
(#110004,#110005),(#110006,#110007),(#110008,#110009),(#110010,#110011),
(#110012,#110013),(#110014,#110015),(#110016,#110017),(#110018,#110019),
(#110020,#110021),(#110022,#110023),(#110024,#110025),(#110026,#110027),
(#110028,#110029),(#110030,#110031),(#110032,#110033),(#110034,#110035),
(#110036,#110037),(#110038,#110039),(#110040,#110041),(#110042,#110043),
(#110044,#110045),(#110046,#110047),(#110048,#110049),(#110050,#110051),
(#110052,#110053),(#110054,#110055),(#110056,#110057),(#110058,#110059),
(#110060,#110061),(#110062,#110063),(#110064,#110065),(#110066,#110067),
(#110068,#110069),(#110070,#110071),(#110072,#110073),(#110074,#110075),
(#110076,#110077),(#110078,#110079),(#110080,#110081),(#110082,#110083),
(#110084,#110085),(#110086,#110087),(#110088,#110089),(#110090,#110091),
(#110092,#110093),(#110094,#110095),(#110096,#110097),(#110098,#110099),
(#110100,#110101),(#110102,#110103),(#110104,#110105),(#110106,#110107),
(#110108,#110109),(#110110,#110111),(#110112,#110113),(#110114,#110115),
(#110116,#110117),(#110118,#110119),(#110120,#110121),(#110122,#110123),
(#110124,#110125),(#110126,#110127),(#110128,#110129),(#110130,#110131),
(#110132,#110133),(#110134,#110135),(#110136,#110137),(#110138,#110139),
(#110140,#110141),(#110142,#110143),(#110144,#110145),(#110146,#110147),
(#110148,#110149),(#110150,#110151),(#110152,#110153),(#110154,#110155),
(#110156,#110157),(#110158,#110159),(#110160,#110161),(#110162,#110163),
(#110164,#110165),(#110166,#110167),(#110168,#110169),(#110170,#110171),
(#110172,#110173),(#110174,#110175),(#110176,#110177),(#110178,#110179),
(#110180,#110181),(#110182,#110183),(#110184,#110185),(#110186,#110187),
(#110188,#110189),(#110190,#110191),(#110192,#110193),(#110194,#110195),
(#110196,#110197),(#110198,#110199),(#110200,#110201),(#110202,#110203),
(#110204,#110205),(#110206,#110207),(#110208,#110209),(#110210,#110211),
(#110212,#110213),(#110214,#110215),(#110216,#110217),(#110218,#110219),
(#110220,#110221),(#110222,#110223),(#110224,#110225),(#110226,#110227),
(#110228,#110229),(#110230,#110231),(#110232,#110233),(#110234,#110235),
(#110236,#110237),(#110238,#110239),(#110240,#110241),(#110242,#110243),
(#110244,#110245),(#110246,#110247),(#110248,#110249),(#110250,#110251),
(#110252,#110253),(#110254,#110255),(#110256,#110257),(#110258,#110259),
(#110260,#110261),(#110262,#110263),(#110264,#110265),(#110266,#110267),
(#110268,#110269),(#110270,#110271),(#110272,#110273),(#110274,#110275),
(#110276,#110277),(#110278,#110279),(#110280,#110281),(#110282,#110283),
(#110284,#110285),(#110286,#110287),(#110288,#110289),(#110290,#110291),
(#110292,#110293),(#110294,#110295),(#110296,#110297),(#110298,#110299),
(#110300,#110301),(#110302,#110303),(#110304,#110305),(#110306,#110307),
(#110308,#110309),(#110310,#110311),(#110312,#110313),(#110314,#110315),
(#110316,#110317),(#110318,#110319),(#110320,#110321),(#110322,#110323),
(#110324,#110325),(#110326,#110327),(#110328,#110329),(#110330,#110331),
(#110332,#110333),(#110334,#110335),(#110336,#110337),(#110338,#110339),
(#110340,#110341),(#110342,#110343),(#110344,#110345),(#110346,#110347),
(#110348,#110349),(#110350,#110351),(#110352,#110353),(#110354,#110355),
(#110356,#110357),(#110358,#110359),(#110360,#110361),(#110362,#110363),
(#110364,#110365),(#110366,#110367),(#110368,#110369),(#110370,#110371),
(#110372,#110373),(#110374,#110375)),.UNSPECIFIED.,.F.,.F.,.F.)
B_SPLINE_SURFACE_WITH_KNOTS((6,1,1,1,1,1,1,1,1,1,1,1,1,1,1,1,1,1,1,1,1,
1,1,1,1,1,1,1,1,1,1,1,1,1,1,1,1,1,1,1,1,1,1,1,1,1,1,1,1,1,1,1,1,1,1,1,1,
1,1,1,1,1,1,1,1,1,1,1,1,1,1,1,1,1,1,1,1,1,1,1,1,1,1,1,1,1,1,1,1,1,1,1,1,
1,1,1,1,1,1,1,1,1,1,1,1,1,1,1,1,1,1,1,1,1,1,1,1,1,1,1,1,1,1,1,1,1,1,1,1,
1,1,1,1,1,1,1,1,1,1,1,1,1,1,1,1,1,1,1,1,1,1,1,1,1,1,1,1,1,1,1,1,1,1,1,1,
1,1,1,1,1,1,1,1,1,1,1,1,1,1,1,1,1,1,1,1,1,1,1,1,1,1,1,1,1,1,1,1,1,1,1,6),
(2,2),(0.,0.005,0.01,0.015,0.02,0.025,0.03,0.035,0.04,0.045,0.05,0.055,
0.06,0.065,0.07,0.075,0.08,0.085,0.09,0.095,0.1,0.105,0.11,0.115,0.12,0.125,
0.13,0.135,0.14,0.145,0.15,0.155,0.16,0.165,0.17,0.175,0.18,0.185,0.19,
0.195,0.2,0.205,0.21,0.215,0.22,0.225,0.23,0.235,0.24,0.245,0.25,0.255,
0.26,0.265,0.27,0.275,0.28,0.285,0.29,0.295,0.3,0.305,0.31,0.315,0.32,0.325,
0.33,0.335,0.34,0.345,0.35,0.355,0.36,0.365,0.37,0.375,0.38,0.385,0.39,
0.395,0.4,0.405,0.41,0.415,0.42,0.425,0.43,0.435,0.44,0.445,0.45,0.455,
0.46,0.465,0.47,0.475,0.48,0.485,0.49,0.495,0.5,0.505,0.51,0.515,0.52,0.525,
0.53,0.535,0.54,0.545,0.55,0.555,0.56,0.565,0.57,0.575,0.58,0.585,0.59,
0.595,0.6,0.605,0.61,0.615,0.62,0.625,0.63,0.635,0.64,0.645,0.65,0.655,
0.66,0.665,0.67,0.675,0.68,0.685,0.690000000000001,0.695000000000001,0.700000000000001,
0.705000000000001,0.710000000000001,0.715000000000001,0.720000000000001,
0.725000000000001,0.730000000000001,0.735000000000001,0.740000000000001,
0.745000000000001,0.750000000000001,0.755000000000001,0.760000000000001,
0.765000000000001,0.770000000000001,0.775000000000001,0.780000000000001,
0.785000000000001,0.790000000000001,0.795000000000001,0.800000000000001,
0.805000000000001,0.810000000000001,0.815000000000001,0.820000000000001,
0.825000000000001,0.830000000000001,0.835000000000001,0.840000000000001,
0.845000000000001,0.850000000000001,0.855000000000001,0.860000000000001,
0.865000000000001,0.870000000000001,0.875000000000001,0.880000000000001,
0.885000000000001,0.890000000000001,0.895000000000001,0.900000000000001,
0.905000000000001,0.910000000000001,0.915000000000001,0.920000000000001,
0.925000000000001,0.930000000000001,0.935000000000001,0.940000000000001,
0.945000000000001,0.950000000000001,0.955000000000001,0.960000000000001,
0.965000000000001,0.970000000000001,0.975000000000001,0.980000000000001,
0.985000000000001,0.990000000000001,0.995000000000001,1.),(0.,1.2),
 .UNSPECIFIED.)
GEOMETRIC_REPRESENTATION_ITEM()
RATIONAL_B_SPLINE_SURFACE(((1.,1.),(1.,1.),(1.,1.),(1.,1.),(1.,1.),(1.,
1.),(1.,1.),(1.,1.),(1.,1.),(1.,1.),(1.,1.),(1.,1.),(1.,1.),(1.,1.),(1.,
1.),(1.,1.),(1.,1.),(1.,1.),(1.,1.),(1.,1.),(1.,1.),(1.,1.),(1.,1.),(1.,
1.),(1.,1.),(1.,1.),(1.,1.),(1.,1.),(1.,1.),(1.,1.),(1.,1.),(1.,1.),(1.,
1.),(1.,1.),(1.,1.),(1.,1.),(1.,1.),(1.,1.),(1.,1.),(1.,1.),(1.,1.),(1.,
1.),(1.,1.),(1.,1.),(1.,1.),(1.,1.),(1.,1.),(1.,1.),(1.,1.),(1.,1.),(1.,
1.),(1.,1.),(1.,1.),(1.,1.),(1.,1.),(1.,1.),(1.,1.),(1.,1.),(1.,1.),(1.,
1.),(1.,1.),(1.,1.),(1.,1.),(1.,1.),(1.,1.),(1.,1.),(1.,1.),(1.,1.),(1.,
1.),(1.,1.),(1.,1.),(1.,1.),(1.,1.),(1.,1.),(1.,1.),(1.,1.),(1.,1.),(1.,
1.),(1.,1.),(1.,1.),(1.,1.),(1.,1.),(1.,1.),(1.,1.),(1.,1.),(1.,1.),(1.,
1.),(1.,1.),(1.,1.),(1.,1.),(1.,1.),(1.,1.),(1.,1.),(1.,1.),(1.,1.),(1.,
1.),(1.,1.),(1.,1.),(1.,1.),(1.,1.),(1.,1.),(1.,1.),(1.,1.),(1.,1.),(1.,
1.),(1.,1.),(1.,1.),(1.,1.),(1.,1.),(1.,1.),(1.,1.),(1.,1.),(1.,1.),(1.,
1.),(1.,1.),(1.,1.),(1.,1.),(1.,1.),(1.,1.),(1.,1.),(1.,1.),(1.,1.),(1.,
1.),(1.,1.),(1.,1.),(1.,1.),(1.,1.),(1.,1.),(1.,1.),(1.,1.),(1.,1.),(1.,
1.),(1.,1.),(1.,1.),(1.,1.),(1.,1.),(1.,1.),(1.,1.),(1.,1.),(1.,1.),(1.,
1.),(1.,1.),(1.,1.),(1.,1.),(1.,1.),(1.,1.),(1.,1.),(1.,1.),(1.,1.),(1.,
1.),(1.,1.),(1.,1.),(1.,1.),(1.,1.),(1.,1.),(1.,1.),(1.,1.),(1.,1.),(1.,
1.),(1.,1.),(1.,1.),(1.,1.),(1.,1.),(1.,1.),(1.,1.),(1.,1.),(1.,1.),(1.,
1.),(1.,1.),(1.,1.),(1.,1.),(1.,1.),(1.,1.),(1.,1.),(1.,1.),(1.,1.),(1.,
1.),(1.,1.),(1.,1.),(1.,1.),(1.,1.),(1.,1.),(1.,1.),(1.,1.),(1.,1.),(1.,
1.),(1.,1.),(1.,1.),(1.,1.),(1.,1.),(1.,1.),(1.,1.),(1.,1.),(1.,1.),(1.,
1.),(1.,1.),(1.,1.),(1.,1.),(1.,1.),(1.,1.),(1.,1.),(1.,1.),(1.,1.),(1.,
1.),(1.,1.)))
REPRESENTATION_ITEM('')
SURFACE()
);
#948=(
BOUNDED_SURFACE()
B_SPLINE_SURFACE(5,1,((#110862,#110863),(#110864,#110865),(#110866,#110867),
(#110868,#110869),(#110870,#110871),(#110872,#110873),(#110874,#110875),
(#110876,#110877),(#110878,#110879),(#110880,#110881),(#110882,#110883),
(#110884,#110885),(#110886,#110887),(#110888,#110889),(#110890,#110891),
(#110892,#110893),(#110894,#110895),(#110896,#110897),(#110898,#110899),
(#110900,#110901),(#110902,#110903),(#110904,#110905),(#110906,#110907),
(#110908,#110909),(#110910,#110911),(#110912,#110913),(#110914,#110915),
(#110916,#110917),(#110918,#110919),(#110920,#110921),(#110922,#110923),
(#110924,#110925),(#110926,#110927),(#110928,#110929),(#110930,#110931),
(#110932,#110933),(#110934,#110935),(#110936,#110937),(#110938,#110939),
(#110940,#110941),(#110942,#110943),(#110944,#110945),(#110946,#110947),
(#110948,#110949),(#110950,#110951),(#110952,#110953),(#110954,#110955),
(#110956,#110957),(#110958,#110959),(#110960,#110961),(#110962,#110963),
(#110964,#110965),(#110966,#110967),(#110968,#110969),(#110970,#110971),
(#110972,#110973),(#110974,#110975),(#110976,#110977),(#110978,#110979),
(#110980,#110981),(#110982,#110983),(#110984,#110985),(#110986,#110987),
(#110988,#110989),(#110990,#110991),(#110992,#110993),(#110994,#110995),
(#110996,#110997),(#110998,#110999),(#111000,#111001),(#111002,#111003),
(#111004,#111005),(#111006,#111007),(#111008,#111009),(#111010,#111011),
(#111012,#111013),(#111014,#111015),(#111016,#111017),(#111018,#111019),
(#111020,#111021),(#111022,#111023),(#111024,#111025),(#111026,#111027),
(#111028,#111029),(#111030,#111031),(#111032,#111033),(#111034,#111035),
(#111036,#111037),(#111038,#111039),(#111040,#111041),(#111042,#111043),
(#111044,#111045),(#111046,#111047),(#111048,#111049),(#111050,#111051),
(#111052,#111053),(#111054,#111055),(#111056,#111057),(#111058,#111059),
(#111060,#111061),(#111062,#111063),(#111064,#111065),(#111066,#111067),
(#111068,#111069),(#111070,#111071),(#111072,#111073),(#111074,#111075),
(#111076,#111077),(#111078,#111079),(#111080,#111081),(#111082,#111083),
(#111084,#111085),(#111086,#111087),(#111088,#111089),(#111090,#111091),
(#111092,#111093),(#111094,#111095),(#111096,#111097),(#111098,#111099),
(#111100,#111101),(#111102,#111103),(#111104,#111105),(#111106,#111107),
(#111108,#111109),(#111110,#111111),(#111112,#111113),(#111114,#111115),
(#111116,#111117),(#111118,#111119),(#111120,#111121),(#111122,#111123),
(#111124,#111125),(#111126,#111127),(#111128,#111129),(#111130,#111131),
(#111132,#111133),(#111134,#111135),(#111136,#111137),(#111138,#111139),
(#111140,#111141),(#111142,#111143),(#111144,#111145),(#111146,#111147),
(#111148,#111149),(#111150,#111151),(#111152,#111153),(#111154,#111155),
(#111156,#111157),(#111158,#111159),(#111160,#111161),(#111162,#111163),
(#111164,#111165),(#111166,#111167),(#111168,#111169),(#111170,#111171),
(#111172,#111173),(#111174,#111175),(#111176,#111177),(#111178,#111179),
(#111180,#111181),(#111182,#111183),(#111184,#111185),(#111186,#111187),
(#111188,#111189),(#111190,#111191),(#111192,#111193),(#111194,#111195),
(#111196,#111197),(#111198,#111199),(#111200,#111201),(#111202,#111203),
(#111204,#111205),(#111206,#111207),(#111208,#111209),(#111210,#111211),
(#111212,#111213),(#111214,#111215),(#111216,#111217),(#111218,#111219),
(#111220,#111221),(#111222,#111223),(#111224,#111225),(#111226,#111227),
(#111228,#111229),(#111230,#111231),(#111232,#111233),(#111234,#111235),
(#111236,#111237),(#111238,#111239),(#111240,#111241),(#111242,#111243),
(#111244,#111245),(#111246,#111247),(#111248,#111249),(#111250,#111251),
(#111252,#111253),(#111254,#111255),(#111256,#111257),(#111258,#111259),
(#111260,#111261),(#111262,#111263),(#111264,#111265),(#111266,#111267),
(#111268,#111269),(#111270,#111271)),.UNSPECIFIED.,.F.,.F.,.F.)
B_SPLINE_SURFACE_WITH_KNOTS((6,1,1,1,1,1,1,1,1,1,1,1,1,1,1,1,1,1,1,1,1,
1,1,1,1,1,1,1,1,1,1,1,1,1,1,1,1,1,1,1,1,1,1,1,1,1,1,1,1,1,1,1,1,1,1,1,1,
1,1,1,1,1,1,1,1,1,1,1,1,1,1,1,1,1,1,1,1,1,1,1,1,1,1,1,1,1,1,1,1,1,1,1,1,
1,1,1,1,1,1,1,1,1,1,1,1,1,1,1,1,1,1,1,1,1,1,1,1,1,1,1,1,1,1,1,1,1,1,1,1,
1,1,1,1,1,1,1,1,1,1,1,1,1,1,1,1,1,1,1,1,1,1,1,1,1,1,1,1,1,1,1,1,1,1,1,1,
1,1,1,1,1,1,1,1,1,1,1,1,1,1,1,1,1,1,1,1,1,1,1,1,1,1,1,1,1,1,1,1,1,1,1,6),
(2,2),(0.,0.005,0.01,0.015,0.02,0.025,0.03,0.035,0.04,0.045,0.05,0.055,
0.06,0.065,0.07,0.075,0.08,0.085,0.09,0.095,0.1,0.105,0.11,0.115,0.12,0.125,
0.13,0.135,0.14,0.145,0.15,0.155,0.16,0.165,0.17,0.175,0.18,0.185,0.19,
0.195,0.2,0.205,0.21,0.215,0.22,0.225,0.23,0.235,0.24,0.245,0.25,0.255,
0.26,0.265,0.27,0.275,0.28,0.285,0.29,0.295,0.3,0.305,0.31,0.315,0.32,0.325,
0.33,0.335,0.34,0.345,0.35,0.355,0.36,0.365,0.37,0.375,0.38,0.385,0.39,
0.395,0.4,0.405,0.41,0.415,0.42,0.425,0.43,0.435,0.44,0.445,0.45,0.455,
0.46,0.465,0.47,0.475,0.48,0.485,0.49,0.495,0.5,0.505,0.51,0.515,0.52,0.525,
0.53,0.535,0.54,0.545,0.55,0.555,0.56,0.565,0.57,0.575,0.58,0.585,0.59,
0.595,0.6,0.605,0.61,0.615,0.62,0.625,0.63,0.635,0.64,0.645,0.65,0.655,
0.66,0.665,0.67,0.675,0.68,0.685,0.690000000000001,0.695000000000001,0.700000000000001,
0.705000000000001,0.710000000000001,0.715000000000001,0.720000000000001,
0.725000000000001,0.730000000000001,0.735000000000001,0.740000000000001,
0.745000000000001,0.750000000000001,0.755000000000001,0.760000000000001,
0.765000000000001,0.770000000000001,0.775000000000001,0.780000000000001,
0.785000000000001,0.790000000000001,0.795000000000001,0.800000000000001,
0.805000000000001,0.810000000000001,0.815000000000001,0.820000000000001,
0.825000000000001,0.830000000000001,0.835000000000001,0.840000000000001,
0.845000000000001,0.850000000000001,0.855000000000001,0.860000000000001,
0.865000000000001,0.870000000000001,0.875000000000001,0.880000000000001,
0.885000000000001,0.890000000000001,0.895000000000001,0.900000000000001,
0.905000000000001,0.910000000000001,0.915000000000001,0.920000000000001,
0.925000000000001,0.930000000000001,0.935000000000001,0.940000000000001,
0.945000000000001,0.950000000000001,0.955000000000001,0.960000000000001,
0.965000000000001,0.970000000000001,0.975000000000001,0.980000000000001,
0.985000000000001,0.990000000000001,0.995000000000001,1.),(0.,1.2),
 .UNSPECIFIED.)
GEOMETRIC_REPRESENTATION_ITEM()
RATIONAL_B_SPLINE_SURFACE(((1.,1.),(1.,1.),(1.,1.),(1.,1.),(1.,1.),(1.,
1.),(1.,1.),(1.,1.),(1.,1.),(1.,1.),(1.,1.),(1.,1.),(1.,1.),(1.,1.),(1.,
1.),(1.,1.),(1.,1.),(1.,1.),(1.,1.),(1.,1.),(1.,1.),(1.,1.),(1.,1.),(1.,
1.),(1.,1.),(1.,1.),(1.,1.),(1.,1.),(1.,1.),(1.,1.),(1.,1.),(1.,1.),(1.,
1.),(1.,1.),(1.,1.),(1.,1.),(1.,1.),(1.,1.),(1.,1.),(1.,1.),(1.,1.),(1.,
1.),(1.,1.),(1.,1.),(1.,1.),(1.,1.),(1.,1.),(1.,1.),(1.,1.),(1.,1.),(1.,
1.),(1.,1.),(1.,1.),(1.,1.),(1.,1.),(1.,1.),(1.,1.),(1.,1.),(1.,1.),(1.,
1.),(1.,1.),(1.,1.),(1.,1.),(1.,1.),(1.,1.),(1.,1.),(1.,1.),(1.,1.),(1.,
1.),(1.,1.),(1.,1.),(1.,1.),(1.,1.),(1.,1.),(1.,1.),(1.,1.),(1.,1.),(1.,
1.),(1.,1.),(1.,1.),(1.,1.),(1.,1.),(1.,1.),(1.,1.),(1.,1.),(1.,1.),(1.,
1.),(1.,1.),(1.,1.),(1.,1.),(1.,1.),(1.,1.),(1.,1.),(1.,1.),(1.,1.),(1.,
1.),(1.,1.),(1.,1.),(1.,1.),(1.,1.),(1.,1.),(1.,1.),(1.,1.),(1.,1.),(1.,
1.),(1.,1.),(1.,1.),(1.,1.),(1.,1.),(1.,1.),(1.,1.),(1.,1.),(1.,1.),(1.,
1.),(1.,1.),(1.,1.),(1.,1.),(1.,1.),(1.,1.),(1.,1.),(1.,1.),(1.,1.),(1.,
1.),(1.,1.),(1.,1.),(1.,1.),(1.,1.),(1.,1.),(1.,1.),(1.,1.),(1.,1.),(1.,
1.),(1.,1.),(1.,1.),(1.,1.),(1.,1.),(1.,1.),(1.,1.),(1.,1.),(1.,1.),(1.,
1.),(1.,1.),(1.,1.),(1.,1.),(1.,1.),(1.,1.),(1.,1.),(1.,1.),(1.,1.),(1.,
1.),(1.,1.),(1.,1.),(1.,1.),(1.,1.),(1.,1.),(1.,1.),(1.,1.),(1.,1.),(1.,
1.),(1.,1.),(1.,1.),(1.,1.),(1.,1.),(1.,1.),(1.,1.),(1.,1.),(1.,1.),(1.,
1.),(1.,1.),(1.,1.),(1.,1.),(1.,1.),(1.,1.),(1.,1.),(1.,1.),(1.,1.),(1.,
1.),(1.,1.),(1.,1.),(1.,1.),(1.,1.),(1.,1.),(1.,1.),(1.,1.),(1.,1.),(1.,
1.),(1.,1.),(1.,1.),(1.,1.),(1.,1.),(1.,1.),(1.,1.),(1.,1.),(1.,1.),(1.,
1.),(1.,1.),(1.,1.),(1.,1.),(1.,1.),(1.,1.),(1.,1.),(1.,1.),(1.,1.),(1.,
1.),(1.,1.)))
REPRESENTATION_ITEM('')
SURFACE()
);
#949=(
BOUNDED_SURFACE()
B_SPLINE_SURFACE(5,1,((#111758,#111759),(#111760,#111761),(#111762,#111763),
(#111764,#111765),(#111766,#111767),(#111768,#111769),(#111770,#111771),
(#111772,#111773),(#111774,#111775),(#111776,#111777),(#111778,#111779),
(#111780,#111781),(#111782,#111783),(#111784,#111785),(#111786,#111787),
(#111788,#111789),(#111790,#111791),(#111792,#111793),(#111794,#111795),
(#111796,#111797),(#111798,#111799),(#111800,#111801),(#111802,#111803),
(#111804,#111805),(#111806,#111807),(#111808,#111809),(#111810,#111811),
(#111812,#111813),(#111814,#111815),(#111816,#111817),(#111818,#111819),
(#111820,#111821),(#111822,#111823),(#111824,#111825),(#111826,#111827),
(#111828,#111829),(#111830,#111831),(#111832,#111833),(#111834,#111835),
(#111836,#111837),(#111838,#111839),(#111840,#111841),(#111842,#111843),
(#111844,#111845),(#111846,#111847),(#111848,#111849),(#111850,#111851),
(#111852,#111853),(#111854,#111855),(#111856,#111857),(#111858,#111859),
(#111860,#111861),(#111862,#111863),(#111864,#111865),(#111866,#111867),
(#111868,#111869),(#111870,#111871),(#111872,#111873),(#111874,#111875),
(#111876,#111877),(#111878,#111879),(#111880,#111881),(#111882,#111883),
(#111884,#111885),(#111886,#111887),(#111888,#111889),(#111890,#111891),
(#111892,#111893),(#111894,#111895),(#111896,#111897),(#111898,#111899),
(#111900,#111901),(#111902,#111903),(#111904,#111905),(#111906,#111907),
(#111908,#111909),(#111910,#111911),(#111912,#111913),(#111914,#111915),
(#111916,#111917),(#111918,#111919),(#111920,#111921),(#111922,#111923),
(#111924,#111925),(#111926,#111927),(#111928,#111929),(#111930,#111931),
(#111932,#111933),(#111934,#111935),(#111936,#111937),(#111938,#111939),
(#111940,#111941),(#111942,#111943),(#111944,#111945),(#111946,#111947),
(#111948,#111949),(#111950,#111951),(#111952,#111953),(#111954,#111955),
(#111956,#111957),(#111958,#111959),(#111960,#111961),(#111962,#111963),
(#111964,#111965),(#111966,#111967),(#111968,#111969),(#111970,#111971),
(#111972,#111973),(#111974,#111975),(#111976,#111977),(#111978,#111979),
(#111980,#111981),(#111982,#111983),(#111984,#111985),(#111986,#111987),
(#111988,#111989),(#111990,#111991),(#111992,#111993),(#111994,#111995),
(#111996,#111997),(#111998,#111999),(#112000,#112001),(#112002,#112003),
(#112004,#112005),(#112006,#112007),(#112008,#112009),(#112010,#112011),
(#112012,#112013),(#112014,#112015),(#112016,#112017),(#112018,#112019),
(#112020,#112021),(#112022,#112023),(#112024,#112025),(#112026,#112027),
(#112028,#112029),(#112030,#112031),(#112032,#112033),(#112034,#112035),
(#112036,#112037),(#112038,#112039),(#112040,#112041),(#112042,#112043),
(#112044,#112045),(#112046,#112047),(#112048,#112049),(#112050,#112051),
(#112052,#112053),(#112054,#112055),(#112056,#112057),(#112058,#112059),
(#112060,#112061),(#112062,#112063),(#112064,#112065),(#112066,#112067),
(#112068,#112069),(#112070,#112071),(#112072,#112073),(#112074,#112075),
(#112076,#112077),(#112078,#112079),(#112080,#112081),(#112082,#112083),
(#112084,#112085),(#112086,#112087),(#112088,#112089),(#112090,#112091),
(#112092,#112093),(#112094,#112095),(#112096,#112097),(#112098,#112099),
(#112100,#112101),(#112102,#112103),(#112104,#112105),(#112106,#112107),
(#112108,#112109),(#112110,#112111),(#112112,#112113),(#112114,#112115),
(#112116,#112117),(#112118,#112119),(#112120,#112121),(#112122,#112123),
(#112124,#112125),(#112126,#112127),(#112128,#112129),(#112130,#112131),
(#112132,#112133),(#112134,#112135),(#112136,#112137),(#112138,#112139),
(#112140,#112141),(#112142,#112143),(#112144,#112145),(#112146,#112147),
(#112148,#112149),(#112150,#112151),(#112152,#112153),(#112154,#112155),
(#112156,#112157),(#112158,#112159),(#112160,#112161),(#112162,#112163),
(#112164,#112165),(#112166,#112167)),.UNSPECIFIED.,.F.,.F.,.F.)
B_SPLINE_SURFACE_WITH_KNOTS((6,1,1,1,1,1,1,1,1,1,1,1,1,1,1,1,1,1,1,1,1,
1,1,1,1,1,1,1,1,1,1,1,1,1,1,1,1,1,1,1,1,1,1,1,1,1,1,1,1,1,1,1,1,1,1,1,1,
1,1,1,1,1,1,1,1,1,1,1,1,1,1,1,1,1,1,1,1,1,1,1,1,1,1,1,1,1,1,1,1,1,1,1,1,
1,1,1,1,1,1,1,1,1,1,1,1,1,1,1,1,1,1,1,1,1,1,1,1,1,1,1,1,1,1,1,1,1,1,1,1,
1,1,1,1,1,1,1,1,1,1,1,1,1,1,1,1,1,1,1,1,1,1,1,1,1,1,1,1,1,1,1,1,1,1,1,1,
1,1,1,1,1,1,1,1,1,1,1,1,1,1,1,1,1,1,1,1,1,1,1,1,1,1,1,1,1,1,1,1,1,1,1,6),
(2,2),(0.,0.005,0.01,0.015,0.02,0.025,0.03,0.035,0.04,0.045,0.05,0.055,
0.06,0.065,0.07,0.075,0.08,0.085,0.09,0.095,0.1,0.105,0.11,0.115,0.12,0.125,
0.13,0.135,0.14,0.145,0.15,0.155,0.16,0.165,0.17,0.175,0.18,0.185,0.19,
0.195,0.2,0.205,0.21,0.215,0.22,0.225,0.23,0.235,0.24,0.245,0.25,0.255,
0.26,0.265,0.27,0.275,0.28,0.285,0.29,0.295,0.3,0.305,0.31,0.315,0.32,0.325,
0.33,0.335,0.34,0.345,0.35,0.355,0.36,0.365,0.37,0.375,0.38,0.385,0.39,
0.395,0.4,0.405,0.41,0.415,0.42,0.425,0.43,0.435,0.44,0.445,0.45,0.455,
0.46,0.465,0.47,0.475,0.48,0.485,0.49,0.495,0.5,0.505,0.51,0.515,0.52,0.525,
0.53,0.535,0.54,0.545,0.55,0.555,0.56,0.565,0.57,0.575,0.58,0.585,0.59,
0.595,0.6,0.605,0.61,0.615,0.62,0.625,0.63,0.635,0.64,0.645,0.65,0.655,
0.66,0.665,0.67,0.675,0.68,0.685,0.690000000000001,0.695000000000001,0.700000000000001,
0.705000000000001,0.710000000000001,0.715000000000001,0.720000000000001,
0.725000000000001,0.730000000000001,0.735000000000001,0.740000000000001,
0.745000000000001,0.750000000000001,0.755000000000001,0.760000000000001,
0.765000000000001,0.770000000000001,0.775000000000001,0.780000000000001,
0.785000000000001,0.790000000000001,0.795000000000001,0.800000000000001,
0.805000000000001,0.810000000000001,0.815000000000001,0.820000000000001,
0.825000000000001,0.830000000000001,0.835000000000001,0.840000000000001,
0.845000000000001,0.850000000000001,0.855000000000001,0.860000000000001,
0.865000000000001,0.870000000000001,0.875000000000001,0.880000000000001,
0.885000000000001,0.890000000000001,0.895000000000001,0.900000000000001,
0.905000000000001,0.910000000000001,0.915000000000001,0.920000000000001,
0.925000000000001,0.930000000000001,0.935000000000001,0.940000000000001,
0.945000000000001,0.950000000000001,0.955000000000001,0.960000000000001,
0.965000000000001,0.970000000000001,0.975000000000001,0.980000000000001,
0.985000000000001,0.990000000000001,0.995000000000001,1.),(0.,1.2),
 .UNSPECIFIED.)
GEOMETRIC_REPRESENTATION_ITEM()
RATIONAL_B_SPLINE_SURFACE(((1.,1.),(1.,1.),(1.,1.),(1.,1.),(1.,1.),(1.,
1.),(1.,1.),(1.,1.),(1.,1.),(1.,1.),(1.,1.),(1.,1.),(1.,1.),(1.,1.),(1.,
1.),(1.,1.),(1.,1.),(1.,1.),(1.,1.),(1.,1.),(1.,1.),(1.,1.),(1.,1.),(1.,
1.),(1.,1.),(1.,1.),(1.,1.),(1.,1.),(1.,1.),(1.,1.),(1.,1.),(1.,1.),(1.,
1.),(1.,1.),(1.,1.),(1.,1.),(1.,1.),(1.,1.),(1.,1.),(1.,1.),(1.,1.),(1.,
1.),(1.,1.),(1.,1.),(1.,1.),(1.,1.),(1.,1.),(1.,1.),(1.,1.),(1.,1.),(1.,
1.),(1.,1.),(1.,1.),(1.,1.),(1.,1.),(1.,1.),(1.,1.),(1.,1.),(1.,1.),(1.,
1.),(1.,1.),(1.,1.),(1.,1.),(1.,1.),(1.,1.),(1.,1.),(1.,1.),(1.,1.),(1.,
1.),(1.,1.),(1.,1.),(1.,1.),(1.,1.),(1.,1.),(1.,1.),(1.,1.),(1.,1.),(1.,
1.),(1.,1.),(1.,1.),(1.,1.),(1.,1.),(1.,1.),(1.,1.),(1.,1.),(1.,1.),(1.,
1.),(1.,1.),(1.,1.),(1.,1.),(1.,1.),(1.,1.),(1.,1.),(1.,1.),(1.,1.),(1.,
1.),(1.,1.),(1.,1.),(1.,1.),(1.,1.),(1.,1.),(1.,1.),(1.,1.),(1.,1.),(1.,
1.),(1.,1.),(1.,1.),(1.,1.),(1.,1.),(1.,1.),(1.,1.),(1.,1.),(1.,1.),(1.,
1.),(1.,1.),(1.,1.),(1.,1.),(1.,1.),(1.,1.),(1.,1.),(1.,1.),(1.,1.),(1.,
1.),(1.,1.),(1.,1.),(1.,1.),(1.,1.),(1.,1.),(1.,1.),(1.,1.),(1.,1.),(1.,
1.),(1.,1.),(1.,1.),(1.,1.),(1.,1.),(1.,1.),(1.,1.),(1.,1.),(1.,1.),(1.,
1.),(1.,1.),(1.,1.),(1.,1.),(1.,1.),(1.,1.),(1.,1.),(1.,1.),(1.,1.),(1.,
1.),(1.,1.),(1.,1.),(1.,1.),(1.,1.),(1.,1.),(1.,1.),(1.,1.),(1.,1.),(1.,
1.),(1.,1.),(1.,1.),(1.,1.),(1.,1.),(1.,1.),(1.,1.),(1.,1.),(1.,1.),(1.,
1.),(1.,1.),(1.,1.),(1.,1.),(1.,1.),(1.,1.),(1.,1.),(1.,1.),(1.,1.),(1.,
1.),(1.,1.),(1.,1.),(1.,1.),(1.,1.),(1.,1.),(1.,1.),(1.,1.),(1.,1.),(1.,
1.),(1.,1.),(1.,1.),(1.,1.),(1.,1.),(1.,1.),(1.,1.),(1.,1.),(1.,1.),(1.,
1.),(1.,1.),(1.,1.),(1.,1.),(1.,1.),(1.,1.),(1.,1.),(1.,1.),(1.,1.),(1.,
1.),(1.,1.)))
REPRESENTATION_ITEM('')
SURFACE()
);
#950=(
BOUNDED_SURFACE()
B_SPLINE_SURFACE(5,1,((#112654,#112655),(#112656,#112657),(#112658,#112659),
(#112660,#112661),(#112662,#112663),(#112664,#112665),(#112666,#112667),
(#112668,#112669),(#112670,#112671),(#112672,#112673),(#112674,#112675),
(#112676,#112677),(#112678,#112679),(#112680,#112681),(#112682,#112683),
(#112684,#112685),(#112686,#112687),(#112688,#112689),(#112690,#112691),
(#112692,#112693),(#112694,#112695),(#112696,#112697),(#112698,#112699),
(#112700,#112701),(#112702,#112703),(#112704,#112705),(#112706,#112707),
(#112708,#112709),(#112710,#112711),(#112712,#112713),(#112714,#112715),
(#112716,#112717),(#112718,#112719),(#112720,#112721),(#112722,#112723),
(#112724,#112725),(#112726,#112727),(#112728,#112729),(#112730,#112731),
(#112732,#112733),(#112734,#112735),(#112736,#112737),(#112738,#112739),
(#112740,#112741),(#112742,#112743),(#112744,#112745),(#112746,#112747),
(#112748,#112749),(#112750,#112751),(#112752,#112753),(#112754,#112755),
(#112756,#112757),(#112758,#112759),(#112760,#112761),(#112762,#112763),
(#112764,#112765),(#112766,#112767),(#112768,#112769),(#112770,#112771),
(#112772,#112773),(#112774,#112775),(#112776,#112777),(#112778,#112779),
(#112780,#112781),(#112782,#112783),(#112784,#112785),(#112786,#112787),
(#112788,#112789),(#112790,#112791),(#112792,#112793),(#112794,#112795),
(#112796,#112797),(#112798,#112799),(#112800,#112801),(#112802,#112803),
(#112804,#112805),(#112806,#112807),(#112808,#112809),(#112810,#112811),
(#112812,#112813),(#112814,#112815),(#112816,#112817),(#112818,#112819),
(#112820,#112821),(#112822,#112823),(#112824,#112825),(#112826,#112827),
(#112828,#112829),(#112830,#112831),(#112832,#112833),(#112834,#112835),
(#112836,#112837),(#112838,#112839),(#112840,#112841),(#112842,#112843),
(#112844,#112845),(#112846,#112847),(#112848,#112849),(#112850,#112851),
(#112852,#112853),(#112854,#112855),(#112856,#112857),(#112858,#112859),
(#112860,#112861),(#112862,#112863),(#112864,#112865),(#112866,#112867),
(#112868,#112869),(#112870,#112871),(#112872,#112873),(#112874,#112875),
(#112876,#112877),(#112878,#112879),(#112880,#112881),(#112882,#112883),
(#112884,#112885),(#112886,#112887),(#112888,#112889),(#112890,#112891),
(#112892,#112893),(#112894,#112895),(#112896,#112897),(#112898,#112899),
(#112900,#112901),(#112902,#112903),(#112904,#112905),(#112906,#112907),
(#112908,#112909),(#112910,#112911),(#112912,#112913),(#112914,#112915),
(#112916,#112917),(#112918,#112919),(#112920,#112921),(#112922,#112923),
(#112924,#112925),(#112926,#112927),(#112928,#112929),(#112930,#112931),
(#112932,#112933),(#112934,#112935),(#112936,#112937),(#112938,#112939),
(#112940,#112941),(#112942,#112943),(#112944,#112945),(#112946,#112947),
(#112948,#112949),(#112950,#112951),(#112952,#112953),(#112954,#112955),
(#112956,#112957),(#112958,#112959),(#112960,#112961),(#112962,#112963),
(#112964,#112965),(#112966,#112967),(#112968,#112969),(#112970,#112971),
(#112972,#112973),(#112974,#112975),(#112976,#112977),(#112978,#112979),
(#112980,#112981),(#112982,#112983),(#112984,#112985),(#112986,#112987),
(#112988,#112989),(#112990,#112991),(#112992,#112993),(#112994,#112995),
(#112996,#112997),(#112998,#112999),(#113000,#113001),(#113002,#113003),
(#113004,#113005),(#113006,#113007),(#113008,#113009),(#113010,#113011),
(#113012,#113013),(#113014,#113015),(#113016,#113017),(#113018,#113019),
(#113020,#113021),(#113022,#113023),(#113024,#113025),(#113026,#113027),
(#113028,#113029),(#113030,#113031),(#113032,#113033),(#113034,#113035),
(#113036,#113037),(#113038,#113039),(#113040,#113041),(#113042,#113043),
(#113044,#113045),(#113046,#113047),(#113048,#113049),(#113050,#113051),
(#113052,#113053),(#113054,#113055),(#113056,#113057),(#113058,#113059),
(#113060,#113061),(#113062,#113063)),.UNSPECIFIED.,.F.,.F.,.F.)
B_SPLINE_SURFACE_WITH_KNOTS((6,1,1,1,1,1,1,1,1,1,1,1,1,1,1,1,1,1,1,1,1,
1,1,1,1,1,1,1,1,1,1,1,1,1,1,1,1,1,1,1,1,1,1,1,1,1,1,1,1,1,1,1,1,1,1,1,1,
1,1,1,1,1,1,1,1,1,1,1,1,1,1,1,1,1,1,1,1,1,1,1,1,1,1,1,1,1,1,1,1,1,1,1,1,
1,1,1,1,1,1,1,1,1,1,1,1,1,1,1,1,1,1,1,1,1,1,1,1,1,1,1,1,1,1,1,1,1,1,1,1,
1,1,1,1,1,1,1,1,1,1,1,1,1,1,1,1,1,1,1,1,1,1,1,1,1,1,1,1,1,1,1,1,1,1,1,1,
1,1,1,1,1,1,1,1,1,1,1,1,1,1,1,1,1,1,1,1,1,1,1,1,1,1,1,1,1,1,1,1,1,1,1,6),
(2,2),(0.,0.005,0.01,0.015,0.02,0.025,0.03,0.035,0.04,0.045,0.05,0.055,
0.06,0.065,0.07,0.075,0.08,0.085,0.09,0.095,0.1,0.105,0.11,0.115,0.12,0.125,
0.13,0.135,0.14,0.145,0.15,0.155,0.16,0.165,0.17,0.175,0.18,0.185,0.19,
0.195,0.2,0.205,0.21,0.215,0.22,0.225,0.23,0.235,0.24,0.245,0.25,0.255,
0.26,0.265,0.27,0.275,0.28,0.285,0.29,0.295,0.3,0.305,0.31,0.315,0.32,0.325,
0.33,0.335,0.34,0.345,0.35,0.355,0.36,0.365,0.37,0.375,0.38,0.385,0.39,
0.395,0.4,0.405,0.41,0.415,0.42,0.425,0.43,0.435,0.44,0.445,0.45,0.455,
0.46,0.465,0.47,0.475,0.48,0.485,0.49,0.495,0.5,0.505,0.51,0.515,0.52,0.525,
0.53,0.535,0.54,0.545,0.55,0.555,0.56,0.565,0.57,0.575,0.58,0.585,0.59,
0.595,0.6,0.605,0.61,0.615,0.62,0.625,0.63,0.635,0.64,0.645,0.65,0.655,
0.66,0.665,0.67,0.675,0.68,0.685,0.690000000000001,0.695000000000001,0.700000000000001,
0.705000000000001,0.710000000000001,0.715000000000001,0.720000000000001,
0.725000000000001,0.730000000000001,0.735000000000001,0.740000000000001,
0.745000000000001,0.750000000000001,0.755000000000001,0.760000000000001,
0.765000000000001,0.770000000000001,0.775000000000001,0.780000000000001,
0.785000000000001,0.790000000000001,0.795000000000001,0.800000000000001,
0.805000000000001,0.810000000000001,0.815000000000001,0.820000000000001,
0.825000000000001,0.830000000000001,0.835000000000001,0.840000000000001,
0.845000000000001,0.850000000000001,0.855000000000001,0.860000000000001,
0.865000000000001,0.870000000000001,0.875000000000001,0.880000000000001,
0.885000000000001,0.890000000000001,0.895000000000001,0.900000000000001,
0.905000000000001,0.910000000000001,0.915000000000001,0.920000000000001,
0.925000000000001,0.930000000000001,0.935000000000001,0.940000000000001,
0.945000000000001,0.950000000000001,0.955000000000001,0.960000000000001,
0.965000000000001,0.970000000000001,0.975000000000001,0.980000000000001,
0.985000000000001,0.990000000000001,0.995000000000001,1.),(0.,1.2),
 .UNSPECIFIED.)
GEOMETRIC_REPRESENTATION_ITEM()
RATIONAL_B_SPLINE_SURFACE(((1.,1.),(1.,1.),(1.,1.),(1.,1.),(1.,1.),(1.,
1.),(1.,1.),(1.,1.),(1.,1.),(1.,1.),(1.,1.),(1.,1.),(1.,1.),(1.,1.),(1.,
1.),(1.,1.),(1.,1.),(1.,1.),(1.,1.),(1.,1.),(1.,1.),(1.,1.),(1.,1.),(1.,
1.),(1.,1.),(1.,1.),(1.,1.),(1.,1.),(1.,1.),(1.,1.),(1.,1.),(1.,1.),(1.,
1.),(1.,1.),(1.,1.),(1.,1.),(1.,1.),(1.,1.),(1.,1.),(1.,1.),(1.,1.),(1.,
1.),(1.,1.),(1.,1.),(1.,1.),(1.,1.),(1.,1.),(1.,1.),(1.,1.),(1.,1.),(1.,
1.),(1.,1.),(1.,1.),(1.,1.),(1.,1.),(1.,1.),(1.,1.),(1.,1.),(1.,1.),(1.,
1.),(1.,1.),(1.,1.),(1.,1.),(1.,1.),(1.,1.),(1.,1.),(1.,1.),(1.,1.),(1.,
1.),(1.,1.),(1.,1.),(1.,1.),(1.,1.),(1.,1.),(1.,1.),(1.,1.),(1.,1.),(1.,
1.),(1.,1.),(1.,1.),(1.,1.),(1.,1.),(1.,1.),(1.,1.),(1.,1.),(1.,1.),(1.,
1.),(1.,1.),(1.,1.),(1.,1.),(1.,1.),(1.,1.),(1.,1.),(1.,1.),(1.,1.),(1.,
1.),(1.,1.),(1.,1.),(1.,1.),(1.,1.),(1.,1.),(1.,1.),(1.,1.),(1.,1.),(1.,
1.),(1.,1.),(1.,1.),(1.,1.),(1.,1.),(1.,1.),(1.,1.),(1.,1.),(1.,1.),(1.,
1.),(1.,1.),(1.,1.),(1.,1.),(1.,1.),(1.,1.),(1.,1.),(1.,1.),(1.,1.),(1.,
1.),(1.,1.),(1.,1.),(1.,1.),(1.,1.),(1.,1.),(1.,1.),(1.,1.),(1.,1.),(1.,
1.),(1.,1.),(1.,1.),(1.,1.),(1.,1.),(1.,1.),(1.,1.),(1.,1.),(1.,1.),(1.,
1.),(1.,1.),(1.,1.),(1.,1.),(1.,1.),(1.,1.),(1.,1.),(1.,1.),(1.,1.),(1.,
1.),(1.,1.),(1.,1.),(1.,1.),(1.,1.),(1.,1.),(1.,1.),(1.,1.),(1.,1.),(1.,
1.),(1.,1.),(1.,1.),(1.,1.),(1.,1.),(1.,1.),(1.,1.),(1.,1.),(1.,1.),(1.,
1.),(1.,1.),(1.,1.),(1.,1.),(1.,1.),(1.,1.),(1.,1.),(1.,1.),(1.,1.),(1.,
1.),(1.,1.),(1.,1.),(1.,1.),(1.,1.),(1.,1.),(1.,1.),(1.,1.),(1.,1.),(1.,
1.),(1.,1.),(1.,1.),(1.,1.),(1.,1.),(1.,1.),(1.,1.),(1.,1.),(1.,1.),(1.,
1.),(1.,1.),(1.,1.),(1.,1.),(1.,1.),(1.,1.),(1.,1.),(1.,1.),(1.,1.),(1.,
1.),(1.,1.)))
REPRESENTATION_ITEM('')
SURFACE()
);
#951=(
BOUNDED_SURFACE()
B_SPLINE_SURFACE(5,1,((#113550,#113551),(#113552,#113553),(#113554,#113555),
(#113556,#113557),(#113558,#113559),(#113560,#113561),(#113562,#113563),
(#113564,#113565),(#113566,#113567),(#113568,#113569),(#113570,#113571),
(#113572,#113573),(#113574,#113575),(#113576,#113577),(#113578,#113579),
(#113580,#113581),(#113582,#113583),(#113584,#113585),(#113586,#113587),
(#113588,#113589),(#113590,#113591),(#113592,#113593),(#113594,#113595),
(#113596,#113597),(#113598,#113599),(#113600,#113601),(#113602,#113603),
(#113604,#113605),(#113606,#113607),(#113608,#113609),(#113610,#113611),
(#113612,#113613),(#113614,#113615),(#113616,#113617),(#113618,#113619),
(#113620,#113621),(#113622,#113623),(#113624,#113625),(#113626,#113627),
(#113628,#113629),(#113630,#113631),(#113632,#113633),(#113634,#113635),
(#113636,#113637),(#113638,#113639),(#113640,#113641),(#113642,#113643),
(#113644,#113645),(#113646,#113647),(#113648,#113649),(#113650,#113651),
(#113652,#113653),(#113654,#113655),(#113656,#113657),(#113658,#113659),
(#113660,#113661),(#113662,#113663),(#113664,#113665),(#113666,#113667),
(#113668,#113669),(#113670,#113671),(#113672,#113673),(#113674,#113675),
(#113676,#113677),(#113678,#113679),(#113680,#113681),(#113682,#113683),
(#113684,#113685),(#113686,#113687),(#113688,#113689),(#113690,#113691),
(#113692,#113693),(#113694,#113695),(#113696,#113697),(#113698,#113699),
(#113700,#113701),(#113702,#113703),(#113704,#113705),(#113706,#113707),
(#113708,#113709),(#113710,#113711),(#113712,#113713),(#113714,#113715),
(#113716,#113717),(#113718,#113719),(#113720,#113721),(#113722,#113723),
(#113724,#113725),(#113726,#113727),(#113728,#113729),(#113730,#113731),
(#113732,#113733),(#113734,#113735),(#113736,#113737),(#113738,#113739),
(#113740,#113741),(#113742,#113743),(#113744,#113745),(#113746,#113747),
(#113748,#113749),(#113750,#113751),(#113752,#113753),(#113754,#113755),
(#113756,#113757),(#113758,#113759),(#113760,#113761),(#113762,#113763),
(#113764,#113765),(#113766,#113767),(#113768,#113769),(#113770,#113771),
(#113772,#113773),(#113774,#113775),(#113776,#113777),(#113778,#113779),
(#113780,#113781),(#113782,#113783),(#113784,#113785),(#113786,#113787),
(#113788,#113789),(#113790,#113791),(#113792,#113793),(#113794,#113795),
(#113796,#113797),(#113798,#113799),(#113800,#113801),(#113802,#113803),
(#113804,#113805),(#113806,#113807),(#113808,#113809),(#113810,#113811),
(#113812,#113813),(#113814,#113815),(#113816,#113817),(#113818,#113819),
(#113820,#113821),(#113822,#113823),(#113824,#113825),(#113826,#113827),
(#113828,#113829),(#113830,#113831),(#113832,#113833),(#113834,#113835),
(#113836,#113837),(#113838,#113839),(#113840,#113841),(#113842,#113843),
(#113844,#113845),(#113846,#113847),(#113848,#113849),(#113850,#113851),
(#113852,#113853),(#113854,#113855),(#113856,#113857),(#113858,#113859),
(#113860,#113861),(#113862,#113863),(#113864,#113865),(#113866,#113867),
(#113868,#113869),(#113870,#113871),(#113872,#113873),(#113874,#113875),
(#113876,#113877),(#113878,#113879),(#113880,#113881),(#113882,#113883),
(#113884,#113885),(#113886,#113887),(#113888,#113889),(#113890,#113891),
(#113892,#113893),(#113894,#113895),(#113896,#113897),(#113898,#113899),
(#113900,#113901),(#113902,#113903),(#113904,#113905),(#113906,#113907),
(#113908,#113909),(#113910,#113911),(#113912,#113913),(#113914,#113915),
(#113916,#113917),(#113918,#113919),(#113920,#113921),(#113922,#113923),
(#113924,#113925),(#113926,#113927),(#113928,#113929),(#113930,#113931),
(#113932,#113933),(#113934,#113935),(#113936,#113937),(#113938,#113939),
(#113940,#113941),(#113942,#113943),(#113944,#113945),(#113946,#113947),
(#113948,#113949),(#113950,#113951),(#113952,#113953),(#113954,#113955),
(#113956,#113957),(#113958,#113959)),.UNSPECIFIED.,.F.,.F.,.F.)
B_SPLINE_SURFACE_WITH_KNOTS((6,1,1,1,1,1,1,1,1,1,1,1,1,1,1,1,1,1,1,1,1,
1,1,1,1,1,1,1,1,1,1,1,1,1,1,1,1,1,1,1,1,1,1,1,1,1,1,1,1,1,1,1,1,1,1,1,1,
1,1,1,1,1,1,1,1,1,1,1,1,1,1,1,1,1,1,1,1,1,1,1,1,1,1,1,1,1,1,1,1,1,1,1,1,
1,1,1,1,1,1,1,1,1,1,1,1,1,1,1,1,1,1,1,1,1,1,1,1,1,1,1,1,1,1,1,1,1,1,1,1,
1,1,1,1,1,1,1,1,1,1,1,1,1,1,1,1,1,1,1,1,1,1,1,1,1,1,1,1,1,1,1,1,1,1,1,1,
1,1,1,1,1,1,1,1,1,1,1,1,1,1,1,1,1,1,1,1,1,1,1,1,1,1,1,1,1,1,1,1,1,1,1,6),
(2,2),(0.,0.005,0.01,0.015,0.02,0.025,0.03,0.035,0.04,0.045,0.05,0.055,
0.06,0.065,0.07,0.075,0.08,0.085,0.09,0.095,0.1,0.105,0.11,0.115,0.12,0.125,
0.13,0.135,0.14,0.145,0.15,0.155,0.16,0.165,0.17,0.175,0.18,0.185,0.19,
0.195,0.2,0.205,0.21,0.215,0.22,0.225,0.23,0.235,0.24,0.245,0.25,0.255,
0.26,0.265,0.27,0.275,0.28,0.285,0.29,0.295,0.3,0.305,0.31,0.315,0.32,0.325,
0.33,0.335,0.34,0.345,0.35,0.355,0.36,0.365,0.37,0.375,0.38,0.385,0.39,
0.395,0.4,0.405,0.41,0.415,0.42,0.425,0.43,0.435,0.44,0.445,0.45,0.455,
0.46,0.465,0.47,0.475,0.48,0.485,0.49,0.495,0.5,0.505,0.51,0.515,0.52,0.525,
0.53,0.535,0.54,0.545,0.55,0.555,0.56,0.565,0.57,0.575,0.58,0.585,0.59,
0.595,0.6,0.605,0.61,0.615,0.62,0.625,0.63,0.635,0.64,0.645,0.65,0.655,
0.66,0.665,0.67,0.675,0.68,0.685,0.690000000000001,0.695000000000001,0.700000000000001,
0.705000000000001,0.710000000000001,0.715000000000001,0.720000000000001,
0.725000000000001,0.730000000000001,0.735000000000001,0.740000000000001,
0.745000000000001,0.750000000000001,0.755000000000001,0.760000000000001,
0.765000000000001,0.770000000000001,0.775000000000001,0.780000000000001,
0.785000000000001,0.790000000000001,0.795000000000001,0.800000000000001,
0.805000000000001,0.810000000000001,0.815000000000001,0.820000000000001,
0.825000000000001,0.830000000000001,0.835000000000001,0.840000000000001,
0.845000000000001,0.850000000000001,0.855000000000001,0.860000000000001,
0.865000000000001,0.870000000000001,0.875000000000001,0.880000000000001,
0.885000000000001,0.890000000000001,0.895000000000001,0.900000000000001,
0.905000000000001,0.910000000000001,0.915000000000001,0.920000000000001,
0.925000000000001,0.930000000000001,0.935000000000001,0.940000000000001,
0.945000000000001,0.950000000000001,0.955000000000001,0.960000000000001,
0.965000000000001,0.970000000000001,0.975000000000001,0.980000000000001,
0.985000000000001,0.990000000000001,0.995000000000001,1.),(0.,1.2),
 .UNSPECIFIED.)
GEOMETRIC_REPRESENTATION_ITEM()
RATIONAL_B_SPLINE_SURFACE(((1.,1.),(1.,1.),(1.,1.),(1.,1.),(1.,1.),(1.,
1.),(1.,1.),(1.,1.),(1.,1.),(1.,1.),(1.,1.),(1.,1.),(1.,1.),(1.,1.),(1.,
1.),(1.,1.),(1.,1.),(1.,1.),(1.,1.),(1.,1.),(1.,1.),(1.,1.),(1.,1.),(1.,
1.),(1.,1.),(1.,1.),(1.,1.),(1.,1.),(1.,1.),(1.,1.),(1.,1.),(1.,1.),(1.,
1.),(1.,1.),(1.,1.),(1.,1.),(1.,1.),(1.,1.),(1.,1.),(1.,1.),(1.,1.),(1.,
1.),(1.,1.),(1.,1.),(1.,1.),(1.,1.),(1.,1.),(1.,1.),(1.,1.),(1.,1.),(1.,
1.),(1.,1.),(1.,1.),(1.,1.),(1.,1.),(1.,1.),(1.,1.),(1.,1.),(1.,1.),(1.,
1.),(1.,1.),(1.,1.),(1.,1.),(1.,1.),(1.,1.),(1.,1.),(1.,1.),(1.,1.),(1.,
1.),(1.,1.),(1.,1.),(1.,1.),(1.,1.),(1.,1.),(1.,1.),(1.,1.),(1.,1.),(1.,
1.),(1.,1.),(1.,1.),(1.,1.),(1.,1.),(1.,1.),(1.,1.),(1.,1.),(1.,1.),(1.,
1.),(1.,1.),(1.,1.),(1.,1.),(1.,1.),(1.,1.),(1.,1.),(1.,1.),(1.,1.),(1.,
1.),(1.,1.),(1.,1.),(1.,1.),(1.,1.),(1.,1.),(1.,1.),(1.,1.),(1.,1.),(1.,
1.),(1.,1.),(1.,1.),(1.,1.),(1.,1.),(1.,1.),(1.,1.),(1.,1.),(1.,1.),(1.,
1.),(1.,1.),(1.,1.),(1.,1.),(1.,1.),(1.,1.),(1.,1.),(1.,1.),(1.,1.),(1.,
1.),(1.,1.),(1.,1.),(1.,1.),(1.,1.),(1.,1.),(1.,1.),(1.,1.),(1.,1.),(1.,
1.),(1.,1.),(1.,1.),(1.,1.),(1.,1.),(1.,1.),(1.,1.),(1.,1.),(1.,1.),(1.,
1.),(1.,1.),(1.,1.),(1.,1.),(1.,1.),(1.,1.),(1.,1.),(1.,1.),(1.,1.),(1.,
1.),(1.,1.),(1.,1.),(1.,1.),(1.,1.),(1.,1.),(1.,1.),(1.,1.),(1.,1.),(1.,
1.),(1.,1.),(1.,1.),(1.,1.),(1.,1.),(1.,1.),(1.,1.),(1.,1.),(1.,1.),(1.,
1.),(1.,1.),(1.,1.),(1.,1.),(1.,1.),(1.,1.),(1.,1.),(1.,1.),(1.,1.),(1.,
1.),(1.,1.),(1.,1.),(1.,1.),(1.,1.),(1.,1.),(1.,1.),(1.,1.),(1.,1.),(1.,
1.),(1.,1.),(1.,1.),(1.,1.),(1.,1.),(1.,1.),(1.,1.),(1.,1.),(1.,1.),(1.,
1.),(1.,1.),(1.,1.),(1.,1.),(1.,1.),(1.,1.),(1.,1.),(1.,1.),(1.,1.),(1.,
1.),(1.,1.)))
REPRESENTATION_ITEM('')
SURFACE()
);
#952=(
BOUNDED_SURFACE()
B_SPLINE_SURFACE(5,1,((#114446,#114447),(#114448,#114449),(#114450,#114451),
(#114452,#114453),(#114454,#114455),(#114456,#114457),(#114458,#114459),
(#114460,#114461),(#114462,#114463),(#114464,#114465),(#114466,#114467),
(#114468,#114469),(#114470,#114471),(#114472,#114473),(#114474,#114475),
(#114476,#114477),(#114478,#114479),(#114480,#114481),(#114482,#114483),
(#114484,#114485),(#114486,#114487),(#114488,#114489),(#114490,#114491),
(#114492,#114493),(#114494,#114495),(#114496,#114497),(#114498,#114499),
(#114500,#114501),(#114502,#114503),(#114504,#114505),(#114506,#114507),
(#114508,#114509),(#114510,#114511),(#114512,#114513),(#114514,#114515),
(#114516,#114517),(#114518,#114519),(#114520,#114521),(#114522,#114523),
(#114524,#114525),(#114526,#114527),(#114528,#114529),(#114530,#114531),
(#114532,#114533),(#114534,#114535),(#114536,#114537),(#114538,#114539),
(#114540,#114541),(#114542,#114543),(#114544,#114545),(#114546,#114547),
(#114548,#114549),(#114550,#114551),(#114552,#114553),(#114554,#114555),
(#114556,#114557),(#114558,#114559),(#114560,#114561),(#114562,#114563),
(#114564,#114565),(#114566,#114567),(#114568,#114569),(#114570,#114571),
(#114572,#114573),(#114574,#114575),(#114576,#114577),(#114578,#114579),
(#114580,#114581),(#114582,#114583),(#114584,#114585),(#114586,#114587),
(#114588,#114589),(#114590,#114591),(#114592,#114593),(#114594,#114595),
(#114596,#114597),(#114598,#114599),(#114600,#114601),(#114602,#114603),
(#114604,#114605),(#114606,#114607),(#114608,#114609),(#114610,#114611),
(#114612,#114613),(#114614,#114615),(#114616,#114617),(#114618,#114619),
(#114620,#114621),(#114622,#114623),(#114624,#114625),(#114626,#114627),
(#114628,#114629),(#114630,#114631),(#114632,#114633),(#114634,#114635),
(#114636,#114637),(#114638,#114639),(#114640,#114641),(#114642,#114643),
(#114644,#114645),(#114646,#114647),(#114648,#114649),(#114650,#114651),
(#114652,#114653),(#114654,#114655),(#114656,#114657),(#114658,#114659),
(#114660,#114661),(#114662,#114663),(#114664,#114665),(#114666,#114667),
(#114668,#114669),(#114670,#114671),(#114672,#114673),(#114674,#114675),
(#114676,#114677),(#114678,#114679),(#114680,#114681),(#114682,#114683),
(#114684,#114685),(#114686,#114687),(#114688,#114689),(#114690,#114691),
(#114692,#114693),(#114694,#114695),(#114696,#114697),(#114698,#114699),
(#114700,#114701),(#114702,#114703),(#114704,#114705),(#114706,#114707),
(#114708,#114709),(#114710,#114711),(#114712,#114713),(#114714,#114715),
(#114716,#114717),(#114718,#114719),(#114720,#114721),(#114722,#114723),
(#114724,#114725),(#114726,#114727),(#114728,#114729),(#114730,#114731),
(#114732,#114733),(#114734,#114735),(#114736,#114737),(#114738,#114739),
(#114740,#114741),(#114742,#114743),(#114744,#114745),(#114746,#114747),
(#114748,#114749),(#114750,#114751),(#114752,#114753),(#114754,#114755),
(#114756,#114757),(#114758,#114759),(#114760,#114761),(#114762,#114763),
(#114764,#114765),(#114766,#114767),(#114768,#114769),(#114770,#114771),
(#114772,#114773),(#114774,#114775),(#114776,#114777),(#114778,#114779),
(#114780,#114781),(#114782,#114783),(#114784,#114785),(#114786,#114787),
(#114788,#114789),(#114790,#114791),(#114792,#114793),(#114794,#114795),
(#114796,#114797),(#114798,#114799),(#114800,#114801),(#114802,#114803),
(#114804,#114805),(#114806,#114807),(#114808,#114809),(#114810,#114811),
(#114812,#114813),(#114814,#114815),(#114816,#114817),(#114818,#114819),
(#114820,#114821),(#114822,#114823),(#114824,#114825),(#114826,#114827),
(#114828,#114829),(#114830,#114831),(#114832,#114833),(#114834,#114835),
(#114836,#114837),(#114838,#114839),(#114840,#114841),(#114842,#114843),
(#114844,#114845),(#114846,#114847),(#114848,#114849),(#114850,#114851),
(#114852,#114853),(#114854,#114855)),.UNSPECIFIED.,.F.,.F.,.F.)
B_SPLINE_SURFACE_WITH_KNOTS((6,1,1,1,1,1,1,1,1,1,1,1,1,1,1,1,1,1,1,1,1,
1,1,1,1,1,1,1,1,1,1,1,1,1,1,1,1,1,1,1,1,1,1,1,1,1,1,1,1,1,1,1,1,1,1,1,1,
1,1,1,1,1,1,1,1,1,1,1,1,1,1,1,1,1,1,1,1,1,1,1,1,1,1,1,1,1,1,1,1,1,1,1,1,
1,1,1,1,1,1,1,1,1,1,1,1,1,1,1,1,1,1,1,1,1,1,1,1,1,1,1,1,1,1,1,1,1,1,1,1,
1,1,1,1,1,1,1,1,1,1,1,1,1,1,1,1,1,1,1,1,1,1,1,1,1,1,1,1,1,1,1,1,1,1,1,1,
1,1,1,1,1,1,1,1,1,1,1,1,1,1,1,1,1,1,1,1,1,1,1,1,1,1,1,1,1,1,1,1,1,1,1,6),
(2,2),(0.,0.005,0.01,0.015,0.02,0.025,0.03,0.035,0.04,0.045,0.05,0.055,
0.06,0.065,0.07,0.075,0.08,0.085,0.09,0.095,0.1,0.105,0.11,0.115,0.12,0.125,
0.13,0.135,0.14,0.145,0.15,0.155,0.16,0.165,0.17,0.175,0.18,0.185,0.19,
0.195,0.2,0.205,0.21,0.215,0.22,0.225,0.23,0.235,0.24,0.245,0.25,0.255,
0.26,0.265,0.27,0.275,0.28,0.285,0.29,0.295,0.3,0.305,0.31,0.315,0.32,0.325,
0.33,0.335,0.34,0.345,0.35,0.355,0.36,0.365,0.37,0.375,0.38,0.385,0.39,
0.395,0.4,0.405,0.41,0.415,0.42,0.425,0.43,0.435,0.44,0.445,0.45,0.455,
0.46,0.465,0.47,0.475,0.48,0.485,0.49,0.495,0.5,0.505,0.51,0.515,0.52,0.525,
0.53,0.535,0.54,0.545,0.55,0.555,0.56,0.565,0.57,0.575,0.58,0.585,0.59,
0.595,0.6,0.605,0.61,0.615,0.62,0.625,0.63,0.635,0.64,0.645,0.65,0.655,
0.66,0.665,0.67,0.675,0.68,0.685,0.690000000000001,0.695000000000001,0.700000000000001,
0.705000000000001,0.710000000000001,0.715000000000001,0.720000000000001,
0.725000000000001,0.730000000000001,0.735000000000001,0.740000000000001,
0.745000000000001,0.750000000000001,0.755000000000001,0.760000000000001,
0.765000000000001,0.770000000000001,0.775000000000001,0.780000000000001,
0.785000000000001,0.790000000000001,0.795000000000001,0.800000000000001,
0.805000000000001,0.810000000000001,0.815000000000001,0.820000000000001,
0.825000000000001,0.830000000000001,0.835000000000001,0.840000000000001,
0.845000000000001,0.850000000000001,0.855000000000001,0.860000000000001,
0.865000000000001,0.870000000000001,0.875000000000001,0.880000000000001,
0.885000000000001,0.890000000000001,0.895000000000001,0.900000000000001,
0.905000000000001,0.910000000000001,0.915000000000001,0.920000000000001,
0.925000000000001,0.930000000000001,0.935000000000001,0.940000000000001,
0.945000000000001,0.950000000000001,0.955000000000001,0.960000000000001,
0.965000000000001,0.970000000000001,0.975000000000001,0.980000000000001,
0.985000000000001,0.990000000000001,0.995000000000001,1.),(0.,1.2),
 .UNSPECIFIED.)
GEOMETRIC_REPRESENTATION_ITEM()
RATIONAL_B_SPLINE_SURFACE(((1.,1.),(1.,1.),(1.,1.),(1.,1.),(1.,1.),(1.,
1.),(1.,1.),(1.,1.),(1.,1.),(1.,1.),(1.,1.),(1.,1.),(1.,1.),(1.,1.),(1.,
1.),(1.,1.),(1.,1.),(1.,1.),(1.,1.),(1.,1.),(1.,1.),(1.,1.),(1.,1.),(1.,
1.),(1.,1.),(1.,1.),(1.,1.),(1.,1.),(1.,1.),(1.,1.),(1.,1.),(1.,1.),(1.,
1.),(1.,1.),(1.,1.),(1.,1.),(1.,1.),(1.,1.),(1.,1.),(1.,1.),(1.,1.),(1.,
1.),(1.,1.),(1.,1.),(1.,1.),(1.,1.),(1.,1.),(1.,1.),(1.,1.),(1.,1.),(1.,
1.),(1.,1.),(1.,1.),(1.,1.),(1.,1.),(1.,1.),(1.,1.),(1.,1.),(1.,1.),(1.,
1.),(1.,1.),(1.,1.),(1.,1.),(1.,1.),(1.,1.),(1.,1.),(1.,1.),(1.,1.),(1.,
1.),(1.,1.),(1.,1.),(1.,1.),(1.,1.),(1.,1.),(1.,1.),(1.,1.),(1.,1.),(1.,
1.),(1.,1.),(1.,1.),(1.,1.),(1.,1.),(1.,1.),(1.,1.),(1.,1.),(1.,1.),(1.,
1.),(1.,1.),(1.,1.),(1.,1.),(1.,1.),(1.,1.),(1.,1.),(1.,1.),(1.,1.),(1.,
1.),(1.,1.),(1.,1.),(1.,1.),(1.,1.),(1.,1.),(1.,1.),(1.,1.),(1.,1.),(1.,
1.),(1.,1.),(1.,1.),(1.,1.),(1.,1.),(1.,1.),(1.,1.),(1.,1.),(1.,1.),(1.,
1.),(1.,1.),(1.,1.),(1.,1.),(1.,1.),(1.,1.),(1.,1.),(1.,1.),(1.,1.),(1.,
1.),(1.,1.),(1.,1.),(1.,1.),(1.,1.),(1.,1.),(1.,1.),(1.,1.),(1.,1.),(1.,
1.),(1.,1.),(1.,1.),(1.,1.),(1.,1.),(1.,1.),(1.,1.),(1.,1.),(1.,1.),(1.,
1.),(1.,1.),(1.,1.),(1.,1.),(1.,1.),(1.,1.),(1.,1.),(1.,1.),(1.,1.),(1.,
1.),(1.,1.),(1.,1.),(1.,1.),(1.,1.),(1.,1.),(1.,1.),(1.,1.),(1.,1.),(1.,
1.),(1.,1.),(1.,1.),(1.,1.),(1.,1.),(1.,1.),(1.,1.),(1.,1.),(1.,1.),(1.,
1.),(1.,1.),(1.,1.),(1.,1.),(1.,1.),(1.,1.),(1.,1.),(1.,1.),(1.,1.),(1.,
1.),(1.,1.),(1.,1.),(1.,1.),(1.,1.),(1.,1.),(1.,1.),(1.,1.),(1.,1.),(1.,
1.),(1.,1.),(1.,1.),(1.,1.),(1.,1.),(1.,1.),(1.,1.),(1.,1.),(1.,1.),(1.,
1.),(1.,1.),(1.,1.),(1.,1.),(1.,1.),(1.,1.),(1.,1.),(1.,1.),(1.,1.),(1.,
1.),(1.,1.)))
REPRESENTATION_ITEM('')
SURFACE()
);
#953=(
BOUNDED_SURFACE()
B_SPLINE_SURFACE(5,1,((#115342,#115343),(#115344,#115345),(#115346,#115347),
(#115348,#115349),(#115350,#115351),(#115352,#115353),(#115354,#115355),
(#115356,#115357),(#115358,#115359),(#115360,#115361),(#115362,#115363),
(#115364,#115365),(#115366,#115367),(#115368,#115369),(#115370,#115371),
(#115372,#115373),(#115374,#115375),(#115376,#115377),(#115378,#115379),
(#115380,#115381),(#115382,#115383),(#115384,#115385),(#115386,#115387),
(#115388,#115389),(#115390,#115391),(#115392,#115393),(#115394,#115395),
(#115396,#115397),(#115398,#115399),(#115400,#115401),(#115402,#115403),
(#115404,#115405),(#115406,#115407),(#115408,#115409),(#115410,#115411),
(#115412,#115413),(#115414,#115415),(#115416,#115417),(#115418,#115419),
(#115420,#115421),(#115422,#115423),(#115424,#115425),(#115426,#115427),
(#115428,#115429),(#115430,#115431),(#115432,#115433),(#115434,#115435),
(#115436,#115437),(#115438,#115439),(#115440,#115441),(#115442,#115443),
(#115444,#115445),(#115446,#115447),(#115448,#115449),(#115450,#115451),
(#115452,#115453),(#115454,#115455),(#115456,#115457),(#115458,#115459),
(#115460,#115461),(#115462,#115463),(#115464,#115465),(#115466,#115467),
(#115468,#115469),(#115470,#115471),(#115472,#115473),(#115474,#115475),
(#115476,#115477),(#115478,#115479),(#115480,#115481),(#115482,#115483),
(#115484,#115485),(#115486,#115487),(#115488,#115489),(#115490,#115491),
(#115492,#115493),(#115494,#115495),(#115496,#115497),(#115498,#115499),
(#115500,#115501),(#115502,#115503),(#115504,#115505),(#115506,#115507),
(#115508,#115509),(#115510,#115511),(#115512,#115513),(#115514,#115515),
(#115516,#115517),(#115518,#115519),(#115520,#115521),(#115522,#115523),
(#115524,#115525),(#115526,#115527),(#115528,#115529),(#115530,#115531),
(#115532,#115533),(#115534,#115535),(#115536,#115537),(#115538,#115539),
(#115540,#115541),(#115542,#115543),(#115544,#115545),(#115546,#115547),
(#115548,#115549),(#115550,#115551),(#115552,#115553),(#115554,#115555),
(#115556,#115557),(#115558,#115559),(#115560,#115561),(#115562,#115563),
(#115564,#115565),(#115566,#115567),(#115568,#115569),(#115570,#115571),
(#115572,#115573),(#115574,#115575),(#115576,#115577),(#115578,#115579),
(#115580,#115581),(#115582,#115583),(#115584,#115585),(#115586,#115587),
(#115588,#115589),(#115590,#115591),(#115592,#115593),(#115594,#115595),
(#115596,#115597),(#115598,#115599),(#115600,#115601),(#115602,#115603),
(#115604,#115605),(#115606,#115607),(#115608,#115609),(#115610,#115611),
(#115612,#115613),(#115614,#115615),(#115616,#115617),(#115618,#115619),
(#115620,#115621),(#115622,#115623),(#115624,#115625),(#115626,#115627),
(#115628,#115629),(#115630,#115631),(#115632,#115633),(#115634,#115635),
(#115636,#115637),(#115638,#115639),(#115640,#115641),(#115642,#115643),
(#115644,#115645),(#115646,#115647),(#115648,#115649),(#115650,#115651),
(#115652,#115653),(#115654,#115655),(#115656,#115657),(#115658,#115659),
(#115660,#115661),(#115662,#115663),(#115664,#115665),(#115666,#115667),
(#115668,#115669),(#115670,#115671),(#115672,#115673),(#115674,#115675),
(#115676,#115677),(#115678,#115679),(#115680,#115681),(#115682,#115683),
(#115684,#115685),(#115686,#115687),(#115688,#115689),(#115690,#115691),
(#115692,#115693),(#115694,#115695),(#115696,#115697),(#115698,#115699),
(#115700,#115701),(#115702,#115703),(#115704,#115705),(#115706,#115707),
(#115708,#115709),(#115710,#115711),(#115712,#115713),(#115714,#115715),
(#115716,#115717),(#115718,#115719),(#115720,#115721),(#115722,#115723),
(#115724,#115725),(#115726,#115727),(#115728,#115729),(#115730,#115731),
(#115732,#115733),(#115734,#115735),(#115736,#115737),(#115738,#115739),
(#115740,#115741),(#115742,#115743),(#115744,#115745),(#115746,#115747),
(#115748,#115749),(#115750,#115751)),.UNSPECIFIED.,.F.,.F.,.F.)
B_SPLINE_SURFACE_WITH_KNOTS((6,1,1,1,1,1,1,1,1,1,1,1,1,1,1,1,1,1,1,1,1,
1,1,1,1,1,1,1,1,1,1,1,1,1,1,1,1,1,1,1,1,1,1,1,1,1,1,1,1,1,1,1,1,1,1,1,1,
1,1,1,1,1,1,1,1,1,1,1,1,1,1,1,1,1,1,1,1,1,1,1,1,1,1,1,1,1,1,1,1,1,1,1,1,
1,1,1,1,1,1,1,1,1,1,1,1,1,1,1,1,1,1,1,1,1,1,1,1,1,1,1,1,1,1,1,1,1,1,1,1,
1,1,1,1,1,1,1,1,1,1,1,1,1,1,1,1,1,1,1,1,1,1,1,1,1,1,1,1,1,1,1,1,1,1,1,1,
1,1,1,1,1,1,1,1,1,1,1,1,1,1,1,1,1,1,1,1,1,1,1,1,1,1,1,1,1,1,1,1,1,1,1,6),
(2,2),(0.,0.005,0.01,0.015,0.02,0.025,0.03,0.035,0.04,0.045,0.05,0.055,
0.06,0.065,0.07,0.075,0.08,0.085,0.09,0.095,0.1,0.105,0.11,0.115,0.12,0.125,
0.13,0.135,0.14,0.145,0.15,0.155,0.16,0.165,0.17,0.175,0.18,0.185,0.19,
0.195,0.2,0.205,0.21,0.215,0.22,0.225,0.23,0.235,0.24,0.245,0.25,0.255,
0.26,0.265,0.27,0.275,0.28,0.285,0.29,0.295,0.3,0.305,0.31,0.315,0.32,0.325,
0.33,0.335,0.34,0.345,0.35,0.355,0.36,0.365,0.37,0.375,0.38,0.385,0.39,
0.395,0.4,0.405,0.41,0.415,0.42,0.425,0.43,0.435,0.44,0.445,0.45,0.455,
0.46,0.465,0.47,0.475,0.48,0.485,0.49,0.495,0.5,0.505,0.51,0.515,0.52,0.525,
0.53,0.535,0.54,0.545,0.55,0.555,0.56,0.565,0.57,0.575,0.58,0.585,0.59,
0.595,0.6,0.605,0.61,0.615,0.62,0.625,0.63,0.635,0.64,0.645,0.65,0.655,
0.66,0.665,0.67,0.675,0.68,0.685,0.690000000000001,0.695000000000001,0.700000000000001,
0.705000000000001,0.710000000000001,0.715000000000001,0.720000000000001,
0.725000000000001,0.730000000000001,0.735000000000001,0.740000000000001,
0.745000000000001,0.750000000000001,0.755000000000001,0.760000000000001,
0.765000000000001,0.770000000000001,0.775000000000001,0.780000000000001,
0.785000000000001,0.790000000000001,0.795000000000001,0.800000000000001,
0.805000000000001,0.810000000000001,0.815000000000001,0.820000000000001,
0.825000000000001,0.830000000000001,0.835000000000001,0.840000000000001,
0.845000000000001,0.850000000000001,0.855000000000001,0.860000000000001,
0.865000000000001,0.870000000000001,0.875000000000001,0.880000000000001,
0.885000000000001,0.890000000000001,0.895000000000001,0.900000000000001,
0.905000000000001,0.910000000000001,0.915000000000001,0.920000000000001,
0.925000000000001,0.930000000000001,0.935000000000001,0.940000000000001,
0.945000000000001,0.950000000000001,0.955000000000001,0.960000000000001,
0.965000000000001,0.970000000000001,0.975000000000001,0.980000000000001,
0.985000000000001,0.990000000000001,0.995000000000001,1.),(0.,1.2),
 .UNSPECIFIED.)
GEOMETRIC_REPRESENTATION_ITEM()
RATIONAL_B_SPLINE_SURFACE(((1.,1.),(1.,1.),(1.,1.),(1.,1.),(1.,1.),(1.,
1.),(1.,1.),(1.,1.),(1.,1.),(1.,1.),(1.,1.),(1.,1.),(1.,1.),(1.,1.),(1.,
1.),(1.,1.),(1.,1.),(1.,1.),(1.,1.),(1.,1.),(1.,1.),(1.,1.),(1.,1.),(1.,
1.),(1.,1.),(1.,1.),(1.,1.),(1.,1.),(1.,1.),(1.,1.),(1.,1.),(1.,1.),(1.,
1.),(1.,1.),(1.,1.),(1.,1.),(1.,1.),(1.,1.),(1.,1.),(1.,1.),(1.,1.),(1.,
1.),(1.,1.),(1.,1.),(1.,1.),(1.,1.),(1.,1.),(1.,1.),(1.,1.),(1.,1.),(1.,
1.),(1.,1.),(1.,1.),(1.,1.),(1.,1.),(1.,1.),(1.,1.),(1.,1.),(1.,1.),(1.,
1.),(1.,1.),(1.,1.),(1.,1.),(1.,1.),(1.,1.),(1.,1.),(1.,1.),(1.,1.),(1.,
1.),(1.,1.),(1.,1.),(1.,1.),(1.,1.),(1.,1.),(1.,1.),(1.,1.),(1.,1.),(1.,
1.),(1.,1.),(1.,1.),(1.,1.),(1.,1.),(1.,1.),(1.,1.),(1.,1.),(1.,1.),(1.,
1.),(1.,1.),(1.,1.),(1.,1.),(1.,1.),(1.,1.),(1.,1.),(1.,1.),(1.,1.),(1.,
1.),(1.,1.),(1.,1.),(1.,1.),(1.,1.),(1.,1.),(1.,1.),(1.,1.),(1.,1.),(1.,
1.),(1.,1.),(1.,1.),(1.,1.),(1.,1.),(1.,1.),(1.,1.),(1.,1.),(1.,1.),(1.,
1.),(1.,1.),(1.,1.),(1.,1.),(1.,1.),(1.,1.),(1.,1.),(1.,1.),(1.,1.),(1.,
1.),(1.,1.),(1.,1.),(1.,1.),(1.,1.),(1.,1.),(1.,1.),(1.,1.),(1.,1.),(1.,
1.),(1.,1.),(1.,1.),(1.,1.),(1.,1.),(1.,1.),(1.,1.),(1.,1.),(1.,1.),(1.,
1.),(1.,1.),(1.,1.),(1.,1.),(1.,1.),(1.,1.),(1.,1.),(1.,1.),(1.,1.),(1.,
1.),(1.,1.),(1.,1.),(1.,1.),(1.,1.),(1.,1.),(1.,1.),(1.,1.),(1.,1.),(1.,
1.),(1.,1.),(1.,1.),(1.,1.),(1.,1.),(1.,1.),(1.,1.),(1.,1.),(1.,1.),(1.,
1.),(1.,1.),(1.,1.),(1.,1.),(1.,1.),(1.,1.),(1.,1.),(1.,1.),(1.,1.),(1.,
1.),(1.,1.),(1.,1.),(1.,1.),(1.,1.),(1.,1.),(1.,1.),(1.,1.),(1.,1.),(1.,
1.),(1.,1.),(1.,1.),(1.,1.),(1.,1.),(1.,1.),(1.,1.),(1.,1.),(1.,1.),(1.,
1.),(1.,1.),(1.,1.),(1.,1.),(1.,1.),(1.,1.),(1.,1.),(1.,1.),(1.,1.),(1.,
1.),(1.,1.)))
REPRESENTATION_ITEM('')
SURFACE()
);
#954=(
BOUNDED_SURFACE()
B_SPLINE_SURFACE(5,1,((#116192,#116193),(#116194,#116195),(#116196,#116197),
(#116198,#116199),(#116200,#116201),(#116202,#116203),(#116204,#116205),
(#116206,#116207),(#116208,#116209),(#116210,#116211),(#116212,#116213),
(#116214,#116215),(#116216,#116217),(#116218,#116219),(#116220,#116221),
(#116222,#116223),(#116224,#116225),(#116226,#116227),(#116228,#116229),
(#116230,#116231),(#116232,#116233),(#116234,#116235),(#116236,#116237),
(#116238,#116239),(#116240,#116241),(#116242,#116243),(#116244,#116245),
(#116246,#116247),(#116248,#116249),(#116250,#116251),(#116252,#116253),
(#116254,#116255),(#116256,#116257),(#116258,#116259),(#116260,#116261),
(#116262,#116263),(#116264,#116265),(#116266,#116267),(#116268,#116269),
(#116270,#116271),(#116272,#116273),(#116274,#116275),(#116276,#116277),
(#116278,#116279),(#116280,#116281),(#116282,#116283),(#116284,#116285),
(#116286,#116287),(#116288,#116289),(#116290,#116291),(#116292,#116293),
(#116294,#116295),(#116296,#116297),(#116298,#116299),(#116300,#116301),
(#116302,#116303),(#116304,#116305),(#116306,#116307),(#116308,#116309),
(#116310,#116311),(#116312,#116313),(#116314,#116315),(#116316,#116317),
(#116318,#116319),(#116320,#116321),(#116322,#116323),(#116324,#116325),
(#116326,#116327),(#116328,#116329),(#116330,#116331),(#116332,#116333),
(#116334,#116335),(#116336,#116337),(#116338,#116339),(#116340,#116341),
(#116342,#116343),(#116344,#116345),(#116346,#116347),(#116348,#116349),
(#116350,#116351),(#116352,#116353),(#116354,#116355),(#116356,#116357),
(#116358,#116359),(#116360,#116361),(#116362,#116363),(#116364,#116365),
(#116366,#116367),(#116368,#116369),(#116370,#116371),(#116372,#116373),
(#116374,#116375),(#116376,#116377),(#116378,#116379),(#116380,#116381),
(#116382,#116383),(#116384,#116385),(#116386,#116387),(#116388,#116389),
(#116390,#116391),(#116392,#116393),(#116394,#116395),(#116396,#116397),
(#116398,#116399),(#116400,#116401),(#116402,#116403),(#116404,#116405),
(#116406,#116407),(#116408,#116409),(#116410,#116411),(#116412,#116413),
(#116414,#116415),(#116416,#116417),(#116418,#116419),(#116420,#116421),
(#116422,#116423),(#116424,#116425),(#116426,#116427),(#116428,#116429),
(#116430,#116431),(#116432,#116433),(#116434,#116435),(#116436,#116437),
(#116438,#116439),(#116440,#116441),(#116442,#116443),(#116444,#116445),
(#116446,#116447),(#116448,#116449),(#116450,#116451),(#116452,#116453),
(#116454,#116455),(#116456,#116457),(#116458,#116459),(#116460,#116461),
(#116462,#116463),(#116464,#116465),(#116466,#116467),(#116468,#116469),
(#116470,#116471),(#116472,#116473),(#116474,#116475),(#116476,#116477),
(#116478,#116479),(#116480,#116481),(#116482,#116483),(#116484,#116485),
(#116486,#116487),(#116488,#116489),(#116490,#116491),(#116492,#116493),
(#116494,#116495),(#116496,#116497),(#116498,#116499),(#116500,#116501),
(#116502,#116503),(#116504,#116505),(#116506,#116507),(#116508,#116509),
(#116510,#116511),(#116512,#116513),(#116514,#116515),(#116516,#116517),
(#116518,#116519),(#116520,#116521),(#116522,#116523),(#116524,#116525),
(#116526,#116527),(#116528,#116529),(#116530,#116531),(#116532,#116533),
(#116534,#116535),(#116536,#116537),(#116538,#116539),(#116540,#116541),
(#116542,#116543),(#116544,#116545),(#116546,#116547),(#116548,#116549),
(#116550,#116551),(#116552,#116553),(#116554,#116555),(#116556,#116557),
(#116558,#116559),(#116560,#116561),(#116562,#116563),(#116564,#116565),
(#116566,#116567),(#116568,#116569),(#116570,#116571),(#116572,#116573),
(#116574,#116575),(#116576,#116577),(#116578,#116579),(#116580,#116581),
(#116582,#116583),(#116584,#116585),(#116586,#116587),(#116588,#116589),
(#116590,#116591),(#116592,#116593),(#116594,#116595),(#116596,#116597),
(#116598,#116599),(#116600,#116601)),.UNSPECIFIED.,.F.,.F.,.F.)
B_SPLINE_SURFACE_WITH_KNOTS((6,1,1,1,1,1,1,1,1,1,1,1,1,1,1,1,1,1,1,1,1,
1,1,1,1,1,1,1,1,1,1,1,1,1,1,1,1,1,1,1,1,1,1,1,1,1,1,1,1,1,1,1,1,1,1,1,1,
1,1,1,1,1,1,1,1,1,1,1,1,1,1,1,1,1,1,1,1,1,1,1,1,1,1,1,1,1,1,1,1,1,1,1,1,
1,1,1,1,1,1,1,1,1,1,1,1,1,1,1,1,1,1,1,1,1,1,1,1,1,1,1,1,1,1,1,1,1,1,1,1,
1,1,1,1,1,1,1,1,1,1,1,1,1,1,1,1,1,1,1,1,1,1,1,1,1,1,1,1,1,1,1,1,1,1,1,1,
1,1,1,1,1,1,1,1,1,1,1,1,1,1,1,1,1,1,1,1,1,1,1,1,1,1,1,1,1,1,1,1,1,1,1,6),
(2,2),(-1.,-0.995000000000001,-0.990000000000001,-0.985000000000001,-0.980000000000001,
-0.975000000000001,-0.970000000000001,-0.965000000000001,-0.960000000000001,
-0.955000000000001,-0.950000000000001,-0.945000000000001,-0.940000000000001,
-0.935000000000001,-0.930000000000001,-0.925000000000001,-0.920000000000001,
-0.915000000000001,-0.910000000000001,-0.905000000000001,-0.900000000000001,
-0.895000000000001,-0.890000000000001,-0.885000000000001,-0.880000000000001,
-0.875000000000001,-0.870000000000001,-0.865000000000001,-0.860000000000001,
-0.855000000000001,-0.850000000000001,-0.845000000000001,-0.840000000000001,
-0.835000000000001,-0.830000000000001,-0.825000000000001,-0.820000000000001,
-0.815000000000001,-0.810000000000001,-0.805000000000001,-0.800000000000001,
-0.795000000000001,-0.790000000000001,-0.785000000000001,-0.780000000000001,
-0.775000000000001,-0.770000000000001,-0.765000000000001,-0.760000000000001,
-0.755000000000001,-0.750000000000001,-0.745000000000001,-0.740000000000001,
-0.735000000000001,-0.730000000000001,-0.725000000000001,-0.720000000000001,
-0.715000000000001,-0.710000000000001,-0.705000000000001,-0.700000000000001,
-0.695000000000001,-0.690000000000001,-0.685,-0.68,-0.675,-0.67,-0.665,
-0.66,-0.655,-0.65,-0.645,-0.64,-0.635,-0.63,-0.625,-0.62,-0.615,-0.61,
-0.605,-0.6,-0.595,-0.59,-0.585,-0.58,-0.575,-0.57,-0.565,-0.56,-0.555,
-0.55,-0.545,-0.54,-0.535,-0.53,-0.525,-0.52,-0.515,-0.51,-0.505,-0.5,-0.495,
-0.49,-0.485,-0.48,-0.475,-0.47,-0.465,-0.46,-0.455,-0.45,-0.445,-0.44,
-0.435,-0.43,-0.425,-0.42,-0.415,-0.41,-0.405,-0.4,-0.395,-0.39,-0.385,
-0.38,-0.375,-0.37,-0.365,-0.36,-0.355,-0.35,-0.345,-0.34,-0.335,-0.33,
-0.325,-0.32,-0.315,-0.31,-0.305,-0.3,-0.295,-0.29,-0.285,-0.28,-0.275,
-0.27,-0.265,-0.26,-0.255,-0.25,-0.245,-0.24,-0.235,-0.23,-0.225,-0.22,
-0.215,-0.21,-0.205,-0.2,-0.195,-0.19,-0.185,-0.18,-0.175,-0.17,-0.165,
-0.16,-0.155,-0.15,-0.145,-0.14,-0.135,-0.13,-0.125,-0.12,-0.115,-0.11,
-0.105,-0.1,-0.095,-0.09,-0.085,-0.08,-0.075,-0.07,-0.065,-0.06,-0.055,
-0.05,-0.045,-0.04,-0.035,-0.03,-0.025,-0.02,-0.015,-0.01,-0.005,0.),(0.,
1.2),.UNSPECIFIED.)
GEOMETRIC_REPRESENTATION_ITEM()
RATIONAL_B_SPLINE_SURFACE(((1.,1.),(1.,1.),(1.,1.),(1.,1.),(1.,1.),(1.,
1.),(1.,1.),(1.,1.),(1.,1.),(1.,1.),(1.,1.),(1.,1.),(1.,1.),(1.,1.),(1.,
1.),(1.,1.),(1.,1.),(1.,1.),(1.,1.),(1.,1.),(1.,1.),(1.,1.),(1.,1.),(1.,
1.),(1.,1.),(1.,1.),(1.,1.),(1.,1.),(1.,1.),(1.,1.),(1.,1.),(1.,1.),(1.,
1.),(1.,1.),(1.,1.),(1.,1.),(1.,1.),(1.,1.),(1.,1.),(1.,1.),(1.,1.),(1.,
1.),(1.,1.),(1.,1.),(1.,1.),(1.,1.),(1.,1.),(1.,1.),(1.,1.),(1.,1.),(1.,
1.),(1.,1.),(1.,1.),(1.,1.),(1.,1.),(1.,1.),(1.,1.),(1.,1.),(1.,1.),(1.,
1.),(1.,1.),(1.,1.),(1.,1.),(1.,1.),(1.,1.),(1.,1.),(1.,1.),(1.,1.),(1.,
1.),(1.,1.),(1.,1.),(1.,1.),(1.,1.),(1.,1.),(1.,1.),(1.,1.),(1.,1.),(1.,
1.),(1.,1.),(1.,1.),(1.,1.),(1.,1.),(1.,1.),(1.,1.),(1.,1.),(1.,1.),(1.,
1.),(1.,1.),(1.,1.),(1.,1.),(1.,1.),(1.,1.),(1.,1.),(1.,1.),(1.,1.),(1.,
1.),(1.,1.),(1.,1.),(1.,1.),(1.,1.),(1.,1.),(1.,1.),(1.,1.),(1.,1.),(1.,
1.),(1.,1.),(1.,1.),(1.,1.),(1.,1.),(1.,1.),(1.,1.),(1.,1.),(1.,1.),(1.,
1.),(1.,1.),(1.,1.),(1.,1.),(1.,1.),(1.,1.),(1.,1.),(1.,1.),(1.,1.),(1.,
1.),(1.,1.),(1.,1.),(1.,1.),(1.,1.),(1.,1.),(1.,1.),(1.,1.),(1.,1.),(1.,
1.),(1.,1.),(1.,1.),(1.,1.),(1.,1.),(1.,1.),(1.,1.),(1.,1.),(1.,1.),(1.,
1.),(1.,1.),(1.,1.),(1.,1.),(1.,1.),(1.,1.),(1.,1.),(1.,1.),(1.,1.),(1.,
1.),(1.,1.),(1.,1.),(1.,1.),(1.,1.),(1.,1.),(1.,1.),(1.,1.),(1.,1.),(1.,
1.),(1.,1.),(1.,1.),(1.,1.),(1.,1.),(1.,1.),(1.,1.),(1.,1.),(1.,1.),(1.,
1.),(1.,1.),(1.,1.),(1.,1.),(1.,1.),(1.,1.),(1.,1.),(1.,1.),(1.,1.),(1.,
1.),(1.,1.),(1.,1.),(1.,1.),(1.,1.),(1.,1.),(1.,1.),(1.,1.),(1.,1.),(1.,
1.),(1.,1.),(1.,1.),(1.,1.),(1.,1.),(1.,1.),(1.,1.),(1.,1.),(1.,1.),(1.,
1.),(1.,1.),(1.,1.),(1.,1.),(1.,1.),(1.,1.),(1.,1.),(1.,1.),(1.,1.),(1.,
1.),(1.,1.)))
REPRESENTATION_ITEM('')
SURFACE()
);
#955=(
BOUNDED_SURFACE()
B_SPLINE_SURFACE(5,1,((#116993,#116994),(#116995,#116996),(#116997,#116998),
(#116999,#117000),(#117001,#117002),(#117003,#117004),(#117005,#117006),
(#117007,#117008),(#117009,#117010),(#117011,#117012),(#117013,#117014),
(#117015,#117016),(#117017,#117018),(#117019,#117020),(#117021,#117022),
(#117023,#117024),(#117025,#117026),(#117027,#117028),(#117029,#117030),
(#117031,#117032),(#117033,#117034),(#117035,#117036),(#117037,#117038),
(#117039,#117040),(#117041,#117042),(#117043,#117044),(#117045,#117046),
(#117047,#117048),(#117049,#117050),(#117051,#117052),(#117053,#117054),
(#117055,#117056),(#117057,#117058),(#117059,#117060),(#117061,#117062),
(#117063,#117064),(#117065,#117066),(#117067,#117068),(#117069,#117070),
(#117071,#117072),(#117073,#117074),(#117075,#117076),(#117077,#117078),
(#117079,#117080),(#117081,#117082),(#117083,#117084),(#117085,#117086),
(#117087,#117088),(#117089,#117090),(#117091,#117092),(#117093,#117094),
(#117095,#117096),(#117097,#117098),(#117099,#117100),(#117101,#117102),
(#117103,#117104),(#117105,#117106),(#117107,#117108),(#117109,#117110),
(#117111,#117112),(#117113,#117114),(#117115,#117116),(#117117,#117118),
(#117119,#117120),(#117121,#117122),(#117123,#117124),(#117125,#117126),
(#117127,#117128),(#117129,#117130),(#117131,#117132),(#117133,#117134),
(#117135,#117136),(#117137,#117138),(#117139,#117140),(#117141,#117142),
(#117143,#117144),(#117145,#117146),(#117147,#117148),(#117149,#117150),
(#117151,#117152),(#117153,#117154),(#117155,#117156),(#117157,#117158),
(#117159,#117160),(#117161,#117162),(#117163,#117164),(#117165,#117166),
(#117167,#117168),(#117169,#117170),(#117171,#117172),(#117173,#117174),
(#117175,#117176),(#117177,#117178),(#117179,#117180),(#117181,#117182),
(#117183,#117184),(#117185,#117186),(#117187,#117188),(#117189,#117190),
(#117191,#117192),(#117193,#117194),(#117195,#117196),(#117197,#117198),
(#117199,#117200),(#117201,#117202),(#117203,#117204),(#117205,#117206),
(#117207,#117208),(#117209,#117210),(#117211,#117212),(#117213,#117214),
(#117215,#117216),(#117217,#117218),(#117219,#117220),(#117221,#117222),
(#117223,#117224),(#117225,#117226),(#117227,#117228),(#117229,#117230),
(#117231,#117232),(#117233,#117234),(#117235,#117236),(#117237,#117238),
(#117239,#117240),(#117241,#117242),(#117243,#117244),(#117245,#117246),
(#117247,#117248),(#117249,#117250),(#117251,#117252),(#117253,#117254),
(#117255,#117256),(#117257,#117258),(#117259,#117260),(#117261,#117262),
(#117263,#117264),(#117265,#117266),(#117267,#117268),(#117269,#117270),
(#117271,#117272),(#117273,#117274),(#117275,#117276),(#117277,#117278),
(#117279,#117280),(#117281,#117282),(#117283,#117284),(#117285,#117286),
(#117287,#117288),(#117289,#117290),(#117291,#117292),(#117293,#117294),
(#117295,#117296),(#117297,#117298),(#117299,#117300),(#117301,#117302),
(#117303,#117304),(#117305,#117306),(#117307,#117308),(#117309,#117310),
(#117311,#117312),(#117313,#117314),(#117315,#117316),(#117317,#117318),
(#117319,#117320),(#117321,#117322),(#117323,#117324),(#117325,#117326),
(#117327,#117328),(#117329,#117330),(#117331,#117332),(#117333,#117334),
(#117335,#117336),(#117337,#117338),(#117339,#117340),(#117341,#117342),
(#117343,#117344),(#117345,#117346),(#117347,#117348),(#117349,#117350),
(#117351,#117352),(#117353,#117354),(#117355,#117356),(#117357,#117358),
(#117359,#117360),(#117361,#117362),(#117363,#117364),(#117365,#117366),
(#117367,#117368),(#117369,#117370),(#117371,#117372),(#117373,#117374),
(#117375,#117376),(#117377,#117378),(#117379,#117380),(#117381,#117382),
(#117383,#117384),(#117385,#117386),(#117387,#117388),(#117389,#117390),
(#117391,#117392),(#117393,#117394),(#117395,#117396),(#117397,#117398),
(#117399,#117400),(#117401,#117402)),.UNSPECIFIED.,.F.,.F.,.F.)
B_SPLINE_SURFACE_WITH_KNOTS((6,1,1,1,1,1,1,1,1,1,1,1,1,1,1,1,1,1,1,1,1,
1,1,1,1,1,1,1,1,1,1,1,1,1,1,1,1,1,1,1,1,1,1,1,1,1,1,1,1,1,1,1,1,1,1,1,1,
1,1,1,1,1,1,1,1,1,1,1,1,1,1,1,1,1,1,1,1,1,1,1,1,1,1,1,1,1,1,1,1,1,1,1,1,
1,1,1,1,1,1,1,1,1,1,1,1,1,1,1,1,1,1,1,1,1,1,1,1,1,1,1,1,1,1,1,1,1,1,1,1,
1,1,1,1,1,1,1,1,1,1,1,1,1,1,1,1,1,1,1,1,1,1,1,1,1,1,1,1,1,1,1,1,1,1,1,1,
1,1,1,1,1,1,1,1,1,1,1,1,1,1,1,1,1,1,1,1,1,1,1,1,1,1,1,1,1,1,1,1,1,1,1,6),
(2,2),(-1.,-0.995000000000001,-0.990000000000001,-0.985000000000001,-0.980000000000001,
-0.975000000000001,-0.970000000000001,-0.965000000000001,-0.960000000000001,
-0.955000000000001,-0.950000000000001,-0.945000000000001,-0.940000000000001,
-0.935000000000001,-0.930000000000001,-0.925000000000001,-0.920000000000001,
-0.915000000000001,-0.910000000000001,-0.905000000000001,-0.900000000000001,
-0.895000000000001,-0.890000000000001,-0.885000000000001,-0.880000000000001,
-0.875000000000001,-0.870000000000001,-0.865000000000001,-0.860000000000001,
-0.855000000000001,-0.850000000000001,-0.845000000000001,-0.840000000000001,
-0.835000000000001,-0.830000000000001,-0.825000000000001,-0.820000000000001,
-0.815000000000001,-0.810000000000001,-0.805000000000001,-0.800000000000001,
-0.795000000000001,-0.790000000000001,-0.785000000000001,-0.780000000000001,
-0.775000000000001,-0.770000000000001,-0.765000000000001,-0.760000000000001,
-0.755000000000001,-0.750000000000001,-0.745000000000001,-0.740000000000001,
-0.735000000000001,-0.730000000000001,-0.725000000000001,-0.720000000000001,
-0.715000000000001,-0.710000000000001,-0.705000000000001,-0.700000000000001,
-0.695000000000001,-0.690000000000001,-0.685,-0.68,-0.675,-0.67,-0.665,
-0.66,-0.655,-0.65,-0.645,-0.64,-0.635,-0.63,-0.625,-0.62,-0.615,-0.61,
-0.605,-0.6,-0.595,-0.59,-0.585,-0.58,-0.575,-0.57,-0.565,-0.56,-0.555,
-0.55,-0.545,-0.54,-0.535,-0.53,-0.525,-0.52,-0.515,-0.51,-0.505,-0.5,-0.495,
-0.49,-0.485,-0.48,-0.475,-0.47,-0.465,-0.46,-0.455,-0.45,-0.445,-0.44,
-0.435,-0.43,-0.425,-0.42,-0.415,-0.41,-0.405,-0.4,-0.395,-0.39,-0.385,
-0.38,-0.375,-0.37,-0.365,-0.36,-0.355,-0.35,-0.345,-0.34,-0.335,-0.33,
-0.325,-0.32,-0.315,-0.31,-0.305,-0.3,-0.295,-0.29,-0.285,-0.28,-0.275,
-0.27,-0.265,-0.26,-0.255,-0.25,-0.245,-0.24,-0.235,-0.23,-0.225,-0.22,
-0.215,-0.21,-0.205,-0.2,-0.195,-0.19,-0.185,-0.18,-0.175,-0.17,-0.165,
-0.16,-0.155,-0.15,-0.145,-0.14,-0.135,-0.13,-0.125,-0.12,-0.115,-0.11,
-0.105,-0.1,-0.095,-0.09,-0.085,-0.08,-0.075,-0.07,-0.065,-0.06,-0.055,
-0.05,-0.045,-0.04,-0.035,-0.03,-0.025,-0.02,-0.015,-0.01,-0.005,0.),(0.,
1.2),.UNSPECIFIED.)
GEOMETRIC_REPRESENTATION_ITEM()
RATIONAL_B_SPLINE_SURFACE(((1.,1.),(1.,1.),(1.,1.),(1.,1.),(1.,1.),(1.,
1.),(1.,1.),(1.,1.),(1.,1.),(1.,1.),(1.,1.),(1.,1.),(1.,1.),(1.,1.),(1.,
1.),(1.,1.),(1.,1.),(1.,1.),(1.,1.),(1.,1.),(1.,1.),(1.,1.),(1.,1.),(1.,
1.),(1.,1.),(1.,1.),(1.,1.),(1.,1.),(1.,1.),(1.,1.),(1.,1.),(1.,1.),(1.,
1.),(1.,1.),(1.,1.),(1.,1.),(1.,1.),(1.,1.),(1.,1.),(1.,1.),(1.,1.),(1.,
1.),(1.,1.),(1.,1.),(1.,1.),(1.,1.),(1.,1.),(1.,1.),(1.,1.),(1.,1.),(1.,
1.),(1.,1.),(1.,1.),(1.,1.),(1.,1.),(1.,1.),(1.,1.),(1.,1.),(1.,1.),(1.,
1.),(1.,1.),(1.,1.),(1.,1.),(1.,1.),(1.,1.),(1.,1.),(1.,1.),(1.,1.),(1.,
1.),(1.,1.),(1.,1.),(1.,1.),(1.,1.),(1.,1.),(1.,1.),(1.,1.),(1.,1.),(1.,
1.),(1.,1.),(1.,1.),(1.,1.),(1.,1.),(1.,1.),(1.,1.),(1.,1.),(1.,1.),(1.,
1.),(1.,1.),(1.,1.),(1.,1.),(1.,1.),(1.,1.),(1.,1.),(1.,1.),(1.,1.),(1.,
1.),(1.,1.),(1.,1.),(1.,1.),(1.,1.),(1.,1.),(1.,1.),(1.,1.),(1.,1.),(1.,
1.),(1.,1.),(1.,1.),(1.,1.),(1.,1.),(1.,1.),(1.,1.),(1.,1.),(1.,1.),(1.,
1.),(1.,1.),(1.,1.),(1.,1.),(1.,1.),(1.,1.),(1.,1.),(1.,1.),(1.,1.),(1.,
1.),(1.,1.),(1.,1.),(1.,1.),(1.,1.),(1.,1.),(1.,1.),(1.,1.),(1.,1.),(1.,
1.),(1.,1.),(1.,1.),(1.,1.),(1.,1.),(1.,1.),(1.,1.),(1.,1.),(1.,1.),(1.,
1.),(1.,1.),(1.,1.),(1.,1.),(1.,1.),(1.,1.),(1.,1.),(1.,1.),(1.,1.),(1.,
1.),(1.,1.),(1.,1.),(1.,1.),(1.,1.),(1.,1.),(1.,1.),(1.,1.),(1.,1.),(1.,
1.),(1.,1.),(1.,1.),(1.,1.),(1.,1.),(1.,1.),(1.,1.),(1.,1.),(1.,1.),(1.,
1.),(1.,1.),(1.,1.),(1.,1.),(1.,1.),(1.,1.),(1.,1.),(1.,1.),(1.,1.),(1.,
1.),(1.,1.),(1.,1.),(1.,1.),(1.,1.),(1.,1.),(1.,1.),(1.,1.),(1.,1.),(1.,
1.),(1.,1.),(1.,1.),(1.,1.),(1.,1.),(1.,1.),(1.,1.),(1.,1.),(1.,1.),(1.,
1.),(1.,1.),(1.,1.),(1.,1.),(1.,1.),(1.,1.),(1.,1.),(1.,1.),(1.,1.),(1.,
1.),(1.,1.)))
REPRESENTATION_ITEM('')
SURFACE()
);
#956=(
BOUNDED_SURFACE()
B_SPLINE_SURFACE(5,1,((#117794,#117795),(#117796,#117797),(#117798,#117799),
(#117800,#117801),(#117802,#117803),(#117804,#117805),(#117806,#117807),
(#117808,#117809),(#117810,#117811),(#117812,#117813),(#117814,#117815),
(#117816,#117817),(#117818,#117819),(#117820,#117821),(#117822,#117823),
(#117824,#117825),(#117826,#117827),(#117828,#117829),(#117830,#117831),
(#117832,#117833),(#117834,#117835),(#117836,#117837),(#117838,#117839),
(#117840,#117841),(#117842,#117843),(#117844,#117845),(#117846,#117847),
(#117848,#117849),(#117850,#117851),(#117852,#117853),(#117854,#117855),
(#117856,#117857),(#117858,#117859),(#117860,#117861),(#117862,#117863),
(#117864,#117865),(#117866,#117867),(#117868,#117869),(#117870,#117871),
(#117872,#117873),(#117874,#117875),(#117876,#117877),(#117878,#117879),
(#117880,#117881),(#117882,#117883),(#117884,#117885),(#117886,#117887),
(#117888,#117889),(#117890,#117891),(#117892,#117893),(#117894,#117895),
(#117896,#117897),(#117898,#117899),(#117900,#117901),(#117902,#117903),
(#117904,#117905),(#117906,#117907),(#117908,#117909),(#117910,#117911),
(#117912,#117913),(#117914,#117915),(#117916,#117917),(#117918,#117919),
(#117920,#117921),(#117922,#117923),(#117924,#117925),(#117926,#117927),
(#117928,#117929),(#117930,#117931),(#117932,#117933),(#117934,#117935),
(#117936,#117937),(#117938,#117939),(#117940,#117941),(#117942,#117943),
(#117944,#117945),(#117946,#117947),(#117948,#117949),(#117950,#117951),
(#117952,#117953),(#117954,#117955),(#117956,#117957),(#117958,#117959),
(#117960,#117961),(#117962,#117963),(#117964,#117965),(#117966,#117967),
(#117968,#117969),(#117970,#117971),(#117972,#117973),(#117974,#117975),
(#117976,#117977),(#117978,#117979),(#117980,#117981),(#117982,#117983),
(#117984,#117985),(#117986,#117987),(#117988,#117989),(#117990,#117991),
(#117992,#117993),(#117994,#117995),(#117996,#117997),(#117998,#117999),
(#118000,#118001),(#118002,#118003),(#118004,#118005),(#118006,#118007),
(#118008,#118009),(#118010,#118011),(#118012,#118013),(#118014,#118015),
(#118016,#118017),(#118018,#118019),(#118020,#118021),(#118022,#118023),
(#118024,#118025),(#118026,#118027),(#118028,#118029),(#118030,#118031),
(#118032,#118033),(#118034,#118035),(#118036,#118037),(#118038,#118039),
(#118040,#118041),(#118042,#118043),(#118044,#118045),(#118046,#118047),
(#118048,#118049),(#118050,#118051),(#118052,#118053),(#118054,#118055),
(#118056,#118057),(#118058,#118059),(#118060,#118061),(#118062,#118063),
(#118064,#118065),(#118066,#118067),(#118068,#118069),(#118070,#118071),
(#118072,#118073),(#118074,#118075),(#118076,#118077),(#118078,#118079),
(#118080,#118081),(#118082,#118083),(#118084,#118085),(#118086,#118087),
(#118088,#118089),(#118090,#118091),(#118092,#118093),(#118094,#118095),
(#118096,#118097),(#118098,#118099),(#118100,#118101),(#118102,#118103),
(#118104,#118105),(#118106,#118107),(#118108,#118109),(#118110,#118111),
(#118112,#118113),(#118114,#118115),(#118116,#118117),(#118118,#118119),
(#118120,#118121),(#118122,#118123),(#118124,#118125),(#118126,#118127),
(#118128,#118129),(#118130,#118131),(#118132,#118133),(#118134,#118135),
(#118136,#118137),(#118138,#118139),(#118140,#118141),(#118142,#118143),
(#118144,#118145),(#118146,#118147),(#118148,#118149),(#118150,#118151),
(#118152,#118153),(#118154,#118155),(#118156,#118157),(#118158,#118159),
(#118160,#118161),(#118162,#118163),(#118164,#118165),(#118166,#118167),
(#118168,#118169),(#118170,#118171),(#118172,#118173),(#118174,#118175),
(#118176,#118177),(#118178,#118179),(#118180,#118181),(#118182,#118183),
(#118184,#118185),(#118186,#118187),(#118188,#118189),(#118190,#118191),
(#118192,#118193),(#118194,#118195),(#118196,#118197),(#118198,#118199),
(#118200,#118201),(#118202,#118203)),.UNSPECIFIED.,.F.,.F.,.F.)
B_SPLINE_SURFACE_WITH_KNOTS((6,1,1,1,1,1,1,1,1,1,1,1,1,1,1,1,1,1,1,1,1,
1,1,1,1,1,1,1,1,1,1,1,1,1,1,1,1,1,1,1,1,1,1,1,1,1,1,1,1,1,1,1,1,1,1,1,1,
1,1,1,1,1,1,1,1,1,1,1,1,1,1,1,1,1,1,1,1,1,1,1,1,1,1,1,1,1,1,1,1,1,1,1,1,
1,1,1,1,1,1,1,1,1,1,1,1,1,1,1,1,1,1,1,1,1,1,1,1,1,1,1,1,1,1,1,1,1,1,1,1,
1,1,1,1,1,1,1,1,1,1,1,1,1,1,1,1,1,1,1,1,1,1,1,1,1,1,1,1,1,1,1,1,1,1,1,1,
1,1,1,1,1,1,1,1,1,1,1,1,1,1,1,1,1,1,1,1,1,1,1,1,1,1,1,1,1,1,1,1,1,1,1,6),
(2,2),(-1.,-0.995000000000001,-0.990000000000001,-0.985000000000001,-0.980000000000001,
-0.975000000000001,-0.970000000000001,-0.965000000000001,-0.960000000000001,
-0.955000000000001,-0.950000000000001,-0.945000000000001,-0.940000000000001,
-0.935000000000001,-0.930000000000001,-0.925000000000001,-0.920000000000001,
-0.915000000000001,-0.910000000000001,-0.905000000000001,-0.900000000000001,
-0.895000000000001,-0.890000000000001,-0.885000000000001,-0.880000000000001,
-0.875000000000001,-0.870000000000001,-0.865000000000001,-0.860000000000001,
-0.855000000000001,-0.850000000000001,-0.845000000000001,-0.840000000000001,
-0.835000000000001,-0.830000000000001,-0.825000000000001,-0.820000000000001,
-0.815000000000001,-0.810000000000001,-0.805000000000001,-0.800000000000001,
-0.795000000000001,-0.790000000000001,-0.785000000000001,-0.780000000000001,
-0.775000000000001,-0.770000000000001,-0.765000000000001,-0.760000000000001,
-0.755000000000001,-0.750000000000001,-0.745000000000001,-0.740000000000001,
-0.735000000000001,-0.730000000000001,-0.725000000000001,-0.720000000000001,
-0.715000000000001,-0.710000000000001,-0.705000000000001,-0.700000000000001,
-0.695000000000001,-0.690000000000001,-0.685,-0.68,-0.675,-0.67,-0.665,
-0.66,-0.655,-0.65,-0.645,-0.64,-0.635,-0.63,-0.625,-0.62,-0.615,-0.61,
-0.605,-0.6,-0.595,-0.59,-0.585,-0.58,-0.575,-0.57,-0.565,-0.56,-0.555,
-0.55,-0.545,-0.54,-0.535,-0.53,-0.525,-0.52,-0.515,-0.51,-0.505,-0.5,-0.495,
-0.49,-0.485,-0.48,-0.475,-0.47,-0.465,-0.46,-0.455,-0.45,-0.445,-0.44,
-0.435,-0.43,-0.425,-0.42,-0.415,-0.41,-0.405,-0.4,-0.395,-0.39,-0.385,
-0.38,-0.375,-0.37,-0.365,-0.36,-0.355,-0.35,-0.345,-0.34,-0.335,-0.33,
-0.325,-0.32,-0.315,-0.31,-0.305,-0.3,-0.295,-0.29,-0.285,-0.28,-0.275,
-0.27,-0.265,-0.26,-0.255,-0.25,-0.245,-0.24,-0.235,-0.23,-0.225,-0.22,
-0.215,-0.21,-0.205,-0.2,-0.195,-0.19,-0.185,-0.18,-0.175,-0.17,-0.165,
-0.16,-0.155,-0.15,-0.145,-0.14,-0.135,-0.13,-0.125,-0.12,-0.115,-0.11,
-0.105,-0.1,-0.095,-0.09,-0.085,-0.08,-0.075,-0.07,-0.065,-0.06,-0.055,
-0.05,-0.045,-0.04,-0.035,-0.03,-0.025,-0.02,-0.015,-0.01,-0.005,0.),(0.,
1.2),.UNSPECIFIED.)
GEOMETRIC_REPRESENTATION_ITEM()
RATIONAL_B_SPLINE_SURFACE(((1.,1.),(1.,1.),(1.,1.),(1.,1.),(1.,1.),(1.,
1.),(1.,1.),(1.,1.),(1.,1.),(1.,1.),(1.,1.),(1.,1.),(1.,1.),(1.,1.),(1.,
1.),(1.,1.),(1.,1.),(1.,1.),(1.,1.),(1.,1.),(1.,1.),(1.,1.),(1.,1.),(1.,
1.),(1.,1.),(1.,1.),(1.,1.),(1.,1.),(1.,1.),(1.,1.),(1.,1.),(1.,1.),(1.,
1.),(1.,1.),(1.,1.),(1.,1.),(1.,1.),(1.,1.),(1.,1.),(1.,1.),(1.,1.),(1.,
1.),(1.,1.),(1.,1.),(1.,1.),(1.,1.),(1.,1.),(1.,1.),(1.,1.),(1.,1.),(1.,
1.),(1.,1.),(1.,1.),(1.,1.),(1.,1.),(1.,1.),(1.,1.),(1.,1.),(1.,1.),(1.,
1.),(1.,1.),(1.,1.),(1.,1.),(1.,1.),(1.,1.),(1.,1.),(1.,1.),(1.,1.),(1.,
1.),(1.,1.),(1.,1.),(1.,1.),(1.,1.),(1.,1.),(1.,1.),(1.,1.),(1.,1.),(1.,
1.),(1.,1.),(1.,1.),(1.,1.),(1.,1.),(1.,1.),(1.,1.),(1.,1.),(1.,1.),(1.,
1.),(1.,1.),(1.,1.),(1.,1.),(1.,1.),(1.,1.),(1.,1.),(1.,1.),(1.,1.),(1.,
1.),(1.,1.),(1.,1.),(1.,1.),(1.,1.),(1.,1.),(1.,1.),(1.,1.),(1.,1.),(1.,
1.),(1.,1.),(1.,1.),(1.,1.),(1.,1.),(1.,1.),(1.,1.),(1.,1.),(1.,1.),(1.,
1.),(1.,1.),(1.,1.),(1.,1.),(1.,1.),(1.,1.),(1.,1.),(1.,1.),(1.,1.),(1.,
1.),(1.,1.),(1.,1.),(1.,1.),(1.,1.),(1.,1.),(1.,1.),(1.,1.),(1.,1.),(1.,
1.),(1.,1.),(1.,1.),(1.,1.),(1.,1.),(1.,1.),(1.,1.),(1.,1.),(1.,1.),(1.,
1.),(1.,1.),(1.,1.),(1.,1.),(1.,1.),(1.,1.),(1.,1.),(1.,1.),(1.,1.),(1.,
1.),(1.,1.),(1.,1.),(1.,1.),(1.,1.),(1.,1.),(1.,1.),(1.,1.),(1.,1.),(1.,
1.),(1.,1.),(1.,1.),(1.,1.),(1.,1.),(1.,1.),(1.,1.),(1.,1.),(1.,1.),(1.,
1.),(1.,1.),(1.,1.),(1.,1.),(1.,1.),(1.,1.),(1.,1.),(1.,1.),(1.,1.),(1.,
1.),(1.,1.),(1.,1.),(1.,1.),(1.,1.),(1.,1.),(1.,1.),(1.,1.),(1.,1.),(1.,
1.),(1.,1.),(1.,1.),(1.,1.),(1.,1.),(1.,1.),(1.,1.),(1.,1.),(1.,1.),(1.,
1.),(1.,1.),(1.,1.),(1.,1.),(1.,1.),(1.,1.),(1.,1.),(1.,1.),(1.,1.),(1.,
1.),(1.,1.)))
REPRESENTATION_ITEM('')
SURFACE()
);
#957=(
BOUNDED_SURFACE()
B_SPLINE_SURFACE(5,1,((#118595,#118596),(#118597,#118598),(#118599,#118600),
(#118601,#118602),(#118603,#118604),(#118605,#118606),(#118607,#118608),
(#118609,#118610),(#118611,#118612),(#118613,#118614),(#118615,#118616),
(#118617,#118618),(#118619,#118620),(#118621,#118622),(#118623,#118624),
(#118625,#118626),(#118627,#118628),(#118629,#118630),(#118631,#118632),
(#118633,#118634),(#118635,#118636),(#118637,#118638),(#118639,#118640),
(#118641,#118642),(#118643,#118644),(#118645,#118646),(#118647,#118648),
(#118649,#118650),(#118651,#118652),(#118653,#118654),(#118655,#118656),
(#118657,#118658),(#118659,#118660),(#118661,#118662),(#118663,#118664),
(#118665,#118666),(#118667,#118668),(#118669,#118670),(#118671,#118672),
(#118673,#118674),(#118675,#118676),(#118677,#118678),(#118679,#118680),
(#118681,#118682),(#118683,#118684),(#118685,#118686),(#118687,#118688),
(#118689,#118690),(#118691,#118692),(#118693,#118694),(#118695,#118696),
(#118697,#118698),(#118699,#118700),(#118701,#118702),(#118703,#118704),
(#118705,#118706),(#118707,#118708),(#118709,#118710),(#118711,#118712),
(#118713,#118714),(#118715,#118716),(#118717,#118718),(#118719,#118720),
(#118721,#118722),(#118723,#118724),(#118725,#118726),(#118727,#118728),
(#118729,#118730),(#118731,#118732),(#118733,#118734),(#118735,#118736),
(#118737,#118738),(#118739,#118740),(#118741,#118742),(#118743,#118744),
(#118745,#118746),(#118747,#118748),(#118749,#118750),(#118751,#118752),
(#118753,#118754),(#118755,#118756),(#118757,#118758),(#118759,#118760),
(#118761,#118762),(#118763,#118764),(#118765,#118766),(#118767,#118768),
(#118769,#118770),(#118771,#118772),(#118773,#118774),(#118775,#118776),
(#118777,#118778),(#118779,#118780),(#118781,#118782),(#118783,#118784),
(#118785,#118786),(#118787,#118788),(#118789,#118790),(#118791,#118792),
(#118793,#118794),(#118795,#118796),(#118797,#118798),(#118799,#118800),
(#118801,#118802),(#118803,#118804),(#118805,#118806),(#118807,#118808),
(#118809,#118810),(#118811,#118812),(#118813,#118814),(#118815,#118816),
(#118817,#118818),(#118819,#118820),(#118821,#118822),(#118823,#118824),
(#118825,#118826),(#118827,#118828),(#118829,#118830),(#118831,#118832),
(#118833,#118834),(#118835,#118836),(#118837,#118838),(#118839,#118840),
(#118841,#118842),(#118843,#118844),(#118845,#118846),(#118847,#118848),
(#118849,#118850),(#118851,#118852),(#118853,#118854),(#118855,#118856),
(#118857,#118858),(#118859,#118860),(#118861,#118862),(#118863,#118864),
(#118865,#118866),(#118867,#118868),(#118869,#118870),(#118871,#118872),
(#118873,#118874),(#118875,#118876),(#118877,#118878),(#118879,#118880),
(#118881,#118882),(#118883,#118884),(#118885,#118886),(#118887,#118888),
(#118889,#118890),(#118891,#118892),(#118893,#118894),(#118895,#118896),
(#118897,#118898),(#118899,#118900),(#118901,#118902),(#118903,#118904),
(#118905,#118906),(#118907,#118908),(#118909,#118910),(#118911,#118912),
(#118913,#118914),(#118915,#118916),(#118917,#118918),(#118919,#118920),
(#118921,#118922),(#118923,#118924),(#118925,#118926),(#118927,#118928),
(#118929,#118930),(#118931,#118932),(#118933,#118934),(#118935,#118936),
(#118937,#118938),(#118939,#118940),(#118941,#118942),(#118943,#118944),
(#118945,#118946),(#118947,#118948),(#118949,#118950),(#118951,#118952),
(#118953,#118954),(#118955,#118956),(#118957,#118958),(#118959,#118960),
(#118961,#118962),(#118963,#118964),(#118965,#118966),(#118967,#118968),
(#118969,#118970),(#118971,#118972),(#118973,#118974),(#118975,#118976),
(#118977,#118978),(#118979,#118980),(#118981,#118982),(#118983,#118984),
(#118985,#118986),(#118987,#118988),(#118989,#118990),(#118991,#118992),
(#118993,#118994),(#118995,#118996),(#118997,#118998),(#118999,#119000),
(#119001,#119002),(#119003,#119004)),.UNSPECIFIED.,.F.,.F.,.F.)
B_SPLINE_SURFACE_WITH_KNOTS((6,1,1,1,1,1,1,1,1,1,1,1,1,1,1,1,1,1,1,1,1,
1,1,1,1,1,1,1,1,1,1,1,1,1,1,1,1,1,1,1,1,1,1,1,1,1,1,1,1,1,1,1,1,1,1,1,1,
1,1,1,1,1,1,1,1,1,1,1,1,1,1,1,1,1,1,1,1,1,1,1,1,1,1,1,1,1,1,1,1,1,1,1,1,
1,1,1,1,1,1,1,1,1,1,1,1,1,1,1,1,1,1,1,1,1,1,1,1,1,1,1,1,1,1,1,1,1,1,1,1,
1,1,1,1,1,1,1,1,1,1,1,1,1,1,1,1,1,1,1,1,1,1,1,1,1,1,1,1,1,1,1,1,1,1,1,1,
1,1,1,1,1,1,1,1,1,1,1,1,1,1,1,1,1,1,1,1,1,1,1,1,1,1,1,1,1,1,1,1,1,1,1,6),
(2,2),(-1.,-0.995000000000001,-0.990000000000001,-0.985000000000001,-0.980000000000001,
-0.975000000000001,-0.970000000000001,-0.965000000000001,-0.960000000000001,
-0.955000000000001,-0.950000000000001,-0.945000000000001,-0.940000000000001,
-0.935000000000001,-0.930000000000001,-0.925000000000001,-0.920000000000001,
-0.915000000000001,-0.910000000000001,-0.905000000000001,-0.900000000000001,
-0.895000000000001,-0.890000000000001,-0.885000000000001,-0.880000000000001,
-0.875000000000001,-0.870000000000001,-0.865000000000001,-0.860000000000001,
-0.855000000000001,-0.850000000000001,-0.845000000000001,-0.840000000000001,
-0.835000000000001,-0.830000000000001,-0.825000000000001,-0.820000000000001,
-0.815000000000001,-0.810000000000001,-0.805000000000001,-0.800000000000001,
-0.795000000000001,-0.790000000000001,-0.785000000000001,-0.780000000000001,
-0.775000000000001,-0.770000000000001,-0.765000000000001,-0.760000000000001,
-0.755000000000001,-0.750000000000001,-0.745000000000001,-0.740000000000001,
-0.735000000000001,-0.730000000000001,-0.725000000000001,-0.720000000000001,
-0.715000000000001,-0.710000000000001,-0.705000000000001,-0.700000000000001,
-0.695000000000001,-0.690000000000001,-0.685,-0.68,-0.675,-0.67,-0.665,
-0.66,-0.655,-0.65,-0.645,-0.64,-0.635,-0.63,-0.625,-0.62,-0.615,-0.61,
-0.605,-0.6,-0.595,-0.59,-0.585,-0.58,-0.575,-0.57,-0.565,-0.56,-0.555,
-0.55,-0.545,-0.54,-0.535,-0.53,-0.525,-0.52,-0.515,-0.51,-0.505,-0.5,-0.495,
-0.49,-0.485,-0.48,-0.475,-0.47,-0.465,-0.46,-0.455,-0.45,-0.445,-0.44,
-0.435,-0.43,-0.425,-0.42,-0.415,-0.41,-0.405,-0.4,-0.395,-0.39,-0.385,
-0.38,-0.375,-0.37,-0.365,-0.36,-0.355,-0.35,-0.345,-0.34,-0.335,-0.33,
-0.325,-0.32,-0.315,-0.31,-0.305,-0.3,-0.295,-0.29,-0.285,-0.28,-0.275,
-0.27,-0.265,-0.26,-0.255,-0.25,-0.245,-0.24,-0.235,-0.23,-0.225,-0.22,
-0.215,-0.21,-0.205,-0.2,-0.195,-0.19,-0.185,-0.18,-0.175,-0.17,-0.165,
-0.16,-0.155,-0.15,-0.145,-0.14,-0.135,-0.13,-0.125,-0.12,-0.115,-0.11,
-0.105,-0.1,-0.095,-0.09,-0.085,-0.08,-0.075,-0.07,-0.065,-0.06,-0.055,
-0.05,-0.045,-0.04,-0.035,-0.03,-0.025,-0.02,-0.015,-0.01,-0.005,0.),(0.,
1.2),.UNSPECIFIED.)
GEOMETRIC_REPRESENTATION_ITEM()
RATIONAL_B_SPLINE_SURFACE(((1.,1.),(1.,1.),(1.,1.),(1.,1.),(1.,1.),(1.,
1.),(1.,1.),(1.,1.),(1.,1.),(1.,1.),(1.,1.),(1.,1.),(1.,1.),(1.,1.),(1.,
1.),(1.,1.),(1.,1.),(1.,1.),(1.,1.),(1.,1.),(1.,1.),(1.,1.),(1.,1.),(1.,
1.),(1.,1.),(1.,1.),(1.,1.),(1.,1.),(1.,1.),(1.,1.),(1.,1.),(1.,1.),(1.,
1.),(1.,1.),(1.,1.),(1.,1.),(1.,1.),(1.,1.),(1.,1.),(1.,1.),(1.,1.),(1.,
1.),(1.,1.),(1.,1.),(1.,1.),(1.,1.),(1.,1.),(1.,1.),(1.,1.),(1.,1.),(1.,
1.),(1.,1.),(1.,1.),(1.,1.),(1.,1.),(1.,1.),(1.,1.),(1.,1.),(1.,1.),(1.,
1.),(1.,1.),(1.,1.),(1.,1.),(1.,1.),(1.,1.),(1.,1.),(1.,1.),(1.,1.),(1.,
1.),(1.,1.),(1.,1.),(1.,1.),(1.,1.),(1.,1.),(1.,1.),(1.,1.),(1.,1.),(1.,
1.),(1.,1.),(1.,1.),(1.,1.),(1.,1.),(1.,1.),(1.,1.),(1.,1.),(1.,1.),(1.,
1.),(1.,1.),(1.,1.),(1.,1.),(1.,1.),(1.,1.),(1.,1.),(1.,1.),(1.,1.),(1.,
1.),(1.,1.),(1.,1.),(1.,1.),(1.,1.),(1.,1.),(1.,1.),(1.,1.),(1.,1.),(1.,
1.),(1.,1.),(1.,1.),(1.,1.),(1.,1.),(1.,1.),(1.,1.),(1.,1.),(1.,1.),(1.,
1.),(1.,1.),(1.,1.),(1.,1.),(1.,1.),(1.,1.),(1.,1.),(1.,1.),(1.,1.),(1.,
1.),(1.,1.),(1.,1.),(1.,1.),(1.,1.),(1.,1.),(1.,1.),(1.,1.),(1.,1.),(1.,
1.),(1.,1.),(1.,1.),(1.,1.),(1.,1.),(1.,1.),(1.,1.),(1.,1.),(1.,1.),(1.,
1.),(1.,1.),(1.,1.),(1.,1.),(1.,1.),(1.,1.),(1.,1.),(1.,1.),(1.,1.),(1.,
1.),(1.,1.),(1.,1.),(1.,1.),(1.,1.),(1.,1.),(1.,1.),(1.,1.),(1.,1.),(1.,
1.),(1.,1.),(1.,1.),(1.,1.),(1.,1.),(1.,1.),(1.,1.),(1.,1.),(1.,1.),(1.,
1.),(1.,1.),(1.,1.),(1.,1.),(1.,1.),(1.,1.),(1.,1.),(1.,1.),(1.,1.),(1.,
1.),(1.,1.),(1.,1.),(1.,1.),(1.,1.),(1.,1.),(1.,1.),(1.,1.),(1.,1.),(1.,
1.),(1.,1.),(1.,1.),(1.,1.),(1.,1.),(1.,1.),(1.,1.),(1.,1.),(1.,1.),(1.,
1.),(1.,1.),(1.,1.),(1.,1.),(1.,1.),(1.,1.),(1.,1.),(1.,1.),(1.,1.),(1.,
1.),(1.,1.)))
REPRESENTATION_ITEM('')
SURFACE()
);
#958=(
BOUNDED_SURFACE()
B_SPLINE_SURFACE(5,1,((#119396,#119397),(#119398,#119399),(#119400,#119401),
(#119402,#119403),(#119404,#119405),(#119406,#119407),(#119408,#119409),
(#119410,#119411),(#119412,#119413),(#119414,#119415),(#119416,#119417),
(#119418,#119419),(#119420,#119421),(#119422,#119423),(#119424,#119425),
(#119426,#119427),(#119428,#119429),(#119430,#119431),(#119432,#119433),
(#119434,#119435),(#119436,#119437),(#119438,#119439),(#119440,#119441),
(#119442,#119443),(#119444,#119445),(#119446,#119447),(#119448,#119449),
(#119450,#119451),(#119452,#119453),(#119454,#119455),(#119456,#119457),
(#119458,#119459),(#119460,#119461),(#119462,#119463),(#119464,#119465),
(#119466,#119467),(#119468,#119469),(#119470,#119471),(#119472,#119473),
(#119474,#119475),(#119476,#119477),(#119478,#119479),(#119480,#119481),
(#119482,#119483),(#119484,#119485),(#119486,#119487),(#119488,#119489),
(#119490,#119491),(#119492,#119493),(#119494,#119495),(#119496,#119497),
(#119498,#119499),(#119500,#119501),(#119502,#119503),(#119504,#119505),
(#119506,#119507),(#119508,#119509),(#119510,#119511),(#119512,#119513),
(#119514,#119515),(#119516,#119517),(#119518,#119519),(#119520,#119521),
(#119522,#119523),(#119524,#119525),(#119526,#119527),(#119528,#119529),
(#119530,#119531),(#119532,#119533),(#119534,#119535),(#119536,#119537),
(#119538,#119539),(#119540,#119541),(#119542,#119543),(#119544,#119545),
(#119546,#119547),(#119548,#119549),(#119550,#119551),(#119552,#119553),
(#119554,#119555),(#119556,#119557),(#119558,#119559),(#119560,#119561),
(#119562,#119563),(#119564,#119565),(#119566,#119567),(#119568,#119569),
(#119570,#119571),(#119572,#119573),(#119574,#119575),(#119576,#119577),
(#119578,#119579),(#119580,#119581),(#119582,#119583),(#119584,#119585),
(#119586,#119587),(#119588,#119589),(#119590,#119591),(#119592,#119593),
(#119594,#119595),(#119596,#119597),(#119598,#119599),(#119600,#119601),
(#119602,#119603),(#119604,#119605),(#119606,#119607),(#119608,#119609),
(#119610,#119611),(#119612,#119613),(#119614,#119615),(#119616,#119617),
(#119618,#119619),(#119620,#119621),(#119622,#119623),(#119624,#119625),
(#119626,#119627),(#119628,#119629),(#119630,#119631),(#119632,#119633),
(#119634,#119635),(#119636,#119637),(#119638,#119639),(#119640,#119641),
(#119642,#119643),(#119644,#119645),(#119646,#119647),(#119648,#119649),
(#119650,#119651),(#119652,#119653),(#119654,#119655),(#119656,#119657),
(#119658,#119659),(#119660,#119661),(#119662,#119663),(#119664,#119665),
(#119666,#119667),(#119668,#119669),(#119670,#119671),(#119672,#119673),
(#119674,#119675),(#119676,#119677),(#119678,#119679),(#119680,#119681),
(#119682,#119683),(#119684,#119685),(#119686,#119687),(#119688,#119689),
(#119690,#119691),(#119692,#119693),(#119694,#119695),(#119696,#119697),
(#119698,#119699),(#119700,#119701),(#119702,#119703),(#119704,#119705),
(#119706,#119707),(#119708,#119709),(#119710,#119711),(#119712,#119713),
(#119714,#119715),(#119716,#119717),(#119718,#119719),(#119720,#119721),
(#119722,#119723),(#119724,#119725),(#119726,#119727),(#119728,#119729),
(#119730,#119731),(#119732,#119733),(#119734,#119735),(#119736,#119737),
(#119738,#119739),(#119740,#119741),(#119742,#119743),(#119744,#119745),
(#119746,#119747),(#119748,#119749),(#119750,#119751),(#119752,#119753),
(#119754,#119755),(#119756,#119757),(#119758,#119759),(#119760,#119761),
(#119762,#119763),(#119764,#119765),(#119766,#119767),(#119768,#119769),
(#119770,#119771),(#119772,#119773),(#119774,#119775),(#119776,#119777),
(#119778,#119779),(#119780,#119781),(#119782,#119783),(#119784,#119785),
(#119786,#119787),(#119788,#119789),(#119790,#119791),(#119792,#119793),
(#119794,#119795),(#119796,#119797),(#119798,#119799),(#119800,#119801),
(#119802,#119803),(#119804,#119805)),.UNSPECIFIED.,.F.,.F.,.F.)
B_SPLINE_SURFACE_WITH_KNOTS((6,1,1,1,1,1,1,1,1,1,1,1,1,1,1,1,1,1,1,1,1,
1,1,1,1,1,1,1,1,1,1,1,1,1,1,1,1,1,1,1,1,1,1,1,1,1,1,1,1,1,1,1,1,1,1,1,1,
1,1,1,1,1,1,1,1,1,1,1,1,1,1,1,1,1,1,1,1,1,1,1,1,1,1,1,1,1,1,1,1,1,1,1,1,
1,1,1,1,1,1,1,1,1,1,1,1,1,1,1,1,1,1,1,1,1,1,1,1,1,1,1,1,1,1,1,1,1,1,1,1,
1,1,1,1,1,1,1,1,1,1,1,1,1,1,1,1,1,1,1,1,1,1,1,1,1,1,1,1,1,1,1,1,1,1,1,1,
1,1,1,1,1,1,1,1,1,1,1,1,1,1,1,1,1,1,1,1,1,1,1,1,1,1,1,1,1,1,1,1,1,1,1,6),
(2,2),(-1.,-0.995000000000001,-0.990000000000001,-0.985000000000001,-0.980000000000001,
-0.975000000000001,-0.970000000000001,-0.965000000000001,-0.960000000000001,
-0.955000000000001,-0.950000000000001,-0.945000000000001,-0.940000000000001,
-0.935000000000001,-0.930000000000001,-0.925000000000001,-0.920000000000001,
-0.915000000000001,-0.910000000000001,-0.905000000000001,-0.900000000000001,
-0.895000000000001,-0.890000000000001,-0.885000000000001,-0.880000000000001,
-0.875000000000001,-0.870000000000001,-0.865000000000001,-0.860000000000001,
-0.855000000000001,-0.850000000000001,-0.845000000000001,-0.840000000000001,
-0.835000000000001,-0.830000000000001,-0.825000000000001,-0.820000000000001,
-0.815000000000001,-0.810000000000001,-0.805000000000001,-0.800000000000001,
-0.795000000000001,-0.790000000000001,-0.785000000000001,-0.780000000000001,
-0.775000000000001,-0.770000000000001,-0.765000000000001,-0.760000000000001,
-0.755000000000001,-0.750000000000001,-0.745000000000001,-0.740000000000001,
-0.735000000000001,-0.730000000000001,-0.725000000000001,-0.720000000000001,
-0.715000000000001,-0.710000000000001,-0.705000000000001,-0.700000000000001,
-0.695000000000001,-0.690000000000001,-0.685,-0.68,-0.675,-0.67,-0.665,
-0.66,-0.655,-0.65,-0.645,-0.64,-0.635,-0.63,-0.625,-0.62,-0.615,-0.61,
-0.605,-0.6,-0.595,-0.59,-0.585,-0.58,-0.575,-0.57,-0.565,-0.56,-0.555,
-0.55,-0.545,-0.54,-0.535,-0.53,-0.525,-0.52,-0.515,-0.51,-0.505,-0.5,-0.495,
-0.49,-0.485,-0.48,-0.475,-0.47,-0.465,-0.46,-0.455,-0.45,-0.445,-0.44,
-0.435,-0.43,-0.425,-0.42,-0.415,-0.41,-0.405,-0.4,-0.395,-0.39,-0.385,
-0.38,-0.375,-0.37,-0.365,-0.36,-0.355,-0.35,-0.345,-0.34,-0.335,-0.33,
-0.325,-0.32,-0.315,-0.31,-0.305,-0.3,-0.295,-0.29,-0.285,-0.28,-0.275,
-0.27,-0.265,-0.26,-0.255,-0.25,-0.245,-0.24,-0.235,-0.23,-0.225,-0.22,
-0.215,-0.21,-0.205,-0.2,-0.195,-0.19,-0.185,-0.18,-0.175,-0.17,-0.165,
-0.16,-0.155,-0.15,-0.145,-0.14,-0.135,-0.13,-0.125,-0.12,-0.115,-0.11,
-0.105,-0.1,-0.095,-0.09,-0.085,-0.08,-0.075,-0.07,-0.065,-0.06,-0.055,
-0.05,-0.045,-0.04,-0.035,-0.03,-0.025,-0.02,-0.015,-0.01,-0.005,0.),(0.,
1.2),.UNSPECIFIED.)
GEOMETRIC_REPRESENTATION_ITEM()
RATIONAL_B_SPLINE_SURFACE(((1.,1.),(1.,1.),(1.,1.),(1.,1.),(1.,1.),(1.,
1.),(1.,1.),(1.,1.),(1.,1.),(1.,1.),(1.,1.),(1.,1.),(1.,1.),(1.,1.),(1.,
1.),(1.,1.),(1.,1.),(1.,1.),(1.,1.),(1.,1.),(1.,1.),(1.,1.),(1.,1.),(1.,
1.),(1.,1.),(1.,1.),(1.,1.),(1.,1.),(1.,1.),(1.,1.),(1.,1.),(1.,1.),(1.,
1.),(1.,1.),(1.,1.),(1.,1.),(1.,1.),(1.,1.),(1.,1.),(1.,1.),(1.,1.),(1.,
1.),(1.,1.),(1.,1.),(1.,1.),(1.,1.),(1.,1.),(1.,1.),(1.,1.),(1.,1.),(1.,
1.),(1.,1.),(1.,1.),(1.,1.),(1.,1.),(1.,1.),(1.,1.),(1.,1.),(1.,1.),(1.,
1.),(1.,1.),(1.,1.),(1.,1.),(1.,1.),(1.,1.),(1.,1.),(1.,1.),(1.,1.),(1.,
1.),(1.,1.),(1.,1.),(1.,1.),(1.,1.),(1.,1.),(1.,1.),(1.,1.),(1.,1.),(1.,
1.),(1.,1.),(1.,1.),(1.,1.),(1.,1.),(1.,1.),(1.,1.),(1.,1.),(1.,1.),(1.,
1.),(1.,1.),(1.,1.),(1.,1.),(1.,1.),(1.,1.),(1.,1.),(1.,1.),(1.,1.),(1.,
1.),(1.,1.),(1.,1.),(1.,1.),(1.,1.),(1.,1.),(1.,1.),(1.,1.),(1.,1.),(1.,
1.),(1.,1.),(1.,1.),(1.,1.),(1.,1.),(1.,1.),(1.,1.),(1.,1.),(1.,1.),(1.,
1.),(1.,1.),(1.,1.),(1.,1.),(1.,1.),(1.,1.),(1.,1.),(1.,1.),(1.,1.),(1.,
1.),(1.,1.),(1.,1.),(1.,1.),(1.,1.),(1.,1.),(1.,1.),(1.,1.),(1.,1.),(1.,
1.),(1.,1.),(1.,1.),(1.,1.),(1.,1.),(1.,1.),(1.,1.),(1.,1.),(1.,1.),(1.,
1.),(1.,1.),(1.,1.),(1.,1.),(1.,1.),(1.,1.),(1.,1.),(1.,1.),(1.,1.),(1.,
1.),(1.,1.),(1.,1.),(1.,1.),(1.,1.),(1.,1.),(1.,1.),(1.,1.),(1.,1.),(1.,
1.),(1.,1.),(1.,1.),(1.,1.),(1.,1.),(1.,1.),(1.,1.),(1.,1.),(1.,1.),(1.,
1.),(1.,1.),(1.,1.),(1.,1.),(1.,1.),(1.,1.),(1.,1.),(1.,1.),(1.,1.),(1.,
1.),(1.,1.),(1.,1.),(1.,1.),(1.,1.),(1.,1.),(1.,1.),(1.,1.),(1.,1.),(1.,
1.),(1.,1.),(1.,1.),(1.,1.),(1.,1.),(1.,1.),(1.,1.),(1.,1.),(1.,1.),(1.,
1.),(1.,1.),(1.,1.),(1.,1.),(1.,1.),(1.,1.),(1.,1.),(1.,1.),(1.,1.),(1.,
1.),(1.,1.)))
REPRESENTATION_ITEM('')
SURFACE()
);
#959=(
BOUNDED_SURFACE()
B_SPLINE_SURFACE(5,1,((#120197,#120198),(#120199,#120200),(#120201,#120202),
(#120203,#120204),(#120205,#120206),(#120207,#120208),(#120209,#120210),
(#120211,#120212),(#120213,#120214),(#120215,#120216),(#120217,#120218),
(#120219,#120220),(#120221,#120222),(#120223,#120224),(#120225,#120226),
(#120227,#120228),(#120229,#120230),(#120231,#120232),(#120233,#120234),
(#120235,#120236),(#120237,#120238),(#120239,#120240),(#120241,#120242),
(#120243,#120244),(#120245,#120246),(#120247,#120248),(#120249,#120250),
(#120251,#120252),(#120253,#120254),(#120255,#120256),(#120257,#120258),
(#120259,#120260),(#120261,#120262),(#120263,#120264),(#120265,#120266),
(#120267,#120268),(#120269,#120270),(#120271,#120272),(#120273,#120274),
(#120275,#120276),(#120277,#120278),(#120279,#120280),(#120281,#120282),
(#120283,#120284),(#120285,#120286),(#120287,#120288),(#120289,#120290),
(#120291,#120292),(#120293,#120294),(#120295,#120296),(#120297,#120298),
(#120299,#120300),(#120301,#120302),(#120303,#120304),(#120305,#120306),
(#120307,#120308),(#120309,#120310),(#120311,#120312),(#120313,#120314),
(#120315,#120316),(#120317,#120318),(#120319,#120320),(#120321,#120322),
(#120323,#120324),(#120325,#120326),(#120327,#120328),(#120329,#120330),
(#120331,#120332),(#120333,#120334),(#120335,#120336),(#120337,#120338),
(#120339,#120340),(#120341,#120342),(#120343,#120344),(#120345,#120346),
(#120347,#120348),(#120349,#120350),(#120351,#120352),(#120353,#120354),
(#120355,#120356),(#120357,#120358),(#120359,#120360),(#120361,#120362),
(#120363,#120364),(#120365,#120366),(#120367,#120368),(#120369,#120370),
(#120371,#120372),(#120373,#120374),(#120375,#120376),(#120377,#120378),
(#120379,#120380),(#120381,#120382),(#120383,#120384),(#120385,#120386),
(#120387,#120388),(#120389,#120390),(#120391,#120392),(#120393,#120394),
(#120395,#120396),(#120397,#120398),(#120399,#120400),(#120401,#120402),
(#120403,#120404),(#120405,#120406),(#120407,#120408),(#120409,#120410),
(#120411,#120412),(#120413,#120414),(#120415,#120416),(#120417,#120418),
(#120419,#120420),(#120421,#120422),(#120423,#120424),(#120425,#120426),
(#120427,#120428),(#120429,#120430),(#120431,#120432),(#120433,#120434),
(#120435,#120436),(#120437,#120438),(#120439,#120440),(#120441,#120442),
(#120443,#120444),(#120445,#120446),(#120447,#120448),(#120449,#120450),
(#120451,#120452),(#120453,#120454),(#120455,#120456),(#120457,#120458),
(#120459,#120460),(#120461,#120462),(#120463,#120464),(#120465,#120466),
(#120467,#120468),(#120469,#120470),(#120471,#120472),(#120473,#120474),
(#120475,#120476),(#120477,#120478),(#120479,#120480),(#120481,#120482),
(#120483,#120484),(#120485,#120486),(#120487,#120488),(#120489,#120490),
(#120491,#120492),(#120493,#120494),(#120495,#120496),(#120497,#120498),
(#120499,#120500),(#120501,#120502),(#120503,#120504),(#120505,#120506),
(#120507,#120508),(#120509,#120510),(#120511,#120512),(#120513,#120514),
(#120515,#120516),(#120517,#120518),(#120519,#120520),(#120521,#120522),
(#120523,#120524),(#120525,#120526),(#120527,#120528),(#120529,#120530),
(#120531,#120532),(#120533,#120534),(#120535,#120536),(#120537,#120538),
(#120539,#120540),(#120541,#120542),(#120543,#120544),(#120545,#120546),
(#120547,#120548),(#120549,#120550),(#120551,#120552),(#120553,#120554),
(#120555,#120556),(#120557,#120558),(#120559,#120560),(#120561,#120562),
(#120563,#120564),(#120565,#120566),(#120567,#120568),(#120569,#120570),
(#120571,#120572),(#120573,#120574),(#120575,#120576),(#120577,#120578),
(#120579,#120580),(#120581,#120582),(#120583,#120584),(#120585,#120586),
(#120587,#120588),(#120589,#120590),(#120591,#120592),(#120593,#120594),
(#120595,#120596),(#120597,#120598),(#120599,#120600),(#120601,#120602),
(#120603,#120604),(#120605,#120606)),.UNSPECIFIED.,.F.,.F.,.F.)
B_SPLINE_SURFACE_WITH_KNOTS((6,1,1,1,1,1,1,1,1,1,1,1,1,1,1,1,1,1,1,1,1,
1,1,1,1,1,1,1,1,1,1,1,1,1,1,1,1,1,1,1,1,1,1,1,1,1,1,1,1,1,1,1,1,1,1,1,1,
1,1,1,1,1,1,1,1,1,1,1,1,1,1,1,1,1,1,1,1,1,1,1,1,1,1,1,1,1,1,1,1,1,1,1,1,
1,1,1,1,1,1,1,1,1,1,1,1,1,1,1,1,1,1,1,1,1,1,1,1,1,1,1,1,1,1,1,1,1,1,1,1,
1,1,1,1,1,1,1,1,1,1,1,1,1,1,1,1,1,1,1,1,1,1,1,1,1,1,1,1,1,1,1,1,1,1,1,1,
1,1,1,1,1,1,1,1,1,1,1,1,1,1,1,1,1,1,1,1,1,1,1,1,1,1,1,1,1,1,1,1,1,1,1,6),
(2,2),(-1.,-0.995000000000001,-0.990000000000001,-0.985000000000001,-0.980000000000001,
-0.975000000000001,-0.970000000000001,-0.965000000000001,-0.960000000000001,
-0.955000000000001,-0.950000000000001,-0.945000000000001,-0.940000000000001,
-0.935000000000001,-0.930000000000001,-0.925000000000001,-0.920000000000001,
-0.915000000000001,-0.910000000000001,-0.905000000000001,-0.900000000000001,
-0.895000000000001,-0.890000000000001,-0.885000000000001,-0.880000000000001,
-0.875000000000001,-0.870000000000001,-0.865000000000001,-0.860000000000001,
-0.855000000000001,-0.850000000000001,-0.845000000000001,-0.840000000000001,
-0.835000000000001,-0.830000000000001,-0.825000000000001,-0.820000000000001,
-0.815000000000001,-0.810000000000001,-0.805000000000001,-0.800000000000001,
-0.795000000000001,-0.790000000000001,-0.785000000000001,-0.780000000000001,
-0.775000000000001,-0.770000000000001,-0.765000000000001,-0.760000000000001,
-0.755000000000001,-0.750000000000001,-0.745000000000001,-0.740000000000001,
-0.735000000000001,-0.730000000000001,-0.725000000000001,-0.720000000000001,
-0.715000000000001,-0.710000000000001,-0.705000000000001,-0.700000000000001,
-0.695000000000001,-0.690000000000001,-0.685,-0.68,-0.675,-0.67,-0.665,
-0.66,-0.655,-0.65,-0.645,-0.64,-0.635,-0.63,-0.625,-0.62,-0.615,-0.61,
-0.605,-0.6,-0.595,-0.59,-0.585,-0.58,-0.575,-0.57,-0.565,-0.56,-0.555,
-0.55,-0.545,-0.54,-0.535,-0.53,-0.525,-0.52,-0.515,-0.51,-0.505,-0.5,-0.495,
-0.49,-0.485,-0.48,-0.475,-0.47,-0.465,-0.46,-0.455,-0.45,-0.445,-0.44,
-0.435,-0.43,-0.425,-0.42,-0.415,-0.41,-0.405,-0.4,-0.395,-0.39,-0.385,
-0.38,-0.375,-0.37,-0.365,-0.36,-0.355,-0.35,-0.345,-0.34,-0.335,-0.33,
-0.325,-0.32,-0.315,-0.31,-0.305,-0.3,-0.295,-0.29,-0.285,-0.28,-0.275,
-0.27,-0.265,-0.26,-0.255,-0.25,-0.245,-0.24,-0.235,-0.23,-0.225,-0.22,
-0.215,-0.21,-0.205,-0.2,-0.195,-0.19,-0.185,-0.18,-0.175,-0.17,-0.165,
-0.16,-0.155,-0.15,-0.145,-0.14,-0.135,-0.13,-0.125,-0.12,-0.115,-0.11,
-0.105,-0.1,-0.095,-0.09,-0.085,-0.08,-0.075,-0.07,-0.065,-0.06,-0.055,
-0.05,-0.045,-0.04,-0.035,-0.03,-0.025,-0.02,-0.015,-0.01,-0.005,0.),(0.,
1.2),.UNSPECIFIED.)
GEOMETRIC_REPRESENTATION_ITEM()
RATIONAL_B_SPLINE_SURFACE(((1.,1.),(1.,1.),(1.,1.),(1.,1.),(1.,1.),(1.,
1.),(1.,1.),(1.,1.),(1.,1.),(1.,1.),(1.,1.),(1.,1.),(1.,1.),(1.,1.),(1.,
1.),(1.,1.),(1.,1.),(1.,1.),(1.,1.),(1.,1.),(1.,1.),(1.,1.),(1.,1.),(1.,
1.),(1.,1.),(1.,1.),(1.,1.),(1.,1.),(1.,1.),(1.,1.),(1.,1.),(1.,1.),(1.,
1.),(1.,1.),(1.,1.),(1.,1.),(1.,1.),(1.,1.),(1.,1.),(1.,1.),(1.,1.),(1.,
1.),(1.,1.),(1.,1.),(1.,1.),(1.,1.),(1.,1.),(1.,1.),(1.,1.),(1.,1.),(1.,
1.),(1.,1.),(1.,1.),(1.,1.),(1.,1.),(1.,1.),(1.,1.),(1.,1.),(1.,1.),(1.,
1.),(1.,1.),(1.,1.),(1.,1.),(1.,1.),(1.,1.),(1.,1.),(1.,1.),(1.,1.),(1.,
1.),(1.,1.),(1.,1.),(1.,1.),(1.,1.),(1.,1.),(1.,1.),(1.,1.),(1.,1.),(1.,
1.),(1.,1.),(1.,1.),(1.,1.),(1.,1.),(1.,1.),(1.,1.),(1.,1.),(1.,1.),(1.,
1.),(1.,1.),(1.,1.),(1.,1.),(1.,1.),(1.,1.),(1.,1.),(1.,1.),(1.,1.),(1.,
1.),(1.,1.),(1.,1.),(1.,1.),(1.,1.),(1.,1.),(1.,1.),(1.,1.),(1.,1.),(1.,
1.),(1.,1.),(1.,1.),(1.,1.),(1.,1.),(1.,1.),(1.,1.),(1.,1.),(1.,1.),(1.,
1.),(1.,1.),(1.,1.),(1.,1.),(1.,1.),(1.,1.),(1.,1.),(1.,1.),(1.,1.),(1.,
1.),(1.,1.),(1.,1.),(1.,1.),(1.,1.),(1.,1.),(1.,1.),(1.,1.),(1.,1.),(1.,
1.),(1.,1.),(1.,1.),(1.,1.),(1.,1.),(1.,1.),(1.,1.),(1.,1.),(1.,1.),(1.,
1.),(1.,1.),(1.,1.),(1.,1.),(1.,1.),(1.,1.),(1.,1.),(1.,1.),(1.,1.),(1.,
1.),(1.,1.),(1.,1.),(1.,1.),(1.,1.),(1.,1.),(1.,1.),(1.,1.),(1.,1.),(1.,
1.),(1.,1.),(1.,1.),(1.,1.),(1.,1.),(1.,1.),(1.,1.),(1.,1.),(1.,1.),(1.,
1.),(1.,1.),(1.,1.),(1.,1.),(1.,1.),(1.,1.),(1.,1.),(1.,1.),(1.,1.),(1.,
1.),(1.,1.),(1.,1.),(1.,1.),(1.,1.),(1.,1.),(1.,1.),(1.,1.),(1.,1.),(1.,
1.),(1.,1.),(1.,1.),(1.,1.),(1.,1.),(1.,1.),(1.,1.),(1.,1.),(1.,1.),(1.,
1.),(1.,1.),(1.,1.),(1.,1.),(1.,1.),(1.,1.),(1.,1.),(1.,1.),(1.,1.),(1.,
1.),(1.,1.)))
REPRESENTATION_ITEM('')
SURFACE()
);
#960=(
BOUNDED_SURFACE()
B_SPLINE_SURFACE(5,1,((#120998,#120999),(#121000,#121001),(#121002,#121003),
(#121004,#121005),(#121006,#121007),(#121008,#121009),(#121010,#121011),
(#121012,#121013),(#121014,#121015),(#121016,#121017),(#121018,#121019),
(#121020,#121021),(#121022,#121023),(#121024,#121025),(#121026,#121027),
(#121028,#121029),(#121030,#121031),(#121032,#121033),(#121034,#121035),
(#121036,#121037),(#121038,#121039),(#121040,#121041),(#121042,#121043),
(#121044,#121045),(#121046,#121047),(#121048,#121049),(#121050,#121051),
(#121052,#121053),(#121054,#121055),(#121056,#121057),(#121058,#121059),
(#121060,#121061),(#121062,#121063),(#121064,#121065),(#121066,#121067),
(#121068,#121069),(#121070,#121071),(#121072,#121073),(#121074,#121075),
(#121076,#121077),(#121078,#121079),(#121080,#121081),(#121082,#121083),
(#121084,#121085),(#121086,#121087),(#121088,#121089),(#121090,#121091),
(#121092,#121093),(#121094,#121095),(#121096,#121097),(#121098,#121099),
(#121100,#121101),(#121102,#121103),(#121104,#121105),(#121106,#121107),
(#121108,#121109),(#121110,#121111),(#121112,#121113),(#121114,#121115),
(#121116,#121117),(#121118,#121119),(#121120,#121121),(#121122,#121123),
(#121124,#121125),(#121126,#121127),(#121128,#121129),(#121130,#121131),
(#121132,#121133),(#121134,#121135),(#121136,#121137),(#121138,#121139),
(#121140,#121141),(#121142,#121143),(#121144,#121145),(#121146,#121147),
(#121148,#121149),(#121150,#121151),(#121152,#121153),(#121154,#121155),
(#121156,#121157),(#121158,#121159),(#121160,#121161),(#121162,#121163),
(#121164,#121165),(#121166,#121167),(#121168,#121169),(#121170,#121171),
(#121172,#121173),(#121174,#121175),(#121176,#121177),(#121178,#121179),
(#121180,#121181),(#121182,#121183),(#121184,#121185),(#121186,#121187),
(#121188,#121189),(#121190,#121191),(#121192,#121193),(#121194,#121195),
(#121196,#121197),(#121198,#121199),(#121200,#121201),(#121202,#121203),
(#121204,#121205),(#121206,#121207),(#121208,#121209),(#121210,#121211),
(#121212,#121213),(#121214,#121215),(#121216,#121217),(#121218,#121219),
(#121220,#121221),(#121222,#121223),(#121224,#121225),(#121226,#121227),
(#121228,#121229),(#121230,#121231),(#121232,#121233),(#121234,#121235),
(#121236,#121237),(#121238,#121239),(#121240,#121241),(#121242,#121243),
(#121244,#121245),(#121246,#121247),(#121248,#121249),(#121250,#121251),
(#121252,#121253),(#121254,#121255),(#121256,#121257),(#121258,#121259),
(#121260,#121261),(#121262,#121263),(#121264,#121265),(#121266,#121267),
(#121268,#121269),(#121270,#121271),(#121272,#121273),(#121274,#121275),
(#121276,#121277),(#121278,#121279),(#121280,#121281),(#121282,#121283),
(#121284,#121285),(#121286,#121287),(#121288,#121289),(#121290,#121291),
(#121292,#121293),(#121294,#121295),(#121296,#121297),(#121298,#121299),
(#121300,#121301),(#121302,#121303),(#121304,#121305),(#121306,#121307),
(#121308,#121309),(#121310,#121311),(#121312,#121313),(#121314,#121315),
(#121316,#121317),(#121318,#121319),(#121320,#121321),(#121322,#121323),
(#121324,#121325),(#121326,#121327),(#121328,#121329),(#121330,#121331),
(#121332,#121333),(#121334,#121335),(#121336,#121337),(#121338,#121339),
(#121340,#121341),(#121342,#121343),(#121344,#121345),(#121346,#121347),
(#121348,#121349),(#121350,#121351),(#121352,#121353),(#121354,#121355),
(#121356,#121357),(#121358,#121359),(#121360,#121361),(#121362,#121363),
(#121364,#121365),(#121366,#121367),(#121368,#121369),(#121370,#121371),
(#121372,#121373),(#121374,#121375),(#121376,#121377),(#121378,#121379),
(#121380,#121381),(#121382,#121383),(#121384,#121385),(#121386,#121387),
(#121388,#121389),(#121390,#121391),(#121392,#121393),(#121394,#121395),
(#121396,#121397),(#121398,#121399),(#121400,#121401),(#121402,#121403),
(#121404,#121405),(#121406,#121407)),.UNSPECIFIED.,.F.,.F.,.F.)
B_SPLINE_SURFACE_WITH_KNOTS((6,1,1,1,1,1,1,1,1,1,1,1,1,1,1,1,1,1,1,1,1,
1,1,1,1,1,1,1,1,1,1,1,1,1,1,1,1,1,1,1,1,1,1,1,1,1,1,1,1,1,1,1,1,1,1,1,1,
1,1,1,1,1,1,1,1,1,1,1,1,1,1,1,1,1,1,1,1,1,1,1,1,1,1,1,1,1,1,1,1,1,1,1,1,
1,1,1,1,1,1,1,1,1,1,1,1,1,1,1,1,1,1,1,1,1,1,1,1,1,1,1,1,1,1,1,1,1,1,1,1,
1,1,1,1,1,1,1,1,1,1,1,1,1,1,1,1,1,1,1,1,1,1,1,1,1,1,1,1,1,1,1,1,1,1,1,1,
1,1,1,1,1,1,1,1,1,1,1,1,1,1,1,1,1,1,1,1,1,1,1,1,1,1,1,1,1,1,1,1,1,1,1,6),
(2,2),(-1.,-0.995000000000001,-0.990000000000001,-0.985000000000001,-0.980000000000001,
-0.975000000000001,-0.970000000000001,-0.965000000000001,-0.960000000000001,
-0.955000000000001,-0.950000000000001,-0.945000000000001,-0.940000000000001,
-0.935000000000001,-0.930000000000001,-0.925000000000001,-0.920000000000001,
-0.915000000000001,-0.910000000000001,-0.905000000000001,-0.900000000000001,
-0.895000000000001,-0.890000000000001,-0.885000000000001,-0.880000000000001,
-0.875000000000001,-0.870000000000001,-0.865000000000001,-0.860000000000001,
-0.855000000000001,-0.850000000000001,-0.845000000000001,-0.840000000000001,
-0.835000000000001,-0.830000000000001,-0.825000000000001,-0.820000000000001,
-0.815000000000001,-0.810000000000001,-0.805000000000001,-0.800000000000001,
-0.795000000000001,-0.790000000000001,-0.785000000000001,-0.780000000000001,
-0.775000000000001,-0.770000000000001,-0.765000000000001,-0.760000000000001,
-0.755000000000001,-0.750000000000001,-0.745000000000001,-0.740000000000001,
-0.735000000000001,-0.730000000000001,-0.725000000000001,-0.720000000000001,
-0.715000000000001,-0.710000000000001,-0.705000000000001,-0.700000000000001,
-0.695000000000001,-0.690000000000001,-0.685,-0.68,-0.675,-0.67,-0.665,
-0.66,-0.655,-0.65,-0.645,-0.64,-0.635,-0.63,-0.625,-0.62,-0.615,-0.61,
-0.605,-0.6,-0.595,-0.59,-0.585,-0.58,-0.575,-0.57,-0.565,-0.56,-0.555,
-0.55,-0.545,-0.54,-0.535,-0.53,-0.525,-0.52,-0.515,-0.51,-0.505,-0.5,-0.495,
-0.49,-0.485,-0.48,-0.475,-0.47,-0.465,-0.46,-0.455,-0.45,-0.445,-0.44,
-0.435,-0.43,-0.425,-0.42,-0.415,-0.41,-0.405,-0.4,-0.395,-0.39,-0.385,
-0.38,-0.375,-0.37,-0.365,-0.36,-0.355,-0.35,-0.345,-0.34,-0.335,-0.33,
-0.325,-0.32,-0.315,-0.31,-0.305,-0.3,-0.295,-0.29,-0.285,-0.28,-0.275,
-0.27,-0.265,-0.26,-0.255,-0.25,-0.245,-0.24,-0.235,-0.23,-0.225,-0.22,
-0.215,-0.21,-0.205,-0.2,-0.195,-0.19,-0.185,-0.18,-0.175,-0.17,-0.165,
-0.16,-0.155,-0.15,-0.145,-0.14,-0.135,-0.13,-0.125,-0.12,-0.115,-0.11,
-0.105,-0.1,-0.095,-0.09,-0.085,-0.08,-0.075,-0.07,-0.065,-0.06,-0.055,
-0.05,-0.045,-0.04,-0.035,-0.03,-0.025,-0.02,-0.015,-0.01,-0.005,0.),(0.,
1.2),.UNSPECIFIED.)
GEOMETRIC_REPRESENTATION_ITEM()
RATIONAL_B_SPLINE_SURFACE(((1.,1.),(1.,1.),(1.,1.),(1.,1.),(1.,1.),(1.,
1.),(1.,1.),(1.,1.),(1.,1.),(1.,1.),(1.,1.),(1.,1.),(1.,1.),(1.,1.),(1.,
1.),(1.,1.),(1.,1.),(1.,1.),(1.,1.),(1.,1.),(1.,1.),(1.,1.),(1.,1.),(1.,
1.),(1.,1.),(1.,1.),(1.,1.),(1.,1.),(1.,1.),(1.,1.),(1.,1.),(1.,1.),(1.,
1.),(1.,1.),(1.,1.),(1.,1.),(1.,1.),(1.,1.),(1.,1.),(1.,1.),(1.,1.),(1.,
1.),(1.,1.),(1.,1.),(1.,1.),(1.,1.),(1.,1.),(1.,1.),(1.,1.),(1.,1.),(1.,
1.),(1.,1.),(1.,1.),(1.,1.),(1.,1.),(1.,1.),(1.,1.),(1.,1.),(1.,1.),(1.,
1.),(1.,1.),(1.,1.),(1.,1.),(1.,1.),(1.,1.),(1.,1.),(1.,1.),(1.,1.),(1.,
1.),(1.,1.),(1.,1.),(1.,1.),(1.,1.),(1.,1.),(1.,1.),(1.,1.),(1.,1.),(1.,
1.),(1.,1.),(1.,1.),(1.,1.),(1.,1.),(1.,1.),(1.,1.),(1.,1.),(1.,1.),(1.,
1.),(1.,1.),(1.,1.),(1.,1.),(1.,1.),(1.,1.),(1.,1.),(1.,1.),(1.,1.),(1.,
1.),(1.,1.),(1.,1.),(1.,1.),(1.,1.),(1.,1.),(1.,1.),(1.,1.),(1.,1.),(1.,
1.),(1.,1.),(1.,1.),(1.,1.),(1.,1.),(1.,1.),(1.,1.),(1.,1.),(1.,1.),(1.,
1.),(1.,1.),(1.,1.),(1.,1.),(1.,1.),(1.,1.),(1.,1.),(1.,1.),(1.,1.),(1.,
1.),(1.,1.),(1.,1.),(1.,1.),(1.,1.),(1.,1.),(1.,1.),(1.,1.),(1.,1.),(1.,
1.),(1.,1.),(1.,1.),(1.,1.),(1.,1.),(1.,1.),(1.,1.),(1.,1.),(1.,1.),(1.,
1.),(1.,1.),(1.,1.),(1.,1.),(1.,1.),(1.,1.),(1.,1.),(1.,1.),(1.,1.),(1.,
1.),(1.,1.),(1.,1.),(1.,1.),(1.,1.),(1.,1.),(1.,1.),(1.,1.),(1.,1.),(1.,
1.),(1.,1.),(1.,1.),(1.,1.),(1.,1.),(1.,1.),(1.,1.),(1.,1.),(1.,1.),(1.,
1.),(1.,1.),(1.,1.),(1.,1.),(1.,1.),(1.,1.),(1.,1.),(1.,1.),(1.,1.),(1.,
1.),(1.,1.),(1.,1.),(1.,1.),(1.,1.),(1.,1.),(1.,1.),(1.,1.),(1.,1.),(1.,
1.),(1.,1.),(1.,1.),(1.,1.),(1.,1.),(1.,1.),(1.,1.),(1.,1.),(1.,1.),(1.,
1.),(1.,1.),(1.,1.),(1.,1.),(1.,1.),(1.,1.),(1.,1.),(1.,1.),(1.,1.),(1.,
1.),(1.,1.)))
REPRESENTATION_ITEM('')
SURFACE()
);
#961=(
BOUNDED_SURFACE()
B_SPLINE_SURFACE(5,1,((#121799,#121800),(#121801,#121802),(#121803,#121804),
(#121805,#121806),(#121807,#121808),(#121809,#121810),(#121811,#121812),
(#121813,#121814),(#121815,#121816),(#121817,#121818),(#121819,#121820),
(#121821,#121822),(#121823,#121824),(#121825,#121826),(#121827,#121828),
(#121829,#121830),(#121831,#121832),(#121833,#121834),(#121835,#121836),
(#121837,#121838),(#121839,#121840),(#121841,#121842),(#121843,#121844),
(#121845,#121846),(#121847,#121848),(#121849,#121850),(#121851,#121852),
(#121853,#121854),(#121855,#121856),(#121857,#121858),(#121859,#121860),
(#121861,#121862),(#121863,#121864),(#121865,#121866),(#121867,#121868),
(#121869,#121870),(#121871,#121872),(#121873,#121874),(#121875,#121876),
(#121877,#121878),(#121879,#121880),(#121881,#121882),(#121883,#121884),
(#121885,#121886),(#121887,#121888),(#121889,#121890),(#121891,#121892),
(#121893,#121894),(#121895,#121896),(#121897,#121898),(#121899,#121900),
(#121901,#121902),(#121903,#121904),(#121905,#121906),(#121907,#121908),
(#121909,#121910),(#121911,#121912),(#121913,#121914),(#121915,#121916),
(#121917,#121918),(#121919,#121920),(#121921,#121922),(#121923,#121924),
(#121925,#121926),(#121927,#121928),(#121929,#121930),(#121931,#121932),
(#121933,#121934),(#121935,#121936),(#121937,#121938),(#121939,#121940),
(#121941,#121942),(#121943,#121944),(#121945,#121946),(#121947,#121948),
(#121949,#121950),(#121951,#121952),(#121953,#121954),(#121955,#121956),
(#121957,#121958),(#121959,#121960),(#121961,#121962),(#121963,#121964),
(#121965,#121966),(#121967,#121968),(#121969,#121970),(#121971,#121972),
(#121973,#121974),(#121975,#121976),(#121977,#121978),(#121979,#121980),
(#121981,#121982),(#121983,#121984),(#121985,#121986),(#121987,#121988),
(#121989,#121990),(#121991,#121992),(#121993,#121994),(#121995,#121996),
(#121997,#121998),(#121999,#122000),(#122001,#122002),(#122003,#122004),
(#122005,#122006),(#122007,#122008),(#122009,#122010),(#122011,#122012),
(#122013,#122014),(#122015,#122016),(#122017,#122018),(#122019,#122020),
(#122021,#122022),(#122023,#122024),(#122025,#122026),(#122027,#122028),
(#122029,#122030),(#122031,#122032),(#122033,#122034),(#122035,#122036),
(#122037,#122038),(#122039,#122040),(#122041,#122042),(#122043,#122044),
(#122045,#122046),(#122047,#122048),(#122049,#122050),(#122051,#122052),
(#122053,#122054),(#122055,#122056),(#122057,#122058),(#122059,#122060),
(#122061,#122062),(#122063,#122064),(#122065,#122066),(#122067,#122068),
(#122069,#122070),(#122071,#122072),(#122073,#122074),(#122075,#122076),
(#122077,#122078),(#122079,#122080),(#122081,#122082),(#122083,#122084),
(#122085,#122086),(#122087,#122088),(#122089,#122090),(#122091,#122092),
(#122093,#122094),(#122095,#122096),(#122097,#122098),(#122099,#122100),
(#122101,#122102),(#122103,#122104),(#122105,#122106),(#122107,#122108),
(#122109,#122110),(#122111,#122112),(#122113,#122114),(#122115,#122116),
(#122117,#122118),(#122119,#122120),(#122121,#122122),(#122123,#122124),
(#122125,#122126),(#122127,#122128),(#122129,#122130),(#122131,#122132),
(#122133,#122134),(#122135,#122136),(#122137,#122138),(#122139,#122140),
(#122141,#122142),(#122143,#122144),(#122145,#122146),(#122147,#122148),
(#122149,#122150),(#122151,#122152),(#122153,#122154),(#122155,#122156),
(#122157,#122158),(#122159,#122160),(#122161,#122162),(#122163,#122164),
(#122165,#122166),(#122167,#122168),(#122169,#122170),(#122171,#122172),
(#122173,#122174),(#122175,#122176),(#122177,#122178),(#122179,#122180),
(#122181,#122182),(#122183,#122184),(#122185,#122186),(#122187,#122188),
(#122189,#122190),(#122191,#122192),(#122193,#122194),(#122195,#122196),
(#122197,#122198),(#122199,#122200),(#122201,#122202),(#122203,#122204),
(#122205,#122206),(#122207,#122208)),.UNSPECIFIED.,.F.,.F.,.F.)
B_SPLINE_SURFACE_WITH_KNOTS((6,1,1,1,1,1,1,1,1,1,1,1,1,1,1,1,1,1,1,1,1,
1,1,1,1,1,1,1,1,1,1,1,1,1,1,1,1,1,1,1,1,1,1,1,1,1,1,1,1,1,1,1,1,1,1,1,1,
1,1,1,1,1,1,1,1,1,1,1,1,1,1,1,1,1,1,1,1,1,1,1,1,1,1,1,1,1,1,1,1,1,1,1,1,
1,1,1,1,1,1,1,1,1,1,1,1,1,1,1,1,1,1,1,1,1,1,1,1,1,1,1,1,1,1,1,1,1,1,1,1,
1,1,1,1,1,1,1,1,1,1,1,1,1,1,1,1,1,1,1,1,1,1,1,1,1,1,1,1,1,1,1,1,1,1,1,1,
1,1,1,1,1,1,1,1,1,1,1,1,1,1,1,1,1,1,1,1,1,1,1,1,1,1,1,1,1,1,1,1,1,1,1,6),
(2,2),(-1.,-0.995000000000001,-0.990000000000001,-0.985000000000001,-0.980000000000001,
-0.975000000000001,-0.970000000000001,-0.965000000000001,-0.960000000000001,
-0.955000000000001,-0.950000000000001,-0.945000000000001,-0.940000000000001,
-0.935000000000001,-0.930000000000001,-0.925000000000001,-0.920000000000001,
-0.915000000000001,-0.910000000000001,-0.905000000000001,-0.900000000000001,
-0.895000000000001,-0.890000000000001,-0.885000000000001,-0.880000000000001,
-0.875000000000001,-0.870000000000001,-0.865000000000001,-0.860000000000001,
-0.855000000000001,-0.850000000000001,-0.845000000000001,-0.840000000000001,
-0.835000000000001,-0.830000000000001,-0.825000000000001,-0.820000000000001,
-0.815000000000001,-0.810000000000001,-0.805000000000001,-0.800000000000001,
-0.795000000000001,-0.790000000000001,-0.785000000000001,-0.780000000000001,
-0.775000000000001,-0.770000000000001,-0.765000000000001,-0.760000000000001,
-0.755000000000001,-0.750000000000001,-0.745000000000001,-0.740000000000001,
-0.735000000000001,-0.730000000000001,-0.725000000000001,-0.720000000000001,
-0.715000000000001,-0.710000000000001,-0.705000000000001,-0.700000000000001,
-0.695000000000001,-0.690000000000001,-0.685,-0.68,-0.675,-0.67,-0.665,
-0.66,-0.655,-0.65,-0.645,-0.64,-0.635,-0.63,-0.625,-0.62,-0.615,-0.61,
-0.605,-0.6,-0.595,-0.59,-0.585,-0.58,-0.575,-0.57,-0.565,-0.56,-0.555,
-0.55,-0.545,-0.54,-0.535,-0.53,-0.525,-0.52,-0.515,-0.51,-0.505,-0.5,-0.495,
-0.49,-0.485,-0.48,-0.475,-0.47,-0.465,-0.46,-0.455,-0.45,-0.445,-0.44,
-0.435,-0.43,-0.425,-0.42,-0.415,-0.41,-0.405,-0.4,-0.395,-0.39,-0.385,
-0.38,-0.375,-0.37,-0.365,-0.36,-0.355,-0.35,-0.345,-0.34,-0.335,-0.33,
-0.325,-0.32,-0.315,-0.31,-0.305,-0.3,-0.295,-0.29,-0.285,-0.28,-0.275,
-0.27,-0.265,-0.26,-0.255,-0.25,-0.245,-0.24,-0.235,-0.23,-0.225,-0.22,
-0.215,-0.21,-0.205,-0.2,-0.195,-0.19,-0.185,-0.18,-0.175,-0.17,-0.165,
-0.16,-0.155,-0.15,-0.145,-0.14,-0.135,-0.13,-0.125,-0.12,-0.115,-0.11,
-0.105,-0.1,-0.095,-0.09,-0.085,-0.08,-0.075,-0.07,-0.065,-0.06,-0.055,
-0.05,-0.045,-0.04,-0.035,-0.03,-0.025,-0.02,-0.015,-0.01,-0.005,0.),(0.,
1.2),.UNSPECIFIED.)
GEOMETRIC_REPRESENTATION_ITEM()
RATIONAL_B_SPLINE_SURFACE(((1.,1.),(1.,1.),(1.,1.),(1.,1.),(1.,1.),(1.,
1.),(1.,1.),(1.,1.),(1.,1.),(1.,1.),(1.,1.),(1.,1.),(1.,1.),(1.,1.),(1.,
1.),(1.,1.),(1.,1.),(1.,1.),(1.,1.),(1.,1.),(1.,1.),(1.,1.),(1.,1.),(1.,
1.),(1.,1.),(1.,1.),(1.,1.),(1.,1.),(1.,1.),(1.,1.),(1.,1.),(1.,1.),(1.,
1.),(1.,1.),(1.,1.),(1.,1.),(1.,1.),(1.,1.),(1.,1.),(1.,1.),(1.,1.),(1.,
1.),(1.,1.),(1.,1.),(1.,1.),(1.,1.),(1.,1.),(1.,1.),(1.,1.),(1.,1.),(1.,
1.),(1.,1.),(1.,1.),(1.,1.),(1.,1.),(1.,1.),(1.,1.),(1.,1.),(1.,1.),(1.,
1.),(1.,1.),(1.,1.),(1.,1.),(1.,1.),(1.,1.),(1.,1.),(1.,1.),(1.,1.),(1.,
1.),(1.,1.),(1.,1.),(1.,1.),(1.,1.),(1.,1.),(1.,1.),(1.,1.),(1.,1.),(1.,
1.),(1.,1.),(1.,1.),(1.,1.),(1.,1.),(1.,1.),(1.,1.),(1.,1.),(1.,1.),(1.,
1.),(1.,1.),(1.,1.),(1.,1.),(1.,1.),(1.,1.),(1.,1.),(1.,1.),(1.,1.),(1.,
1.),(1.,1.),(1.,1.),(1.,1.),(1.,1.),(1.,1.),(1.,1.),(1.,1.),(1.,1.),(1.,
1.),(1.,1.),(1.,1.),(1.,1.),(1.,1.),(1.,1.),(1.,1.),(1.,1.),(1.,1.),(1.,
1.),(1.,1.),(1.,1.),(1.,1.),(1.,1.),(1.,1.),(1.,1.),(1.,1.),(1.,1.),(1.,
1.),(1.,1.),(1.,1.),(1.,1.),(1.,1.),(1.,1.),(1.,1.),(1.,1.),(1.,1.),(1.,
1.),(1.,1.),(1.,1.),(1.,1.),(1.,1.),(1.,1.),(1.,1.),(1.,1.),(1.,1.),(1.,
1.),(1.,1.),(1.,1.),(1.,1.),(1.,1.),(1.,1.),(1.,1.),(1.,1.),(1.,1.),(1.,
1.),(1.,1.),(1.,1.),(1.,1.),(1.,1.),(1.,1.),(1.,1.),(1.,1.),(1.,1.),(1.,
1.),(1.,1.),(1.,1.),(1.,1.),(1.,1.),(1.,1.),(1.,1.),(1.,1.),(1.,1.),(1.,
1.),(1.,1.),(1.,1.),(1.,1.),(1.,1.),(1.,1.),(1.,1.),(1.,1.),(1.,1.),(1.,
1.),(1.,1.),(1.,1.),(1.,1.),(1.,1.),(1.,1.),(1.,1.),(1.,1.),(1.,1.),(1.,
1.),(1.,1.),(1.,1.),(1.,1.),(1.,1.),(1.,1.),(1.,1.),(1.,1.),(1.,1.),(1.,
1.),(1.,1.),(1.,1.),(1.,1.),(1.,1.),(1.,1.),(1.,1.),(1.,1.),(1.,1.),(1.,
1.),(1.,1.)))
REPRESENTATION_ITEM('')
SURFACE()
);
#962=(
BOUNDED_SURFACE()
B_SPLINE_SURFACE(5,1,((#122600,#122601),(#122602,#122603),(#122604,#122605),
(#122606,#122607),(#122608,#122609),(#122610,#122611),(#122612,#122613),
(#122614,#122615),(#122616,#122617),(#122618,#122619),(#122620,#122621),
(#122622,#122623),(#122624,#122625),(#122626,#122627),(#122628,#122629),
(#122630,#122631),(#122632,#122633),(#122634,#122635),(#122636,#122637),
(#122638,#122639),(#122640,#122641),(#122642,#122643),(#122644,#122645),
(#122646,#122647),(#122648,#122649),(#122650,#122651),(#122652,#122653),
(#122654,#122655),(#122656,#122657),(#122658,#122659),(#122660,#122661),
(#122662,#122663),(#122664,#122665),(#122666,#122667),(#122668,#122669),
(#122670,#122671),(#122672,#122673),(#122674,#122675),(#122676,#122677),
(#122678,#122679),(#122680,#122681),(#122682,#122683),(#122684,#122685),
(#122686,#122687),(#122688,#122689),(#122690,#122691),(#122692,#122693),
(#122694,#122695),(#122696,#122697),(#122698,#122699),(#122700,#122701),
(#122702,#122703),(#122704,#122705),(#122706,#122707),(#122708,#122709),
(#122710,#122711),(#122712,#122713),(#122714,#122715),(#122716,#122717),
(#122718,#122719),(#122720,#122721),(#122722,#122723),(#122724,#122725),
(#122726,#122727),(#122728,#122729),(#122730,#122731),(#122732,#122733),
(#122734,#122735),(#122736,#122737),(#122738,#122739),(#122740,#122741),
(#122742,#122743),(#122744,#122745),(#122746,#122747),(#122748,#122749),
(#122750,#122751),(#122752,#122753),(#122754,#122755),(#122756,#122757),
(#122758,#122759),(#122760,#122761),(#122762,#122763),(#122764,#122765),
(#122766,#122767),(#122768,#122769),(#122770,#122771),(#122772,#122773),
(#122774,#122775),(#122776,#122777),(#122778,#122779),(#122780,#122781),
(#122782,#122783),(#122784,#122785),(#122786,#122787),(#122788,#122789),
(#122790,#122791),(#122792,#122793),(#122794,#122795),(#122796,#122797),
(#122798,#122799),(#122800,#122801),(#122802,#122803),(#122804,#122805),
(#122806,#122807),(#122808,#122809),(#122810,#122811),(#122812,#122813),
(#122814,#122815),(#122816,#122817),(#122818,#122819),(#122820,#122821),
(#122822,#122823),(#122824,#122825),(#122826,#122827),(#122828,#122829),
(#122830,#122831),(#122832,#122833),(#122834,#122835),(#122836,#122837),
(#122838,#122839),(#122840,#122841),(#122842,#122843),(#122844,#122845),
(#122846,#122847),(#122848,#122849),(#122850,#122851),(#122852,#122853),
(#122854,#122855),(#122856,#122857),(#122858,#122859),(#122860,#122861),
(#122862,#122863),(#122864,#122865),(#122866,#122867),(#122868,#122869),
(#122870,#122871),(#122872,#122873),(#122874,#122875),(#122876,#122877),
(#122878,#122879),(#122880,#122881),(#122882,#122883),(#122884,#122885),
(#122886,#122887),(#122888,#122889),(#122890,#122891),(#122892,#122893),
(#122894,#122895),(#122896,#122897),(#122898,#122899),(#122900,#122901),
(#122902,#122903),(#122904,#122905),(#122906,#122907),(#122908,#122909),
(#122910,#122911),(#122912,#122913),(#122914,#122915),(#122916,#122917),
(#122918,#122919),(#122920,#122921),(#122922,#122923),(#122924,#122925),
(#122926,#122927),(#122928,#122929),(#122930,#122931),(#122932,#122933),
(#122934,#122935),(#122936,#122937),(#122938,#122939),(#122940,#122941),
(#122942,#122943),(#122944,#122945),(#122946,#122947),(#122948,#122949),
(#122950,#122951),(#122952,#122953),(#122954,#122955),(#122956,#122957),
(#122958,#122959),(#122960,#122961),(#122962,#122963),(#122964,#122965),
(#122966,#122967),(#122968,#122969),(#122970,#122971),(#122972,#122973),
(#122974,#122975),(#122976,#122977),(#122978,#122979),(#122980,#122981),
(#122982,#122983),(#122984,#122985),(#122986,#122987),(#122988,#122989),
(#122990,#122991),(#122992,#122993),(#122994,#122995),(#122996,#122997),
(#122998,#122999),(#123000,#123001),(#123002,#123003),(#123004,#123005),
(#123006,#123007),(#123008,#123009)),.UNSPECIFIED.,.F.,.F.,.F.)
B_SPLINE_SURFACE_WITH_KNOTS((6,1,1,1,1,1,1,1,1,1,1,1,1,1,1,1,1,1,1,1,1,
1,1,1,1,1,1,1,1,1,1,1,1,1,1,1,1,1,1,1,1,1,1,1,1,1,1,1,1,1,1,1,1,1,1,1,1,
1,1,1,1,1,1,1,1,1,1,1,1,1,1,1,1,1,1,1,1,1,1,1,1,1,1,1,1,1,1,1,1,1,1,1,1,
1,1,1,1,1,1,1,1,1,1,1,1,1,1,1,1,1,1,1,1,1,1,1,1,1,1,1,1,1,1,1,1,1,1,1,1,
1,1,1,1,1,1,1,1,1,1,1,1,1,1,1,1,1,1,1,1,1,1,1,1,1,1,1,1,1,1,1,1,1,1,1,1,
1,1,1,1,1,1,1,1,1,1,1,1,1,1,1,1,1,1,1,1,1,1,1,1,1,1,1,1,1,1,1,1,1,1,1,6),
(2,2),(-1.,-0.995000000000001,-0.990000000000001,-0.985000000000001,-0.980000000000001,
-0.975000000000001,-0.970000000000001,-0.965000000000001,-0.960000000000001,
-0.955000000000001,-0.950000000000001,-0.945000000000001,-0.940000000000001,
-0.935000000000001,-0.930000000000001,-0.925000000000001,-0.920000000000001,
-0.915000000000001,-0.910000000000001,-0.905000000000001,-0.900000000000001,
-0.895000000000001,-0.890000000000001,-0.885000000000001,-0.880000000000001,
-0.875000000000001,-0.870000000000001,-0.865000000000001,-0.860000000000001,
-0.855000000000001,-0.850000000000001,-0.845000000000001,-0.840000000000001,
-0.835000000000001,-0.830000000000001,-0.825000000000001,-0.820000000000001,
-0.815000000000001,-0.810000000000001,-0.805000000000001,-0.800000000000001,
-0.795000000000001,-0.790000000000001,-0.785000000000001,-0.780000000000001,
-0.775000000000001,-0.770000000000001,-0.765000000000001,-0.760000000000001,
-0.755000000000001,-0.750000000000001,-0.745000000000001,-0.740000000000001,
-0.735000000000001,-0.730000000000001,-0.725000000000001,-0.720000000000001,
-0.715000000000001,-0.710000000000001,-0.705000000000001,-0.700000000000001,
-0.695000000000001,-0.690000000000001,-0.685,-0.68,-0.675,-0.67,-0.665,
-0.66,-0.655,-0.65,-0.645,-0.64,-0.635,-0.63,-0.625,-0.62,-0.615,-0.61,
-0.605,-0.6,-0.595,-0.59,-0.585,-0.58,-0.575,-0.57,-0.565,-0.56,-0.555,
-0.55,-0.545,-0.54,-0.535,-0.53,-0.525,-0.52,-0.515,-0.51,-0.505,-0.5,-0.495,
-0.49,-0.485,-0.48,-0.475,-0.47,-0.465,-0.46,-0.455,-0.45,-0.445,-0.44,
-0.435,-0.43,-0.425,-0.42,-0.415,-0.41,-0.405,-0.4,-0.395,-0.39,-0.385,
-0.38,-0.375,-0.37,-0.365,-0.36,-0.355,-0.35,-0.345,-0.34,-0.335,-0.33,
-0.325,-0.32,-0.315,-0.31,-0.305,-0.3,-0.295,-0.29,-0.285,-0.28,-0.275,
-0.27,-0.265,-0.26,-0.255,-0.25,-0.245,-0.24,-0.235,-0.23,-0.225,-0.22,
-0.215,-0.21,-0.205,-0.2,-0.195,-0.19,-0.185,-0.18,-0.175,-0.17,-0.165,
-0.16,-0.155,-0.15,-0.145,-0.14,-0.135,-0.13,-0.125,-0.12,-0.115,-0.11,
-0.105,-0.1,-0.095,-0.09,-0.085,-0.08,-0.075,-0.07,-0.065,-0.06,-0.055,
-0.05,-0.045,-0.04,-0.035,-0.03,-0.025,-0.02,-0.015,-0.01,-0.005,0.),(0.,
1.2),.UNSPECIFIED.)
GEOMETRIC_REPRESENTATION_ITEM()
RATIONAL_B_SPLINE_SURFACE(((1.,1.),(1.,1.),(1.,1.),(1.,1.),(1.,1.),(1.,
1.),(1.,1.),(1.,1.),(1.,1.),(1.,1.),(1.,1.),(1.,1.),(1.,1.),(1.,1.),(1.,
1.),(1.,1.),(1.,1.),(1.,1.),(1.,1.),(1.,1.),(1.,1.),(1.,1.),(1.,1.),(1.,
1.),(1.,1.),(1.,1.),(1.,1.),(1.,1.),(1.,1.),(1.,1.),(1.,1.),(1.,1.),(1.,
1.),(1.,1.),(1.,1.),(1.,1.),(1.,1.),(1.,1.),(1.,1.),(1.,1.),(1.,1.),(1.,
1.),(1.,1.),(1.,1.),(1.,1.),(1.,1.),(1.,1.),(1.,1.),(1.,1.),(1.,1.),(1.,
1.),(1.,1.),(1.,1.),(1.,1.),(1.,1.),(1.,1.),(1.,1.),(1.,1.),(1.,1.),(1.,
1.),(1.,1.),(1.,1.),(1.,1.),(1.,1.),(1.,1.),(1.,1.),(1.,1.),(1.,1.),(1.,
1.),(1.,1.),(1.,1.),(1.,1.),(1.,1.),(1.,1.),(1.,1.),(1.,1.),(1.,1.),(1.,
1.),(1.,1.),(1.,1.),(1.,1.),(1.,1.),(1.,1.),(1.,1.),(1.,1.),(1.,1.),(1.,
1.),(1.,1.),(1.,1.),(1.,1.),(1.,1.),(1.,1.),(1.,1.),(1.,1.),(1.,1.),(1.,
1.),(1.,1.),(1.,1.),(1.,1.),(1.,1.),(1.,1.),(1.,1.),(1.,1.),(1.,1.),(1.,
1.),(1.,1.),(1.,1.),(1.,1.),(1.,1.),(1.,1.),(1.,1.),(1.,1.),(1.,1.),(1.,
1.),(1.,1.),(1.,1.),(1.,1.),(1.,1.),(1.,1.),(1.,1.),(1.,1.),(1.,1.),(1.,
1.),(1.,1.),(1.,1.),(1.,1.),(1.,1.),(1.,1.),(1.,1.),(1.,1.),(1.,1.),(1.,
1.),(1.,1.),(1.,1.),(1.,1.),(1.,1.),(1.,1.),(1.,1.),(1.,1.),(1.,1.),(1.,
1.),(1.,1.),(1.,1.),(1.,1.),(1.,1.),(1.,1.),(1.,1.),(1.,1.),(1.,1.),(1.,
1.),(1.,1.),(1.,1.),(1.,1.),(1.,1.),(1.,1.),(1.,1.),(1.,1.),(1.,1.),(1.,
1.),(1.,1.),(1.,1.),(1.,1.),(1.,1.),(1.,1.),(1.,1.),(1.,1.),(1.,1.),(1.,
1.),(1.,1.),(1.,1.),(1.,1.),(1.,1.),(1.,1.),(1.,1.),(1.,1.),(1.,1.),(1.,
1.),(1.,1.),(1.,1.),(1.,1.),(1.,1.),(1.,1.),(1.,1.),(1.,1.),(1.,1.),(1.,
1.),(1.,1.),(1.,1.),(1.,1.),(1.,1.),(1.,1.),(1.,1.),(1.,1.),(1.,1.),(1.,
1.),(1.,1.),(1.,1.),(1.,1.),(1.,1.),(1.,1.),(1.,1.),(1.,1.),(1.,1.),(1.,
1.),(1.,1.)))
REPRESENTATION_ITEM('')
SURFACE()
);
#963=(
BOUNDED_SURFACE()
B_SPLINE_SURFACE(5,1,((#123401,#123402),(#123403,#123404),(#123405,#123406),
(#123407,#123408),(#123409,#123410),(#123411,#123412),(#123413,#123414),
(#123415,#123416),(#123417,#123418),(#123419,#123420),(#123421,#123422),
(#123423,#123424),(#123425,#123426),(#123427,#123428),(#123429,#123430),
(#123431,#123432),(#123433,#123434),(#123435,#123436),(#123437,#123438),
(#123439,#123440),(#123441,#123442),(#123443,#123444),(#123445,#123446),
(#123447,#123448),(#123449,#123450),(#123451,#123452),(#123453,#123454),
(#123455,#123456),(#123457,#123458),(#123459,#123460),(#123461,#123462),
(#123463,#123464),(#123465,#123466),(#123467,#123468),(#123469,#123470),
(#123471,#123472),(#123473,#123474),(#123475,#123476),(#123477,#123478),
(#123479,#123480),(#123481,#123482),(#123483,#123484),(#123485,#123486),
(#123487,#123488),(#123489,#123490),(#123491,#123492),(#123493,#123494),
(#123495,#123496),(#123497,#123498),(#123499,#123500),(#123501,#123502),
(#123503,#123504),(#123505,#123506),(#123507,#123508),(#123509,#123510),
(#123511,#123512),(#123513,#123514),(#123515,#123516),(#123517,#123518),
(#123519,#123520),(#123521,#123522),(#123523,#123524),(#123525,#123526),
(#123527,#123528),(#123529,#123530),(#123531,#123532),(#123533,#123534),
(#123535,#123536),(#123537,#123538),(#123539,#123540),(#123541,#123542),
(#123543,#123544),(#123545,#123546),(#123547,#123548),(#123549,#123550),
(#123551,#123552),(#123553,#123554),(#123555,#123556),(#123557,#123558),
(#123559,#123560),(#123561,#123562),(#123563,#123564),(#123565,#123566),
(#123567,#123568),(#123569,#123570),(#123571,#123572),(#123573,#123574),
(#123575,#123576),(#123577,#123578),(#123579,#123580),(#123581,#123582),
(#123583,#123584),(#123585,#123586),(#123587,#123588),(#123589,#123590),
(#123591,#123592),(#123593,#123594),(#123595,#123596),(#123597,#123598),
(#123599,#123600),(#123601,#123602),(#123603,#123604),(#123605,#123606),
(#123607,#123608),(#123609,#123610),(#123611,#123612),(#123613,#123614),
(#123615,#123616),(#123617,#123618),(#123619,#123620),(#123621,#123622),
(#123623,#123624),(#123625,#123626),(#123627,#123628),(#123629,#123630),
(#123631,#123632),(#123633,#123634),(#123635,#123636),(#123637,#123638),
(#123639,#123640),(#123641,#123642),(#123643,#123644),(#123645,#123646),
(#123647,#123648),(#123649,#123650),(#123651,#123652),(#123653,#123654),
(#123655,#123656),(#123657,#123658),(#123659,#123660),(#123661,#123662),
(#123663,#123664),(#123665,#123666),(#123667,#123668),(#123669,#123670),
(#123671,#123672),(#123673,#123674),(#123675,#123676),(#123677,#123678),
(#123679,#123680),(#123681,#123682),(#123683,#123684),(#123685,#123686),
(#123687,#123688),(#123689,#123690),(#123691,#123692),(#123693,#123694),
(#123695,#123696),(#123697,#123698),(#123699,#123700),(#123701,#123702),
(#123703,#123704),(#123705,#123706),(#123707,#123708),(#123709,#123710),
(#123711,#123712),(#123713,#123714),(#123715,#123716),(#123717,#123718),
(#123719,#123720),(#123721,#123722),(#123723,#123724),(#123725,#123726),
(#123727,#123728),(#123729,#123730),(#123731,#123732),(#123733,#123734),
(#123735,#123736),(#123737,#123738),(#123739,#123740),(#123741,#123742),
(#123743,#123744),(#123745,#123746),(#123747,#123748),(#123749,#123750),
(#123751,#123752),(#123753,#123754),(#123755,#123756),(#123757,#123758),
(#123759,#123760),(#123761,#123762),(#123763,#123764),(#123765,#123766),
(#123767,#123768),(#123769,#123770),(#123771,#123772),(#123773,#123774),
(#123775,#123776),(#123777,#123778),(#123779,#123780),(#123781,#123782),
(#123783,#123784),(#123785,#123786),(#123787,#123788),(#123789,#123790),
(#123791,#123792),(#123793,#123794),(#123795,#123796),(#123797,#123798),
(#123799,#123800),(#123801,#123802),(#123803,#123804),(#123805,#123806),
(#123807,#123808),(#123809,#123810)),.UNSPECIFIED.,.F.,.F.,.F.)
B_SPLINE_SURFACE_WITH_KNOTS((6,1,1,1,1,1,1,1,1,1,1,1,1,1,1,1,1,1,1,1,1,
1,1,1,1,1,1,1,1,1,1,1,1,1,1,1,1,1,1,1,1,1,1,1,1,1,1,1,1,1,1,1,1,1,1,1,1,
1,1,1,1,1,1,1,1,1,1,1,1,1,1,1,1,1,1,1,1,1,1,1,1,1,1,1,1,1,1,1,1,1,1,1,1,
1,1,1,1,1,1,1,1,1,1,1,1,1,1,1,1,1,1,1,1,1,1,1,1,1,1,1,1,1,1,1,1,1,1,1,1,
1,1,1,1,1,1,1,1,1,1,1,1,1,1,1,1,1,1,1,1,1,1,1,1,1,1,1,1,1,1,1,1,1,1,1,1,
1,1,1,1,1,1,1,1,1,1,1,1,1,1,1,1,1,1,1,1,1,1,1,1,1,1,1,1,1,1,1,1,1,1,1,6),
(2,2),(-1.,-0.995000000000001,-0.990000000000001,-0.985000000000001,-0.980000000000001,
-0.975000000000001,-0.970000000000001,-0.965000000000001,-0.960000000000001,
-0.955000000000001,-0.950000000000001,-0.945000000000001,-0.940000000000001,
-0.935000000000001,-0.930000000000001,-0.925000000000001,-0.920000000000001,
-0.915000000000001,-0.910000000000001,-0.905000000000001,-0.900000000000001,
-0.895000000000001,-0.890000000000001,-0.885000000000001,-0.880000000000001,
-0.875000000000001,-0.870000000000001,-0.865000000000001,-0.860000000000001,
-0.855000000000001,-0.850000000000001,-0.845000000000001,-0.840000000000001,
-0.835000000000001,-0.830000000000001,-0.825000000000001,-0.820000000000001,
-0.815000000000001,-0.810000000000001,-0.805000000000001,-0.800000000000001,
-0.795000000000001,-0.790000000000001,-0.785000000000001,-0.780000000000001,
-0.775000000000001,-0.770000000000001,-0.765000000000001,-0.760000000000001,
-0.755000000000001,-0.750000000000001,-0.745000000000001,-0.740000000000001,
-0.735000000000001,-0.730000000000001,-0.725000000000001,-0.720000000000001,
-0.715000000000001,-0.710000000000001,-0.705000000000001,-0.700000000000001,
-0.695000000000001,-0.690000000000001,-0.685,-0.68,-0.675,-0.67,-0.665,
-0.66,-0.655,-0.65,-0.645,-0.64,-0.635,-0.63,-0.625,-0.62,-0.615,-0.61,
-0.605,-0.6,-0.595,-0.59,-0.585,-0.58,-0.575,-0.57,-0.565,-0.56,-0.555,
-0.55,-0.545,-0.54,-0.535,-0.53,-0.525,-0.52,-0.515,-0.51,-0.505,-0.5,-0.495,
-0.49,-0.485,-0.48,-0.475,-0.47,-0.465,-0.46,-0.455,-0.45,-0.445,-0.44,
-0.435,-0.43,-0.425,-0.42,-0.415,-0.41,-0.405,-0.4,-0.395,-0.39,-0.385,
-0.38,-0.375,-0.37,-0.365,-0.36,-0.355,-0.35,-0.345,-0.34,-0.335,-0.33,
-0.325,-0.32,-0.315,-0.31,-0.305,-0.3,-0.295,-0.29,-0.285,-0.28,-0.275,
-0.27,-0.265,-0.26,-0.255,-0.25,-0.245,-0.24,-0.235,-0.23,-0.225,-0.22,
-0.215,-0.21,-0.205,-0.2,-0.195,-0.19,-0.185,-0.18,-0.175,-0.17,-0.165,
-0.16,-0.155,-0.15,-0.145,-0.14,-0.135,-0.13,-0.125,-0.12,-0.115,-0.11,
-0.105,-0.1,-0.095,-0.09,-0.085,-0.08,-0.075,-0.07,-0.065,-0.06,-0.055,
-0.05,-0.045,-0.04,-0.035,-0.03,-0.025,-0.02,-0.015,-0.01,-0.005,0.),(0.,
1.2),.UNSPECIFIED.)
GEOMETRIC_REPRESENTATION_ITEM()
RATIONAL_B_SPLINE_SURFACE(((1.,1.),(1.,1.),(1.,1.),(1.,1.),(1.,1.),(1.,
1.),(1.,1.),(1.,1.),(1.,1.),(1.,1.),(1.,1.),(1.,1.),(1.,1.),(1.,1.),(1.,
1.),(1.,1.),(1.,1.),(1.,1.),(1.,1.),(1.,1.),(1.,1.),(1.,1.),(1.,1.),(1.,
1.),(1.,1.),(1.,1.),(1.,1.),(1.,1.),(1.,1.),(1.,1.),(1.,1.),(1.,1.),(1.,
1.),(1.,1.),(1.,1.),(1.,1.),(1.,1.),(1.,1.),(1.,1.),(1.,1.),(1.,1.),(1.,
1.),(1.,1.),(1.,1.),(1.,1.),(1.,1.),(1.,1.),(1.,1.),(1.,1.),(1.,1.),(1.,
1.),(1.,1.),(1.,1.),(1.,1.),(1.,1.),(1.,1.),(1.,1.),(1.,1.),(1.,1.),(1.,
1.),(1.,1.),(1.,1.),(1.,1.),(1.,1.),(1.,1.),(1.,1.),(1.,1.),(1.,1.),(1.,
1.),(1.,1.),(1.,1.),(1.,1.),(1.,1.),(1.,1.),(1.,1.),(1.,1.),(1.,1.),(1.,
1.),(1.,1.),(1.,1.),(1.,1.),(1.,1.),(1.,1.),(1.,1.),(1.,1.),(1.,1.),(1.,
1.),(1.,1.),(1.,1.),(1.,1.),(1.,1.),(1.,1.),(1.,1.),(1.,1.),(1.,1.),(1.,
1.),(1.,1.),(1.,1.),(1.,1.),(1.,1.),(1.,1.),(1.,1.),(1.,1.),(1.,1.),(1.,
1.),(1.,1.),(1.,1.),(1.,1.),(1.,1.),(1.,1.),(1.,1.),(1.,1.),(1.,1.),(1.,
1.),(1.,1.),(1.,1.),(1.,1.),(1.,1.),(1.,1.),(1.,1.),(1.,1.),(1.,1.),(1.,
1.),(1.,1.),(1.,1.),(1.,1.),(1.,1.),(1.,1.),(1.,1.),(1.,1.),(1.,1.),(1.,
1.),(1.,1.),(1.,1.),(1.,1.),(1.,1.),(1.,1.),(1.,1.),(1.,1.),(1.,1.),(1.,
1.),(1.,1.),(1.,1.),(1.,1.),(1.,1.),(1.,1.),(1.,1.),(1.,1.),(1.,1.),(1.,
1.),(1.,1.),(1.,1.),(1.,1.),(1.,1.),(1.,1.),(1.,1.),(1.,1.),(1.,1.),(1.,
1.),(1.,1.),(1.,1.),(1.,1.),(1.,1.),(1.,1.),(1.,1.),(1.,1.),(1.,1.),(1.,
1.),(1.,1.),(1.,1.),(1.,1.),(1.,1.),(1.,1.),(1.,1.),(1.,1.),(1.,1.),(1.,
1.),(1.,1.),(1.,1.),(1.,1.),(1.,1.),(1.,1.),(1.,1.),(1.,1.),(1.,1.),(1.,
1.),(1.,1.),(1.,1.),(1.,1.),(1.,1.),(1.,1.),(1.,1.),(1.,1.),(1.,1.),(1.,
1.),(1.,1.),(1.,1.),(1.,1.),(1.,1.),(1.,1.),(1.,1.),(1.,1.),(1.,1.),(1.,
1.),(1.,1.)))
REPRESENTATION_ITEM('')
SURFACE()
);
#964=(
BOUNDED_SURFACE()
B_SPLINE_SURFACE(5,1,((#124202,#124203),(#124204,#124205),(#124206,#124207),
(#124208,#124209),(#124210,#124211),(#124212,#124213),(#124214,#124215),
(#124216,#124217),(#124218,#124219),(#124220,#124221),(#124222,#124223),
(#124224,#124225),(#124226,#124227),(#124228,#124229),(#124230,#124231),
(#124232,#124233),(#124234,#124235),(#124236,#124237),(#124238,#124239),
(#124240,#124241),(#124242,#124243),(#124244,#124245),(#124246,#124247),
(#124248,#124249),(#124250,#124251),(#124252,#124253),(#124254,#124255),
(#124256,#124257),(#124258,#124259),(#124260,#124261),(#124262,#124263),
(#124264,#124265),(#124266,#124267),(#124268,#124269),(#124270,#124271),
(#124272,#124273),(#124274,#124275),(#124276,#124277),(#124278,#124279),
(#124280,#124281),(#124282,#124283),(#124284,#124285),(#124286,#124287),
(#124288,#124289),(#124290,#124291),(#124292,#124293),(#124294,#124295),
(#124296,#124297),(#124298,#124299),(#124300,#124301),(#124302,#124303),
(#124304,#124305),(#124306,#124307),(#124308,#124309),(#124310,#124311),
(#124312,#124313),(#124314,#124315),(#124316,#124317),(#124318,#124319),
(#124320,#124321),(#124322,#124323),(#124324,#124325),(#124326,#124327),
(#124328,#124329),(#124330,#124331),(#124332,#124333),(#124334,#124335),
(#124336,#124337),(#124338,#124339),(#124340,#124341),(#124342,#124343),
(#124344,#124345),(#124346,#124347),(#124348,#124349),(#124350,#124351),
(#124352,#124353),(#124354,#124355),(#124356,#124357),(#124358,#124359),
(#124360,#124361),(#124362,#124363),(#124364,#124365),(#124366,#124367),
(#124368,#124369),(#124370,#124371),(#124372,#124373),(#124374,#124375),
(#124376,#124377),(#124378,#124379),(#124380,#124381),(#124382,#124383),
(#124384,#124385),(#124386,#124387),(#124388,#124389),(#124390,#124391),
(#124392,#124393),(#124394,#124395),(#124396,#124397),(#124398,#124399),
(#124400,#124401),(#124402,#124403),(#124404,#124405),(#124406,#124407),
(#124408,#124409),(#124410,#124411),(#124412,#124413),(#124414,#124415),
(#124416,#124417),(#124418,#124419),(#124420,#124421),(#124422,#124423),
(#124424,#124425),(#124426,#124427),(#124428,#124429),(#124430,#124431),
(#124432,#124433),(#124434,#124435),(#124436,#124437),(#124438,#124439),
(#124440,#124441),(#124442,#124443),(#124444,#124445),(#124446,#124447),
(#124448,#124449),(#124450,#124451),(#124452,#124453),(#124454,#124455),
(#124456,#124457),(#124458,#124459),(#124460,#124461),(#124462,#124463),
(#124464,#124465),(#124466,#124467),(#124468,#124469),(#124470,#124471),
(#124472,#124473),(#124474,#124475),(#124476,#124477),(#124478,#124479),
(#124480,#124481),(#124482,#124483),(#124484,#124485),(#124486,#124487),
(#124488,#124489),(#124490,#124491),(#124492,#124493),(#124494,#124495),
(#124496,#124497),(#124498,#124499),(#124500,#124501),(#124502,#124503),
(#124504,#124505),(#124506,#124507),(#124508,#124509),(#124510,#124511),
(#124512,#124513),(#124514,#124515),(#124516,#124517),(#124518,#124519),
(#124520,#124521),(#124522,#124523),(#124524,#124525),(#124526,#124527),
(#124528,#124529),(#124530,#124531),(#124532,#124533),(#124534,#124535),
(#124536,#124537),(#124538,#124539),(#124540,#124541),(#124542,#124543),
(#124544,#124545),(#124546,#124547),(#124548,#124549),(#124550,#124551),
(#124552,#124553),(#124554,#124555),(#124556,#124557),(#124558,#124559),
(#124560,#124561),(#124562,#124563),(#124564,#124565),(#124566,#124567),
(#124568,#124569),(#124570,#124571),(#124572,#124573),(#124574,#124575),
(#124576,#124577),(#124578,#124579),(#124580,#124581),(#124582,#124583),
(#124584,#124585),(#124586,#124587),(#124588,#124589),(#124590,#124591),
(#124592,#124593),(#124594,#124595),(#124596,#124597),(#124598,#124599),
(#124600,#124601),(#124602,#124603),(#124604,#124605),(#124606,#124607),
(#124608,#124609),(#124610,#124611)),.UNSPECIFIED.,.F.,.F.,.F.)
B_SPLINE_SURFACE_WITH_KNOTS((6,1,1,1,1,1,1,1,1,1,1,1,1,1,1,1,1,1,1,1,1,
1,1,1,1,1,1,1,1,1,1,1,1,1,1,1,1,1,1,1,1,1,1,1,1,1,1,1,1,1,1,1,1,1,1,1,1,
1,1,1,1,1,1,1,1,1,1,1,1,1,1,1,1,1,1,1,1,1,1,1,1,1,1,1,1,1,1,1,1,1,1,1,1,
1,1,1,1,1,1,1,1,1,1,1,1,1,1,1,1,1,1,1,1,1,1,1,1,1,1,1,1,1,1,1,1,1,1,1,1,
1,1,1,1,1,1,1,1,1,1,1,1,1,1,1,1,1,1,1,1,1,1,1,1,1,1,1,1,1,1,1,1,1,1,1,1,
1,1,1,1,1,1,1,1,1,1,1,1,1,1,1,1,1,1,1,1,1,1,1,1,1,1,1,1,1,1,1,1,1,1,1,6),
(2,2),(-1.,-0.995000000000001,-0.990000000000001,-0.985000000000001,-0.980000000000001,
-0.975000000000001,-0.970000000000001,-0.965000000000001,-0.960000000000001,
-0.955000000000001,-0.950000000000001,-0.945000000000001,-0.940000000000001,
-0.935000000000001,-0.930000000000001,-0.925000000000001,-0.920000000000001,
-0.915000000000001,-0.910000000000001,-0.905000000000001,-0.900000000000001,
-0.895000000000001,-0.890000000000001,-0.885000000000001,-0.880000000000001,
-0.875000000000001,-0.870000000000001,-0.865000000000001,-0.860000000000001,
-0.855000000000001,-0.850000000000001,-0.845000000000001,-0.840000000000001,
-0.835000000000001,-0.830000000000001,-0.825000000000001,-0.820000000000001,
-0.815000000000001,-0.810000000000001,-0.805000000000001,-0.800000000000001,
-0.795000000000001,-0.790000000000001,-0.785000000000001,-0.780000000000001,
-0.775000000000001,-0.770000000000001,-0.765000000000001,-0.760000000000001,
-0.755000000000001,-0.750000000000001,-0.745000000000001,-0.740000000000001,
-0.735000000000001,-0.730000000000001,-0.725000000000001,-0.720000000000001,
-0.715000000000001,-0.710000000000001,-0.705000000000001,-0.700000000000001,
-0.695000000000001,-0.690000000000001,-0.685,-0.68,-0.675,-0.67,-0.665,
-0.66,-0.655,-0.65,-0.645,-0.64,-0.635,-0.63,-0.625,-0.62,-0.615,-0.61,
-0.605,-0.6,-0.595,-0.59,-0.585,-0.58,-0.575,-0.57,-0.565,-0.56,-0.555,
-0.55,-0.545,-0.54,-0.535,-0.53,-0.525,-0.52,-0.515,-0.51,-0.505,-0.5,-0.495,
-0.49,-0.485,-0.48,-0.475,-0.47,-0.465,-0.46,-0.455,-0.45,-0.445,-0.44,
-0.435,-0.43,-0.425,-0.42,-0.415,-0.41,-0.405,-0.4,-0.395,-0.39,-0.385,
-0.38,-0.375,-0.37,-0.365,-0.36,-0.355,-0.35,-0.345,-0.34,-0.335,-0.33,
-0.325,-0.32,-0.315,-0.31,-0.305,-0.3,-0.295,-0.29,-0.285,-0.28,-0.275,
-0.27,-0.265,-0.26,-0.255,-0.25,-0.245,-0.24,-0.235,-0.23,-0.225,-0.22,
-0.215,-0.21,-0.205,-0.2,-0.195,-0.19,-0.185,-0.18,-0.175,-0.17,-0.165,
-0.16,-0.155,-0.15,-0.145,-0.14,-0.135,-0.13,-0.125,-0.12,-0.115,-0.11,
-0.105,-0.1,-0.095,-0.09,-0.085,-0.08,-0.075,-0.07,-0.065,-0.06,-0.055,
-0.05,-0.045,-0.04,-0.035,-0.03,-0.025,-0.02,-0.015,-0.01,-0.005,0.),(0.,
1.2),.UNSPECIFIED.)
GEOMETRIC_REPRESENTATION_ITEM()
RATIONAL_B_SPLINE_SURFACE(((1.,1.),(1.,1.),(1.,1.),(1.,1.),(1.,1.),(1.,
1.),(1.,1.),(1.,1.),(1.,1.),(1.,1.),(1.,1.),(1.,1.),(1.,1.),(1.,1.),(1.,
1.),(1.,1.),(1.,1.),(1.,1.),(1.,1.),(1.,1.),(1.,1.),(1.,1.),(1.,1.),(1.,
1.),(1.,1.),(1.,1.),(1.,1.),(1.,1.),(1.,1.),(1.,1.),(1.,1.),(1.,1.),(1.,
1.),(1.,1.),(1.,1.),(1.,1.),(1.,1.),(1.,1.),(1.,1.),(1.,1.),(1.,1.),(1.,
1.),(1.,1.),(1.,1.),(1.,1.),(1.,1.),(1.,1.),(1.,1.),(1.,1.),(1.,1.),(1.,
1.),(1.,1.),(1.,1.),(1.,1.),(1.,1.),(1.,1.),(1.,1.),(1.,1.),(1.,1.),(1.,
1.),(1.,1.),(1.,1.),(1.,1.),(1.,1.),(1.,1.),(1.,1.),(1.,1.),(1.,1.),(1.,
1.),(1.,1.),(1.,1.),(1.,1.),(1.,1.),(1.,1.),(1.,1.),(1.,1.),(1.,1.),(1.,
1.),(1.,1.),(1.,1.),(1.,1.),(1.,1.),(1.,1.),(1.,1.),(1.,1.),(1.,1.),(1.,
1.),(1.,1.),(1.,1.),(1.,1.),(1.,1.),(1.,1.),(1.,1.),(1.,1.),(1.,1.),(1.,
1.),(1.,1.),(1.,1.),(1.,1.),(1.,1.),(1.,1.),(1.,1.),(1.,1.),(1.,1.),(1.,
1.),(1.,1.),(1.,1.),(1.,1.),(1.,1.),(1.,1.),(1.,1.),(1.,1.),(1.,1.),(1.,
1.),(1.,1.),(1.,1.),(1.,1.),(1.,1.),(1.,1.),(1.,1.),(1.,1.),(1.,1.),(1.,
1.),(1.,1.),(1.,1.),(1.,1.),(1.,1.),(1.,1.),(1.,1.),(1.,1.),(1.,1.),(1.,
1.),(1.,1.),(1.,1.),(1.,1.),(1.,1.),(1.,1.),(1.,1.),(1.,1.),(1.,1.),(1.,
1.),(1.,1.),(1.,1.),(1.,1.),(1.,1.),(1.,1.),(1.,1.),(1.,1.),(1.,1.),(1.,
1.),(1.,1.),(1.,1.),(1.,1.),(1.,1.),(1.,1.),(1.,1.),(1.,1.),(1.,1.),(1.,
1.),(1.,1.),(1.,1.),(1.,1.),(1.,1.),(1.,1.),(1.,1.),(1.,1.),(1.,1.),(1.,
1.),(1.,1.),(1.,1.),(1.,1.),(1.,1.),(1.,1.),(1.,1.),(1.,1.),(1.,1.),(1.,
1.),(1.,1.),(1.,1.),(1.,1.),(1.,1.),(1.,1.),(1.,1.),(1.,1.),(1.,1.),(1.,
1.),(1.,1.),(1.,1.),(1.,1.),(1.,1.),(1.,1.),(1.,1.),(1.,1.),(1.,1.),(1.,
1.),(1.,1.),(1.,1.),(1.,1.),(1.,1.),(1.,1.),(1.,1.),(1.,1.),(1.,1.),(1.,
1.),(1.,1.)))
REPRESENTATION_ITEM('')
SURFACE()
);
#965=(
BOUNDED_SURFACE()
B_SPLINE_SURFACE(5,1,((#125003,#125004),(#125005,#125006),(#125007,#125008),
(#125009,#125010),(#125011,#125012),(#125013,#125014),(#125015,#125016),
(#125017,#125018),(#125019,#125020),(#125021,#125022),(#125023,#125024),
(#125025,#125026),(#125027,#125028),(#125029,#125030),(#125031,#125032),
(#125033,#125034),(#125035,#125036),(#125037,#125038),(#125039,#125040),
(#125041,#125042),(#125043,#125044),(#125045,#125046),(#125047,#125048),
(#125049,#125050),(#125051,#125052),(#125053,#125054),(#125055,#125056),
(#125057,#125058),(#125059,#125060),(#125061,#125062),(#125063,#125064),
(#125065,#125066),(#125067,#125068),(#125069,#125070),(#125071,#125072),
(#125073,#125074),(#125075,#125076),(#125077,#125078),(#125079,#125080),
(#125081,#125082),(#125083,#125084),(#125085,#125086),(#125087,#125088),
(#125089,#125090),(#125091,#125092),(#125093,#125094),(#125095,#125096),
(#125097,#125098),(#125099,#125100),(#125101,#125102),(#125103,#125104),
(#125105,#125106),(#125107,#125108),(#125109,#125110),(#125111,#125112),
(#125113,#125114),(#125115,#125116),(#125117,#125118),(#125119,#125120),
(#125121,#125122),(#125123,#125124),(#125125,#125126),(#125127,#125128),
(#125129,#125130),(#125131,#125132),(#125133,#125134),(#125135,#125136),
(#125137,#125138),(#125139,#125140),(#125141,#125142),(#125143,#125144),
(#125145,#125146),(#125147,#125148),(#125149,#125150),(#125151,#125152),
(#125153,#125154),(#125155,#125156),(#125157,#125158),(#125159,#125160),
(#125161,#125162),(#125163,#125164),(#125165,#125166),(#125167,#125168),
(#125169,#125170),(#125171,#125172),(#125173,#125174),(#125175,#125176),
(#125177,#125178),(#125179,#125180),(#125181,#125182),(#125183,#125184),
(#125185,#125186),(#125187,#125188),(#125189,#125190),(#125191,#125192),
(#125193,#125194),(#125195,#125196),(#125197,#125198),(#125199,#125200),
(#125201,#125202),(#125203,#125204),(#125205,#125206),(#125207,#125208),
(#125209,#125210),(#125211,#125212),(#125213,#125214),(#125215,#125216),
(#125217,#125218),(#125219,#125220),(#125221,#125222),(#125223,#125224),
(#125225,#125226),(#125227,#125228),(#125229,#125230),(#125231,#125232),
(#125233,#125234),(#125235,#125236),(#125237,#125238),(#125239,#125240),
(#125241,#125242),(#125243,#125244),(#125245,#125246),(#125247,#125248),
(#125249,#125250),(#125251,#125252),(#125253,#125254),(#125255,#125256),
(#125257,#125258),(#125259,#125260),(#125261,#125262),(#125263,#125264),
(#125265,#125266),(#125267,#125268),(#125269,#125270),(#125271,#125272),
(#125273,#125274),(#125275,#125276),(#125277,#125278),(#125279,#125280),
(#125281,#125282),(#125283,#125284),(#125285,#125286),(#125287,#125288),
(#125289,#125290),(#125291,#125292),(#125293,#125294),(#125295,#125296),
(#125297,#125298),(#125299,#125300),(#125301,#125302),(#125303,#125304),
(#125305,#125306),(#125307,#125308),(#125309,#125310),(#125311,#125312),
(#125313,#125314),(#125315,#125316),(#125317,#125318),(#125319,#125320),
(#125321,#125322),(#125323,#125324),(#125325,#125326),(#125327,#125328),
(#125329,#125330),(#125331,#125332),(#125333,#125334),(#125335,#125336),
(#125337,#125338),(#125339,#125340),(#125341,#125342),(#125343,#125344),
(#125345,#125346),(#125347,#125348),(#125349,#125350),(#125351,#125352),
(#125353,#125354),(#125355,#125356),(#125357,#125358),(#125359,#125360),
(#125361,#125362),(#125363,#125364),(#125365,#125366),(#125367,#125368),
(#125369,#125370),(#125371,#125372),(#125373,#125374),(#125375,#125376),
(#125377,#125378),(#125379,#125380),(#125381,#125382),(#125383,#125384),
(#125385,#125386),(#125387,#125388),(#125389,#125390),(#125391,#125392),
(#125393,#125394),(#125395,#125396),(#125397,#125398),(#125399,#125400),
(#125401,#125402),(#125403,#125404),(#125405,#125406),(#125407,#125408),
(#125409,#125410),(#125411,#125412)),.UNSPECIFIED.,.F.,.F.,.F.)
B_SPLINE_SURFACE_WITH_KNOTS((6,1,1,1,1,1,1,1,1,1,1,1,1,1,1,1,1,1,1,1,1,
1,1,1,1,1,1,1,1,1,1,1,1,1,1,1,1,1,1,1,1,1,1,1,1,1,1,1,1,1,1,1,1,1,1,1,1,
1,1,1,1,1,1,1,1,1,1,1,1,1,1,1,1,1,1,1,1,1,1,1,1,1,1,1,1,1,1,1,1,1,1,1,1,
1,1,1,1,1,1,1,1,1,1,1,1,1,1,1,1,1,1,1,1,1,1,1,1,1,1,1,1,1,1,1,1,1,1,1,1,
1,1,1,1,1,1,1,1,1,1,1,1,1,1,1,1,1,1,1,1,1,1,1,1,1,1,1,1,1,1,1,1,1,1,1,1,
1,1,1,1,1,1,1,1,1,1,1,1,1,1,1,1,1,1,1,1,1,1,1,1,1,1,1,1,1,1,1,1,1,1,1,6),
(2,2),(-1.,-0.995000000000001,-0.990000000000001,-0.985000000000001,-0.980000000000001,
-0.975000000000001,-0.970000000000001,-0.965000000000001,-0.960000000000001,
-0.955000000000001,-0.950000000000001,-0.945000000000001,-0.940000000000001,
-0.935000000000001,-0.930000000000001,-0.925000000000001,-0.920000000000001,
-0.915000000000001,-0.910000000000001,-0.905000000000001,-0.900000000000001,
-0.895000000000001,-0.890000000000001,-0.885000000000001,-0.880000000000001,
-0.875000000000001,-0.870000000000001,-0.865000000000001,-0.860000000000001,
-0.855000000000001,-0.850000000000001,-0.845000000000001,-0.840000000000001,
-0.835000000000001,-0.830000000000001,-0.825000000000001,-0.820000000000001,
-0.815000000000001,-0.810000000000001,-0.805000000000001,-0.800000000000001,
-0.795000000000001,-0.790000000000001,-0.785000000000001,-0.780000000000001,
-0.775000000000001,-0.770000000000001,-0.765000000000001,-0.760000000000001,
-0.755000000000001,-0.750000000000001,-0.745000000000001,-0.740000000000001,
-0.735000000000001,-0.730000000000001,-0.725000000000001,-0.720000000000001,
-0.715000000000001,-0.710000000000001,-0.705000000000001,-0.700000000000001,
-0.695000000000001,-0.690000000000001,-0.685,-0.68,-0.675,-0.67,-0.665,
-0.66,-0.655,-0.65,-0.645,-0.64,-0.635,-0.63,-0.625,-0.62,-0.615,-0.61,
-0.605,-0.6,-0.595,-0.59,-0.585,-0.58,-0.575,-0.57,-0.565,-0.56,-0.555,
-0.55,-0.545,-0.54,-0.535,-0.53,-0.525,-0.52,-0.515,-0.51,-0.505,-0.5,-0.495,
-0.49,-0.485,-0.48,-0.475,-0.47,-0.465,-0.46,-0.455,-0.45,-0.445,-0.44,
-0.435,-0.43,-0.425,-0.42,-0.415,-0.41,-0.405,-0.4,-0.395,-0.39,-0.385,
-0.38,-0.375,-0.37,-0.365,-0.36,-0.355,-0.35,-0.345,-0.34,-0.335,-0.33,
-0.325,-0.32,-0.315,-0.31,-0.305,-0.3,-0.295,-0.29,-0.285,-0.28,-0.275,
-0.27,-0.265,-0.26,-0.255,-0.25,-0.245,-0.24,-0.235,-0.23,-0.225,-0.22,
-0.215,-0.21,-0.205,-0.2,-0.195,-0.19,-0.185,-0.18,-0.175,-0.17,-0.165,
-0.16,-0.155,-0.15,-0.145,-0.14,-0.135,-0.13,-0.125,-0.12,-0.115,-0.11,
-0.105,-0.1,-0.095,-0.09,-0.085,-0.08,-0.075,-0.07,-0.065,-0.06,-0.055,
-0.05,-0.045,-0.04,-0.035,-0.03,-0.025,-0.02,-0.015,-0.01,-0.005,0.),(0.,
1.2),.UNSPECIFIED.)
GEOMETRIC_REPRESENTATION_ITEM()
RATIONAL_B_SPLINE_SURFACE(((1.,1.),(1.,1.),(1.,1.),(1.,1.),(1.,1.),(1.,
1.),(1.,1.),(1.,1.),(1.,1.),(1.,1.),(1.,1.),(1.,1.),(1.,1.),(1.,1.),(1.,
1.),(1.,1.),(1.,1.),(1.,1.),(1.,1.),(1.,1.),(1.,1.),(1.,1.),(1.,1.),(1.,
1.),(1.,1.),(1.,1.),(1.,1.),(1.,1.),(1.,1.),(1.,1.),(1.,1.),(1.,1.),(1.,
1.),(1.,1.),(1.,1.),(1.,1.),(1.,1.),(1.,1.),(1.,1.),(1.,1.),(1.,1.),(1.,
1.),(1.,1.),(1.,1.),(1.,1.),(1.,1.),(1.,1.),(1.,1.),(1.,1.),(1.,1.),(1.,
1.),(1.,1.),(1.,1.),(1.,1.),(1.,1.),(1.,1.),(1.,1.),(1.,1.),(1.,1.),(1.,
1.),(1.,1.),(1.,1.),(1.,1.),(1.,1.),(1.,1.),(1.,1.),(1.,1.),(1.,1.),(1.,
1.),(1.,1.),(1.,1.),(1.,1.),(1.,1.),(1.,1.),(1.,1.),(1.,1.),(1.,1.),(1.,
1.),(1.,1.),(1.,1.),(1.,1.),(1.,1.),(1.,1.),(1.,1.),(1.,1.),(1.,1.),(1.,
1.),(1.,1.),(1.,1.),(1.,1.),(1.,1.),(1.,1.),(1.,1.),(1.,1.),(1.,1.),(1.,
1.),(1.,1.),(1.,1.),(1.,1.),(1.,1.),(1.,1.),(1.,1.),(1.,1.),(1.,1.),(1.,
1.),(1.,1.),(1.,1.),(1.,1.),(1.,1.),(1.,1.),(1.,1.),(1.,1.),(1.,1.),(1.,
1.),(1.,1.),(1.,1.),(1.,1.),(1.,1.),(1.,1.),(1.,1.),(1.,1.),(1.,1.),(1.,
1.),(1.,1.),(1.,1.),(1.,1.),(1.,1.),(1.,1.),(1.,1.),(1.,1.),(1.,1.),(1.,
1.),(1.,1.),(1.,1.),(1.,1.),(1.,1.),(1.,1.),(1.,1.),(1.,1.),(1.,1.),(1.,
1.),(1.,1.),(1.,1.),(1.,1.),(1.,1.),(1.,1.),(1.,1.),(1.,1.),(1.,1.),(1.,
1.),(1.,1.),(1.,1.),(1.,1.),(1.,1.),(1.,1.),(1.,1.),(1.,1.),(1.,1.),(1.,
1.),(1.,1.),(1.,1.),(1.,1.),(1.,1.),(1.,1.),(1.,1.),(1.,1.),(1.,1.),(1.,
1.),(1.,1.),(1.,1.),(1.,1.),(1.,1.),(1.,1.),(1.,1.),(1.,1.),(1.,1.),(1.,
1.),(1.,1.),(1.,1.),(1.,1.),(1.,1.),(1.,1.),(1.,1.),(1.,1.),(1.,1.),(1.,
1.),(1.,1.),(1.,1.),(1.,1.),(1.,1.),(1.,1.),(1.,1.),(1.,1.),(1.,1.),(1.,
1.),(1.,1.),(1.,1.),(1.,1.),(1.,1.),(1.,1.),(1.,1.),(1.,1.),(1.,1.),(1.,
1.),(1.,1.)))
REPRESENTATION_ITEM('')
SURFACE()
);
#966=(
BOUNDED_SURFACE()
B_SPLINE_SURFACE(5,1,((#125804,#125805),(#125806,#125807),(#125808,#125809),
(#125810,#125811),(#125812,#125813),(#125814,#125815),(#125816,#125817),
(#125818,#125819),(#125820,#125821),(#125822,#125823),(#125824,#125825),
(#125826,#125827),(#125828,#125829),(#125830,#125831),(#125832,#125833),
(#125834,#125835),(#125836,#125837),(#125838,#125839),(#125840,#125841),
(#125842,#125843),(#125844,#125845),(#125846,#125847),(#125848,#125849),
(#125850,#125851),(#125852,#125853),(#125854,#125855),(#125856,#125857),
(#125858,#125859),(#125860,#125861),(#125862,#125863),(#125864,#125865),
(#125866,#125867),(#125868,#125869),(#125870,#125871),(#125872,#125873),
(#125874,#125875),(#125876,#125877),(#125878,#125879),(#125880,#125881),
(#125882,#125883),(#125884,#125885),(#125886,#125887),(#125888,#125889),
(#125890,#125891),(#125892,#125893),(#125894,#125895),(#125896,#125897),
(#125898,#125899),(#125900,#125901),(#125902,#125903),(#125904,#125905),
(#125906,#125907),(#125908,#125909),(#125910,#125911),(#125912,#125913),
(#125914,#125915),(#125916,#125917),(#125918,#125919),(#125920,#125921),
(#125922,#125923),(#125924,#125925),(#125926,#125927),(#125928,#125929),
(#125930,#125931),(#125932,#125933),(#125934,#125935),(#125936,#125937),
(#125938,#125939),(#125940,#125941),(#125942,#125943),(#125944,#125945),
(#125946,#125947),(#125948,#125949),(#125950,#125951),(#125952,#125953),
(#125954,#125955),(#125956,#125957),(#125958,#125959),(#125960,#125961),
(#125962,#125963),(#125964,#125965),(#125966,#125967),(#125968,#125969),
(#125970,#125971),(#125972,#125973),(#125974,#125975),(#125976,#125977),
(#125978,#125979),(#125980,#125981),(#125982,#125983),(#125984,#125985),
(#125986,#125987),(#125988,#125989),(#125990,#125991),(#125992,#125993),
(#125994,#125995),(#125996,#125997),(#125998,#125999),(#126000,#126001),
(#126002,#126003),(#126004,#126005),(#126006,#126007),(#126008,#126009),
(#126010,#126011),(#126012,#126013),(#126014,#126015),(#126016,#126017),
(#126018,#126019),(#126020,#126021),(#126022,#126023),(#126024,#126025),
(#126026,#126027),(#126028,#126029),(#126030,#126031),(#126032,#126033),
(#126034,#126035),(#126036,#126037),(#126038,#126039),(#126040,#126041),
(#126042,#126043),(#126044,#126045),(#126046,#126047),(#126048,#126049),
(#126050,#126051),(#126052,#126053),(#126054,#126055),(#126056,#126057),
(#126058,#126059),(#126060,#126061),(#126062,#126063),(#126064,#126065),
(#126066,#126067),(#126068,#126069),(#126070,#126071),(#126072,#126073),
(#126074,#126075),(#126076,#126077),(#126078,#126079),(#126080,#126081),
(#126082,#126083),(#126084,#126085),(#126086,#126087),(#126088,#126089),
(#126090,#126091),(#126092,#126093),(#126094,#126095),(#126096,#126097),
(#126098,#126099),(#126100,#126101),(#126102,#126103),(#126104,#126105),
(#126106,#126107),(#126108,#126109),(#126110,#126111),(#126112,#126113),
(#126114,#126115),(#126116,#126117),(#126118,#126119),(#126120,#126121),
(#126122,#126123),(#126124,#126125),(#126126,#126127),(#126128,#126129),
(#126130,#126131),(#126132,#126133),(#126134,#126135),(#126136,#126137),
(#126138,#126139),(#126140,#126141),(#126142,#126143),(#126144,#126145),
(#126146,#126147),(#126148,#126149),(#126150,#126151),(#126152,#126153),
(#126154,#126155),(#126156,#126157),(#126158,#126159),(#126160,#126161),
(#126162,#126163),(#126164,#126165),(#126166,#126167),(#126168,#126169),
(#126170,#126171),(#126172,#126173),(#126174,#126175),(#126176,#126177),
(#126178,#126179),(#126180,#126181),(#126182,#126183),(#126184,#126185),
(#126186,#126187),(#126188,#126189),(#126190,#126191),(#126192,#126193),
(#126194,#126195),(#126196,#126197),(#126198,#126199),(#126200,#126201),
(#126202,#126203),(#126204,#126205),(#126206,#126207),(#126208,#126209),
(#126210,#126211),(#126212,#126213)),.UNSPECIFIED.,.F.,.F.,.F.)
B_SPLINE_SURFACE_WITH_KNOTS((6,1,1,1,1,1,1,1,1,1,1,1,1,1,1,1,1,1,1,1,1,
1,1,1,1,1,1,1,1,1,1,1,1,1,1,1,1,1,1,1,1,1,1,1,1,1,1,1,1,1,1,1,1,1,1,1,1,
1,1,1,1,1,1,1,1,1,1,1,1,1,1,1,1,1,1,1,1,1,1,1,1,1,1,1,1,1,1,1,1,1,1,1,1,
1,1,1,1,1,1,1,1,1,1,1,1,1,1,1,1,1,1,1,1,1,1,1,1,1,1,1,1,1,1,1,1,1,1,1,1,
1,1,1,1,1,1,1,1,1,1,1,1,1,1,1,1,1,1,1,1,1,1,1,1,1,1,1,1,1,1,1,1,1,1,1,1,
1,1,1,1,1,1,1,1,1,1,1,1,1,1,1,1,1,1,1,1,1,1,1,1,1,1,1,1,1,1,1,1,1,1,1,6),
(2,2),(-1.,-0.995000000000001,-0.990000000000001,-0.985000000000001,-0.980000000000001,
-0.975000000000001,-0.970000000000001,-0.965000000000001,-0.960000000000001,
-0.955000000000001,-0.950000000000001,-0.945000000000001,-0.940000000000001,
-0.935000000000001,-0.930000000000001,-0.925000000000001,-0.920000000000001,
-0.915000000000001,-0.910000000000001,-0.905000000000001,-0.900000000000001,
-0.895000000000001,-0.890000000000001,-0.885000000000001,-0.880000000000001,
-0.875000000000001,-0.870000000000001,-0.865000000000001,-0.860000000000001,
-0.855000000000001,-0.850000000000001,-0.845000000000001,-0.840000000000001,
-0.835000000000001,-0.830000000000001,-0.825000000000001,-0.820000000000001,
-0.815000000000001,-0.810000000000001,-0.805000000000001,-0.800000000000001,
-0.795000000000001,-0.790000000000001,-0.785000000000001,-0.780000000000001,
-0.775000000000001,-0.770000000000001,-0.765000000000001,-0.760000000000001,
-0.755000000000001,-0.750000000000001,-0.745000000000001,-0.740000000000001,
-0.735000000000001,-0.730000000000001,-0.725000000000001,-0.720000000000001,
-0.715000000000001,-0.710000000000001,-0.705000000000001,-0.700000000000001,
-0.695000000000001,-0.690000000000001,-0.685,-0.68,-0.675,-0.67,-0.665,
-0.66,-0.655,-0.65,-0.645,-0.64,-0.635,-0.63,-0.625,-0.62,-0.615,-0.61,
-0.605,-0.6,-0.595,-0.59,-0.585,-0.58,-0.575,-0.57,-0.565,-0.56,-0.555,
-0.55,-0.545,-0.54,-0.535,-0.53,-0.525,-0.52,-0.515,-0.51,-0.505,-0.5,-0.495,
-0.49,-0.485,-0.48,-0.475,-0.47,-0.465,-0.46,-0.455,-0.45,-0.445,-0.44,
-0.435,-0.43,-0.425,-0.42,-0.415,-0.41,-0.405,-0.4,-0.395,-0.39,-0.385,
-0.38,-0.375,-0.37,-0.365,-0.36,-0.355,-0.35,-0.345,-0.34,-0.335,-0.33,
-0.325,-0.32,-0.315,-0.31,-0.305,-0.3,-0.295,-0.29,-0.285,-0.28,-0.275,
-0.27,-0.265,-0.26,-0.255,-0.25,-0.245,-0.24,-0.235,-0.23,-0.225,-0.22,
-0.215,-0.21,-0.205,-0.2,-0.195,-0.19,-0.185,-0.18,-0.175,-0.17,-0.165,
-0.16,-0.155,-0.15,-0.145,-0.14,-0.135,-0.13,-0.125,-0.12,-0.115,-0.11,
-0.105,-0.1,-0.095,-0.09,-0.085,-0.08,-0.075,-0.07,-0.065,-0.06,-0.055,
-0.05,-0.045,-0.04,-0.035,-0.03,-0.025,-0.02,-0.015,-0.01,-0.005,0.),(0.,
1.2),.UNSPECIFIED.)
GEOMETRIC_REPRESENTATION_ITEM()
RATIONAL_B_SPLINE_SURFACE(((1.,1.),(1.,1.),(1.,1.),(1.,1.),(1.,1.),(1.,
1.),(1.,1.),(1.,1.),(1.,1.),(1.,1.),(1.,1.),(1.,1.),(1.,1.),(1.,1.),(1.,
1.),(1.,1.),(1.,1.),(1.,1.),(1.,1.),(1.,1.),(1.,1.),(1.,1.),(1.,1.),(1.,
1.),(1.,1.),(1.,1.),(1.,1.),(1.,1.),(1.,1.),(1.,1.),(1.,1.),(1.,1.),(1.,
1.),(1.,1.),(1.,1.),(1.,1.),(1.,1.),(1.,1.),(1.,1.),(1.,1.),(1.,1.),(1.,
1.),(1.,1.),(1.,1.),(1.,1.),(1.,1.),(1.,1.),(1.,1.),(1.,1.),(1.,1.),(1.,
1.),(1.,1.),(1.,1.),(1.,1.),(1.,1.),(1.,1.),(1.,1.),(1.,1.),(1.,1.),(1.,
1.),(1.,1.),(1.,1.),(1.,1.),(1.,1.),(1.,1.),(1.,1.),(1.,1.),(1.,1.),(1.,
1.),(1.,1.),(1.,1.),(1.,1.),(1.,1.),(1.,1.),(1.,1.),(1.,1.),(1.,1.),(1.,
1.),(1.,1.),(1.,1.),(1.,1.),(1.,1.),(1.,1.),(1.,1.),(1.,1.),(1.,1.),(1.,
1.),(1.,1.),(1.,1.),(1.,1.),(1.,1.),(1.,1.),(1.,1.),(1.,1.),(1.,1.),(1.,
1.),(1.,1.),(1.,1.),(1.,1.),(1.,1.),(1.,1.),(1.,1.),(1.,1.),(1.,1.),(1.,
1.),(1.,1.),(1.,1.),(1.,1.),(1.,1.),(1.,1.),(1.,1.),(1.,1.),(1.,1.),(1.,
1.),(1.,1.),(1.,1.),(1.,1.),(1.,1.),(1.,1.),(1.,1.),(1.,1.),(1.,1.),(1.,
1.),(1.,1.),(1.,1.),(1.,1.),(1.,1.),(1.,1.),(1.,1.),(1.,1.),(1.,1.),(1.,
1.),(1.,1.),(1.,1.),(1.,1.),(1.,1.),(1.,1.),(1.,1.),(1.,1.),(1.,1.),(1.,
1.),(1.,1.),(1.,1.),(1.,1.),(1.,1.),(1.,1.),(1.,1.),(1.,1.),(1.,1.),(1.,
1.),(1.,1.),(1.,1.),(1.,1.),(1.,1.),(1.,1.),(1.,1.),(1.,1.),(1.,1.),(1.,
1.),(1.,1.),(1.,1.),(1.,1.),(1.,1.),(1.,1.),(1.,1.),(1.,1.),(1.,1.),(1.,
1.),(1.,1.),(1.,1.),(1.,1.),(1.,1.),(1.,1.),(1.,1.),(1.,1.),(1.,1.),(1.,
1.),(1.,1.),(1.,1.),(1.,1.),(1.,1.),(1.,1.),(1.,1.),(1.,1.),(1.,1.),(1.,
1.),(1.,1.),(1.,1.),(1.,1.),(1.,1.),(1.,1.),(1.,1.),(1.,1.),(1.,1.),(1.,
1.),(1.,1.),(1.,1.),(1.,1.),(1.,1.),(1.,1.),(1.,1.),(1.,1.),(1.,1.),(1.,
1.),(1.,1.)))
REPRESENTATION_ITEM('')
SURFACE()
);
#967=(
BOUNDED_SURFACE()
B_SPLINE_SURFACE(5,1,((#126605,#126606),(#126607,#126608),(#126609,#126610),
(#126611,#126612),(#126613,#126614),(#126615,#126616),(#126617,#126618),
(#126619,#126620),(#126621,#126622),(#126623,#126624),(#126625,#126626),
(#126627,#126628),(#126629,#126630),(#126631,#126632),(#126633,#126634),
(#126635,#126636),(#126637,#126638),(#126639,#126640),(#126641,#126642),
(#126643,#126644),(#126645,#126646),(#126647,#126648),(#126649,#126650),
(#126651,#126652),(#126653,#126654),(#126655,#126656),(#126657,#126658),
(#126659,#126660),(#126661,#126662),(#126663,#126664),(#126665,#126666),
(#126667,#126668),(#126669,#126670),(#126671,#126672),(#126673,#126674),
(#126675,#126676),(#126677,#126678),(#126679,#126680),(#126681,#126682),
(#126683,#126684),(#126685,#126686),(#126687,#126688),(#126689,#126690),
(#126691,#126692),(#126693,#126694),(#126695,#126696),(#126697,#126698),
(#126699,#126700),(#126701,#126702),(#126703,#126704),(#126705,#126706),
(#126707,#126708),(#126709,#126710),(#126711,#126712),(#126713,#126714),
(#126715,#126716),(#126717,#126718),(#126719,#126720),(#126721,#126722),
(#126723,#126724),(#126725,#126726),(#126727,#126728),(#126729,#126730),
(#126731,#126732),(#126733,#126734),(#126735,#126736),(#126737,#126738),
(#126739,#126740),(#126741,#126742),(#126743,#126744),(#126745,#126746),
(#126747,#126748),(#126749,#126750),(#126751,#126752),(#126753,#126754),
(#126755,#126756),(#126757,#126758),(#126759,#126760),(#126761,#126762),
(#126763,#126764),(#126765,#126766),(#126767,#126768),(#126769,#126770),
(#126771,#126772),(#126773,#126774),(#126775,#126776),(#126777,#126778),
(#126779,#126780),(#126781,#126782),(#126783,#126784),(#126785,#126786),
(#126787,#126788),(#126789,#126790),(#126791,#126792),(#126793,#126794),
(#126795,#126796),(#126797,#126798),(#126799,#126800),(#126801,#126802),
(#126803,#126804),(#126805,#126806),(#126807,#126808),(#126809,#126810),
(#126811,#126812),(#126813,#126814),(#126815,#126816),(#126817,#126818),
(#126819,#126820),(#126821,#126822),(#126823,#126824),(#126825,#126826),
(#126827,#126828),(#126829,#126830),(#126831,#126832),(#126833,#126834),
(#126835,#126836),(#126837,#126838),(#126839,#126840),(#126841,#126842),
(#126843,#126844),(#126845,#126846),(#126847,#126848),(#126849,#126850),
(#126851,#126852),(#126853,#126854),(#126855,#126856),(#126857,#126858),
(#126859,#126860),(#126861,#126862),(#126863,#126864),(#126865,#126866),
(#126867,#126868),(#126869,#126870),(#126871,#126872),(#126873,#126874),
(#126875,#126876),(#126877,#126878),(#126879,#126880),(#126881,#126882),
(#126883,#126884),(#126885,#126886),(#126887,#126888),(#126889,#126890),
(#126891,#126892),(#126893,#126894),(#126895,#126896),(#126897,#126898),
(#126899,#126900),(#126901,#126902),(#126903,#126904),(#126905,#126906),
(#126907,#126908),(#126909,#126910),(#126911,#126912),(#126913,#126914),
(#126915,#126916),(#126917,#126918),(#126919,#126920),(#126921,#126922),
(#126923,#126924),(#126925,#126926),(#126927,#126928),(#126929,#126930),
(#126931,#126932),(#126933,#126934),(#126935,#126936),(#126937,#126938),
(#126939,#126940),(#126941,#126942),(#126943,#126944),(#126945,#126946),
(#126947,#126948),(#126949,#126950),(#126951,#126952),(#126953,#126954),
(#126955,#126956),(#126957,#126958),(#126959,#126960),(#126961,#126962),
(#126963,#126964),(#126965,#126966),(#126967,#126968),(#126969,#126970),
(#126971,#126972),(#126973,#126974),(#126975,#126976),(#126977,#126978),
(#126979,#126980),(#126981,#126982),(#126983,#126984),(#126985,#126986),
(#126987,#126988),(#126989,#126990),(#126991,#126992),(#126993,#126994),
(#126995,#126996),(#126997,#126998),(#126999,#127000),(#127001,#127002),
(#127003,#127004),(#127005,#127006),(#127007,#127008),(#127009,#127010),
(#127011,#127012),(#127013,#127014)),.UNSPECIFIED.,.F.,.F.,.F.)
B_SPLINE_SURFACE_WITH_KNOTS((6,1,1,1,1,1,1,1,1,1,1,1,1,1,1,1,1,1,1,1,1,
1,1,1,1,1,1,1,1,1,1,1,1,1,1,1,1,1,1,1,1,1,1,1,1,1,1,1,1,1,1,1,1,1,1,1,1,
1,1,1,1,1,1,1,1,1,1,1,1,1,1,1,1,1,1,1,1,1,1,1,1,1,1,1,1,1,1,1,1,1,1,1,1,
1,1,1,1,1,1,1,1,1,1,1,1,1,1,1,1,1,1,1,1,1,1,1,1,1,1,1,1,1,1,1,1,1,1,1,1,
1,1,1,1,1,1,1,1,1,1,1,1,1,1,1,1,1,1,1,1,1,1,1,1,1,1,1,1,1,1,1,1,1,1,1,1,
1,1,1,1,1,1,1,1,1,1,1,1,1,1,1,1,1,1,1,1,1,1,1,1,1,1,1,1,1,1,1,1,1,1,1,6),
(2,2),(-1.,-0.995000000000001,-0.990000000000001,-0.985000000000001,-0.980000000000001,
-0.975000000000001,-0.970000000000001,-0.965000000000001,-0.960000000000001,
-0.955000000000001,-0.950000000000001,-0.945000000000001,-0.940000000000001,
-0.935000000000001,-0.930000000000001,-0.925000000000001,-0.920000000000001,
-0.915000000000001,-0.910000000000001,-0.905000000000001,-0.900000000000001,
-0.895000000000001,-0.890000000000001,-0.885000000000001,-0.880000000000001,
-0.875000000000001,-0.870000000000001,-0.865000000000001,-0.860000000000001,
-0.855000000000001,-0.850000000000001,-0.845000000000001,-0.840000000000001,
-0.835000000000001,-0.830000000000001,-0.825000000000001,-0.820000000000001,
-0.815000000000001,-0.810000000000001,-0.805000000000001,-0.800000000000001,
-0.795000000000001,-0.790000000000001,-0.785000000000001,-0.780000000000001,
-0.775000000000001,-0.770000000000001,-0.765000000000001,-0.760000000000001,
-0.755000000000001,-0.750000000000001,-0.745000000000001,-0.740000000000001,
-0.735000000000001,-0.730000000000001,-0.725000000000001,-0.720000000000001,
-0.715000000000001,-0.710000000000001,-0.705000000000001,-0.700000000000001,
-0.695000000000001,-0.690000000000001,-0.685,-0.68,-0.675,-0.67,-0.665,
-0.66,-0.655,-0.65,-0.645,-0.64,-0.635,-0.63,-0.625,-0.62,-0.615,-0.61,
-0.605,-0.6,-0.595,-0.59,-0.585,-0.58,-0.575,-0.57,-0.565,-0.56,-0.555,
-0.55,-0.545,-0.54,-0.535,-0.53,-0.525,-0.52,-0.515,-0.51,-0.505,-0.5,-0.495,
-0.49,-0.485,-0.48,-0.475,-0.47,-0.465,-0.46,-0.455,-0.45,-0.445,-0.44,
-0.435,-0.43,-0.425,-0.42,-0.415,-0.41,-0.405,-0.4,-0.395,-0.39,-0.385,
-0.38,-0.375,-0.37,-0.365,-0.36,-0.355,-0.35,-0.345,-0.34,-0.335,-0.33,
-0.325,-0.32,-0.315,-0.31,-0.305,-0.3,-0.295,-0.29,-0.285,-0.28,-0.275,
-0.27,-0.265,-0.26,-0.255,-0.25,-0.245,-0.24,-0.235,-0.23,-0.225,-0.22,
-0.215,-0.21,-0.205,-0.2,-0.195,-0.19,-0.185,-0.18,-0.175,-0.17,-0.165,
-0.16,-0.155,-0.15,-0.145,-0.14,-0.135,-0.13,-0.125,-0.12,-0.115,-0.11,
-0.105,-0.1,-0.095,-0.09,-0.085,-0.08,-0.075,-0.07,-0.065,-0.06,-0.055,
-0.05,-0.045,-0.04,-0.035,-0.03,-0.025,-0.02,-0.015,-0.01,-0.005,0.),(0.,
1.2),.UNSPECIFIED.)
GEOMETRIC_REPRESENTATION_ITEM()
RATIONAL_B_SPLINE_SURFACE(((1.,1.),(1.,1.),(1.,1.),(1.,1.),(1.,1.),(1.,
1.),(1.,1.),(1.,1.),(1.,1.),(1.,1.),(1.,1.),(1.,1.),(1.,1.),(1.,1.),(1.,
1.),(1.,1.),(1.,1.),(1.,1.),(1.,1.),(1.,1.),(1.,1.),(1.,1.),(1.,1.),(1.,
1.),(1.,1.),(1.,1.),(1.,1.),(1.,1.),(1.,1.),(1.,1.),(1.,1.),(1.,1.),(1.,
1.),(1.,1.),(1.,1.),(1.,1.),(1.,1.),(1.,1.),(1.,1.),(1.,1.),(1.,1.),(1.,
1.),(1.,1.),(1.,1.),(1.,1.),(1.,1.),(1.,1.),(1.,1.),(1.,1.),(1.,1.),(1.,
1.),(1.,1.),(1.,1.),(1.,1.),(1.,1.),(1.,1.),(1.,1.),(1.,1.),(1.,1.),(1.,
1.),(1.,1.),(1.,1.),(1.,1.),(1.,1.),(1.,1.),(1.,1.),(1.,1.),(1.,1.),(1.,
1.),(1.,1.),(1.,1.),(1.,1.),(1.,1.),(1.,1.),(1.,1.),(1.,1.),(1.,1.),(1.,
1.),(1.,1.),(1.,1.),(1.,1.),(1.,1.),(1.,1.),(1.,1.),(1.,1.),(1.,1.),(1.,
1.),(1.,1.),(1.,1.),(1.,1.),(1.,1.),(1.,1.),(1.,1.),(1.,1.),(1.,1.),(1.,
1.),(1.,1.),(1.,1.),(1.,1.),(1.,1.),(1.,1.),(1.,1.),(1.,1.),(1.,1.),(1.,
1.),(1.,1.),(1.,1.),(1.,1.),(1.,1.),(1.,1.),(1.,1.),(1.,1.),(1.,1.),(1.,
1.),(1.,1.),(1.,1.),(1.,1.),(1.,1.),(1.,1.),(1.,1.),(1.,1.),(1.,1.),(1.,
1.),(1.,1.),(1.,1.),(1.,1.),(1.,1.),(1.,1.),(1.,1.),(1.,1.),(1.,1.),(1.,
1.),(1.,1.),(1.,1.),(1.,1.),(1.,1.),(1.,1.),(1.,1.),(1.,1.),(1.,1.),(1.,
1.),(1.,1.),(1.,1.),(1.,1.),(1.,1.),(1.,1.),(1.,1.),(1.,1.),(1.,1.),(1.,
1.),(1.,1.),(1.,1.),(1.,1.),(1.,1.),(1.,1.),(1.,1.),(1.,1.),(1.,1.),(1.,
1.),(1.,1.),(1.,1.),(1.,1.),(1.,1.),(1.,1.),(1.,1.),(1.,1.),(1.,1.),(1.,
1.),(1.,1.),(1.,1.),(1.,1.),(1.,1.),(1.,1.),(1.,1.),(1.,1.),(1.,1.),(1.,
1.),(1.,1.),(1.,1.),(1.,1.),(1.,1.),(1.,1.),(1.,1.),(1.,1.),(1.,1.),(1.,
1.),(1.,1.),(1.,1.),(1.,1.),(1.,1.),(1.,1.),(1.,1.),(1.,1.),(1.,1.),(1.,
1.),(1.,1.),(1.,1.),(1.,1.),(1.,1.),(1.,1.),(1.,1.),(1.,1.),(1.,1.),(1.,
1.),(1.,1.)))
REPRESENTATION_ITEM('')
SURFACE()
);
#968=(
BOUNDED_SURFACE()
B_SPLINE_SURFACE(5,1,((#127406,#127407),(#127408,#127409),(#127410,#127411),
(#127412,#127413),(#127414,#127415),(#127416,#127417),(#127418,#127419),
(#127420,#127421),(#127422,#127423),(#127424,#127425),(#127426,#127427),
(#127428,#127429),(#127430,#127431),(#127432,#127433),(#127434,#127435),
(#127436,#127437),(#127438,#127439),(#127440,#127441),(#127442,#127443),
(#127444,#127445),(#127446,#127447),(#127448,#127449),(#127450,#127451),
(#127452,#127453),(#127454,#127455),(#127456,#127457),(#127458,#127459),
(#127460,#127461),(#127462,#127463),(#127464,#127465),(#127466,#127467),
(#127468,#127469),(#127470,#127471),(#127472,#127473),(#127474,#127475),
(#127476,#127477),(#127478,#127479),(#127480,#127481),(#127482,#127483),
(#127484,#127485),(#127486,#127487),(#127488,#127489),(#127490,#127491),
(#127492,#127493),(#127494,#127495),(#127496,#127497),(#127498,#127499),
(#127500,#127501),(#127502,#127503),(#127504,#127505),(#127506,#127507),
(#127508,#127509),(#127510,#127511),(#127512,#127513),(#127514,#127515),
(#127516,#127517),(#127518,#127519),(#127520,#127521),(#127522,#127523),
(#127524,#127525),(#127526,#127527),(#127528,#127529),(#127530,#127531),
(#127532,#127533),(#127534,#127535),(#127536,#127537),(#127538,#127539),
(#127540,#127541),(#127542,#127543),(#127544,#127545),(#127546,#127547),
(#127548,#127549),(#127550,#127551),(#127552,#127553),(#127554,#127555),
(#127556,#127557),(#127558,#127559),(#127560,#127561),(#127562,#127563),
(#127564,#127565),(#127566,#127567),(#127568,#127569),(#127570,#127571),
(#127572,#127573),(#127574,#127575),(#127576,#127577),(#127578,#127579),
(#127580,#127581),(#127582,#127583),(#127584,#127585),(#127586,#127587),
(#127588,#127589),(#127590,#127591),(#127592,#127593),(#127594,#127595),
(#127596,#127597),(#127598,#127599),(#127600,#127601),(#127602,#127603),
(#127604,#127605),(#127606,#127607),(#127608,#127609),(#127610,#127611),
(#127612,#127613),(#127614,#127615),(#127616,#127617),(#127618,#127619),
(#127620,#127621),(#127622,#127623),(#127624,#127625),(#127626,#127627),
(#127628,#127629),(#127630,#127631),(#127632,#127633),(#127634,#127635),
(#127636,#127637),(#127638,#127639),(#127640,#127641),(#127642,#127643),
(#127644,#127645),(#127646,#127647),(#127648,#127649),(#127650,#127651),
(#127652,#127653),(#127654,#127655),(#127656,#127657),(#127658,#127659),
(#127660,#127661),(#127662,#127663),(#127664,#127665),(#127666,#127667),
(#127668,#127669),(#127670,#127671),(#127672,#127673),(#127674,#127675),
(#127676,#127677),(#127678,#127679),(#127680,#127681),(#127682,#127683),
(#127684,#127685),(#127686,#127687),(#127688,#127689),(#127690,#127691),
(#127692,#127693),(#127694,#127695),(#127696,#127697),(#127698,#127699),
(#127700,#127701),(#127702,#127703),(#127704,#127705),(#127706,#127707),
(#127708,#127709),(#127710,#127711),(#127712,#127713),(#127714,#127715),
(#127716,#127717),(#127718,#127719),(#127720,#127721),(#127722,#127723),
(#127724,#127725),(#127726,#127727),(#127728,#127729),(#127730,#127731),
(#127732,#127733),(#127734,#127735),(#127736,#127737),(#127738,#127739),
(#127740,#127741),(#127742,#127743),(#127744,#127745),(#127746,#127747),
(#127748,#127749),(#127750,#127751),(#127752,#127753),(#127754,#127755),
(#127756,#127757),(#127758,#127759),(#127760,#127761),(#127762,#127763),
(#127764,#127765),(#127766,#127767),(#127768,#127769),(#127770,#127771),
(#127772,#127773),(#127774,#127775),(#127776,#127777),(#127778,#127779),
(#127780,#127781),(#127782,#127783),(#127784,#127785),(#127786,#127787),
(#127788,#127789),(#127790,#127791),(#127792,#127793),(#127794,#127795),
(#127796,#127797),(#127798,#127799),(#127800,#127801),(#127802,#127803),
(#127804,#127805),(#127806,#127807),(#127808,#127809),(#127810,#127811),
(#127812,#127813),(#127814,#127815)),.UNSPECIFIED.,.F.,.F.,.F.)
B_SPLINE_SURFACE_WITH_KNOTS((6,1,1,1,1,1,1,1,1,1,1,1,1,1,1,1,1,1,1,1,1,
1,1,1,1,1,1,1,1,1,1,1,1,1,1,1,1,1,1,1,1,1,1,1,1,1,1,1,1,1,1,1,1,1,1,1,1,
1,1,1,1,1,1,1,1,1,1,1,1,1,1,1,1,1,1,1,1,1,1,1,1,1,1,1,1,1,1,1,1,1,1,1,1,
1,1,1,1,1,1,1,1,1,1,1,1,1,1,1,1,1,1,1,1,1,1,1,1,1,1,1,1,1,1,1,1,1,1,1,1,
1,1,1,1,1,1,1,1,1,1,1,1,1,1,1,1,1,1,1,1,1,1,1,1,1,1,1,1,1,1,1,1,1,1,1,1,
1,1,1,1,1,1,1,1,1,1,1,1,1,1,1,1,1,1,1,1,1,1,1,1,1,1,1,1,1,1,1,1,1,1,1,6),
(2,2),(-1.,-0.995000000000001,-0.990000000000001,-0.985000000000001,-0.980000000000001,
-0.975000000000001,-0.970000000000001,-0.965000000000001,-0.960000000000001,
-0.955000000000001,-0.950000000000001,-0.945000000000001,-0.940000000000001,
-0.935000000000001,-0.930000000000001,-0.925000000000001,-0.920000000000001,
-0.915000000000001,-0.910000000000001,-0.905000000000001,-0.900000000000001,
-0.895000000000001,-0.890000000000001,-0.885000000000001,-0.880000000000001,
-0.875000000000001,-0.870000000000001,-0.865000000000001,-0.860000000000001,
-0.855000000000001,-0.850000000000001,-0.845000000000001,-0.840000000000001,
-0.835000000000001,-0.830000000000001,-0.825000000000001,-0.820000000000001,
-0.815000000000001,-0.810000000000001,-0.805000000000001,-0.800000000000001,
-0.795000000000001,-0.790000000000001,-0.785000000000001,-0.780000000000001,
-0.775000000000001,-0.770000000000001,-0.765000000000001,-0.760000000000001,
-0.755000000000001,-0.750000000000001,-0.745000000000001,-0.740000000000001,
-0.735000000000001,-0.730000000000001,-0.725000000000001,-0.720000000000001,
-0.715000000000001,-0.710000000000001,-0.705000000000001,-0.700000000000001,
-0.695000000000001,-0.690000000000001,-0.685,-0.68,-0.675,-0.67,-0.665,
-0.66,-0.655,-0.65,-0.645,-0.64,-0.635,-0.63,-0.625,-0.62,-0.615,-0.61,
-0.605,-0.6,-0.595,-0.59,-0.585,-0.58,-0.575,-0.57,-0.565,-0.56,-0.555,
-0.55,-0.545,-0.54,-0.535,-0.53,-0.525,-0.52,-0.515,-0.51,-0.505,-0.5,-0.495,
-0.49,-0.485,-0.48,-0.475,-0.47,-0.465,-0.46,-0.455,-0.45,-0.445,-0.44,
-0.435,-0.43,-0.425,-0.42,-0.415,-0.41,-0.405,-0.4,-0.395,-0.39,-0.385,
-0.38,-0.375,-0.37,-0.365,-0.36,-0.355,-0.35,-0.345,-0.34,-0.335,-0.33,
-0.325,-0.32,-0.315,-0.31,-0.305,-0.3,-0.295,-0.29,-0.285,-0.28,-0.275,
-0.27,-0.265,-0.26,-0.255,-0.25,-0.245,-0.24,-0.235,-0.23,-0.225,-0.22,
-0.215,-0.21,-0.205,-0.2,-0.195,-0.19,-0.185,-0.18,-0.175,-0.17,-0.165,
-0.16,-0.155,-0.15,-0.145,-0.14,-0.135,-0.13,-0.125,-0.12,-0.115,-0.11,
-0.105,-0.1,-0.095,-0.09,-0.085,-0.08,-0.075,-0.07,-0.065,-0.06,-0.055,
-0.05,-0.045,-0.04,-0.035,-0.03,-0.025,-0.02,-0.015,-0.01,-0.005,0.),(0.,
1.2),.UNSPECIFIED.)
GEOMETRIC_REPRESENTATION_ITEM()
RATIONAL_B_SPLINE_SURFACE(((1.,1.),(1.,1.),(1.,1.),(1.,1.),(1.,1.),(1.,
1.),(1.,1.),(1.,1.),(1.,1.),(1.,1.),(1.,1.),(1.,1.),(1.,1.),(1.,1.),(1.,
1.),(1.,1.),(1.,1.),(1.,1.),(1.,1.),(1.,1.),(1.,1.),(1.,1.),(1.,1.),(1.,
1.),(1.,1.),(1.,1.),(1.,1.),(1.,1.),(1.,1.),(1.,1.),(1.,1.),(1.,1.),(1.,
1.),(1.,1.),(1.,1.),(1.,1.),(1.,1.),(1.,1.),(1.,1.),(1.,1.),(1.,1.),(1.,
1.),(1.,1.),(1.,1.),(1.,1.),(1.,1.),(1.,1.),(1.,1.),(1.,1.),(1.,1.),(1.,
1.),(1.,1.),(1.,1.),(1.,1.),(1.,1.),(1.,1.),(1.,1.),(1.,1.),(1.,1.),(1.,
1.),(1.,1.),(1.,1.),(1.,1.),(1.,1.),(1.,1.),(1.,1.),(1.,1.),(1.,1.),(1.,
1.),(1.,1.),(1.,1.),(1.,1.),(1.,1.),(1.,1.),(1.,1.),(1.,1.),(1.,1.),(1.,
1.),(1.,1.),(1.,1.),(1.,1.),(1.,1.),(1.,1.),(1.,1.),(1.,1.),(1.,1.),(1.,
1.),(1.,1.),(1.,1.),(1.,1.),(1.,1.),(1.,1.),(1.,1.),(1.,1.),(1.,1.),(1.,
1.),(1.,1.),(1.,1.),(1.,1.),(1.,1.),(1.,1.),(1.,1.),(1.,1.),(1.,1.),(1.,
1.),(1.,1.),(1.,1.),(1.,1.),(1.,1.),(1.,1.),(1.,1.),(1.,1.),(1.,1.),(1.,
1.),(1.,1.),(1.,1.),(1.,1.),(1.,1.),(1.,1.),(1.,1.),(1.,1.),(1.,1.),(1.,
1.),(1.,1.),(1.,1.),(1.,1.),(1.,1.),(1.,1.),(1.,1.),(1.,1.),(1.,1.),(1.,
1.),(1.,1.),(1.,1.),(1.,1.),(1.,1.),(1.,1.),(1.,1.),(1.,1.),(1.,1.),(1.,
1.),(1.,1.),(1.,1.),(1.,1.),(1.,1.),(1.,1.),(1.,1.),(1.,1.),(1.,1.),(1.,
1.),(1.,1.),(1.,1.),(1.,1.),(1.,1.),(1.,1.),(1.,1.),(1.,1.),(1.,1.),(1.,
1.),(1.,1.),(1.,1.),(1.,1.),(1.,1.),(1.,1.),(1.,1.),(1.,1.),(1.,1.),(1.,
1.),(1.,1.),(1.,1.),(1.,1.),(1.,1.),(1.,1.),(1.,1.),(1.,1.),(1.,1.),(1.,
1.),(1.,1.),(1.,1.),(1.,1.),(1.,1.),(1.,1.),(1.,1.),(1.,1.),(1.,1.),(1.,
1.),(1.,1.),(1.,1.),(1.,1.),(1.,1.),(1.,1.),(1.,1.),(1.,1.),(1.,1.),(1.,
1.),(1.,1.),(1.,1.),(1.,1.),(1.,1.),(1.,1.),(1.,1.),(1.,1.),(1.,1.),(1.,
1.),(1.,1.)))
REPRESENTATION_ITEM('')
SURFACE()
);
#969=(
BOUNDED_SURFACE()
B_SPLINE_SURFACE(5,1,((#128207,#128208),(#128209,#128210),(#128211,#128212),
(#128213,#128214),(#128215,#128216),(#128217,#128218),(#128219,#128220),
(#128221,#128222),(#128223,#128224),(#128225,#128226),(#128227,#128228),
(#128229,#128230),(#128231,#128232),(#128233,#128234),(#128235,#128236),
(#128237,#128238),(#128239,#128240),(#128241,#128242),(#128243,#128244),
(#128245,#128246),(#128247,#128248),(#128249,#128250),(#128251,#128252),
(#128253,#128254),(#128255,#128256),(#128257,#128258),(#128259,#128260),
(#128261,#128262),(#128263,#128264),(#128265,#128266),(#128267,#128268),
(#128269,#128270),(#128271,#128272),(#128273,#128274),(#128275,#128276),
(#128277,#128278),(#128279,#128280),(#128281,#128282),(#128283,#128284),
(#128285,#128286),(#128287,#128288),(#128289,#128290),(#128291,#128292),
(#128293,#128294),(#128295,#128296),(#128297,#128298),(#128299,#128300),
(#128301,#128302),(#128303,#128304),(#128305,#128306),(#128307,#128308),
(#128309,#128310),(#128311,#128312),(#128313,#128314),(#128315,#128316),
(#128317,#128318),(#128319,#128320),(#128321,#128322),(#128323,#128324),
(#128325,#128326),(#128327,#128328),(#128329,#128330),(#128331,#128332),
(#128333,#128334),(#128335,#128336),(#128337,#128338),(#128339,#128340),
(#128341,#128342),(#128343,#128344),(#128345,#128346),(#128347,#128348),
(#128349,#128350),(#128351,#128352),(#128353,#128354),(#128355,#128356),
(#128357,#128358),(#128359,#128360),(#128361,#128362),(#128363,#128364),
(#128365,#128366),(#128367,#128368),(#128369,#128370),(#128371,#128372),
(#128373,#128374),(#128375,#128376),(#128377,#128378),(#128379,#128380),
(#128381,#128382),(#128383,#128384),(#128385,#128386),(#128387,#128388),
(#128389,#128390),(#128391,#128392),(#128393,#128394),(#128395,#128396),
(#128397,#128398),(#128399,#128400),(#128401,#128402),(#128403,#128404),
(#128405,#128406),(#128407,#128408),(#128409,#128410),(#128411,#128412),
(#128413,#128414),(#128415,#128416),(#128417,#128418),(#128419,#128420),
(#128421,#128422),(#128423,#128424),(#128425,#128426),(#128427,#128428),
(#128429,#128430),(#128431,#128432),(#128433,#128434),(#128435,#128436),
(#128437,#128438),(#128439,#128440),(#128441,#128442),(#128443,#128444),
(#128445,#128446),(#128447,#128448),(#128449,#128450),(#128451,#128452),
(#128453,#128454),(#128455,#128456),(#128457,#128458),(#128459,#128460),
(#128461,#128462),(#128463,#128464),(#128465,#128466),(#128467,#128468),
(#128469,#128470),(#128471,#128472),(#128473,#128474),(#128475,#128476),
(#128477,#128478),(#128479,#128480),(#128481,#128482),(#128483,#128484),
(#128485,#128486),(#128487,#128488),(#128489,#128490),(#128491,#128492),
(#128493,#128494),(#128495,#128496),(#128497,#128498),(#128499,#128500),
(#128501,#128502),(#128503,#128504),(#128505,#128506),(#128507,#128508),
(#128509,#128510),(#128511,#128512),(#128513,#128514),(#128515,#128516),
(#128517,#128518),(#128519,#128520),(#128521,#128522),(#128523,#128524),
(#128525,#128526),(#128527,#128528),(#128529,#128530),(#128531,#128532),
(#128533,#128534),(#128535,#128536),(#128537,#128538),(#128539,#128540),
(#128541,#128542),(#128543,#128544),(#128545,#128546),(#128547,#128548),
(#128549,#128550),(#128551,#128552),(#128553,#128554),(#128555,#128556),
(#128557,#128558),(#128559,#128560),(#128561,#128562),(#128563,#128564),
(#128565,#128566),(#128567,#128568),(#128569,#128570),(#128571,#128572),
(#128573,#128574),(#128575,#128576),(#128577,#128578),(#128579,#128580),
(#128581,#128582),(#128583,#128584),(#128585,#128586),(#128587,#128588),
(#128589,#128590),(#128591,#128592),(#128593,#128594),(#128595,#128596),
(#128597,#128598),(#128599,#128600),(#128601,#128602),(#128603,#128604),
(#128605,#128606),(#128607,#128608),(#128609,#128610),(#128611,#128612),
(#128613,#128614),(#128615,#128616)),.UNSPECIFIED.,.F.,.F.,.F.)
B_SPLINE_SURFACE_WITH_KNOTS((6,1,1,1,1,1,1,1,1,1,1,1,1,1,1,1,1,1,1,1,1,
1,1,1,1,1,1,1,1,1,1,1,1,1,1,1,1,1,1,1,1,1,1,1,1,1,1,1,1,1,1,1,1,1,1,1,1,
1,1,1,1,1,1,1,1,1,1,1,1,1,1,1,1,1,1,1,1,1,1,1,1,1,1,1,1,1,1,1,1,1,1,1,1,
1,1,1,1,1,1,1,1,1,1,1,1,1,1,1,1,1,1,1,1,1,1,1,1,1,1,1,1,1,1,1,1,1,1,1,1,
1,1,1,1,1,1,1,1,1,1,1,1,1,1,1,1,1,1,1,1,1,1,1,1,1,1,1,1,1,1,1,1,1,1,1,1,
1,1,1,1,1,1,1,1,1,1,1,1,1,1,1,1,1,1,1,1,1,1,1,1,1,1,1,1,1,1,1,1,1,1,1,6),
(2,2),(-1.,-0.995000000000001,-0.990000000000001,-0.985000000000001,-0.980000000000001,
-0.975000000000001,-0.970000000000001,-0.965000000000001,-0.960000000000001,
-0.955000000000001,-0.950000000000001,-0.945000000000001,-0.940000000000001,
-0.935000000000001,-0.930000000000001,-0.925000000000001,-0.920000000000001,
-0.915000000000001,-0.910000000000001,-0.905000000000001,-0.900000000000001,
-0.895000000000001,-0.890000000000001,-0.885000000000001,-0.880000000000001,
-0.875000000000001,-0.870000000000001,-0.865000000000001,-0.860000000000001,
-0.855000000000001,-0.850000000000001,-0.845000000000001,-0.840000000000001,
-0.835000000000001,-0.830000000000001,-0.825000000000001,-0.820000000000001,
-0.815000000000001,-0.810000000000001,-0.805000000000001,-0.800000000000001,
-0.795000000000001,-0.790000000000001,-0.785000000000001,-0.780000000000001,
-0.775000000000001,-0.770000000000001,-0.765000000000001,-0.760000000000001,
-0.755000000000001,-0.750000000000001,-0.745000000000001,-0.740000000000001,
-0.735000000000001,-0.730000000000001,-0.725000000000001,-0.720000000000001,
-0.715000000000001,-0.710000000000001,-0.705000000000001,-0.700000000000001,
-0.695000000000001,-0.690000000000001,-0.685,-0.68,-0.675,-0.67,-0.665,
-0.66,-0.655,-0.65,-0.645,-0.64,-0.635,-0.63,-0.625,-0.62,-0.615,-0.61,
-0.605,-0.6,-0.595,-0.59,-0.585,-0.58,-0.575,-0.57,-0.565,-0.56,-0.555,
-0.55,-0.545,-0.54,-0.535,-0.53,-0.525,-0.52,-0.515,-0.51,-0.505,-0.5,-0.495,
-0.49,-0.485,-0.48,-0.475,-0.47,-0.465,-0.46,-0.455,-0.45,-0.445,-0.44,
-0.435,-0.43,-0.425,-0.42,-0.415,-0.41,-0.405,-0.4,-0.395,-0.39,-0.385,
-0.38,-0.375,-0.37,-0.365,-0.36,-0.355,-0.35,-0.345,-0.34,-0.335,-0.33,
-0.325,-0.32,-0.315,-0.31,-0.305,-0.3,-0.295,-0.29,-0.285,-0.28,-0.275,
-0.27,-0.265,-0.26,-0.255,-0.25,-0.245,-0.24,-0.235,-0.23,-0.225,-0.22,
-0.215,-0.21,-0.205,-0.2,-0.195,-0.19,-0.185,-0.18,-0.175,-0.17,-0.165,
-0.16,-0.155,-0.15,-0.145,-0.14,-0.135,-0.13,-0.125,-0.12,-0.115,-0.11,
-0.105,-0.1,-0.095,-0.09,-0.085,-0.08,-0.075,-0.07,-0.065,-0.06,-0.055,
-0.05,-0.045,-0.04,-0.035,-0.03,-0.025,-0.02,-0.015,-0.01,-0.005,0.),(0.,
1.2),.UNSPECIFIED.)
GEOMETRIC_REPRESENTATION_ITEM()
RATIONAL_B_SPLINE_SURFACE(((1.,1.),(1.,1.),(1.,1.),(1.,1.),(1.,1.),(1.,
1.),(1.,1.),(1.,1.),(1.,1.),(1.,1.),(1.,1.),(1.,1.),(1.,1.),(1.,1.),(1.,
1.),(1.,1.),(1.,1.),(1.,1.),(1.,1.),(1.,1.),(1.,1.),(1.,1.),(1.,1.),(1.,
1.),(1.,1.),(1.,1.),(1.,1.),(1.,1.),(1.,1.),(1.,1.),(1.,1.),(1.,1.),(1.,
1.),(1.,1.),(1.,1.),(1.,1.),(1.,1.),(1.,1.),(1.,1.),(1.,1.),(1.,1.),(1.,
1.),(1.,1.),(1.,1.),(1.,1.),(1.,1.),(1.,1.),(1.,1.),(1.,1.),(1.,1.),(1.,
1.),(1.,1.),(1.,1.),(1.,1.),(1.,1.),(1.,1.),(1.,1.),(1.,1.),(1.,1.),(1.,
1.),(1.,1.),(1.,1.),(1.,1.),(1.,1.),(1.,1.),(1.,1.),(1.,1.),(1.,1.),(1.,
1.),(1.,1.),(1.,1.),(1.,1.),(1.,1.),(1.,1.),(1.,1.),(1.,1.),(1.,1.),(1.,
1.),(1.,1.),(1.,1.),(1.,1.),(1.,1.),(1.,1.),(1.,1.),(1.,1.),(1.,1.),(1.,
1.),(1.,1.),(1.,1.),(1.,1.),(1.,1.),(1.,1.),(1.,1.),(1.,1.),(1.,1.),(1.,
1.),(1.,1.),(1.,1.),(1.,1.),(1.,1.),(1.,1.),(1.,1.),(1.,1.),(1.,1.),(1.,
1.),(1.,1.),(1.,1.),(1.,1.),(1.,1.),(1.,1.),(1.,1.),(1.,1.),(1.,1.),(1.,
1.),(1.,1.),(1.,1.),(1.,1.),(1.,1.),(1.,1.),(1.,1.),(1.,1.),(1.,1.),(1.,
1.),(1.,1.),(1.,1.),(1.,1.),(1.,1.),(1.,1.),(1.,1.),(1.,1.),(1.,1.),(1.,
1.),(1.,1.),(1.,1.),(1.,1.),(1.,1.),(1.,1.),(1.,1.),(1.,1.),(1.,1.),(1.,
1.),(1.,1.),(1.,1.),(1.,1.),(1.,1.),(1.,1.),(1.,1.),(1.,1.),(1.,1.),(1.,
1.),(1.,1.),(1.,1.),(1.,1.),(1.,1.),(1.,1.),(1.,1.),(1.,1.),(1.,1.),(1.,
1.),(1.,1.),(1.,1.),(1.,1.),(1.,1.),(1.,1.),(1.,1.),(1.,1.),(1.,1.),(1.,
1.),(1.,1.),(1.,1.),(1.,1.),(1.,1.),(1.,1.),(1.,1.),(1.,1.),(1.,1.),(1.,
1.),(1.,1.),(1.,1.),(1.,1.),(1.,1.),(1.,1.),(1.,1.),(1.,1.),(1.,1.),(1.,
1.),(1.,1.),(1.,1.),(1.,1.),(1.,1.),(1.,1.),(1.,1.),(1.,1.),(1.,1.),(1.,
1.),(1.,1.),(1.,1.),(1.,1.),(1.,1.),(1.,1.),(1.,1.),(1.,1.),(1.,1.),(1.,
1.),(1.,1.)))
REPRESENTATION_ITEM('')
SURFACE()
);
#970=(
BOUNDED_SURFACE()
B_SPLINE_SURFACE(5,1,((#129008,#129009),(#129010,#129011),(#129012,#129013),
(#129014,#129015),(#129016,#129017),(#129018,#129019),(#129020,#129021),
(#129022,#129023),(#129024,#129025),(#129026,#129027),(#129028,#129029),
(#129030,#129031),(#129032,#129033),(#129034,#129035),(#129036,#129037),
(#129038,#129039),(#129040,#129041),(#129042,#129043),(#129044,#129045),
(#129046,#129047),(#129048,#129049),(#129050,#129051),(#129052,#129053),
(#129054,#129055),(#129056,#129057),(#129058,#129059),(#129060,#129061),
(#129062,#129063),(#129064,#129065),(#129066,#129067),(#129068,#129069),
(#129070,#129071),(#129072,#129073),(#129074,#129075),(#129076,#129077),
(#129078,#129079),(#129080,#129081),(#129082,#129083),(#129084,#129085),
(#129086,#129087),(#129088,#129089),(#129090,#129091),(#129092,#129093),
(#129094,#129095),(#129096,#129097),(#129098,#129099),(#129100,#129101),
(#129102,#129103),(#129104,#129105),(#129106,#129107),(#129108,#129109),
(#129110,#129111),(#129112,#129113),(#129114,#129115),(#129116,#129117),
(#129118,#129119),(#129120,#129121),(#129122,#129123),(#129124,#129125),
(#129126,#129127),(#129128,#129129),(#129130,#129131),(#129132,#129133),
(#129134,#129135),(#129136,#129137),(#129138,#129139),(#129140,#129141),
(#129142,#129143),(#129144,#129145),(#129146,#129147),(#129148,#129149),
(#129150,#129151),(#129152,#129153),(#129154,#129155),(#129156,#129157),
(#129158,#129159),(#129160,#129161),(#129162,#129163),(#129164,#129165),
(#129166,#129167),(#129168,#129169),(#129170,#129171),(#129172,#129173),
(#129174,#129175),(#129176,#129177),(#129178,#129179),(#129180,#129181),
(#129182,#129183),(#129184,#129185),(#129186,#129187),(#129188,#129189),
(#129190,#129191),(#129192,#129193),(#129194,#129195),(#129196,#129197),
(#129198,#129199),(#129200,#129201),(#129202,#129203),(#129204,#129205),
(#129206,#129207),(#129208,#129209),(#129210,#129211),(#129212,#129213),
(#129214,#129215),(#129216,#129217),(#129218,#129219),(#129220,#129221),
(#129222,#129223),(#129224,#129225),(#129226,#129227),(#129228,#129229),
(#129230,#129231),(#129232,#129233),(#129234,#129235),(#129236,#129237),
(#129238,#129239),(#129240,#129241),(#129242,#129243),(#129244,#129245),
(#129246,#129247),(#129248,#129249),(#129250,#129251),(#129252,#129253),
(#129254,#129255),(#129256,#129257),(#129258,#129259),(#129260,#129261),
(#129262,#129263),(#129264,#129265),(#129266,#129267),(#129268,#129269),
(#129270,#129271),(#129272,#129273),(#129274,#129275),(#129276,#129277),
(#129278,#129279),(#129280,#129281),(#129282,#129283),(#129284,#129285),
(#129286,#129287),(#129288,#129289),(#129290,#129291),(#129292,#129293),
(#129294,#129295),(#129296,#129297),(#129298,#129299),(#129300,#129301),
(#129302,#129303),(#129304,#129305),(#129306,#129307),(#129308,#129309),
(#129310,#129311),(#129312,#129313),(#129314,#129315),(#129316,#129317),
(#129318,#129319),(#129320,#129321),(#129322,#129323),(#129324,#129325),
(#129326,#129327),(#129328,#129329),(#129330,#129331),(#129332,#129333),
(#129334,#129335),(#129336,#129337),(#129338,#129339),(#129340,#129341),
(#129342,#129343),(#129344,#129345),(#129346,#129347),(#129348,#129349),
(#129350,#129351),(#129352,#129353),(#129354,#129355),(#129356,#129357),
(#129358,#129359),(#129360,#129361),(#129362,#129363),(#129364,#129365),
(#129366,#129367),(#129368,#129369),(#129370,#129371),(#129372,#129373),
(#129374,#129375),(#129376,#129377),(#129378,#129379),(#129380,#129381),
(#129382,#129383),(#129384,#129385),(#129386,#129387),(#129388,#129389),
(#129390,#129391),(#129392,#129393),(#129394,#129395),(#129396,#129397),
(#129398,#129399),(#129400,#129401),(#129402,#129403),(#129404,#129405),
(#129406,#129407),(#129408,#129409),(#129410,#129411),(#129412,#129413),
(#129414,#129415),(#129416,#129417)),.UNSPECIFIED.,.F.,.F.,.F.)
B_SPLINE_SURFACE_WITH_KNOTS((6,1,1,1,1,1,1,1,1,1,1,1,1,1,1,1,1,1,1,1,1,
1,1,1,1,1,1,1,1,1,1,1,1,1,1,1,1,1,1,1,1,1,1,1,1,1,1,1,1,1,1,1,1,1,1,1,1,
1,1,1,1,1,1,1,1,1,1,1,1,1,1,1,1,1,1,1,1,1,1,1,1,1,1,1,1,1,1,1,1,1,1,1,1,
1,1,1,1,1,1,1,1,1,1,1,1,1,1,1,1,1,1,1,1,1,1,1,1,1,1,1,1,1,1,1,1,1,1,1,1,
1,1,1,1,1,1,1,1,1,1,1,1,1,1,1,1,1,1,1,1,1,1,1,1,1,1,1,1,1,1,1,1,1,1,1,1,
1,1,1,1,1,1,1,1,1,1,1,1,1,1,1,1,1,1,1,1,1,1,1,1,1,1,1,1,1,1,1,1,1,1,1,6),
(2,2),(-1.,-0.995000000000001,-0.990000000000001,-0.985000000000001,-0.980000000000001,
-0.975000000000001,-0.970000000000001,-0.965000000000001,-0.960000000000001,
-0.955000000000001,-0.950000000000001,-0.945000000000001,-0.940000000000001,
-0.935000000000001,-0.930000000000001,-0.925000000000001,-0.920000000000001,
-0.915000000000001,-0.910000000000001,-0.905000000000001,-0.900000000000001,
-0.895000000000001,-0.890000000000001,-0.885000000000001,-0.880000000000001,
-0.875000000000001,-0.870000000000001,-0.865000000000001,-0.860000000000001,
-0.855000000000001,-0.850000000000001,-0.845000000000001,-0.840000000000001,
-0.835000000000001,-0.830000000000001,-0.825000000000001,-0.820000000000001,
-0.815000000000001,-0.810000000000001,-0.805000000000001,-0.800000000000001,
-0.795000000000001,-0.790000000000001,-0.785000000000001,-0.780000000000001,
-0.775000000000001,-0.770000000000001,-0.765000000000001,-0.760000000000001,
-0.755000000000001,-0.750000000000001,-0.745000000000001,-0.740000000000001,
-0.735000000000001,-0.730000000000001,-0.725000000000001,-0.720000000000001,
-0.715000000000001,-0.710000000000001,-0.705000000000001,-0.700000000000001,
-0.695000000000001,-0.690000000000001,-0.685,-0.68,-0.675,-0.67,-0.665,
-0.66,-0.655,-0.65,-0.645,-0.64,-0.635,-0.63,-0.625,-0.62,-0.615,-0.61,
-0.605,-0.6,-0.595,-0.59,-0.585,-0.58,-0.575,-0.57,-0.565,-0.56,-0.555,
-0.55,-0.545,-0.54,-0.535,-0.53,-0.525,-0.52,-0.515,-0.51,-0.505,-0.5,-0.495,
-0.49,-0.485,-0.48,-0.475,-0.47,-0.465,-0.46,-0.455,-0.45,-0.445,-0.44,
-0.435,-0.43,-0.425,-0.42,-0.415,-0.41,-0.405,-0.4,-0.395,-0.39,-0.385,
-0.38,-0.375,-0.37,-0.365,-0.36,-0.355,-0.35,-0.345,-0.34,-0.335,-0.33,
-0.325,-0.32,-0.315,-0.31,-0.305,-0.3,-0.295,-0.29,-0.285,-0.28,-0.275,
-0.27,-0.265,-0.26,-0.255,-0.25,-0.245,-0.24,-0.235,-0.23,-0.225,-0.22,
-0.215,-0.21,-0.205,-0.2,-0.195,-0.19,-0.185,-0.18,-0.175,-0.17,-0.165,
-0.16,-0.155,-0.15,-0.145,-0.14,-0.135,-0.13,-0.125,-0.12,-0.115,-0.11,
-0.105,-0.1,-0.095,-0.09,-0.085,-0.08,-0.075,-0.07,-0.065,-0.06,-0.055,
-0.05,-0.045,-0.04,-0.035,-0.03,-0.025,-0.02,-0.015,-0.01,-0.005,0.),(0.,
1.2),.UNSPECIFIED.)
GEOMETRIC_REPRESENTATION_ITEM()
RATIONAL_B_SPLINE_SURFACE(((1.,1.),(1.,1.),(1.,1.),(1.,1.),(1.,1.),(1.,
1.),(1.,1.),(1.,1.),(1.,1.),(1.,1.),(1.,1.),(1.,1.),(1.,1.),(1.,1.),(1.,
1.),(1.,1.),(1.,1.),(1.,1.),(1.,1.),(1.,1.),(1.,1.),(1.,1.),(1.,1.),(1.,
1.),(1.,1.),(1.,1.),(1.,1.),(1.,1.),(1.,1.),(1.,1.),(1.,1.),(1.,1.),(1.,
1.),(1.,1.),(1.,1.),(1.,1.),(1.,1.),(1.,1.),(1.,1.),(1.,1.),(1.,1.),(1.,
1.),(1.,1.),(1.,1.),(1.,1.),(1.,1.),(1.,1.),(1.,1.),(1.,1.),(1.,1.),(1.,
1.),(1.,1.),(1.,1.),(1.,1.),(1.,1.),(1.,1.),(1.,1.),(1.,1.),(1.,1.),(1.,
1.),(1.,1.),(1.,1.),(1.,1.),(1.,1.),(1.,1.),(1.,1.),(1.,1.),(1.,1.),(1.,
1.),(1.,1.),(1.,1.),(1.,1.),(1.,1.),(1.,1.),(1.,1.),(1.,1.),(1.,1.),(1.,
1.),(1.,1.),(1.,1.),(1.,1.),(1.,1.),(1.,1.),(1.,1.),(1.,1.),(1.,1.),(1.,
1.),(1.,1.),(1.,1.),(1.,1.),(1.,1.),(1.,1.),(1.,1.),(1.,1.),(1.,1.),(1.,
1.),(1.,1.),(1.,1.),(1.,1.),(1.,1.),(1.,1.),(1.,1.),(1.,1.),(1.,1.),(1.,
1.),(1.,1.),(1.,1.),(1.,1.),(1.,1.),(1.,1.),(1.,1.),(1.,1.),(1.,1.),(1.,
1.),(1.,1.),(1.,1.),(1.,1.),(1.,1.),(1.,1.),(1.,1.),(1.,1.),(1.,1.),(1.,
1.),(1.,1.),(1.,1.),(1.,1.),(1.,1.),(1.,1.),(1.,1.),(1.,1.),(1.,1.),(1.,
1.),(1.,1.),(1.,1.),(1.,1.),(1.,1.),(1.,1.),(1.,1.),(1.,1.),(1.,1.),(1.,
1.),(1.,1.),(1.,1.),(1.,1.),(1.,1.),(1.,1.),(1.,1.),(1.,1.),(1.,1.),(1.,
1.),(1.,1.),(1.,1.),(1.,1.),(1.,1.),(1.,1.),(1.,1.),(1.,1.),(1.,1.),(1.,
1.),(1.,1.),(1.,1.),(1.,1.),(1.,1.),(1.,1.),(1.,1.),(1.,1.),(1.,1.),(1.,
1.),(1.,1.),(1.,1.),(1.,1.),(1.,1.),(1.,1.),(1.,1.),(1.,1.),(1.,1.),(1.,
1.),(1.,1.),(1.,1.),(1.,1.),(1.,1.),(1.,1.),(1.,1.),(1.,1.),(1.,1.),(1.,
1.),(1.,1.),(1.,1.),(1.,1.),(1.,1.),(1.,1.),(1.,1.),(1.,1.),(1.,1.),(1.,
1.),(1.,1.),(1.,1.),(1.,1.),(1.,1.),(1.,1.),(1.,1.),(1.,1.),(1.,1.),(1.,
1.),(1.,1.)))
REPRESENTATION_ITEM('')
SURFACE()
);
#971=(
BOUNDED_SURFACE()
B_SPLINE_SURFACE(5,1,((#129809,#129810),(#129811,#129812),(#129813,#129814),
(#129815,#129816),(#129817,#129818),(#129819,#129820),(#129821,#129822),
(#129823,#129824),(#129825,#129826),(#129827,#129828),(#129829,#129830),
(#129831,#129832),(#129833,#129834),(#129835,#129836),(#129837,#129838),
(#129839,#129840),(#129841,#129842),(#129843,#129844),(#129845,#129846),
(#129847,#129848),(#129849,#129850),(#129851,#129852),(#129853,#129854),
(#129855,#129856),(#129857,#129858),(#129859,#129860),(#129861,#129862),
(#129863,#129864),(#129865,#129866),(#129867,#129868),(#129869,#129870),
(#129871,#129872),(#129873,#129874),(#129875,#129876),(#129877,#129878),
(#129879,#129880),(#129881,#129882),(#129883,#129884),(#129885,#129886),
(#129887,#129888),(#129889,#129890),(#129891,#129892),(#129893,#129894),
(#129895,#129896),(#129897,#129898),(#129899,#129900),(#129901,#129902),
(#129903,#129904),(#129905,#129906),(#129907,#129908),(#129909,#129910),
(#129911,#129912),(#129913,#129914),(#129915,#129916),(#129917,#129918),
(#129919,#129920),(#129921,#129922),(#129923,#129924),(#129925,#129926),
(#129927,#129928),(#129929,#129930),(#129931,#129932),(#129933,#129934),
(#129935,#129936),(#129937,#129938),(#129939,#129940),(#129941,#129942),
(#129943,#129944),(#129945,#129946),(#129947,#129948),(#129949,#129950),
(#129951,#129952),(#129953,#129954),(#129955,#129956),(#129957,#129958),
(#129959,#129960),(#129961,#129962),(#129963,#129964),(#129965,#129966),
(#129967,#129968),(#129969,#129970),(#129971,#129972),(#129973,#129974),
(#129975,#129976),(#129977,#129978),(#129979,#129980),(#129981,#129982),
(#129983,#129984),(#129985,#129986),(#129987,#129988),(#129989,#129990),
(#129991,#129992),(#129993,#129994),(#129995,#129996),(#129997,#129998),
(#129999,#130000),(#130001,#130002),(#130003,#130004),(#130005,#130006),
(#130007,#130008),(#130009,#130010),(#130011,#130012),(#130013,#130014),
(#130015,#130016),(#130017,#130018),(#130019,#130020),(#130021,#130022),
(#130023,#130024),(#130025,#130026),(#130027,#130028),(#130029,#130030),
(#130031,#130032),(#130033,#130034),(#130035,#130036),(#130037,#130038),
(#130039,#130040),(#130041,#130042),(#130043,#130044),(#130045,#130046),
(#130047,#130048),(#130049,#130050),(#130051,#130052),(#130053,#130054),
(#130055,#130056),(#130057,#130058),(#130059,#130060),(#130061,#130062),
(#130063,#130064),(#130065,#130066),(#130067,#130068),(#130069,#130070),
(#130071,#130072),(#130073,#130074),(#130075,#130076),(#130077,#130078),
(#130079,#130080),(#130081,#130082),(#130083,#130084),(#130085,#130086),
(#130087,#130088),(#130089,#130090),(#130091,#130092),(#130093,#130094),
(#130095,#130096),(#130097,#130098),(#130099,#130100),(#130101,#130102),
(#130103,#130104),(#130105,#130106),(#130107,#130108),(#130109,#130110),
(#130111,#130112),(#130113,#130114),(#130115,#130116),(#130117,#130118),
(#130119,#130120),(#130121,#130122),(#130123,#130124),(#130125,#130126),
(#130127,#130128),(#130129,#130130),(#130131,#130132),(#130133,#130134),
(#130135,#130136),(#130137,#130138),(#130139,#130140),(#130141,#130142),
(#130143,#130144),(#130145,#130146),(#130147,#130148),(#130149,#130150),
(#130151,#130152),(#130153,#130154),(#130155,#130156),(#130157,#130158),
(#130159,#130160),(#130161,#130162),(#130163,#130164),(#130165,#130166),
(#130167,#130168),(#130169,#130170),(#130171,#130172),(#130173,#130174),
(#130175,#130176),(#130177,#130178),(#130179,#130180),(#130181,#130182),
(#130183,#130184),(#130185,#130186),(#130187,#130188),(#130189,#130190),
(#130191,#130192),(#130193,#130194),(#130195,#130196),(#130197,#130198),
(#130199,#130200),(#130201,#130202),(#130203,#130204),(#130205,#130206),
(#130207,#130208),(#130209,#130210),(#130211,#130212),(#130213,#130214),
(#130215,#130216),(#130217,#130218)),.UNSPECIFIED.,.F.,.F.,.F.)
B_SPLINE_SURFACE_WITH_KNOTS((6,1,1,1,1,1,1,1,1,1,1,1,1,1,1,1,1,1,1,1,1,
1,1,1,1,1,1,1,1,1,1,1,1,1,1,1,1,1,1,1,1,1,1,1,1,1,1,1,1,1,1,1,1,1,1,1,1,
1,1,1,1,1,1,1,1,1,1,1,1,1,1,1,1,1,1,1,1,1,1,1,1,1,1,1,1,1,1,1,1,1,1,1,1,
1,1,1,1,1,1,1,1,1,1,1,1,1,1,1,1,1,1,1,1,1,1,1,1,1,1,1,1,1,1,1,1,1,1,1,1,
1,1,1,1,1,1,1,1,1,1,1,1,1,1,1,1,1,1,1,1,1,1,1,1,1,1,1,1,1,1,1,1,1,1,1,1,
1,1,1,1,1,1,1,1,1,1,1,1,1,1,1,1,1,1,1,1,1,1,1,1,1,1,1,1,1,1,1,1,1,1,1,6),
(2,2),(-1.,-0.995000000000001,-0.990000000000001,-0.985000000000001,-0.980000000000001,
-0.975000000000001,-0.970000000000001,-0.965000000000001,-0.960000000000001,
-0.955000000000001,-0.950000000000001,-0.945000000000001,-0.940000000000001,
-0.935000000000001,-0.930000000000001,-0.925000000000001,-0.920000000000001,
-0.915000000000001,-0.910000000000001,-0.905000000000001,-0.900000000000001,
-0.895000000000001,-0.890000000000001,-0.885000000000001,-0.880000000000001,
-0.875000000000001,-0.870000000000001,-0.865000000000001,-0.860000000000001,
-0.855000000000001,-0.850000000000001,-0.845000000000001,-0.840000000000001,
-0.835000000000001,-0.830000000000001,-0.825000000000001,-0.820000000000001,
-0.815000000000001,-0.810000000000001,-0.805000000000001,-0.800000000000001,
-0.795000000000001,-0.790000000000001,-0.785000000000001,-0.780000000000001,
-0.775000000000001,-0.770000000000001,-0.765000000000001,-0.760000000000001,
-0.755000000000001,-0.750000000000001,-0.745000000000001,-0.740000000000001,
-0.735000000000001,-0.730000000000001,-0.725000000000001,-0.720000000000001,
-0.715000000000001,-0.710000000000001,-0.705000000000001,-0.700000000000001,
-0.695000000000001,-0.690000000000001,-0.685,-0.68,-0.675,-0.67,-0.665,
-0.66,-0.655,-0.65,-0.645,-0.64,-0.635,-0.63,-0.625,-0.62,-0.615,-0.61,
-0.605,-0.6,-0.595,-0.59,-0.585,-0.58,-0.575,-0.57,-0.565,-0.56,-0.555,
-0.55,-0.545,-0.54,-0.535,-0.53,-0.525,-0.52,-0.515,-0.51,-0.505,-0.5,-0.495,
-0.49,-0.485,-0.48,-0.475,-0.47,-0.465,-0.46,-0.455,-0.45,-0.445,-0.44,
-0.435,-0.43,-0.425,-0.42,-0.415,-0.41,-0.405,-0.4,-0.395,-0.39,-0.385,
-0.38,-0.375,-0.37,-0.365,-0.36,-0.355,-0.35,-0.345,-0.34,-0.335,-0.33,
-0.325,-0.32,-0.315,-0.31,-0.305,-0.3,-0.295,-0.29,-0.285,-0.28,-0.275,
-0.27,-0.265,-0.26,-0.255,-0.25,-0.245,-0.24,-0.235,-0.23,-0.225,-0.22,
-0.215,-0.21,-0.205,-0.2,-0.195,-0.19,-0.185,-0.18,-0.175,-0.17,-0.165,
-0.16,-0.155,-0.15,-0.145,-0.14,-0.135,-0.13,-0.125,-0.12,-0.115,-0.11,
-0.105,-0.1,-0.095,-0.09,-0.085,-0.08,-0.075,-0.07,-0.065,-0.06,-0.055,
-0.05,-0.045,-0.04,-0.035,-0.03,-0.025,-0.02,-0.015,-0.01,-0.005,0.),(0.,
1.2),.UNSPECIFIED.)
GEOMETRIC_REPRESENTATION_ITEM()
RATIONAL_B_SPLINE_SURFACE(((1.,1.),(1.,1.),(1.,1.),(1.,1.),(1.,1.),(1.,
1.),(1.,1.),(1.,1.),(1.,1.),(1.,1.),(1.,1.),(1.,1.),(1.,1.),(1.,1.),(1.,
1.),(1.,1.),(1.,1.),(1.,1.),(1.,1.),(1.,1.),(1.,1.),(1.,1.),(1.,1.),(1.,
1.),(1.,1.),(1.,1.),(1.,1.),(1.,1.),(1.,1.),(1.,1.),(1.,1.),(1.,1.),(1.,
1.),(1.,1.),(1.,1.),(1.,1.),(1.,1.),(1.,1.),(1.,1.),(1.,1.),(1.,1.),(1.,
1.),(1.,1.),(1.,1.),(1.,1.),(1.,1.),(1.,1.),(1.,1.),(1.,1.),(1.,1.),(1.,
1.),(1.,1.),(1.,1.),(1.,1.),(1.,1.),(1.,1.),(1.,1.),(1.,1.),(1.,1.),(1.,
1.),(1.,1.),(1.,1.),(1.,1.),(1.,1.),(1.,1.),(1.,1.),(1.,1.),(1.,1.),(1.,
1.),(1.,1.),(1.,1.),(1.,1.),(1.,1.),(1.,1.),(1.,1.),(1.,1.),(1.,1.),(1.,
1.),(1.,1.),(1.,1.),(1.,1.),(1.,1.),(1.,1.),(1.,1.),(1.,1.),(1.,1.),(1.,
1.),(1.,1.),(1.,1.),(1.,1.),(1.,1.),(1.,1.),(1.,1.),(1.,1.),(1.,1.),(1.,
1.),(1.,1.),(1.,1.),(1.,1.),(1.,1.),(1.,1.),(1.,1.),(1.,1.),(1.,1.),(1.,
1.),(1.,1.),(1.,1.),(1.,1.),(1.,1.),(1.,1.),(1.,1.),(1.,1.),(1.,1.),(1.,
1.),(1.,1.),(1.,1.),(1.,1.),(1.,1.),(1.,1.),(1.,1.),(1.,1.),(1.,1.),(1.,
1.),(1.,1.),(1.,1.),(1.,1.),(1.,1.),(1.,1.),(1.,1.),(1.,1.),(1.,1.),(1.,
1.),(1.,1.),(1.,1.),(1.,1.),(1.,1.),(1.,1.),(1.,1.),(1.,1.),(1.,1.),(1.,
1.),(1.,1.),(1.,1.),(1.,1.),(1.,1.),(1.,1.),(1.,1.),(1.,1.),(1.,1.),(1.,
1.),(1.,1.),(1.,1.),(1.,1.),(1.,1.),(1.,1.),(1.,1.),(1.,1.),(1.,1.),(1.,
1.),(1.,1.),(1.,1.),(1.,1.),(1.,1.),(1.,1.),(1.,1.),(1.,1.),(1.,1.),(1.,
1.),(1.,1.),(1.,1.),(1.,1.),(1.,1.),(1.,1.),(1.,1.),(1.,1.),(1.,1.),(1.,
1.),(1.,1.),(1.,1.),(1.,1.),(1.,1.),(1.,1.),(1.,1.),(1.,1.),(1.,1.),(1.,
1.),(1.,1.),(1.,1.),(1.,1.),(1.,1.),(1.,1.),(1.,1.),(1.,1.),(1.,1.),(1.,
1.),(1.,1.),(1.,1.),(1.,1.),(1.,1.),(1.,1.),(1.,1.),(1.,1.),(1.,1.),(1.,
1.),(1.,1.)))
REPRESENTATION_ITEM('')
SURFACE()
);
#972=(
BOUNDED_SURFACE()
B_SPLINE_SURFACE(5,1,((#130610,#130611),(#130612,#130613),(#130614,#130615),
(#130616,#130617),(#130618,#130619),(#130620,#130621),(#130622,#130623),
(#130624,#130625),(#130626,#130627),(#130628,#130629),(#130630,#130631),
(#130632,#130633),(#130634,#130635),(#130636,#130637),(#130638,#130639),
(#130640,#130641),(#130642,#130643),(#130644,#130645),(#130646,#130647),
(#130648,#130649),(#130650,#130651),(#130652,#130653),(#130654,#130655),
(#130656,#130657),(#130658,#130659),(#130660,#130661),(#130662,#130663),
(#130664,#130665),(#130666,#130667),(#130668,#130669),(#130670,#130671),
(#130672,#130673),(#130674,#130675),(#130676,#130677),(#130678,#130679),
(#130680,#130681),(#130682,#130683),(#130684,#130685),(#130686,#130687),
(#130688,#130689),(#130690,#130691),(#130692,#130693),(#130694,#130695),
(#130696,#130697),(#130698,#130699),(#130700,#130701),(#130702,#130703),
(#130704,#130705),(#130706,#130707),(#130708,#130709),(#130710,#130711),
(#130712,#130713),(#130714,#130715),(#130716,#130717),(#130718,#130719),
(#130720,#130721),(#130722,#130723),(#130724,#130725),(#130726,#130727),
(#130728,#130729),(#130730,#130731),(#130732,#130733),(#130734,#130735),
(#130736,#130737),(#130738,#130739),(#130740,#130741),(#130742,#130743),
(#130744,#130745),(#130746,#130747),(#130748,#130749),(#130750,#130751),
(#130752,#130753),(#130754,#130755),(#130756,#130757),(#130758,#130759),
(#130760,#130761),(#130762,#130763),(#130764,#130765),(#130766,#130767),
(#130768,#130769),(#130770,#130771),(#130772,#130773),(#130774,#130775),
(#130776,#130777),(#130778,#130779),(#130780,#130781),(#130782,#130783),
(#130784,#130785),(#130786,#130787),(#130788,#130789),(#130790,#130791),
(#130792,#130793),(#130794,#130795),(#130796,#130797),(#130798,#130799),
(#130800,#130801),(#130802,#130803),(#130804,#130805),(#130806,#130807),
(#130808,#130809),(#130810,#130811),(#130812,#130813),(#130814,#130815),
(#130816,#130817),(#130818,#130819),(#130820,#130821),(#130822,#130823),
(#130824,#130825),(#130826,#130827),(#130828,#130829),(#130830,#130831),
(#130832,#130833),(#130834,#130835),(#130836,#130837),(#130838,#130839),
(#130840,#130841),(#130842,#130843),(#130844,#130845),(#130846,#130847),
(#130848,#130849),(#130850,#130851),(#130852,#130853),(#130854,#130855),
(#130856,#130857),(#130858,#130859),(#130860,#130861),(#130862,#130863),
(#130864,#130865),(#130866,#130867),(#130868,#130869),(#130870,#130871),
(#130872,#130873),(#130874,#130875),(#130876,#130877),(#130878,#130879),
(#130880,#130881),(#130882,#130883),(#130884,#130885),(#130886,#130887),
(#130888,#130889),(#130890,#130891),(#130892,#130893),(#130894,#130895),
(#130896,#130897),(#130898,#130899),(#130900,#130901),(#130902,#130903),
(#130904,#130905),(#130906,#130907),(#130908,#130909),(#130910,#130911),
(#130912,#130913),(#130914,#130915),(#130916,#130917),(#130918,#130919),
(#130920,#130921),(#130922,#130923),(#130924,#130925),(#130926,#130927),
(#130928,#130929),(#130930,#130931),(#130932,#130933),(#130934,#130935),
(#130936,#130937),(#130938,#130939),(#130940,#130941),(#130942,#130943),
(#130944,#130945),(#130946,#130947),(#130948,#130949),(#130950,#130951),
(#130952,#130953),(#130954,#130955),(#130956,#130957),(#130958,#130959),
(#130960,#130961),(#130962,#130963),(#130964,#130965),(#130966,#130967),
(#130968,#130969),(#130970,#130971),(#130972,#130973),(#130974,#130975),
(#130976,#130977),(#130978,#130979),(#130980,#130981),(#130982,#130983),
(#130984,#130985),(#130986,#130987),(#130988,#130989),(#130990,#130991),
(#130992,#130993),(#130994,#130995),(#130996,#130997),(#130998,#130999),
(#131000,#131001),(#131002,#131003),(#131004,#131005),(#131006,#131007),
(#131008,#131009),(#131010,#131011),(#131012,#131013),(#131014,#131015),
(#131016,#131017),(#131018,#131019)),.UNSPECIFIED.,.F.,.F.,.F.)
B_SPLINE_SURFACE_WITH_KNOTS((6,1,1,1,1,1,1,1,1,1,1,1,1,1,1,1,1,1,1,1,1,
1,1,1,1,1,1,1,1,1,1,1,1,1,1,1,1,1,1,1,1,1,1,1,1,1,1,1,1,1,1,1,1,1,1,1,1,
1,1,1,1,1,1,1,1,1,1,1,1,1,1,1,1,1,1,1,1,1,1,1,1,1,1,1,1,1,1,1,1,1,1,1,1,
1,1,1,1,1,1,1,1,1,1,1,1,1,1,1,1,1,1,1,1,1,1,1,1,1,1,1,1,1,1,1,1,1,1,1,1,
1,1,1,1,1,1,1,1,1,1,1,1,1,1,1,1,1,1,1,1,1,1,1,1,1,1,1,1,1,1,1,1,1,1,1,1,
1,1,1,1,1,1,1,1,1,1,1,1,1,1,1,1,1,1,1,1,1,1,1,1,1,1,1,1,1,1,1,1,1,1,1,6),
(2,2),(-1.,-0.995000000000001,-0.990000000000001,-0.985000000000001,-0.980000000000001,
-0.975000000000001,-0.970000000000001,-0.965000000000001,-0.960000000000001,
-0.955000000000001,-0.950000000000001,-0.945000000000001,-0.940000000000001,
-0.935000000000001,-0.930000000000001,-0.925000000000001,-0.920000000000001,
-0.915000000000001,-0.910000000000001,-0.905000000000001,-0.900000000000001,
-0.895000000000001,-0.890000000000001,-0.885000000000001,-0.880000000000001,
-0.875000000000001,-0.870000000000001,-0.865000000000001,-0.860000000000001,
-0.855000000000001,-0.850000000000001,-0.845000000000001,-0.840000000000001,
-0.835000000000001,-0.830000000000001,-0.825000000000001,-0.820000000000001,
-0.815000000000001,-0.810000000000001,-0.805000000000001,-0.800000000000001,
-0.795000000000001,-0.790000000000001,-0.785000000000001,-0.780000000000001,
-0.775000000000001,-0.770000000000001,-0.765000000000001,-0.760000000000001,
-0.755000000000001,-0.750000000000001,-0.745000000000001,-0.740000000000001,
-0.735000000000001,-0.730000000000001,-0.725000000000001,-0.720000000000001,
-0.715000000000001,-0.710000000000001,-0.705000000000001,-0.700000000000001,
-0.695000000000001,-0.690000000000001,-0.685,-0.68,-0.675,-0.67,-0.665,
-0.66,-0.655,-0.65,-0.645,-0.64,-0.635,-0.63,-0.625,-0.62,-0.615,-0.61,
-0.605,-0.6,-0.595,-0.59,-0.585,-0.58,-0.575,-0.57,-0.565,-0.56,-0.555,
-0.55,-0.545,-0.54,-0.535,-0.53,-0.525,-0.52,-0.515,-0.51,-0.505,-0.5,-0.495,
-0.49,-0.485,-0.48,-0.475,-0.47,-0.465,-0.46,-0.455,-0.45,-0.445,-0.44,
-0.435,-0.43,-0.425,-0.42,-0.415,-0.41,-0.405,-0.4,-0.395,-0.39,-0.385,
-0.38,-0.375,-0.37,-0.365,-0.36,-0.355,-0.35,-0.345,-0.34,-0.335,-0.33,
-0.325,-0.32,-0.315,-0.31,-0.305,-0.3,-0.295,-0.29,-0.285,-0.28,-0.275,
-0.27,-0.265,-0.26,-0.255,-0.25,-0.245,-0.24,-0.235,-0.23,-0.225,-0.22,
-0.215,-0.21,-0.205,-0.2,-0.195,-0.19,-0.185,-0.18,-0.175,-0.17,-0.165,
-0.16,-0.155,-0.15,-0.145,-0.14,-0.135,-0.13,-0.125,-0.12,-0.115,-0.11,
-0.105,-0.1,-0.095,-0.09,-0.085,-0.08,-0.075,-0.07,-0.065,-0.06,-0.055,
-0.05,-0.045,-0.04,-0.035,-0.03,-0.025,-0.02,-0.015,-0.01,-0.005,0.),(0.,
1.2),.UNSPECIFIED.)
GEOMETRIC_REPRESENTATION_ITEM()
RATIONAL_B_SPLINE_SURFACE(((1.,1.),(1.,1.),(1.,1.),(1.,1.),(1.,1.),(1.,
1.),(1.,1.),(1.,1.),(1.,1.),(1.,1.),(1.,1.),(1.,1.),(1.,1.),(1.,1.),(1.,
1.),(1.,1.),(1.,1.),(1.,1.),(1.,1.),(1.,1.),(1.,1.),(1.,1.),(1.,1.),(1.,
1.),(1.,1.),(1.,1.),(1.,1.),(1.,1.),(1.,1.),(1.,1.),(1.,1.),(1.,1.),(1.,
1.),(1.,1.),(1.,1.),(1.,1.),(1.,1.),(1.,1.),(1.,1.),(1.,1.),(1.,1.),(1.,
1.),(1.,1.),(1.,1.),(1.,1.),(1.,1.),(1.,1.),(1.,1.),(1.,1.),(1.,1.),(1.,
1.),(1.,1.),(1.,1.),(1.,1.),(1.,1.),(1.,1.),(1.,1.),(1.,1.),(1.,1.),(1.,
1.),(1.,1.),(1.,1.),(1.,1.),(1.,1.),(1.,1.),(1.,1.),(1.,1.),(1.,1.),(1.,
1.),(1.,1.),(1.,1.),(1.,1.),(1.,1.),(1.,1.),(1.,1.),(1.,1.),(1.,1.),(1.,
1.),(1.,1.),(1.,1.),(1.,1.),(1.,1.),(1.,1.),(1.,1.),(1.,1.),(1.,1.),(1.,
1.),(1.,1.),(1.,1.),(1.,1.),(1.,1.),(1.,1.),(1.,1.),(1.,1.),(1.,1.),(1.,
1.),(1.,1.),(1.,1.),(1.,1.),(1.,1.),(1.,1.),(1.,1.),(1.,1.),(1.,1.),(1.,
1.),(1.,1.),(1.,1.),(1.,1.),(1.,1.),(1.,1.),(1.,1.),(1.,1.),(1.,1.),(1.,
1.),(1.,1.),(1.,1.),(1.,1.),(1.,1.),(1.,1.),(1.,1.),(1.,1.),(1.,1.),(1.,
1.),(1.,1.),(1.,1.),(1.,1.),(1.,1.),(1.,1.),(1.,1.),(1.,1.),(1.,1.),(1.,
1.),(1.,1.),(1.,1.),(1.,1.),(1.,1.),(1.,1.),(1.,1.),(1.,1.),(1.,1.),(1.,
1.),(1.,1.),(1.,1.),(1.,1.),(1.,1.),(1.,1.),(1.,1.),(1.,1.),(1.,1.),(1.,
1.),(1.,1.),(1.,1.),(1.,1.),(1.,1.),(1.,1.),(1.,1.),(1.,1.),(1.,1.),(1.,
1.),(1.,1.),(1.,1.),(1.,1.),(1.,1.),(1.,1.),(1.,1.),(1.,1.),(1.,1.),(1.,
1.),(1.,1.),(1.,1.),(1.,1.),(1.,1.),(1.,1.),(1.,1.),(1.,1.),(1.,1.),(1.,
1.),(1.,1.),(1.,1.),(1.,1.),(1.,1.),(1.,1.),(1.,1.),(1.,1.),(1.,1.),(1.,
1.),(1.,1.),(1.,1.),(1.,1.),(1.,1.),(1.,1.),(1.,1.),(1.,1.),(1.,1.),(1.,
1.),(1.,1.),(1.,1.),(1.,1.),(1.,1.),(1.,1.),(1.,1.),(1.,1.),(1.,1.),(1.,
1.),(1.,1.)))
REPRESENTATION_ITEM('')
SURFACE()
);
#973=(
BOUNDED_SURFACE()
B_SPLINE_SURFACE(5,1,((#131411,#131412),(#131413,#131414),(#131415,#131416),
(#131417,#131418),(#131419,#131420),(#131421,#131422),(#131423,#131424),
(#131425,#131426),(#131427,#131428),(#131429,#131430),(#131431,#131432),
(#131433,#131434),(#131435,#131436),(#131437,#131438),(#131439,#131440),
(#131441,#131442),(#131443,#131444),(#131445,#131446),(#131447,#131448),
(#131449,#131450),(#131451,#131452),(#131453,#131454),(#131455,#131456),
(#131457,#131458),(#131459,#131460),(#131461,#131462),(#131463,#131464),
(#131465,#131466),(#131467,#131468),(#131469,#131470),(#131471,#131472),
(#131473,#131474),(#131475,#131476),(#131477,#131478),(#131479,#131480),
(#131481,#131482),(#131483,#131484),(#131485,#131486),(#131487,#131488),
(#131489,#131490),(#131491,#131492),(#131493,#131494),(#131495,#131496),
(#131497,#131498),(#131499,#131500),(#131501,#131502),(#131503,#131504),
(#131505,#131506),(#131507,#131508),(#131509,#131510),(#131511,#131512),
(#131513,#131514),(#131515,#131516),(#131517,#131518),(#131519,#131520),
(#131521,#131522),(#131523,#131524),(#131525,#131526),(#131527,#131528),
(#131529,#131530),(#131531,#131532),(#131533,#131534),(#131535,#131536),
(#131537,#131538),(#131539,#131540),(#131541,#131542),(#131543,#131544),
(#131545,#131546),(#131547,#131548),(#131549,#131550),(#131551,#131552),
(#131553,#131554),(#131555,#131556),(#131557,#131558),(#131559,#131560),
(#131561,#131562),(#131563,#131564),(#131565,#131566),(#131567,#131568),
(#131569,#131570),(#131571,#131572),(#131573,#131574),(#131575,#131576),
(#131577,#131578),(#131579,#131580),(#131581,#131582),(#131583,#131584),
(#131585,#131586),(#131587,#131588),(#131589,#131590),(#131591,#131592),
(#131593,#131594),(#131595,#131596),(#131597,#131598),(#131599,#131600),
(#131601,#131602),(#131603,#131604),(#131605,#131606),(#131607,#131608),
(#131609,#131610),(#131611,#131612),(#131613,#131614),(#131615,#131616),
(#131617,#131618),(#131619,#131620),(#131621,#131622),(#131623,#131624),
(#131625,#131626),(#131627,#131628),(#131629,#131630),(#131631,#131632),
(#131633,#131634),(#131635,#131636),(#131637,#131638),(#131639,#131640),
(#131641,#131642),(#131643,#131644),(#131645,#131646),(#131647,#131648),
(#131649,#131650),(#131651,#131652),(#131653,#131654),(#131655,#131656),
(#131657,#131658),(#131659,#131660),(#131661,#131662),(#131663,#131664),
(#131665,#131666),(#131667,#131668),(#131669,#131670),(#131671,#131672),
(#131673,#131674),(#131675,#131676),(#131677,#131678),(#131679,#131680),
(#131681,#131682),(#131683,#131684),(#131685,#131686),(#131687,#131688),
(#131689,#131690),(#131691,#131692),(#131693,#131694),(#131695,#131696),
(#131697,#131698),(#131699,#131700),(#131701,#131702),(#131703,#131704),
(#131705,#131706),(#131707,#131708),(#131709,#131710),(#131711,#131712),
(#131713,#131714),(#131715,#131716),(#131717,#131718),(#131719,#131720),
(#131721,#131722),(#131723,#131724),(#131725,#131726),(#131727,#131728),
(#131729,#131730),(#131731,#131732),(#131733,#131734),(#131735,#131736),
(#131737,#131738),(#131739,#131740),(#131741,#131742),(#131743,#131744),
(#131745,#131746),(#131747,#131748),(#131749,#131750),(#131751,#131752),
(#131753,#131754),(#131755,#131756),(#131757,#131758),(#131759,#131760),
(#131761,#131762),(#131763,#131764),(#131765,#131766),(#131767,#131768),
(#131769,#131770),(#131771,#131772),(#131773,#131774),(#131775,#131776),
(#131777,#131778),(#131779,#131780),(#131781,#131782),(#131783,#131784),
(#131785,#131786),(#131787,#131788),(#131789,#131790),(#131791,#131792),
(#131793,#131794),(#131795,#131796),(#131797,#131798),(#131799,#131800),
(#131801,#131802),(#131803,#131804),(#131805,#131806),(#131807,#131808),
(#131809,#131810),(#131811,#131812),(#131813,#131814),(#131815,#131816),
(#131817,#131818),(#131819,#131820)),.UNSPECIFIED.,.F.,.F.,.F.)
B_SPLINE_SURFACE_WITH_KNOTS((6,1,1,1,1,1,1,1,1,1,1,1,1,1,1,1,1,1,1,1,1,
1,1,1,1,1,1,1,1,1,1,1,1,1,1,1,1,1,1,1,1,1,1,1,1,1,1,1,1,1,1,1,1,1,1,1,1,
1,1,1,1,1,1,1,1,1,1,1,1,1,1,1,1,1,1,1,1,1,1,1,1,1,1,1,1,1,1,1,1,1,1,1,1,
1,1,1,1,1,1,1,1,1,1,1,1,1,1,1,1,1,1,1,1,1,1,1,1,1,1,1,1,1,1,1,1,1,1,1,1,
1,1,1,1,1,1,1,1,1,1,1,1,1,1,1,1,1,1,1,1,1,1,1,1,1,1,1,1,1,1,1,1,1,1,1,1,
1,1,1,1,1,1,1,1,1,1,1,1,1,1,1,1,1,1,1,1,1,1,1,1,1,1,1,1,1,1,1,1,1,1,1,6),
(2,2),(-1.,-0.995000000000001,-0.990000000000001,-0.985000000000001,-0.980000000000001,
-0.975000000000001,-0.970000000000001,-0.965000000000001,-0.960000000000001,
-0.955000000000001,-0.950000000000001,-0.945000000000001,-0.940000000000001,
-0.935000000000001,-0.930000000000001,-0.925000000000001,-0.920000000000001,
-0.915000000000001,-0.910000000000001,-0.905000000000001,-0.900000000000001,
-0.895000000000001,-0.890000000000001,-0.885000000000001,-0.880000000000001,
-0.875000000000001,-0.870000000000001,-0.865000000000001,-0.860000000000001,
-0.855000000000001,-0.850000000000001,-0.845000000000001,-0.840000000000001,
-0.835000000000001,-0.830000000000001,-0.825000000000001,-0.820000000000001,
-0.815000000000001,-0.810000000000001,-0.805000000000001,-0.800000000000001,
-0.795000000000001,-0.790000000000001,-0.785000000000001,-0.780000000000001,
-0.775000000000001,-0.770000000000001,-0.765000000000001,-0.760000000000001,
-0.755000000000001,-0.750000000000001,-0.745000000000001,-0.740000000000001,
-0.735000000000001,-0.730000000000001,-0.725000000000001,-0.720000000000001,
-0.715000000000001,-0.710000000000001,-0.705000000000001,-0.700000000000001,
-0.695000000000001,-0.690000000000001,-0.685,-0.68,-0.675,-0.67,-0.665,
-0.66,-0.655,-0.65,-0.645,-0.64,-0.635,-0.63,-0.625,-0.62,-0.615,-0.61,
-0.605,-0.6,-0.595,-0.59,-0.585,-0.58,-0.575,-0.57,-0.565,-0.56,-0.555,
-0.55,-0.545,-0.54,-0.535,-0.53,-0.525,-0.52,-0.515,-0.51,-0.505,-0.5,-0.495,
-0.49,-0.485,-0.48,-0.475,-0.47,-0.465,-0.46,-0.455,-0.45,-0.445,-0.44,
-0.435,-0.43,-0.425,-0.42,-0.415,-0.41,-0.405,-0.4,-0.395,-0.39,-0.385,
-0.38,-0.375,-0.37,-0.365,-0.36,-0.355,-0.35,-0.345,-0.34,-0.335,-0.33,
-0.325,-0.32,-0.315,-0.31,-0.305,-0.3,-0.295,-0.29,-0.285,-0.28,-0.275,
-0.27,-0.265,-0.26,-0.255,-0.25,-0.245,-0.24,-0.235,-0.23,-0.225,-0.22,
-0.215,-0.21,-0.205,-0.2,-0.195,-0.19,-0.185,-0.18,-0.175,-0.17,-0.165,
-0.16,-0.155,-0.15,-0.145,-0.14,-0.135,-0.13,-0.125,-0.12,-0.115,-0.11,
-0.105,-0.1,-0.095,-0.09,-0.085,-0.08,-0.075,-0.07,-0.065,-0.06,-0.055,
-0.05,-0.045,-0.04,-0.035,-0.03,-0.025,-0.02,-0.015,-0.01,-0.005,0.),(0.,
1.2),.UNSPECIFIED.)
GEOMETRIC_REPRESENTATION_ITEM()
RATIONAL_B_SPLINE_SURFACE(((1.,1.),(1.,1.),(1.,1.),(1.,1.),(1.,1.),(1.,
1.),(1.,1.),(1.,1.),(1.,1.),(1.,1.),(1.,1.),(1.,1.),(1.,1.),(1.,1.),(1.,
1.),(1.,1.),(1.,1.),(1.,1.),(1.,1.),(1.,1.),(1.,1.),(1.,1.),(1.,1.),(1.,
1.),(1.,1.),(1.,1.),(1.,1.),(1.,1.),(1.,1.),(1.,1.),(1.,1.),(1.,1.),(1.,
1.),(1.,1.),(1.,1.),(1.,1.),(1.,1.),(1.,1.),(1.,1.),(1.,1.),(1.,1.),(1.,
1.),(1.,1.),(1.,1.),(1.,1.),(1.,1.),(1.,1.),(1.,1.),(1.,1.),(1.,1.),(1.,
1.),(1.,1.),(1.,1.),(1.,1.),(1.,1.),(1.,1.),(1.,1.),(1.,1.),(1.,1.),(1.,
1.),(1.,1.),(1.,1.),(1.,1.),(1.,1.),(1.,1.),(1.,1.),(1.,1.),(1.,1.),(1.,
1.),(1.,1.),(1.,1.),(1.,1.),(1.,1.),(1.,1.),(1.,1.),(1.,1.),(1.,1.),(1.,
1.),(1.,1.),(1.,1.),(1.,1.),(1.,1.),(1.,1.),(1.,1.),(1.,1.),(1.,1.),(1.,
1.),(1.,1.),(1.,1.),(1.,1.),(1.,1.),(1.,1.),(1.,1.),(1.,1.),(1.,1.),(1.,
1.),(1.,1.),(1.,1.),(1.,1.),(1.,1.),(1.,1.),(1.,1.),(1.,1.),(1.,1.),(1.,
1.),(1.,1.),(1.,1.),(1.,1.),(1.,1.),(1.,1.),(1.,1.),(1.,1.),(1.,1.),(1.,
1.),(1.,1.),(1.,1.),(1.,1.),(1.,1.),(1.,1.),(1.,1.),(1.,1.),(1.,1.),(1.,
1.),(1.,1.),(1.,1.),(1.,1.),(1.,1.),(1.,1.),(1.,1.),(1.,1.),(1.,1.),(1.,
1.),(1.,1.),(1.,1.),(1.,1.),(1.,1.),(1.,1.),(1.,1.),(1.,1.),(1.,1.),(1.,
1.),(1.,1.),(1.,1.),(1.,1.),(1.,1.),(1.,1.),(1.,1.),(1.,1.),(1.,1.),(1.,
1.),(1.,1.),(1.,1.),(1.,1.),(1.,1.),(1.,1.),(1.,1.),(1.,1.),(1.,1.),(1.,
1.),(1.,1.),(1.,1.),(1.,1.),(1.,1.),(1.,1.),(1.,1.),(1.,1.),(1.,1.),(1.,
1.),(1.,1.),(1.,1.),(1.,1.),(1.,1.),(1.,1.),(1.,1.),(1.,1.),(1.,1.),(1.,
1.),(1.,1.),(1.,1.),(1.,1.),(1.,1.),(1.,1.),(1.,1.),(1.,1.),(1.,1.),(1.,
1.),(1.,1.),(1.,1.),(1.,1.),(1.,1.),(1.,1.),(1.,1.),(1.,1.),(1.,1.),(1.,
1.),(1.,1.),(1.,1.),(1.,1.),(1.,1.),(1.,1.),(1.,1.),(1.,1.),(1.,1.),(1.,
1.),(1.,1.)))
REPRESENTATION_ITEM('')
SURFACE()
);
#974=(
BOUNDED_SURFACE()
B_SPLINE_SURFACE(5,1,((#132212,#132213),(#132214,#132215),(#132216,#132217),
(#132218,#132219),(#132220,#132221),(#132222,#132223),(#132224,#132225),
(#132226,#132227),(#132228,#132229),(#132230,#132231),(#132232,#132233),
(#132234,#132235),(#132236,#132237),(#132238,#132239),(#132240,#132241),
(#132242,#132243),(#132244,#132245),(#132246,#132247),(#132248,#132249),
(#132250,#132251),(#132252,#132253),(#132254,#132255),(#132256,#132257),
(#132258,#132259),(#132260,#132261),(#132262,#132263),(#132264,#132265),
(#132266,#132267),(#132268,#132269),(#132270,#132271),(#132272,#132273),
(#132274,#132275),(#132276,#132277),(#132278,#132279),(#132280,#132281),
(#132282,#132283),(#132284,#132285),(#132286,#132287),(#132288,#132289),
(#132290,#132291),(#132292,#132293),(#132294,#132295),(#132296,#132297),
(#132298,#132299),(#132300,#132301),(#132302,#132303),(#132304,#132305),
(#132306,#132307),(#132308,#132309),(#132310,#132311),(#132312,#132313),
(#132314,#132315),(#132316,#132317),(#132318,#132319),(#132320,#132321),
(#132322,#132323),(#132324,#132325),(#132326,#132327),(#132328,#132329),
(#132330,#132331),(#132332,#132333),(#132334,#132335),(#132336,#132337),
(#132338,#132339),(#132340,#132341),(#132342,#132343),(#132344,#132345),
(#132346,#132347),(#132348,#132349),(#132350,#132351),(#132352,#132353),
(#132354,#132355),(#132356,#132357),(#132358,#132359),(#132360,#132361),
(#132362,#132363),(#132364,#132365),(#132366,#132367),(#132368,#132369),
(#132370,#132371),(#132372,#132373),(#132374,#132375),(#132376,#132377),
(#132378,#132379),(#132380,#132381),(#132382,#132383),(#132384,#132385),
(#132386,#132387),(#132388,#132389),(#132390,#132391),(#132392,#132393),
(#132394,#132395),(#132396,#132397),(#132398,#132399),(#132400,#132401),
(#132402,#132403),(#132404,#132405),(#132406,#132407),(#132408,#132409),
(#132410,#132411),(#132412,#132413),(#132414,#132415),(#132416,#132417),
(#132418,#132419),(#132420,#132421),(#132422,#132423),(#132424,#132425),
(#132426,#132427),(#132428,#132429),(#132430,#132431),(#132432,#132433),
(#132434,#132435),(#132436,#132437),(#132438,#132439),(#132440,#132441),
(#132442,#132443),(#132444,#132445),(#132446,#132447),(#132448,#132449),
(#132450,#132451),(#132452,#132453),(#132454,#132455),(#132456,#132457),
(#132458,#132459),(#132460,#132461),(#132462,#132463),(#132464,#132465),
(#132466,#132467),(#132468,#132469),(#132470,#132471),(#132472,#132473),
(#132474,#132475),(#132476,#132477),(#132478,#132479),(#132480,#132481),
(#132482,#132483),(#132484,#132485),(#132486,#132487),(#132488,#132489),
(#132490,#132491),(#132492,#132493),(#132494,#132495),(#132496,#132497),
(#132498,#132499),(#132500,#132501),(#132502,#132503),(#132504,#132505),
(#132506,#132507),(#132508,#132509),(#132510,#132511),(#132512,#132513),
(#132514,#132515),(#132516,#132517),(#132518,#132519),(#132520,#132521),
(#132522,#132523),(#132524,#132525),(#132526,#132527),(#132528,#132529),
(#132530,#132531),(#132532,#132533),(#132534,#132535),(#132536,#132537),
(#132538,#132539),(#132540,#132541),(#132542,#132543),(#132544,#132545),
(#132546,#132547),(#132548,#132549),(#132550,#132551),(#132552,#132553),
(#132554,#132555),(#132556,#132557),(#132558,#132559),(#132560,#132561),
(#132562,#132563),(#132564,#132565),(#132566,#132567),(#132568,#132569),
(#132570,#132571),(#132572,#132573),(#132574,#132575),(#132576,#132577),
(#132578,#132579),(#132580,#132581),(#132582,#132583),(#132584,#132585),
(#132586,#132587),(#132588,#132589),(#132590,#132591),(#132592,#132593),
(#132594,#132595),(#132596,#132597),(#132598,#132599),(#132600,#132601),
(#132602,#132603),(#132604,#132605),(#132606,#132607),(#132608,#132609),
(#132610,#132611),(#132612,#132613),(#132614,#132615),(#132616,#132617),
(#132618,#132619),(#132620,#132621)),.UNSPECIFIED.,.F.,.F.,.F.)
B_SPLINE_SURFACE_WITH_KNOTS((6,1,1,1,1,1,1,1,1,1,1,1,1,1,1,1,1,1,1,1,1,
1,1,1,1,1,1,1,1,1,1,1,1,1,1,1,1,1,1,1,1,1,1,1,1,1,1,1,1,1,1,1,1,1,1,1,1,
1,1,1,1,1,1,1,1,1,1,1,1,1,1,1,1,1,1,1,1,1,1,1,1,1,1,1,1,1,1,1,1,1,1,1,1,
1,1,1,1,1,1,1,1,1,1,1,1,1,1,1,1,1,1,1,1,1,1,1,1,1,1,1,1,1,1,1,1,1,1,1,1,
1,1,1,1,1,1,1,1,1,1,1,1,1,1,1,1,1,1,1,1,1,1,1,1,1,1,1,1,1,1,1,1,1,1,1,1,
1,1,1,1,1,1,1,1,1,1,1,1,1,1,1,1,1,1,1,1,1,1,1,1,1,1,1,1,1,1,1,1,1,1,1,6),
(2,2),(-1.,-0.995000000000001,-0.990000000000001,-0.985000000000001,-0.980000000000001,
-0.975000000000001,-0.970000000000001,-0.965000000000001,-0.960000000000001,
-0.955000000000001,-0.950000000000001,-0.945000000000001,-0.940000000000001,
-0.935000000000001,-0.930000000000001,-0.925000000000001,-0.920000000000001,
-0.915000000000001,-0.910000000000001,-0.905000000000001,-0.900000000000001,
-0.895000000000001,-0.890000000000001,-0.885000000000001,-0.880000000000001,
-0.875000000000001,-0.870000000000001,-0.865000000000001,-0.860000000000001,
-0.855000000000001,-0.850000000000001,-0.845000000000001,-0.840000000000001,
-0.835000000000001,-0.830000000000001,-0.825000000000001,-0.820000000000001,
-0.815000000000001,-0.810000000000001,-0.805000000000001,-0.800000000000001,
-0.795000000000001,-0.790000000000001,-0.785000000000001,-0.780000000000001,
-0.775000000000001,-0.770000000000001,-0.765000000000001,-0.760000000000001,
-0.755000000000001,-0.750000000000001,-0.745000000000001,-0.740000000000001,
-0.735000000000001,-0.730000000000001,-0.725000000000001,-0.720000000000001,
-0.715000000000001,-0.710000000000001,-0.705000000000001,-0.700000000000001,
-0.695000000000001,-0.690000000000001,-0.685,-0.68,-0.675,-0.67,-0.665,
-0.66,-0.655,-0.65,-0.645,-0.64,-0.635,-0.63,-0.625,-0.62,-0.615,-0.61,
-0.605,-0.6,-0.595,-0.59,-0.585,-0.58,-0.575,-0.57,-0.565,-0.56,-0.555,
-0.55,-0.545,-0.54,-0.535,-0.53,-0.525,-0.52,-0.515,-0.51,-0.505,-0.5,-0.495,
-0.49,-0.485,-0.48,-0.475,-0.47,-0.465,-0.46,-0.455,-0.45,-0.445,-0.44,
-0.435,-0.43,-0.425,-0.42,-0.415,-0.41,-0.405,-0.4,-0.395,-0.39,-0.385,
-0.38,-0.375,-0.37,-0.365,-0.36,-0.355,-0.35,-0.345,-0.34,-0.335,-0.33,
-0.325,-0.32,-0.315,-0.31,-0.305,-0.3,-0.295,-0.29,-0.285,-0.28,-0.275,
-0.27,-0.265,-0.26,-0.255,-0.25,-0.245,-0.24,-0.235,-0.23,-0.225,-0.22,
-0.215,-0.21,-0.205,-0.2,-0.195,-0.19,-0.185,-0.18,-0.175,-0.17,-0.165,
-0.16,-0.155,-0.15,-0.145,-0.14,-0.135,-0.13,-0.125,-0.12,-0.115,-0.11,
-0.105,-0.1,-0.095,-0.09,-0.085,-0.08,-0.075,-0.07,-0.065,-0.06,-0.055,
-0.05,-0.045,-0.04,-0.035,-0.03,-0.025,-0.02,-0.015,-0.01,-0.005,0.),(0.,
1.2),.UNSPECIFIED.)
GEOMETRIC_REPRESENTATION_ITEM()
RATIONAL_B_SPLINE_SURFACE(((1.,1.),(1.,1.),(1.,1.),(1.,1.),(1.,1.),(1.,
1.),(1.,1.),(1.,1.),(1.,1.),(1.,1.),(1.,1.),(1.,1.),(1.,1.),(1.,1.),(1.,
1.),(1.,1.),(1.,1.),(1.,1.),(1.,1.),(1.,1.),(1.,1.),(1.,1.),(1.,1.),(1.,
1.),(1.,1.),(1.,1.),(1.,1.),(1.,1.),(1.,1.),(1.,1.),(1.,1.),(1.,1.),(1.,
1.),(1.,1.),(1.,1.),(1.,1.),(1.,1.),(1.,1.),(1.,1.),(1.,1.),(1.,1.),(1.,
1.),(1.,1.),(1.,1.),(1.,1.),(1.,1.),(1.,1.),(1.,1.),(1.,1.),(1.,1.),(1.,
1.),(1.,1.),(1.,1.),(1.,1.),(1.,1.),(1.,1.),(1.,1.),(1.,1.),(1.,1.),(1.,
1.),(1.,1.),(1.,1.),(1.,1.),(1.,1.),(1.,1.),(1.,1.),(1.,1.),(1.,1.),(1.,
1.),(1.,1.),(1.,1.),(1.,1.),(1.,1.),(1.,1.),(1.,1.),(1.,1.),(1.,1.),(1.,
1.),(1.,1.),(1.,1.),(1.,1.),(1.,1.),(1.,1.),(1.,1.),(1.,1.),(1.,1.),(1.,
1.),(1.,1.),(1.,1.),(1.,1.),(1.,1.),(1.,1.),(1.,1.),(1.,1.),(1.,1.),(1.,
1.),(1.,1.),(1.,1.),(1.,1.),(1.,1.),(1.,1.),(1.,1.),(1.,1.),(1.,1.),(1.,
1.),(1.,1.),(1.,1.),(1.,1.),(1.,1.),(1.,1.),(1.,1.),(1.,1.),(1.,1.),(1.,
1.),(1.,1.),(1.,1.),(1.,1.),(1.,1.),(1.,1.),(1.,1.),(1.,1.),(1.,1.),(1.,
1.),(1.,1.),(1.,1.),(1.,1.),(1.,1.),(1.,1.),(1.,1.),(1.,1.),(1.,1.),(1.,
1.),(1.,1.),(1.,1.),(1.,1.),(1.,1.),(1.,1.),(1.,1.),(1.,1.),(1.,1.),(1.,
1.),(1.,1.),(1.,1.),(1.,1.),(1.,1.),(1.,1.),(1.,1.),(1.,1.),(1.,1.),(1.,
1.),(1.,1.),(1.,1.),(1.,1.),(1.,1.),(1.,1.),(1.,1.),(1.,1.),(1.,1.),(1.,
1.),(1.,1.),(1.,1.),(1.,1.),(1.,1.),(1.,1.),(1.,1.),(1.,1.),(1.,1.),(1.,
1.),(1.,1.),(1.,1.),(1.,1.),(1.,1.),(1.,1.),(1.,1.),(1.,1.),(1.,1.),(1.,
1.),(1.,1.),(1.,1.),(1.,1.),(1.,1.),(1.,1.),(1.,1.),(1.,1.),(1.,1.),(1.,
1.),(1.,1.),(1.,1.),(1.,1.),(1.,1.),(1.,1.),(1.,1.),(1.,1.),(1.,1.),(1.,
1.),(1.,1.),(1.,1.),(1.,1.),(1.,1.),(1.,1.),(1.,1.),(1.,1.),(1.,1.),(1.,
1.),(1.,1.)))
REPRESENTATION_ITEM('')
SURFACE()
);
#975=(
BOUNDED_SURFACE()
B_SPLINE_SURFACE(5,1,((#133013,#133014),(#133015,#133016),(#133017,#133018),
(#133019,#133020),(#133021,#133022),(#133023,#133024),(#133025,#133026),
(#133027,#133028),(#133029,#133030),(#133031,#133032),(#133033,#133034),
(#133035,#133036),(#133037,#133038),(#133039,#133040),(#133041,#133042),
(#133043,#133044),(#133045,#133046),(#133047,#133048),(#133049,#133050),
(#133051,#133052),(#133053,#133054),(#133055,#133056),(#133057,#133058),
(#133059,#133060),(#133061,#133062),(#133063,#133064),(#133065,#133066),
(#133067,#133068),(#133069,#133070),(#133071,#133072),(#133073,#133074),
(#133075,#133076),(#133077,#133078),(#133079,#133080),(#133081,#133082),
(#133083,#133084),(#133085,#133086),(#133087,#133088),(#133089,#133090),
(#133091,#133092),(#133093,#133094),(#133095,#133096),(#133097,#133098),
(#133099,#133100),(#133101,#133102),(#133103,#133104),(#133105,#133106),
(#133107,#133108),(#133109,#133110),(#133111,#133112),(#133113,#133114),
(#133115,#133116),(#133117,#133118),(#133119,#133120),(#133121,#133122),
(#133123,#133124),(#133125,#133126),(#133127,#133128),(#133129,#133130),
(#133131,#133132),(#133133,#133134),(#133135,#133136),(#133137,#133138),
(#133139,#133140),(#133141,#133142),(#133143,#133144),(#133145,#133146),
(#133147,#133148),(#133149,#133150),(#133151,#133152),(#133153,#133154),
(#133155,#133156),(#133157,#133158),(#133159,#133160),(#133161,#133162),
(#133163,#133164),(#133165,#133166),(#133167,#133168),(#133169,#133170),
(#133171,#133172),(#133173,#133174),(#133175,#133176),(#133177,#133178),
(#133179,#133180),(#133181,#133182),(#133183,#133184),(#133185,#133186),
(#133187,#133188),(#133189,#133190),(#133191,#133192),(#133193,#133194),
(#133195,#133196),(#133197,#133198),(#133199,#133200),(#133201,#133202),
(#133203,#133204),(#133205,#133206),(#133207,#133208),(#133209,#133210),
(#133211,#133212),(#133213,#133214),(#133215,#133216),(#133217,#133218),
(#133219,#133220),(#133221,#133222),(#133223,#133224),(#133225,#133226),
(#133227,#133228),(#133229,#133230),(#133231,#133232),(#133233,#133234),
(#133235,#133236),(#133237,#133238),(#133239,#133240),(#133241,#133242),
(#133243,#133244),(#133245,#133246),(#133247,#133248),(#133249,#133250),
(#133251,#133252),(#133253,#133254),(#133255,#133256),(#133257,#133258),
(#133259,#133260),(#133261,#133262),(#133263,#133264),(#133265,#133266),
(#133267,#133268),(#133269,#133270),(#133271,#133272),(#133273,#133274),
(#133275,#133276),(#133277,#133278),(#133279,#133280),(#133281,#133282),
(#133283,#133284),(#133285,#133286),(#133287,#133288),(#133289,#133290),
(#133291,#133292),(#133293,#133294),(#133295,#133296),(#133297,#133298),
(#133299,#133300),(#133301,#133302),(#133303,#133304),(#133305,#133306),
(#133307,#133308),(#133309,#133310),(#133311,#133312),(#133313,#133314),
(#133315,#133316),(#133317,#133318),(#133319,#133320),(#133321,#133322),
(#133323,#133324),(#133325,#133326),(#133327,#133328),(#133329,#133330),
(#133331,#133332),(#133333,#133334),(#133335,#133336),(#133337,#133338),
(#133339,#133340),(#133341,#133342),(#133343,#133344),(#133345,#133346),
(#133347,#133348),(#133349,#133350),(#133351,#133352),(#133353,#133354),
(#133355,#133356),(#133357,#133358),(#133359,#133360),(#133361,#133362),
(#133363,#133364),(#133365,#133366),(#133367,#133368),(#133369,#133370),
(#133371,#133372),(#133373,#133374),(#133375,#133376),(#133377,#133378),
(#133379,#133380),(#133381,#133382),(#133383,#133384),(#133385,#133386),
(#133387,#133388),(#133389,#133390),(#133391,#133392),(#133393,#133394),
(#133395,#133396),(#133397,#133398),(#133399,#133400),(#133401,#133402),
(#133403,#133404),(#133405,#133406),(#133407,#133408),(#133409,#133410),
(#133411,#133412),(#133413,#133414),(#133415,#133416),(#133417,#133418),
(#133419,#133420),(#133421,#133422)),.UNSPECIFIED.,.F.,.F.,.F.)
B_SPLINE_SURFACE_WITH_KNOTS((6,1,1,1,1,1,1,1,1,1,1,1,1,1,1,1,1,1,1,1,1,
1,1,1,1,1,1,1,1,1,1,1,1,1,1,1,1,1,1,1,1,1,1,1,1,1,1,1,1,1,1,1,1,1,1,1,1,
1,1,1,1,1,1,1,1,1,1,1,1,1,1,1,1,1,1,1,1,1,1,1,1,1,1,1,1,1,1,1,1,1,1,1,1,
1,1,1,1,1,1,1,1,1,1,1,1,1,1,1,1,1,1,1,1,1,1,1,1,1,1,1,1,1,1,1,1,1,1,1,1,
1,1,1,1,1,1,1,1,1,1,1,1,1,1,1,1,1,1,1,1,1,1,1,1,1,1,1,1,1,1,1,1,1,1,1,1,
1,1,1,1,1,1,1,1,1,1,1,1,1,1,1,1,1,1,1,1,1,1,1,1,1,1,1,1,1,1,1,1,1,1,1,6),
(2,2),(-1.,-0.995000000000001,-0.990000000000001,-0.985000000000001,-0.980000000000001,
-0.975000000000001,-0.970000000000001,-0.965000000000001,-0.960000000000001,
-0.955000000000001,-0.950000000000001,-0.945000000000001,-0.940000000000001,
-0.935000000000001,-0.930000000000001,-0.925000000000001,-0.920000000000001,
-0.915000000000001,-0.910000000000001,-0.905000000000001,-0.900000000000001,
-0.895000000000001,-0.890000000000001,-0.885000000000001,-0.880000000000001,
-0.875000000000001,-0.870000000000001,-0.865000000000001,-0.860000000000001,
-0.855000000000001,-0.850000000000001,-0.845000000000001,-0.840000000000001,
-0.835000000000001,-0.830000000000001,-0.825000000000001,-0.820000000000001,
-0.815000000000001,-0.810000000000001,-0.805000000000001,-0.800000000000001,
-0.795000000000001,-0.790000000000001,-0.785000000000001,-0.780000000000001,
-0.775000000000001,-0.770000000000001,-0.765000000000001,-0.760000000000001,
-0.755000000000001,-0.750000000000001,-0.745000000000001,-0.740000000000001,
-0.735000000000001,-0.730000000000001,-0.725000000000001,-0.720000000000001,
-0.715000000000001,-0.710000000000001,-0.705000000000001,-0.700000000000001,
-0.695000000000001,-0.690000000000001,-0.685,-0.68,-0.675,-0.67,-0.665,
-0.66,-0.655,-0.65,-0.645,-0.64,-0.635,-0.63,-0.625,-0.62,-0.615,-0.61,
-0.605,-0.6,-0.595,-0.59,-0.585,-0.58,-0.575,-0.57,-0.565,-0.56,-0.555,
-0.55,-0.545,-0.54,-0.535,-0.53,-0.525,-0.52,-0.515,-0.51,-0.505,-0.5,-0.495,
-0.49,-0.485,-0.48,-0.475,-0.47,-0.465,-0.46,-0.455,-0.45,-0.445,-0.44,
-0.435,-0.43,-0.425,-0.42,-0.415,-0.41,-0.405,-0.4,-0.395,-0.39,-0.385,
-0.38,-0.375,-0.37,-0.365,-0.36,-0.355,-0.35,-0.345,-0.34,-0.335,-0.33,
-0.325,-0.32,-0.315,-0.31,-0.305,-0.3,-0.295,-0.29,-0.285,-0.28,-0.275,
-0.27,-0.265,-0.26,-0.255,-0.25,-0.245,-0.24,-0.235,-0.23,-0.225,-0.22,
-0.215,-0.21,-0.205,-0.2,-0.195,-0.19,-0.185,-0.18,-0.175,-0.17,-0.165,
-0.16,-0.155,-0.15,-0.145,-0.14,-0.135,-0.13,-0.125,-0.12,-0.115,-0.11,
-0.105,-0.1,-0.095,-0.09,-0.085,-0.08,-0.075,-0.07,-0.065,-0.06,-0.055,
-0.05,-0.045,-0.04,-0.035,-0.03,-0.025,-0.02,-0.015,-0.01,-0.005,0.),(0.,
1.2),.UNSPECIFIED.)
GEOMETRIC_REPRESENTATION_ITEM()
RATIONAL_B_SPLINE_SURFACE(((1.,1.),(1.,1.),(1.,1.),(1.,1.),(1.,1.),(1.,
1.),(1.,1.),(1.,1.),(1.,1.),(1.,1.),(1.,1.),(1.,1.),(1.,1.),(1.,1.),(1.,
1.),(1.,1.),(1.,1.),(1.,1.),(1.,1.),(1.,1.),(1.,1.),(1.,1.),(1.,1.),(1.,
1.),(1.,1.),(1.,1.),(1.,1.),(1.,1.),(1.,1.),(1.,1.),(1.,1.),(1.,1.),(1.,
1.),(1.,1.),(1.,1.),(1.,1.),(1.,1.),(1.,1.),(1.,1.),(1.,1.),(1.,1.),(1.,
1.),(1.,1.),(1.,1.),(1.,1.),(1.,1.),(1.,1.),(1.,1.),(1.,1.),(1.,1.),(1.,
1.),(1.,1.),(1.,1.),(1.,1.),(1.,1.),(1.,1.),(1.,1.),(1.,1.),(1.,1.),(1.,
1.),(1.,1.),(1.,1.),(1.,1.),(1.,1.),(1.,1.),(1.,1.),(1.,1.),(1.,1.),(1.,
1.),(1.,1.),(1.,1.),(1.,1.),(1.,1.),(1.,1.),(1.,1.),(1.,1.),(1.,1.),(1.,
1.),(1.,1.),(1.,1.),(1.,1.),(1.,1.),(1.,1.),(1.,1.),(1.,1.),(1.,1.),(1.,
1.),(1.,1.),(1.,1.),(1.,1.),(1.,1.),(1.,1.),(1.,1.),(1.,1.),(1.,1.),(1.,
1.),(1.,1.),(1.,1.),(1.,1.),(1.,1.),(1.,1.),(1.,1.),(1.,1.),(1.,1.),(1.,
1.),(1.,1.),(1.,1.),(1.,1.),(1.,1.),(1.,1.),(1.,1.),(1.,1.),(1.,1.),(1.,
1.),(1.,1.),(1.,1.),(1.,1.),(1.,1.),(1.,1.),(1.,1.),(1.,1.),(1.,1.),(1.,
1.),(1.,1.),(1.,1.),(1.,1.),(1.,1.),(1.,1.),(1.,1.),(1.,1.),(1.,1.),(1.,
1.),(1.,1.),(1.,1.),(1.,1.),(1.,1.),(1.,1.),(1.,1.),(1.,1.),(1.,1.),(1.,
1.),(1.,1.),(1.,1.),(1.,1.),(1.,1.),(1.,1.),(1.,1.),(1.,1.),(1.,1.),(1.,
1.),(1.,1.),(1.,1.),(1.,1.),(1.,1.),(1.,1.),(1.,1.),(1.,1.),(1.,1.),(1.,
1.),(1.,1.),(1.,1.),(1.,1.),(1.,1.),(1.,1.),(1.,1.),(1.,1.),(1.,1.),(1.,
1.),(1.,1.),(1.,1.),(1.,1.),(1.,1.),(1.,1.),(1.,1.),(1.,1.),(1.,1.),(1.,
1.),(1.,1.),(1.,1.),(1.,1.),(1.,1.),(1.,1.),(1.,1.),(1.,1.),(1.,1.),(1.,
1.),(1.,1.),(1.,1.),(1.,1.),(1.,1.),(1.,1.),(1.,1.),(1.,1.),(1.,1.),(1.,
1.),(1.,1.),(1.,1.),(1.,1.),(1.,1.),(1.,1.),(1.,1.),(1.,1.),(1.,1.),(1.,
1.),(1.,1.)))
REPRESENTATION_ITEM('')
SURFACE()
);
#976=(
BOUNDED_SURFACE()
B_SPLINE_SURFACE(5,1,((#133814,#133815),(#133816,#133817),(#133818,#133819),
(#133820,#133821),(#133822,#133823),(#133824,#133825),(#133826,#133827),
(#133828,#133829),(#133830,#133831),(#133832,#133833),(#133834,#133835),
(#133836,#133837),(#133838,#133839),(#133840,#133841),(#133842,#133843),
(#133844,#133845),(#133846,#133847),(#133848,#133849),(#133850,#133851),
(#133852,#133853),(#133854,#133855),(#133856,#133857),(#133858,#133859),
(#133860,#133861),(#133862,#133863),(#133864,#133865),(#133866,#133867),
(#133868,#133869),(#133870,#133871),(#133872,#133873),(#133874,#133875),
(#133876,#133877),(#133878,#133879),(#133880,#133881),(#133882,#133883),
(#133884,#133885),(#133886,#133887),(#133888,#133889),(#133890,#133891),
(#133892,#133893),(#133894,#133895),(#133896,#133897),(#133898,#133899),
(#133900,#133901),(#133902,#133903),(#133904,#133905),(#133906,#133907),
(#133908,#133909),(#133910,#133911),(#133912,#133913),(#133914,#133915),
(#133916,#133917),(#133918,#133919),(#133920,#133921),(#133922,#133923),
(#133924,#133925),(#133926,#133927),(#133928,#133929),(#133930,#133931),
(#133932,#133933),(#133934,#133935),(#133936,#133937),(#133938,#133939),
(#133940,#133941),(#133942,#133943),(#133944,#133945),(#133946,#133947),
(#133948,#133949),(#133950,#133951),(#133952,#133953),(#133954,#133955),
(#133956,#133957),(#133958,#133959),(#133960,#133961),(#133962,#133963),
(#133964,#133965),(#133966,#133967),(#133968,#133969),(#133970,#133971),
(#133972,#133973),(#133974,#133975),(#133976,#133977),(#133978,#133979),
(#133980,#133981),(#133982,#133983),(#133984,#133985),(#133986,#133987),
(#133988,#133989),(#133990,#133991),(#133992,#133993),(#133994,#133995),
(#133996,#133997),(#133998,#133999),(#134000,#134001),(#134002,#134003),
(#134004,#134005),(#134006,#134007),(#134008,#134009),(#134010,#134011),
(#134012,#134013),(#134014,#134015),(#134016,#134017),(#134018,#134019),
(#134020,#134021),(#134022,#134023),(#134024,#134025),(#134026,#134027),
(#134028,#134029),(#134030,#134031),(#134032,#134033),(#134034,#134035),
(#134036,#134037),(#134038,#134039),(#134040,#134041),(#134042,#134043),
(#134044,#134045),(#134046,#134047),(#134048,#134049),(#134050,#134051),
(#134052,#134053),(#134054,#134055),(#134056,#134057),(#134058,#134059),
(#134060,#134061),(#134062,#134063),(#134064,#134065),(#134066,#134067),
(#134068,#134069),(#134070,#134071),(#134072,#134073),(#134074,#134075),
(#134076,#134077),(#134078,#134079),(#134080,#134081),(#134082,#134083),
(#134084,#134085),(#134086,#134087),(#134088,#134089),(#134090,#134091),
(#134092,#134093),(#134094,#134095),(#134096,#134097),(#134098,#134099),
(#134100,#134101),(#134102,#134103),(#134104,#134105),(#134106,#134107),
(#134108,#134109),(#134110,#134111),(#134112,#134113),(#134114,#134115),
(#134116,#134117),(#134118,#134119),(#134120,#134121),(#134122,#134123),
(#134124,#134125),(#134126,#134127),(#134128,#134129),(#134130,#134131),
(#134132,#134133),(#134134,#134135),(#134136,#134137),(#134138,#134139),
(#134140,#134141),(#134142,#134143),(#134144,#134145),(#134146,#134147),
(#134148,#134149),(#134150,#134151),(#134152,#134153),(#134154,#134155),
(#134156,#134157),(#134158,#134159),(#134160,#134161),(#134162,#134163),
(#134164,#134165),(#134166,#134167),(#134168,#134169),(#134170,#134171),
(#134172,#134173),(#134174,#134175),(#134176,#134177),(#134178,#134179),
(#134180,#134181),(#134182,#134183),(#134184,#134185),(#134186,#134187),
(#134188,#134189),(#134190,#134191),(#134192,#134193),(#134194,#134195),
(#134196,#134197),(#134198,#134199),(#134200,#134201),(#134202,#134203),
(#134204,#134205),(#134206,#134207),(#134208,#134209),(#134210,#134211),
(#134212,#134213),(#134214,#134215),(#134216,#134217),(#134218,#134219),
(#134220,#134221),(#134222,#134223)),.UNSPECIFIED.,.F.,.F.,.F.)
B_SPLINE_SURFACE_WITH_KNOTS((6,1,1,1,1,1,1,1,1,1,1,1,1,1,1,1,1,1,1,1,1,
1,1,1,1,1,1,1,1,1,1,1,1,1,1,1,1,1,1,1,1,1,1,1,1,1,1,1,1,1,1,1,1,1,1,1,1,
1,1,1,1,1,1,1,1,1,1,1,1,1,1,1,1,1,1,1,1,1,1,1,1,1,1,1,1,1,1,1,1,1,1,1,1,
1,1,1,1,1,1,1,1,1,1,1,1,1,1,1,1,1,1,1,1,1,1,1,1,1,1,1,1,1,1,1,1,1,1,1,1,
1,1,1,1,1,1,1,1,1,1,1,1,1,1,1,1,1,1,1,1,1,1,1,1,1,1,1,1,1,1,1,1,1,1,1,1,
1,1,1,1,1,1,1,1,1,1,1,1,1,1,1,1,1,1,1,1,1,1,1,1,1,1,1,1,1,1,1,1,1,1,1,6),
(2,2),(-1.,-0.995000000000001,-0.990000000000001,-0.985000000000001,-0.980000000000001,
-0.975000000000001,-0.970000000000001,-0.965000000000001,-0.960000000000001,
-0.955000000000001,-0.950000000000001,-0.945000000000001,-0.940000000000001,
-0.935000000000001,-0.930000000000001,-0.925000000000001,-0.920000000000001,
-0.915000000000001,-0.910000000000001,-0.905000000000001,-0.900000000000001,
-0.895000000000001,-0.890000000000001,-0.885000000000001,-0.880000000000001,
-0.875000000000001,-0.870000000000001,-0.865000000000001,-0.860000000000001,
-0.855000000000001,-0.850000000000001,-0.845000000000001,-0.840000000000001,
-0.835000000000001,-0.830000000000001,-0.825000000000001,-0.820000000000001,
-0.815000000000001,-0.810000000000001,-0.805000000000001,-0.800000000000001,
-0.795000000000001,-0.790000000000001,-0.785000000000001,-0.780000000000001,
-0.775000000000001,-0.770000000000001,-0.765000000000001,-0.760000000000001,
-0.755000000000001,-0.750000000000001,-0.745000000000001,-0.740000000000001,
-0.735000000000001,-0.730000000000001,-0.725000000000001,-0.720000000000001,
-0.715000000000001,-0.710000000000001,-0.705000000000001,-0.700000000000001,
-0.695000000000001,-0.690000000000001,-0.685,-0.68,-0.675,-0.67,-0.665,
-0.66,-0.655,-0.65,-0.645,-0.64,-0.635,-0.63,-0.625,-0.62,-0.615,-0.61,
-0.605,-0.6,-0.595,-0.59,-0.585,-0.58,-0.575,-0.57,-0.565,-0.56,-0.555,
-0.55,-0.545,-0.54,-0.535,-0.53,-0.525,-0.52,-0.515,-0.51,-0.505,-0.5,-0.495,
-0.49,-0.485,-0.48,-0.475,-0.47,-0.465,-0.46,-0.455,-0.45,-0.445,-0.44,
-0.435,-0.43,-0.425,-0.42,-0.415,-0.41,-0.405,-0.4,-0.395,-0.39,-0.385,
-0.38,-0.375,-0.37,-0.365,-0.36,-0.355,-0.35,-0.345,-0.34,-0.335,-0.33,
-0.325,-0.32,-0.315,-0.31,-0.305,-0.3,-0.295,-0.29,-0.285,-0.28,-0.275,
-0.27,-0.265,-0.26,-0.255,-0.25,-0.245,-0.24,-0.235,-0.23,-0.225,-0.22,
-0.215,-0.21,-0.205,-0.2,-0.195,-0.19,-0.185,-0.18,-0.175,-0.17,-0.165,
-0.16,-0.155,-0.15,-0.145,-0.14,-0.135,-0.13,-0.125,-0.12,-0.115,-0.11,
-0.105,-0.1,-0.095,-0.09,-0.085,-0.08,-0.075,-0.07,-0.065,-0.06,-0.055,
-0.05,-0.045,-0.04,-0.035,-0.03,-0.025,-0.02,-0.015,-0.01,-0.005,0.),(0.,
1.2),.UNSPECIFIED.)
GEOMETRIC_REPRESENTATION_ITEM()
RATIONAL_B_SPLINE_SURFACE(((1.,1.),(1.,1.),(1.,1.),(1.,1.),(1.,1.),(1.,
1.),(1.,1.),(1.,1.),(1.,1.),(1.,1.),(1.,1.),(1.,1.),(1.,1.),(1.,1.),(1.,
1.),(1.,1.),(1.,1.),(1.,1.),(1.,1.),(1.,1.),(1.,1.),(1.,1.),(1.,1.),(1.,
1.),(1.,1.),(1.,1.),(1.,1.),(1.,1.),(1.,1.),(1.,1.),(1.,1.),(1.,1.),(1.,
1.),(1.,1.),(1.,1.),(1.,1.),(1.,1.),(1.,1.),(1.,1.),(1.,1.),(1.,1.),(1.,
1.),(1.,1.),(1.,1.),(1.,1.),(1.,1.),(1.,1.),(1.,1.),(1.,1.),(1.,1.),(1.,
1.),(1.,1.),(1.,1.),(1.,1.),(1.,1.),(1.,1.),(1.,1.),(1.,1.),(1.,1.),(1.,
1.),(1.,1.),(1.,1.),(1.,1.),(1.,1.),(1.,1.),(1.,1.),(1.,1.),(1.,1.),(1.,
1.),(1.,1.),(1.,1.),(1.,1.),(1.,1.),(1.,1.),(1.,1.),(1.,1.),(1.,1.),(1.,
1.),(1.,1.),(1.,1.),(1.,1.),(1.,1.),(1.,1.),(1.,1.),(1.,1.),(1.,1.),(1.,
1.),(1.,1.),(1.,1.),(1.,1.),(1.,1.),(1.,1.),(1.,1.),(1.,1.),(1.,1.),(1.,
1.),(1.,1.),(1.,1.),(1.,1.),(1.,1.),(1.,1.),(1.,1.),(1.,1.),(1.,1.),(1.,
1.),(1.,1.),(1.,1.),(1.,1.),(1.,1.),(1.,1.),(1.,1.),(1.,1.),(1.,1.),(1.,
1.),(1.,1.),(1.,1.),(1.,1.),(1.,1.),(1.,1.),(1.,1.),(1.,1.),(1.,1.),(1.,
1.),(1.,1.),(1.,1.),(1.,1.),(1.,1.),(1.,1.),(1.,1.),(1.,1.),(1.,1.),(1.,
1.),(1.,1.),(1.,1.),(1.,1.),(1.,1.),(1.,1.),(1.,1.),(1.,1.),(1.,1.),(1.,
1.),(1.,1.),(1.,1.),(1.,1.),(1.,1.),(1.,1.),(1.,1.),(1.,1.),(1.,1.),(1.,
1.),(1.,1.),(1.,1.),(1.,1.),(1.,1.),(1.,1.),(1.,1.),(1.,1.),(1.,1.),(1.,
1.),(1.,1.),(1.,1.),(1.,1.),(1.,1.),(1.,1.),(1.,1.),(1.,1.),(1.,1.),(1.,
1.),(1.,1.),(1.,1.),(1.,1.),(1.,1.),(1.,1.),(1.,1.),(1.,1.),(1.,1.),(1.,
1.),(1.,1.),(1.,1.),(1.,1.),(1.,1.),(1.,1.),(1.,1.),(1.,1.),(1.,1.),(1.,
1.),(1.,1.),(1.,1.),(1.,1.),(1.,1.),(1.,1.),(1.,1.),(1.,1.),(1.,1.),(1.,
1.),(1.,1.),(1.,1.),(1.,1.),(1.,1.),(1.,1.),(1.,1.),(1.,1.),(1.,1.),(1.,
1.),(1.,1.)))
REPRESENTATION_ITEM('')
SURFACE()
);
#977=(
BOUNDED_SURFACE()
B_SPLINE_SURFACE(5,1,((#134615,#134616),(#134617,#134618),(#134619,#134620),
(#134621,#134622),(#134623,#134624),(#134625,#134626),(#134627,#134628),
(#134629,#134630),(#134631,#134632),(#134633,#134634),(#134635,#134636),
(#134637,#134638),(#134639,#134640),(#134641,#134642),(#134643,#134644),
(#134645,#134646),(#134647,#134648),(#134649,#134650),(#134651,#134652),
(#134653,#134654),(#134655,#134656),(#134657,#134658),(#134659,#134660),
(#134661,#134662),(#134663,#134664),(#134665,#134666),(#134667,#134668),
(#134669,#134670),(#134671,#134672),(#134673,#134674),(#134675,#134676),
(#134677,#134678),(#134679,#134680),(#134681,#134682),(#134683,#134684),
(#134685,#134686),(#134687,#134688),(#134689,#134690),(#134691,#134692),
(#134693,#134694),(#134695,#134696),(#134697,#134698),(#134699,#134700),
(#134701,#134702),(#134703,#134704),(#134705,#134706),(#134707,#134708),
(#134709,#134710),(#134711,#134712),(#134713,#134714),(#134715,#134716),
(#134717,#134718),(#134719,#134720),(#134721,#134722),(#134723,#134724),
(#134725,#134726),(#134727,#134728),(#134729,#134730),(#134731,#134732),
(#134733,#134734),(#134735,#134736),(#134737,#134738),(#134739,#134740),
(#134741,#134742),(#134743,#134744),(#134745,#134746),(#134747,#134748),
(#134749,#134750),(#134751,#134752),(#134753,#134754),(#134755,#134756),
(#134757,#134758),(#134759,#134760),(#134761,#134762),(#134763,#134764),
(#134765,#134766),(#134767,#134768),(#134769,#134770),(#134771,#134772),
(#134773,#134774),(#134775,#134776),(#134777,#134778),(#134779,#134780),
(#134781,#134782),(#134783,#134784),(#134785,#134786),(#134787,#134788),
(#134789,#134790),(#134791,#134792),(#134793,#134794),(#134795,#134796),
(#134797,#134798),(#134799,#134800),(#134801,#134802),(#134803,#134804),
(#134805,#134806),(#134807,#134808),(#134809,#134810),(#134811,#134812),
(#134813,#134814),(#134815,#134816),(#134817,#134818),(#134819,#134820),
(#134821,#134822),(#134823,#134824),(#134825,#134826),(#134827,#134828),
(#134829,#134830),(#134831,#134832),(#134833,#134834),(#134835,#134836),
(#134837,#134838),(#134839,#134840),(#134841,#134842),(#134843,#134844),
(#134845,#134846),(#134847,#134848),(#134849,#134850),(#134851,#134852),
(#134853,#134854),(#134855,#134856),(#134857,#134858),(#134859,#134860),
(#134861,#134862),(#134863,#134864),(#134865,#134866),(#134867,#134868),
(#134869,#134870),(#134871,#134872),(#134873,#134874),(#134875,#134876),
(#134877,#134878),(#134879,#134880),(#134881,#134882),(#134883,#134884),
(#134885,#134886),(#134887,#134888),(#134889,#134890),(#134891,#134892),
(#134893,#134894),(#134895,#134896),(#134897,#134898),(#134899,#134900),
(#134901,#134902),(#134903,#134904),(#134905,#134906),(#134907,#134908),
(#134909,#134910),(#134911,#134912),(#134913,#134914),(#134915,#134916),
(#134917,#134918),(#134919,#134920),(#134921,#134922),(#134923,#134924),
(#134925,#134926),(#134927,#134928),(#134929,#134930),(#134931,#134932),
(#134933,#134934),(#134935,#134936),(#134937,#134938),(#134939,#134940),
(#134941,#134942),(#134943,#134944),(#134945,#134946),(#134947,#134948),
(#134949,#134950),(#134951,#134952),(#134953,#134954),(#134955,#134956),
(#134957,#134958),(#134959,#134960),(#134961,#134962),(#134963,#134964),
(#134965,#134966),(#134967,#134968),(#134969,#134970),(#134971,#134972),
(#134973,#134974),(#134975,#134976),(#134977,#134978),(#134979,#134980),
(#134981,#134982),(#134983,#134984),(#134985,#134986),(#134987,#134988),
(#134989,#134990),(#134991,#134992),(#134993,#134994),(#134995,#134996),
(#134997,#134998),(#134999,#135000),(#135001,#135002),(#135003,#135004),
(#135005,#135006),(#135007,#135008),(#135009,#135010),(#135011,#135012),
(#135013,#135014),(#135015,#135016),(#135017,#135018),(#135019,#135020),
(#135021,#135022),(#135023,#135024)),.UNSPECIFIED.,.F.,.F.,.F.)
B_SPLINE_SURFACE_WITH_KNOTS((6,1,1,1,1,1,1,1,1,1,1,1,1,1,1,1,1,1,1,1,1,
1,1,1,1,1,1,1,1,1,1,1,1,1,1,1,1,1,1,1,1,1,1,1,1,1,1,1,1,1,1,1,1,1,1,1,1,
1,1,1,1,1,1,1,1,1,1,1,1,1,1,1,1,1,1,1,1,1,1,1,1,1,1,1,1,1,1,1,1,1,1,1,1,
1,1,1,1,1,1,1,1,1,1,1,1,1,1,1,1,1,1,1,1,1,1,1,1,1,1,1,1,1,1,1,1,1,1,1,1,
1,1,1,1,1,1,1,1,1,1,1,1,1,1,1,1,1,1,1,1,1,1,1,1,1,1,1,1,1,1,1,1,1,1,1,1,
1,1,1,1,1,1,1,1,1,1,1,1,1,1,1,1,1,1,1,1,1,1,1,1,1,1,1,1,1,1,1,1,1,1,1,6),
(2,2),(-1.,-0.995000000000001,-0.990000000000001,-0.985000000000001,-0.980000000000001,
-0.975000000000001,-0.970000000000001,-0.965000000000001,-0.960000000000001,
-0.955000000000001,-0.950000000000001,-0.945000000000001,-0.940000000000001,
-0.935000000000001,-0.930000000000001,-0.925000000000001,-0.920000000000001,
-0.915000000000001,-0.910000000000001,-0.905000000000001,-0.900000000000001,
-0.895000000000001,-0.890000000000001,-0.885000000000001,-0.880000000000001,
-0.875000000000001,-0.870000000000001,-0.865000000000001,-0.860000000000001,
-0.855000000000001,-0.850000000000001,-0.845000000000001,-0.840000000000001,
-0.835000000000001,-0.830000000000001,-0.825000000000001,-0.820000000000001,
-0.815000000000001,-0.810000000000001,-0.805000000000001,-0.800000000000001,
-0.795000000000001,-0.790000000000001,-0.785000000000001,-0.780000000000001,
-0.775000000000001,-0.770000000000001,-0.765000000000001,-0.760000000000001,
-0.755000000000001,-0.750000000000001,-0.745000000000001,-0.740000000000001,
-0.735000000000001,-0.730000000000001,-0.725000000000001,-0.720000000000001,
-0.715000000000001,-0.710000000000001,-0.705000000000001,-0.700000000000001,
-0.695000000000001,-0.690000000000001,-0.685,-0.68,-0.675,-0.67,-0.665,
-0.66,-0.655,-0.65,-0.645,-0.64,-0.635,-0.63,-0.625,-0.62,-0.615,-0.61,
-0.605,-0.6,-0.595,-0.59,-0.585,-0.58,-0.575,-0.57,-0.565,-0.56,-0.555,
-0.55,-0.545,-0.54,-0.535,-0.53,-0.525,-0.52,-0.515,-0.51,-0.505,-0.5,-0.495,
-0.49,-0.485,-0.48,-0.475,-0.47,-0.465,-0.46,-0.455,-0.45,-0.445,-0.44,
-0.435,-0.43,-0.425,-0.42,-0.415,-0.41,-0.405,-0.4,-0.395,-0.39,-0.385,
-0.38,-0.375,-0.37,-0.365,-0.36,-0.355,-0.35,-0.345,-0.34,-0.335,-0.33,
-0.325,-0.32,-0.315,-0.31,-0.305,-0.3,-0.295,-0.29,-0.285,-0.28,-0.275,
-0.27,-0.265,-0.26,-0.255,-0.25,-0.245,-0.24,-0.235,-0.23,-0.225,-0.22,
-0.215,-0.21,-0.205,-0.2,-0.195,-0.19,-0.185,-0.18,-0.175,-0.17,-0.165,
-0.16,-0.155,-0.15,-0.145,-0.14,-0.135,-0.13,-0.125,-0.12,-0.115,-0.11,
-0.105,-0.1,-0.095,-0.09,-0.085,-0.08,-0.075,-0.07,-0.065,-0.06,-0.055,
-0.05,-0.045,-0.04,-0.035,-0.03,-0.025,-0.02,-0.015,-0.01,-0.005,0.),(0.,
1.2),.UNSPECIFIED.)
GEOMETRIC_REPRESENTATION_ITEM()
RATIONAL_B_SPLINE_SURFACE(((1.,1.),(1.,1.),(1.,1.),(1.,1.),(1.,1.),(1.,
1.),(1.,1.),(1.,1.),(1.,1.),(1.,1.),(1.,1.),(1.,1.),(1.,1.),(1.,1.),(1.,
1.),(1.,1.),(1.,1.),(1.,1.),(1.,1.),(1.,1.),(1.,1.),(1.,1.),(1.,1.),(1.,
1.),(1.,1.),(1.,1.),(1.,1.),(1.,1.),(1.,1.),(1.,1.),(1.,1.),(1.,1.),(1.,
1.),(1.,1.),(1.,1.),(1.,1.),(1.,1.),(1.,1.),(1.,1.),(1.,1.),(1.,1.),(1.,
1.),(1.,1.),(1.,1.),(1.,1.),(1.,1.),(1.,1.),(1.,1.),(1.,1.),(1.,1.),(1.,
1.),(1.,1.),(1.,1.),(1.,1.),(1.,1.),(1.,1.),(1.,1.),(1.,1.),(1.,1.),(1.,
1.),(1.,1.),(1.,1.),(1.,1.),(1.,1.),(1.,1.),(1.,1.),(1.,1.),(1.,1.),(1.,
1.),(1.,1.),(1.,1.),(1.,1.),(1.,1.),(1.,1.),(1.,1.),(1.,1.),(1.,1.),(1.,
1.),(1.,1.),(1.,1.),(1.,1.),(1.,1.),(1.,1.),(1.,1.),(1.,1.),(1.,1.),(1.,
1.),(1.,1.),(1.,1.),(1.,1.),(1.,1.),(1.,1.),(1.,1.),(1.,1.),(1.,1.),(1.,
1.),(1.,1.),(1.,1.),(1.,1.),(1.,1.),(1.,1.),(1.,1.),(1.,1.),(1.,1.),(1.,
1.),(1.,1.),(1.,1.),(1.,1.),(1.,1.),(1.,1.),(1.,1.),(1.,1.),(1.,1.),(1.,
1.),(1.,1.),(1.,1.),(1.,1.),(1.,1.),(1.,1.),(1.,1.),(1.,1.),(1.,1.),(1.,
1.),(1.,1.),(1.,1.),(1.,1.),(1.,1.),(1.,1.),(1.,1.),(1.,1.),(1.,1.),(1.,
1.),(1.,1.),(1.,1.),(1.,1.),(1.,1.),(1.,1.),(1.,1.),(1.,1.),(1.,1.),(1.,
1.),(1.,1.),(1.,1.),(1.,1.),(1.,1.),(1.,1.),(1.,1.),(1.,1.),(1.,1.),(1.,
1.),(1.,1.),(1.,1.),(1.,1.),(1.,1.),(1.,1.),(1.,1.),(1.,1.),(1.,1.),(1.,
1.),(1.,1.),(1.,1.),(1.,1.),(1.,1.),(1.,1.),(1.,1.),(1.,1.),(1.,1.),(1.,
1.),(1.,1.),(1.,1.),(1.,1.),(1.,1.),(1.,1.),(1.,1.),(1.,1.),(1.,1.),(1.,
1.),(1.,1.),(1.,1.),(1.,1.),(1.,1.),(1.,1.),(1.,1.),(1.,1.),(1.,1.),(1.,
1.),(1.,1.),(1.,1.),(1.,1.),(1.,1.),(1.,1.),(1.,1.),(1.,1.),(1.,1.),(1.,
1.),(1.,1.),(1.,1.),(1.,1.),(1.,1.),(1.,1.),(1.,1.),(1.,1.),(1.,1.),(1.,
1.),(1.,1.)))
REPRESENTATION_ITEM('')
SURFACE()
);
#978=(
BOUNDED_SURFACE()
B_SPLINE_SURFACE(5,1,((#135416,#135417),(#135418,#135419),(#135420,#135421),
(#135422,#135423),(#135424,#135425),(#135426,#135427),(#135428,#135429),
(#135430,#135431),(#135432,#135433),(#135434,#135435),(#135436,#135437),
(#135438,#135439),(#135440,#135441),(#135442,#135443),(#135444,#135445),
(#135446,#135447),(#135448,#135449),(#135450,#135451),(#135452,#135453),
(#135454,#135455),(#135456,#135457),(#135458,#135459),(#135460,#135461),
(#135462,#135463),(#135464,#135465),(#135466,#135467),(#135468,#135469),
(#135470,#135471),(#135472,#135473),(#135474,#135475),(#135476,#135477),
(#135478,#135479),(#135480,#135481),(#135482,#135483),(#135484,#135485),
(#135486,#135487),(#135488,#135489),(#135490,#135491),(#135492,#135493),
(#135494,#135495),(#135496,#135497),(#135498,#135499),(#135500,#135501),
(#135502,#135503),(#135504,#135505),(#135506,#135507),(#135508,#135509),
(#135510,#135511),(#135512,#135513),(#135514,#135515),(#135516,#135517),
(#135518,#135519),(#135520,#135521),(#135522,#135523),(#135524,#135525),
(#135526,#135527),(#135528,#135529),(#135530,#135531),(#135532,#135533),
(#135534,#135535),(#135536,#135537),(#135538,#135539),(#135540,#135541),
(#135542,#135543),(#135544,#135545),(#135546,#135547),(#135548,#135549),
(#135550,#135551),(#135552,#135553),(#135554,#135555),(#135556,#135557),
(#135558,#135559),(#135560,#135561),(#135562,#135563),(#135564,#135565),
(#135566,#135567),(#135568,#135569),(#135570,#135571),(#135572,#135573),
(#135574,#135575),(#135576,#135577),(#135578,#135579),(#135580,#135581),
(#135582,#135583),(#135584,#135585),(#135586,#135587),(#135588,#135589),
(#135590,#135591),(#135592,#135593),(#135594,#135595),(#135596,#135597),
(#135598,#135599),(#135600,#135601),(#135602,#135603),(#135604,#135605),
(#135606,#135607),(#135608,#135609),(#135610,#135611),(#135612,#135613),
(#135614,#135615),(#135616,#135617),(#135618,#135619),(#135620,#135621),
(#135622,#135623),(#135624,#135625),(#135626,#135627),(#135628,#135629),
(#135630,#135631),(#135632,#135633),(#135634,#135635),(#135636,#135637),
(#135638,#135639),(#135640,#135641),(#135642,#135643),(#135644,#135645),
(#135646,#135647),(#135648,#135649),(#135650,#135651),(#135652,#135653),
(#135654,#135655),(#135656,#135657),(#135658,#135659),(#135660,#135661),
(#135662,#135663),(#135664,#135665),(#135666,#135667),(#135668,#135669),
(#135670,#135671),(#135672,#135673),(#135674,#135675),(#135676,#135677),
(#135678,#135679),(#135680,#135681),(#135682,#135683),(#135684,#135685),
(#135686,#135687),(#135688,#135689),(#135690,#135691),(#135692,#135693),
(#135694,#135695),(#135696,#135697),(#135698,#135699),(#135700,#135701),
(#135702,#135703),(#135704,#135705),(#135706,#135707),(#135708,#135709),
(#135710,#135711),(#135712,#135713),(#135714,#135715),(#135716,#135717),
(#135718,#135719),(#135720,#135721),(#135722,#135723),(#135724,#135725),
(#135726,#135727),(#135728,#135729),(#135730,#135731),(#135732,#135733),
(#135734,#135735),(#135736,#135737),(#135738,#135739),(#135740,#135741),
(#135742,#135743),(#135744,#135745),(#135746,#135747),(#135748,#135749),
(#135750,#135751),(#135752,#135753),(#135754,#135755),(#135756,#135757),
(#135758,#135759),(#135760,#135761),(#135762,#135763),(#135764,#135765),
(#135766,#135767),(#135768,#135769),(#135770,#135771),(#135772,#135773),
(#135774,#135775),(#135776,#135777),(#135778,#135779),(#135780,#135781),
(#135782,#135783),(#135784,#135785),(#135786,#135787),(#135788,#135789),
(#135790,#135791),(#135792,#135793),(#135794,#135795),(#135796,#135797),
(#135798,#135799),(#135800,#135801),(#135802,#135803),(#135804,#135805),
(#135806,#135807),(#135808,#135809),(#135810,#135811),(#135812,#135813),
(#135814,#135815),(#135816,#135817),(#135818,#135819),(#135820,#135821),
(#135822,#135823),(#135824,#135825)),.UNSPECIFIED.,.F.,.F.,.F.)
B_SPLINE_SURFACE_WITH_KNOTS((6,1,1,1,1,1,1,1,1,1,1,1,1,1,1,1,1,1,1,1,1,
1,1,1,1,1,1,1,1,1,1,1,1,1,1,1,1,1,1,1,1,1,1,1,1,1,1,1,1,1,1,1,1,1,1,1,1,
1,1,1,1,1,1,1,1,1,1,1,1,1,1,1,1,1,1,1,1,1,1,1,1,1,1,1,1,1,1,1,1,1,1,1,1,
1,1,1,1,1,1,1,1,1,1,1,1,1,1,1,1,1,1,1,1,1,1,1,1,1,1,1,1,1,1,1,1,1,1,1,1,
1,1,1,1,1,1,1,1,1,1,1,1,1,1,1,1,1,1,1,1,1,1,1,1,1,1,1,1,1,1,1,1,1,1,1,1,
1,1,1,1,1,1,1,1,1,1,1,1,1,1,1,1,1,1,1,1,1,1,1,1,1,1,1,1,1,1,1,1,1,1,1,6),
(2,2),(-1.,-0.995000000000001,-0.990000000000001,-0.985000000000001,-0.980000000000001,
-0.975000000000001,-0.970000000000001,-0.965000000000001,-0.960000000000001,
-0.955000000000001,-0.950000000000001,-0.945000000000001,-0.940000000000001,
-0.935000000000001,-0.930000000000001,-0.925000000000001,-0.920000000000001,
-0.915000000000001,-0.910000000000001,-0.905000000000001,-0.900000000000001,
-0.895000000000001,-0.890000000000001,-0.885000000000001,-0.880000000000001,
-0.875000000000001,-0.870000000000001,-0.865000000000001,-0.860000000000001,
-0.855000000000001,-0.850000000000001,-0.845000000000001,-0.840000000000001,
-0.835000000000001,-0.830000000000001,-0.825000000000001,-0.820000000000001,
-0.815000000000001,-0.810000000000001,-0.805000000000001,-0.800000000000001,
-0.795000000000001,-0.790000000000001,-0.785000000000001,-0.780000000000001,
-0.775000000000001,-0.770000000000001,-0.765000000000001,-0.760000000000001,
-0.755000000000001,-0.750000000000001,-0.745000000000001,-0.740000000000001,
-0.735000000000001,-0.730000000000001,-0.725000000000001,-0.720000000000001,
-0.715000000000001,-0.710000000000001,-0.705000000000001,-0.700000000000001,
-0.695000000000001,-0.690000000000001,-0.685,-0.68,-0.675,-0.67,-0.665,
-0.66,-0.655,-0.65,-0.645,-0.64,-0.635,-0.63,-0.625,-0.62,-0.615,-0.61,
-0.605,-0.6,-0.595,-0.59,-0.585,-0.58,-0.575,-0.57,-0.565,-0.56,-0.555,
-0.55,-0.545,-0.54,-0.535,-0.53,-0.525,-0.52,-0.515,-0.51,-0.505,-0.5,-0.495,
-0.49,-0.485,-0.48,-0.475,-0.47,-0.465,-0.46,-0.455,-0.45,-0.445,-0.44,
-0.435,-0.43,-0.425,-0.42,-0.415,-0.41,-0.405,-0.4,-0.395,-0.39,-0.385,
-0.38,-0.375,-0.37,-0.365,-0.36,-0.355,-0.35,-0.345,-0.34,-0.335,-0.33,
-0.325,-0.32,-0.315,-0.31,-0.305,-0.3,-0.295,-0.29,-0.285,-0.28,-0.275,
-0.27,-0.265,-0.26,-0.255,-0.25,-0.245,-0.24,-0.235,-0.23,-0.225,-0.22,
-0.215,-0.21,-0.205,-0.2,-0.195,-0.19,-0.185,-0.18,-0.175,-0.17,-0.165,
-0.16,-0.155,-0.15,-0.145,-0.14,-0.135,-0.13,-0.125,-0.12,-0.115,-0.11,
-0.105,-0.1,-0.095,-0.09,-0.085,-0.08,-0.075,-0.07,-0.065,-0.06,-0.055,
-0.05,-0.045,-0.04,-0.035,-0.03,-0.025,-0.02,-0.015,-0.01,-0.005,0.),(0.,
1.2),.UNSPECIFIED.)
GEOMETRIC_REPRESENTATION_ITEM()
RATIONAL_B_SPLINE_SURFACE(((1.,1.),(1.,1.),(1.,1.),(1.,1.),(1.,1.),(1.,
1.),(1.,1.),(1.,1.),(1.,1.),(1.,1.),(1.,1.),(1.,1.),(1.,1.),(1.,1.),(1.,
1.),(1.,1.),(1.,1.),(1.,1.),(1.,1.),(1.,1.),(1.,1.),(1.,1.),(1.,1.),(1.,
1.),(1.,1.),(1.,1.),(1.,1.),(1.,1.),(1.,1.),(1.,1.),(1.,1.),(1.,1.),(1.,
1.),(1.,1.),(1.,1.),(1.,1.),(1.,1.),(1.,1.),(1.,1.),(1.,1.),(1.,1.),(1.,
1.),(1.,1.),(1.,1.),(1.,1.),(1.,1.),(1.,1.),(1.,1.),(1.,1.),(1.,1.),(1.,
1.),(1.,1.),(1.,1.),(1.,1.),(1.,1.),(1.,1.),(1.,1.),(1.,1.),(1.,1.),(1.,
1.),(1.,1.),(1.,1.),(1.,1.),(1.,1.),(1.,1.),(1.,1.),(1.,1.),(1.,1.),(1.,
1.),(1.,1.),(1.,1.),(1.,1.),(1.,1.),(1.,1.),(1.,1.),(1.,1.),(1.,1.),(1.,
1.),(1.,1.),(1.,1.),(1.,1.),(1.,1.),(1.,1.),(1.,1.),(1.,1.),(1.,1.),(1.,
1.),(1.,1.),(1.,1.),(1.,1.),(1.,1.),(1.,1.),(1.,1.),(1.,1.),(1.,1.),(1.,
1.),(1.,1.),(1.,1.),(1.,1.),(1.,1.),(1.,1.),(1.,1.),(1.,1.),(1.,1.),(1.,
1.),(1.,1.),(1.,1.),(1.,1.),(1.,1.),(1.,1.),(1.,1.),(1.,1.),(1.,1.),(1.,
1.),(1.,1.),(1.,1.),(1.,1.),(1.,1.),(1.,1.),(1.,1.),(1.,1.),(1.,1.),(1.,
1.),(1.,1.),(1.,1.),(1.,1.),(1.,1.),(1.,1.),(1.,1.),(1.,1.),(1.,1.),(1.,
1.),(1.,1.),(1.,1.),(1.,1.),(1.,1.),(1.,1.),(1.,1.),(1.,1.),(1.,1.),(1.,
1.),(1.,1.),(1.,1.),(1.,1.),(1.,1.),(1.,1.),(1.,1.),(1.,1.),(1.,1.),(1.,
1.),(1.,1.),(1.,1.),(1.,1.),(1.,1.),(1.,1.),(1.,1.),(1.,1.),(1.,1.),(1.,
1.),(1.,1.),(1.,1.),(1.,1.),(1.,1.),(1.,1.),(1.,1.),(1.,1.),(1.,1.),(1.,
1.),(1.,1.),(1.,1.),(1.,1.),(1.,1.),(1.,1.),(1.,1.),(1.,1.),(1.,1.),(1.,
1.),(1.,1.),(1.,1.),(1.,1.),(1.,1.),(1.,1.),(1.,1.),(1.,1.),(1.,1.),(1.,
1.),(1.,1.),(1.,1.),(1.,1.),(1.,1.),(1.,1.),(1.,1.),(1.,1.),(1.,1.),(1.,
1.),(1.,1.),(1.,1.),(1.,1.),(1.,1.),(1.,1.),(1.,1.),(1.,1.),(1.,1.),(1.,
1.),(1.,1.)))
REPRESENTATION_ITEM('')
SURFACE()
);
#979=(
BOUNDED_SURFACE()
B_SPLINE_SURFACE(5,1,((#136217,#136218),(#136219,#136220),(#136221,#136222),
(#136223,#136224),(#136225,#136226),(#136227,#136228),(#136229,#136230),
(#136231,#136232),(#136233,#136234),(#136235,#136236),(#136237,#136238),
(#136239,#136240),(#136241,#136242),(#136243,#136244),(#136245,#136246),
(#136247,#136248),(#136249,#136250),(#136251,#136252),(#136253,#136254),
(#136255,#136256),(#136257,#136258),(#136259,#136260),(#136261,#136262),
(#136263,#136264),(#136265,#136266),(#136267,#136268),(#136269,#136270),
(#136271,#136272),(#136273,#136274),(#136275,#136276),(#136277,#136278),
(#136279,#136280),(#136281,#136282),(#136283,#136284),(#136285,#136286),
(#136287,#136288),(#136289,#136290),(#136291,#136292),(#136293,#136294),
(#136295,#136296),(#136297,#136298),(#136299,#136300),(#136301,#136302),
(#136303,#136304),(#136305,#136306),(#136307,#136308),(#136309,#136310),
(#136311,#136312),(#136313,#136314),(#136315,#136316),(#136317,#136318),
(#136319,#136320),(#136321,#136322),(#136323,#136324),(#136325,#136326),
(#136327,#136328),(#136329,#136330),(#136331,#136332),(#136333,#136334),
(#136335,#136336),(#136337,#136338),(#136339,#136340),(#136341,#136342),
(#136343,#136344),(#136345,#136346),(#136347,#136348),(#136349,#136350),
(#136351,#136352),(#136353,#136354),(#136355,#136356),(#136357,#136358),
(#136359,#136360),(#136361,#136362),(#136363,#136364),(#136365,#136366),
(#136367,#136368),(#136369,#136370),(#136371,#136372),(#136373,#136374),
(#136375,#136376),(#136377,#136378),(#136379,#136380),(#136381,#136382),
(#136383,#136384),(#136385,#136386),(#136387,#136388),(#136389,#136390),
(#136391,#136392),(#136393,#136394),(#136395,#136396),(#136397,#136398),
(#136399,#136400),(#136401,#136402),(#136403,#136404),(#136405,#136406),
(#136407,#136408),(#136409,#136410),(#136411,#136412),(#136413,#136414),
(#136415,#136416),(#136417,#136418),(#136419,#136420),(#136421,#136422),
(#136423,#136424),(#136425,#136426),(#136427,#136428),(#136429,#136430),
(#136431,#136432),(#136433,#136434),(#136435,#136436),(#136437,#136438),
(#136439,#136440),(#136441,#136442),(#136443,#136444),(#136445,#136446),
(#136447,#136448),(#136449,#136450),(#136451,#136452),(#136453,#136454),
(#136455,#136456),(#136457,#136458),(#136459,#136460),(#136461,#136462),
(#136463,#136464),(#136465,#136466),(#136467,#136468),(#136469,#136470),
(#136471,#136472),(#136473,#136474),(#136475,#136476),(#136477,#136478),
(#136479,#136480),(#136481,#136482),(#136483,#136484),(#136485,#136486),
(#136487,#136488),(#136489,#136490),(#136491,#136492),(#136493,#136494),
(#136495,#136496),(#136497,#136498),(#136499,#136500),(#136501,#136502),
(#136503,#136504),(#136505,#136506),(#136507,#136508),(#136509,#136510),
(#136511,#136512),(#136513,#136514),(#136515,#136516),(#136517,#136518),
(#136519,#136520),(#136521,#136522),(#136523,#136524),(#136525,#136526),
(#136527,#136528),(#136529,#136530),(#136531,#136532),(#136533,#136534),
(#136535,#136536),(#136537,#136538),(#136539,#136540),(#136541,#136542),
(#136543,#136544),(#136545,#136546),(#136547,#136548),(#136549,#136550),
(#136551,#136552),(#136553,#136554),(#136555,#136556),(#136557,#136558),
(#136559,#136560),(#136561,#136562),(#136563,#136564),(#136565,#136566),
(#136567,#136568),(#136569,#136570),(#136571,#136572),(#136573,#136574),
(#136575,#136576),(#136577,#136578),(#136579,#136580),(#136581,#136582),
(#136583,#136584),(#136585,#136586),(#136587,#136588),(#136589,#136590),
(#136591,#136592),(#136593,#136594),(#136595,#136596),(#136597,#136598),
(#136599,#136600),(#136601,#136602),(#136603,#136604),(#136605,#136606),
(#136607,#136608),(#136609,#136610),(#136611,#136612),(#136613,#136614),
(#136615,#136616),(#136617,#136618),(#136619,#136620),(#136621,#136622),
(#136623,#136624),(#136625,#136626)),.UNSPECIFIED.,.F.,.F.,.F.)
B_SPLINE_SURFACE_WITH_KNOTS((6,1,1,1,1,1,1,1,1,1,1,1,1,1,1,1,1,1,1,1,1,
1,1,1,1,1,1,1,1,1,1,1,1,1,1,1,1,1,1,1,1,1,1,1,1,1,1,1,1,1,1,1,1,1,1,1,1,
1,1,1,1,1,1,1,1,1,1,1,1,1,1,1,1,1,1,1,1,1,1,1,1,1,1,1,1,1,1,1,1,1,1,1,1,
1,1,1,1,1,1,1,1,1,1,1,1,1,1,1,1,1,1,1,1,1,1,1,1,1,1,1,1,1,1,1,1,1,1,1,1,
1,1,1,1,1,1,1,1,1,1,1,1,1,1,1,1,1,1,1,1,1,1,1,1,1,1,1,1,1,1,1,1,1,1,1,1,
1,1,1,1,1,1,1,1,1,1,1,1,1,1,1,1,1,1,1,1,1,1,1,1,1,1,1,1,1,1,1,1,1,1,1,6),
(2,2),(-1.,-0.995000000000001,-0.990000000000001,-0.985000000000001,-0.980000000000001,
-0.975000000000001,-0.970000000000001,-0.965000000000001,-0.960000000000001,
-0.955000000000001,-0.950000000000001,-0.945000000000001,-0.940000000000001,
-0.935000000000001,-0.930000000000001,-0.925000000000001,-0.920000000000001,
-0.915000000000001,-0.910000000000001,-0.905000000000001,-0.900000000000001,
-0.895000000000001,-0.890000000000001,-0.885000000000001,-0.880000000000001,
-0.875000000000001,-0.870000000000001,-0.865000000000001,-0.860000000000001,
-0.855000000000001,-0.850000000000001,-0.845000000000001,-0.840000000000001,
-0.835000000000001,-0.830000000000001,-0.825000000000001,-0.820000000000001,
-0.815000000000001,-0.810000000000001,-0.805000000000001,-0.800000000000001,
-0.795000000000001,-0.790000000000001,-0.785000000000001,-0.780000000000001,
-0.775000000000001,-0.770000000000001,-0.765000000000001,-0.760000000000001,
-0.755000000000001,-0.750000000000001,-0.745000000000001,-0.740000000000001,
-0.735000000000001,-0.730000000000001,-0.725000000000001,-0.720000000000001,
-0.715000000000001,-0.710000000000001,-0.705000000000001,-0.700000000000001,
-0.695000000000001,-0.690000000000001,-0.685,-0.68,-0.675,-0.67,-0.665,
-0.66,-0.655,-0.65,-0.645,-0.64,-0.635,-0.63,-0.625,-0.62,-0.615,-0.61,
-0.605,-0.6,-0.595,-0.59,-0.585,-0.58,-0.575,-0.57,-0.565,-0.56,-0.555,
-0.55,-0.545,-0.54,-0.535,-0.53,-0.525,-0.52,-0.515,-0.51,-0.505,-0.5,-0.495,
-0.49,-0.485,-0.48,-0.475,-0.47,-0.465,-0.46,-0.455,-0.45,-0.445,-0.44,
-0.435,-0.43,-0.425,-0.42,-0.415,-0.41,-0.405,-0.4,-0.395,-0.39,-0.385,
-0.38,-0.375,-0.37,-0.365,-0.36,-0.355,-0.35,-0.345,-0.34,-0.335,-0.33,
-0.325,-0.32,-0.315,-0.31,-0.305,-0.3,-0.295,-0.29,-0.285,-0.28,-0.275,
-0.27,-0.265,-0.26,-0.255,-0.25,-0.245,-0.24,-0.235,-0.23,-0.225,-0.22,
-0.215,-0.21,-0.205,-0.2,-0.195,-0.19,-0.185,-0.18,-0.175,-0.17,-0.165,
-0.16,-0.155,-0.15,-0.145,-0.14,-0.135,-0.13,-0.125,-0.12,-0.115,-0.11,
-0.105,-0.1,-0.095,-0.09,-0.085,-0.08,-0.075,-0.07,-0.065,-0.06,-0.055,
-0.05,-0.045,-0.04,-0.035,-0.03,-0.025,-0.02,-0.015,-0.01,-0.005,0.),(0.,
1.2),.UNSPECIFIED.)
GEOMETRIC_REPRESENTATION_ITEM()
RATIONAL_B_SPLINE_SURFACE(((1.,1.),(1.,1.),(1.,1.),(1.,1.),(1.,1.),(1.,
1.),(1.,1.),(1.,1.),(1.,1.),(1.,1.),(1.,1.),(1.,1.),(1.,1.),(1.,1.),(1.,
1.),(1.,1.),(1.,1.),(1.,1.),(1.,1.),(1.,1.),(1.,1.),(1.,1.),(1.,1.),(1.,
1.),(1.,1.),(1.,1.),(1.,1.),(1.,1.),(1.,1.),(1.,1.),(1.,1.),(1.,1.),(1.,
1.),(1.,1.),(1.,1.),(1.,1.),(1.,1.),(1.,1.),(1.,1.),(1.,1.),(1.,1.),(1.,
1.),(1.,1.),(1.,1.),(1.,1.),(1.,1.),(1.,1.),(1.,1.),(1.,1.),(1.,1.),(1.,
1.),(1.,1.),(1.,1.),(1.,1.),(1.,1.),(1.,1.),(1.,1.),(1.,1.),(1.,1.),(1.,
1.),(1.,1.),(1.,1.),(1.,1.),(1.,1.),(1.,1.),(1.,1.),(1.,1.),(1.,1.),(1.,
1.),(1.,1.),(1.,1.),(1.,1.),(1.,1.),(1.,1.),(1.,1.),(1.,1.),(1.,1.),(1.,
1.),(1.,1.),(1.,1.),(1.,1.),(1.,1.),(1.,1.),(1.,1.),(1.,1.),(1.,1.),(1.,
1.),(1.,1.),(1.,1.),(1.,1.),(1.,1.),(1.,1.),(1.,1.),(1.,1.),(1.,1.),(1.,
1.),(1.,1.),(1.,1.),(1.,1.),(1.,1.),(1.,1.),(1.,1.),(1.,1.),(1.,1.),(1.,
1.),(1.,1.),(1.,1.),(1.,1.),(1.,1.),(1.,1.),(1.,1.),(1.,1.),(1.,1.),(1.,
1.),(1.,1.),(1.,1.),(1.,1.),(1.,1.),(1.,1.),(1.,1.),(1.,1.),(1.,1.),(1.,
1.),(1.,1.),(1.,1.),(1.,1.),(1.,1.),(1.,1.),(1.,1.),(1.,1.),(1.,1.),(1.,
1.),(1.,1.),(1.,1.),(1.,1.),(1.,1.),(1.,1.),(1.,1.),(1.,1.),(1.,1.),(1.,
1.),(1.,1.),(1.,1.),(1.,1.),(1.,1.),(1.,1.),(1.,1.),(1.,1.),(1.,1.),(1.,
1.),(1.,1.),(1.,1.),(1.,1.),(1.,1.),(1.,1.),(1.,1.),(1.,1.),(1.,1.),(1.,
1.),(1.,1.),(1.,1.),(1.,1.),(1.,1.),(1.,1.),(1.,1.),(1.,1.),(1.,1.),(1.,
1.),(1.,1.),(1.,1.),(1.,1.),(1.,1.),(1.,1.),(1.,1.),(1.,1.),(1.,1.),(1.,
1.),(1.,1.),(1.,1.),(1.,1.),(1.,1.),(1.,1.),(1.,1.),(1.,1.),(1.,1.),(1.,
1.),(1.,1.),(1.,1.),(1.,1.),(1.,1.),(1.,1.),(1.,1.),(1.,1.),(1.,1.),(1.,
1.),(1.,1.),(1.,1.),(1.,1.),(1.,1.),(1.,1.),(1.,1.),(1.,1.),(1.,1.),(1.,
1.),(1.,1.)))
REPRESENTATION_ITEM('')
SURFACE()
);
#980=(
BOUNDED_SURFACE()
B_SPLINE_SURFACE(5,1,((#137018,#137019),(#137020,#137021),(#137022,#137023),
(#137024,#137025),(#137026,#137027),(#137028,#137029),(#137030,#137031),
(#137032,#137033),(#137034,#137035),(#137036,#137037),(#137038,#137039),
(#137040,#137041),(#137042,#137043),(#137044,#137045),(#137046,#137047),
(#137048,#137049),(#137050,#137051),(#137052,#137053),(#137054,#137055),
(#137056,#137057),(#137058,#137059),(#137060,#137061),(#137062,#137063),
(#137064,#137065),(#137066,#137067),(#137068,#137069),(#137070,#137071),
(#137072,#137073),(#137074,#137075),(#137076,#137077),(#137078,#137079),
(#137080,#137081),(#137082,#137083),(#137084,#137085),(#137086,#137087),
(#137088,#137089),(#137090,#137091),(#137092,#137093),(#137094,#137095),
(#137096,#137097),(#137098,#137099),(#137100,#137101),(#137102,#137103),
(#137104,#137105),(#137106,#137107),(#137108,#137109),(#137110,#137111),
(#137112,#137113),(#137114,#137115),(#137116,#137117),(#137118,#137119),
(#137120,#137121),(#137122,#137123),(#137124,#137125),(#137126,#137127),
(#137128,#137129),(#137130,#137131),(#137132,#137133),(#137134,#137135),
(#137136,#137137),(#137138,#137139),(#137140,#137141),(#137142,#137143),
(#137144,#137145),(#137146,#137147),(#137148,#137149),(#137150,#137151),
(#137152,#137153),(#137154,#137155),(#137156,#137157),(#137158,#137159),
(#137160,#137161),(#137162,#137163),(#137164,#137165),(#137166,#137167),
(#137168,#137169),(#137170,#137171),(#137172,#137173),(#137174,#137175),
(#137176,#137177),(#137178,#137179),(#137180,#137181),(#137182,#137183),
(#137184,#137185),(#137186,#137187),(#137188,#137189),(#137190,#137191),
(#137192,#137193),(#137194,#137195),(#137196,#137197),(#137198,#137199),
(#137200,#137201),(#137202,#137203),(#137204,#137205),(#137206,#137207),
(#137208,#137209),(#137210,#137211),(#137212,#137213),(#137214,#137215),
(#137216,#137217),(#137218,#137219),(#137220,#137221),(#137222,#137223),
(#137224,#137225),(#137226,#137227),(#137228,#137229),(#137230,#137231),
(#137232,#137233),(#137234,#137235),(#137236,#137237),(#137238,#137239),
(#137240,#137241),(#137242,#137243),(#137244,#137245),(#137246,#137247),
(#137248,#137249),(#137250,#137251),(#137252,#137253),(#137254,#137255),
(#137256,#137257),(#137258,#137259),(#137260,#137261),(#137262,#137263),
(#137264,#137265),(#137266,#137267),(#137268,#137269),(#137270,#137271),
(#137272,#137273),(#137274,#137275),(#137276,#137277),(#137278,#137279),
(#137280,#137281),(#137282,#137283),(#137284,#137285),(#137286,#137287),
(#137288,#137289),(#137290,#137291),(#137292,#137293),(#137294,#137295),
(#137296,#137297),(#137298,#137299),(#137300,#137301),(#137302,#137303),
(#137304,#137305),(#137306,#137307),(#137308,#137309),(#137310,#137311),
(#137312,#137313),(#137314,#137315),(#137316,#137317),(#137318,#137319),
(#137320,#137321),(#137322,#137323),(#137324,#137325),(#137326,#137327),
(#137328,#137329),(#137330,#137331),(#137332,#137333),(#137334,#137335),
(#137336,#137337),(#137338,#137339),(#137340,#137341),(#137342,#137343),
(#137344,#137345),(#137346,#137347),(#137348,#137349),(#137350,#137351),
(#137352,#137353),(#137354,#137355),(#137356,#137357),(#137358,#137359),
(#137360,#137361),(#137362,#137363),(#137364,#137365),(#137366,#137367),
(#137368,#137369),(#137370,#137371),(#137372,#137373),(#137374,#137375),
(#137376,#137377),(#137378,#137379),(#137380,#137381),(#137382,#137383),
(#137384,#137385),(#137386,#137387),(#137388,#137389),(#137390,#137391),
(#137392,#137393),(#137394,#137395),(#137396,#137397),(#137398,#137399),
(#137400,#137401),(#137402,#137403),(#137404,#137405),(#137406,#137407),
(#137408,#137409),(#137410,#137411),(#137412,#137413),(#137414,#137415),
(#137416,#137417),(#137418,#137419),(#137420,#137421),(#137422,#137423),
(#137424,#137425),(#137426,#137427)),.UNSPECIFIED.,.F.,.F.,.F.)
B_SPLINE_SURFACE_WITH_KNOTS((6,1,1,1,1,1,1,1,1,1,1,1,1,1,1,1,1,1,1,1,1,
1,1,1,1,1,1,1,1,1,1,1,1,1,1,1,1,1,1,1,1,1,1,1,1,1,1,1,1,1,1,1,1,1,1,1,1,
1,1,1,1,1,1,1,1,1,1,1,1,1,1,1,1,1,1,1,1,1,1,1,1,1,1,1,1,1,1,1,1,1,1,1,1,
1,1,1,1,1,1,1,1,1,1,1,1,1,1,1,1,1,1,1,1,1,1,1,1,1,1,1,1,1,1,1,1,1,1,1,1,
1,1,1,1,1,1,1,1,1,1,1,1,1,1,1,1,1,1,1,1,1,1,1,1,1,1,1,1,1,1,1,1,1,1,1,1,
1,1,1,1,1,1,1,1,1,1,1,1,1,1,1,1,1,1,1,1,1,1,1,1,1,1,1,1,1,1,1,1,1,1,1,6),
(2,2),(-1.,-0.995000000000001,-0.990000000000001,-0.985000000000001,-0.980000000000001,
-0.975000000000001,-0.970000000000001,-0.965000000000001,-0.960000000000001,
-0.955000000000001,-0.950000000000001,-0.945000000000001,-0.940000000000001,
-0.935000000000001,-0.930000000000001,-0.925000000000001,-0.920000000000001,
-0.915000000000001,-0.910000000000001,-0.905000000000001,-0.900000000000001,
-0.895000000000001,-0.890000000000001,-0.885000000000001,-0.880000000000001,
-0.875000000000001,-0.870000000000001,-0.865000000000001,-0.860000000000001,
-0.855000000000001,-0.850000000000001,-0.845000000000001,-0.840000000000001,
-0.835000000000001,-0.830000000000001,-0.825000000000001,-0.820000000000001,
-0.815000000000001,-0.810000000000001,-0.805000000000001,-0.800000000000001,
-0.795000000000001,-0.790000000000001,-0.785000000000001,-0.780000000000001,
-0.775000000000001,-0.770000000000001,-0.765000000000001,-0.760000000000001,
-0.755000000000001,-0.750000000000001,-0.745000000000001,-0.740000000000001,
-0.735000000000001,-0.730000000000001,-0.725000000000001,-0.720000000000001,
-0.715000000000001,-0.710000000000001,-0.705000000000001,-0.700000000000001,
-0.695000000000001,-0.690000000000001,-0.685,-0.68,-0.675,-0.67,-0.665,
-0.66,-0.655,-0.65,-0.645,-0.64,-0.635,-0.63,-0.625,-0.62,-0.615,-0.61,
-0.605,-0.6,-0.595,-0.59,-0.585,-0.58,-0.575,-0.57,-0.565,-0.56,-0.555,
-0.55,-0.545,-0.54,-0.535,-0.53,-0.525,-0.52,-0.515,-0.51,-0.505,-0.5,-0.495,
-0.49,-0.485,-0.48,-0.475,-0.47,-0.465,-0.46,-0.455,-0.45,-0.445,-0.44,
-0.435,-0.43,-0.425,-0.42,-0.415,-0.41,-0.405,-0.4,-0.395,-0.39,-0.385,
-0.38,-0.375,-0.37,-0.365,-0.36,-0.355,-0.35,-0.345,-0.34,-0.335,-0.33,
-0.325,-0.32,-0.315,-0.31,-0.305,-0.3,-0.295,-0.29,-0.285,-0.28,-0.275,
-0.27,-0.265,-0.26,-0.255,-0.25,-0.245,-0.24,-0.235,-0.23,-0.225,-0.22,
-0.215,-0.21,-0.205,-0.2,-0.195,-0.19,-0.185,-0.18,-0.175,-0.17,-0.165,
-0.16,-0.155,-0.15,-0.145,-0.14,-0.135,-0.13,-0.125,-0.12,-0.115,-0.11,
-0.105,-0.1,-0.095,-0.09,-0.085,-0.08,-0.075,-0.07,-0.065,-0.06,-0.055,
-0.05,-0.045,-0.04,-0.035,-0.03,-0.025,-0.02,-0.015,-0.01,-0.005,0.),(0.,
1.2),.UNSPECIFIED.)
GEOMETRIC_REPRESENTATION_ITEM()
RATIONAL_B_SPLINE_SURFACE(((1.,1.),(1.,1.),(1.,1.),(1.,1.),(1.,1.),(1.,
1.),(1.,1.),(1.,1.),(1.,1.),(1.,1.),(1.,1.),(1.,1.),(1.,1.),(1.,1.),(1.,
1.),(1.,1.),(1.,1.),(1.,1.),(1.,1.),(1.,1.),(1.,1.),(1.,1.),(1.,1.),(1.,
1.),(1.,1.),(1.,1.),(1.,1.),(1.,1.),(1.,1.),(1.,1.),(1.,1.),(1.,1.),(1.,
1.),(1.,1.),(1.,1.),(1.,1.),(1.,1.),(1.,1.),(1.,1.),(1.,1.),(1.,1.),(1.,
1.),(1.,1.),(1.,1.),(1.,1.),(1.,1.),(1.,1.),(1.,1.),(1.,1.),(1.,1.),(1.,
1.),(1.,1.),(1.,1.),(1.,1.),(1.,1.),(1.,1.),(1.,1.),(1.,1.),(1.,1.),(1.,
1.),(1.,1.),(1.,1.),(1.,1.),(1.,1.),(1.,1.),(1.,1.),(1.,1.),(1.,1.),(1.,
1.),(1.,1.),(1.,1.),(1.,1.),(1.,1.),(1.,1.),(1.,1.),(1.,1.),(1.,1.),(1.,
1.),(1.,1.),(1.,1.),(1.,1.),(1.,1.),(1.,1.),(1.,1.),(1.,1.),(1.,1.),(1.,
1.),(1.,1.),(1.,1.),(1.,1.),(1.,1.),(1.,1.),(1.,1.),(1.,1.),(1.,1.),(1.,
1.),(1.,1.),(1.,1.),(1.,1.),(1.,1.),(1.,1.),(1.,1.),(1.,1.),(1.,1.),(1.,
1.),(1.,1.),(1.,1.),(1.,1.),(1.,1.),(1.,1.),(1.,1.),(1.,1.),(1.,1.),(1.,
1.),(1.,1.),(1.,1.),(1.,1.),(1.,1.),(1.,1.),(1.,1.),(1.,1.),(1.,1.),(1.,
1.),(1.,1.),(1.,1.),(1.,1.),(1.,1.),(1.,1.),(1.,1.),(1.,1.),(1.,1.),(1.,
1.),(1.,1.),(1.,1.),(1.,1.),(1.,1.),(1.,1.),(1.,1.),(1.,1.),(1.,1.),(1.,
1.),(1.,1.),(1.,1.),(1.,1.),(1.,1.),(1.,1.),(1.,1.),(1.,1.),(1.,1.),(1.,
1.),(1.,1.),(1.,1.),(1.,1.),(1.,1.),(1.,1.),(1.,1.),(1.,1.),(1.,1.),(1.,
1.),(1.,1.),(1.,1.),(1.,1.),(1.,1.),(1.,1.),(1.,1.),(1.,1.),(1.,1.),(1.,
1.),(1.,1.),(1.,1.),(1.,1.),(1.,1.),(1.,1.),(1.,1.),(1.,1.),(1.,1.),(1.,
1.),(1.,1.),(1.,1.),(1.,1.),(1.,1.),(1.,1.),(1.,1.),(1.,1.),(1.,1.),(1.,
1.),(1.,1.),(1.,1.),(1.,1.),(1.,1.),(1.,1.),(1.,1.),(1.,1.),(1.,1.),(1.,
1.),(1.,1.),(1.,1.),(1.,1.),(1.,1.),(1.,1.),(1.,1.),(1.,1.),(1.,1.),(1.,
1.),(1.,1.)))
REPRESENTATION_ITEM('')
SURFACE()
);
#981=(
BOUNDED_SURFACE()
B_SPLINE_SURFACE(5,1,((#137819,#137820),(#137821,#137822),(#137823,#137824),
(#137825,#137826),(#137827,#137828),(#137829,#137830),(#137831,#137832),
(#137833,#137834),(#137835,#137836),(#137837,#137838),(#137839,#137840),
(#137841,#137842),(#137843,#137844),(#137845,#137846),(#137847,#137848),
(#137849,#137850),(#137851,#137852),(#137853,#137854),(#137855,#137856),
(#137857,#137858),(#137859,#137860),(#137861,#137862),(#137863,#137864),
(#137865,#137866),(#137867,#137868),(#137869,#137870),(#137871,#137872),
(#137873,#137874),(#137875,#137876),(#137877,#137878),(#137879,#137880),
(#137881,#137882),(#137883,#137884),(#137885,#137886),(#137887,#137888),
(#137889,#137890),(#137891,#137892),(#137893,#137894),(#137895,#137896),
(#137897,#137898),(#137899,#137900),(#137901,#137902),(#137903,#137904),
(#137905,#137906),(#137907,#137908),(#137909,#137910),(#137911,#137912),
(#137913,#137914),(#137915,#137916),(#137917,#137918),(#137919,#137920),
(#137921,#137922),(#137923,#137924),(#137925,#137926),(#137927,#137928),
(#137929,#137930),(#137931,#137932),(#137933,#137934),(#137935,#137936),
(#137937,#137938),(#137939,#137940),(#137941,#137942),(#137943,#137944),
(#137945,#137946),(#137947,#137948),(#137949,#137950),(#137951,#137952),
(#137953,#137954),(#137955,#137956),(#137957,#137958),(#137959,#137960),
(#137961,#137962),(#137963,#137964),(#137965,#137966),(#137967,#137968),
(#137969,#137970),(#137971,#137972),(#137973,#137974),(#137975,#137976),
(#137977,#137978),(#137979,#137980),(#137981,#137982),(#137983,#137984),
(#137985,#137986),(#137987,#137988),(#137989,#137990),(#137991,#137992),
(#137993,#137994),(#137995,#137996),(#137997,#137998),(#137999,#138000),
(#138001,#138002),(#138003,#138004),(#138005,#138006),(#138007,#138008),
(#138009,#138010),(#138011,#138012),(#138013,#138014),(#138015,#138016),
(#138017,#138018),(#138019,#138020),(#138021,#138022),(#138023,#138024),
(#138025,#138026),(#138027,#138028),(#138029,#138030),(#138031,#138032),
(#138033,#138034),(#138035,#138036),(#138037,#138038),(#138039,#138040),
(#138041,#138042),(#138043,#138044),(#138045,#138046),(#138047,#138048),
(#138049,#138050),(#138051,#138052),(#138053,#138054),(#138055,#138056),
(#138057,#138058),(#138059,#138060),(#138061,#138062),(#138063,#138064),
(#138065,#138066),(#138067,#138068),(#138069,#138070),(#138071,#138072),
(#138073,#138074),(#138075,#138076),(#138077,#138078),(#138079,#138080),
(#138081,#138082),(#138083,#138084),(#138085,#138086),(#138087,#138088),
(#138089,#138090),(#138091,#138092),(#138093,#138094),(#138095,#138096),
(#138097,#138098),(#138099,#138100),(#138101,#138102),(#138103,#138104),
(#138105,#138106),(#138107,#138108),(#138109,#138110),(#138111,#138112),
(#138113,#138114),(#138115,#138116),(#138117,#138118),(#138119,#138120),
(#138121,#138122),(#138123,#138124),(#138125,#138126),(#138127,#138128),
(#138129,#138130),(#138131,#138132),(#138133,#138134),(#138135,#138136),
(#138137,#138138),(#138139,#138140),(#138141,#138142),(#138143,#138144),
(#138145,#138146),(#138147,#138148),(#138149,#138150),(#138151,#138152),
(#138153,#138154),(#138155,#138156),(#138157,#138158),(#138159,#138160),
(#138161,#138162),(#138163,#138164),(#138165,#138166),(#138167,#138168),
(#138169,#138170),(#138171,#138172),(#138173,#138174),(#138175,#138176),
(#138177,#138178),(#138179,#138180),(#138181,#138182),(#138183,#138184),
(#138185,#138186),(#138187,#138188),(#138189,#138190),(#138191,#138192),
(#138193,#138194),(#138195,#138196),(#138197,#138198),(#138199,#138200),
(#138201,#138202),(#138203,#138204),(#138205,#138206),(#138207,#138208),
(#138209,#138210),(#138211,#138212),(#138213,#138214),(#138215,#138216),
(#138217,#138218),(#138219,#138220),(#138221,#138222),(#138223,#138224),
(#138225,#138226),(#138227,#138228)),.UNSPECIFIED.,.F.,.F.,.F.)
B_SPLINE_SURFACE_WITH_KNOTS((6,1,1,1,1,1,1,1,1,1,1,1,1,1,1,1,1,1,1,1,1,
1,1,1,1,1,1,1,1,1,1,1,1,1,1,1,1,1,1,1,1,1,1,1,1,1,1,1,1,1,1,1,1,1,1,1,1,
1,1,1,1,1,1,1,1,1,1,1,1,1,1,1,1,1,1,1,1,1,1,1,1,1,1,1,1,1,1,1,1,1,1,1,1,
1,1,1,1,1,1,1,1,1,1,1,1,1,1,1,1,1,1,1,1,1,1,1,1,1,1,1,1,1,1,1,1,1,1,1,1,
1,1,1,1,1,1,1,1,1,1,1,1,1,1,1,1,1,1,1,1,1,1,1,1,1,1,1,1,1,1,1,1,1,1,1,1,
1,1,1,1,1,1,1,1,1,1,1,1,1,1,1,1,1,1,1,1,1,1,1,1,1,1,1,1,1,1,1,1,1,1,1,6),
(2,2),(-1.,-0.995000000000001,-0.990000000000001,-0.985000000000001,-0.980000000000001,
-0.975000000000001,-0.970000000000001,-0.965000000000001,-0.960000000000001,
-0.955000000000001,-0.950000000000001,-0.945000000000001,-0.940000000000001,
-0.935000000000001,-0.930000000000001,-0.925000000000001,-0.920000000000001,
-0.915000000000001,-0.910000000000001,-0.905000000000001,-0.900000000000001,
-0.895000000000001,-0.890000000000001,-0.885000000000001,-0.880000000000001,
-0.875000000000001,-0.870000000000001,-0.865000000000001,-0.860000000000001,
-0.855000000000001,-0.850000000000001,-0.845000000000001,-0.840000000000001,
-0.835000000000001,-0.830000000000001,-0.825000000000001,-0.820000000000001,
-0.815000000000001,-0.810000000000001,-0.805000000000001,-0.800000000000001,
-0.795000000000001,-0.790000000000001,-0.785000000000001,-0.780000000000001,
-0.775000000000001,-0.770000000000001,-0.765000000000001,-0.760000000000001,
-0.755000000000001,-0.750000000000001,-0.745000000000001,-0.740000000000001,
-0.735000000000001,-0.730000000000001,-0.725000000000001,-0.720000000000001,
-0.715000000000001,-0.710000000000001,-0.705000000000001,-0.700000000000001,
-0.695000000000001,-0.690000000000001,-0.685,-0.68,-0.675,-0.67,-0.665,
-0.66,-0.655,-0.65,-0.645,-0.64,-0.635,-0.63,-0.625,-0.62,-0.615,-0.61,
-0.605,-0.6,-0.595,-0.59,-0.585,-0.58,-0.575,-0.57,-0.565,-0.56,-0.555,
-0.55,-0.545,-0.54,-0.535,-0.53,-0.525,-0.52,-0.515,-0.51,-0.505,-0.5,-0.495,
-0.49,-0.485,-0.48,-0.475,-0.47,-0.465,-0.46,-0.455,-0.45,-0.445,-0.44,
-0.435,-0.43,-0.425,-0.42,-0.415,-0.41,-0.405,-0.4,-0.395,-0.39,-0.385,
-0.38,-0.375,-0.37,-0.365,-0.36,-0.355,-0.35,-0.345,-0.34,-0.335,-0.33,
-0.325,-0.32,-0.315,-0.31,-0.305,-0.3,-0.295,-0.29,-0.285,-0.28,-0.275,
-0.27,-0.265,-0.26,-0.255,-0.25,-0.245,-0.24,-0.235,-0.23,-0.225,-0.22,
-0.215,-0.21,-0.205,-0.2,-0.195,-0.19,-0.185,-0.18,-0.175,-0.17,-0.165,
-0.16,-0.155,-0.15,-0.145,-0.14,-0.135,-0.13,-0.125,-0.12,-0.115,-0.11,
-0.105,-0.1,-0.095,-0.09,-0.085,-0.08,-0.075,-0.07,-0.065,-0.06,-0.055,
-0.05,-0.045,-0.04,-0.035,-0.03,-0.025,-0.02,-0.015,-0.01,-0.005,0.),(0.,
1.2),.UNSPECIFIED.)
GEOMETRIC_REPRESENTATION_ITEM()
RATIONAL_B_SPLINE_SURFACE(((1.,1.),(1.,1.),(1.,1.),(1.,1.),(1.,1.),(1.,
1.),(1.,1.),(1.,1.),(1.,1.),(1.,1.),(1.,1.),(1.,1.),(1.,1.),(1.,1.),(1.,
1.),(1.,1.),(1.,1.),(1.,1.),(1.,1.),(1.,1.),(1.,1.),(1.,1.),(1.,1.),(1.,
1.),(1.,1.),(1.,1.),(1.,1.),(1.,1.),(1.,1.),(1.,1.),(1.,1.),(1.,1.),(1.,
1.),(1.,1.),(1.,1.),(1.,1.),(1.,1.),(1.,1.),(1.,1.),(1.,1.),(1.,1.),(1.,
1.),(1.,1.),(1.,1.),(1.,1.),(1.,1.),(1.,1.),(1.,1.),(1.,1.),(1.,1.),(1.,
1.),(1.,1.),(1.,1.),(1.,1.),(1.,1.),(1.,1.),(1.,1.),(1.,1.),(1.,1.),(1.,
1.),(1.,1.),(1.,1.),(1.,1.),(1.,1.),(1.,1.),(1.,1.),(1.,1.),(1.,1.),(1.,
1.),(1.,1.),(1.,1.),(1.,1.),(1.,1.),(1.,1.),(1.,1.),(1.,1.),(1.,1.),(1.,
1.),(1.,1.),(1.,1.),(1.,1.),(1.,1.),(1.,1.),(1.,1.),(1.,1.),(1.,1.),(1.,
1.),(1.,1.),(1.,1.),(1.,1.),(1.,1.),(1.,1.),(1.,1.),(1.,1.),(1.,1.),(1.,
1.),(1.,1.),(1.,1.),(1.,1.),(1.,1.),(1.,1.),(1.,1.),(1.,1.),(1.,1.),(1.,
1.),(1.,1.),(1.,1.),(1.,1.),(1.,1.),(1.,1.),(1.,1.),(1.,1.),(1.,1.),(1.,
1.),(1.,1.),(1.,1.),(1.,1.),(1.,1.),(1.,1.),(1.,1.),(1.,1.),(1.,1.),(1.,
1.),(1.,1.),(1.,1.),(1.,1.),(1.,1.),(1.,1.),(1.,1.),(1.,1.),(1.,1.),(1.,
1.),(1.,1.),(1.,1.),(1.,1.),(1.,1.),(1.,1.),(1.,1.),(1.,1.),(1.,1.),(1.,
1.),(1.,1.),(1.,1.),(1.,1.),(1.,1.),(1.,1.),(1.,1.),(1.,1.),(1.,1.),(1.,
1.),(1.,1.),(1.,1.),(1.,1.),(1.,1.),(1.,1.),(1.,1.),(1.,1.),(1.,1.),(1.,
1.),(1.,1.),(1.,1.),(1.,1.),(1.,1.),(1.,1.),(1.,1.),(1.,1.),(1.,1.),(1.,
1.),(1.,1.),(1.,1.),(1.,1.),(1.,1.),(1.,1.),(1.,1.),(1.,1.),(1.,1.),(1.,
1.),(1.,1.),(1.,1.),(1.,1.),(1.,1.),(1.,1.),(1.,1.),(1.,1.),(1.,1.),(1.,
1.),(1.,1.),(1.,1.),(1.,1.),(1.,1.),(1.,1.),(1.,1.),(1.,1.),(1.,1.),(1.,
1.),(1.,1.),(1.,1.),(1.,1.),(1.,1.),(1.,1.),(1.,1.),(1.,1.),(1.,1.),(1.,
1.),(1.,1.)))
REPRESENTATION_ITEM('')
SURFACE()
);
#982=(
BOUNDED_SURFACE()
B_SPLINE_SURFACE(5,1,((#138620,#138621),(#138622,#138623),(#138624,#138625),
(#138626,#138627),(#138628,#138629),(#138630,#138631),(#138632,#138633),
(#138634,#138635),(#138636,#138637),(#138638,#138639),(#138640,#138641),
(#138642,#138643),(#138644,#138645),(#138646,#138647),(#138648,#138649),
(#138650,#138651),(#138652,#138653),(#138654,#138655),(#138656,#138657),
(#138658,#138659),(#138660,#138661),(#138662,#138663),(#138664,#138665),
(#138666,#138667),(#138668,#138669),(#138670,#138671),(#138672,#138673),
(#138674,#138675),(#138676,#138677),(#138678,#138679),(#138680,#138681),
(#138682,#138683),(#138684,#138685),(#138686,#138687),(#138688,#138689),
(#138690,#138691),(#138692,#138693),(#138694,#138695),(#138696,#138697),
(#138698,#138699),(#138700,#138701),(#138702,#138703),(#138704,#138705),
(#138706,#138707),(#138708,#138709),(#138710,#138711),(#138712,#138713),
(#138714,#138715),(#138716,#138717),(#138718,#138719),(#138720,#138721),
(#138722,#138723),(#138724,#138725),(#138726,#138727),(#138728,#138729),
(#138730,#138731),(#138732,#138733),(#138734,#138735),(#138736,#138737),
(#138738,#138739),(#138740,#138741),(#138742,#138743),(#138744,#138745),
(#138746,#138747),(#138748,#138749),(#138750,#138751),(#138752,#138753),
(#138754,#138755),(#138756,#138757),(#138758,#138759),(#138760,#138761),
(#138762,#138763),(#138764,#138765),(#138766,#138767),(#138768,#138769),
(#138770,#138771),(#138772,#138773),(#138774,#138775),(#138776,#138777),
(#138778,#138779),(#138780,#138781),(#138782,#138783),(#138784,#138785),
(#138786,#138787),(#138788,#138789),(#138790,#138791),(#138792,#138793),
(#138794,#138795),(#138796,#138797),(#138798,#138799),(#138800,#138801),
(#138802,#138803),(#138804,#138805),(#138806,#138807),(#138808,#138809),
(#138810,#138811),(#138812,#138813),(#138814,#138815),(#138816,#138817),
(#138818,#138819),(#138820,#138821),(#138822,#138823),(#138824,#138825),
(#138826,#138827),(#138828,#138829),(#138830,#138831),(#138832,#138833),
(#138834,#138835),(#138836,#138837),(#138838,#138839),(#138840,#138841),
(#138842,#138843),(#138844,#138845),(#138846,#138847),(#138848,#138849),
(#138850,#138851),(#138852,#138853),(#138854,#138855),(#138856,#138857),
(#138858,#138859),(#138860,#138861),(#138862,#138863),(#138864,#138865),
(#138866,#138867),(#138868,#138869),(#138870,#138871),(#138872,#138873),
(#138874,#138875),(#138876,#138877),(#138878,#138879),(#138880,#138881),
(#138882,#138883),(#138884,#138885),(#138886,#138887),(#138888,#138889),
(#138890,#138891),(#138892,#138893),(#138894,#138895),(#138896,#138897),
(#138898,#138899),(#138900,#138901),(#138902,#138903),(#138904,#138905),
(#138906,#138907),(#138908,#138909),(#138910,#138911),(#138912,#138913),
(#138914,#138915),(#138916,#138917),(#138918,#138919),(#138920,#138921),
(#138922,#138923),(#138924,#138925),(#138926,#138927),(#138928,#138929),
(#138930,#138931),(#138932,#138933),(#138934,#138935),(#138936,#138937),
(#138938,#138939),(#138940,#138941),(#138942,#138943),(#138944,#138945),
(#138946,#138947),(#138948,#138949),(#138950,#138951),(#138952,#138953),
(#138954,#138955),(#138956,#138957),(#138958,#138959),(#138960,#138961),
(#138962,#138963),(#138964,#138965),(#138966,#138967),(#138968,#138969),
(#138970,#138971),(#138972,#138973),(#138974,#138975),(#138976,#138977),
(#138978,#138979),(#138980,#138981),(#138982,#138983),(#138984,#138985),
(#138986,#138987),(#138988,#138989),(#138990,#138991),(#138992,#138993),
(#138994,#138995),(#138996,#138997),(#138998,#138999),(#139000,#139001),
(#139002,#139003),(#139004,#139005),(#139006,#139007),(#139008,#139009),
(#139010,#139011),(#139012,#139013),(#139014,#139015),(#139016,#139017),
(#139018,#139019),(#139020,#139021),(#139022,#139023),(#139024,#139025),
(#139026,#139027),(#139028,#139029)),.UNSPECIFIED.,.F.,.F.,.F.)
B_SPLINE_SURFACE_WITH_KNOTS((6,1,1,1,1,1,1,1,1,1,1,1,1,1,1,1,1,1,1,1,1,
1,1,1,1,1,1,1,1,1,1,1,1,1,1,1,1,1,1,1,1,1,1,1,1,1,1,1,1,1,1,1,1,1,1,1,1,
1,1,1,1,1,1,1,1,1,1,1,1,1,1,1,1,1,1,1,1,1,1,1,1,1,1,1,1,1,1,1,1,1,1,1,1,
1,1,1,1,1,1,1,1,1,1,1,1,1,1,1,1,1,1,1,1,1,1,1,1,1,1,1,1,1,1,1,1,1,1,1,1,
1,1,1,1,1,1,1,1,1,1,1,1,1,1,1,1,1,1,1,1,1,1,1,1,1,1,1,1,1,1,1,1,1,1,1,1,
1,1,1,1,1,1,1,1,1,1,1,1,1,1,1,1,1,1,1,1,1,1,1,1,1,1,1,1,1,1,1,1,1,1,1,6),
(2,2),(-1.,-0.995000000000001,-0.990000000000001,-0.985000000000001,-0.980000000000001,
-0.975000000000001,-0.970000000000001,-0.965000000000001,-0.960000000000001,
-0.955000000000001,-0.950000000000001,-0.945000000000001,-0.940000000000001,
-0.935000000000001,-0.930000000000001,-0.925000000000001,-0.920000000000001,
-0.915000000000001,-0.910000000000001,-0.905000000000001,-0.900000000000001,
-0.895000000000001,-0.890000000000001,-0.885000000000001,-0.880000000000001,
-0.875000000000001,-0.870000000000001,-0.865000000000001,-0.860000000000001,
-0.855000000000001,-0.850000000000001,-0.845000000000001,-0.840000000000001,
-0.835000000000001,-0.830000000000001,-0.825000000000001,-0.820000000000001,
-0.815000000000001,-0.810000000000001,-0.805000000000001,-0.800000000000001,
-0.795000000000001,-0.790000000000001,-0.785000000000001,-0.780000000000001,
-0.775000000000001,-0.770000000000001,-0.765000000000001,-0.760000000000001,
-0.755000000000001,-0.750000000000001,-0.745000000000001,-0.740000000000001,
-0.735000000000001,-0.730000000000001,-0.725000000000001,-0.720000000000001,
-0.715000000000001,-0.710000000000001,-0.705000000000001,-0.700000000000001,
-0.695000000000001,-0.690000000000001,-0.685,-0.68,-0.675,-0.67,-0.665,
-0.66,-0.655,-0.65,-0.645,-0.64,-0.635,-0.63,-0.625,-0.62,-0.615,-0.61,
-0.605,-0.6,-0.595,-0.59,-0.585,-0.58,-0.575,-0.57,-0.565,-0.56,-0.555,
-0.55,-0.545,-0.54,-0.535,-0.53,-0.525,-0.52,-0.515,-0.51,-0.505,-0.5,-0.495,
-0.49,-0.485,-0.48,-0.475,-0.47,-0.465,-0.46,-0.455,-0.45,-0.445,-0.44,
-0.435,-0.43,-0.425,-0.42,-0.415,-0.41,-0.405,-0.4,-0.395,-0.39,-0.385,
-0.38,-0.375,-0.37,-0.365,-0.36,-0.355,-0.35,-0.345,-0.34,-0.335,-0.33,
-0.325,-0.32,-0.315,-0.31,-0.305,-0.3,-0.295,-0.29,-0.285,-0.28,-0.275,
-0.27,-0.265,-0.26,-0.255,-0.25,-0.245,-0.24,-0.235,-0.23,-0.225,-0.22,
-0.215,-0.21,-0.205,-0.2,-0.195,-0.19,-0.185,-0.18,-0.175,-0.17,-0.165,
-0.16,-0.155,-0.15,-0.145,-0.14,-0.135,-0.13,-0.125,-0.12,-0.115,-0.11,
-0.105,-0.1,-0.095,-0.09,-0.085,-0.08,-0.075,-0.07,-0.065,-0.06,-0.055,
-0.05,-0.045,-0.04,-0.035,-0.03,-0.025,-0.02,-0.015,-0.01,-0.005,0.),(0.,
1.2),.UNSPECIFIED.)
GEOMETRIC_REPRESENTATION_ITEM()
RATIONAL_B_SPLINE_SURFACE(((1.,1.),(1.,1.),(1.,1.),(1.,1.),(1.,1.),(1.,
1.),(1.,1.),(1.,1.),(1.,1.),(1.,1.),(1.,1.),(1.,1.),(1.,1.),(1.,1.),(1.,
1.),(1.,1.),(1.,1.),(1.,1.),(1.,1.),(1.,1.),(1.,1.),(1.,1.),(1.,1.),(1.,
1.),(1.,1.),(1.,1.),(1.,1.),(1.,1.),(1.,1.),(1.,1.),(1.,1.),(1.,1.),(1.,
1.),(1.,1.),(1.,1.),(1.,1.),(1.,1.),(1.,1.),(1.,1.),(1.,1.),(1.,1.),(1.,
1.),(1.,1.),(1.,1.),(1.,1.),(1.,1.),(1.,1.),(1.,1.),(1.,1.),(1.,1.),(1.,
1.),(1.,1.),(1.,1.),(1.,1.),(1.,1.),(1.,1.),(1.,1.),(1.,1.),(1.,1.),(1.,
1.),(1.,1.),(1.,1.),(1.,1.),(1.,1.),(1.,1.),(1.,1.),(1.,1.),(1.,1.),(1.,
1.),(1.,1.),(1.,1.),(1.,1.),(1.,1.),(1.,1.),(1.,1.),(1.,1.),(1.,1.),(1.,
1.),(1.,1.),(1.,1.),(1.,1.),(1.,1.),(1.,1.),(1.,1.),(1.,1.),(1.,1.),(1.,
1.),(1.,1.),(1.,1.),(1.,1.),(1.,1.),(1.,1.),(1.,1.),(1.,1.),(1.,1.),(1.,
1.),(1.,1.),(1.,1.),(1.,1.),(1.,1.),(1.,1.),(1.,1.),(1.,1.),(1.,1.),(1.,
1.),(1.,1.),(1.,1.),(1.,1.),(1.,1.),(1.,1.),(1.,1.),(1.,1.),(1.,1.),(1.,
1.),(1.,1.),(1.,1.),(1.,1.),(1.,1.),(1.,1.),(1.,1.),(1.,1.),(1.,1.),(1.,
1.),(1.,1.),(1.,1.),(1.,1.),(1.,1.),(1.,1.),(1.,1.),(1.,1.),(1.,1.),(1.,
1.),(1.,1.),(1.,1.),(1.,1.),(1.,1.),(1.,1.),(1.,1.),(1.,1.),(1.,1.),(1.,
1.),(1.,1.),(1.,1.),(1.,1.),(1.,1.),(1.,1.),(1.,1.),(1.,1.),(1.,1.),(1.,
1.),(1.,1.),(1.,1.),(1.,1.),(1.,1.),(1.,1.),(1.,1.),(1.,1.),(1.,1.),(1.,
1.),(1.,1.),(1.,1.),(1.,1.),(1.,1.),(1.,1.),(1.,1.),(1.,1.),(1.,1.),(1.,
1.),(1.,1.),(1.,1.),(1.,1.),(1.,1.),(1.,1.),(1.,1.),(1.,1.),(1.,1.),(1.,
1.),(1.,1.),(1.,1.),(1.,1.),(1.,1.),(1.,1.),(1.,1.),(1.,1.),(1.,1.),(1.,
1.),(1.,1.),(1.,1.),(1.,1.),(1.,1.),(1.,1.),(1.,1.),(1.,1.),(1.,1.),(1.,
1.),(1.,1.),(1.,1.),(1.,1.),(1.,1.),(1.,1.),(1.,1.),(1.,1.),(1.,1.),(1.,
1.),(1.,1.)))
REPRESENTATION_ITEM('')
SURFACE()
);
#983=(
BOUNDED_SURFACE()
B_SPLINE_SURFACE(5,1,((#139421,#139422),(#139423,#139424),(#139425,#139426),
(#139427,#139428),(#139429,#139430),(#139431,#139432),(#139433,#139434),
(#139435,#139436),(#139437,#139438),(#139439,#139440),(#139441,#139442),
(#139443,#139444),(#139445,#139446),(#139447,#139448),(#139449,#139450),
(#139451,#139452),(#139453,#139454),(#139455,#139456),(#139457,#139458),
(#139459,#139460),(#139461,#139462),(#139463,#139464),(#139465,#139466),
(#139467,#139468),(#139469,#139470),(#139471,#139472),(#139473,#139474),
(#139475,#139476),(#139477,#139478),(#139479,#139480),(#139481,#139482),
(#139483,#139484),(#139485,#139486),(#139487,#139488),(#139489,#139490),
(#139491,#139492),(#139493,#139494),(#139495,#139496),(#139497,#139498),
(#139499,#139500),(#139501,#139502),(#139503,#139504),(#139505,#139506),
(#139507,#139508),(#139509,#139510),(#139511,#139512),(#139513,#139514),
(#139515,#139516),(#139517,#139518),(#139519,#139520),(#139521,#139522),
(#139523,#139524),(#139525,#139526),(#139527,#139528),(#139529,#139530),
(#139531,#139532),(#139533,#139534),(#139535,#139536),(#139537,#139538),
(#139539,#139540),(#139541,#139542),(#139543,#139544),(#139545,#139546),
(#139547,#139548),(#139549,#139550),(#139551,#139552),(#139553,#139554),
(#139555,#139556),(#139557,#139558),(#139559,#139560),(#139561,#139562),
(#139563,#139564),(#139565,#139566),(#139567,#139568),(#139569,#139570),
(#139571,#139572),(#139573,#139574),(#139575,#139576),(#139577,#139578),
(#139579,#139580),(#139581,#139582),(#139583,#139584),(#139585,#139586),
(#139587,#139588),(#139589,#139590),(#139591,#139592),(#139593,#139594),
(#139595,#139596),(#139597,#139598),(#139599,#139600),(#139601,#139602),
(#139603,#139604),(#139605,#139606),(#139607,#139608),(#139609,#139610),
(#139611,#139612),(#139613,#139614),(#139615,#139616),(#139617,#139618),
(#139619,#139620),(#139621,#139622),(#139623,#139624),(#139625,#139626),
(#139627,#139628),(#139629,#139630),(#139631,#139632),(#139633,#139634),
(#139635,#139636),(#139637,#139638),(#139639,#139640),(#139641,#139642),
(#139643,#139644),(#139645,#139646),(#139647,#139648),(#139649,#139650),
(#139651,#139652),(#139653,#139654),(#139655,#139656),(#139657,#139658),
(#139659,#139660),(#139661,#139662),(#139663,#139664),(#139665,#139666),
(#139667,#139668),(#139669,#139670),(#139671,#139672),(#139673,#139674),
(#139675,#139676),(#139677,#139678),(#139679,#139680),(#139681,#139682),
(#139683,#139684),(#139685,#139686),(#139687,#139688),(#139689,#139690),
(#139691,#139692),(#139693,#139694),(#139695,#139696),(#139697,#139698),
(#139699,#139700),(#139701,#139702),(#139703,#139704),(#139705,#139706),
(#139707,#139708),(#139709,#139710),(#139711,#139712),(#139713,#139714),
(#139715,#139716),(#139717,#139718),(#139719,#139720),(#139721,#139722),
(#139723,#139724),(#139725,#139726),(#139727,#139728),(#139729,#139730),
(#139731,#139732),(#139733,#139734),(#139735,#139736),(#139737,#139738),
(#139739,#139740),(#139741,#139742),(#139743,#139744),(#139745,#139746),
(#139747,#139748),(#139749,#139750),(#139751,#139752),(#139753,#139754),
(#139755,#139756),(#139757,#139758),(#139759,#139760),(#139761,#139762),
(#139763,#139764),(#139765,#139766),(#139767,#139768),(#139769,#139770),
(#139771,#139772),(#139773,#139774),(#139775,#139776),(#139777,#139778),
(#139779,#139780),(#139781,#139782),(#139783,#139784),(#139785,#139786),
(#139787,#139788),(#139789,#139790),(#139791,#139792),(#139793,#139794),
(#139795,#139796),(#139797,#139798),(#139799,#139800),(#139801,#139802),
(#139803,#139804),(#139805,#139806),(#139807,#139808),(#139809,#139810),
(#139811,#139812),(#139813,#139814),(#139815,#139816),(#139817,#139818),
(#139819,#139820),(#139821,#139822),(#139823,#139824),(#139825,#139826),
(#139827,#139828),(#139829,#139830)),.UNSPECIFIED.,.F.,.F.,.F.)
B_SPLINE_SURFACE_WITH_KNOTS((6,1,1,1,1,1,1,1,1,1,1,1,1,1,1,1,1,1,1,1,1,
1,1,1,1,1,1,1,1,1,1,1,1,1,1,1,1,1,1,1,1,1,1,1,1,1,1,1,1,1,1,1,1,1,1,1,1,
1,1,1,1,1,1,1,1,1,1,1,1,1,1,1,1,1,1,1,1,1,1,1,1,1,1,1,1,1,1,1,1,1,1,1,1,
1,1,1,1,1,1,1,1,1,1,1,1,1,1,1,1,1,1,1,1,1,1,1,1,1,1,1,1,1,1,1,1,1,1,1,1,
1,1,1,1,1,1,1,1,1,1,1,1,1,1,1,1,1,1,1,1,1,1,1,1,1,1,1,1,1,1,1,1,1,1,1,1,
1,1,1,1,1,1,1,1,1,1,1,1,1,1,1,1,1,1,1,1,1,1,1,1,1,1,1,1,1,1,1,1,1,1,1,6),
(2,2),(-1.,-0.995000000000001,-0.990000000000001,-0.985000000000001,-0.980000000000001,
-0.975000000000001,-0.970000000000001,-0.965000000000001,-0.960000000000001,
-0.955000000000001,-0.950000000000001,-0.945000000000001,-0.940000000000001,
-0.935000000000001,-0.930000000000001,-0.925000000000001,-0.920000000000001,
-0.915000000000001,-0.910000000000001,-0.905000000000001,-0.900000000000001,
-0.895000000000001,-0.890000000000001,-0.885000000000001,-0.880000000000001,
-0.875000000000001,-0.870000000000001,-0.865000000000001,-0.860000000000001,
-0.855000000000001,-0.850000000000001,-0.845000000000001,-0.840000000000001,
-0.835000000000001,-0.830000000000001,-0.825000000000001,-0.820000000000001,
-0.815000000000001,-0.810000000000001,-0.805000000000001,-0.800000000000001,
-0.795000000000001,-0.790000000000001,-0.785000000000001,-0.780000000000001,
-0.775000000000001,-0.770000000000001,-0.765000000000001,-0.760000000000001,
-0.755000000000001,-0.750000000000001,-0.745000000000001,-0.740000000000001,
-0.735000000000001,-0.730000000000001,-0.725000000000001,-0.720000000000001,
-0.715000000000001,-0.710000000000001,-0.705000000000001,-0.700000000000001,
-0.695000000000001,-0.690000000000001,-0.685,-0.68,-0.675,-0.67,-0.665,
-0.66,-0.655,-0.65,-0.645,-0.64,-0.635,-0.63,-0.625,-0.62,-0.615,-0.61,
-0.605,-0.6,-0.595,-0.59,-0.585,-0.58,-0.575,-0.57,-0.565,-0.56,-0.555,
-0.55,-0.545,-0.54,-0.535,-0.53,-0.525,-0.52,-0.515,-0.51,-0.505,-0.5,-0.495,
-0.49,-0.485,-0.48,-0.475,-0.47,-0.465,-0.46,-0.455,-0.45,-0.445,-0.44,
-0.435,-0.43,-0.425,-0.42,-0.415,-0.41,-0.405,-0.4,-0.395,-0.39,-0.385,
-0.38,-0.375,-0.37,-0.365,-0.36,-0.355,-0.35,-0.345,-0.34,-0.335,-0.33,
-0.325,-0.32,-0.315,-0.31,-0.305,-0.3,-0.295,-0.29,-0.285,-0.28,-0.275,
-0.27,-0.265,-0.26,-0.255,-0.25,-0.245,-0.24,-0.235,-0.23,-0.225,-0.22,
-0.215,-0.21,-0.205,-0.2,-0.195,-0.19,-0.185,-0.18,-0.175,-0.17,-0.165,
-0.16,-0.155,-0.15,-0.145,-0.14,-0.135,-0.13,-0.125,-0.12,-0.115,-0.11,
-0.105,-0.1,-0.095,-0.09,-0.085,-0.08,-0.075,-0.07,-0.065,-0.06,-0.055,
-0.05,-0.045,-0.04,-0.035,-0.03,-0.025,-0.02,-0.015,-0.01,-0.005,0.),(0.,
1.2),.UNSPECIFIED.)
GEOMETRIC_REPRESENTATION_ITEM()
RATIONAL_B_SPLINE_SURFACE(((1.,1.),(1.,1.),(1.,1.),(1.,1.),(1.,1.),(1.,
1.),(1.,1.),(1.,1.),(1.,1.),(1.,1.),(1.,1.),(1.,1.),(1.,1.),(1.,1.),(1.,
1.),(1.,1.),(1.,1.),(1.,1.),(1.,1.),(1.,1.),(1.,1.),(1.,1.),(1.,1.),(1.,
1.),(1.,1.),(1.,1.),(1.,1.),(1.,1.),(1.,1.),(1.,1.),(1.,1.),(1.,1.),(1.,
1.),(1.,1.),(1.,1.),(1.,1.),(1.,1.),(1.,1.),(1.,1.),(1.,1.),(1.,1.),(1.,
1.),(1.,1.),(1.,1.),(1.,1.),(1.,1.),(1.,1.),(1.,1.),(1.,1.),(1.,1.),(1.,
1.),(1.,1.),(1.,1.),(1.,1.),(1.,1.),(1.,1.),(1.,1.),(1.,1.),(1.,1.),(1.,
1.),(1.,1.),(1.,1.),(1.,1.),(1.,1.),(1.,1.),(1.,1.),(1.,1.),(1.,1.),(1.,
1.),(1.,1.),(1.,1.),(1.,1.),(1.,1.),(1.,1.),(1.,1.),(1.,1.),(1.,1.),(1.,
1.),(1.,1.),(1.,1.),(1.,1.),(1.,1.),(1.,1.),(1.,1.),(1.,1.),(1.,1.),(1.,
1.),(1.,1.),(1.,1.),(1.,1.),(1.,1.),(1.,1.),(1.,1.),(1.,1.),(1.,1.),(1.,
1.),(1.,1.),(1.,1.),(1.,1.),(1.,1.),(1.,1.),(1.,1.),(1.,1.),(1.,1.),(1.,
1.),(1.,1.),(1.,1.),(1.,1.),(1.,1.),(1.,1.),(1.,1.),(1.,1.),(1.,1.),(1.,
1.),(1.,1.),(1.,1.),(1.,1.),(1.,1.),(1.,1.),(1.,1.),(1.,1.),(1.,1.),(1.,
1.),(1.,1.),(1.,1.),(1.,1.),(1.,1.),(1.,1.),(1.,1.),(1.,1.),(1.,1.),(1.,
1.),(1.,1.),(1.,1.),(1.,1.),(1.,1.),(1.,1.),(1.,1.),(1.,1.),(1.,1.),(1.,
1.),(1.,1.),(1.,1.),(1.,1.),(1.,1.),(1.,1.),(1.,1.),(1.,1.),(1.,1.),(1.,
1.),(1.,1.),(1.,1.),(1.,1.),(1.,1.),(1.,1.),(1.,1.),(1.,1.),(1.,1.),(1.,
1.),(1.,1.),(1.,1.),(1.,1.),(1.,1.),(1.,1.),(1.,1.),(1.,1.),(1.,1.),(1.,
1.),(1.,1.),(1.,1.),(1.,1.),(1.,1.),(1.,1.),(1.,1.),(1.,1.),(1.,1.),(1.,
1.),(1.,1.),(1.,1.),(1.,1.),(1.,1.),(1.,1.),(1.,1.),(1.,1.),(1.,1.),(1.,
1.),(1.,1.),(1.,1.),(1.,1.),(1.,1.),(1.,1.),(1.,1.),(1.,1.),(1.,1.),(1.,
1.),(1.,1.),(1.,1.),(1.,1.),(1.,1.),(1.,1.),(1.,1.),(1.,1.),(1.,1.),(1.,
1.),(1.,1.)))
REPRESENTATION_ITEM('')
SURFACE()
);
#984=(
BOUNDED_SURFACE()
B_SPLINE_SURFACE(5,1,((#140222,#140223),(#140224,#140225),(#140226,#140227),
(#140228,#140229),(#140230,#140231),(#140232,#140233),(#140234,#140235),
(#140236,#140237),(#140238,#140239),(#140240,#140241),(#140242,#140243),
(#140244,#140245),(#140246,#140247),(#140248,#140249),(#140250,#140251),
(#140252,#140253),(#140254,#140255),(#140256,#140257),(#140258,#140259),
(#140260,#140261),(#140262,#140263),(#140264,#140265),(#140266,#140267),
(#140268,#140269),(#140270,#140271),(#140272,#140273),(#140274,#140275),
(#140276,#140277),(#140278,#140279),(#140280,#140281),(#140282,#140283),
(#140284,#140285),(#140286,#140287),(#140288,#140289),(#140290,#140291),
(#140292,#140293),(#140294,#140295),(#140296,#140297),(#140298,#140299),
(#140300,#140301),(#140302,#140303),(#140304,#140305),(#140306,#140307),
(#140308,#140309),(#140310,#140311),(#140312,#140313),(#140314,#140315),
(#140316,#140317),(#140318,#140319),(#140320,#140321),(#140322,#140323),
(#140324,#140325),(#140326,#140327),(#140328,#140329),(#140330,#140331),
(#140332,#140333),(#140334,#140335),(#140336,#140337),(#140338,#140339),
(#140340,#140341),(#140342,#140343),(#140344,#140345),(#140346,#140347),
(#140348,#140349),(#140350,#140351),(#140352,#140353),(#140354,#140355),
(#140356,#140357),(#140358,#140359),(#140360,#140361),(#140362,#140363),
(#140364,#140365),(#140366,#140367),(#140368,#140369),(#140370,#140371),
(#140372,#140373),(#140374,#140375),(#140376,#140377),(#140378,#140379),
(#140380,#140381),(#140382,#140383),(#140384,#140385),(#140386,#140387),
(#140388,#140389),(#140390,#140391),(#140392,#140393),(#140394,#140395),
(#140396,#140397),(#140398,#140399),(#140400,#140401),(#140402,#140403),
(#140404,#140405),(#140406,#140407),(#140408,#140409),(#140410,#140411),
(#140412,#140413),(#140414,#140415),(#140416,#140417),(#140418,#140419),
(#140420,#140421),(#140422,#140423),(#140424,#140425),(#140426,#140427),
(#140428,#140429),(#140430,#140431),(#140432,#140433),(#140434,#140435),
(#140436,#140437),(#140438,#140439),(#140440,#140441),(#140442,#140443),
(#140444,#140445),(#140446,#140447),(#140448,#140449),(#140450,#140451),
(#140452,#140453),(#140454,#140455),(#140456,#140457),(#140458,#140459),
(#140460,#140461),(#140462,#140463),(#140464,#140465),(#140466,#140467),
(#140468,#140469),(#140470,#140471),(#140472,#140473),(#140474,#140475),
(#140476,#140477),(#140478,#140479),(#140480,#140481),(#140482,#140483),
(#140484,#140485),(#140486,#140487),(#140488,#140489),(#140490,#140491),
(#140492,#140493),(#140494,#140495),(#140496,#140497),(#140498,#140499),
(#140500,#140501),(#140502,#140503),(#140504,#140505),(#140506,#140507),
(#140508,#140509),(#140510,#140511),(#140512,#140513),(#140514,#140515),
(#140516,#140517),(#140518,#140519),(#140520,#140521),(#140522,#140523),
(#140524,#140525),(#140526,#140527),(#140528,#140529),(#140530,#140531),
(#140532,#140533),(#140534,#140535),(#140536,#140537),(#140538,#140539),
(#140540,#140541),(#140542,#140543),(#140544,#140545),(#140546,#140547),
(#140548,#140549),(#140550,#140551),(#140552,#140553),(#140554,#140555),
(#140556,#140557),(#140558,#140559),(#140560,#140561),(#140562,#140563),
(#140564,#140565),(#140566,#140567),(#140568,#140569),(#140570,#140571),
(#140572,#140573),(#140574,#140575),(#140576,#140577),(#140578,#140579),
(#140580,#140581),(#140582,#140583),(#140584,#140585),(#140586,#140587),
(#140588,#140589),(#140590,#140591),(#140592,#140593),(#140594,#140595),
(#140596,#140597),(#140598,#140599),(#140600,#140601),(#140602,#140603),
(#140604,#140605),(#140606,#140607),(#140608,#140609),(#140610,#140611),
(#140612,#140613),(#140614,#140615),(#140616,#140617),(#140618,#140619),
(#140620,#140621),(#140622,#140623),(#140624,#140625),(#140626,#140627),
(#140628,#140629),(#140630,#140631)),.UNSPECIFIED.,.F.,.F.,.F.)
B_SPLINE_SURFACE_WITH_KNOTS((6,1,1,1,1,1,1,1,1,1,1,1,1,1,1,1,1,1,1,1,1,
1,1,1,1,1,1,1,1,1,1,1,1,1,1,1,1,1,1,1,1,1,1,1,1,1,1,1,1,1,1,1,1,1,1,1,1,
1,1,1,1,1,1,1,1,1,1,1,1,1,1,1,1,1,1,1,1,1,1,1,1,1,1,1,1,1,1,1,1,1,1,1,1,
1,1,1,1,1,1,1,1,1,1,1,1,1,1,1,1,1,1,1,1,1,1,1,1,1,1,1,1,1,1,1,1,1,1,1,1,
1,1,1,1,1,1,1,1,1,1,1,1,1,1,1,1,1,1,1,1,1,1,1,1,1,1,1,1,1,1,1,1,1,1,1,1,
1,1,1,1,1,1,1,1,1,1,1,1,1,1,1,1,1,1,1,1,1,1,1,1,1,1,1,1,1,1,1,1,1,1,1,6),
(2,2),(-1.,-0.995000000000001,-0.990000000000001,-0.985000000000001,-0.980000000000001,
-0.975000000000001,-0.970000000000001,-0.965000000000001,-0.960000000000001,
-0.955000000000001,-0.950000000000001,-0.945000000000001,-0.940000000000001,
-0.935000000000001,-0.930000000000001,-0.925000000000001,-0.920000000000001,
-0.915000000000001,-0.910000000000001,-0.905000000000001,-0.900000000000001,
-0.895000000000001,-0.890000000000001,-0.885000000000001,-0.880000000000001,
-0.875000000000001,-0.870000000000001,-0.865000000000001,-0.860000000000001,
-0.855000000000001,-0.850000000000001,-0.845000000000001,-0.840000000000001,
-0.835000000000001,-0.830000000000001,-0.825000000000001,-0.820000000000001,
-0.815000000000001,-0.810000000000001,-0.805000000000001,-0.800000000000001,
-0.795000000000001,-0.790000000000001,-0.785000000000001,-0.780000000000001,
-0.775000000000001,-0.770000000000001,-0.765000000000001,-0.760000000000001,
-0.755000000000001,-0.750000000000001,-0.745000000000001,-0.740000000000001,
-0.735000000000001,-0.730000000000001,-0.725000000000001,-0.720000000000001,
-0.715000000000001,-0.710000000000001,-0.705000000000001,-0.700000000000001,
-0.695000000000001,-0.690000000000001,-0.685,-0.68,-0.675,-0.67,-0.665,
-0.66,-0.655,-0.65,-0.645,-0.64,-0.635,-0.63,-0.625,-0.62,-0.615,-0.61,
-0.605,-0.6,-0.595,-0.59,-0.585,-0.58,-0.575,-0.57,-0.565,-0.56,-0.555,
-0.55,-0.545,-0.54,-0.535,-0.53,-0.525,-0.52,-0.515,-0.51,-0.505,-0.5,-0.495,
-0.49,-0.485,-0.48,-0.475,-0.47,-0.465,-0.46,-0.455,-0.45,-0.445,-0.44,
-0.435,-0.43,-0.425,-0.42,-0.415,-0.41,-0.405,-0.4,-0.395,-0.39,-0.385,
-0.38,-0.375,-0.37,-0.365,-0.36,-0.355,-0.35,-0.345,-0.34,-0.335,-0.33,
-0.325,-0.32,-0.315,-0.31,-0.305,-0.3,-0.295,-0.29,-0.285,-0.28,-0.275,
-0.27,-0.265,-0.26,-0.255,-0.25,-0.245,-0.24,-0.235,-0.23,-0.225,-0.22,
-0.215,-0.21,-0.205,-0.2,-0.195,-0.19,-0.185,-0.18,-0.175,-0.17,-0.165,
-0.16,-0.155,-0.15,-0.145,-0.14,-0.135,-0.13,-0.125,-0.12,-0.115,-0.11,
-0.105,-0.1,-0.095,-0.09,-0.085,-0.08,-0.075,-0.07,-0.065,-0.06,-0.055,
-0.05,-0.045,-0.04,-0.035,-0.03,-0.025,-0.02,-0.015,-0.01,-0.005,0.),(0.,
1.2),.UNSPECIFIED.)
GEOMETRIC_REPRESENTATION_ITEM()
RATIONAL_B_SPLINE_SURFACE(((1.,1.),(1.,1.),(1.,1.),(1.,1.),(1.,1.),(1.,
1.),(1.,1.),(1.,1.),(1.,1.),(1.,1.),(1.,1.),(1.,1.),(1.,1.),(1.,1.),(1.,
1.),(1.,1.),(1.,1.),(1.,1.),(1.,1.),(1.,1.),(1.,1.),(1.,1.),(1.,1.),(1.,
1.),(1.,1.),(1.,1.),(1.,1.),(1.,1.),(1.,1.),(1.,1.),(1.,1.),(1.,1.),(1.,
1.),(1.,1.),(1.,1.),(1.,1.),(1.,1.),(1.,1.),(1.,1.),(1.,1.),(1.,1.),(1.,
1.),(1.,1.),(1.,1.),(1.,1.),(1.,1.),(1.,1.),(1.,1.),(1.,1.),(1.,1.),(1.,
1.),(1.,1.),(1.,1.),(1.,1.),(1.,1.),(1.,1.),(1.,1.),(1.,1.),(1.,1.),(1.,
1.),(1.,1.),(1.,1.),(1.,1.),(1.,1.),(1.,1.),(1.,1.),(1.,1.),(1.,1.),(1.,
1.),(1.,1.),(1.,1.),(1.,1.),(1.,1.),(1.,1.),(1.,1.),(1.,1.),(1.,1.),(1.,
1.),(1.,1.),(1.,1.),(1.,1.),(1.,1.),(1.,1.),(1.,1.),(1.,1.),(1.,1.),(1.,
1.),(1.,1.),(1.,1.),(1.,1.),(1.,1.),(1.,1.),(1.,1.),(1.,1.),(1.,1.),(1.,
1.),(1.,1.),(1.,1.),(1.,1.),(1.,1.),(1.,1.),(1.,1.),(1.,1.),(1.,1.),(1.,
1.),(1.,1.),(1.,1.),(1.,1.),(1.,1.),(1.,1.),(1.,1.),(1.,1.),(1.,1.),(1.,
1.),(1.,1.),(1.,1.),(1.,1.),(1.,1.),(1.,1.),(1.,1.),(1.,1.),(1.,1.),(1.,
1.),(1.,1.),(1.,1.),(1.,1.),(1.,1.),(1.,1.),(1.,1.),(1.,1.),(1.,1.),(1.,
1.),(1.,1.),(1.,1.),(1.,1.),(1.,1.),(1.,1.),(1.,1.),(1.,1.),(1.,1.),(1.,
1.),(1.,1.),(1.,1.),(1.,1.),(1.,1.),(1.,1.),(1.,1.),(1.,1.),(1.,1.),(1.,
1.),(1.,1.),(1.,1.),(1.,1.),(1.,1.),(1.,1.),(1.,1.),(1.,1.),(1.,1.),(1.,
1.),(1.,1.),(1.,1.),(1.,1.),(1.,1.),(1.,1.),(1.,1.),(1.,1.),(1.,1.),(1.,
1.),(1.,1.),(1.,1.),(1.,1.),(1.,1.),(1.,1.),(1.,1.),(1.,1.),(1.,1.),(1.,
1.),(1.,1.),(1.,1.),(1.,1.),(1.,1.),(1.,1.),(1.,1.),(1.,1.),(1.,1.),(1.,
1.),(1.,1.),(1.,1.),(1.,1.),(1.,1.),(1.,1.),(1.,1.),(1.,1.),(1.,1.),(1.,
1.),(1.,1.),(1.,1.),(1.,1.),(1.,1.),(1.,1.),(1.,1.),(1.,1.),(1.,1.),(1.,
1.),(1.,1.)))
REPRESENTATION_ITEM('')
SURFACE()
);
#985=(
BOUNDED_SURFACE()
B_SPLINE_SURFACE(5,1,((#141023,#141024),(#141025,#141026),(#141027,#141028),
(#141029,#141030),(#141031,#141032),(#141033,#141034),(#141035,#141036),
(#141037,#141038),(#141039,#141040),(#141041,#141042),(#141043,#141044),
(#141045,#141046),(#141047,#141048),(#141049,#141050),(#141051,#141052),
(#141053,#141054),(#141055,#141056),(#141057,#141058),(#141059,#141060),
(#141061,#141062),(#141063,#141064),(#141065,#141066),(#141067,#141068),
(#141069,#141070),(#141071,#141072),(#141073,#141074),(#141075,#141076),
(#141077,#141078),(#141079,#141080),(#141081,#141082),(#141083,#141084),
(#141085,#141086),(#141087,#141088),(#141089,#141090),(#141091,#141092),
(#141093,#141094),(#141095,#141096),(#141097,#141098),(#141099,#141100),
(#141101,#141102),(#141103,#141104),(#141105,#141106),(#141107,#141108),
(#141109,#141110),(#141111,#141112),(#141113,#141114),(#141115,#141116),
(#141117,#141118),(#141119,#141120),(#141121,#141122),(#141123,#141124),
(#141125,#141126),(#141127,#141128),(#141129,#141130),(#141131,#141132),
(#141133,#141134),(#141135,#141136),(#141137,#141138),(#141139,#141140),
(#141141,#141142),(#141143,#141144),(#141145,#141146),(#141147,#141148),
(#141149,#141150),(#141151,#141152),(#141153,#141154),(#141155,#141156),
(#141157,#141158),(#141159,#141160),(#141161,#141162),(#141163,#141164),
(#141165,#141166),(#141167,#141168),(#141169,#141170),(#141171,#141172),
(#141173,#141174),(#141175,#141176),(#141177,#141178),(#141179,#141180),
(#141181,#141182),(#141183,#141184),(#141185,#141186),(#141187,#141188),
(#141189,#141190),(#141191,#141192),(#141193,#141194),(#141195,#141196),
(#141197,#141198),(#141199,#141200),(#141201,#141202),(#141203,#141204),
(#141205,#141206),(#141207,#141208),(#141209,#141210),(#141211,#141212),
(#141213,#141214),(#141215,#141216),(#141217,#141218),(#141219,#141220),
(#141221,#141222),(#141223,#141224),(#141225,#141226),(#141227,#141228),
(#141229,#141230),(#141231,#141232),(#141233,#141234),(#141235,#141236),
(#141237,#141238),(#141239,#141240),(#141241,#141242),(#141243,#141244),
(#141245,#141246),(#141247,#141248),(#141249,#141250),(#141251,#141252),
(#141253,#141254),(#141255,#141256),(#141257,#141258),(#141259,#141260),
(#141261,#141262),(#141263,#141264),(#141265,#141266),(#141267,#141268),
(#141269,#141270),(#141271,#141272),(#141273,#141274),(#141275,#141276),
(#141277,#141278),(#141279,#141280),(#141281,#141282),(#141283,#141284),
(#141285,#141286),(#141287,#141288),(#141289,#141290),(#141291,#141292),
(#141293,#141294),(#141295,#141296),(#141297,#141298),(#141299,#141300),
(#141301,#141302),(#141303,#141304),(#141305,#141306),(#141307,#141308),
(#141309,#141310),(#141311,#141312),(#141313,#141314),(#141315,#141316),
(#141317,#141318),(#141319,#141320),(#141321,#141322),(#141323,#141324),
(#141325,#141326),(#141327,#141328),(#141329,#141330),(#141331,#141332),
(#141333,#141334),(#141335,#141336),(#141337,#141338),(#141339,#141340),
(#141341,#141342),(#141343,#141344),(#141345,#141346),(#141347,#141348),
(#141349,#141350),(#141351,#141352),(#141353,#141354),(#141355,#141356),
(#141357,#141358),(#141359,#141360),(#141361,#141362),(#141363,#141364),
(#141365,#141366),(#141367,#141368),(#141369,#141370),(#141371,#141372),
(#141373,#141374),(#141375,#141376),(#141377,#141378),(#141379,#141380),
(#141381,#141382),(#141383,#141384),(#141385,#141386),(#141387,#141388),
(#141389,#141390),(#141391,#141392),(#141393,#141394),(#141395,#141396),
(#141397,#141398),(#141399,#141400),(#141401,#141402),(#141403,#141404),
(#141405,#141406),(#141407,#141408),(#141409,#141410),(#141411,#141412),
(#141413,#141414),(#141415,#141416),(#141417,#141418),(#141419,#141420),
(#141421,#141422),(#141423,#141424),(#141425,#141426),(#141427,#141428),
(#141429,#141430),(#141431,#141432)),.UNSPECIFIED.,.F.,.F.,.F.)
B_SPLINE_SURFACE_WITH_KNOTS((6,1,1,1,1,1,1,1,1,1,1,1,1,1,1,1,1,1,1,1,1,
1,1,1,1,1,1,1,1,1,1,1,1,1,1,1,1,1,1,1,1,1,1,1,1,1,1,1,1,1,1,1,1,1,1,1,1,
1,1,1,1,1,1,1,1,1,1,1,1,1,1,1,1,1,1,1,1,1,1,1,1,1,1,1,1,1,1,1,1,1,1,1,1,
1,1,1,1,1,1,1,1,1,1,1,1,1,1,1,1,1,1,1,1,1,1,1,1,1,1,1,1,1,1,1,1,1,1,1,1,
1,1,1,1,1,1,1,1,1,1,1,1,1,1,1,1,1,1,1,1,1,1,1,1,1,1,1,1,1,1,1,1,1,1,1,1,
1,1,1,1,1,1,1,1,1,1,1,1,1,1,1,1,1,1,1,1,1,1,1,1,1,1,1,1,1,1,1,1,1,1,1,6),
(2,2),(-1.,-0.995000000000001,-0.990000000000001,-0.985000000000001,-0.980000000000001,
-0.975000000000001,-0.970000000000001,-0.965000000000001,-0.960000000000001,
-0.955000000000001,-0.950000000000001,-0.945000000000001,-0.940000000000001,
-0.935000000000001,-0.930000000000001,-0.925000000000001,-0.920000000000001,
-0.915000000000001,-0.910000000000001,-0.905000000000001,-0.900000000000001,
-0.895000000000001,-0.890000000000001,-0.885000000000001,-0.880000000000001,
-0.875000000000001,-0.870000000000001,-0.865000000000001,-0.860000000000001,
-0.855000000000001,-0.850000000000001,-0.845000000000001,-0.840000000000001,
-0.835000000000001,-0.830000000000001,-0.825000000000001,-0.820000000000001,
-0.815000000000001,-0.810000000000001,-0.805000000000001,-0.800000000000001,
-0.795000000000001,-0.790000000000001,-0.785000000000001,-0.780000000000001,
-0.775000000000001,-0.770000000000001,-0.765000000000001,-0.760000000000001,
-0.755000000000001,-0.750000000000001,-0.745000000000001,-0.740000000000001,
-0.735000000000001,-0.730000000000001,-0.725000000000001,-0.720000000000001,
-0.715000000000001,-0.710000000000001,-0.705000000000001,-0.700000000000001,
-0.695000000000001,-0.690000000000001,-0.685,-0.68,-0.675,-0.67,-0.665,
-0.66,-0.655,-0.65,-0.645,-0.64,-0.635,-0.63,-0.625,-0.62,-0.615,-0.61,
-0.605,-0.6,-0.595,-0.59,-0.585,-0.58,-0.575,-0.57,-0.565,-0.56,-0.555,
-0.55,-0.545,-0.54,-0.535,-0.53,-0.525,-0.52,-0.515,-0.51,-0.505,-0.5,-0.495,
-0.49,-0.485,-0.48,-0.475,-0.47,-0.465,-0.46,-0.455,-0.45,-0.445,-0.44,
-0.435,-0.43,-0.425,-0.42,-0.415,-0.41,-0.405,-0.4,-0.395,-0.39,-0.385,
-0.38,-0.375,-0.37,-0.365,-0.36,-0.355,-0.35,-0.345,-0.34,-0.335,-0.33,
-0.325,-0.32,-0.315,-0.31,-0.305,-0.3,-0.295,-0.29,-0.285,-0.28,-0.275,
-0.27,-0.265,-0.26,-0.255,-0.25,-0.245,-0.24,-0.235,-0.23,-0.225,-0.22,
-0.215,-0.21,-0.205,-0.2,-0.195,-0.19,-0.185,-0.18,-0.175,-0.17,-0.165,
-0.16,-0.155,-0.15,-0.145,-0.14,-0.135,-0.13,-0.125,-0.12,-0.115,-0.11,
-0.105,-0.1,-0.095,-0.09,-0.085,-0.08,-0.075,-0.07,-0.065,-0.06,-0.055,
-0.05,-0.045,-0.04,-0.035,-0.03,-0.025,-0.02,-0.015,-0.01,-0.005,0.),(0.,
1.2),.UNSPECIFIED.)
GEOMETRIC_REPRESENTATION_ITEM()
RATIONAL_B_SPLINE_SURFACE(((1.,1.),(1.,1.),(1.,1.),(1.,1.),(1.,1.),(1.,
1.),(1.,1.),(1.,1.),(1.,1.),(1.,1.),(1.,1.),(1.,1.),(1.,1.),(1.,1.),(1.,
1.),(1.,1.),(1.,1.),(1.,1.),(1.,1.),(1.,1.),(1.,1.),(1.,1.),(1.,1.),(1.,
1.),(1.,1.),(1.,1.),(1.,1.),(1.,1.),(1.,1.),(1.,1.),(1.,1.),(1.,1.),(1.,
1.),(1.,1.),(1.,1.),(1.,1.),(1.,1.),(1.,1.),(1.,1.),(1.,1.),(1.,1.),(1.,
1.),(1.,1.),(1.,1.),(1.,1.),(1.,1.),(1.,1.),(1.,1.),(1.,1.),(1.,1.),(1.,
1.),(1.,1.),(1.,1.),(1.,1.),(1.,1.),(1.,1.),(1.,1.),(1.,1.),(1.,1.),(1.,
1.),(1.,1.),(1.,1.),(1.,1.),(1.,1.),(1.,1.),(1.,1.),(1.,1.),(1.,1.),(1.,
1.),(1.,1.),(1.,1.),(1.,1.),(1.,1.),(1.,1.),(1.,1.),(1.,1.),(1.,1.),(1.,
1.),(1.,1.),(1.,1.),(1.,1.),(1.,1.),(1.,1.),(1.,1.),(1.,1.),(1.,1.),(1.,
1.),(1.,1.),(1.,1.),(1.,1.),(1.,1.),(1.,1.),(1.,1.),(1.,1.),(1.,1.),(1.,
1.),(1.,1.),(1.,1.),(1.,1.),(1.,1.),(1.,1.),(1.,1.),(1.,1.),(1.,1.),(1.,
1.),(1.,1.),(1.,1.),(1.,1.),(1.,1.),(1.,1.),(1.,1.),(1.,1.),(1.,1.),(1.,
1.),(1.,1.),(1.,1.),(1.,1.),(1.,1.),(1.,1.),(1.,1.),(1.,1.),(1.,1.),(1.,
1.),(1.,1.),(1.,1.),(1.,1.),(1.,1.),(1.,1.),(1.,1.),(1.,1.),(1.,1.),(1.,
1.),(1.,1.),(1.,1.),(1.,1.),(1.,1.),(1.,1.),(1.,1.),(1.,1.),(1.,1.),(1.,
1.),(1.,1.),(1.,1.),(1.,1.),(1.,1.),(1.,1.),(1.,1.),(1.,1.),(1.,1.),(1.,
1.),(1.,1.),(1.,1.),(1.,1.),(1.,1.),(1.,1.),(1.,1.),(1.,1.),(1.,1.),(1.,
1.),(1.,1.),(1.,1.),(1.,1.),(1.,1.),(1.,1.),(1.,1.),(1.,1.),(1.,1.),(1.,
1.),(1.,1.),(1.,1.),(1.,1.),(1.,1.),(1.,1.),(1.,1.),(1.,1.),(1.,1.),(1.,
1.),(1.,1.),(1.,1.),(1.,1.),(1.,1.),(1.,1.),(1.,1.),(1.,1.),(1.,1.),(1.,
1.),(1.,1.),(1.,1.),(1.,1.),(1.,1.),(1.,1.),(1.,1.),(1.,1.),(1.,1.),(1.,
1.),(1.,1.),(1.,1.),(1.,1.),(1.,1.),(1.,1.),(1.,1.),(1.,1.),(1.,1.),(1.,
1.),(1.,1.)))
REPRESENTATION_ITEM('')
SURFACE()
);
#986=(
BOUNDED_SURFACE()
B_SPLINE_SURFACE(5,1,((#141824,#141825),(#141826,#141827),(#141828,#141829),
(#141830,#141831),(#141832,#141833),(#141834,#141835),(#141836,#141837),
(#141838,#141839),(#141840,#141841),(#141842,#141843),(#141844,#141845),
(#141846,#141847),(#141848,#141849),(#141850,#141851),(#141852,#141853),
(#141854,#141855),(#141856,#141857),(#141858,#141859),(#141860,#141861),
(#141862,#141863),(#141864,#141865),(#141866,#141867),(#141868,#141869),
(#141870,#141871),(#141872,#141873),(#141874,#141875),(#141876,#141877),
(#141878,#141879),(#141880,#141881),(#141882,#141883),(#141884,#141885),
(#141886,#141887),(#141888,#141889),(#141890,#141891),(#141892,#141893),
(#141894,#141895),(#141896,#141897),(#141898,#141899),(#141900,#141901),
(#141902,#141903),(#141904,#141905),(#141906,#141907),(#141908,#141909),
(#141910,#141911),(#141912,#141913),(#141914,#141915),(#141916,#141917),
(#141918,#141919),(#141920,#141921),(#141922,#141923),(#141924,#141925),
(#141926,#141927),(#141928,#141929),(#141930,#141931),(#141932,#141933),
(#141934,#141935),(#141936,#141937),(#141938,#141939),(#141940,#141941),
(#141942,#141943),(#141944,#141945),(#141946,#141947),(#141948,#141949),
(#141950,#141951),(#141952,#141953),(#141954,#141955),(#141956,#141957),
(#141958,#141959),(#141960,#141961),(#141962,#141963),(#141964,#141965),
(#141966,#141967),(#141968,#141969),(#141970,#141971),(#141972,#141973),
(#141974,#141975),(#141976,#141977),(#141978,#141979),(#141980,#141981),
(#141982,#141983),(#141984,#141985),(#141986,#141987),(#141988,#141989),
(#141990,#141991),(#141992,#141993),(#141994,#141995),(#141996,#141997),
(#141998,#141999),(#142000,#142001),(#142002,#142003),(#142004,#142005),
(#142006,#142007),(#142008,#142009),(#142010,#142011),(#142012,#142013),
(#142014,#142015),(#142016,#142017),(#142018,#142019),(#142020,#142021),
(#142022,#142023),(#142024,#142025),(#142026,#142027),(#142028,#142029),
(#142030,#142031),(#142032,#142033),(#142034,#142035),(#142036,#142037),
(#142038,#142039),(#142040,#142041),(#142042,#142043),(#142044,#142045),
(#142046,#142047),(#142048,#142049),(#142050,#142051),(#142052,#142053),
(#142054,#142055),(#142056,#142057),(#142058,#142059),(#142060,#142061),
(#142062,#142063),(#142064,#142065),(#142066,#142067),(#142068,#142069),
(#142070,#142071),(#142072,#142073),(#142074,#142075),(#142076,#142077),
(#142078,#142079),(#142080,#142081),(#142082,#142083),(#142084,#142085),
(#142086,#142087),(#142088,#142089),(#142090,#142091),(#142092,#142093),
(#142094,#142095),(#142096,#142097),(#142098,#142099),(#142100,#142101),
(#142102,#142103),(#142104,#142105),(#142106,#142107),(#142108,#142109),
(#142110,#142111),(#142112,#142113),(#142114,#142115),(#142116,#142117),
(#142118,#142119),(#142120,#142121),(#142122,#142123),(#142124,#142125),
(#142126,#142127),(#142128,#142129),(#142130,#142131),(#142132,#142133),
(#142134,#142135),(#142136,#142137),(#142138,#142139),(#142140,#142141),
(#142142,#142143),(#142144,#142145),(#142146,#142147),(#142148,#142149),
(#142150,#142151),(#142152,#142153),(#142154,#142155),(#142156,#142157),
(#142158,#142159),(#142160,#142161),(#142162,#142163),(#142164,#142165),
(#142166,#142167),(#142168,#142169),(#142170,#142171),(#142172,#142173),
(#142174,#142175),(#142176,#142177),(#142178,#142179),(#142180,#142181),
(#142182,#142183),(#142184,#142185),(#142186,#142187),(#142188,#142189),
(#142190,#142191),(#142192,#142193),(#142194,#142195),(#142196,#142197),
(#142198,#142199),(#142200,#142201),(#142202,#142203),(#142204,#142205),
(#142206,#142207),(#142208,#142209),(#142210,#142211),(#142212,#142213),
(#142214,#142215),(#142216,#142217),(#142218,#142219),(#142220,#142221),
(#142222,#142223),(#142224,#142225),(#142226,#142227),(#142228,#142229),
(#142230,#142231),(#142232,#142233)),.UNSPECIFIED.,.F.,.F.,.F.)
B_SPLINE_SURFACE_WITH_KNOTS((6,1,1,1,1,1,1,1,1,1,1,1,1,1,1,1,1,1,1,1,1,
1,1,1,1,1,1,1,1,1,1,1,1,1,1,1,1,1,1,1,1,1,1,1,1,1,1,1,1,1,1,1,1,1,1,1,1,
1,1,1,1,1,1,1,1,1,1,1,1,1,1,1,1,1,1,1,1,1,1,1,1,1,1,1,1,1,1,1,1,1,1,1,1,
1,1,1,1,1,1,1,1,1,1,1,1,1,1,1,1,1,1,1,1,1,1,1,1,1,1,1,1,1,1,1,1,1,1,1,1,
1,1,1,1,1,1,1,1,1,1,1,1,1,1,1,1,1,1,1,1,1,1,1,1,1,1,1,1,1,1,1,1,1,1,1,1,
1,1,1,1,1,1,1,1,1,1,1,1,1,1,1,1,1,1,1,1,1,1,1,1,1,1,1,1,1,1,1,1,1,1,1,6),
(2,2),(-1.,-0.995000000000001,-0.990000000000001,-0.985000000000001,-0.980000000000001,
-0.975000000000001,-0.970000000000001,-0.965000000000001,-0.960000000000001,
-0.955000000000001,-0.950000000000001,-0.945000000000001,-0.940000000000001,
-0.935000000000001,-0.930000000000001,-0.925000000000001,-0.920000000000001,
-0.915000000000001,-0.910000000000001,-0.905000000000001,-0.900000000000001,
-0.895000000000001,-0.890000000000001,-0.885000000000001,-0.880000000000001,
-0.875000000000001,-0.870000000000001,-0.865000000000001,-0.860000000000001,
-0.855000000000001,-0.850000000000001,-0.845000000000001,-0.840000000000001,
-0.835000000000001,-0.830000000000001,-0.825000000000001,-0.820000000000001,
-0.815000000000001,-0.810000000000001,-0.805000000000001,-0.800000000000001,
-0.795000000000001,-0.790000000000001,-0.785000000000001,-0.780000000000001,
-0.775000000000001,-0.770000000000001,-0.765000000000001,-0.760000000000001,
-0.755000000000001,-0.750000000000001,-0.745000000000001,-0.740000000000001,
-0.735000000000001,-0.730000000000001,-0.725000000000001,-0.720000000000001,
-0.715000000000001,-0.710000000000001,-0.705000000000001,-0.700000000000001,
-0.695000000000001,-0.690000000000001,-0.685,-0.68,-0.675,-0.67,-0.665,
-0.66,-0.655,-0.65,-0.645,-0.64,-0.635,-0.63,-0.625,-0.62,-0.615,-0.61,
-0.605,-0.6,-0.595,-0.59,-0.585,-0.58,-0.575,-0.57,-0.565,-0.56,-0.555,
-0.55,-0.545,-0.54,-0.535,-0.53,-0.525,-0.52,-0.515,-0.51,-0.505,-0.5,-0.495,
-0.49,-0.485,-0.48,-0.475,-0.47,-0.465,-0.46,-0.455,-0.45,-0.445,-0.44,
-0.435,-0.43,-0.425,-0.42,-0.415,-0.41,-0.405,-0.4,-0.395,-0.39,-0.385,
-0.38,-0.375,-0.37,-0.365,-0.36,-0.355,-0.35,-0.345,-0.34,-0.335,-0.33,
-0.325,-0.32,-0.315,-0.31,-0.305,-0.3,-0.295,-0.29,-0.285,-0.28,-0.275,
-0.27,-0.265,-0.26,-0.255,-0.25,-0.245,-0.24,-0.235,-0.23,-0.225,-0.22,
-0.215,-0.21,-0.205,-0.2,-0.195,-0.19,-0.185,-0.18,-0.175,-0.17,-0.165,
-0.16,-0.155,-0.15,-0.145,-0.14,-0.135,-0.13,-0.125,-0.12,-0.115,-0.11,
-0.105,-0.1,-0.095,-0.09,-0.085,-0.08,-0.075,-0.07,-0.065,-0.06,-0.055,
-0.05,-0.045,-0.04,-0.035,-0.03,-0.025,-0.02,-0.015,-0.01,-0.005,0.),(0.,
1.2),.UNSPECIFIED.)
GEOMETRIC_REPRESENTATION_ITEM()
RATIONAL_B_SPLINE_SURFACE(((1.,1.),(1.,1.),(1.,1.),(1.,1.),(1.,1.),(1.,
1.),(1.,1.),(1.,1.),(1.,1.),(1.,1.),(1.,1.),(1.,1.),(1.,1.),(1.,1.),(1.,
1.),(1.,1.),(1.,1.),(1.,1.),(1.,1.),(1.,1.),(1.,1.),(1.,1.),(1.,1.),(1.,
1.),(1.,1.),(1.,1.),(1.,1.),(1.,1.),(1.,1.),(1.,1.),(1.,1.),(1.,1.),(1.,
1.),(1.,1.),(1.,1.),(1.,1.),(1.,1.),(1.,1.),(1.,1.),(1.,1.),(1.,1.),(1.,
1.),(1.,1.),(1.,1.),(1.,1.),(1.,1.),(1.,1.),(1.,1.),(1.,1.),(1.,1.),(1.,
1.),(1.,1.),(1.,1.),(1.,1.),(1.,1.),(1.,1.),(1.,1.),(1.,1.),(1.,1.),(1.,
1.),(1.,1.),(1.,1.),(1.,1.),(1.,1.),(1.,1.),(1.,1.),(1.,1.),(1.,1.),(1.,
1.),(1.,1.),(1.,1.),(1.,1.),(1.,1.),(1.,1.),(1.,1.),(1.,1.),(1.,1.),(1.,
1.),(1.,1.),(1.,1.),(1.,1.),(1.,1.),(1.,1.),(1.,1.),(1.,1.),(1.,1.),(1.,
1.),(1.,1.),(1.,1.),(1.,1.),(1.,1.),(1.,1.),(1.,1.),(1.,1.),(1.,1.),(1.,
1.),(1.,1.),(1.,1.),(1.,1.),(1.,1.),(1.,1.),(1.,1.),(1.,1.),(1.,1.),(1.,
1.),(1.,1.),(1.,1.),(1.,1.),(1.,1.),(1.,1.),(1.,1.),(1.,1.),(1.,1.),(1.,
1.),(1.,1.),(1.,1.),(1.,1.),(1.,1.),(1.,1.),(1.,1.),(1.,1.),(1.,1.),(1.,
1.),(1.,1.),(1.,1.),(1.,1.),(1.,1.),(1.,1.),(1.,1.),(1.,1.),(1.,1.),(1.,
1.),(1.,1.),(1.,1.),(1.,1.),(1.,1.),(1.,1.),(1.,1.),(1.,1.),(1.,1.),(1.,
1.),(1.,1.),(1.,1.),(1.,1.),(1.,1.),(1.,1.),(1.,1.),(1.,1.),(1.,1.),(1.,
1.),(1.,1.),(1.,1.),(1.,1.),(1.,1.),(1.,1.),(1.,1.),(1.,1.),(1.,1.),(1.,
1.),(1.,1.),(1.,1.),(1.,1.),(1.,1.),(1.,1.),(1.,1.),(1.,1.),(1.,1.),(1.,
1.),(1.,1.),(1.,1.),(1.,1.),(1.,1.),(1.,1.),(1.,1.),(1.,1.),(1.,1.),(1.,
1.),(1.,1.),(1.,1.),(1.,1.),(1.,1.),(1.,1.),(1.,1.),(1.,1.),(1.,1.),(1.,
1.),(1.,1.),(1.,1.),(1.,1.),(1.,1.),(1.,1.),(1.,1.),(1.,1.),(1.,1.),(1.,
1.),(1.,1.),(1.,1.),(1.,1.),(1.,1.),(1.,1.),(1.,1.),(1.,1.),(1.,1.),(1.,
1.),(1.,1.)))
REPRESENTATION_ITEM('')
SURFACE()
);
#987=(
BOUNDED_SURFACE()
B_SPLINE_SURFACE(5,1,((#142625,#142626),(#142627,#142628),(#142629,#142630),
(#142631,#142632),(#142633,#142634),(#142635,#142636),(#142637,#142638),
(#142639,#142640),(#142641,#142642),(#142643,#142644),(#142645,#142646),
(#142647,#142648),(#142649,#142650),(#142651,#142652),(#142653,#142654),
(#142655,#142656),(#142657,#142658),(#142659,#142660),(#142661,#142662),
(#142663,#142664),(#142665,#142666),(#142667,#142668),(#142669,#142670),
(#142671,#142672),(#142673,#142674),(#142675,#142676),(#142677,#142678),
(#142679,#142680),(#142681,#142682),(#142683,#142684),(#142685,#142686),
(#142687,#142688),(#142689,#142690),(#142691,#142692),(#142693,#142694),
(#142695,#142696),(#142697,#142698),(#142699,#142700),(#142701,#142702),
(#142703,#142704),(#142705,#142706),(#142707,#142708),(#142709,#142710),
(#142711,#142712),(#142713,#142714),(#142715,#142716),(#142717,#142718),
(#142719,#142720),(#142721,#142722),(#142723,#142724),(#142725,#142726),
(#142727,#142728),(#142729,#142730),(#142731,#142732),(#142733,#142734),
(#142735,#142736),(#142737,#142738),(#142739,#142740),(#142741,#142742),
(#142743,#142744),(#142745,#142746),(#142747,#142748),(#142749,#142750),
(#142751,#142752),(#142753,#142754),(#142755,#142756),(#142757,#142758),
(#142759,#142760),(#142761,#142762),(#142763,#142764),(#142765,#142766),
(#142767,#142768),(#142769,#142770),(#142771,#142772),(#142773,#142774),
(#142775,#142776),(#142777,#142778),(#142779,#142780),(#142781,#142782),
(#142783,#142784),(#142785,#142786),(#142787,#142788),(#142789,#142790),
(#142791,#142792),(#142793,#142794),(#142795,#142796),(#142797,#142798),
(#142799,#142800),(#142801,#142802),(#142803,#142804),(#142805,#142806),
(#142807,#142808),(#142809,#142810),(#142811,#142812),(#142813,#142814),
(#142815,#142816),(#142817,#142818),(#142819,#142820),(#142821,#142822),
(#142823,#142824),(#142825,#142826),(#142827,#142828),(#142829,#142830),
(#142831,#142832),(#142833,#142834),(#142835,#142836),(#142837,#142838),
(#142839,#142840),(#142841,#142842),(#142843,#142844),(#142845,#142846),
(#142847,#142848),(#142849,#142850),(#142851,#142852),(#142853,#142854),
(#142855,#142856),(#142857,#142858),(#142859,#142860),(#142861,#142862),
(#142863,#142864),(#142865,#142866),(#142867,#142868),(#142869,#142870),
(#142871,#142872),(#142873,#142874),(#142875,#142876),(#142877,#142878),
(#142879,#142880),(#142881,#142882),(#142883,#142884),(#142885,#142886),
(#142887,#142888),(#142889,#142890),(#142891,#142892),(#142893,#142894),
(#142895,#142896),(#142897,#142898),(#142899,#142900),(#142901,#142902),
(#142903,#142904),(#142905,#142906),(#142907,#142908),(#142909,#142910),
(#142911,#142912),(#142913,#142914),(#142915,#142916),(#142917,#142918),
(#142919,#142920),(#142921,#142922),(#142923,#142924),(#142925,#142926),
(#142927,#142928),(#142929,#142930),(#142931,#142932),(#142933,#142934),
(#142935,#142936),(#142937,#142938),(#142939,#142940),(#142941,#142942),
(#142943,#142944),(#142945,#142946),(#142947,#142948),(#142949,#142950),
(#142951,#142952),(#142953,#142954),(#142955,#142956),(#142957,#142958),
(#142959,#142960),(#142961,#142962),(#142963,#142964),(#142965,#142966),
(#142967,#142968),(#142969,#142970),(#142971,#142972),(#142973,#142974),
(#142975,#142976),(#142977,#142978),(#142979,#142980),(#142981,#142982),
(#142983,#142984),(#142985,#142986),(#142987,#142988),(#142989,#142990),
(#142991,#142992),(#142993,#142994),(#142995,#142996),(#142997,#142998),
(#142999,#143000),(#143001,#143002),(#143003,#143004),(#143005,#143006),
(#143007,#143008),(#143009,#143010),(#143011,#143012),(#143013,#143014),
(#143015,#143016),(#143017,#143018),(#143019,#143020),(#143021,#143022),
(#143023,#143024),(#143025,#143026),(#143027,#143028),(#143029,#143030),
(#143031,#143032),(#143033,#143034)),.UNSPECIFIED.,.F.,.F.,.F.)
B_SPLINE_SURFACE_WITH_KNOTS((6,1,1,1,1,1,1,1,1,1,1,1,1,1,1,1,1,1,1,1,1,
1,1,1,1,1,1,1,1,1,1,1,1,1,1,1,1,1,1,1,1,1,1,1,1,1,1,1,1,1,1,1,1,1,1,1,1,
1,1,1,1,1,1,1,1,1,1,1,1,1,1,1,1,1,1,1,1,1,1,1,1,1,1,1,1,1,1,1,1,1,1,1,1,
1,1,1,1,1,1,1,1,1,1,1,1,1,1,1,1,1,1,1,1,1,1,1,1,1,1,1,1,1,1,1,1,1,1,1,1,
1,1,1,1,1,1,1,1,1,1,1,1,1,1,1,1,1,1,1,1,1,1,1,1,1,1,1,1,1,1,1,1,1,1,1,1,
1,1,1,1,1,1,1,1,1,1,1,1,1,1,1,1,1,1,1,1,1,1,1,1,1,1,1,1,1,1,1,1,1,1,1,6),
(2,2),(-1.,-0.995000000000001,-0.990000000000001,-0.985000000000001,-0.980000000000001,
-0.975000000000001,-0.970000000000001,-0.965000000000001,-0.960000000000001,
-0.955000000000001,-0.950000000000001,-0.945000000000001,-0.940000000000001,
-0.935000000000001,-0.930000000000001,-0.925000000000001,-0.920000000000001,
-0.915000000000001,-0.910000000000001,-0.905000000000001,-0.900000000000001,
-0.895000000000001,-0.890000000000001,-0.885000000000001,-0.880000000000001,
-0.875000000000001,-0.870000000000001,-0.865000000000001,-0.860000000000001,
-0.855000000000001,-0.850000000000001,-0.845000000000001,-0.840000000000001,
-0.835000000000001,-0.830000000000001,-0.825000000000001,-0.820000000000001,
-0.815000000000001,-0.810000000000001,-0.805000000000001,-0.800000000000001,
-0.795000000000001,-0.790000000000001,-0.785000000000001,-0.780000000000001,
-0.775000000000001,-0.770000000000001,-0.765000000000001,-0.760000000000001,
-0.755000000000001,-0.750000000000001,-0.745000000000001,-0.740000000000001,
-0.735000000000001,-0.730000000000001,-0.725000000000001,-0.720000000000001,
-0.715000000000001,-0.710000000000001,-0.705000000000001,-0.700000000000001,
-0.695000000000001,-0.690000000000001,-0.685,-0.68,-0.675,-0.67,-0.665,
-0.66,-0.655,-0.65,-0.645,-0.64,-0.635,-0.63,-0.625,-0.62,-0.615,-0.61,
-0.605,-0.6,-0.595,-0.59,-0.585,-0.58,-0.575,-0.57,-0.565,-0.56,-0.555,
-0.55,-0.545,-0.54,-0.535,-0.53,-0.525,-0.52,-0.515,-0.51,-0.505,-0.5,-0.495,
-0.49,-0.485,-0.48,-0.475,-0.47,-0.465,-0.46,-0.455,-0.45,-0.445,-0.44,
-0.435,-0.43,-0.425,-0.42,-0.415,-0.41,-0.405,-0.4,-0.395,-0.39,-0.385,
-0.38,-0.375,-0.37,-0.365,-0.36,-0.355,-0.35,-0.345,-0.34,-0.335,-0.33,
-0.325,-0.32,-0.315,-0.31,-0.305,-0.3,-0.295,-0.29,-0.285,-0.28,-0.275,
-0.27,-0.265,-0.26,-0.255,-0.25,-0.245,-0.24,-0.235,-0.23,-0.225,-0.22,
-0.215,-0.21,-0.205,-0.2,-0.195,-0.19,-0.185,-0.18,-0.175,-0.17,-0.165,
-0.16,-0.155,-0.15,-0.145,-0.14,-0.135,-0.13,-0.125,-0.12,-0.115,-0.11,
-0.105,-0.1,-0.095,-0.09,-0.085,-0.08,-0.075,-0.07,-0.065,-0.06,-0.055,
-0.05,-0.045,-0.04,-0.035,-0.03,-0.025,-0.02,-0.015,-0.01,-0.005,0.),(0.,
1.2),.UNSPECIFIED.)
GEOMETRIC_REPRESENTATION_ITEM()
RATIONAL_B_SPLINE_SURFACE(((1.,1.),(1.,1.),(1.,1.),(1.,1.),(1.,1.),(1.,
1.),(1.,1.),(1.,1.),(1.,1.),(1.,1.),(1.,1.),(1.,1.),(1.,1.),(1.,1.),(1.,
1.),(1.,1.),(1.,1.),(1.,1.),(1.,1.),(1.,1.),(1.,1.),(1.,1.),(1.,1.),(1.,
1.),(1.,1.),(1.,1.),(1.,1.),(1.,1.),(1.,1.),(1.,1.),(1.,1.),(1.,1.),(1.,
1.),(1.,1.),(1.,1.),(1.,1.),(1.,1.),(1.,1.),(1.,1.),(1.,1.),(1.,1.),(1.,
1.),(1.,1.),(1.,1.),(1.,1.),(1.,1.),(1.,1.),(1.,1.),(1.,1.),(1.,1.),(1.,
1.),(1.,1.),(1.,1.),(1.,1.),(1.,1.),(1.,1.),(1.,1.),(1.,1.),(1.,1.),(1.,
1.),(1.,1.),(1.,1.),(1.,1.),(1.,1.),(1.,1.),(1.,1.),(1.,1.),(1.,1.),(1.,
1.),(1.,1.),(1.,1.),(1.,1.),(1.,1.),(1.,1.),(1.,1.),(1.,1.),(1.,1.),(1.,
1.),(1.,1.),(1.,1.),(1.,1.),(1.,1.),(1.,1.),(1.,1.),(1.,1.),(1.,1.),(1.,
1.),(1.,1.),(1.,1.),(1.,1.),(1.,1.),(1.,1.),(1.,1.),(1.,1.),(1.,1.),(1.,
1.),(1.,1.),(1.,1.),(1.,1.),(1.,1.),(1.,1.),(1.,1.),(1.,1.),(1.,1.),(1.,
1.),(1.,1.),(1.,1.),(1.,1.),(1.,1.),(1.,1.),(1.,1.),(1.,1.),(1.,1.),(1.,
1.),(1.,1.),(1.,1.),(1.,1.),(1.,1.),(1.,1.),(1.,1.),(1.,1.),(1.,1.),(1.,
1.),(1.,1.),(1.,1.),(1.,1.),(1.,1.),(1.,1.),(1.,1.),(1.,1.),(1.,1.),(1.,
1.),(1.,1.),(1.,1.),(1.,1.),(1.,1.),(1.,1.),(1.,1.),(1.,1.),(1.,1.),(1.,
1.),(1.,1.),(1.,1.),(1.,1.),(1.,1.),(1.,1.),(1.,1.),(1.,1.),(1.,1.),(1.,
1.),(1.,1.),(1.,1.),(1.,1.),(1.,1.),(1.,1.),(1.,1.),(1.,1.),(1.,1.),(1.,
1.),(1.,1.),(1.,1.),(1.,1.),(1.,1.),(1.,1.),(1.,1.),(1.,1.),(1.,1.),(1.,
1.),(1.,1.),(1.,1.),(1.,1.),(1.,1.),(1.,1.),(1.,1.),(1.,1.),(1.,1.),(1.,
1.),(1.,1.),(1.,1.),(1.,1.),(1.,1.),(1.,1.),(1.,1.),(1.,1.),(1.,1.),(1.,
1.),(1.,1.),(1.,1.),(1.,1.),(1.,1.),(1.,1.),(1.,1.),(1.,1.),(1.,1.),(1.,
1.),(1.,1.),(1.,1.),(1.,1.),(1.,1.),(1.,1.),(1.,1.),(1.,1.),(1.,1.),(1.,
1.),(1.,1.)))
REPRESENTATION_ITEM('')
SURFACE()
);
#988=(
BOUNDED_SURFACE()
B_SPLINE_SURFACE(5,1,((#143426,#143427),(#143428,#143429),(#143430,#143431),
(#143432,#143433),(#143434,#143435),(#143436,#143437),(#143438,#143439),
(#143440,#143441),(#143442,#143443),(#143444,#143445),(#143446,#143447),
(#143448,#143449),(#143450,#143451),(#143452,#143453),(#143454,#143455),
(#143456,#143457),(#143458,#143459),(#143460,#143461),(#143462,#143463),
(#143464,#143465),(#143466,#143467),(#143468,#143469),(#143470,#143471),
(#143472,#143473),(#143474,#143475),(#143476,#143477),(#143478,#143479),
(#143480,#143481),(#143482,#143483),(#143484,#143485),(#143486,#143487),
(#143488,#143489),(#143490,#143491),(#143492,#143493),(#143494,#143495),
(#143496,#143497),(#143498,#143499),(#143500,#143501),(#143502,#143503),
(#143504,#143505),(#143506,#143507),(#143508,#143509),(#143510,#143511),
(#143512,#143513),(#143514,#143515),(#143516,#143517),(#143518,#143519),
(#143520,#143521),(#143522,#143523),(#143524,#143525),(#143526,#143527),
(#143528,#143529),(#143530,#143531),(#143532,#143533),(#143534,#143535),
(#143536,#143537),(#143538,#143539),(#143540,#143541),(#143542,#143543),
(#143544,#143545),(#143546,#143547),(#143548,#143549),(#143550,#143551),
(#143552,#143553),(#143554,#143555),(#143556,#143557),(#143558,#143559),
(#143560,#143561),(#143562,#143563),(#143564,#143565),(#143566,#143567),
(#143568,#143569),(#143570,#143571),(#143572,#143573),(#143574,#143575),
(#143576,#143577),(#143578,#143579),(#143580,#143581),(#143582,#143583),
(#143584,#143585),(#143586,#143587),(#143588,#143589),(#143590,#143591),
(#143592,#143593),(#143594,#143595),(#143596,#143597),(#143598,#143599),
(#143600,#143601),(#143602,#143603),(#143604,#143605),(#143606,#143607),
(#143608,#143609),(#143610,#143611),(#143612,#143613),(#143614,#143615),
(#143616,#143617),(#143618,#143619),(#143620,#143621),(#143622,#143623),
(#143624,#143625),(#143626,#143627),(#143628,#143629),(#143630,#143631),
(#143632,#143633),(#143634,#143635),(#143636,#143637),(#143638,#143639),
(#143640,#143641),(#143642,#143643),(#143644,#143645),(#143646,#143647),
(#143648,#143649),(#143650,#143651),(#143652,#143653),(#143654,#143655),
(#143656,#143657),(#143658,#143659),(#143660,#143661),(#143662,#143663),
(#143664,#143665),(#143666,#143667),(#143668,#143669),(#143670,#143671),
(#143672,#143673),(#143674,#143675),(#143676,#143677),(#143678,#143679),
(#143680,#143681),(#143682,#143683),(#143684,#143685),(#143686,#143687),
(#143688,#143689),(#143690,#143691),(#143692,#143693),(#143694,#143695),
(#143696,#143697),(#143698,#143699),(#143700,#143701),(#143702,#143703),
(#143704,#143705),(#143706,#143707),(#143708,#143709),(#143710,#143711),
(#143712,#143713),(#143714,#143715),(#143716,#143717),(#143718,#143719),
(#143720,#143721),(#143722,#143723),(#143724,#143725),(#143726,#143727),
(#143728,#143729),(#143730,#143731),(#143732,#143733),(#143734,#143735),
(#143736,#143737),(#143738,#143739),(#143740,#143741),(#143742,#143743),
(#143744,#143745),(#143746,#143747),(#143748,#143749),(#143750,#143751),
(#143752,#143753),(#143754,#143755),(#143756,#143757),(#143758,#143759),
(#143760,#143761),(#143762,#143763),(#143764,#143765),(#143766,#143767),
(#143768,#143769),(#143770,#143771),(#143772,#143773),(#143774,#143775),
(#143776,#143777),(#143778,#143779),(#143780,#143781),(#143782,#143783),
(#143784,#143785),(#143786,#143787),(#143788,#143789),(#143790,#143791),
(#143792,#143793),(#143794,#143795),(#143796,#143797),(#143798,#143799),
(#143800,#143801),(#143802,#143803),(#143804,#143805),(#143806,#143807),
(#143808,#143809),(#143810,#143811),(#143812,#143813),(#143814,#143815),
(#143816,#143817),(#143818,#143819),(#143820,#143821),(#143822,#143823),
(#143824,#143825),(#143826,#143827),(#143828,#143829),(#143830,#143831),
(#143832,#143833),(#143834,#143835)),.UNSPECIFIED.,.F.,.F.,.F.)
B_SPLINE_SURFACE_WITH_KNOTS((6,1,1,1,1,1,1,1,1,1,1,1,1,1,1,1,1,1,1,1,1,
1,1,1,1,1,1,1,1,1,1,1,1,1,1,1,1,1,1,1,1,1,1,1,1,1,1,1,1,1,1,1,1,1,1,1,1,
1,1,1,1,1,1,1,1,1,1,1,1,1,1,1,1,1,1,1,1,1,1,1,1,1,1,1,1,1,1,1,1,1,1,1,1,
1,1,1,1,1,1,1,1,1,1,1,1,1,1,1,1,1,1,1,1,1,1,1,1,1,1,1,1,1,1,1,1,1,1,1,1,
1,1,1,1,1,1,1,1,1,1,1,1,1,1,1,1,1,1,1,1,1,1,1,1,1,1,1,1,1,1,1,1,1,1,1,1,
1,1,1,1,1,1,1,1,1,1,1,1,1,1,1,1,1,1,1,1,1,1,1,1,1,1,1,1,1,1,1,1,1,1,1,6),
(2,2),(-1.,-0.995000000000001,-0.990000000000001,-0.985000000000001,-0.980000000000001,
-0.975000000000001,-0.970000000000001,-0.965000000000001,-0.960000000000001,
-0.955000000000001,-0.950000000000001,-0.945000000000001,-0.940000000000001,
-0.935000000000001,-0.930000000000001,-0.925000000000001,-0.920000000000001,
-0.915000000000001,-0.910000000000001,-0.905000000000001,-0.900000000000001,
-0.895000000000001,-0.890000000000001,-0.885000000000001,-0.880000000000001,
-0.875000000000001,-0.870000000000001,-0.865000000000001,-0.860000000000001,
-0.855000000000001,-0.850000000000001,-0.845000000000001,-0.840000000000001,
-0.835000000000001,-0.830000000000001,-0.825000000000001,-0.820000000000001,
-0.815000000000001,-0.810000000000001,-0.805000000000001,-0.800000000000001,
-0.795000000000001,-0.790000000000001,-0.785000000000001,-0.780000000000001,
-0.775000000000001,-0.770000000000001,-0.765000000000001,-0.760000000000001,
-0.755000000000001,-0.750000000000001,-0.745000000000001,-0.740000000000001,
-0.735000000000001,-0.730000000000001,-0.725000000000001,-0.720000000000001,
-0.715000000000001,-0.710000000000001,-0.705000000000001,-0.700000000000001,
-0.695000000000001,-0.690000000000001,-0.685,-0.68,-0.675,-0.67,-0.665,
-0.66,-0.655,-0.65,-0.645,-0.64,-0.635,-0.63,-0.625,-0.62,-0.615,-0.61,
-0.605,-0.6,-0.595,-0.59,-0.585,-0.58,-0.575,-0.57,-0.565,-0.56,-0.555,
-0.55,-0.545,-0.54,-0.535,-0.53,-0.525,-0.52,-0.515,-0.51,-0.505,-0.5,-0.495,
-0.49,-0.485,-0.48,-0.475,-0.47,-0.465,-0.46,-0.455,-0.45,-0.445,-0.44,
-0.435,-0.43,-0.425,-0.42,-0.415,-0.41,-0.405,-0.4,-0.395,-0.39,-0.385,
-0.38,-0.375,-0.37,-0.365,-0.36,-0.355,-0.35,-0.345,-0.34,-0.335,-0.33,
-0.325,-0.32,-0.315,-0.31,-0.305,-0.3,-0.295,-0.29,-0.285,-0.28,-0.275,
-0.27,-0.265,-0.26,-0.255,-0.25,-0.245,-0.24,-0.235,-0.23,-0.225,-0.22,
-0.215,-0.21,-0.205,-0.2,-0.195,-0.19,-0.185,-0.18,-0.175,-0.17,-0.165,
-0.16,-0.155,-0.15,-0.145,-0.14,-0.135,-0.13,-0.125,-0.12,-0.115,-0.11,
-0.105,-0.1,-0.095,-0.09,-0.085,-0.08,-0.075,-0.07,-0.065,-0.06,-0.055,
-0.05,-0.045,-0.04,-0.035,-0.03,-0.025,-0.02,-0.015,-0.01,-0.005,0.),(0.,
1.2),.UNSPECIFIED.)
GEOMETRIC_REPRESENTATION_ITEM()
RATIONAL_B_SPLINE_SURFACE(((1.,1.),(1.,1.),(1.,1.),(1.,1.),(1.,1.),(1.,
1.),(1.,1.),(1.,1.),(1.,1.),(1.,1.),(1.,1.),(1.,1.),(1.,1.),(1.,1.),(1.,
1.),(1.,1.),(1.,1.),(1.,1.),(1.,1.),(1.,1.),(1.,1.),(1.,1.),(1.,1.),(1.,
1.),(1.,1.),(1.,1.),(1.,1.),(1.,1.),(1.,1.),(1.,1.),(1.,1.),(1.,1.),(1.,
1.),(1.,1.),(1.,1.),(1.,1.),(1.,1.),(1.,1.),(1.,1.),(1.,1.),(1.,1.),(1.,
1.),(1.,1.),(1.,1.),(1.,1.),(1.,1.),(1.,1.),(1.,1.),(1.,1.),(1.,1.),(1.,
1.),(1.,1.),(1.,1.),(1.,1.),(1.,1.),(1.,1.),(1.,1.),(1.,1.),(1.,1.),(1.,
1.),(1.,1.),(1.,1.),(1.,1.),(1.,1.),(1.,1.),(1.,1.),(1.,1.),(1.,1.),(1.,
1.),(1.,1.),(1.,1.),(1.,1.),(1.,1.),(1.,1.),(1.,1.),(1.,1.),(1.,1.),(1.,
1.),(1.,1.),(1.,1.),(1.,1.),(1.,1.),(1.,1.),(1.,1.),(1.,1.),(1.,1.),(1.,
1.),(1.,1.),(1.,1.),(1.,1.),(1.,1.),(1.,1.),(1.,1.),(1.,1.),(1.,1.),(1.,
1.),(1.,1.),(1.,1.),(1.,1.),(1.,1.),(1.,1.),(1.,1.),(1.,1.),(1.,1.),(1.,
1.),(1.,1.),(1.,1.),(1.,1.),(1.,1.),(1.,1.),(1.,1.),(1.,1.),(1.,1.),(1.,
1.),(1.,1.),(1.,1.),(1.,1.),(1.,1.),(1.,1.),(1.,1.),(1.,1.),(1.,1.),(1.,
1.),(1.,1.),(1.,1.),(1.,1.),(1.,1.),(1.,1.),(1.,1.),(1.,1.),(1.,1.),(1.,
1.),(1.,1.),(1.,1.),(1.,1.),(1.,1.),(1.,1.),(1.,1.),(1.,1.),(1.,1.),(1.,
1.),(1.,1.),(1.,1.),(1.,1.),(1.,1.),(1.,1.),(1.,1.),(1.,1.),(1.,1.),(1.,
1.),(1.,1.),(1.,1.),(1.,1.),(1.,1.),(1.,1.),(1.,1.),(1.,1.),(1.,1.),(1.,
1.),(1.,1.),(1.,1.),(1.,1.),(1.,1.),(1.,1.),(1.,1.),(1.,1.),(1.,1.),(1.,
1.),(1.,1.),(1.,1.),(1.,1.),(1.,1.),(1.,1.),(1.,1.),(1.,1.),(1.,1.),(1.,
1.),(1.,1.),(1.,1.),(1.,1.),(1.,1.),(1.,1.),(1.,1.),(1.,1.),(1.,1.),(1.,
1.),(1.,1.),(1.,1.),(1.,1.),(1.,1.),(1.,1.),(1.,1.),(1.,1.),(1.,1.),(1.,
1.),(1.,1.),(1.,1.),(1.,1.),(1.,1.),(1.,1.),(1.,1.),(1.,1.),(1.,1.),(1.,
1.),(1.,1.)))
REPRESENTATION_ITEM('')
SURFACE()
);
#989=(
BOUNDED_SURFACE()
B_SPLINE_SURFACE(5,1,((#144227,#144228),(#144229,#144230),(#144231,#144232),
(#144233,#144234),(#144235,#144236),(#144237,#144238),(#144239,#144240),
(#144241,#144242),(#144243,#144244),(#144245,#144246),(#144247,#144248),
(#144249,#144250),(#144251,#144252),(#144253,#144254),(#144255,#144256),
(#144257,#144258),(#144259,#144260),(#144261,#144262),(#144263,#144264),
(#144265,#144266),(#144267,#144268),(#144269,#144270),(#144271,#144272),
(#144273,#144274),(#144275,#144276),(#144277,#144278),(#144279,#144280),
(#144281,#144282),(#144283,#144284),(#144285,#144286),(#144287,#144288),
(#144289,#144290),(#144291,#144292),(#144293,#144294),(#144295,#144296),
(#144297,#144298),(#144299,#144300),(#144301,#144302),(#144303,#144304),
(#144305,#144306),(#144307,#144308),(#144309,#144310),(#144311,#144312),
(#144313,#144314),(#144315,#144316),(#144317,#144318),(#144319,#144320),
(#144321,#144322),(#144323,#144324),(#144325,#144326),(#144327,#144328),
(#144329,#144330),(#144331,#144332),(#144333,#144334),(#144335,#144336),
(#144337,#144338),(#144339,#144340),(#144341,#144342),(#144343,#144344),
(#144345,#144346),(#144347,#144348),(#144349,#144350),(#144351,#144352),
(#144353,#144354),(#144355,#144356),(#144357,#144358),(#144359,#144360),
(#144361,#144362),(#144363,#144364),(#144365,#144366),(#144367,#144368),
(#144369,#144370),(#144371,#144372),(#144373,#144374),(#144375,#144376),
(#144377,#144378),(#144379,#144380),(#144381,#144382),(#144383,#144384),
(#144385,#144386),(#144387,#144388),(#144389,#144390),(#144391,#144392),
(#144393,#144394),(#144395,#144396),(#144397,#144398),(#144399,#144400),
(#144401,#144402),(#144403,#144404),(#144405,#144406),(#144407,#144408),
(#144409,#144410),(#144411,#144412),(#144413,#144414),(#144415,#144416),
(#144417,#144418),(#144419,#144420),(#144421,#144422),(#144423,#144424),
(#144425,#144426),(#144427,#144428),(#144429,#144430),(#144431,#144432),
(#144433,#144434),(#144435,#144436),(#144437,#144438),(#144439,#144440),
(#144441,#144442),(#144443,#144444),(#144445,#144446),(#144447,#144448),
(#144449,#144450),(#144451,#144452),(#144453,#144454),(#144455,#144456),
(#144457,#144458),(#144459,#144460),(#144461,#144462),(#144463,#144464),
(#144465,#144466),(#144467,#144468),(#144469,#144470),(#144471,#144472),
(#144473,#144474),(#144475,#144476),(#144477,#144478),(#144479,#144480),
(#144481,#144482),(#144483,#144484),(#144485,#144486),(#144487,#144488),
(#144489,#144490),(#144491,#144492),(#144493,#144494),(#144495,#144496),
(#144497,#144498),(#144499,#144500),(#144501,#144502),(#144503,#144504),
(#144505,#144506),(#144507,#144508),(#144509,#144510),(#144511,#144512),
(#144513,#144514),(#144515,#144516),(#144517,#144518),(#144519,#144520),
(#144521,#144522),(#144523,#144524),(#144525,#144526),(#144527,#144528),
(#144529,#144530),(#144531,#144532),(#144533,#144534),(#144535,#144536),
(#144537,#144538),(#144539,#144540),(#144541,#144542),(#144543,#144544),
(#144545,#144546),(#144547,#144548),(#144549,#144550),(#144551,#144552),
(#144553,#144554),(#144555,#144556),(#144557,#144558),(#144559,#144560),
(#144561,#144562),(#144563,#144564),(#144565,#144566),(#144567,#144568),
(#144569,#144570),(#144571,#144572),(#144573,#144574),(#144575,#144576),
(#144577,#144578),(#144579,#144580),(#144581,#144582),(#144583,#144584),
(#144585,#144586),(#144587,#144588),(#144589,#144590),(#144591,#144592),
(#144593,#144594),(#144595,#144596),(#144597,#144598),(#144599,#144600),
(#144601,#144602),(#144603,#144604),(#144605,#144606),(#144607,#144608),
(#144609,#144610),(#144611,#144612),(#144613,#144614),(#144615,#144616),
(#144617,#144618),(#144619,#144620),(#144621,#144622),(#144623,#144624),
(#144625,#144626),(#144627,#144628),(#144629,#144630),(#144631,#144632),
(#144633,#144634),(#144635,#144636)),.UNSPECIFIED.,.F.,.F.,.F.)
B_SPLINE_SURFACE_WITH_KNOTS((6,1,1,1,1,1,1,1,1,1,1,1,1,1,1,1,1,1,1,1,1,
1,1,1,1,1,1,1,1,1,1,1,1,1,1,1,1,1,1,1,1,1,1,1,1,1,1,1,1,1,1,1,1,1,1,1,1,
1,1,1,1,1,1,1,1,1,1,1,1,1,1,1,1,1,1,1,1,1,1,1,1,1,1,1,1,1,1,1,1,1,1,1,1,
1,1,1,1,1,1,1,1,1,1,1,1,1,1,1,1,1,1,1,1,1,1,1,1,1,1,1,1,1,1,1,1,1,1,1,1,
1,1,1,1,1,1,1,1,1,1,1,1,1,1,1,1,1,1,1,1,1,1,1,1,1,1,1,1,1,1,1,1,1,1,1,1,
1,1,1,1,1,1,1,1,1,1,1,1,1,1,1,1,1,1,1,1,1,1,1,1,1,1,1,1,1,1,1,1,1,1,1,6),
(2,2),(-1.,-0.995000000000001,-0.990000000000001,-0.985000000000001,-0.980000000000001,
-0.975000000000001,-0.970000000000001,-0.965000000000001,-0.960000000000001,
-0.955000000000001,-0.950000000000001,-0.945000000000001,-0.940000000000001,
-0.935000000000001,-0.930000000000001,-0.925000000000001,-0.920000000000001,
-0.915000000000001,-0.910000000000001,-0.905000000000001,-0.900000000000001,
-0.895000000000001,-0.890000000000001,-0.885000000000001,-0.880000000000001,
-0.875000000000001,-0.870000000000001,-0.865000000000001,-0.860000000000001,
-0.855000000000001,-0.850000000000001,-0.845000000000001,-0.840000000000001,
-0.835000000000001,-0.830000000000001,-0.825000000000001,-0.820000000000001,
-0.815000000000001,-0.810000000000001,-0.805000000000001,-0.800000000000001,
-0.795000000000001,-0.790000000000001,-0.785000000000001,-0.780000000000001,
-0.775000000000001,-0.770000000000001,-0.765000000000001,-0.760000000000001,
-0.755000000000001,-0.750000000000001,-0.745000000000001,-0.740000000000001,
-0.735000000000001,-0.730000000000001,-0.725000000000001,-0.720000000000001,
-0.715000000000001,-0.710000000000001,-0.705000000000001,-0.700000000000001,
-0.695000000000001,-0.690000000000001,-0.685,-0.68,-0.675,-0.67,-0.665,
-0.66,-0.655,-0.65,-0.645,-0.64,-0.635,-0.63,-0.625,-0.62,-0.615,-0.61,
-0.605,-0.6,-0.595,-0.59,-0.585,-0.58,-0.575,-0.57,-0.565,-0.56,-0.555,
-0.55,-0.545,-0.54,-0.535,-0.53,-0.525,-0.52,-0.515,-0.51,-0.505,-0.5,-0.495,
-0.49,-0.485,-0.48,-0.475,-0.47,-0.465,-0.46,-0.455,-0.45,-0.445,-0.44,
-0.435,-0.43,-0.425,-0.42,-0.415,-0.41,-0.405,-0.4,-0.395,-0.39,-0.385,
-0.38,-0.375,-0.37,-0.365,-0.36,-0.355,-0.35,-0.345,-0.34,-0.335,-0.33,
-0.325,-0.32,-0.315,-0.31,-0.305,-0.3,-0.295,-0.29,-0.285,-0.28,-0.275,
-0.27,-0.265,-0.26,-0.255,-0.25,-0.245,-0.24,-0.235,-0.23,-0.225,-0.22,
-0.215,-0.21,-0.205,-0.2,-0.195,-0.19,-0.185,-0.18,-0.175,-0.17,-0.165,
-0.16,-0.155,-0.15,-0.145,-0.14,-0.135,-0.13,-0.125,-0.12,-0.115,-0.11,
-0.105,-0.1,-0.095,-0.09,-0.085,-0.08,-0.075,-0.07,-0.065,-0.06,-0.055,
-0.05,-0.045,-0.04,-0.035,-0.03,-0.025,-0.02,-0.015,-0.01,-0.005,0.),(0.,
1.2),.UNSPECIFIED.)
GEOMETRIC_REPRESENTATION_ITEM()
RATIONAL_B_SPLINE_SURFACE(((1.,1.),(1.,1.),(1.,1.),(1.,1.),(1.,1.),(1.,
1.),(1.,1.),(1.,1.),(1.,1.),(1.,1.),(1.,1.),(1.,1.),(1.,1.),(1.,1.),(1.,
1.),(1.,1.),(1.,1.),(1.,1.),(1.,1.),(1.,1.),(1.,1.),(1.,1.),(1.,1.),(1.,
1.),(1.,1.),(1.,1.),(1.,1.),(1.,1.),(1.,1.),(1.,1.),(1.,1.),(1.,1.),(1.,
1.),(1.,1.),(1.,1.),(1.,1.),(1.,1.),(1.,1.),(1.,1.),(1.,1.),(1.,1.),(1.,
1.),(1.,1.),(1.,1.),(1.,1.),(1.,1.),(1.,1.),(1.,1.),(1.,1.),(1.,1.),(1.,
1.),(1.,1.),(1.,1.),(1.,1.),(1.,1.),(1.,1.),(1.,1.),(1.,1.),(1.,1.),(1.,
1.),(1.,1.),(1.,1.),(1.,1.),(1.,1.),(1.,1.),(1.,1.),(1.,1.),(1.,1.),(1.,
1.),(1.,1.),(1.,1.),(1.,1.),(1.,1.),(1.,1.),(1.,1.),(1.,1.),(1.,1.),(1.,
1.),(1.,1.),(1.,1.),(1.,1.),(1.,1.),(1.,1.),(1.,1.),(1.,1.),(1.,1.),(1.,
1.),(1.,1.),(1.,1.),(1.,1.),(1.,1.),(1.,1.),(1.,1.),(1.,1.),(1.,1.),(1.,
1.),(1.,1.),(1.,1.),(1.,1.),(1.,1.),(1.,1.),(1.,1.),(1.,1.),(1.,1.),(1.,
1.),(1.,1.),(1.,1.),(1.,1.),(1.,1.),(1.,1.),(1.,1.),(1.,1.),(1.,1.),(1.,
1.),(1.,1.),(1.,1.),(1.,1.),(1.,1.),(1.,1.),(1.,1.),(1.,1.),(1.,1.),(1.,
1.),(1.,1.),(1.,1.),(1.,1.),(1.,1.),(1.,1.),(1.,1.),(1.,1.),(1.,1.),(1.,
1.),(1.,1.),(1.,1.),(1.,1.),(1.,1.),(1.,1.),(1.,1.),(1.,1.),(1.,1.),(1.,
1.),(1.,1.),(1.,1.),(1.,1.),(1.,1.),(1.,1.),(1.,1.),(1.,1.),(1.,1.),(1.,
1.),(1.,1.),(1.,1.),(1.,1.),(1.,1.),(1.,1.),(1.,1.),(1.,1.),(1.,1.),(1.,
1.),(1.,1.),(1.,1.),(1.,1.),(1.,1.),(1.,1.),(1.,1.),(1.,1.),(1.,1.),(1.,
1.),(1.,1.),(1.,1.),(1.,1.),(1.,1.),(1.,1.),(1.,1.),(1.,1.),(1.,1.),(1.,
1.),(1.,1.),(1.,1.),(1.,1.),(1.,1.),(1.,1.),(1.,1.),(1.,1.),(1.,1.),(1.,
1.),(1.,1.),(1.,1.),(1.,1.),(1.,1.),(1.,1.),(1.,1.),(1.,1.),(1.,1.),(1.,
1.),(1.,1.),(1.,1.),(1.,1.),(1.,1.),(1.,1.),(1.,1.),(1.,1.),(1.,1.),(1.,
1.),(1.,1.)))
REPRESENTATION_ITEM('')
SURFACE()
);
#990=(
BOUNDED_SURFACE()
B_SPLINE_SURFACE(5,1,((#145028,#145029),(#145030,#145031),(#145032,#145033),
(#145034,#145035),(#145036,#145037),(#145038,#145039),(#145040,#145041),
(#145042,#145043),(#145044,#145045),(#145046,#145047),(#145048,#145049),
(#145050,#145051),(#145052,#145053),(#145054,#145055),(#145056,#145057),
(#145058,#145059),(#145060,#145061),(#145062,#145063),(#145064,#145065),
(#145066,#145067),(#145068,#145069),(#145070,#145071),(#145072,#145073),
(#145074,#145075),(#145076,#145077),(#145078,#145079),(#145080,#145081),
(#145082,#145083),(#145084,#145085),(#145086,#145087),(#145088,#145089),
(#145090,#145091),(#145092,#145093),(#145094,#145095),(#145096,#145097),
(#145098,#145099),(#145100,#145101),(#145102,#145103),(#145104,#145105),
(#145106,#145107),(#145108,#145109),(#145110,#145111),(#145112,#145113),
(#145114,#145115),(#145116,#145117),(#145118,#145119),(#145120,#145121),
(#145122,#145123),(#145124,#145125),(#145126,#145127),(#145128,#145129),
(#145130,#145131),(#145132,#145133),(#145134,#145135),(#145136,#145137),
(#145138,#145139),(#145140,#145141),(#145142,#145143),(#145144,#145145),
(#145146,#145147),(#145148,#145149),(#145150,#145151),(#145152,#145153),
(#145154,#145155),(#145156,#145157),(#145158,#145159),(#145160,#145161),
(#145162,#145163),(#145164,#145165),(#145166,#145167),(#145168,#145169),
(#145170,#145171),(#145172,#145173),(#145174,#145175),(#145176,#145177),
(#145178,#145179),(#145180,#145181),(#145182,#145183),(#145184,#145185),
(#145186,#145187),(#145188,#145189),(#145190,#145191),(#145192,#145193),
(#145194,#145195),(#145196,#145197),(#145198,#145199),(#145200,#145201),
(#145202,#145203),(#145204,#145205),(#145206,#145207),(#145208,#145209),
(#145210,#145211),(#145212,#145213),(#145214,#145215),(#145216,#145217),
(#145218,#145219),(#145220,#145221),(#145222,#145223),(#145224,#145225),
(#145226,#145227),(#145228,#145229),(#145230,#145231),(#145232,#145233),
(#145234,#145235),(#145236,#145237),(#145238,#145239),(#145240,#145241),
(#145242,#145243),(#145244,#145245),(#145246,#145247),(#145248,#145249),
(#145250,#145251),(#145252,#145253),(#145254,#145255),(#145256,#145257),
(#145258,#145259),(#145260,#145261),(#145262,#145263),(#145264,#145265),
(#145266,#145267),(#145268,#145269),(#145270,#145271),(#145272,#145273),
(#145274,#145275),(#145276,#145277),(#145278,#145279),(#145280,#145281),
(#145282,#145283),(#145284,#145285),(#145286,#145287),(#145288,#145289),
(#145290,#145291),(#145292,#145293),(#145294,#145295),(#145296,#145297),
(#145298,#145299),(#145300,#145301),(#145302,#145303),(#145304,#145305),
(#145306,#145307),(#145308,#145309),(#145310,#145311),(#145312,#145313),
(#145314,#145315),(#145316,#145317),(#145318,#145319),(#145320,#145321),
(#145322,#145323),(#145324,#145325),(#145326,#145327),(#145328,#145329),
(#145330,#145331),(#145332,#145333),(#145334,#145335),(#145336,#145337),
(#145338,#145339),(#145340,#145341),(#145342,#145343),(#145344,#145345),
(#145346,#145347),(#145348,#145349),(#145350,#145351),(#145352,#145353),
(#145354,#145355),(#145356,#145357),(#145358,#145359),(#145360,#145361),
(#145362,#145363),(#145364,#145365),(#145366,#145367),(#145368,#145369),
(#145370,#145371),(#145372,#145373),(#145374,#145375),(#145376,#145377),
(#145378,#145379),(#145380,#145381),(#145382,#145383),(#145384,#145385),
(#145386,#145387),(#145388,#145389),(#145390,#145391),(#145392,#145393),
(#145394,#145395),(#145396,#145397),(#145398,#145399),(#145400,#145401),
(#145402,#145403),(#145404,#145405),(#145406,#145407),(#145408,#145409),
(#145410,#145411),(#145412,#145413),(#145414,#145415),(#145416,#145417),
(#145418,#145419),(#145420,#145421),(#145422,#145423),(#145424,#145425),
(#145426,#145427),(#145428,#145429),(#145430,#145431),(#145432,#145433),
(#145434,#145435),(#145436,#145437)),.UNSPECIFIED.,.F.,.F.,.F.)
B_SPLINE_SURFACE_WITH_KNOTS((6,1,1,1,1,1,1,1,1,1,1,1,1,1,1,1,1,1,1,1,1,
1,1,1,1,1,1,1,1,1,1,1,1,1,1,1,1,1,1,1,1,1,1,1,1,1,1,1,1,1,1,1,1,1,1,1,1,
1,1,1,1,1,1,1,1,1,1,1,1,1,1,1,1,1,1,1,1,1,1,1,1,1,1,1,1,1,1,1,1,1,1,1,1,
1,1,1,1,1,1,1,1,1,1,1,1,1,1,1,1,1,1,1,1,1,1,1,1,1,1,1,1,1,1,1,1,1,1,1,1,
1,1,1,1,1,1,1,1,1,1,1,1,1,1,1,1,1,1,1,1,1,1,1,1,1,1,1,1,1,1,1,1,1,1,1,1,
1,1,1,1,1,1,1,1,1,1,1,1,1,1,1,1,1,1,1,1,1,1,1,1,1,1,1,1,1,1,1,1,1,1,1,6),
(2,2),(-1.,-0.995000000000001,-0.990000000000001,-0.985000000000001,-0.980000000000001,
-0.975000000000001,-0.970000000000001,-0.965000000000001,-0.960000000000001,
-0.955000000000001,-0.950000000000001,-0.945000000000001,-0.940000000000001,
-0.935000000000001,-0.930000000000001,-0.925000000000001,-0.920000000000001,
-0.915000000000001,-0.910000000000001,-0.905000000000001,-0.900000000000001,
-0.895000000000001,-0.890000000000001,-0.885000000000001,-0.880000000000001,
-0.875000000000001,-0.870000000000001,-0.865000000000001,-0.860000000000001,
-0.855000000000001,-0.850000000000001,-0.845000000000001,-0.840000000000001,
-0.835000000000001,-0.830000000000001,-0.825000000000001,-0.820000000000001,
-0.815000000000001,-0.810000000000001,-0.805000000000001,-0.800000000000001,
-0.795000000000001,-0.790000000000001,-0.785000000000001,-0.780000000000001,
-0.775000000000001,-0.770000000000001,-0.765000000000001,-0.760000000000001,
-0.755000000000001,-0.750000000000001,-0.745000000000001,-0.740000000000001,
-0.735000000000001,-0.730000000000001,-0.725000000000001,-0.720000000000001,
-0.715000000000001,-0.710000000000001,-0.705000000000001,-0.700000000000001,
-0.695000000000001,-0.690000000000001,-0.685,-0.68,-0.675,-0.67,-0.665,
-0.66,-0.655,-0.65,-0.645,-0.64,-0.635,-0.63,-0.625,-0.62,-0.615,-0.61,
-0.605,-0.6,-0.595,-0.59,-0.585,-0.58,-0.575,-0.57,-0.565,-0.56,-0.555,
-0.55,-0.545,-0.54,-0.535,-0.53,-0.525,-0.52,-0.515,-0.51,-0.505,-0.5,-0.495,
-0.49,-0.485,-0.48,-0.475,-0.47,-0.465,-0.46,-0.455,-0.45,-0.445,-0.44,
-0.435,-0.43,-0.425,-0.42,-0.415,-0.41,-0.405,-0.4,-0.395,-0.39,-0.385,
-0.38,-0.375,-0.37,-0.365,-0.36,-0.355,-0.35,-0.345,-0.34,-0.335,-0.33,
-0.325,-0.32,-0.315,-0.31,-0.305,-0.3,-0.295,-0.29,-0.285,-0.28,-0.275,
-0.27,-0.265,-0.26,-0.255,-0.25,-0.245,-0.24,-0.235,-0.23,-0.225,-0.22,
-0.215,-0.21,-0.205,-0.2,-0.195,-0.19,-0.185,-0.18,-0.175,-0.17,-0.165,
-0.16,-0.155,-0.15,-0.145,-0.14,-0.135,-0.13,-0.125,-0.12,-0.115,-0.11,
-0.105,-0.1,-0.095,-0.09,-0.085,-0.08,-0.075,-0.07,-0.065,-0.06,-0.055,
-0.05,-0.045,-0.04,-0.035,-0.03,-0.025,-0.02,-0.015,-0.01,-0.005,0.),(0.,
1.2),.UNSPECIFIED.)
GEOMETRIC_REPRESENTATION_ITEM()
RATIONAL_B_SPLINE_SURFACE(((1.,1.),(1.,1.),(1.,1.),(1.,1.),(1.,1.),(1.,
1.),(1.,1.),(1.,1.),(1.,1.),(1.,1.),(1.,1.),(1.,1.),(1.,1.),(1.,1.),(1.,
1.),(1.,1.),(1.,1.),(1.,1.),(1.,1.),(1.,1.),(1.,1.),(1.,1.),(1.,1.),(1.,
1.),(1.,1.),(1.,1.),(1.,1.),(1.,1.),(1.,1.),(1.,1.),(1.,1.),(1.,1.),(1.,
1.),(1.,1.),(1.,1.),(1.,1.),(1.,1.),(1.,1.),(1.,1.),(1.,1.),(1.,1.),(1.,
1.),(1.,1.),(1.,1.),(1.,1.),(1.,1.),(1.,1.),(1.,1.),(1.,1.),(1.,1.),(1.,
1.),(1.,1.),(1.,1.),(1.,1.),(1.,1.),(1.,1.),(1.,1.),(1.,1.),(1.,1.),(1.,
1.),(1.,1.),(1.,1.),(1.,1.),(1.,1.),(1.,1.),(1.,1.),(1.,1.),(1.,1.),(1.,
1.),(1.,1.),(1.,1.),(1.,1.),(1.,1.),(1.,1.),(1.,1.),(1.,1.),(1.,1.),(1.,
1.),(1.,1.),(1.,1.),(1.,1.),(1.,1.),(1.,1.),(1.,1.),(1.,1.),(1.,1.),(1.,
1.),(1.,1.),(1.,1.),(1.,1.),(1.,1.),(1.,1.),(1.,1.),(1.,1.),(1.,1.),(1.,
1.),(1.,1.),(1.,1.),(1.,1.),(1.,1.),(1.,1.),(1.,1.),(1.,1.),(1.,1.),(1.,
1.),(1.,1.),(1.,1.),(1.,1.),(1.,1.),(1.,1.),(1.,1.),(1.,1.),(1.,1.),(1.,
1.),(1.,1.),(1.,1.),(1.,1.),(1.,1.),(1.,1.),(1.,1.),(1.,1.),(1.,1.),(1.,
1.),(1.,1.),(1.,1.),(1.,1.),(1.,1.),(1.,1.),(1.,1.),(1.,1.),(1.,1.),(1.,
1.),(1.,1.),(1.,1.),(1.,1.),(1.,1.),(1.,1.),(1.,1.),(1.,1.),(1.,1.),(1.,
1.),(1.,1.),(1.,1.),(1.,1.),(1.,1.),(1.,1.),(1.,1.),(1.,1.),(1.,1.),(1.,
1.),(1.,1.),(1.,1.),(1.,1.),(1.,1.),(1.,1.),(1.,1.),(1.,1.),(1.,1.),(1.,
1.),(1.,1.),(1.,1.),(1.,1.),(1.,1.),(1.,1.),(1.,1.),(1.,1.),(1.,1.),(1.,
1.),(1.,1.),(1.,1.),(1.,1.),(1.,1.),(1.,1.),(1.,1.),(1.,1.),(1.,1.),(1.,
1.),(1.,1.),(1.,1.),(1.,1.),(1.,1.),(1.,1.),(1.,1.),(1.,1.),(1.,1.),(1.,
1.),(1.,1.),(1.,1.),(1.,1.),(1.,1.),(1.,1.),(1.,1.),(1.,1.),(1.,1.),(1.,
1.),(1.,1.),(1.,1.),(1.,1.),(1.,1.),(1.,1.),(1.,1.),(1.,1.),(1.,1.),(1.,
1.),(1.,1.)))
REPRESENTATION_ITEM('')
SURFACE()
);
#991=(
BOUNDED_SURFACE()
B_SPLINE_SURFACE(5,1,((#145829,#145830),(#145831,#145832),(#145833,#145834),
(#145835,#145836),(#145837,#145838),(#145839,#145840),(#145841,#145842),
(#145843,#145844),(#145845,#145846),(#145847,#145848),(#145849,#145850),
(#145851,#145852),(#145853,#145854),(#145855,#145856),(#145857,#145858),
(#145859,#145860),(#145861,#145862),(#145863,#145864),(#145865,#145866),
(#145867,#145868),(#145869,#145870),(#145871,#145872),(#145873,#145874),
(#145875,#145876),(#145877,#145878),(#145879,#145880),(#145881,#145882),
(#145883,#145884),(#145885,#145886),(#145887,#145888),(#145889,#145890),
(#145891,#145892),(#145893,#145894),(#145895,#145896),(#145897,#145898),
(#145899,#145900),(#145901,#145902),(#145903,#145904),(#145905,#145906),
(#145907,#145908),(#145909,#145910),(#145911,#145912),(#145913,#145914),
(#145915,#145916),(#145917,#145918),(#145919,#145920),(#145921,#145922),
(#145923,#145924),(#145925,#145926),(#145927,#145928),(#145929,#145930),
(#145931,#145932),(#145933,#145934),(#145935,#145936),(#145937,#145938),
(#145939,#145940),(#145941,#145942),(#145943,#145944),(#145945,#145946),
(#145947,#145948),(#145949,#145950),(#145951,#145952),(#145953,#145954),
(#145955,#145956),(#145957,#145958),(#145959,#145960),(#145961,#145962),
(#145963,#145964),(#145965,#145966),(#145967,#145968),(#145969,#145970),
(#145971,#145972),(#145973,#145974),(#145975,#145976),(#145977,#145978),
(#145979,#145980),(#145981,#145982),(#145983,#145984),(#145985,#145986),
(#145987,#145988),(#145989,#145990),(#145991,#145992),(#145993,#145994),
(#145995,#145996),(#145997,#145998),(#145999,#146000),(#146001,#146002),
(#146003,#146004),(#146005,#146006),(#146007,#146008),(#146009,#146010),
(#146011,#146012),(#146013,#146014),(#146015,#146016),(#146017,#146018),
(#146019,#146020),(#146021,#146022),(#146023,#146024),(#146025,#146026),
(#146027,#146028),(#146029,#146030),(#146031,#146032),(#146033,#146034),
(#146035,#146036),(#146037,#146038),(#146039,#146040),(#146041,#146042),
(#146043,#146044),(#146045,#146046),(#146047,#146048),(#146049,#146050),
(#146051,#146052),(#146053,#146054),(#146055,#146056),(#146057,#146058),
(#146059,#146060),(#146061,#146062),(#146063,#146064),(#146065,#146066),
(#146067,#146068),(#146069,#146070),(#146071,#146072),(#146073,#146074),
(#146075,#146076),(#146077,#146078),(#146079,#146080),(#146081,#146082),
(#146083,#146084),(#146085,#146086),(#146087,#146088),(#146089,#146090),
(#146091,#146092),(#146093,#146094),(#146095,#146096),(#146097,#146098),
(#146099,#146100),(#146101,#146102),(#146103,#146104),(#146105,#146106),
(#146107,#146108),(#146109,#146110),(#146111,#146112),(#146113,#146114),
(#146115,#146116),(#146117,#146118),(#146119,#146120),(#146121,#146122),
(#146123,#146124),(#146125,#146126),(#146127,#146128),(#146129,#146130),
(#146131,#146132),(#146133,#146134),(#146135,#146136),(#146137,#146138),
(#146139,#146140),(#146141,#146142),(#146143,#146144),(#146145,#146146),
(#146147,#146148),(#146149,#146150),(#146151,#146152),(#146153,#146154),
(#146155,#146156),(#146157,#146158),(#146159,#146160),(#146161,#146162),
(#146163,#146164),(#146165,#146166),(#146167,#146168),(#146169,#146170),
(#146171,#146172),(#146173,#146174),(#146175,#146176),(#146177,#146178),
(#146179,#146180),(#146181,#146182),(#146183,#146184),(#146185,#146186),
(#146187,#146188),(#146189,#146190),(#146191,#146192),(#146193,#146194),
(#146195,#146196),(#146197,#146198),(#146199,#146200),(#146201,#146202),
(#146203,#146204),(#146205,#146206),(#146207,#146208),(#146209,#146210),
(#146211,#146212),(#146213,#146214),(#146215,#146216),(#146217,#146218),
(#146219,#146220),(#146221,#146222),(#146223,#146224),(#146225,#146226),
(#146227,#146228),(#146229,#146230),(#146231,#146232),(#146233,#146234),
(#146235,#146236),(#146237,#146238)),.UNSPECIFIED.,.F.,.F.,.F.)
B_SPLINE_SURFACE_WITH_KNOTS((6,1,1,1,1,1,1,1,1,1,1,1,1,1,1,1,1,1,1,1,1,
1,1,1,1,1,1,1,1,1,1,1,1,1,1,1,1,1,1,1,1,1,1,1,1,1,1,1,1,1,1,1,1,1,1,1,1,
1,1,1,1,1,1,1,1,1,1,1,1,1,1,1,1,1,1,1,1,1,1,1,1,1,1,1,1,1,1,1,1,1,1,1,1,
1,1,1,1,1,1,1,1,1,1,1,1,1,1,1,1,1,1,1,1,1,1,1,1,1,1,1,1,1,1,1,1,1,1,1,1,
1,1,1,1,1,1,1,1,1,1,1,1,1,1,1,1,1,1,1,1,1,1,1,1,1,1,1,1,1,1,1,1,1,1,1,1,
1,1,1,1,1,1,1,1,1,1,1,1,1,1,1,1,1,1,1,1,1,1,1,1,1,1,1,1,1,1,1,1,1,1,1,6),
(2,2),(-1.,-0.995000000000001,-0.990000000000001,-0.985000000000001,-0.980000000000001,
-0.975000000000001,-0.970000000000001,-0.965000000000001,-0.960000000000001,
-0.955000000000001,-0.950000000000001,-0.945000000000001,-0.940000000000001,
-0.935000000000001,-0.930000000000001,-0.925000000000001,-0.920000000000001,
-0.915000000000001,-0.910000000000001,-0.905000000000001,-0.900000000000001,
-0.895000000000001,-0.890000000000001,-0.885000000000001,-0.880000000000001,
-0.875000000000001,-0.870000000000001,-0.865000000000001,-0.860000000000001,
-0.855000000000001,-0.850000000000001,-0.845000000000001,-0.840000000000001,
-0.835000000000001,-0.830000000000001,-0.825000000000001,-0.820000000000001,
-0.815000000000001,-0.810000000000001,-0.805000000000001,-0.800000000000001,
-0.795000000000001,-0.790000000000001,-0.785000000000001,-0.780000000000001,
-0.775000000000001,-0.770000000000001,-0.765000000000001,-0.760000000000001,
-0.755000000000001,-0.750000000000001,-0.745000000000001,-0.740000000000001,
-0.735000000000001,-0.730000000000001,-0.725000000000001,-0.720000000000001,
-0.715000000000001,-0.710000000000001,-0.705000000000001,-0.700000000000001,
-0.695000000000001,-0.690000000000001,-0.685,-0.68,-0.675,-0.67,-0.665,
-0.66,-0.655,-0.65,-0.645,-0.64,-0.635,-0.63,-0.625,-0.62,-0.615,-0.61,
-0.605,-0.6,-0.595,-0.59,-0.585,-0.58,-0.575,-0.57,-0.565,-0.56,-0.555,
-0.55,-0.545,-0.54,-0.535,-0.53,-0.525,-0.52,-0.515,-0.51,-0.505,-0.5,-0.495,
-0.49,-0.485,-0.48,-0.475,-0.47,-0.465,-0.46,-0.455,-0.45,-0.445,-0.44,
-0.435,-0.43,-0.425,-0.42,-0.415,-0.41,-0.405,-0.4,-0.395,-0.39,-0.385,
-0.38,-0.375,-0.37,-0.365,-0.36,-0.355,-0.35,-0.345,-0.34,-0.335,-0.33,
-0.325,-0.32,-0.315,-0.31,-0.305,-0.3,-0.295,-0.29,-0.285,-0.28,-0.275,
-0.27,-0.265,-0.26,-0.255,-0.25,-0.245,-0.24,-0.235,-0.23,-0.225,-0.22,
-0.215,-0.21,-0.205,-0.2,-0.195,-0.19,-0.185,-0.18,-0.175,-0.17,-0.165,
-0.16,-0.155,-0.15,-0.145,-0.14,-0.135,-0.13,-0.125,-0.12,-0.115,-0.11,
-0.105,-0.1,-0.095,-0.09,-0.085,-0.08,-0.075,-0.07,-0.065,-0.06,-0.055,
-0.05,-0.045,-0.04,-0.035,-0.03,-0.025,-0.02,-0.015,-0.01,-0.005,0.),(0.,
1.2),.UNSPECIFIED.)
GEOMETRIC_REPRESENTATION_ITEM()
RATIONAL_B_SPLINE_SURFACE(((1.,1.),(1.,1.),(1.,1.),(1.,1.),(1.,1.),(1.,
1.),(1.,1.),(1.,1.),(1.,1.),(1.,1.),(1.,1.),(1.,1.),(1.,1.),(1.,1.),(1.,
1.),(1.,1.),(1.,1.),(1.,1.),(1.,1.),(1.,1.),(1.,1.),(1.,1.),(1.,1.),(1.,
1.),(1.,1.),(1.,1.),(1.,1.),(1.,1.),(1.,1.),(1.,1.),(1.,1.),(1.,1.),(1.,
1.),(1.,1.),(1.,1.),(1.,1.),(1.,1.),(1.,1.),(1.,1.),(1.,1.),(1.,1.),(1.,
1.),(1.,1.),(1.,1.),(1.,1.),(1.,1.),(1.,1.),(1.,1.),(1.,1.),(1.,1.),(1.,
1.),(1.,1.),(1.,1.),(1.,1.),(1.,1.),(1.,1.),(1.,1.),(1.,1.),(1.,1.),(1.,
1.),(1.,1.),(1.,1.),(1.,1.),(1.,1.),(1.,1.),(1.,1.),(1.,1.),(1.,1.),(1.,
1.),(1.,1.),(1.,1.),(1.,1.),(1.,1.),(1.,1.),(1.,1.),(1.,1.),(1.,1.),(1.,
1.),(1.,1.),(1.,1.),(1.,1.),(1.,1.),(1.,1.),(1.,1.),(1.,1.),(1.,1.),(1.,
1.),(1.,1.),(1.,1.),(1.,1.),(1.,1.),(1.,1.),(1.,1.),(1.,1.),(1.,1.),(1.,
1.),(1.,1.),(1.,1.),(1.,1.),(1.,1.),(1.,1.),(1.,1.),(1.,1.),(1.,1.),(1.,
1.),(1.,1.),(1.,1.),(1.,1.),(1.,1.),(1.,1.),(1.,1.),(1.,1.),(1.,1.),(1.,
1.),(1.,1.),(1.,1.),(1.,1.),(1.,1.),(1.,1.),(1.,1.),(1.,1.),(1.,1.),(1.,
1.),(1.,1.),(1.,1.),(1.,1.),(1.,1.),(1.,1.),(1.,1.),(1.,1.),(1.,1.),(1.,
1.),(1.,1.),(1.,1.),(1.,1.),(1.,1.),(1.,1.),(1.,1.),(1.,1.),(1.,1.),(1.,
1.),(1.,1.),(1.,1.),(1.,1.),(1.,1.),(1.,1.),(1.,1.),(1.,1.),(1.,1.),(1.,
1.),(1.,1.),(1.,1.),(1.,1.),(1.,1.),(1.,1.),(1.,1.),(1.,1.),(1.,1.),(1.,
1.),(1.,1.),(1.,1.),(1.,1.),(1.,1.),(1.,1.),(1.,1.),(1.,1.),(1.,1.),(1.,
1.),(1.,1.),(1.,1.),(1.,1.),(1.,1.),(1.,1.),(1.,1.),(1.,1.),(1.,1.),(1.,
1.),(1.,1.),(1.,1.),(1.,1.),(1.,1.),(1.,1.),(1.,1.),(1.,1.),(1.,1.),(1.,
1.),(1.,1.),(1.,1.),(1.,1.),(1.,1.),(1.,1.),(1.,1.),(1.,1.),(1.,1.),(1.,
1.),(1.,1.),(1.,1.),(1.,1.),(1.,1.),(1.,1.),(1.,1.),(1.,1.),(1.,1.),(1.,
1.),(1.,1.)))
REPRESENTATION_ITEM('')
SURFACE()
);
#992=(
BOUNDED_SURFACE()
B_SPLINE_SURFACE(5,1,((#146630,#146631),(#146632,#146633),(#146634,#146635),
(#146636,#146637),(#146638,#146639),(#146640,#146641),(#146642,#146643),
(#146644,#146645),(#146646,#146647),(#146648,#146649),(#146650,#146651),
(#146652,#146653),(#146654,#146655),(#146656,#146657),(#146658,#146659),
(#146660,#146661),(#146662,#146663),(#146664,#146665),(#146666,#146667),
(#146668,#146669),(#146670,#146671),(#146672,#146673),(#146674,#146675),
(#146676,#146677),(#146678,#146679),(#146680,#146681),(#146682,#146683),
(#146684,#146685),(#146686,#146687),(#146688,#146689),(#146690,#146691),
(#146692,#146693),(#146694,#146695),(#146696,#146697),(#146698,#146699),
(#146700,#146701),(#146702,#146703),(#146704,#146705),(#146706,#146707),
(#146708,#146709),(#146710,#146711),(#146712,#146713),(#146714,#146715),
(#146716,#146717),(#146718,#146719),(#146720,#146721),(#146722,#146723),
(#146724,#146725),(#146726,#146727),(#146728,#146729),(#146730,#146731),
(#146732,#146733),(#146734,#146735),(#146736,#146737),(#146738,#146739),
(#146740,#146741),(#146742,#146743),(#146744,#146745),(#146746,#146747),
(#146748,#146749),(#146750,#146751),(#146752,#146753),(#146754,#146755),
(#146756,#146757),(#146758,#146759),(#146760,#146761),(#146762,#146763),
(#146764,#146765),(#146766,#146767),(#146768,#146769),(#146770,#146771),
(#146772,#146773),(#146774,#146775),(#146776,#146777),(#146778,#146779),
(#146780,#146781),(#146782,#146783),(#146784,#146785),(#146786,#146787),
(#146788,#146789),(#146790,#146791),(#146792,#146793),(#146794,#146795),
(#146796,#146797),(#146798,#146799),(#146800,#146801),(#146802,#146803),
(#146804,#146805),(#146806,#146807),(#146808,#146809),(#146810,#146811),
(#146812,#146813),(#146814,#146815),(#146816,#146817),(#146818,#146819),
(#146820,#146821),(#146822,#146823),(#146824,#146825),(#146826,#146827),
(#146828,#146829),(#146830,#146831),(#146832,#146833),(#146834,#146835),
(#146836,#146837),(#146838,#146839),(#146840,#146841),(#146842,#146843),
(#146844,#146845),(#146846,#146847),(#146848,#146849),(#146850,#146851),
(#146852,#146853),(#146854,#146855),(#146856,#146857),(#146858,#146859),
(#146860,#146861),(#146862,#146863),(#146864,#146865),(#146866,#146867),
(#146868,#146869),(#146870,#146871),(#146872,#146873),(#146874,#146875),
(#146876,#146877),(#146878,#146879),(#146880,#146881),(#146882,#146883),
(#146884,#146885),(#146886,#146887),(#146888,#146889),(#146890,#146891),
(#146892,#146893),(#146894,#146895),(#146896,#146897),(#146898,#146899),
(#146900,#146901),(#146902,#146903),(#146904,#146905),(#146906,#146907),
(#146908,#146909),(#146910,#146911),(#146912,#146913),(#146914,#146915),
(#146916,#146917),(#146918,#146919),(#146920,#146921),(#146922,#146923),
(#146924,#146925),(#146926,#146927),(#146928,#146929),(#146930,#146931),
(#146932,#146933),(#146934,#146935),(#146936,#146937),(#146938,#146939),
(#146940,#146941),(#146942,#146943),(#146944,#146945),(#146946,#146947),
(#146948,#146949),(#146950,#146951),(#146952,#146953),(#146954,#146955),
(#146956,#146957),(#146958,#146959),(#146960,#146961),(#146962,#146963),
(#146964,#146965),(#146966,#146967),(#146968,#146969),(#146970,#146971),
(#146972,#146973),(#146974,#146975),(#146976,#146977),(#146978,#146979),
(#146980,#146981),(#146982,#146983),(#146984,#146985),(#146986,#146987),
(#146988,#146989),(#146990,#146991),(#146992,#146993),(#146994,#146995),
(#146996,#146997),(#146998,#146999),(#147000,#147001),(#147002,#147003),
(#147004,#147005),(#147006,#147007),(#147008,#147009),(#147010,#147011),
(#147012,#147013),(#147014,#147015),(#147016,#147017),(#147018,#147019),
(#147020,#147021),(#147022,#147023),(#147024,#147025),(#147026,#147027),
(#147028,#147029),(#147030,#147031),(#147032,#147033),(#147034,#147035),
(#147036,#147037),(#147038,#147039)),.UNSPECIFIED.,.F.,.F.,.F.)
B_SPLINE_SURFACE_WITH_KNOTS((6,1,1,1,1,1,1,1,1,1,1,1,1,1,1,1,1,1,1,1,1,
1,1,1,1,1,1,1,1,1,1,1,1,1,1,1,1,1,1,1,1,1,1,1,1,1,1,1,1,1,1,1,1,1,1,1,1,
1,1,1,1,1,1,1,1,1,1,1,1,1,1,1,1,1,1,1,1,1,1,1,1,1,1,1,1,1,1,1,1,1,1,1,1,
1,1,1,1,1,1,1,1,1,1,1,1,1,1,1,1,1,1,1,1,1,1,1,1,1,1,1,1,1,1,1,1,1,1,1,1,
1,1,1,1,1,1,1,1,1,1,1,1,1,1,1,1,1,1,1,1,1,1,1,1,1,1,1,1,1,1,1,1,1,1,1,1,
1,1,1,1,1,1,1,1,1,1,1,1,1,1,1,1,1,1,1,1,1,1,1,1,1,1,1,1,1,1,1,1,1,1,1,6),
(2,2),(-1.,-0.995000000000001,-0.990000000000001,-0.985000000000001,-0.980000000000001,
-0.975000000000001,-0.970000000000001,-0.965000000000001,-0.960000000000001,
-0.955000000000001,-0.950000000000001,-0.945000000000001,-0.940000000000001,
-0.935000000000001,-0.930000000000001,-0.925000000000001,-0.920000000000001,
-0.915000000000001,-0.910000000000001,-0.905000000000001,-0.900000000000001,
-0.895000000000001,-0.890000000000001,-0.885000000000001,-0.880000000000001,
-0.875000000000001,-0.870000000000001,-0.865000000000001,-0.860000000000001,
-0.855000000000001,-0.850000000000001,-0.845000000000001,-0.840000000000001,
-0.835000000000001,-0.830000000000001,-0.825000000000001,-0.820000000000001,
-0.815000000000001,-0.810000000000001,-0.805000000000001,-0.800000000000001,
-0.795000000000001,-0.790000000000001,-0.785000000000001,-0.780000000000001,
-0.775000000000001,-0.770000000000001,-0.765000000000001,-0.760000000000001,
-0.755000000000001,-0.750000000000001,-0.745000000000001,-0.740000000000001,
-0.735000000000001,-0.730000000000001,-0.725000000000001,-0.720000000000001,
-0.715000000000001,-0.710000000000001,-0.705000000000001,-0.700000000000001,
-0.695000000000001,-0.690000000000001,-0.685,-0.68,-0.675,-0.67,-0.665,
-0.66,-0.655,-0.65,-0.645,-0.64,-0.635,-0.63,-0.625,-0.62,-0.615,-0.61,
-0.605,-0.6,-0.595,-0.59,-0.585,-0.58,-0.575,-0.57,-0.565,-0.56,-0.555,
-0.55,-0.545,-0.54,-0.535,-0.53,-0.525,-0.52,-0.515,-0.51,-0.505,-0.5,-0.495,
-0.49,-0.485,-0.48,-0.475,-0.47,-0.465,-0.46,-0.455,-0.45,-0.445,-0.44,
-0.435,-0.43,-0.425,-0.42,-0.415,-0.41,-0.405,-0.4,-0.395,-0.39,-0.385,
-0.38,-0.375,-0.37,-0.365,-0.36,-0.355,-0.35,-0.345,-0.34,-0.335,-0.33,
-0.325,-0.32,-0.315,-0.31,-0.305,-0.3,-0.295,-0.29,-0.285,-0.28,-0.275,
-0.27,-0.265,-0.26,-0.255,-0.25,-0.245,-0.24,-0.235,-0.23,-0.225,-0.22,
-0.215,-0.21,-0.205,-0.2,-0.195,-0.19,-0.185,-0.18,-0.175,-0.17,-0.165,
-0.16,-0.155,-0.15,-0.145,-0.14,-0.135,-0.13,-0.125,-0.12,-0.115,-0.11,
-0.105,-0.1,-0.095,-0.09,-0.085,-0.08,-0.075,-0.07,-0.065,-0.06,-0.055,
-0.05,-0.045,-0.04,-0.035,-0.03,-0.025,-0.02,-0.015,-0.01,-0.005,0.),(0.,
1.2),.UNSPECIFIED.)
GEOMETRIC_REPRESENTATION_ITEM()
RATIONAL_B_SPLINE_SURFACE(((1.,1.),(1.,1.),(1.,1.),(1.,1.),(1.,1.),(1.,
1.),(1.,1.),(1.,1.),(1.,1.),(1.,1.),(1.,1.),(1.,1.),(1.,1.),(1.,1.),(1.,
1.),(1.,1.),(1.,1.),(1.,1.),(1.,1.),(1.,1.),(1.,1.),(1.,1.),(1.,1.),(1.,
1.),(1.,1.),(1.,1.),(1.,1.),(1.,1.),(1.,1.),(1.,1.),(1.,1.),(1.,1.),(1.,
1.),(1.,1.),(1.,1.),(1.,1.),(1.,1.),(1.,1.),(1.,1.),(1.,1.),(1.,1.),(1.,
1.),(1.,1.),(1.,1.),(1.,1.),(1.,1.),(1.,1.),(1.,1.),(1.,1.),(1.,1.),(1.,
1.),(1.,1.),(1.,1.),(1.,1.),(1.,1.),(1.,1.),(1.,1.),(1.,1.),(1.,1.),(1.,
1.),(1.,1.),(1.,1.),(1.,1.),(1.,1.),(1.,1.),(1.,1.),(1.,1.),(1.,1.),(1.,
1.),(1.,1.),(1.,1.),(1.,1.),(1.,1.),(1.,1.),(1.,1.),(1.,1.),(1.,1.),(1.,
1.),(1.,1.),(1.,1.),(1.,1.),(1.,1.),(1.,1.),(1.,1.),(1.,1.),(1.,1.),(1.,
1.),(1.,1.),(1.,1.),(1.,1.),(1.,1.),(1.,1.),(1.,1.),(1.,1.),(1.,1.),(1.,
1.),(1.,1.),(1.,1.),(1.,1.),(1.,1.),(1.,1.),(1.,1.),(1.,1.),(1.,1.),(1.,
1.),(1.,1.),(1.,1.),(1.,1.),(1.,1.),(1.,1.),(1.,1.),(1.,1.),(1.,1.),(1.,
1.),(1.,1.),(1.,1.),(1.,1.),(1.,1.),(1.,1.),(1.,1.),(1.,1.),(1.,1.),(1.,
1.),(1.,1.),(1.,1.),(1.,1.),(1.,1.),(1.,1.),(1.,1.),(1.,1.),(1.,1.),(1.,
1.),(1.,1.),(1.,1.),(1.,1.),(1.,1.),(1.,1.),(1.,1.),(1.,1.),(1.,1.),(1.,
1.),(1.,1.),(1.,1.),(1.,1.),(1.,1.),(1.,1.),(1.,1.),(1.,1.),(1.,1.),(1.,
1.),(1.,1.),(1.,1.),(1.,1.),(1.,1.),(1.,1.),(1.,1.),(1.,1.),(1.,1.),(1.,
1.),(1.,1.),(1.,1.),(1.,1.),(1.,1.),(1.,1.),(1.,1.),(1.,1.),(1.,1.),(1.,
1.),(1.,1.),(1.,1.),(1.,1.),(1.,1.),(1.,1.),(1.,1.),(1.,1.),(1.,1.),(1.,
1.),(1.,1.),(1.,1.),(1.,1.),(1.,1.),(1.,1.),(1.,1.),(1.,1.),(1.,1.),(1.,
1.),(1.,1.),(1.,1.),(1.,1.),(1.,1.),(1.,1.),(1.,1.),(1.,1.),(1.,1.),(1.,
1.),(1.,1.),(1.,1.),(1.,1.),(1.,1.),(1.,1.),(1.,1.),(1.,1.),(1.,1.),(1.,
1.),(1.,1.)))
REPRESENTATION_ITEM('')
SURFACE()
);
#993=(
BOUNDED_SURFACE()
B_SPLINE_SURFACE(5,1,((#147431,#147432),(#147433,#147434),(#147435,#147436),
(#147437,#147438),(#147439,#147440),(#147441,#147442),(#147443,#147444),
(#147445,#147446),(#147447,#147448),(#147449,#147450),(#147451,#147452),
(#147453,#147454),(#147455,#147456),(#147457,#147458),(#147459,#147460),
(#147461,#147462),(#147463,#147464),(#147465,#147466),(#147467,#147468),
(#147469,#147470),(#147471,#147472),(#147473,#147474),(#147475,#147476),
(#147477,#147478),(#147479,#147480),(#147481,#147482),(#147483,#147484),
(#147485,#147486),(#147487,#147488),(#147489,#147490),(#147491,#147492),
(#147493,#147494),(#147495,#147496),(#147497,#147498),(#147499,#147500),
(#147501,#147502),(#147503,#147504),(#147505,#147506),(#147507,#147508),
(#147509,#147510),(#147511,#147512),(#147513,#147514),(#147515,#147516),
(#147517,#147518),(#147519,#147520),(#147521,#147522),(#147523,#147524),
(#147525,#147526),(#147527,#147528),(#147529,#147530),(#147531,#147532),
(#147533,#147534),(#147535,#147536),(#147537,#147538),(#147539,#147540),
(#147541,#147542),(#147543,#147544),(#147545,#147546),(#147547,#147548),
(#147549,#147550),(#147551,#147552),(#147553,#147554),(#147555,#147556),
(#147557,#147558),(#147559,#147560),(#147561,#147562),(#147563,#147564),
(#147565,#147566),(#147567,#147568),(#147569,#147570),(#147571,#147572),
(#147573,#147574),(#147575,#147576),(#147577,#147578),(#147579,#147580),
(#147581,#147582),(#147583,#147584),(#147585,#147586),(#147587,#147588),
(#147589,#147590),(#147591,#147592),(#147593,#147594),(#147595,#147596),
(#147597,#147598),(#147599,#147600),(#147601,#147602),(#147603,#147604),
(#147605,#147606),(#147607,#147608),(#147609,#147610),(#147611,#147612),
(#147613,#147614),(#147615,#147616),(#147617,#147618),(#147619,#147620),
(#147621,#147622),(#147623,#147624),(#147625,#147626),(#147627,#147628),
(#147629,#147630),(#147631,#147632),(#147633,#147634),(#147635,#147636),
(#147637,#147638),(#147639,#147640),(#147641,#147642),(#147643,#147644),
(#147645,#147646),(#147647,#147648),(#147649,#147650),(#147651,#147652),
(#147653,#147654),(#147655,#147656),(#147657,#147658),(#147659,#147660),
(#147661,#147662),(#147663,#147664),(#147665,#147666),(#147667,#147668),
(#147669,#147670),(#147671,#147672),(#147673,#147674),(#147675,#147676),
(#147677,#147678),(#147679,#147680),(#147681,#147682),(#147683,#147684),
(#147685,#147686),(#147687,#147688),(#147689,#147690),(#147691,#147692),
(#147693,#147694),(#147695,#147696),(#147697,#147698),(#147699,#147700),
(#147701,#147702),(#147703,#147704),(#147705,#147706),(#147707,#147708),
(#147709,#147710),(#147711,#147712),(#147713,#147714),(#147715,#147716),
(#147717,#147718),(#147719,#147720),(#147721,#147722),(#147723,#147724),
(#147725,#147726),(#147727,#147728),(#147729,#147730),(#147731,#147732),
(#147733,#147734),(#147735,#147736),(#147737,#147738),(#147739,#147740),
(#147741,#147742),(#147743,#147744),(#147745,#147746),(#147747,#147748),
(#147749,#147750),(#147751,#147752),(#147753,#147754),(#147755,#147756),
(#147757,#147758),(#147759,#147760),(#147761,#147762),(#147763,#147764),
(#147765,#147766),(#147767,#147768),(#147769,#147770),(#147771,#147772),
(#147773,#147774),(#147775,#147776),(#147777,#147778),(#147779,#147780),
(#147781,#147782),(#147783,#147784),(#147785,#147786),(#147787,#147788),
(#147789,#147790),(#147791,#147792),(#147793,#147794),(#147795,#147796),
(#147797,#147798),(#147799,#147800),(#147801,#147802),(#147803,#147804),
(#147805,#147806),(#147807,#147808),(#147809,#147810),(#147811,#147812),
(#147813,#147814),(#147815,#147816),(#147817,#147818),(#147819,#147820),
(#147821,#147822),(#147823,#147824),(#147825,#147826),(#147827,#147828),
(#147829,#147830),(#147831,#147832),(#147833,#147834),(#147835,#147836),
(#147837,#147838),(#147839,#147840)),.UNSPECIFIED.,.F.,.F.,.F.)
B_SPLINE_SURFACE_WITH_KNOTS((6,1,1,1,1,1,1,1,1,1,1,1,1,1,1,1,1,1,1,1,1,
1,1,1,1,1,1,1,1,1,1,1,1,1,1,1,1,1,1,1,1,1,1,1,1,1,1,1,1,1,1,1,1,1,1,1,1,
1,1,1,1,1,1,1,1,1,1,1,1,1,1,1,1,1,1,1,1,1,1,1,1,1,1,1,1,1,1,1,1,1,1,1,1,
1,1,1,1,1,1,1,1,1,1,1,1,1,1,1,1,1,1,1,1,1,1,1,1,1,1,1,1,1,1,1,1,1,1,1,1,
1,1,1,1,1,1,1,1,1,1,1,1,1,1,1,1,1,1,1,1,1,1,1,1,1,1,1,1,1,1,1,1,1,1,1,1,
1,1,1,1,1,1,1,1,1,1,1,1,1,1,1,1,1,1,1,1,1,1,1,1,1,1,1,1,1,1,1,1,1,1,1,6),
(2,2),(-1.,-0.995000000000001,-0.990000000000001,-0.985000000000001,-0.980000000000001,
-0.975000000000001,-0.970000000000001,-0.965000000000001,-0.960000000000001,
-0.955000000000001,-0.950000000000001,-0.945000000000001,-0.940000000000001,
-0.935000000000001,-0.930000000000001,-0.925000000000001,-0.920000000000001,
-0.915000000000001,-0.910000000000001,-0.905000000000001,-0.900000000000001,
-0.895000000000001,-0.890000000000001,-0.885000000000001,-0.880000000000001,
-0.875000000000001,-0.870000000000001,-0.865000000000001,-0.860000000000001,
-0.855000000000001,-0.850000000000001,-0.845000000000001,-0.840000000000001,
-0.835000000000001,-0.830000000000001,-0.825000000000001,-0.820000000000001,
-0.815000000000001,-0.810000000000001,-0.805000000000001,-0.800000000000001,
-0.795000000000001,-0.790000000000001,-0.785000000000001,-0.780000000000001,
-0.775000000000001,-0.770000000000001,-0.765000000000001,-0.760000000000001,
-0.755000000000001,-0.750000000000001,-0.745000000000001,-0.740000000000001,
-0.735000000000001,-0.730000000000001,-0.725000000000001,-0.720000000000001,
-0.715000000000001,-0.710000000000001,-0.705000000000001,-0.700000000000001,
-0.695000000000001,-0.690000000000001,-0.685,-0.68,-0.675,-0.67,-0.665,
-0.66,-0.655,-0.65,-0.645,-0.64,-0.635,-0.63,-0.625,-0.62,-0.615,-0.61,
-0.605,-0.6,-0.595,-0.59,-0.585,-0.58,-0.575,-0.57,-0.565,-0.56,-0.555,
-0.55,-0.545,-0.54,-0.535,-0.53,-0.525,-0.52,-0.515,-0.51,-0.505,-0.5,-0.495,
-0.49,-0.485,-0.48,-0.475,-0.47,-0.465,-0.46,-0.455,-0.45,-0.445,-0.44,
-0.435,-0.43,-0.425,-0.42,-0.415,-0.41,-0.405,-0.4,-0.395,-0.39,-0.385,
-0.38,-0.375,-0.37,-0.365,-0.36,-0.355,-0.35,-0.345,-0.34,-0.335,-0.33,
-0.325,-0.32,-0.315,-0.31,-0.305,-0.3,-0.295,-0.29,-0.285,-0.28,-0.275,
-0.27,-0.265,-0.26,-0.255,-0.25,-0.245,-0.24,-0.235,-0.23,-0.225,-0.22,
-0.215,-0.21,-0.205,-0.2,-0.195,-0.19,-0.185,-0.18,-0.175,-0.17,-0.165,
-0.16,-0.155,-0.15,-0.145,-0.14,-0.135,-0.13,-0.125,-0.12,-0.115,-0.11,
-0.105,-0.1,-0.095,-0.09,-0.085,-0.08,-0.075,-0.07,-0.065,-0.06,-0.055,
-0.05,-0.045,-0.04,-0.035,-0.03,-0.025,-0.02,-0.015,-0.01,-0.005,0.),(0.,
1.2),.UNSPECIFIED.)
GEOMETRIC_REPRESENTATION_ITEM()
RATIONAL_B_SPLINE_SURFACE(((1.,1.),(1.,1.),(1.,1.),(1.,1.),(1.,1.),(1.,
1.),(1.,1.),(1.,1.),(1.,1.),(1.,1.),(1.,1.),(1.,1.),(1.,1.),(1.,1.),(1.,
1.),(1.,1.),(1.,1.),(1.,1.),(1.,1.),(1.,1.),(1.,1.),(1.,1.),(1.,1.),(1.,
1.),(1.,1.),(1.,1.),(1.,1.),(1.,1.),(1.,1.),(1.,1.),(1.,1.),(1.,1.),(1.,
1.),(1.,1.),(1.,1.),(1.,1.),(1.,1.),(1.,1.),(1.,1.),(1.,1.),(1.,1.),(1.,
1.),(1.,1.),(1.,1.),(1.,1.),(1.,1.),(1.,1.),(1.,1.),(1.,1.),(1.,1.),(1.,
1.),(1.,1.),(1.,1.),(1.,1.),(1.,1.),(1.,1.),(1.,1.),(1.,1.),(1.,1.),(1.,
1.),(1.,1.),(1.,1.),(1.,1.),(1.,1.),(1.,1.),(1.,1.),(1.,1.),(1.,1.),(1.,
1.),(1.,1.),(1.,1.),(1.,1.),(1.,1.),(1.,1.),(1.,1.),(1.,1.),(1.,1.),(1.,
1.),(1.,1.),(1.,1.),(1.,1.),(1.,1.),(1.,1.),(1.,1.),(1.,1.),(1.,1.),(1.,
1.),(1.,1.),(1.,1.),(1.,1.),(1.,1.),(1.,1.),(1.,1.),(1.,1.),(1.,1.),(1.,
1.),(1.,1.),(1.,1.),(1.,1.),(1.,1.),(1.,1.),(1.,1.),(1.,1.),(1.,1.),(1.,
1.),(1.,1.),(1.,1.),(1.,1.),(1.,1.),(1.,1.),(1.,1.),(1.,1.),(1.,1.),(1.,
1.),(1.,1.),(1.,1.),(1.,1.),(1.,1.),(1.,1.),(1.,1.),(1.,1.),(1.,1.),(1.,
1.),(1.,1.),(1.,1.),(1.,1.),(1.,1.),(1.,1.),(1.,1.),(1.,1.),(1.,1.),(1.,
1.),(1.,1.),(1.,1.),(1.,1.),(1.,1.),(1.,1.),(1.,1.),(1.,1.),(1.,1.),(1.,
1.),(1.,1.),(1.,1.),(1.,1.),(1.,1.),(1.,1.),(1.,1.),(1.,1.),(1.,1.),(1.,
1.),(1.,1.),(1.,1.),(1.,1.),(1.,1.),(1.,1.),(1.,1.),(1.,1.),(1.,1.),(1.,
1.),(1.,1.),(1.,1.),(1.,1.),(1.,1.),(1.,1.),(1.,1.),(1.,1.),(1.,1.),(1.,
1.),(1.,1.),(1.,1.),(1.,1.),(1.,1.),(1.,1.),(1.,1.),(1.,1.),(1.,1.),(1.,
1.),(1.,1.),(1.,1.),(1.,1.),(1.,1.),(1.,1.),(1.,1.),(1.,1.),(1.,1.),(1.,
1.),(1.,1.),(1.,1.),(1.,1.),(1.,1.),(1.,1.),(1.,1.),(1.,1.),(1.,1.),(1.,
1.),(1.,1.),(1.,1.),(1.,1.),(1.,1.),(1.,1.),(1.,1.),(1.,1.),(1.,1.),(1.,
1.),(1.,1.)))
REPRESENTATION_ITEM('')
SURFACE()
);
#994=(
BOUNDED_SURFACE()
B_SPLINE_SURFACE(5,1,((#148232,#148233),(#148234,#148235),(#148236,#148237),
(#148238,#148239),(#148240,#148241),(#148242,#148243),(#148244,#148245),
(#148246,#148247),(#148248,#148249),(#148250,#148251),(#148252,#148253),
(#148254,#148255),(#148256,#148257),(#148258,#148259),(#148260,#148261),
(#148262,#148263),(#148264,#148265),(#148266,#148267),(#148268,#148269),
(#148270,#148271),(#148272,#148273),(#148274,#148275),(#148276,#148277),
(#148278,#148279),(#148280,#148281),(#148282,#148283),(#148284,#148285),
(#148286,#148287),(#148288,#148289),(#148290,#148291),(#148292,#148293),
(#148294,#148295),(#148296,#148297),(#148298,#148299),(#148300,#148301),
(#148302,#148303),(#148304,#148305),(#148306,#148307),(#148308,#148309),
(#148310,#148311),(#148312,#148313),(#148314,#148315),(#148316,#148317),
(#148318,#148319),(#148320,#148321),(#148322,#148323),(#148324,#148325),
(#148326,#148327),(#148328,#148329),(#148330,#148331),(#148332,#148333),
(#148334,#148335),(#148336,#148337),(#148338,#148339),(#148340,#148341),
(#148342,#148343),(#148344,#148345),(#148346,#148347),(#148348,#148349),
(#148350,#148351),(#148352,#148353),(#148354,#148355),(#148356,#148357),
(#148358,#148359),(#148360,#148361),(#148362,#148363),(#148364,#148365),
(#148366,#148367),(#148368,#148369),(#148370,#148371),(#148372,#148373),
(#148374,#148375),(#148376,#148377),(#148378,#148379),(#148380,#148381),
(#148382,#148383),(#148384,#148385),(#148386,#148387),(#148388,#148389),
(#148390,#148391),(#148392,#148393),(#148394,#148395),(#148396,#148397),
(#148398,#148399),(#148400,#148401),(#148402,#148403),(#148404,#148405),
(#148406,#148407),(#148408,#148409),(#148410,#148411),(#148412,#148413),
(#148414,#148415),(#148416,#148417),(#148418,#148419),(#148420,#148421),
(#148422,#148423),(#148424,#148425),(#148426,#148427),(#148428,#148429),
(#148430,#148431),(#148432,#148433),(#148434,#148435),(#148436,#148437),
(#148438,#148439),(#148440,#148441),(#148442,#148443),(#148444,#148445),
(#148446,#148447),(#148448,#148449),(#148450,#148451),(#148452,#148453),
(#148454,#148455),(#148456,#148457),(#148458,#148459),(#148460,#148461),
(#148462,#148463),(#148464,#148465),(#148466,#148467),(#148468,#148469),
(#148470,#148471),(#148472,#148473),(#148474,#148475),(#148476,#148477),
(#148478,#148479),(#148480,#148481),(#148482,#148483),(#148484,#148485),
(#148486,#148487),(#148488,#148489),(#148490,#148491),(#148492,#148493),
(#148494,#148495),(#148496,#148497),(#148498,#148499),(#148500,#148501),
(#148502,#148503),(#148504,#148505),(#148506,#148507),(#148508,#148509),
(#148510,#148511),(#148512,#148513),(#148514,#148515),(#148516,#148517),
(#148518,#148519),(#148520,#148521),(#148522,#148523),(#148524,#148525),
(#148526,#148527),(#148528,#148529),(#148530,#148531),(#148532,#148533),
(#148534,#148535),(#148536,#148537),(#148538,#148539),(#148540,#148541),
(#148542,#148543),(#148544,#148545),(#148546,#148547),(#148548,#148549),
(#148550,#148551),(#148552,#148553),(#148554,#148555),(#148556,#148557),
(#148558,#148559),(#148560,#148561),(#148562,#148563),(#148564,#148565),
(#148566,#148567),(#148568,#148569),(#148570,#148571),(#148572,#148573),
(#148574,#148575),(#148576,#148577),(#148578,#148579),(#148580,#148581),
(#148582,#148583),(#148584,#148585),(#148586,#148587),(#148588,#148589),
(#148590,#148591),(#148592,#148593),(#148594,#148595),(#148596,#148597),
(#148598,#148599),(#148600,#148601),(#148602,#148603),(#148604,#148605),
(#148606,#148607),(#148608,#148609),(#148610,#148611),(#148612,#148613),
(#148614,#148615),(#148616,#148617),(#148618,#148619),(#148620,#148621),
(#148622,#148623),(#148624,#148625),(#148626,#148627),(#148628,#148629),
(#148630,#148631),(#148632,#148633),(#148634,#148635),(#148636,#148637),
(#148638,#148639),(#148640,#148641)),.UNSPECIFIED.,.F.,.F.,.F.)
B_SPLINE_SURFACE_WITH_KNOTS((6,1,1,1,1,1,1,1,1,1,1,1,1,1,1,1,1,1,1,1,1,
1,1,1,1,1,1,1,1,1,1,1,1,1,1,1,1,1,1,1,1,1,1,1,1,1,1,1,1,1,1,1,1,1,1,1,1,
1,1,1,1,1,1,1,1,1,1,1,1,1,1,1,1,1,1,1,1,1,1,1,1,1,1,1,1,1,1,1,1,1,1,1,1,
1,1,1,1,1,1,1,1,1,1,1,1,1,1,1,1,1,1,1,1,1,1,1,1,1,1,1,1,1,1,1,1,1,1,1,1,
1,1,1,1,1,1,1,1,1,1,1,1,1,1,1,1,1,1,1,1,1,1,1,1,1,1,1,1,1,1,1,1,1,1,1,1,
1,1,1,1,1,1,1,1,1,1,1,1,1,1,1,1,1,1,1,1,1,1,1,1,1,1,1,1,1,1,1,1,1,1,1,6),
(2,2),(-1.,-0.995000000000001,-0.990000000000001,-0.985000000000001,-0.980000000000001,
-0.975000000000001,-0.970000000000001,-0.965000000000001,-0.960000000000001,
-0.955000000000001,-0.950000000000001,-0.945000000000001,-0.940000000000001,
-0.935000000000001,-0.930000000000001,-0.925000000000001,-0.920000000000001,
-0.915000000000001,-0.910000000000001,-0.905000000000001,-0.900000000000001,
-0.895000000000001,-0.890000000000001,-0.885000000000001,-0.880000000000001,
-0.875000000000001,-0.870000000000001,-0.865000000000001,-0.860000000000001,
-0.855000000000001,-0.850000000000001,-0.845000000000001,-0.840000000000001,
-0.835000000000001,-0.830000000000001,-0.825000000000001,-0.820000000000001,
-0.815000000000001,-0.810000000000001,-0.805000000000001,-0.800000000000001,
-0.795000000000001,-0.790000000000001,-0.785000000000001,-0.780000000000001,
-0.775000000000001,-0.770000000000001,-0.765000000000001,-0.760000000000001,
-0.755000000000001,-0.750000000000001,-0.745000000000001,-0.740000000000001,
-0.735000000000001,-0.730000000000001,-0.725000000000001,-0.720000000000001,
-0.715000000000001,-0.710000000000001,-0.705000000000001,-0.700000000000001,
-0.695000000000001,-0.690000000000001,-0.685,-0.68,-0.675,-0.67,-0.665,
-0.66,-0.655,-0.65,-0.645,-0.64,-0.635,-0.63,-0.625,-0.62,-0.615,-0.61,
-0.605,-0.6,-0.595,-0.59,-0.585,-0.58,-0.575,-0.57,-0.565,-0.56,-0.555,
-0.55,-0.545,-0.54,-0.535,-0.53,-0.525,-0.52,-0.515,-0.51,-0.505,-0.5,-0.495,
-0.49,-0.485,-0.48,-0.475,-0.47,-0.465,-0.46,-0.455,-0.45,-0.445,-0.44,
-0.435,-0.43,-0.425,-0.42,-0.415,-0.41,-0.405,-0.4,-0.395,-0.39,-0.385,
-0.38,-0.375,-0.37,-0.365,-0.36,-0.355,-0.35,-0.345,-0.34,-0.335,-0.33,
-0.325,-0.32,-0.315,-0.31,-0.305,-0.3,-0.295,-0.29,-0.285,-0.28,-0.275,
-0.27,-0.265,-0.26,-0.255,-0.25,-0.245,-0.24,-0.235,-0.23,-0.225,-0.22,
-0.215,-0.21,-0.205,-0.2,-0.195,-0.19,-0.185,-0.18,-0.175,-0.17,-0.165,
-0.16,-0.155,-0.15,-0.145,-0.14,-0.135,-0.13,-0.125,-0.12,-0.115,-0.11,
-0.105,-0.1,-0.095,-0.09,-0.085,-0.08,-0.075,-0.07,-0.065,-0.06,-0.055,
-0.05,-0.045,-0.04,-0.035,-0.03,-0.025,-0.02,-0.015,-0.01,-0.005,0.),(0.,
1.2),.UNSPECIFIED.)
GEOMETRIC_REPRESENTATION_ITEM()
RATIONAL_B_SPLINE_SURFACE(((1.,1.),(1.,1.),(1.,1.),(1.,1.),(1.,1.),(1.,
1.),(1.,1.),(1.,1.),(1.,1.),(1.,1.),(1.,1.),(1.,1.),(1.,1.),(1.,1.),(1.,
1.),(1.,1.),(1.,1.),(1.,1.),(1.,1.),(1.,1.),(1.,1.),(1.,1.),(1.,1.),(1.,
1.),(1.,1.),(1.,1.),(1.,1.),(1.,1.),(1.,1.),(1.,1.),(1.,1.),(1.,1.),(1.,
1.),(1.,1.),(1.,1.),(1.,1.),(1.,1.),(1.,1.),(1.,1.),(1.,1.),(1.,1.),(1.,
1.),(1.,1.),(1.,1.),(1.,1.),(1.,1.),(1.,1.),(1.,1.),(1.,1.),(1.,1.),(1.,
1.),(1.,1.),(1.,1.),(1.,1.),(1.,1.),(1.,1.),(1.,1.),(1.,1.),(1.,1.),(1.,
1.),(1.,1.),(1.,1.),(1.,1.),(1.,1.),(1.,1.),(1.,1.),(1.,1.),(1.,1.),(1.,
1.),(1.,1.),(1.,1.),(1.,1.),(1.,1.),(1.,1.),(1.,1.),(1.,1.),(1.,1.),(1.,
1.),(1.,1.),(1.,1.),(1.,1.),(1.,1.),(1.,1.),(1.,1.),(1.,1.),(1.,1.),(1.,
1.),(1.,1.),(1.,1.),(1.,1.),(1.,1.),(1.,1.),(1.,1.),(1.,1.),(1.,1.),(1.,
1.),(1.,1.),(1.,1.),(1.,1.),(1.,1.),(1.,1.),(1.,1.),(1.,1.),(1.,1.),(1.,
1.),(1.,1.),(1.,1.),(1.,1.),(1.,1.),(1.,1.),(1.,1.),(1.,1.),(1.,1.),(1.,
1.),(1.,1.),(1.,1.),(1.,1.),(1.,1.),(1.,1.),(1.,1.),(1.,1.),(1.,1.),(1.,
1.),(1.,1.),(1.,1.),(1.,1.),(1.,1.),(1.,1.),(1.,1.),(1.,1.),(1.,1.),(1.,
1.),(1.,1.),(1.,1.),(1.,1.),(1.,1.),(1.,1.),(1.,1.),(1.,1.),(1.,1.),(1.,
1.),(1.,1.),(1.,1.),(1.,1.),(1.,1.),(1.,1.),(1.,1.),(1.,1.),(1.,1.),(1.,
1.),(1.,1.),(1.,1.),(1.,1.),(1.,1.),(1.,1.),(1.,1.),(1.,1.),(1.,1.),(1.,
1.),(1.,1.),(1.,1.),(1.,1.),(1.,1.),(1.,1.),(1.,1.),(1.,1.),(1.,1.),(1.,
1.),(1.,1.),(1.,1.),(1.,1.),(1.,1.),(1.,1.),(1.,1.),(1.,1.),(1.,1.),(1.,
1.),(1.,1.),(1.,1.),(1.,1.),(1.,1.),(1.,1.),(1.,1.),(1.,1.),(1.,1.),(1.,
1.),(1.,1.),(1.,1.),(1.,1.),(1.,1.),(1.,1.),(1.,1.),(1.,1.),(1.,1.),(1.,
1.),(1.,1.),(1.,1.),(1.,1.),(1.,1.),(1.,1.),(1.,1.),(1.,1.),(1.,1.),(1.,
1.),(1.,1.)))
REPRESENTATION_ITEM('')
SURFACE()
);
#995=(
BOUNDED_SURFACE()
B_SPLINE_SURFACE(5,1,((#149033,#149034),(#149035,#149036),(#149037,#149038),
(#149039,#149040),(#149041,#149042),(#149043,#149044),(#149045,#149046),
(#149047,#149048),(#149049,#149050),(#149051,#149052),(#149053,#149054),
(#149055,#149056),(#149057,#149058),(#149059,#149060),(#149061,#149062),
(#149063,#149064),(#149065,#149066),(#149067,#149068),(#149069,#149070),
(#149071,#149072),(#149073,#149074),(#149075,#149076),(#149077,#149078),
(#149079,#149080),(#149081,#149082),(#149083,#149084),(#149085,#149086),
(#149087,#149088),(#149089,#149090),(#149091,#149092),(#149093,#149094),
(#149095,#149096),(#149097,#149098),(#149099,#149100),(#149101,#149102),
(#149103,#149104),(#149105,#149106),(#149107,#149108),(#149109,#149110),
(#149111,#149112),(#149113,#149114),(#149115,#149116),(#149117,#149118),
(#149119,#149120),(#149121,#149122),(#149123,#149124),(#149125,#149126),
(#149127,#149128),(#149129,#149130),(#149131,#149132),(#149133,#149134),
(#149135,#149136),(#149137,#149138),(#149139,#149140),(#149141,#149142),
(#149143,#149144),(#149145,#149146),(#149147,#149148),(#149149,#149150),
(#149151,#149152),(#149153,#149154),(#149155,#149156),(#149157,#149158),
(#149159,#149160),(#149161,#149162),(#149163,#149164),(#149165,#149166),
(#149167,#149168),(#149169,#149170),(#149171,#149172),(#149173,#149174),
(#149175,#149176),(#149177,#149178),(#149179,#149180),(#149181,#149182),
(#149183,#149184),(#149185,#149186),(#149187,#149188),(#149189,#149190),
(#149191,#149192),(#149193,#149194),(#149195,#149196),(#149197,#149198),
(#149199,#149200),(#149201,#149202),(#149203,#149204),(#149205,#149206),
(#149207,#149208),(#149209,#149210),(#149211,#149212),(#149213,#149214),
(#149215,#149216),(#149217,#149218),(#149219,#149220),(#149221,#149222),
(#149223,#149224),(#149225,#149226),(#149227,#149228),(#149229,#149230),
(#149231,#149232),(#149233,#149234),(#149235,#149236),(#149237,#149238),
(#149239,#149240),(#149241,#149242),(#149243,#149244),(#149245,#149246),
(#149247,#149248),(#149249,#149250),(#149251,#149252),(#149253,#149254),
(#149255,#149256),(#149257,#149258),(#149259,#149260),(#149261,#149262),
(#149263,#149264),(#149265,#149266),(#149267,#149268),(#149269,#149270),
(#149271,#149272),(#149273,#149274),(#149275,#149276),(#149277,#149278),
(#149279,#149280),(#149281,#149282),(#149283,#149284),(#149285,#149286),
(#149287,#149288),(#149289,#149290),(#149291,#149292),(#149293,#149294),
(#149295,#149296),(#149297,#149298),(#149299,#149300),(#149301,#149302),
(#149303,#149304),(#149305,#149306),(#149307,#149308),(#149309,#149310),
(#149311,#149312),(#149313,#149314),(#149315,#149316),(#149317,#149318),
(#149319,#149320),(#149321,#149322),(#149323,#149324),(#149325,#149326),
(#149327,#149328),(#149329,#149330),(#149331,#149332),(#149333,#149334),
(#149335,#149336),(#149337,#149338),(#149339,#149340),(#149341,#149342),
(#149343,#149344),(#149345,#149346),(#149347,#149348),(#149349,#149350),
(#149351,#149352),(#149353,#149354),(#149355,#149356),(#149357,#149358),
(#149359,#149360),(#149361,#149362),(#149363,#149364),(#149365,#149366),
(#149367,#149368),(#149369,#149370),(#149371,#149372),(#149373,#149374),
(#149375,#149376),(#149377,#149378),(#149379,#149380),(#149381,#149382),
(#149383,#149384),(#149385,#149386),(#149387,#149388),(#149389,#149390),
(#149391,#149392),(#149393,#149394),(#149395,#149396),(#149397,#149398),
(#149399,#149400),(#149401,#149402),(#149403,#149404),(#149405,#149406),
(#149407,#149408),(#149409,#149410),(#149411,#149412),(#149413,#149414),
(#149415,#149416),(#149417,#149418),(#149419,#149420),(#149421,#149422),
(#149423,#149424),(#149425,#149426),(#149427,#149428),(#149429,#149430),
(#149431,#149432),(#149433,#149434),(#149435,#149436),(#149437,#149438),
(#149439,#149440),(#149441,#149442)),.UNSPECIFIED.,.F.,.F.,.F.)
B_SPLINE_SURFACE_WITH_KNOTS((6,1,1,1,1,1,1,1,1,1,1,1,1,1,1,1,1,1,1,1,1,
1,1,1,1,1,1,1,1,1,1,1,1,1,1,1,1,1,1,1,1,1,1,1,1,1,1,1,1,1,1,1,1,1,1,1,1,
1,1,1,1,1,1,1,1,1,1,1,1,1,1,1,1,1,1,1,1,1,1,1,1,1,1,1,1,1,1,1,1,1,1,1,1,
1,1,1,1,1,1,1,1,1,1,1,1,1,1,1,1,1,1,1,1,1,1,1,1,1,1,1,1,1,1,1,1,1,1,1,1,
1,1,1,1,1,1,1,1,1,1,1,1,1,1,1,1,1,1,1,1,1,1,1,1,1,1,1,1,1,1,1,1,1,1,1,1,
1,1,1,1,1,1,1,1,1,1,1,1,1,1,1,1,1,1,1,1,1,1,1,1,1,1,1,1,1,1,1,1,1,1,1,6),
(2,2),(-1.,-0.995000000000001,-0.990000000000001,-0.985000000000001,-0.980000000000001,
-0.975000000000001,-0.970000000000001,-0.965000000000001,-0.960000000000001,
-0.955000000000001,-0.950000000000001,-0.945000000000001,-0.940000000000001,
-0.935000000000001,-0.930000000000001,-0.925000000000001,-0.920000000000001,
-0.915000000000001,-0.910000000000001,-0.905000000000001,-0.900000000000001,
-0.895000000000001,-0.890000000000001,-0.885000000000001,-0.880000000000001,
-0.875000000000001,-0.870000000000001,-0.865000000000001,-0.860000000000001,
-0.855000000000001,-0.850000000000001,-0.845000000000001,-0.840000000000001,
-0.835000000000001,-0.830000000000001,-0.825000000000001,-0.820000000000001,
-0.815000000000001,-0.810000000000001,-0.805000000000001,-0.800000000000001,
-0.795000000000001,-0.790000000000001,-0.785000000000001,-0.780000000000001,
-0.775000000000001,-0.770000000000001,-0.765000000000001,-0.760000000000001,
-0.755000000000001,-0.750000000000001,-0.745000000000001,-0.740000000000001,
-0.735000000000001,-0.730000000000001,-0.725000000000001,-0.720000000000001,
-0.715000000000001,-0.710000000000001,-0.705000000000001,-0.700000000000001,
-0.695000000000001,-0.690000000000001,-0.685,-0.68,-0.675,-0.67,-0.665,
-0.66,-0.655,-0.65,-0.645,-0.64,-0.635,-0.63,-0.625,-0.62,-0.615,-0.61,
-0.605,-0.6,-0.595,-0.59,-0.585,-0.58,-0.575,-0.57,-0.565,-0.56,-0.555,
-0.55,-0.545,-0.54,-0.535,-0.53,-0.525,-0.52,-0.515,-0.51,-0.505,-0.5,-0.495,
-0.49,-0.485,-0.48,-0.475,-0.47,-0.465,-0.46,-0.455,-0.45,-0.445,-0.44,
-0.435,-0.43,-0.425,-0.42,-0.415,-0.41,-0.405,-0.4,-0.395,-0.39,-0.385,
-0.38,-0.375,-0.37,-0.365,-0.36,-0.355,-0.35,-0.345,-0.34,-0.335,-0.33,
-0.325,-0.32,-0.315,-0.31,-0.305,-0.3,-0.295,-0.29,-0.285,-0.28,-0.275,
-0.27,-0.265,-0.26,-0.255,-0.25,-0.245,-0.24,-0.235,-0.23,-0.225,-0.22,
-0.215,-0.21,-0.205,-0.2,-0.195,-0.19,-0.185,-0.18,-0.175,-0.17,-0.165,
-0.16,-0.155,-0.15,-0.145,-0.14,-0.135,-0.13,-0.125,-0.12,-0.115,-0.11,
-0.105,-0.1,-0.095,-0.09,-0.085,-0.08,-0.075,-0.07,-0.065,-0.06,-0.055,
-0.05,-0.045,-0.04,-0.035,-0.03,-0.025,-0.02,-0.015,-0.01,-0.005,0.),(0.,
1.2),.UNSPECIFIED.)
GEOMETRIC_REPRESENTATION_ITEM()
RATIONAL_B_SPLINE_SURFACE(((1.,1.),(1.,1.),(1.,1.),(1.,1.),(1.,1.),(1.,
1.),(1.,1.),(1.,1.),(1.,1.),(1.,1.),(1.,1.),(1.,1.),(1.,1.),(1.,1.),(1.,
1.),(1.,1.),(1.,1.),(1.,1.),(1.,1.),(1.,1.),(1.,1.),(1.,1.),(1.,1.),(1.,
1.),(1.,1.),(1.,1.),(1.,1.),(1.,1.),(1.,1.),(1.,1.),(1.,1.),(1.,1.),(1.,
1.),(1.,1.),(1.,1.),(1.,1.),(1.,1.),(1.,1.),(1.,1.),(1.,1.),(1.,1.),(1.,
1.),(1.,1.),(1.,1.),(1.,1.),(1.,1.),(1.,1.),(1.,1.),(1.,1.),(1.,1.),(1.,
1.),(1.,1.),(1.,1.),(1.,1.),(1.,1.),(1.,1.),(1.,1.),(1.,1.),(1.,1.),(1.,
1.),(1.,1.),(1.,1.),(1.,1.),(1.,1.),(1.,1.),(1.,1.),(1.,1.),(1.,1.),(1.,
1.),(1.,1.),(1.,1.),(1.,1.),(1.,1.),(1.,1.),(1.,1.),(1.,1.),(1.,1.),(1.,
1.),(1.,1.),(1.,1.),(1.,1.),(1.,1.),(1.,1.),(1.,1.),(1.,1.),(1.,1.),(1.,
1.),(1.,1.),(1.,1.),(1.,1.),(1.,1.),(1.,1.),(1.,1.),(1.,1.),(1.,1.),(1.,
1.),(1.,1.),(1.,1.),(1.,1.),(1.,1.),(1.,1.),(1.,1.),(1.,1.),(1.,1.),(1.,
1.),(1.,1.),(1.,1.),(1.,1.),(1.,1.),(1.,1.),(1.,1.),(1.,1.),(1.,1.),(1.,
1.),(1.,1.),(1.,1.),(1.,1.),(1.,1.),(1.,1.),(1.,1.),(1.,1.),(1.,1.),(1.,
1.),(1.,1.),(1.,1.),(1.,1.),(1.,1.),(1.,1.),(1.,1.),(1.,1.),(1.,1.),(1.,
1.),(1.,1.),(1.,1.),(1.,1.),(1.,1.),(1.,1.),(1.,1.),(1.,1.),(1.,1.),(1.,
1.),(1.,1.),(1.,1.),(1.,1.),(1.,1.),(1.,1.),(1.,1.),(1.,1.),(1.,1.),(1.,
1.),(1.,1.),(1.,1.),(1.,1.),(1.,1.),(1.,1.),(1.,1.),(1.,1.),(1.,1.),(1.,
1.),(1.,1.),(1.,1.),(1.,1.),(1.,1.),(1.,1.),(1.,1.),(1.,1.),(1.,1.),(1.,
1.),(1.,1.),(1.,1.),(1.,1.),(1.,1.),(1.,1.),(1.,1.),(1.,1.),(1.,1.),(1.,
1.),(1.,1.),(1.,1.),(1.,1.),(1.,1.),(1.,1.),(1.,1.),(1.,1.),(1.,1.),(1.,
1.),(1.,1.),(1.,1.),(1.,1.),(1.,1.),(1.,1.),(1.,1.),(1.,1.),(1.,1.),(1.,
1.),(1.,1.),(1.,1.),(1.,1.),(1.,1.),(1.,1.),(1.,1.),(1.,1.),(1.,1.),(1.,
1.),(1.,1.)))
REPRESENTATION_ITEM('')
SURFACE()
);
#996=(
BOUNDED_SURFACE()
B_SPLINE_SURFACE(5,1,((#149834,#149835),(#149836,#149837),(#149838,#149839),
(#149840,#149841),(#149842,#149843),(#149844,#149845),(#149846,#149847),
(#149848,#149849),(#149850,#149851),(#149852,#149853),(#149854,#149855),
(#149856,#149857),(#149858,#149859),(#149860,#149861),(#149862,#149863),
(#149864,#149865),(#149866,#149867),(#149868,#149869),(#149870,#149871),
(#149872,#149873),(#149874,#149875),(#149876,#149877),(#149878,#149879),
(#149880,#149881),(#149882,#149883),(#149884,#149885),(#149886,#149887),
(#149888,#149889),(#149890,#149891),(#149892,#149893),(#149894,#149895),
(#149896,#149897),(#149898,#149899),(#149900,#149901),(#149902,#149903),
(#149904,#149905),(#149906,#149907),(#149908,#149909),(#149910,#149911),
(#149912,#149913),(#149914,#149915),(#149916,#149917),(#149918,#149919),
(#149920,#149921),(#149922,#149923),(#149924,#149925),(#149926,#149927),
(#149928,#149929),(#149930,#149931),(#149932,#149933),(#149934,#149935),
(#149936,#149937),(#149938,#149939),(#149940,#149941),(#149942,#149943),
(#149944,#149945),(#149946,#149947),(#149948,#149949),(#149950,#149951),
(#149952,#149953),(#149954,#149955),(#149956,#149957),(#149958,#149959),
(#149960,#149961),(#149962,#149963),(#149964,#149965),(#149966,#149967),
(#149968,#149969),(#149970,#149971),(#149972,#149973),(#149974,#149975),
(#149976,#149977),(#149978,#149979),(#149980,#149981),(#149982,#149983),
(#149984,#149985),(#149986,#149987),(#149988,#149989),(#149990,#149991),
(#149992,#149993),(#149994,#149995),(#149996,#149997),(#149998,#149999),
(#150000,#150001),(#150002,#150003),(#150004,#150005),(#150006,#150007),
(#150008,#150009),(#150010,#150011),(#150012,#150013),(#150014,#150015),
(#150016,#150017),(#150018,#150019),(#150020,#150021),(#150022,#150023),
(#150024,#150025),(#150026,#150027),(#150028,#150029),(#150030,#150031),
(#150032,#150033),(#150034,#150035),(#150036,#150037),(#150038,#150039),
(#150040,#150041),(#150042,#150043),(#150044,#150045),(#150046,#150047),
(#150048,#150049),(#150050,#150051),(#150052,#150053),(#150054,#150055),
(#150056,#150057),(#150058,#150059),(#150060,#150061),(#150062,#150063),
(#150064,#150065),(#150066,#150067),(#150068,#150069),(#150070,#150071),
(#150072,#150073),(#150074,#150075),(#150076,#150077),(#150078,#150079),
(#150080,#150081),(#150082,#150083),(#150084,#150085),(#150086,#150087),
(#150088,#150089),(#150090,#150091),(#150092,#150093),(#150094,#150095),
(#150096,#150097),(#150098,#150099),(#150100,#150101),(#150102,#150103),
(#150104,#150105),(#150106,#150107),(#150108,#150109),(#150110,#150111),
(#150112,#150113),(#150114,#150115),(#150116,#150117),(#150118,#150119),
(#150120,#150121),(#150122,#150123),(#150124,#150125),(#150126,#150127),
(#150128,#150129),(#150130,#150131),(#150132,#150133),(#150134,#150135),
(#150136,#150137),(#150138,#150139),(#150140,#150141),(#150142,#150143),
(#150144,#150145),(#150146,#150147),(#150148,#150149),(#150150,#150151),
(#150152,#150153),(#150154,#150155),(#150156,#150157),(#150158,#150159),
(#150160,#150161),(#150162,#150163),(#150164,#150165),(#150166,#150167),
(#150168,#150169),(#150170,#150171),(#150172,#150173),(#150174,#150175),
(#150176,#150177),(#150178,#150179),(#150180,#150181),(#150182,#150183),
(#150184,#150185),(#150186,#150187),(#150188,#150189),(#150190,#150191),
(#150192,#150193),(#150194,#150195),(#150196,#150197),(#150198,#150199),
(#150200,#150201),(#150202,#150203),(#150204,#150205),(#150206,#150207),
(#150208,#150209),(#150210,#150211),(#150212,#150213),(#150214,#150215),
(#150216,#150217),(#150218,#150219),(#150220,#150221),(#150222,#150223),
(#150224,#150225),(#150226,#150227),(#150228,#150229),(#150230,#150231),
(#150232,#150233),(#150234,#150235),(#150236,#150237),(#150238,#150239),
(#150240,#150241),(#150242,#150243)),.UNSPECIFIED.,.F.,.F.,.F.)
B_SPLINE_SURFACE_WITH_KNOTS((6,1,1,1,1,1,1,1,1,1,1,1,1,1,1,1,1,1,1,1,1,
1,1,1,1,1,1,1,1,1,1,1,1,1,1,1,1,1,1,1,1,1,1,1,1,1,1,1,1,1,1,1,1,1,1,1,1,
1,1,1,1,1,1,1,1,1,1,1,1,1,1,1,1,1,1,1,1,1,1,1,1,1,1,1,1,1,1,1,1,1,1,1,1,
1,1,1,1,1,1,1,1,1,1,1,1,1,1,1,1,1,1,1,1,1,1,1,1,1,1,1,1,1,1,1,1,1,1,1,1,
1,1,1,1,1,1,1,1,1,1,1,1,1,1,1,1,1,1,1,1,1,1,1,1,1,1,1,1,1,1,1,1,1,1,1,1,
1,1,1,1,1,1,1,1,1,1,1,1,1,1,1,1,1,1,1,1,1,1,1,1,1,1,1,1,1,1,1,1,1,1,1,6),
(2,2),(-1.,-0.995000000000001,-0.990000000000001,-0.985000000000001,-0.980000000000001,
-0.975000000000001,-0.970000000000001,-0.965000000000001,-0.960000000000001,
-0.955000000000001,-0.950000000000001,-0.945000000000001,-0.940000000000001,
-0.935000000000001,-0.930000000000001,-0.925000000000001,-0.920000000000001,
-0.915000000000001,-0.910000000000001,-0.905000000000001,-0.900000000000001,
-0.895000000000001,-0.890000000000001,-0.885000000000001,-0.880000000000001,
-0.875000000000001,-0.870000000000001,-0.865000000000001,-0.860000000000001,
-0.855000000000001,-0.850000000000001,-0.845000000000001,-0.840000000000001,
-0.835000000000001,-0.830000000000001,-0.825000000000001,-0.820000000000001,
-0.815000000000001,-0.810000000000001,-0.805000000000001,-0.800000000000001,
-0.795000000000001,-0.790000000000001,-0.785000000000001,-0.780000000000001,
-0.775000000000001,-0.770000000000001,-0.765000000000001,-0.760000000000001,
-0.755000000000001,-0.750000000000001,-0.745000000000001,-0.740000000000001,
-0.735000000000001,-0.730000000000001,-0.725000000000001,-0.720000000000001,
-0.715000000000001,-0.710000000000001,-0.705000000000001,-0.700000000000001,
-0.695000000000001,-0.690000000000001,-0.685,-0.68,-0.675,-0.67,-0.665,
-0.66,-0.655,-0.65,-0.645,-0.64,-0.635,-0.63,-0.625,-0.62,-0.615,-0.61,
-0.605,-0.6,-0.595,-0.59,-0.585,-0.58,-0.575,-0.57,-0.565,-0.56,-0.555,
-0.55,-0.545,-0.54,-0.535,-0.53,-0.525,-0.52,-0.515,-0.51,-0.505,-0.5,-0.495,
-0.49,-0.485,-0.48,-0.475,-0.47,-0.465,-0.46,-0.455,-0.45,-0.445,-0.44,
-0.435,-0.43,-0.425,-0.42,-0.415,-0.41,-0.405,-0.4,-0.395,-0.39,-0.385,
-0.38,-0.375,-0.37,-0.365,-0.36,-0.355,-0.35,-0.345,-0.34,-0.335,-0.33,
-0.325,-0.32,-0.315,-0.31,-0.305,-0.3,-0.295,-0.29,-0.285,-0.28,-0.275,
-0.27,-0.265,-0.26,-0.255,-0.25,-0.245,-0.24,-0.235,-0.23,-0.225,-0.22,
-0.215,-0.21,-0.205,-0.2,-0.195,-0.19,-0.185,-0.18,-0.175,-0.17,-0.165,
-0.16,-0.155,-0.15,-0.145,-0.14,-0.135,-0.13,-0.125,-0.12,-0.115,-0.11,
-0.105,-0.1,-0.095,-0.09,-0.085,-0.08,-0.075,-0.07,-0.065,-0.06,-0.055,
-0.05,-0.045,-0.04,-0.035,-0.03,-0.025,-0.02,-0.015,-0.01,-0.005,0.),(0.,
1.2),.UNSPECIFIED.)
GEOMETRIC_REPRESENTATION_ITEM()
RATIONAL_B_SPLINE_SURFACE(((1.,1.),(1.,1.),(1.,1.),(1.,1.),(1.,1.),(1.,
1.),(1.,1.),(1.,1.),(1.,1.),(1.,1.),(1.,1.),(1.,1.),(1.,1.),(1.,1.),(1.,
1.),(1.,1.),(1.,1.),(1.,1.),(1.,1.),(1.,1.),(1.,1.),(1.,1.),(1.,1.),(1.,
1.),(1.,1.),(1.,1.),(1.,1.),(1.,1.),(1.,1.),(1.,1.),(1.,1.),(1.,1.),(1.,
1.),(1.,1.),(1.,1.),(1.,1.),(1.,1.),(1.,1.),(1.,1.),(1.,1.),(1.,1.),(1.,
1.),(1.,1.),(1.,1.),(1.,1.),(1.,1.),(1.,1.),(1.,1.),(1.,1.),(1.,1.),(1.,
1.),(1.,1.),(1.,1.),(1.,1.),(1.,1.),(1.,1.),(1.,1.),(1.,1.),(1.,1.),(1.,
1.),(1.,1.),(1.,1.),(1.,1.),(1.,1.),(1.,1.),(1.,1.),(1.,1.),(1.,1.),(1.,
1.),(1.,1.),(1.,1.),(1.,1.),(1.,1.),(1.,1.),(1.,1.),(1.,1.),(1.,1.),(1.,
1.),(1.,1.),(1.,1.),(1.,1.),(1.,1.),(1.,1.),(1.,1.),(1.,1.),(1.,1.),(1.,
1.),(1.,1.),(1.,1.),(1.,1.),(1.,1.),(1.,1.),(1.,1.),(1.,1.),(1.,1.),(1.,
1.),(1.,1.),(1.,1.),(1.,1.),(1.,1.),(1.,1.),(1.,1.),(1.,1.),(1.,1.),(1.,
1.),(1.,1.),(1.,1.),(1.,1.),(1.,1.),(1.,1.),(1.,1.),(1.,1.),(1.,1.),(1.,
1.),(1.,1.),(1.,1.),(1.,1.),(1.,1.),(1.,1.),(1.,1.),(1.,1.),(1.,1.),(1.,
1.),(1.,1.),(1.,1.),(1.,1.),(1.,1.),(1.,1.),(1.,1.),(1.,1.),(1.,1.),(1.,
1.),(1.,1.),(1.,1.),(1.,1.),(1.,1.),(1.,1.),(1.,1.),(1.,1.),(1.,1.),(1.,
1.),(1.,1.),(1.,1.),(1.,1.),(1.,1.),(1.,1.),(1.,1.),(1.,1.),(1.,1.),(1.,
1.),(1.,1.),(1.,1.),(1.,1.),(1.,1.),(1.,1.),(1.,1.),(1.,1.),(1.,1.),(1.,
1.),(1.,1.),(1.,1.),(1.,1.),(1.,1.),(1.,1.),(1.,1.),(1.,1.),(1.,1.),(1.,
1.),(1.,1.),(1.,1.),(1.,1.),(1.,1.),(1.,1.),(1.,1.),(1.,1.),(1.,1.),(1.,
1.),(1.,1.),(1.,1.),(1.,1.),(1.,1.),(1.,1.),(1.,1.),(1.,1.),(1.,1.),(1.,
1.),(1.,1.),(1.,1.),(1.,1.),(1.,1.),(1.,1.),(1.,1.),(1.,1.),(1.,1.),(1.,
1.),(1.,1.),(1.,1.),(1.,1.),(1.,1.),(1.,1.),(1.,1.),(1.,1.),(1.,1.),(1.,
1.),(1.,1.)))
REPRESENTATION_ITEM('')
SURFACE()
);
#997=(
BOUNDED_SURFACE()
B_SPLINE_SURFACE(5,1,((#150635,#150636),(#150637,#150638),(#150639,#150640),
(#150641,#150642),(#150643,#150644),(#150645,#150646),(#150647,#150648),
(#150649,#150650),(#150651,#150652),(#150653,#150654),(#150655,#150656),
(#150657,#150658),(#150659,#150660),(#150661,#150662),(#150663,#150664),
(#150665,#150666),(#150667,#150668),(#150669,#150670),(#150671,#150672),
(#150673,#150674),(#150675,#150676),(#150677,#150678),(#150679,#150680),
(#150681,#150682),(#150683,#150684),(#150685,#150686),(#150687,#150688),
(#150689,#150690),(#150691,#150692),(#150693,#150694),(#150695,#150696),
(#150697,#150698),(#150699,#150700),(#150701,#150702),(#150703,#150704),
(#150705,#150706),(#150707,#150708),(#150709,#150710),(#150711,#150712),
(#150713,#150714),(#150715,#150716),(#150717,#150718),(#150719,#150720),
(#150721,#150722),(#150723,#150724),(#150725,#150726),(#150727,#150728),
(#150729,#150730),(#150731,#150732),(#150733,#150734),(#150735,#150736),
(#150737,#150738),(#150739,#150740),(#150741,#150742),(#150743,#150744),
(#150745,#150746),(#150747,#150748),(#150749,#150750),(#150751,#150752),
(#150753,#150754),(#150755,#150756),(#150757,#150758),(#150759,#150760),
(#150761,#150762),(#150763,#150764),(#150765,#150766),(#150767,#150768),
(#150769,#150770),(#150771,#150772),(#150773,#150774),(#150775,#150776),
(#150777,#150778),(#150779,#150780),(#150781,#150782),(#150783,#150784),
(#150785,#150786),(#150787,#150788),(#150789,#150790),(#150791,#150792),
(#150793,#150794),(#150795,#150796),(#150797,#150798),(#150799,#150800),
(#150801,#150802),(#150803,#150804),(#150805,#150806),(#150807,#150808),
(#150809,#150810),(#150811,#150812),(#150813,#150814),(#150815,#150816),
(#150817,#150818),(#150819,#150820),(#150821,#150822),(#150823,#150824),
(#150825,#150826),(#150827,#150828),(#150829,#150830),(#150831,#150832),
(#150833,#150834),(#150835,#150836),(#150837,#150838),(#150839,#150840),
(#150841,#150842),(#150843,#150844),(#150845,#150846),(#150847,#150848),
(#150849,#150850),(#150851,#150852),(#150853,#150854),(#150855,#150856),
(#150857,#150858),(#150859,#150860),(#150861,#150862),(#150863,#150864),
(#150865,#150866),(#150867,#150868),(#150869,#150870),(#150871,#150872),
(#150873,#150874),(#150875,#150876),(#150877,#150878),(#150879,#150880),
(#150881,#150882),(#150883,#150884),(#150885,#150886),(#150887,#150888),
(#150889,#150890),(#150891,#150892),(#150893,#150894),(#150895,#150896),
(#150897,#150898),(#150899,#150900),(#150901,#150902),(#150903,#150904),
(#150905,#150906),(#150907,#150908),(#150909,#150910),(#150911,#150912),
(#150913,#150914),(#150915,#150916),(#150917,#150918),(#150919,#150920),
(#150921,#150922),(#150923,#150924),(#150925,#150926),(#150927,#150928),
(#150929,#150930),(#150931,#150932),(#150933,#150934),(#150935,#150936),
(#150937,#150938),(#150939,#150940),(#150941,#150942),(#150943,#150944),
(#150945,#150946),(#150947,#150948),(#150949,#150950),(#150951,#150952),
(#150953,#150954),(#150955,#150956),(#150957,#150958),(#150959,#150960),
(#150961,#150962),(#150963,#150964),(#150965,#150966),(#150967,#150968),
(#150969,#150970),(#150971,#150972),(#150973,#150974),(#150975,#150976),
(#150977,#150978),(#150979,#150980),(#150981,#150982),(#150983,#150984),
(#150985,#150986),(#150987,#150988),(#150989,#150990),(#150991,#150992),
(#150993,#150994),(#150995,#150996),(#150997,#150998),(#150999,#151000),
(#151001,#151002),(#151003,#151004),(#151005,#151006),(#151007,#151008),
(#151009,#151010),(#151011,#151012),(#151013,#151014),(#151015,#151016),
(#151017,#151018),(#151019,#151020),(#151021,#151022),(#151023,#151024),
(#151025,#151026),(#151027,#151028),(#151029,#151030),(#151031,#151032),
(#151033,#151034),(#151035,#151036),(#151037,#151038),(#151039,#151040),
(#151041,#151042),(#151043,#151044)),.UNSPECIFIED.,.F.,.F.,.F.)
B_SPLINE_SURFACE_WITH_KNOTS((6,1,1,1,1,1,1,1,1,1,1,1,1,1,1,1,1,1,1,1,1,
1,1,1,1,1,1,1,1,1,1,1,1,1,1,1,1,1,1,1,1,1,1,1,1,1,1,1,1,1,1,1,1,1,1,1,1,
1,1,1,1,1,1,1,1,1,1,1,1,1,1,1,1,1,1,1,1,1,1,1,1,1,1,1,1,1,1,1,1,1,1,1,1,
1,1,1,1,1,1,1,1,1,1,1,1,1,1,1,1,1,1,1,1,1,1,1,1,1,1,1,1,1,1,1,1,1,1,1,1,
1,1,1,1,1,1,1,1,1,1,1,1,1,1,1,1,1,1,1,1,1,1,1,1,1,1,1,1,1,1,1,1,1,1,1,1,
1,1,1,1,1,1,1,1,1,1,1,1,1,1,1,1,1,1,1,1,1,1,1,1,1,1,1,1,1,1,1,1,1,1,1,6),
(2,2),(-1.,-0.995000000000001,-0.990000000000001,-0.985000000000001,-0.980000000000001,
-0.975000000000001,-0.970000000000001,-0.965000000000001,-0.960000000000001,
-0.955000000000001,-0.950000000000001,-0.945000000000001,-0.940000000000001,
-0.935000000000001,-0.930000000000001,-0.925000000000001,-0.920000000000001,
-0.915000000000001,-0.910000000000001,-0.905000000000001,-0.900000000000001,
-0.895000000000001,-0.890000000000001,-0.885000000000001,-0.880000000000001,
-0.875000000000001,-0.870000000000001,-0.865000000000001,-0.860000000000001,
-0.855000000000001,-0.850000000000001,-0.845000000000001,-0.840000000000001,
-0.835000000000001,-0.830000000000001,-0.825000000000001,-0.820000000000001,
-0.815000000000001,-0.810000000000001,-0.805000000000001,-0.800000000000001,
-0.795000000000001,-0.790000000000001,-0.785000000000001,-0.780000000000001,
-0.775000000000001,-0.770000000000001,-0.765000000000001,-0.760000000000001,
-0.755000000000001,-0.750000000000001,-0.745000000000001,-0.740000000000001,
-0.735000000000001,-0.730000000000001,-0.725000000000001,-0.720000000000001,
-0.715000000000001,-0.710000000000001,-0.705000000000001,-0.700000000000001,
-0.695000000000001,-0.690000000000001,-0.685,-0.68,-0.675,-0.67,-0.665,
-0.66,-0.655,-0.65,-0.645,-0.64,-0.635,-0.63,-0.625,-0.62,-0.615,-0.61,
-0.605,-0.6,-0.595,-0.59,-0.585,-0.58,-0.575,-0.57,-0.565,-0.56,-0.555,
-0.55,-0.545,-0.54,-0.535,-0.53,-0.525,-0.52,-0.515,-0.51,-0.505,-0.5,-0.495,
-0.49,-0.485,-0.48,-0.475,-0.47,-0.465,-0.46,-0.455,-0.45,-0.445,-0.44,
-0.435,-0.43,-0.425,-0.42,-0.415,-0.41,-0.405,-0.4,-0.395,-0.39,-0.385,
-0.38,-0.375,-0.37,-0.365,-0.36,-0.355,-0.35,-0.345,-0.34,-0.335,-0.33,
-0.325,-0.32,-0.315,-0.31,-0.305,-0.3,-0.295,-0.29,-0.285,-0.28,-0.275,
-0.27,-0.265,-0.26,-0.255,-0.25,-0.245,-0.24,-0.235,-0.23,-0.225,-0.22,
-0.215,-0.21,-0.205,-0.2,-0.195,-0.19,-0.185,-0.18,-0.175,-0.17,-0.165,
-0.16,-0.155,-0.15,-0.145,-0.14,-0.135,-0.13,-0.125,-0.12,-0.115,-0.11,
-0.105,-0.1,-0.095,-0.09,-0.085,-0.08,-0.075,-0.07,-0.065,-0.06,-0.055,
-0.05,-0.045,-0.04,-0.035,-0.03,-0.025,-0.02,-0.015,-0.01,-0.005,0.),(0.,
1.2),.UNSPECIFIED.)
GEOMETRIC_REPRESENTATION_ITEM()
RATIONAL_B_SPLINE_SURFACE(((1.,1.),(1.,1.),(1.,1.),(1.,1.),(1.,1.),(1.,
1.),(1.,1.),(1.,1.),(1.,1.),(1.,1.),(1.,1.),(1.,1.),(1.,1.),(1.,1.),(1.,
1.),(1.,1.),(1.,1.),(1.,1.),(1.,1.),(1.,1.),(1.,1.),(1.,1.),(1.,1.),(1.,
1.),(1.,1.),(1.,1.),(1.,1.),(1.,1.),(1.,1.),(1.,1.),(1.,1.),(1.,1.),(1.,
1.),(1.,1.),(1.,1.),(1.,1.),(1.,1.),(1.,1.),(1.,1.),(1.,1.),(1.,1.),(1.,
1.),(1.,1.),(1.,1.),(1.,1.),(1.,1.),(1.,1.),(1.,1.),(1.,1.),(1.,1.),(1.,
1.),(1.,1.),(1.,1.),(1.,1.),(1.,1.),(1.,1.),(1.,1.),(1.,1.),(1.,1.),(1.,
1.),(1.,1.),(1.,1.),(1.,1.),(1.,1.),(1.,1.),(1.,1.),(1.,1.),(1.,1.),(1.,
1.),(1.,1.),(1.,1.),(1.,1.),(1.,1.),(1.,1.),(1.,1.),(1.,1.),(1.,1.),(1.,
1.),(1.,1.),(1.,1.),(1.,1.),(1.,1.),(1.,1.),(1.,1.),(1.,1.),(1.,1.),(1.,
1.),(1.,1.),(1.,1.),(1.,1.),(1.,1.),(1.,1.),(1.,1.),(1.,1.),(1.,1.),(1.,
1.),(1.,1.),(1.,1.),(1.,1.),(1.,1.),(1.,1.),(1.,1.),(1.,1.),(1.,1.),(1.,
1.),(1.,1.),(1.,1.),(1.,1.),(1.,1.),(1.,1.),(1.,1.),(1.,1.),(1.,1.),(1.,
1.),(1.,1.),(1.,1.),(1.,1.),(1.,1.),(1.,1.),(1.,1.),(1.,1.),(1.,1.),(1.,
1.),(1.,1.),(1.,1.),(1.,1.),(1.,1.),(1.,1.),(1.,1.),(1.,1.),(1.,1.),(1.,
1.),(1.,1.),(1.,1.),(1.,1.),(1.,1.),(1.,1.),(1.,1.),(1.,1.),(1.,1.),(1.,
1.),(1.,1.),(1.,1.),(1.,1.),(1.,1.),(1.,1.),(1.,1.),(1.,1.),(1.,1.),(1.,
1.),(1.,1.),(1.,1.),(1.,1.),(1.,1.),(1.,1.),(1.,1.),(1.,1.),(1.,1.),(1.,
1.),(1.,1.),(1.,1.),(1.,1.),(1.,1.),(1.,1.),(1.,1.),(1.,1.),(1.,1.),(1.,
1.),(1.,1.),(1.,1.),(1.,1.),(1.,1.),(1.,1.),(1.,1.),(1.,1.),(1.,1.),(1.,
1.),(1.,1.),(1.,1.),(1.,1.),(1.,1.),(1.,1.),(1.,1.),(1.,1.),(1.,1.),(1.,
1.),(1.,1.),(1.,1.),(1.,1.),(1.,1.),(1.,1.),(1.,1.),(1.,1.),(1.,1.),(1.,
1.),(1.,1.),(1.,1.),(1.,1.),(1.,1.),(1.,1.),(1.,1.),(1.,1.),(1.,1.),(1.,
1.),(1.,1.)))
REPRESENTATION_ITEM('')
SURFACE()
);
#998=(
BOUNDED_SURFACE()
B_SPLINE_SURFACE(5,1,((#151436,#151437),(#151438,#151439),(#151440,#151441),
(#151442,#151443),(#151444,#151445),(#151446,#151447),(#151448,#151449),
(#151450,#151451),(#151452,#151453),(#151454,#151455),(#151456,#151457),
(#151458,#151459),(#151460,#151461),(#151462,#151463),(#151464,#151465),
(#151466,#151467),(#151468,#151469),(#151470,#151471),(#151472,#151473),
(#151474,#151475),(#151476,#151477),(#151478,#151479),(#151480,#151481),
(#151482,#151483),(#151484,#151485),(#151486,#151487),(#151488,#151489),
(#151490,#151491),(#151492,#151493),(#151494,#151495),(#151496,#151497),
(#151498,#151499),(#151500,#151501),(#151502,#151503),(#151504,#151505),
(#151506,#151507),(#151508,#151509),(#151510,#151511),(#151512,#151513),
(#151514,#151515),(#151516,#151517),(#151518,#151519),(#151520,#151521),
(#151522,#151523),(#151524,#151525),(#151526,#151527),(#151528,#151529),
(#151530,#151531),(#151532,#151533),(#151534,#151535),(#151536,#151537),
(#151538,#151539),(#151540,#151541),(#151542,#151543),(#151544,#151545),
(#151546,#151547),(#151548,#151549),(#151550,#151551),(#151552,#151553),
(#151554,#151555),(#151556,#151557),(#151558,#151559),(#151560,#151561),
(#151562,#151563),(#151564,#151565),(#151566,#151567),(#151568,#151569),
(#151570,#151571),(#151572,#151573),(#151574,#151575),(#151576,#151577),
(#151578,#151579),(#151580,#151581),(#151582,#151583),(#151584,#151585),
(#151586,#151587),(#151588,#151589),(#151590,#151591),(#151592,#151593),
(#151594,#151595),(#151596,#151597),(#151598,#151599),(#151600,#151601),
(#151602,#151603),(#151604,#151605),(#151606,#151607),(#151608,#151609),
(#151610,#151611),(#151612,#151613),(#151614,#151615),(#151616,#151617),
(#151618,#151619),(#151620,#151621),(#151622,#151623),(#151624,#151625),
(#151626,#151627),(#151628,#151629),(#151630,#151631),(#151632,#151633),
(#151634,#151635),(#151636,#151637),(#151638,#151639),(#151640,#151641),
(#151642,#151643),(#151644,#151645),(#151646,#151647),(#151648,#151649),
(#151650,#151651),(#151652,#151653),(#151654,#151655),(#151656,#151657),
(#151658,#151659),(#151660,#151661),(#151662,#151663),(#151664,#151665),
(#151666,#151667),(#151668,#151669),(#151670,#151671),(#151672,#151673),
(#151674,#151675),(#151676,#151677),(#151678,#151679),(#151680,#151681),
(#151682,#151683),(#151684,#151685),(#151686,#151687),(#151688,#151689),
(#151690,#151691),(#151692,#151693),(#151694,#151695),(#151696,#151697),
(#151698,#151699),(#151700,#151701),(#151702,#151703),(#151704,#151705),
(#151706,#151707),(#151708,#151709),(#151710,#151711),(#151712,#151713),
(#151714,#151715),(#151716,#151717),(#151718,#151719),(#151720,#151721),
(#151722,#151723),(#151724,#151725),(#151726,#151727),(#151728,#151729),
(#151730,#151731),(#151732,#151733),(#151734,#151735),(#151736,#151737),
(#151738,#151739),(#151740,#151741),(#151742,#151743),(#151744,#151745),
(#151746,#151747),(#151748,#151749),(#151750,#151751),(#151752,#151753),
(#151754,#151755),(#151756,#151757),(#151758,#151759),(#151760,#151761),
(#151762,#151763),(#151764,#151765),(#151766,#151767),(#151768,#151769),
(#151770,#151771),(#151772,#151773),(#151774,#151775),(#151776,#151777),
(#151778,#151779),(#151780,#151781),(#151782,#151783),(#151784,#151785),
(#151786,#151787),(#151788,#151789),(#151790,#151791),(#151792,#151793),
(#151794,#151795),(#151796,#151797),(#151798,#151799),(#151800,#151801),
(#151802,#151803),(#151804,#151805),(#151806,#151807),(#151808,#151809),
(#151810,#151811),(#151812,#151813),(#151814,#151815),(#151816,#151817),
(#151818,#151819),(#151820,#151821),(#151822,#151823),(#151824,#151825),
(#151826,#151827),(#151828,#151829),(#151830,#151831),(#151832,#151833),
(#151834,#151835),(#151836,#151837),(#151838,#151839),(#151840,#151841),
(#151842,#151843),(#151844,#151845)),.UNSPECIFIED.,.F.,.F.,.F.)
B_SPLINE_SURFACE_WITH_KNOTS((6,1,1,1,1,1,1,1,1,1,1,1,1,1,1,1,1,1,1,1,1,
1,1,1,1,1,1,1,1,1,1,1,1,1,1,1,1,1,1,1,1,1,1,1,1,1,1,1,1,1,1,1,1,1,1,1,1,
1,1,1,1,1,1,1,1,1,1,1,1,1,1,1,1,1,1,1,1,1,1,1,1,1,1,1,1,1,1,1,1,1,1,1,1,
1,1,1,1,1,1,1,1,1,1,1,1,1,1,1,1,1,1,1,1,1,1,1,1,1,1,1,1,1,1,1,1,1,1,1,1,
1,1,1,1,1,1,1,1,1,1,1,1,1,1,1,1,1,1,1,1,1,1,1,1,1,1,1,1,1,1,1,1,1,1,1,1,
1,1,1,1,1,1,1,1,1,1,1,1,1,1,1,1,1,1,1,1,1,1,1,1,1,1,1,1,1,1,1,1,1,1,1,6),
(2,2),(-1.,-0.995000000000001,-0.990000000000001,-0.985000000000001,-0.980000000000001,
-0.975000000000001,-0.970000000000001,-0.965000000000001,-0.960000000000001,
-0.955000000000001,-0.950000000000001,-0.945000000000001,-0.940000000000001,
-0.935000000000001,-0.930000000000001,-0.925000000000001,-0.920000000000001,
-0.915000000000001,-0.910000000000001,-0.905000000000001,-0.900000000000001,
-0.895000000000001,-0.890000000000001,-0.885000000000001,-0.880000000000001,
-0.875000000000001,-0.870000000000001,-0.865000000000001,-0.860000000000001,
-0.855000000000001,-0.850000000000001,-0.845000000000001,-0.840000000000001,
-0.835000000000001,-0.830000000000001,-0.825000000000001,-0.820000000000001,
-0.815000000000001,-0.810000000000001,-0.805000000000001,-0.800000000000001,
-0.795000000000001,-0.790000000000001,-0.785000000000001,-0.780000000000001,
-0.775000000000001,-0.770000000000001,-0.765000000000001,-0.760000000000001,
-0.755000000000001,-0.750000000000001,-0.745000000000001,-0.740000000000001,
-0.735000000000001,-0.730000000000001,-0.725000000000001,-0.720000000000001,
-0.715000000000001,-0.710000000000001,-0.705000000000001,-0.700000000000001,
-0.695000000000001,-0.690000000000001,-0.685,-0.68,-0.675,-0.67,-0.665,
-0.66,-0.655,-0.65,-0.645,-0.64,-0.635,-0.63,-0.625,-0.62,-0.615,-0.61,
-0.605,-0.6,-0.595,-0.59,-0.585,-0.58,-0.575,-0.57,-0.565,-0.56,-0.555,
-0.55,-0.545,-0.54,-0.535,-0.53,-0.525,-0.52,-0.515,-0.51,-0.505,-0.5,-0.495,
-0.49,-0.485,-0.48,-0.475,-0.47,-0.465,-0.46,-0.455,-0.45,-0.445,-0.44,
-0.435,-0.43,-0.425,-0.42,-0.415,-0.41,-0.405,-0.4,-0.395,-0.39,-0.385,
-0.38,-0.375,-0.37,-0.365,-0.36,-0.355,-0.35,-0.345,-0.34,-0.335,-0.33,
-0.325,-0.32,-0.315,-0.31,-0.305,-0.3,-0.295,-0.29,-0.285,-0.28,-0.275,
-0.27,-0.265,-0.26,-0.255,-0.25,-0.245,-0.24,-0.235,-0.23,-0.225,-0.22,
-0.215,-0.21,-0.205,-0.2,-0.195,-0.19,-0.185,-0.18,-0.175,-0.17,-0.165,
-0.16,-0.155,-0.15,-0.145,-0.14,-0.135,-0.13,-0.125,-0.12,-0.115,-0.11,
-0.105,-0.1,-0.095,-0.09,-0.085,-0.08,-0.075,-0.07,-0.065,-0.06,-0.055,
-0.05,-0.045,-0.04,-0.035,-0.03,-0.025,-0.02,-0.015,-0.01,-0.005,0.),(0.,
1.2),.UNSPECIFIED.)
GEOMETRIC_REPRESENTATION_ITEM()
RATIONAL_B_SPLINE_SURFACE(((1.,1.),(1.,1.),(1.,1.),(1.,1.),(1.,1.),(1.,
1.),(1.,1.),(1.,1.),(1.,1.),(1.,1.),(1.,1.),(1.,1.),(1.,1.),(1.,1.),(1.,
1.),(1.,1.),(1.,1.),(1.,1.),(1.,1.),(1.,1.),(1.,1.),(1.,1.),(1.,1.),(1.,
1.),(1.,1.),(1.,1.),(1.,1.),(1.,1.),(1.,1.),(1.,1.),(1.,1.),(1.,1.),(1.,
1.),(1.,1.),(1.,1.),(1.,1.),(1.,1.),(1.,1.),(1.,1.),(1.,1.),(1.,1.),(1.,
1.),(1.,1.),(1.,1.),(1.,1.),(1.,1.),(1.,1.),(1.,1.),(1.,1.),(1.,1.),(1.,
1.),(1.,1.),(1.,1.),(1.,1.),(1.,1.),(1.,1.),(1.,1.),(1.,1.),(1.,1.),(1.,
1.),(1.,1.),(1.,1.),(1.,1.),(1.,1.),(1.,1.),(1.,1.),(1.,1.),(1.,1.),(1.,
1.),(1.,1.),(1.,1.),(1.,1.),(1.,1.),(1.,1.),(1.,1.),(1.,1.),(1.,1.),(1.,
1.),(1.,1.),(1.,1.),(1.,1.),(1.,1.),(1.,1.),(1.,1.),(1.,1.),(1.,1.),(1.,
1.),(1.,1.),(1.,1.),(1.,1.),(1.,1.),(1.,1.),(1.,1.),(1.,1.),(1.,1.),(1.,
1.),(1.,1.),(1.,1.),(1.,1.),(1.,1.),(1.,1.),(1.,1.),(1.,1.),(1.,1.),(1.,
1.),(1.,1.),(1.,1.),(1.,1.),(1.,1.),(1.,1.),(1.,1.),(1.,1.),(1.,1.),(1.,
1.),(1.,1.),(1.,1.),(1.,1.),(1.,1.),(1.,1.),(1.,1.),(1.,1.),(1.,1.),(1.,
1.),(1.,1.),(1.,1.),(1.,1.),(1.,1.),(1.,1.),(1.,1.),(1.,1.),(1.,1.),(1.,
1.),(1.,1.),(1.,1.),(1.,1.),(1.,1.),(1.,1.),(1.,1.),(1.,1.),(1.,1.),(1.,
1.),(1.,1.),(1.,1.),(1.,1.),(1.,1.),(1.,1.),(1.,1.),(1.,1.),(1.,1.),(1.,
1.),(1.,1.),(1.,1.),(1.,1.),(1.,1.),(1.,1.),(1.,1.),(1.,1.),(1.,1.),(1.,
1.),(1.,1.),(1.,1.),(1.,1.),(1.,1.),(1.,1.),(1.,1.),(1.,1.),(1.,1.),(1.,
1.),(1.,1.),(1.,1.),(1.,1.),(1.,1.),(1.,1.),(1.,1.),(1.,1.),(1.,1.),(1.,
1.),(1.,1.),(1.,1.),(1.,1.),(1.,1.),(1.,1.),(1.,1.),(1.,1.),(1.,1.),(1.,
1.),(1.,1.),(1.,1.),(1.,1.),(1.,1.),(1.,1.),(1.,1.),(1.,1.),(1.,1.),(1.,
1.),(1.,1.),(1.,1.),(1.,1.),(1.,1.),(1.,1.),(1.,1.),(1.,1.),(1.,1.),(1.,
1.),(1.,1.)))
REPRESENTATION_ITEM('')
SURFACE()
);
#999=(
BOUNDED_SURFACE()
B_SPLINE_SURFACE(5,1,((#152237,#152238),(#152239,#152240),(#152241,#152242),
(#152243,#152244),(#152245,#152246),(#152247,#152248),(#152249,#152250),
(#152251,#152252),(#152253,#152254),(#152255,#152256),(#152257,#152258),
(#152259,#152260),(#152261,#152262),(#152263,#152264),(#152265,#152266),
(#152267,#152268),(#152269,#152270),(#152271,#152272),(#152273,#152274),
(#152275,#152276),(#152277,#152278),(#152279,#152280),(#152281,#152282),
(#152283,#152284),(#152285,#152286),(#152287,#152288),(#152289,#152290),
(#152291,#152292),(#152293,#152294),(#152295,#152296),(#152297,#152298),
(#152299,#152300),(#152301,#152302),(#152303,#152304),(#152305,#152306),
(#152307,#152308),(#152309,#152310),(#152311,#152312),(#152313,#152314),
(#152315,#152316),(#152317,#152318),(#152319,#152320),(#152321,#152322),
(#152323,#152324),(#152325,#152326),(#152327,#152328),(#152329,#152330),
(#152331,#152332),(#152333,#152334),(#152335,#152336),(#152337,#152338),
(#152339,#152340),(#152341,#152342),(#152343,#152344),(#152345,#152346),
(#152347,#152348),(#152349,#152350),(#152351,#152352),(#152353,#152354),
(#152355,#152356),(#152357,#152358),(#152359,#152360),(#152361,#152362),
(#152363,#152364),(#152365,#152366),(#152367,#152368),(#152369,#152370),
(#152371,#152372),(#152373,#152374),(#152375,#152376),(#152377,#152378),
(#152379,#152380),(#152381,#152382),(#152383,#152384),(#152385,#152386),
(#152387,#152388),(#152389,#152390),(#152391,#152392),(#152393,#152394),
(#152395,#152396),(#152397,#152398),(#152399,#152400),(#152401,#152402),
(#152403,#152404),(#152405,#152406),(#152407,#152408),(#152409,#152410),
(#152411,#152412),(#152413,#152414),(#152415,#152416),(#152417,#152418),
(#152419,#152420),(#152421,#152422),(#152423,#152424),(#152425,#152426),
(#152427,#152428),(#152429,#152430),(#152431,#152432),(#152433,#152434),
(#152435,#152436),(#152437,#152438),(#152439,#152440),(#152441,#152442),
(#152443,#152444),(#152445,#152446),(#152447,#152448),(#152449,#152450),
(#152451,#152452),(#152453,#152454),(#152455,#152456),(#152457,#152458),
(#152459,#152460),(#152461,#152462),(#152463,#152464),(#152465,#152466),
(#152467,#152468),(#152469,#152470),(#152471,#152472),(#152473,#152474),
(#152475,#152476),(#152477,#152478),(#152479,#152480),(#152481,#152482),
(#152483,#152484),(#152485,#152486),(#152487,#152488),(#152489,#152490),
(#152491,#152492),(#152493,#152494),(#152495,#152496),(#152497,#152498),
(#152499,#152500),(#152501,#152502),(#152503,#152504),(#152505,#152506),
(#152507,#152508),(#152509,#152510),(#152511,#152512),(#152513,#152514),
(#152515,#152516),(#152517,#152518),(#152519,#152520),(#152521,#152522),
(#152523,#152524),(#152525,#152526),(#152527,#152528),(#152529,#152530),
(#152531,#152532),(#152533,#152534),(#152535,#152536),(#152537,#152538),
(#152539,#152540),(#152541,#152542),(#152543,#152544),(#152545,#152546),
(#152547,#152548),(#152549,#152550),(#152551,#152552),(#152553,#152554),
(#152555,#152556),(#152557,#152558),(#152559,#152560),(#152561,#152562),
(#152563,#152564),(#152565,#152566),(#152567,#152568),(#152569,#152570),
(#152571,#152572),(#152573,#152574),(#152575,#152576),(#152577,#152578),
(#152579,#152580),(#152581,#152582),(#152583,#152584),(#152585,#152586),
(#152587,#152588),(#152589,#152590),(#152591,#152592),(#152593,#152594),
(#152595,#152596),(#152597,#152598),(#152599,#152600),(#152601,#152602),
(#152603,#152604),(#152605,#152606),(#152607,#152608),(#152609,#152610),
(#152611,#152612),(#152613,#152614),(#152615,#152616),(#152617,#152618),
(#152619,#152620),(#152621,#152622),(#152623,#152624),(#152625,#152626),
(#152627,#152628),(#152629,#152630),(#152631,#152632),(#152633,#152634),
(#152635,#152636),(#152637,#152638),(#152639,#152640),(#152641,#152642),
(#152643,#152644),(#152645,#152646)),.UNSPECIFIED.,.F.,.F.,.F.)
B_SPLINE_SURFACE_WITH_KNOTS((6,1,1,1,1,1,1,1,1,1,1,1,1,1,1,1,1,1,1,1,1,
1,1,1,1,1,1,1,1,1,1,1,1,1,1,1,1,1,1,1,1,1,1,1,1,1,1,1,1,1,1,1,1,1,1,1,1,
1,1,1,1,1,1,1,1,1,1,1,1,1,1,1,1,1,1,1,1,1,1,1,1,1,1,1,1,1,1,1,1,1,1,1,1,
1,1,1,1,1,1,1,1,1,1,1,1,1,1,1,1,1,1,1,1,1,1,1,1,1,1,1,1,1,1,1,1,1,1,1,1,
1,1,1,1,1,1,1,1,1,1,1,1,1,1,1,1,1,1,1,1,1,1,1,1,1,1,1,1,1,1,1,1,1,1,1,1,
1,1,1,1,1,1,1,1,1,1,1,1,1,1,1,1,1,1,1,1,1,1,1,1,1,1,1,1,1,1,1,1,1,1,1,6),
(2,2),(-1.,-0.995000000000001,-0.990000000000001,-0.985000000000001,-0.980000000000001,
-0.975000000000001,-0.970000000000001,-0.965000000000001,-0.960000000000001,
-0.955000000000001,-0.950000000000001,-0.945000000000001,-0.940000000000001,
-0.935000000000001,-0.930000000000001,-0.925000000000001,-0.920000000000001,
-0.915000000000001,-0.910000000000001,-0.905000000000001,-0.900000000000001,
-0.895000000000001,-0.890000000000001,-0.885000000000001,-0.880000000000001,
-0.875000000000001,-0.870000000000001,-0.865000000000001,-0.860000000000001,
-0.855000000000001,-0.850000000000001,-0.845000000000001,-0.840000000000001,
-0.835000000000001,-0.830000000000001,-0.825000000000001,-0.820000000000001,
-0.815000000000001,-0.810000000000001,-0.805000000000001,-0.800000000000001,
-0.795000000000001,-0.790000000000001,-0.785000000000001,-0.780000000000001,
-0.775000000000001,-0.770000000000001,-0.765000000000001,-0.760000000000001,
-0.755000000000001,-0.750000000000001,-0.745000000000001,-0.740000000000001,
-0.735000000000001,-0.730000000000001,-0.725000000000001,-0.720000000000001,
-0.715000000000001,-0.710000000000001,-0.705000000000001,-0.700000000000001,
-0.695000000000001,-0.690000000000001,-0.685,-0.68,-0.675,-0.67,-0.665,
-0.66,-0.655,-0.65,-0.645,-0.64,-0.635,-0.63,-0.625,-0.62,-0.615,-0.61,
-0.605,-0.6,-0.595,-0.59,-0.585,-0.58,-0.575,-0.57,-0.565,-0.56,-0.555,
-0.55,-0.545,-0.54,-0.535,-0.53,-0.525,-0.52,-0.515,-0.51,-0.505,-0.5,-0.495,
-0.49,-0.485,-0.48,-0.475,-0.47,-0.465,-0.46,-0.455,-0.45,-0.445,-0.44,
-0.435,-0.43,-0.425,-0.42,-0.415,-0.41,-0.405,-0.4,-0.395,-0.39,-0.385,
-0.38,-0.375,-0.37,-0.365,-0.36,-0.355,-0.35,-0.345,-0.34,-0.335,-0.33,
-0.325,-0.32,-0.315,-0.31,-0.305,-0.3,-0.295,-0.29,-0.285,-0.28,-0.275,
-0.27,-0.265,-0.26,-0.255,-0.25,-0.245,-0.24,-0.235,-0.23,-0.225,-0.22,
-0.215,-0.21,-0.205,-0.2,-0.195,-0.19,-0.185,-0.18,-0.175,-0.17,-0.165,
-0.16,-0.155,-0.15,-0.145,-0.14,-0.135,-0.13,-0.125,-0.12,-0.115,-0.11,
-0.105,-0.1,-0.095,-0.09,-0.085,-0.08,-0.075,-0.07,-0.065,-0.06,-0.055,
-0.05,-0.045,-0.04,-0.035,-0.03,-0.025,-0.02,-0.015,-0.01,-0.005,0.),(0.,
1.2),.UNSPECIFIED.)
GEOMETRIC_REPRESENTATION_ITEM()
RATIONAL_B_SPLINE_SURFACE(((1.,1.),(1.,1.),(1.,1.),(1.,1.),(1.,1.),(1.,
1.),(1.,1.),(1.,1.),(1.,1.),(1.,1.),(1.,1.),(1.,1.),(1.,1.),(1.,1.),(1.,
1.),(1.,1.),(1.,1.),(1.,1.),(1.,1.),(1.,1.),(1.,1.),(1.,1.),(1.,1.),(1.,
1.),(1.,1.),(1.,1.),(1.,1.),(1.,1.),(1.,1.),(1.,1.),(1.,1.),(1.,1.),(1.,
1.),(1.,1.),(1.,1.),(1.,1.),(1.,1.),(1.,1.),(1.,1.),(1.,1.),(1.,1.),(1.,
1.),(1.,1.),(1.,1.),(1.,1.),(1.,1.),(1.,1.),(1.,1.),(1.,1.),(1.,1.),(1.,
1.),(1.,1.),(1.,1.),(1.,1.),(1.,1.),(1.,1.),(1.,1.),(1.,1.),(1.,1.),(1.,
1.),(1.,1.),(1.,1.),(1.,1.),(1.,1.),(1.,1.),(1.,1.),(1.,1.),(1.,1.),(1.,
1.),(1.,1.),(1.,1.),(1.,1.),(1.,1.),(1.,1.),(1.,1.),(1.,1.),(1.,1.),(1.,
1.),(1.,1.),(1.,1.),(1.,1.),(1.,1.),(1.,1.),(1.,1.),(1.,1.),(1.,1.),(1.,
1.),(1.,1.),(1.,1.),(1.,1.),(1.,1.),(1.,1.),(1.,1.),(1.,1.),(1.,1.),(1.,
1.),(1.,1.),(1.,1.),(1.,1.),(1.,1.),(1.,1.),(1.,1.),(1.,1.),(1.,1.),(1.,
1.),(1.,1.),(1.,1.),(1.,1.),(1.,1.),(1.,1.),(1.,1.),(1.,1.),(1.,1.),(1.,
1.),(1.,1.),(1.,1.),(1.,1.),(1.,1.),(1.,1.),(1.,1.),(1.,1.),(1.,1.),(1.,
1.),(1.,1.),(1.,1.),(1.,1.),(1.,1.),(1.,1.),(1.,1.),(1.,1.),(1.,1.),(1.,
1.),(1.,1.),(1.,1.),(1.,1.),(1.,1.),(1.,1.),(1.,1.),(1.,1.),(1.,1.),(1.,
1.),(1.,1.),(1.,1.),(1.,1.),(1.,1.),(1.,1.),(1.,1.),(1.,1.),(1.,1.),(1.,
1.),(1.,1.),(1.,1.),(1.,1.),(1.,1.),(1.,1.),(1.,1.),(1.,1.),(1.,1.),(1.,
1.),(1.,1.),(1.,1.),(1.,1.),(1.,1.),(1.,1.),(1.,1.),(1.,1.),(1.,1.),(1.,
1.),(1.,1.),(1.,1.),(1.,1.),(1.,1.),(1.,1.),(1.,1.),(1.,1.),(1.,1.),(1.,
1.),(1.,1.),(1.,1.),(1.,1.),(1.,1.),(1.,1.),(1.,1.),(1.,1.),(1.,1.),(1.,
1.),(1.,1.),(1.,1.),(1.,1.),(1.,1.),(1.,1.),(1.,1.),(1.,1.),(1.,1.),(1.,
1.),(1.,1.),(1.,1.),(1.,1.),(1.,1.),(1.,1.),(1.,1.),(1.,1.),(1.,1.),(1.,
1.),(1.,1.)))
REPRESENTATION_ITEM('')
SURFACE()
);
#1000=(
BOUNDED_SURFACE()
B_SPLINE_SURFACE(5,1,((#153038,#153039),(#153040,#153041),(#153042,#153043),
(#153044,#153045),(#153046,#153047),(#153048,#153049),(#153050,#153051),
(#153052,#153053),(#153054,#153055),(#153056,#153057),(#153058,#153059),
(#153060,#153061),(#153062,#153063),(#153064,#153065),(#153066,#153067),
(#153068,#153069),(#153070,#153071),(#153072,#153073),(#153074,#153075),
(#153076,#153077),(#153078,#153079),(#153080,#153081),(#153082,#153083),
(#153084,#153085),(#153086,#153087),(#153088,#153089),(#153090,#153091),
(#153092,#153093),(#153094,#153095),(#153096,#153097),(#153098,#153099),
(#153100,#153101),(#153102,#153103),(#153104,#153105),(#153106,#153107),
(#153108,#153109),(#153110,#153111),(#153112,#153113),(#153114,#153115),
(#153116,#153117),(#153118,#153119),(#153120,#153121),(#153122,#153123),
(#153124,#153125),(#153126,#153127),(#153128,#153129),(#153130,#153131),
(#153132,#153133),(#153134,#153135),(#153136,#153137),(#153138,#153139),
(#153140,#153141),(#153142,#153143),(#153144,#153145),(#153146,#153147),
(#153148,#153149),(#153150,#153151),(#153152,#153153),(#153154,#153155),
(#153156,#153157),(#153158,#153159),(#153160,#153161),(#153162,#153163),
(#153164,#153165),(#153166,#153167),(#153168,#153169),(#153170,#153171),
(#153172,#153173),(#153174,#153175),(#153176,#153177),(#153178,#153179),
(#153180,#153181),(#153182,#153183),(#153184,#153185),(#153186,#153187),
(#153188,#153189),(#153190,#153191),(#153192,#153193),(#153194,#153195),
(#153196,#153197),(#153198,#153199),(#153200,#153201),(#153202,#153203),
(#153204,#153205),(#153206,#153207),(#153208,#153209),(#153210,#153211),
(#153212,#153213),(#153214,#153215),(#153216,#153217),(#153218,#153219),
(#153220,#153221),(#153222,#153223),(#153224,#153225),(#153226,#153227),
(#153228,#153229),(#153230,#153231),(#153232,#153233),(#153234,#153235),
(#153236,#153237),(#153238,#153239),(#153240,#153241),(#153242,#153243),
(#153244,#153245),(#153246,#153247),(#153248,#153249),(#153250,#153251),
(#153252,#153253),(#153254,#153255),(#153256,#153257),(#153258,#153259),
(#153260,#153261),(#153262,#153263),(#153264,#153265),(#153266,#153267),
(#153268,#153269),(#153270,#153271),(#153272,#153273),(#153274,#153275),
(#153276,#153277),(#153278,#153279),(#153280,#153281),(#153282,#153283),
(#153284,#153285),(#153286,#153287),(#153288,#153289),(#153290,#153291),
(#153292,#153293),(#153294,#153295),(#153296,#153297),(#153298,#153299),
(#153300,#153301),(#153302,#153303),(#153304,#153305),(#153306,#153307),
(#153308,#153309),(#153310,#153311),(#153312,#153313),(#153314,#153315),
(#153316,#153317),(#153318,#153319),(#153320,#153321),(#153322,#153323),
(#153324,#153325),(#153326,#153327),(#153328,#153329),(#153330,#153331),
(#153332,#153333),(#153334,#153335),(#153336,#153337),(#153338,#153339),
(#153340,#153341),(#153342,#153343),(#153344,#153345),(#153346,#153347),
(#153348,#153349),(#153350,#153351),(#153352,#153353),(#153354,#153355),
(#153356,#153357),(#153358,#153359),(#153360,#153361),(#153362,#153363),
(#153364,#153365),(#153366,#153367),(#153368,#153369),(#153370,#153371),
(#153372,#153373),(#153374,#153375),(#153376,#153377),(#153378,#153379),
(#153380,#153381),(#153382,#153383),(#153384,#153385),(#153386,#153387),
(#153388,#153389),(#153390,#153391),(#153392,#153393),(#153394,#153395),
(#153396,#153397),(#153398,#153399),(#153400,#153401),(#153402,#153403),
(#153404,#153405),(#153406,#153407),(#153408,#153409),(#153410,#153411),
(#153412,#153413),(#153414,#153415),(#153416,#153417),(#153418,#153419),
(#153420,#153421),(#153422,#153423),(#153424,#153425),(#153426,#153427),
(#153428,#153429),(#153430,#153431),(#153432,#153433),(#153434,#153435),
(#153436,#153437),(#153438,#153439),(#153440,#153441),(#153442,#153443),
(#153444,#153445),(#153446,#153447)),.UNSPECIFIED.,.F.,.F.,.F.)
B_SPLINE_SURFACE_WITH_KNOTS((6,1,1,1,1,1,1,1,1,1,1,1,1,1,1,1,1,1,1,1,1,
1,1,1,1,1,1,1,1,1,1,1,1,1,1,1,1,1,1,1,1,1,1,1,1,1,1,1,1,1,1,1,1,1,1,1,1,
1,1,1,1,1,1,1,1,1,1,1,1,1,1,1,1,1,1,1,1,1,1,1,1,1,1,1,1,1,1,1,1,1,1,1,1,
1,1,1,1,1,1,1,1,1,1,1,1,1,1,1,1,1,1,1,1,1,1,1,1,1,1,1,1,1,1,1,1,1,1,1,1,
1,1,1,1,1,1,1,1,1,1,1,1,1,1,1,1,1,1,1,1,1,1,1,1,1,1,1,1,1,1,1,1,1,1,1,1,
1,1,1,1,1,1,1,1,1,1,1,1,1,1,1,1,1,1,1,1,1,1,1,1,1,1,1,1,1,1,1,1,1,1,1,6),
(2,2),(-1.,-0.995000000000001,-0.990000000000001,-0.985000000000001,-0.980000000000001,
-0.975000000000001,-0.970000000000001,-0.965000000000001,-0.960000000000001,
-0.955000000000001,-0.950000000000001,-0.945000000000001,-0.940000000000001,
-0.935000000000001,-0.930000000000001,-0.925000000000001,-0.920000000000001,
-0.915000000000001,-0.910000000000001,-0.905000000000001,-0.900000000000001,
-0.895000000000001,-0.890000000000001,-0.885000000000001,-0.880000000000001,
-0.875000000000001,-0.870000000000001,-0.865000000000001,-0.860000000000001,
-0.855000000000001,-0.850000000000001,-0.845000000000001,-0.840000000000001,
-0.835000000000001,-0.830000000000001,-0.825000000000001,-0.820000000000001,
-0.815000000000001,-0.810000000000001,-0.805000000000001,-0.800000000000001,
-0.795000000000001,-0.790000000000001,-0.785000000000001,-0.780000000000001,
-0.775000000000001,-0.770000000000001,-0.765000000000001,-0.760000000000001,
-0.755000000000001,-0.750000000000001,-0.745000000000001,-0.740000000000001,
-0.735000000000001,-0.730000000000001,-0.725000000000001,-0.720000000000001,
-0.715000000000001,-0.710000000000001,-0.705000000000001,-0.700000000000001,
-0.695000000000001,-0.690000000000001,-0.685,-0.68,-0.675,-0.67,-0.665,
-0.66,-0.655,-0.65,-0.645,-0.64,-0.635,-0.63,-0.625,-0.62,-0.615,-0.61,
-0.605,-0.6,-0.595,-0.59,-0.585,-0.58,-0.575,-0.57,-0.565,-0.56,-0.555,
-0.55,-0.545,-0.54,-0.535,-0.53,-0.525,-0.52,-0.515,-0.51,-0.505,-0.5,-0.495,
-0.49,-0.485,-0.48,-0.475,-0.47,-0.465,-0.46,-0.455,-0.45,-0.445,-0.44,
-0.435,-0.43,-0.425,-0.42,-0.415,-0.41,-0.405,-0.4,-0.395,-0.39,-0.385,
-0.38,-0.375,-0.37,-0.365,-0.36,-0.355,-0.35,-0.345,-0.34,-0.335,-0.33,
-0.325,-0.32,-0.315,-0.31,-0.305,-0.3,-0.295,-0.29,-0.285,-0.28,-0.275,
-0.27,-0.265,-0.26,-0.255,-0.25,-0.245,-0.24,-0.235,-0.23,-0.225,-0.22,
-0.215,-0.21,-0.205,-0.2,-0.195,-0.19,-0.185,-0.18,-0.175,-0.17,-0.165,
-0.16,-0.155,-0.15,-0.145,-0.14,-0.135,-0.13,-0.125,-0.12,-0.115,-0.11,
-0.105,-0.1,-0.095,-0.09,-0.085,-0.08,-0.075,-0.07,-0.065,-0.06,-0.055,
-0.05,-0.045,-0.04,-0.035,-0.03,-0.025,-0.02,-0.015,-0.01,-0.005,0.),(0.,
1.2),.UNSPECIFIED.)
GEOMETRIC_REPRESENTATION_ITEM()
RATIONAL_B_SPLINE_SURFACE(((1.,1.),(1.,1.),(1.,1.),(1.,1.),(1.,1.),(1.,
1.),(1.,1.),(1.,1.),(1.,1.),(1.,1.),(1.,1.),(1.,1.),(1.,1.),(1.,1.),(1.,
1.),(1.,1.),(1.,1.),(1.,1.),(1.,1.),(1.,1.),(1.,1.),(1.,1.),(1.,1.),(1.,
1.),(1.,1.),(1.,1.),(1.,1.),(1.,1.),(1.,1.),(1.,1.),(1.,1.),(1.,1.),(1.,
1.),(1.,1.),(1.,1.),(1.,1.),(1.,1.),(1.,1.),(1.,1.),(1.,1.),(1.,1.),(1.,
1.),(1.,1.),(1.,1.),(1.,1.),(1.,1.),(1.,1.),(1.,1.),(1.,1.),(1.,1.),(1.,
1.),(1.,1.),(1.,1.),(1.,1.),(1.,1.),(1.,1.),(1.,1.),(1.,1.),(1.,1.),(1.,
1.),(1.,1.),(1.,1.),(1.,1.),(1.,1.),(1.,1.),(1.,1.),(1.,1.),(1.,1.),(1.,
1.),(1.,1.),(1.,1.),(1.,1.),(1.,1.),(1.,1.),(1.,1.),(1.,1.),(1.,1.),(1.,
1.),(1.,1.),(1.,1.),(1.,1.),(1.,1.),(1.,1.),(1.,1.),(1.,1.),(1.,1.),(1.,
1.),(1.,1.),(1.,1.),(1.,1.),(1.,1.),(1.,1.),(1.,1.),(1.,1.),(1.,1.),(1.,
1.),(1.,1.),(1.,1.),(1.,1.),(1.,1.),(1.,1.),(1.,1.),(1.,1.),(1.,1.),(1.,
1.),(1.,1.),(1.,1.),(1.,1.),(1.,1.),(1.,1.),(1.,1.),(1.,1.),(1.,1.),(1.,
1.),(1.,1.),(1.,1.),(1.,1.),(1.,1.),(1.,1.),(1.,1.),(1.,1.),(1.,1.),(1.,
1.),(1.,1.),(1.,1.),(1.,1.),(1.,1.),(1.,1.),(1.,1.),(1.,1.),(1.,1.),(1.,
1.),(1.,1.),(1.,1.),(1.,1.),(1.,1.),(1.,1.),(1.,1.),(1.,1.),(1.,1.),(1.,
1.),(1.,1.),(1.,1.),(1.,1.),(1.,1.),(1.,1.),(1.,1.),(1.,1.),(1.,1.),(1.,
1.),(1.,1.),(1.,1.),(1.,1.),(1.,1.),(1.,1.),(1.,1.),(1.,1.),(1.,1.),(1.,
1.),(1.,1.),(1.,1.),(1.,1.),(1.,1.),(1.,1.),(1.,1.),(1.,1.),(1.,1.),(1.,
1.),(1.,1.),(1.,1.),(1.,1.),(1.,1.),(1.,1.),(1.,1.),(1.,1.),(1.,1.),(1.,
1.),(1.,1.),(1.,1.),(1.,1.),(1.,1.),(1.,1.),(1.,1.),(1.,1.),(1.,1.),(1.,
1.),(1.,1.),(1.,1.),(1.,1.),(1.,1.),(1.,1.),(1.,1.),(1.,1.),(1.,1.),(1.,
1.),(1.,1.),(1.,1.),(1.,1.),(1.,1.),(1.,1.),(1.,1.),(1.,1.),(1.,1.),(1.,
1.),(1.,1.)))
REPRESENTATION_ITEM('')
SURFACE()
);
#1001=(
BOUNDED_SURFACE()
B_SPLINE_SURFACE(5,1,((#153839,#153840),(#153841,#153842),(#153843,#153844),
(#153845,#153846),(#153847,#153848),(#153849,#153850),(#153851,#153852),
(#153853,#153854),(#153855,#153856),(#153857,#153858),(#153859,#153860),
(#153861,#153862),(#153863,#153864),(#153865,#153866),(#153867,#153868),
(#153869,#153870),(#153871,#153872),(#153873,#153874),(#153875,#153876),
(#153877,#153878),(#153879,#153880),(#153881,#153882),(#153883,#153884),
(#153885,#153886),(#153887,#153888),(#153889,#153890),(#153891,#153892),
(#153893,#153894),(#153895,#153896),(#153897,#153898),(#153899,#153900),
(#153901,#153902),(#153903,#153904),(#153905,#153906),(#153907,#153908),
(#153909,#153910),(#153911,#153912),(#153913,#153914),(#153915,#153916),
(#153917,#153918),(#153919,#153920),(#153921,#153922),(#153923,#153924),
(#153925,#153926),(#153927,#153928),(#153929,#153930),(#153931,#153932),
(#153933,#153934),(#153935,#153936),(#153937,#153938),(#153939,#153940),
(#153941,#153942),(#153943,#153944),(#153945,#153946),(#153947,#153948),
(#153949,#153950),(#153951,#153952),(#153953,#153954),(#153955,#153956),
(#153957,#153958),(#153959,#153960),(#153961,#153962),(#153963,#153964),
(#153965,#153966),(#153967,#153968),(#153969,#153970),(#153971,#153972),
(#153973,#153974),(#153975,#153976),(#153977,#153978),(#153979,#153980),
(#153981,#153982),(#153983,#153984),(#153985,#153986),(#153987,#153988),
(#153989,#153990),(#153991,#153992),(#153993,#153994),(#153995,#153996),
(#153997,#153998),(#153999,#154000),(#154001,#154002),(#154003,#154004),
(#154005,#154006),(#154007,#154008),(#154009,#154010),(#154011,#154012),
(#154013,#154014),(#154015,#154016),(#154017,#154018),(#154019,#154020),
(#154021,#154022),(#154023,#154024),(#154025,#154026),(#154027,#154028),
(#154029,#154030),(#154031,#154032),(#154033,#154034),(#154035,#154036),
(#154037,#154038),(#154039,#154040),(#154041,#154042),(#154043,#154044),
(#154045,#154046),(#154047,#154048),(#154049,#154050),(#154051,#154052),
(#154053,#154054),(#154055,#154056),(#154057,#154058),(#154059,#154060),
(#154061,#154062),(#154063,#154064),(#154065,#154066),(#154067,#154068),
(#154069,#154070),(#154071,#154072),(#154073,#154074),(#154075,#154076),
(#154077,#154078),(#154079,#154080),(#154081,#154082),(#154083,#154084),
(#154085,#154086),(#154087,#154088),(#154089,#154090),(#154091,#154092),
(#154093,#154094),(#154095,#154096),(#154097,#154098),(#154099,#154100),
(#154101,#154102),(#154103,#154104),(#154105,#154106),(#154107,#154108),
(#154109,#154110),(#154111,#154112),(#154113,#154114),(#154115,#154116),
(#154117,#154118),(#154119,#154120),(#154121,#154122),(#154123,#154124),
(#154125,#154126),(#154127,#154128),(#154129,#154130),(#154131,#154132),
(#154133,#154134),(#154135,#154136),(#154137,#154138),(#154139,#154140),
(#154141,#154142),(#154143,#154144),(#154145,#154146),(#154147,#154148),
(#154149,#154150),(#154151,#154152),(#154153,#154154),(#154155,#154156),
(#154157,#154158),(#154159,#154160),(#154161,#154162),(#154163,#154164),
(#154165,#154166),(#154167,#154168),(#154169,#154170),(#154171,#154172),
(#154173,#154174),(#154175,#154176),(#154177,#154178),(#154179,#154180),
(#154181,#154182),(#154183,#154184),(#154185,#154186),(#154187,#154188),
(#154189,#154190),(#154191,#154192),(#154193,#154194),(#154195,#154196),
(#154197,#154198),(#154199,#154200),(#154201,#154202),(#154203,#154204),
(#154205,#154206),(#154207,#154208),(#154209,#154210),(#154211,#154212),
(#154213,#154214),(#154215,#154216),(#154217,#154218),(#154219,#154220),
(#154221,#154222),(#154223,#154224),(#154225,#154226),(#154227,#154228),
(#154229,#154230),(#154231,#154232),(#154233,#154234),(#154235,#154236),
(#154237,#154238),(#154239,#154240),(#154241,#154242),(#154243,#154244),
(#154245,#154246),(#154247,#154248)),.UNSPECIFIED.,.F.,.F.,.F.)
B_SPLINE_SURFACE_WITH_KNOTS((6,1,1,1,1,1,1,1,1,1,1,1,1,1,1,1,1,1,1,1,1,
1,1,1,1,1,1,1,1,1,1,1,1,1,1,1,1,1,1,1,1,1,1,1,1,1,1,1,1,1,1,1,1,1,1,1,1,
1,1,1,1,1,1,1,1,1,1,1,1,1,1,1,1,1,1,1,1,1,1,1,1,1,1,1,1,1,1,1,1,1,1,1,1,
1,1,1,1,1,1,1,1,1,1,1,1,1,1,1,1,1,1,1,1,1,1,1,1,1,1,1,1,1,1,1,1,1,1,1,1,
1,1,1,1,1,1,1,1,1,1,1,1,1,1,1,1,1,1,1,1,1,1,1,1,1,1,1,1,1,1,1,1,1,1,1,1,
1,1,1,1,1,1,1,1,1,1,1,1,1,1,1,1,1,1,1,1,1,1,1,1,1,1,1,1,1,1,1,1,1,1,1,6),
(2,2),(-1.,-0.995000000000001,-0.990000000000001,-0.985000000000001,-0.980000000000001,
-0.975000000000001,-0.970000000000001,-0.965000000000001,-0.960000000000001,
-0.955000000000001,-0.950000000000001,-0.945000000000001,-0.940000000000001,
-0.935000000000001,-0.930000000000001,-0.925000000000001,-0.920000000000001,
-0.915000000000001,-0.910000000000001,-0.905000000000001,-0.900000000000001,
-0.895000000000001,-0.890000000000001,-0.885000000000001,-0.880000000000001,
-0.875000000000001,-0.870000000000001,-0.865000000000001,-0.860000000000001,
-0.855000000000001,-0.850000000000001,-0.845000000000001,-0.840000000000001,
-0.835000000000001,-0.830000000000001,-0.825000000000001,-0.820000000000001,
-0.815000000000001,-0.810000000000001,-0.805000000000001,-0.800000000000001,
-0.795000000000001,-0.790000000000001,-0.785000000000001,-0.780000000000001,
-0.775000000000001,-0.770000000000001,-0.765000000000001,-0.760000000000001,
-0.755000000000001,-0.750000000000001,-0.745000000000001,-0.740000000000001,
-0.735000000000001,-0.730000000000001,-0.725000000000001,-0.720000000000001,
-0.715000000000001,-0.710000000000001,-0.705000000000001,-0.700000000000001,
-0.695000000000001,-0.690000000000001,-0.685,-0.68,-0.675,-0.67,-0.665,
-0.66,-0.655,-0.65,-0.645,-0.64,-0.635,-0.63,-0.625,-0.62,-0.615,-0.61,
-0.605,-0.6,-0.595,-0.59,-0.585,-0.58,-0.575,-0.57,-0.565,-0.56,-0.555,
-0.55,-0.545,-0.54,-0.535,-0.53,-0.525,-0.52,-0.515,-0.51,-0.505,-0.5,-0.495,
-0.49,-0.485,-0.48,-0.475,-0.47,-0.465,-0.46,-0.455,-0.45,-0.445,-0.44,
-0.435,-0.43,-0.425,-0.42,-0.415,-0.41,-0.405,-0.4,-0.395,-0.39,-0.385,
-0.38,-0.375,-0.37,-0.365,-0.36,-0.355,-0.35,-0.345,-0.34,-0.335,-0.33,
-0.325,-0.32,-0.315,-0.31,-0.305,-0.3,-0.295,-0.29,-0.285,-0.28,-0.275,
-0.27,-0.265,-0.26,-0.255,-0.25,-0.245,-0.24,-0.235,-0.23,-0.225,-0.22,
-0.215,-0.21,-0.205,-0.2,-0.195,-0.19,-0.185,-0.18,-0.175,-0.17,-0.165,
-0.16,-0.155,-0.15,-0.145,-0.14,-0.135,-0.13,-0.125,-0.12,-0.115,-0.11,
-0.105,-0.1,-0.095,-0.09,-0.085,-0.08,-0.075,-0.07,-0.065,-0.06,-0.055,
-0.05,-0.045,-0.04,-0.035,-0.03,-0.025,-0.02,-0.015,-0.01,-0.005,0.),(0.,
1.2),.UNSPECIFIED.)
GEOMETRIC_REPRESENTATION_ITEM()
RATIONAL_B_SPLINE_SURFACE(((1.,1.),(1.,1.),(1.,1.),(1.,1.),(1.,1.),(1.,
1.),(1.,1.),(1.,1.),(1.,1.),(1.,1.),(1.,1.),(1.,1.),(1.,1.),(1.,1.),(1.,
1.),(1.,1.),(1.,1.),(1.,1.),(1.,1.),(1.,1.),(1.,1.),(1.,1.),(1.,1.),(1.,
1.),(1.,1.),(1.,1.),(1.,1.),(1.,1.),(1.,1.),(1.,1.),(1.,1.),(1.,1.),(1.,
1.),(1.,1.),(1.,1.),(1.,1.),(1.,1.),(1.,1.),(1.,1.),(1.,1.),(1.,1.),(1.,
1.),(1.,1.),(1.,1.),(1.,1.),(1.,1.),(1.,1.),(1.,1.),(1.,1.),(1.,1.),(1.,
1.),(1.,1.),(1.,1.),(1.,1.),(1.,1.),(1.,1.),(1.,1.),(1.,1.),(1.,1.),(1.,
1.),(1.,1.),(1.,1.),(1.,1.),(1.,1.),(1.,1.),(1.,1.),(1.,1.),(1.,1.),(1.,
1.),(1.,1.),(1.,1.),(1.,1.),(1.,1.),(1.,1.),(1.,1.),(1.,1.),(1.,1.),(1.,
1.),(1.,1.),(1.,1.),(1.,1.),(1.,1.),(1.,1.),(1.,1.),(1.,1.),(1.,1.),(1.,
1.),(1.,1.),(1.,1.),(1.,1.),(1.,1.),(1.,1.),(1.,1.),(1.,1.),(1.,1.),(1.,
1.),(1.,1.),(1.,1.),(1.,1.),(1.,1.),(1.,1.),(1.,1.),(1.,1.),(1.,1.),(1.,
1.),(1.,1.),(1.,1.),(1.,1.),(1.,1.),(1.,1.),(1.,1.),(1.,1.),(1.,1.),(1.,
1.),(1.,1.),(1.,1.),(1.,1.),(1.,1.),(1.,1.),(1.,1.),(1.,1.),(1.,1.),(1.,
1.),(1.,1.),(1.,1.),(1.,1.),(1.,1.),(1.,1.),(1.,1.),(1.,1.),(1.,1.),(1.,
1.),(1.,1.),(1.,1.),(1.,1.),(1.,1.),(1.,1.),(1.,1.),(1.,1.),(1.,1.),(1.,
1.),(1.,1.),(1.,1.),(1.,1.),(1.,1.),(1.,1.),(1.,1.),(1.,1.),(1.,1.),(1.,
1.),(1.,1.),(1.,1.),(1.,1.),(1.,1.),(1.,1.),(1.,1.),(1.,1.),(1.,1.),(1.,
1.),(1.,1.),(1.,1.),(1.,1.),(1.,1.),(1.,1.),(1.,1.),(1.,1.),(1.,1.),(1.,
1.),(1.,1.),(1.,1.),(1.,1.),(1.,1.),(1.,1.),(1.,1.),(1.,1.),(1.,1.),(1.,
1.),(1.,1.),(1.,1.),(1.,1.),(1.,1.),(1.,1.),(1.,1.),(1.,1.),(1.,1.),(1.,
1.),(1.,1.),(1.,1.),(1.,1.),(1.,1.),(1.,1.),(1.,1.),(1.,1.),(1.,1.),(1.,
1.),(1.,1.),(1.,1.),(1.,1.),(1.,1.),(1.,1.),(1.,1.),(1.,1.),(1.,1.),(1.,
1.),(1.,1.)))
REPRESENTATION_ITEM('')
SURFACE()
);
#1002=(
BOUNDED_SURFACE()
B_SPLINE_SURFACE(5,1,((#154640,#154641),(#154642,#154643),(#154644,#154645),
(#154646,#154647),(#154648,#154649),(#154650,#154651),(#154652,#154653),
(#154654,#154655),(#154656,#154657),(#154658,#154659),(#154660,#154661),
(#154662,#154663),(#154664,#154665),(#154666,#154667),(#154668,#154669),
(#154670,#154671),(#154672,#154673),(#154674,#154675),(#154676,#154677),
(#154678,#154679),(#154680,#154681),(#154682,#154683),(#154684,#154685),
(#154686,#154687),(#154688,#154689),(#154690,#154691),(#154692,#154693),
(#154694,#154695),(#154696,#154697),(#154698,#154699),(#154700,#154701),
(#154702,#154703),(#154704,#154705),(#154706,#154707),(#154708,#154709),
(#154710,#154711),(#154712,#154713),(#154714,#154715),(#154716,#154717),
(#154718,#154719),(#154720,#154721),(#154722,#154723),(#154724,#154725),
(#154726,#154727),(#154728,#154729),(#154730,#154731),(#154732,#154733),
(#154734,#154735),(#154736,#154737),(#154738,#154739),(#154740,#154741),
(#154742,#154743),(#154744,#154745),(#154746,#154747),(#154748,#154749),
(#154750,#154751),(#154752,#154753),(#154754,#154755),(#154756,#154757),
(#154758,#154759),(#154760,#154761),(#154762,#154763),(#154764,#154765),
(#154766,#154767),(#154768,#154769),(#154770,#154771),(#154772,#154773),
(#154774,#154775),(#154776,#154777),(#154778,#154779),(#154780,#154781),
(#154782,#154783),(#154784,#154785),(#154786,#154787),(#154788,#154789),
(#154790,#154791),(#154792,#154793),(#154794,#154795),(#154796,#154797),
(#154798,#154799),(#154800,#154801),(#154802,#154803),(#154804,#154805),
(#154806,#154807),(#154808,#154809),(#154810,#154811),(#154812,#154813),
(#154814,#154815),(#154816,#154817),(#154818,#154819),(#154820,#154821),
(#154822,#154823),(#154824,#154825),(#154826,#154827),(#154828,#154829),
(#154830,#154831),(#154832,#154833),(#154834,#154835),(#154836,#154837),
(#154838,#154839),(#154840,#154841),(#154842,#154843),(#154844,#154845),
(#154846,#154847),(#154848,#154849),(#154850,#154851),(#154852,#154853),
(#154854,#154855),(#154856,#154857),(#154858,#154859),(#154860,#154861),
(#154862,#154863),(#154864,#154865),(#154866,#154867),(#154868,#154869),
(#154870,#154871),(#154872,#154873),(#154874,#154875),(#154876,#154877),
(#154878,#154879),(#154880,#154881),(#154882,#154883),(#154884,#154885),
(#154886,#154887),(#154888,#154889),(#154890,#154891),(#154892,#154893),
(#154894,#154895),(#154896,#154897),(#154898,#154899),(#154900,#154901),
(#154902,#154903),(#154904,#154905),(#154906,#154907),(#154908,#154909),
(#154910,#154911),(#154912,#154913),(#154914,#154915),(#154916,#154917),
(#154918,#154919),(#154920,#154921),(#154922,#154923),(#154924,#154925),
(#154926,#154927),(#154928,#154929),(#154930,#154931),(#154932,#154933),
(#154934,#154935),(#154936,#154937),(#154938,#154939),(#154940,#154941),
(#154942,#154943),(#154944,#154945),(#154946,#154947),(#154948,#154949),
(#154950,#154951),(#154952,#154953),(#154954,#154955),(#154956,#154957),
(#154958,#154959),(#154960,#154961),(#154962,#154963),(#154964,#154965),
(#154966,#154967),(#154968,#154969),(#154970,#154971),(#154972,#154973),
(#154974,#154975),(#154976,#154977),(#154978,#154979),(#154980,#154981),
(#154982,#154983),(#154984,#154985),(#154986,#154987),(#154988,#154989),
(#154990,#154991),(#154992,#154993),(#154994,#154995),(#154996,#154997),
(#154998,#154999),(#155000,#155001),(#155002,#155003),(#155004,#155005),
(#155006,#155007),(#155008,#155009),(#155010,#155011),(#155012,#155013),
(#155014,#155015),(#155016,#155017),(#155018,#155019),(#155020,#155021),
(#155022,#155023),(#155024,#155025),(#155026,#155027),(#155028,#155029),
(#155030,#155031),(#155032,#155033),(#155034,#155035),(#155036,#155037),
(#155038,#155039),(#155040,#155041),(#155042,#155043),(#155044,#155045),
(#155046,#155047),(#155048,#155049)),.UNSPECIFIED.,.F.,.F.,.F.)
B_SPLINE_SURFACE_WITH_KNOTS((6,1,1,1,1,1,1,1,1,1,1,1,1,1,1,1,1,1,1,1,1,
1,1,1,1,1,1,1,1,1,1,1,1,1,1,1,1,1,1,1,1,1,1,1,1,1,1,1,1,1,1,1,1,1,1,1,1,
1,1,1,1,1,1,1,1,1,1,1,1,1,1,1,1,1,1,1,1,1,1,1,1,1,1,1,1,1,1,1,1,1,1,1,1,
1,1,1,1,1,1,1,1,1,1,1,1,1,1,1,1,1,1,1,1,1,1,1,1,1,1,1,1,1,1,1,1,1,1,1,1,
1,1,1,1,1,1,1,1,1,1,1,1,1,1,1,1,1,1,1,1,1,1,1,1,1,1,1,1,1,1,1,1,1,1,1,1,
1,1,1,1,1,1,1,1,1,1,1,1,1,1,1,1,1,1,1,1,1,1,1,1,1,1,1,1,1,1,1,1,1,1,1,6),
(2,2),(-1.,-0.995000000000001,-0.990000000000001,-0.985000000000001,-0.980000000000001,
-0.975000000000001,-0.970000000000001,-0.965000000000001,-0.960000000000001,
-0.955000000000001,-0.950000000000001,-0.945000000000001,-0.940000000000001,
-0.935000000000001,-0.930000000000001,-0.925000000000001,-0.920000000000001,
-0.915000000000001,-0.910000000000001,-0.905000000000001,-0.900000000000001,
-0.895000000000001,-0.890000000000001,-0.885000000000001,-0.880000000000001,
-0.875000000000001,-0.870000000000001,-0.865000000000001,-0.860000000000001,
-0.855000000000001,-0.850000000000001,-0.845000000000001,-0.840000000000001,
-0.835000000000001,-0.830000000000001,-0.825000000000001,-0.820000000000001,
-0.815000000000001,-0.810000000000001,-0.805000000000001,-0.800000000000001,
-0.795000000000001,-0.790000000000001,-0.785000000000001,-0.780000000000001,
-0.775000000000001,-0.770000000000001,-0.765000000000001,-0.760000000000001,
-0.755000000000001,-0.750000000000001,-0.745000000000001,-0.740000000000001,
-0.735000000000001,-0.730000000000001,-0.725000000000001,-0.720000000000001,
-0.715000000000001,-0.710000000000001,-0.705000000000001,-0.700000000000001,
-0.695000000000001,-0.690000000000001,-0.685,-0.68,-0.675,-0.67,-0.665,
-0.66,-0.655,-0.65,-0.645,-0.64,-0.635,-0.63,-0.625,-0.62,-0.615,-0.61,
-0.605,-0.6,-0.595,-0.59,-0.585,-0.58,-0.575,-0.57,-0.565,-0.56,-0.555,
-0.55,-0.545,-0.54,-0.535,-0.53,-0.525,-0.52,-0.515,-0.51,-0.505,-0.5,-0.495,
-0.49,-0.485,-0.48,-0.475,-0.47,-0.465,-0.46,-0.455,-0.45,-0.445,-0.44,
-0.435,-0.43,-0.425,-0.42,-0.415,-0.41,-0.405,-0.4,-0.395,-0.39,-0.385,
-0.38,-0.375,-0.37,-0.365,-0.36,-0.355,-0.35,-0.345,-0.34,-0.335,-0.33,
-0.325,-0.32,-0.315,-0.31,-0.305,-0.3,-0.295,-0.29,-0.285,-0.28,-0.275,
-0.27,-0.265,-0.26,-0.255,-0.25,-0.245,-0.24,-0.235,-0.23,-0.225,-0.22,
-0.215,-0.21,-0.205,-0.2,-0.195,-0.19,-0.185,-0.18,-0.175,-0.17,-0.165,
-0.16,-0.155,-0.15,-0.145,-0.14,-0.135,-0.13,-0.125,-0.12,-0.115,-0.11,
-0.105,-0.1,-0.095,-0.09,-0.085,-0.08,-0.075,-0.07,-0.065,-0.06,-0.055,
-0.05,-0.045,-0.04,-0.035,-0.03,-0.025,-0.02,-0.015,-0.01,-0.005,0.),(0.,
1.2),.UNSPECIFIED.)
GEOMETRIC_REPRESENTATION_ITEM()
RATIONAL_B_SPLINE_SURFACE(((1.,1.),(1.,1.),(1.,1.),(1.,1.),(1.,1.),(1.,
1.),(1.,1.),(1.,1.),(1.,1.),(1.,1.),(1.,1.),(1.,1.),(1.,1.),(1.,1.),(1.,
1.),(1.,1.),(1.,1.),(1.,1.),(1.,1.),(1.,1.),(1.,1.),(1.,1.),(1.,1.),(1.,
1.),(1.,1.),(1.,1.),(1.,1.),(1.,1.),(1.,1.),(1.,1.),(1.,1.),(1.,1.),(1.,
1.),(1.,1.),(1.,1.),(1.,1.),(1.,1.),(1.,1.),(1.,1.),(1.,1.),(1.,1.),(1.,
1.),(1.,1.),(1.,1.),(1.,1.),(1.,1.),(1.,1.),(1.,1.),(1.,1.),(1.,1.),(1.,
1.),(1.,1.),(1.,1.),(1.,1.),(1.,1.),(1.,1.),(1.,1.),(1.,1.),(1.,1.),(1.,
1.),(1.,1.),(1.,1.),(1.,1.),(1.,1.),(1.,1.),(1.,1.),(1.,1.),(1.,1.),(1.,
1.),(1.,1.),(1.,1.),(1.,1.),(1.,1.),(1.,1.),(1.,1.),(1.,1.),(1.,1.),(1.,
1.),(1.,1.),(1.,1.),(1.,1.),(1.,1.),(1.,1.),(1.,1.),(1.,1.),(1.,1.),(1.,
1.),(1.,1.),(1.,1.),(1.,1.),(1.,1.),(1.,1.),(1.,1.),(1.,1.),(1.,1.),(1.,
1.),(1.,1.),(1.,1.),(1.,1.),(1.,1.),(1.,1.),(1.,1.),(1.,1.),(1.,1.),(1.,
1.),(1.,1.),(1.,1.),(1.,1.),(1.,1.),(1.,1.),(1.,1.),(1.,1.),(1.,1.),(1.,
1.),(1.,1.),(1.,1.),(1.,1.),(1.,1.),(1.,1.),(1.,1.),(1.,1.),(1.,1.),(1.,
1.),(1.,1.),(1.,1.),(1.,1.),(1.,1.),(1.,1.),(1.,1.),(1.,1.),(1.,1.),(1.,
1.),(1.,1.),(1.,1.),(1.,1.),(1.,1.),(1.,1.),(1.,1.),(1.,1.),(1.,1.),(1.,
1.),(1.,1.),(1.,1.),(1.,1.),(1.,1.),(1.,1.),(1.,1.),(1.,1.),(1.,1.),(1.,
1.),(1.,1.),(1.,1.),(1.,1.),(1.,1.),(1.,1.),(1.,1.),(1.,1.),(1.,1.),(1.,
1.),(1.,1.),(1.,1.),(1.,1.),(1.,1.),(1.,1.),(1.,1.),(1.,1.),(1.,1.),(1.,
1.),(1.,1.),(1.,1.),(1.,1.),(1.,1.),(1.,1.),(1.,1.),(1.,1.),(1.,1.),(1.,
1.),(1.,1.),(1.,1.),(1.,1.),(1.,1.),(1.,1.),(1.,1.),(1.,1.),(1.,1.),(1.,
1.),(1.,1.),(1.,1.),(1.,1.),(1.,1.),(1.,1.),(1.,1.),(1.,1.),(1.,1.),(1.,
1.),(1.,1.),(1.,1.),(1.,1.),(1.,1.),(1.,1.),(1.,1.),(1.,1.),(1.,1.),(1.,
1.),(1.,1.)))
REPRESENTATION_ITEM('')
SURFACE()
);
#1003=(
BOUNDED_SURFACE()
B_SPLINE_SURFACE(5,1,((#155441,#155442),(#155443,#155444),(#155445,#155446),
(#155447,#155448),(#155449,#155450),(#155451,#155452),(#155453,#155454),
(#155455,#155456),(#155457,#155458),(#155459,#155460),(#155461,#155462),
(#155463,#155464),(#155465,#155466),(#155467,#155468),(#155469,#155470),
(#155471,#155472),(#155473,#155474),(#155475,#155476),(#155477,#155478),
(#155479,#155480),(#155481,#155482),(#155483,#155484),(#155485,#155486),
(#155487,#155488),(#155489,#155490),(#155491,#155492),(#155493,#155494),
(#155495,#155496),(#155497,#155498),(#155499,#155500),(#155501,#155502),
(#155503,#155504),(#155505,#155506),(#155507,#155508),(#155509,#155510),
(#155511,#155512),(#155513,#155514),(#155515,#155516),(#155517,#155518),
(#155519,#155520),(#155521,#155522),(#155523,#155524),(#155525,#155526),
(#155527,#155528),(#155529,#155530),(#155531,#155532),(#155533,#155534),
(#155535,#155536),(#155537,#155538),(#155539,#155540),(#155541,#155542),
(#155543,#155544),(#155545,#155546),(#155547,#155548),(#155549,#155550),
(#155551,#155552),(#155553,#155554),(#155555,#155556),(#155557,#155558),
(#155559,#155560),(#155561,#155562),(#155563,#155564),(#155565,#155566),
(#155567,#155568),(#155569,#155570),(#155571,#155572),(#155573,#155574),
(#155575,#155576),(#155577,#155578),(#155579,#155580),(#155581,#155582),
(#155583,#155584),(#155585,#155586),(#155587,#155588),(#155589,#155590),
(#155591,#155592),(#155593,#155594),(#155595,#155596),(#155597,#155598),
(#155599,#155600),(#155601,#155602),(#155603,#155604),(#155605,#155606),
(#155607,#155608),(#155609,#155610),(#155611,#155612),(#155613,#155614),
(#155615,#155616),(#155617,#155618),(#155619,#155620),(#155621,#155622),
(#155623,#155624),(#155625,#155626),(#155627,#155628),(#155629,#155630),
(#155631,#155632),(#155633,#155634),(#155635,#155636),(#155637,#155638),
(#155639,#155640),(#155641,#155642),(#155643,#155644),(#155645,#155646),
(#155647,#155648),(#155649,#155650),(#155651,#155652),(#155653,#155654),
(#155655,#155656),(#155657,#155658),(#155659,#155660),(#155661,#155662),
(#155663,#155664),(#155665,#155666),(#155667,#155668),(#155669,#155670),
(#155671,#155672),(#155673,#155674),(#155675,#155676),(#155677,#155678),
(#155679,#155680),(#155681,#155682),(#155683,#155684),(#155685,#155686),
(#155687,#155688),(#155689,#155690),(#155691,#155692),(#155693,#155694),
(#155695,#155696),(#155697,#155698),(#155699,#155700),(#155701,#155702),
(#155703,#155704),(#155705,#155706),(#155707,#155708),(#155709,#155710),
(#155711,#155712),(#155713,#155714),(#155715,#155716),(#155717,#155718),
(#155719,#155720),(#155721,#155722),(#155723,#155724),(#155725,#155726),
(#155727,#155728),(#155729,#155730),(#155731,#155732),(#155733,#155734),
(#155735,#155736),(#155737,#155738),(#155739,#155740),(#155741,#155742),
(#155743,#155744),(#155745,#155746),(#155747,#155748),(#155749,#155750),
(#155751,#155752),(#155753,#155754),(#155755,#155756),(#155757,#155758),
(#155759,#155760),(#155761,#155762),(#155763,#155764),(#155765,#155766),
(#155767,#155768),(#155769,#155770),(#155771,#155772),(#155773,#155774),
(#155775,#155776),(#155777,#155778),(#155779,#155780),(#155781,#155782),
(#155783,#155784),(#155785,#155786),(#155787,#155788),(#155789,#155790),
(#155791,#155792),(#155793,#155794),(#155795,#155796),(#155797,#155798),
(#155799,#155800),(#155801,#155802),(#155803,#155804),(#155805,#155806),
(#155807,#155808),(#155809,#155810),(#155811,#155812),(#155813,#155814),
(#155815,#155816),(#155817,#155818),(#155819,#155820),(#155821,#155822),
(#155823,#155824),(#155825,#155826),(#155827,#155828),(#155829,#155830),
(#155831,#155832),(#155833,#155834),(#155835,#155836),(#155837,#155838),
(#155839,#155840),(#155841,#155842),(#155843,#155844),(#155845,#155846),
(#155847,#155848),(#155849,#155850)),.UNSPECIFIED.,.F.,.F.,.F.)
B_SPLINE_SURFACE_WITH_KNOTS((6,1,1,1,1,1,1,1,1,1,1,1,1,1,1,1,1,1,1,1,1,
1,1,1,1,1,1,1,1,1,1,1,1,1,1,1,1,1,1,1,1,1,1,1,1,1,1,1,1,1,1,1,1,1,1,1,1,
1,1,1,1,1,1,1,1,1,1,1,1,1,1,1,1,1,1,1,1,1,1,1,1,1,1,1,1,1,1,1,1,1,1,1,1,
1,1,1,1,1,1,1,1,1,1,1,1,1,1,1,1,1,1,1,1,1,1,1,1,1,1,1,1,1,1,1,1,1,1,1,1,
1,1,1,1,1,1,1,1,1,1,1,1,1,1,1,1,1,1,1,1,1,1,1,1,1,1,1,1,1,1,1,1,1,1,1,1,
1,1,1,1,1,1,1,1,1,1,1,1,1,1,1,1,1,1,1,1,1,1,1,1,1,1,1,1,1,1,1,1,1,1,1,6),
(2,2),(-1.,-0.995000000000001,-0.990000000000001,-0.985000000000001,-0.980000000000001,
-0.975000000000001,-0.970000000000001,-0.965000000000001,-0.960000000000001,
-0.955000000000001,-0.950000000000001,-0.945000000000001,-0.940000000000001,
-0.935000000000001,-0.930000000000001,-0.925000000000001,-0.920000000000001,
-0.915000000000001,-0.910000000000001,-0.905000000000001,-0.900000000000001,
-0.895000000000001,-0.890000000000001,-0.885000000000001,-0.880000000000001,
-0.875000000000001,-0.870000000000001,-0.865000000000001,-0.860000000000001,
-0.855000000000001,-0.850000000000001,-0.845000000000001,-0.840000000000001,
-0.835000000000001,-0.830000000000001,-0.825000000000001,-0.820000000000001,
-0.815000000000001,-0.810000000000001,-0.805000000000001,-0.800000000000001,
-0.795000000000001,-0.790000000000001,-0.785000000000001,-0.780000000000001,
-0.775000000000001,-0.770000000000001,-0.765000000000001,-0.760000000000001,
-0.755000000000001,-0.750000000000001,-0.745000000000001,-0.740000000000001,
-0.735000000000001,-0.730000000000001,-0.725000000000001,-0.720000000000001,
-0.715000000000001,-0.710000000000001,-0.705000000000001,-0.700000000000001,
-0.695000000000001,-0.690000000000001,-0.685,-0.68,-0.675,-0.67,-0.665,
-0.66,-0.655,-0.65,-0.645,-0.64,-0.635,-0.63,-0.625,-0.62,-0.615,-0.61,
-0.605,-0.6,-0.595,-0.59,-0.585,-0.58,-0.575,-0.57,-0.565,-0.56,-0.555,
-0.55,-0.545,-0.54,-0.535,-0.53,-0.525,-0.52,-0.515,-0.51,-0.505,-0.5,-0.495,
-0.49,-0.485,-0.48,-0.475,-0.47,-0.465,-0.46,-0.455,-0.45,-0.445,-0.44,
-0.435,-0.43,-0.425,-0.42,-0.415,-0.41,-0.405,-0.4,-0.395,-0.39,-0.385,
-0.38,-0.375,-0.37,-0.365,-0.36,-0.355,-0.35,-0.345,-0.34,-0.335,-0.33,
-0.325,-0.32,-0.315,-0.31,-0.305,-0.3,-0.295,-0.29,-0.285,-0.28,-0.275,
-0.27,-0.265,-0.26,-0.255,-0.25,-0.245,-0.24,-0.235,-0.23,-0.225,-0.22,
-0.215,-0.21,-0.205,-0.2,-0.195,-0.19,-0.185,-0.18,-0.175,-0.17,-0.165,
-0.16,-0.155,-0.15,-0.145,-0.14,-0.135,-0.13,-0.125,-0.12,-0.115,-0.11,
-0.105,-0.1,-0.095,-0.09,-0.085,-0.08,-0.075,-0.07,-0.065,-0.06,-0.055,
-0.05,-0.045,-0.04,-0.035,-0.03,-0.025,-0.02,-0.015,-0.01,-0.005,0.),(0.,
1.2),.UNSPECIFIED.)
GEOMETRIC_REPRESENTATION_ITEM()
RATIONAL_B_SPLINE_SURFACE(((1.,1.),(1.,1.),(1.,1.),(1.,1.),(1.,1.),(1.,
1.),(1.,1.),(1.,1.),(1.,1.),(1.,1.),(1.,1.),(1.,1.),(1.,1.),(1.,1.),(1.,
1.),(1.,1.),(1.,1.),(1.,1.),(1.,1.),(1.,1.),(1.,1.),(1.,1.),(1.,1.),(1.,
1.),(1.,1.),(1.,1.),(1.,1.),(1.,1.),(1.,1.),(1.,1.),(1.,1.),(1.,1.),(1.,
1.),(1.,1.),(1.,1.),(1.,1.),(1.,1.),(1.,1.),(1.,1.),(1.,1.),(1.,1.),(1.,
1.),(1.,1.),(1.,1.),(1.,1.),(1.,1.),(1.,1.),(1.,1.),(1.,1.),(1.,1.),(1.,
1.),(1.,1.),(1.,1.),(1.,1.),(1.,1.),(1.,1.),(1.,1.),(1.,1.),(1.,1.),(1.,
1.),(1.,1.),(1.,1.),(1.,1.),(1.,1.),(1.,1.),(1.,1.),(1.,1.),(1.,1.),(1.,
1.),(1.,1.),(1.,1.),(1.,1.),(1.,1.),(1.,1.),(1.,1.),(1.,1.),(1.,1.),(1.,
1.),(1.,1.),(1.,1.),(1.,1.),(1.,1.),(1.,1.),(1.,1.),(1.,1.),(1.,1.),(1.,
1.),(1.,1.),(1.,1.),(1.,1.),(1.,1.),(1.,1.),(1.,1.),(1.,1.),(1.,1.),(1.,
1.),(1.,1.),(1.,1.),(1.,1.),(1.,1.),(1.,1.),(1.,1.),(1.,1.),(1.,1.),(1.,
1.),(1.,1.),(1.,1.),(1.,1.),(1.,1.),(1.,1.),(1.,1.),(1.,1.),(1.,1.),(1.,
1.),(1.,1.),(1.,1.),(1.,1.),(1.,1.),(1.,1.),(1.,1.),(1.,1.),(1.,1.),(1.,
1.),(1.,1.),(1.,1.),(1.,1.),(1.,1.),(1.,1.),(1.,1.),(1.,1.),(1.,1.),(1.,
1.),(1.,1.),(1.,1.),(1.,1.),(1.,1.),(1.,1.),(1.,1.),(1.,1.),(1.,1.),(1.,
1.),(1.,1.),(1.,1.),(1.,1.),(1.,1.),(1.,1.),(1.,1.),(1.,1.),(1.,1.),(1.,
1.),(1.,1.),(1.,1.),(1.,1.),(1.,1.),(1.,1.),(1.,1.),(1.,1.),(1.,1.),(1.,
1.),(1.,1.),(1.,1.),(1.,1.),(1.,1.),(1.,1.),(1.,1.),(1.,1.),(1.,1.),(1.,
1.),(1.,1.),(1.,1.),(1.,1.),(1.,1.),(1.,1.),(1.,1.),(1.,1.),(1.,1.),(1.,
1.),(1.,1.),(1.,1.),(1.,1.),(1.,1.),(1.,1.),(1.,1.),(1.,1.),(1.,1.),(1.,
1.),(1.,1.),(1.,1.),(1.,1.),(1.,1.),(1.,1.),(1.,1.),(1.,1.),(1.,1.),(1.,
1.),(1.,1.),(1.,1.),(1.,1.),(1.,1.),(1.,1.),(1.,1.),(1.,1.),(1.,1.),(1.,
1.),(1.,1.)))
REPRESENTATION_ITEM('')
SURFACE()
);
#1004=(
BOUNDED_SURFACE()
B_SPLINE_SURFACE(5,1,((#156242,#156243),(#156244,#156245),(#156246,#156247),
(#156248,#156249),(#156250,#156251),(#156252,#156253),(#156254,#156255),
(#156256,#156257),(#156258,#156259),(#156260,#156261),(#156262,#156263),
(#156264,#156265),(#156266,#156267),(#156268,#156269),(#156270,#156271),
(#156272,#156273),(#156274,#156275),(#156276,#156277),(#156278,#156279),
(#156280,#156281),(#156282,#156283),(#156284,#156285),(#156286,#156287),
(#156288,#156289),(#156290,#156291),(#156292,#156293),(#156294,#156295),
(#156296,#156297),(#156298,#156299),(#156300,#156301),(#156302,#156303),
(#156304,#156305),(#156306,#156307),(#156308,#156309),(#156310,#156311),
(#156312,#156313),(#156314,#156315),(#156316,#156317),(#156318,#156319),
(#156320,#156321),(#156322,#156323),(#156324,#156325),(#156326,#156327),
(#156328,#156329),(#156330,#156331),(#156332,#156333),(#156334,#156335),
(#156336,#156337),(#156338,#156339),(#156340,#156341),(#156342,#156343),
(#156344,#156345),(#156346,#156347),(#156348,#156349),(#156350,#156351),
(#156352,#156353),(#156354,#156355),(#156356,#156357),(#156358,#156359),
(#156360,#156361),(#156362,#156363),(#156364,#156365),(#156366,#156367),
(#156368,#156369),(#156370,#156371),(#156372,#156373),(#156374,#156375),
(#156376,#156377),(#156378,#156379),(#156380,#156381),(#156382,#156383),
(#156384,#156385),(#156386,#156387),(#156388,#156389),(#156390,#156391),
(#156392,#156393),(#156394,#156395),(#156396,#156397),(#156398,#156399),
(#156400,#156401),(#156402,#156403),(#156404,#156405),(#156406,#156407),
(#156408,#156409),(#156410,#156411),(#156412,#156413),(#156414,#156415),
(#156416,#156417),(#156418,#156419),(#156420,#156421),(#156422,#156423),
(#156424,#156425),(#156426,#156427),(#156428,#156429),(#156430,#156431),
(#156432,#156433),(#156434,#156435),(#156436,#156437),(#156438,#156439),
(#156440,#156441),(#156442,#156443),(#156444,#156445),(#156446,#156447),
(#156448,#156449),(#156450,#156451),(#156452,#156453),(#156454,#156455),
(#156456,#156457),(#156458,#156459),(#156460,#156461),(#156462,#156463),
(#156464,#156465),(#156466,#156467),(#156468,#156469),(#156470,#156471),
(#156472,#156473),(#156474,#156475),(#156476,#156477),(#156478,#156479),
(#156480,#156481),(#156482,#156483),(#156484,#156485),(#156486,#156487),
(#156488,#156489),(#156490,#156491),(#156492,#156493),(#156494,#156495),
(#156496,#156497),(#156498,#156499),(#156500,#156501),(#156502,#156503),
(#156504,#156505),(#156506,#156507),(#156508,#156509),(#156510,#156511),
(#156512,#156513),(#156514,#156515),(#156516,#156517),(#156518,#156519),
(#156520,#156521),(#156522,#156523),(#156524,#156525),(#156526,#156527),
(#156528,#156529),(#156530,#156531),(#156532,#156533),(#156534,#156535),
(#156536,#156537),(#156538,#156539),(#156540,#156541),(#156542,#156543),
(#156544,#156545),(#156546,#156547),(#156548,#156549),(#156550,#156551),
(#156552,#156553),(#156554,#156555),(#156556,#156557),(#156558,#156559),
(#156560,#156561),(#156562,#156563),(#156564,#156565),(#156566,#156567),
(#156568,#156569),(#156570,#156571),(#156572,#156573),(#156574,#156575),
(#156576,#156577),(#156578,#156579),(#156580,#156581),(#156582,#156583),
(#156584,#156585),(#156586,#156587),(#156588,#156589),(#156590,#156591),
(#156592,#156593),(#156594,#156595),(#156596,#156597),(#156598,#156599),
(#156600,#156601),(#156602,#156603),(#156604,#156605),(#156606,#156607),
(#156608,#156609),(#156610,#156611),(#156612,#156613),(#156614,#156615),
(#156616,#156617),(#156618,#156619),(#156620,#156621),(#156622,#156623),
(#156624,#156625),(#156626,#156627),(#156628,#156629),(#156630,#156631),
(#156632,#156633),(#156634,#156635),(#156636,#156637),(#156638,#156639),
(#156640,#156641),(#156642,#156643),(#156644,#156645),(#156646,#156647),
(#156648,#156649),(#156650,#156651)),.UNSPECIFIED.,.F.,.F.,.F.)
B_SPLINE_SURFACE_WITH_KNOTS((6,1,1,1,1,1,1,1,1,1,1,1,1,1,1,1,1,1,1,1,1,
1,1,1,1,1,1,1,1,1,1,1,1,1,1,1,1,1,1,1,1,1,1,1,1,1,1,1,1,1,1,1,1,1,1,1,1,
1,1,1,1,1,1,1,1,1,1,1,1,1,1,1,1,1,1,1,1,1,1,1,1,1,1,1,1,1,1,1,1,1,1,1,1,
1,1,1,1,1,1,1,1,1,1,1,1,1,1,1,1,1,1,1,1,1,1,1,1,1,1,1,1,1,1,1,1,1,1,1,1,
1,1,1,1,1,1,1,1,1,1,1,1,1,1,1,1,1,1,1,1,1,1,1,1,1,1,1,1,1,1,1,1,1,1,1,1,
1,1,1,1,1,1,1,1,1,1,1,1,1,1,1,1,1,1,1,1,1,1,1,1,1,1,1,1,1,1,1,1,1,1,1,6),
(2,2),(-1.,-0.995000000000001,-0.990000000000001,-0.985000000000001,-0.980000000000001,
-0.975000000000001,-0.970000000000001,-0.965000000000001,-0.960000000000001,
-0.955000000000001,-0.950000000000001,-0.945000000000001,-0.940000000000001,
-0.935000000000001,-0.930000000000001,-0.925000000000001,-0.920000000000001,
-0.915000000000001,-0.910000000000001,-0.905000000000001,-0.900000000000001,
-0.895000000000001,-0.890000000000001,-0.885000000000001,-0.880000000000001,
-0.875000000000001,-0.870000000000001,-0.865000000000001,-0.860000000000001,
-0.855000000000001,-0.850000000000001,-0.845000000000001,-0.840000000000001,
-0.835000000000001,-0.830000000000001,-0.825000000000001,-0.820000000000001,
-0.815000000000001,-0.810000000000001,-0.805000000000001,-0.800000000000001,
-0.795000000000001,-0.790000000000001,-0.785000000000001,-0.780000000000001,
-0.775000000000001,-0.770000000000001,-0.765000000000001,-0.760000000000001,
-0.755000000000001,-0.750000000000001,-0.745000000000001,-0.740000000000001,
-0.735000000000001,-0.730000000000001,-0.725000000000001,-0.720000000000001,
-0.715000000000001,-0.710000000000001,-0.705000000000001,-0.700000000000001,
-0.695000000000001,-0.690000000000001,-0.685,-0.68,-0.675,-0.67,-0.665,
-0.66,-0.655,-0.65,-0.645,-0.64,-0.635,-0.63,-0.625,-0.62,-0.615,-0.61,
-0.605,-0.6,-0.595,-0.59,-0.585,-0.58,-0.575,-0.57,-0.565,-0.56,-0.555,
-0.55,-0.545,-0.54,-0.535,-0.53,-0.525,-0.52,-0.515,-0.51,-0.505,-0.5,-0.495,
-0.49,-0.485,-0.48,-0.475,-0.47,-0.465,-0.46,-0.455,-0.45,-0.445,-0.44,
-0.435,-0.43,-0.425,-0.42,-0.415,-0.41,-0.405,-0.4,-0.395,-0.39,-0.385,
-0.38,-0.375,-0.37,-0.365,-0.36,-0.355,-0.35,-0.345,-0.34,-0.335,-0.33,
-0.325,-0.32,-0.315,-0.31,-0.305,-0.3,-0.295,-0.29,-0.285,-0.28,-0.275,
-0.27,-0.265,-0.26,-0.255,-0.25,-0.245,-0.24,-0.235,-0.23,-0.225,-0.22,
-0.215,-0.21,-0.205,-0.2,-0.195,-0.19,-0.185,-0.18,-0.175,-0.17,-0.165,
-0.16,-0.155,-0.15,-0.145,-0.14,-0.135,-0.13,-0.125,-0.12,-0.115,-0.11,
-0.105,-0.1,-0.095,-0.09,-0.085,-0.08,-0.075,-0.07,-0.065,-0.06,-0.055,
-0.05,-0.045,-0.04,-0.035,-0.03,-0.025,-0.02,-0.015,-0.01,-0.005,0.),(0.,
1.2),.UNSPECIFIED.)
GEOMETRIC_REPRESENTATION_ITEM()
RATIONAL_B_SPLINE_SURFACE(((1.,1.),(1.,1.),(1.,1.),(1.,1.),(1.,1.),(1.,
1.),(1.,1.),(1.,1.),(1.,1.),(1.,1.),(1.,1.),(1.,1.),(1.,1.),(1.,1.),(1.,
1.),(1.,1.),(1.,1.),(1.,1.),(1.,1.),(1.,1.),(1.,1.),(1.,1.),(1.,1.),(1.,
1.),(1.,1.),(1.,1.),(1.,1.),(1.,1.),(1.,1.),(1.,1.),(1.,1.),(1.,1.),(1.,
1.),(1.,1.),(1.,1.),(1.,1.),(1.,1.),(1.,1.),(1.,1.),(1.,1.),(1.,1.),(1.,
1.),(1.,1.),(1.,1.),(1.,1.),(1.,1.),(1.,1.),(1.,1.),(1.,1.),(1.,1.),(1.,
1.),(1.,1.),(1.,1.),(1.,1.),(1.,1.),(1.,1.),(1.,1.),(1.,1.),(1.,1.),(1.,
1.),(1.,1.),(1.,1.),(1.,1.),(1.,1.),(1.,1.),(1.,1.),(1.,1.),(1.,1.),(1.,
1.),(1.,1.),(1.,1.),(1.,1.),(1.,1.),(1.,1.),(1.,1.),(1.,1.),(1.,1.),(1.,
1.),(1.,1.),(1.,1.),(1.,1.),(1.,1.),(1.,1.),(1.,1.),(1.,1.),(1.,1.),(1.,
1.),(1.,1.),(1.,1.),(1.,1.),(1.,1.),(1.,1.),(1.,1.),(1.,1.),(1.,1.),(1.,
1.),(1.,1.),(1.,1.),(1.,1.),(1.,1.),(1.,1.),(1.,1.),(1.,1.),(1.,1.),(1.,
1.),(1.,1.),(1.,1.),(1.,1.),(1.,1.),(1.,1.),(1.,1.),(1.,1.),(1.,1.),(1.,
1.),(1.,1.),(1.,1.),(1.,1.),(1.,1.),(1.,1.),(1.,1.),(1.,1.),(1.,1.),(1.,
1.),(1.,1.),(1.,1.),(1.,1.),(1.,1.),(1.,1.),(1.,1.),(1.,1.),(1.,1.),(1.,
1.),(1.,1.),(1.,1.),(1.,1.),(1.,1.),(1.,1.),(1.,1.),(1.,1.),(1.,1.),(1.,
1.),(1.,1.),(1.,1.),(1.,1.),(1.,1.),(1.,1.),(1.,1.),(1.,1.),(1.,1.),(1.,
1.),(1.,1.),(1.,1.),(1.,1.),(1.,1.),(1.,1.),(1.,1.),(1.,1.),(1.,1.),(1.,
1.),(1.,1.),(1.,1.),(1.,1.),(1.,1.),(1.,1.),(1.,1.),(1.,1.),(1.,1.),(1.,
1.),(1.,1.),(1.,1.),(1.,1.),(1.,1.),(1.,1.),(1.,1.),(1.,1.),(1.,1.),(1.,
1.),(1.,1.),(1.,1.),(1.,1.),(1.,1.),(1.,1.),(1.,1.),(1.,1.),(1.,1.),(1.,
1.),(1.,1.),(1.,1.),(1.,1.),(1.,1.),(1.,1.),(1.,1.),(1.,1.),(1.,1.),(1.,
1.),(1.,1.),(1.,1.),(1.,1.),(1.,1.),(1.,1.),(1.,1.),(1.,1.),(1.,1.),(1.,
1.),(1.,1.)))
REPRESENTATION_ITEM('')
SURFACE()
);
#1005=(
BOUNDED_SURFACE()
B_SPLINE_SURFACE(5,1,((#157043,#157044),(#157045,#157046),(#157047,#157048),
(#157049,#157050),(#157051,#157052),(#157053,#157054),(#157055,#157056),
(#157057,#157058),(#157059,#157060),(#157061,#157062),(#157063,#157064),
(#157065,#157066),(#157067,#157068),(#157069,#157070),(#157071,#157072),
(#157073,#157074),(#157075,#157076),(#157077,#157078),(#157079,#157080),
(#157081,#157082),(#157083,#157084),(#157085,#157086),(#157087,#157088),
(#157089,#157090),(#157091,#157092),(#157093,#157094),(#157095,#157096),
(#157097,#157098),(#157099,#157100),(#157101,#157102),(#157103,#157104),
(#157105,#157106),(#157107,#157108),(#157109,#157110),(#157111,#157112),
(#157113,#157114),(#157115,#157116),(#157117,#157118),(#157119,#157120),
(#157121,#157122),(#157123,#157124),(#157125,#157126),(#157127,#157128),
(#157129,#157130),(#157131,#157132),(#157133,#157134),(#157135,#157136),
(#157137,#157138),(#157139,#157140),(#157141,#157142),(#157143,#157144),
(#157145,#157146),(#157147,#157148),(#157149,#157150),(#157151,#157152),
(#157153,#157154),(#157155,#157156),(#157157,#157158),(#157159,#157160),
(#157161,#157162),(#157163,#157164),(#157165,#157166),(#157167,#157168),
(#157169,#157170),(#157171,#157172),(#157173,#157174),(#157175,#157176),
(#157177,#157178),(#157179,#157180),(#157181,#157182),(#157183,#157184),
(#157185,#157186),(#157187,#157188),(#157189,#157190),(#157191,#157192),
(#157193,#157194),(#157195,#157196),(#157197,#157198),(#157199,#157200),
(#157201,#157202),(#157203,#157204),(#157205,#157206),(#157207,#157208),
(#157209,#157210),(#157211,#157212),(#157213,#157214),(#157215,#157216),
(#157217,#157218),(#157219,#157220),(#157221,#157222),(#157223,#157224),
(#157225,#157226),(#157227,#157228),(#157229,#157230),(#157231,#157232),
(#157233,#157234),(#157235,#157236),(#157237,#157238),(#157239,#157240),
(#157241,#157242),(#157243,#157244),(#157245,#157246),(#157247,#157248),
(#157249,#157250),(#157251,#157252),(#157253,#157254),(#157255,#157256),
(#157257,#157258),(#157259,#157260),(#157261,#157262),(#157263,#157264),
(#157265,#157266),(#157267,#157268),(#157269,#157270),(#157271,#157272),
(#157273,#157274),(#157275,#157276),(#157277,#157278),(#157279,#157280),
(#157281,#157282),(#157283,#157284),(#157285,#157286),(#157287,#157288),
(#157289,#157290),(#157291,#157292),(#157293,#157294),(#157295,#157296),
(#157297,#157298),(#157299,#157300),(#157301,#157302),(#157303,#157304),
(#157305,#157306),(#157307,#157308),(#157309,#157310),(#157311,#157312),
(#157313,#157314),(#157315,#157316),(#157317,#157318),(#157319,#157320),
(#157321,#157322),(#157323,#157324),(#157325,#157326),(#157327,#157328),
(#157329,#157330),(#157331,#157332),(#157333,#157334),(#157335,#157336),
(#157337,#157338),(#157339,#157340),(#157341,#157342),(#157343,#157344),
(#157345,#157346),(#157347,#157348),(#157349,#157350),(#157351,#157352),
(#157353,#157354),(#157355,#157356),(#157357,#157358),(#157359,#157360),
(#157361,#157362),(#157363,#157364),(#157365,#157366),(#157367,#157368),
(#157369,#157370),(#157371,#157372),(#157373,#157374),(#157375,#157376),
(#157377,#157378),(#157379,#157380),(#157381,#157382),(#157383,#157384),
(#157385,#157386),(#157387,#157388),(#157389,#157390),(#157391,#157392),
(#157393,#157394),(#157395,#157396),(#157397,#157398),(#157399,#157400),
(#157401,#157402),(#157403,#157404),(#157405,#157406),(#157407,#157408),
(#157409,#157410),(#157411,#157412),(#157413,#157414),(#157415,#157416),
(#157417,#157418),(#157419,#157420),(#157421,#157422),(#157423,#157424),
(#157425,#157426),(#157427,#157428),(#157429,#157430),(#157431,#157432),
(#157433,#157434),(#157435,#157436),(#157437,#157438),(#157439,#157440),
(#157441,#157442),(#157443,#157444),(#157445,#157446),(#157447,#157448),
(#157449,#157450),(#157451,#157452)),.UNSPECIFIED.,.F.,.F.,.F.)
B_SPLINE_SURFACE_WITH_KNOTS((6,1,1,1,1,1,1,1,1,1,1,1,1,1,1,1,1,1,1,1,1,
1,1,1,1,1,1,1,1,1,1,1,1,1,1,1,1,1,1,1,1,1,1,1,1,1,1,1,1,1,1,1,1,1,1,1,1,
1,1,1,1,1,1,1,1,1,1,1,1,1,1,1,1,1,1,1,1,1,1,1,1,1,1,1,1,1,1,1,1,1,1,1,1,
1,1,1,1,1,1,1,1,1,1,1,1,1,1,1,1,1,1,1,1,1,1,1,1,1,1,1,1,1,1,1,1,1,1,1,1,
1,1,1,1,1,1,1,1,1,1,1,1,1,1,1,1,1,1,1,1,1,1,1,1,1,1,1,1,1,1,1,1,1,1,1,1,
1,1,1,1,1,1,1,1,1,1,1,1,1,1,1,1,1,1,1,1,1,1,1,1,1,1,1,1,1,1,1,1,1,1,1,6),
(2,2),(-1.,-0.995000000000001,-0.990000000000001,-0.985000000000001,-0.980000000000001,
-0.975000000000001,-0.970000000000001,-0.965000000000001,-0.960000000000001,
-0.955000000000001,-0.950000000000001,-0.945000000000001,-0.940000000000001,
-0.935000000000001,-0.930000000000001,-0.925000000000001,-0.920000000000001,
-0.915000000000001,-0.910000000000001,-0.905000000000001,-0.900000000000001,
-0.895000000000001,-0.890000000000001,-0.885000000000001,-0.880000000000001,
-0.875000000000001,-0.870000000000001,-0.865000000000001,-0.860000000000001,
-0.855000000000001,-0.850000000000001,-0.845000000000001,-0.840000000000001,
-0.835000000000001,-0.830000000000001,-0.825000000000001,-0.820000000000001,
-0.815000000000001,-0.810000000000001,-0.805000000000001,-0.800000000000001,
-0.795000000000001,-0.790000000000001,-0.785000000000001,-0.780000000000001,
-0.775000000000001,-0.770000000000001,-0.765000000000001,-0.760000000000001,
-0.755000000000001,-0.750000000000001,-0.745000000000001,-0.740000000000001,
-0.735000000000001,-0.730000000000001,-0.725000000000001,-0.720000000000001,
-0.715000000000001,-0.710000000000001,-0.705000000000001,-0.700000000000001,
-0.695000000000001,-0.690000000000001,-0.685,-0.68,-0.675,-0.67,-0.665,
-0.66,-0.655,-0.65,-0.645,-0.64,-0.635,-0.63,-0.625,-0.62,-0.615,-0.61,
-0.605,-0.6,-0.595,-0.59,-0.585,-0.58,-0.575,-0.57,-0.565,-0.56,-0.555,
-0.55,-0.545,-0.54,-0.535,-0.53,-0.525,-0.52,-0.515,-0.51,-0.505,-0.5,-0.495,
-0.49,-0.485,-0.48,-0.475,-0.47,-0.465,-0.46,-0.455,-0.45,-0.445,-0.44,
-0.435,-0.43,-0.425,-0.42,-0.415,-0.41,-0.405,-0.4,-0.395,-0.39,-0.385,
-0.38,-0.375,-0.37,-0.365,-0.36,-0.355,-0.35,-0.345,-0.34,-0.335,-0.33,
-0.325,-0.32,-0.315,-0.31,-0.305,-0.3,-0.295,-0.29,-0.285,-0.28,-0.275,
-0.27,-0.265,-0.26,-0.255,-0.25,-0.245,-0.24,-0.235,-0.23,-0.225,-0.22,
-0.215,-0.21,-0.205,-0.2,-0.195,-0.19,-0.185,-0.18,-0.175,-0.17,-0.165,
-0.16,-0.155,-0.15,-0.145,-0.14,-0.135,-0.13,-0.125,-0.12,-0.115,-0.11,
-0.105,-0.1,-0.095,-0.09,-0.085,-0.08,-0.075,-0.07,-0.065,-0.06,-0.055,
-0.05,-0.045,-0.04,-0.035,-0.03,-0.025,-0.02,-0.015,-0.01,-0.005,0.),(0.,
1.2),.UNSPECIFIED.)
GEOMETRIC_REPRESENTATION_ITEM()
RATIONAL_B_SPLINE_SURFACE(((1.,1.),(1.,1.),(1.,1.),(1.,1.),(1.,1.),(1.,
1.),(1.,1.),(1.,1.),(1.,1.),(1.,1.),(1.,1.),(1.,1.),(1.,1.),(1.,1.),(1.,
1.),(1.,1.),(1.,1.),(1.,1.),(1.,1.),(1.,1.),(1.,1.),(1.,1.),(1.,1.),(1.,
1.),(1.,1.),(1.,1.),(1.,1.),(1.,1.),(1.,1.),(1.,1.),(1.,1.),(1.,1.),(1.,
1.),(1.,1.),(1.,1.),(1.,1.),(1.,1.),(1.,1.),(1.,1.),(1.,1.),(1.,1.),(1.,
1.),(1.,1.),(1.,1.),(1.,1.),(1.,1.),(1.,1.),(1.,1.),(1.,1.),(1.,1.),(1.,
1.),(1.,1.),(1.,1.),(1.,1.),(1.,1.),(1.,1.),(1.,1.),(1.,1.),(1.,1.),(1.,
1.),(1.,1.),(1.,1.),(1.,1.),(1.,1.),(1.,1.),(1.,1.),(1.,1.),(1.,1.),(1.,
1.),(1.,1.),(1.,1.),(1.,1.),(1.,1.),(1.,1.),(1.,1.),(1.,1.),(1.,1.),(1.,
1.),(1.,1.),(1.,1.),(1.,1.),(1.,1.),(1.,1.),(1.,1.),(1.,1.),(1.,1.),(1.,
1.),(1.,1.),(1.,1.),(1.,1.),(1.,1.),(1.,1.),(1.,1.),(1.,1.),(1.,1.),(1.,
1.),(1.,1.),(1.,1.),(1.,1.),(1.,1.),(1.,1.),(1.,1.),(1.,1.),(1.,1.),(1.,
1.),(1.,1.),(1.,1.),(1.,1.),(1.,1.),(1.,1.),(1.,1.),(1.,1.),(1.,1.),(1.,
1.),(1.,1.),(1.,1.),(1.,1.),(1.,1.),(1.,1.),(1.,1.),(1.,1.),(1.,1.),(1.,
1.),(1.,1.),(1.,1.),(1.,1.),(1.,1.),(1.,1.),(1.,1.),(1.,1.),(1.,1.),(1.,
1.),(1.,1.),(1.,1.),(1.,1.),(1.,1.),(1.,1.),(1.,1.),(1.,1.),(1.,1.),(1.,
1.),(1.,1.),(1.,1.),(1.,1.),(1.,1.),(1.,1.),(1.,1.),(1.,1.),(1.,1.),(1.,
1.),(1.,1.),(1.,1.),(1.,1.),(1.,1.),(1.,1.),(1.,1.),(1.,1.),(1.,1.),(1.,
1.),(1.,1.),(1.,1.),(1.,1.),(1.,1.),(1.,1.),(1.,1.),(1.,1.),(1.,1.),(1.,
1.),(1.,1.),(1.,1.),(1.,1.),(1.,1.),(1.,1.),(1.,1.),(1.,1.),(1.,1.),(1.,
1.),(1.,1.),(1.,1.),(1.,1.),(1.,1.),(1.,1.),(1.,1.),(1.,1.),(1.,1.),(1.,
1.),(1.,1.),(1.,1.),(1.,1.),(1.,1.),(1.,1.),(1.,1.),(1.,1.),(1.,1.),(1.,
1.),(1.,1.),(1.,1.),(1.,1.),(1.,1.),(1.,1.),(1.,1.),(1.,1.),(1.,1.),(1.,
1.),(1.,1.)))
REPRESENTATION_ITEM('')
SURFACE()
);
#1006=(
BOUNDED_SURFACE()
B_SPLINE_SURFACE(5,1,((#157844,#157845),(#157846,#157847),(#157848,#157849),
(#157850,#157851),(#157852,#157853),(#157854,#157855),(#157856,#157857),
(#157858,#157859),(#157860,#157861),(#157862,#157863),(#157864,#157865),
(#157866,#157867),(#157868,#157869),(#157870,#157871),(#157872,#157873),
(#157874,#157875),(#157876,#157877),(#157878,#157879),(#157880,#157881),
(#157882,#157883),(#157884,#157885),(#157886,#157887),(#157888,#157889),
(#157890,#157891),(#157892,#157893),(#157894,#157895),(#157896,#157897),
(#157898,#157899),(#157900,#157901),(#157902,#157903),(#157904,#157905),
(#157906,#157907),(#157908,#157909),(#157910,#157911),(#157912,#157913),
(#157914,#157915),(#157916,#157917),(#157918,#157919),(#157920,#157921),
(#157922,#157923),(#157924,#157925),(#157926,#157927),(#157928,#157929),
(#157930,#157931),(#157932,#157933),(#157934,#157935),(#157936,#157937),
(#157938,#157939),(#157940,#157941),(#157942,#157943),(#157944,#157945),
(#157946,#157947),(#157948,#157949),(#157950,#157951),(#157952,#157953),
(#157954,#157955),(#157956,#157957),(#157958,#157959),(#157960,#157961),
(#157962,#157963),(#157964,#157965),(#157966,#157967),(#157968,#157969),
(#157970,#157971),(#157972,#157973),(#157974,#157975),(#157976,#157977),
(#157978,#157979),(#157980,#157981),(#157982,#157983),(#157984,#157985),
(#157986,#157987),(#157988,#157989),(#157990,#157991),(#157992,#157993),
(#157994,#157995),(#157996,#157997),(#157998,#157999),(#158000,#158001),
(#158002,#158003),(#158004,#158005),(#158006,#158007),(#158008,#158009),
(#158010,#158011),(#158012,#158013),(#158014,#158015),(#158016,#158017),
(#158018,#158019),(#158020,#158021),(#158022,#158023),(#158024,#158025),
(#158026,#158027),(#158028,#158029),(#158030,#158031),(#158032,#158033),
(#158034,#158035),(#158036,#158037),(#158038,#158039),(#158040,#158041),
(#158042,#158043),(#158044,#158045),(#158046,#158047),(#158048,#158049),
(#158050,#158051),(#158052,#158053),(#158054,#158055),(#158056,#158057),
(#158058,#158059),(#158060,#158061),(#158062,#158063),(#158064,#158065),
(#158066,#158067),(#158068,#158069),(#158070,#158071),(#158072,#158073),
(#158074,#158075),(#158076,#158077),(#158078,#158079),(#158080,#158081),
(#158082,#158083),(#158084,#158085),(#158086,#158087),(#158088,#158089),
(#158090,#158091),(#158092,#158093),(#158094,#158095),(#158096,#158097),
(#158098,#158099),(#158100,#158101),(#158102,#158103),(#158104,#158105),
(#158106,#158107),(#158108,#158109),(#158110,#158111),(#158112,#158113),
(#158114,#158115),(#158116,#158117),(#158118,#158119),(#158120,#158121),
(#158122,#158123),(#158124,#158125),(#158126,#158127),(#158128,#158129),
(#158130,#158131),(#158132,#158133),(#158134,#158135),(#158136,#158137),
(#158138,#158139),(#158140,#158141),(#158142,#158143),(#158144,#158145),
(#158146,#158147),(#158148,#158149),(#158150,#158151),(#158152,#158153),
(#158154,#158155),(#158156,#158157),(#158158,#158159),(#158160,#158161),
(#158162,#158163),(#158164,#158165),(#158166,#158167),(#158168,#158169),
(#158170,#158171),(#158172,#158173),(#158174,#158175),(#158176,#158177),
(#158178,#158179),(#158180,#158181),(#158182,#158183),(#158184,#158185),
(#158186,#158187),(#158188,#158189),(#158190,#158191),(#158192,#158193),
(#158194,#158195),(#158196,#158197),(#158198,#158199),(#158200,#158201),
(#158202,#158203),(#158204,#158205),(#158206,#158207),(#158208,#158209),
(#158210,#158211),(#158212,#158213),(#158214,#158215),(#158216,#158217),
(#158218,#158219),(#158220,#158221),(#158222,#158223),(#158224,#158225),
(#158226,#158227),(#158228,#158229),(#158230,#158231),(#158232,#158233),
(#158234,#158235),(#158236,#158237),(#158238,#158239),(#158240,#158241),
(#158242,#158243),(#158244,#158245),(#158246,#158247),(#158248,#158249),
(#158250,#158251),(#158252,#158253)),.UNSPECIFIED.,.F.,.F.,.F.)
B_SPLINE_SURFACE_WITH_KNOTS((6,1,1,1,1,1,1,1,1,1,1,1,1,1,1,1,1,1,1,1,1,
1,1,1,1,1,1,1,1,1,1,1,1,1,1,1,1,1,1,1,1,1,1,1,1,1,1,1,1,1,1,1,1,1,1,1,1,
1,1,1,1,1,1,1,1,1,1,1,1,1,1,1,1,1,1,1,1,1,1,1,1,1,1,1,1,1,1,1,1,1,1,1,1,
1,1,1,1,1,1,1,1,1,1,1,1,1,1,1,1,1,1,1,1,1,1,1,1,1,1,1,1,1,1,1,1,1,1,1,1,
1,1,1,1,1,1,1,1,1,1,1,1,1,1,1,1,1,1,1,1,1,1,1,1,1,1,1,1,1,1,1,1,1,1,1,1,
1,1,1,1,1,1,1,1,1,1,1,1,1,1,1,1,1,1,1,1,1,1,1,1,1,1,1,1,1,1,1,1,1,1,1,6),
(2,2),(-1.,-0.995000000000001,-0.990000000000001,-0.985000000000001,-0.980000000000001,
-0.975000000000001,-0.970000000000001,-0.965000000000001,-0.960000000000001,
-0.955000000000001,-0.950000000000001,-0.945000000000001,-0.940000000000001,
-0.935000000000001,-0.930000000000001,-0.925000000000001,-0.920000000000001,
-0.915000000000001,-0.910000000000001,-0.905000000000001,-0.900000000000001,
-0.895000000000001,-0.890000000000001,-0.885000000000001,-0.880000000000001,
-0.875000000000001,-0.870000000000001,-0.865000000000001,-0.860000000000001,
-0.855000000000001,-0.850000000000001,-0.845000000000001,-0.840000000000001,
-0.835000000000001,-0.830000000000001,-0.825000000000001,-0.820000000000001,
-0.815000000000001,-0.810000000000001,-0.805000000000001,-0.800000000000001,
-0.795000000000001,-0.790000000000001,-0.785000000000001,-0.780000000000001,
-0.775000000000001,-0.770000000000001,-0.765000000000001,-0.760000000000001,
-0.755000000000001,-0.750000000000001,-0.745000000000001,-0.740000000000001,
-0.735000000000001,-0.730000000000001,-0.725000000000001,-0.720000000000001,
-0.715000000000001,-0.710000000000001,-0.705000000000001,-0.700000000000001,
-0.695000000000001,-0.690000000000001,-0.685,-0.68,-0.675,-0.67,-0.665,
-0.66,-0.655,-0.65,-0.645,-0.64,-0.635,-0.63,-0.625,-0.62,-0.615,-0.61,
-0.605,-0.6,-0.595,-0.59,-0.585,-0.58,-0.575,-0.57,-0.565,-0.56,-0.555,
-0.55,-0.545,-0.54,-0.535,-0.53,-0.525,-0.52,-0.515,-0.51,-0.505,-0.5,-0.495,
-0.49,-0.485,-0.48,-0.475,-0.47,-0.465,-0.46,-0.455,-0.45,-0.445,-0.44,
-0.435,-0.43,-0.425,-0.42,-0.415,-0.41,-0.405,-0.4,-0.395,-0.39,-0.385,
-0.38,-0.375,-0.37,-0.365,-0.36,-0.355,-0.35,-0.345,-0.34,-0.335,-0.33,
-0.325,-0.32,-0.315,-0.31,-0.305,-0.3,-0.295,-0.29,-0.285,-0.28,-0.275,
-0.27,-0.265,-0.26,-0.255,-0.25,-0.245,-0.24,-0.235,-0.23,-0.225,-0.22,
-0.215,-0.21,-0.205,-0.2,-0.195,-0.19,-0.185,-0.18,-0.175,-0.17,-0.165,
-0.16,-0.155,-0.15,-0.145,-0.14,-0.135,-0.13,-0.125,-0.12,-0.115,-0.11,
-0.105,-0.1,-0.095,-0.09,-0.085,-0.08,-0.075,-0.07,-0.065,-0.06,-0.055,
-0.05,-0.045,-0.04,-0.035,-0.03,-0.025,-0.02,-0.015,-0.01,-0.005,0.),(0.,
1.2),.UNSPECIFIED.)
GEOMETRIC_REPRESENTATION_ITEM()
RATIONAL_B_SPLINE_SURFACE(((1.,1.),(1.,1.),(1.,1.),(1.,1.),(1.,1.),(1.,
1.),(1.,1.),(1.,1.),(1.,1.),(1.,1.),(1.,1.),(1.,1.),(1.,1.),(1.,1.),(1.,
1.),(1.,1.),(1.,1.),(1.,1.),(1.,1.),(1.,1.),(1.,1.),(1.,1.),(1.,1.),(1.,
1.),(1.,1.),(1.,1.),(1.,1.),(1.,1.),(1.,1.),(1.,1.),(1.,1.),(1.,1.),(1.,
1.),(1.,1.),(1.,1.),(1.,1.),(1.,1.),(1.,1.),(1.,1.),(1.,1.),(1.,1.),(1.,
1.),(1.,1.),(1.,1.),(1.,1.),(1.,1.),(1.,1.),(1.,1.),(1.,1.),(1.,1.),(1.,
1.),(1.,1.),(1.,1.),(1.,1.),(1.,1.),(1.,1.),(1.,1.),(1.,1.),(1.,1.),(1.,
1.),(1.,1.),(1.,1.),(1.,1.),(1.,1.),(1.,1.),(1.,1.),(1.,1.),(1.,1.),(1.,
1.),(1.,1.),(1.,1.),(1.,1.),(1.,1.),(1.,1.),(1.,1.),(1.,1.),(1.,1.),(1.,
1.),(1.,1.),(1.,1.),(1.,1.),(1.,1.),(1.,1.),(1.,1.),(1.,1.),(1.,1.),(1.,
1.),(1.,1.),(1.,1.),(1.,1.),(1.,1.),(1.,1.),(1.,1.),(1.,1.),(1.,1.),(1.,
1.),(1.,1.),(1.,1.),(1.,1.),(1.,1.),(1.,1.),(1.,1.),(1.,1.),(1.,1.),(1.,
1.),(1.,1.),(1.,1.),(1.,1.),(1.,1.),(1.,1.),(1.,1.),(1.,1.),(1.,1.),(1.,
1.),(1.,1.),(1.,1.),(1.,1.),(1.,1.),(1.,1.),(1.,1.),(1.,1.),(1.,1.),(1.,
1.),(1.,1.),(1.,1.),(1.,1.),(1.,1.),(1.,1.),(1.,1.),(1.,1.),(1.,1.),(1.,
1.),(1.,1.),(1.,1.),(1.,1.),(1.,1.),(1.,1.),(1.,1.),(1.,1.),(1.,1.),(1.,
1.),(1.,1.),(1.,1.),(1.,1.),(1.,1.),(1.,1.),(1.,1.),(1.,1.),(1.,1.),(1.,
1.),(1.,1.),(1.,1.),(1.,1.),(1.,1.),(1.,1.),(1.,1.),(1.,1.),(1.,1.),(1.,
1.),(1.,1.),(1.,1.),(1.,1.),(1.,1.),(1.,1.),(1.,1.),(1.,1.),(1.,1.),(1.,
1.),(1.,1.),(1.,1.),(1.,1.),(1.,1.),(1.,1.),(1.,1.),(1.,1.),(1.,1.),(1.,
1.),(1.,1.),(1.,1.),(1.,1.),(1.,1.),(1.,1.),(1.,1.),(1.,1.),(1.,1.),(1.,
1.),(1.,1.),(1.,1.),(1.,1.),(1.,1.),(1.,1.),(1.,1.),(1.,1.),(1.,1.),(1.,
1.),(1.,1.),(1.,1.),(1.,1.),(1.,1.),(1.,1.),(1.,1.),(1.,1.),(1.,1.),(1.,
1.),(1.,1.)))
REPRESENTATION_ITEM('')
SURFACE()
);
#1007=(
BOUNDED_SURFACE()
B_SPLINE_SURFACE(5,1,((#158645,#158646),(#158647,#158648),(#158649,#158650),
(#158651,#158652),(#158653,#158654),(#158655,#158656),(#158657,#158658),
(#158659,#158660),(#158661,#158662),(#158663,#158664),(#158665,#158666),
(#158667,#158668),(#158669,#158670),(#158671,#158672),(#158673,#158674),
(#158675,#158676),(#158677,#158678),(#158679,#158680),(#158681,#158682),
(#158683,#158684),(#158685,#158686),(#158687,#158688),(#158689,#158690),
(#158691,#158692),(#158693,#158694),(#158695,#158696),(#158697,#158698),
(#158699,#158700),(#158701,#158702),(#158703,#158704),(#158705,#158706),
(#158707,#158708),(#158709,#158710),(#158711,#158712),(#158713,#158714),
(#158715,#158716),(#158717,#158718),(#158719,#158720),(#158721,#158722),
(#158723,#158724),(#158725,#158726),(#158727,#158728),(#158729,#158730),
(#158731,#158732),(#158733,#158734),(#158735,#158736),(#158737,#158738),
(#158739,#158740),(#158741,#158742),(#158743,#158744),(#158745,#158746),
(#158747,#158748),(#158749,#158750),(#158751,#158752),(#158753,#158754),
(#158755,#158756),(#158757,#158758),(#158759,#158760),(#158761,#158762),
(#158763,#158764),(#158765,#158766),(#158767,#158768),(#158769,#158770),
(#158771,#158772),(#158773,#158774),(#158775,#158776),(#158777,#158778),
(#158779,#158780),(#158781,#158782),(#158783,#158784),(#158785,#158786),
(#158787,#158788),(#158789,#158790),(#158791,#158792),(#158793,#158794),
(#158795,#158796),(#158797,#158798),(#158799,#158800),(#158801,#158802),
(#158803,#158804),(#158805,#158806),(#158807,#158808),(#158809,#158810),
(#158811,#158812),(#158813,#158814),(#158815,#158816),(#158817,#158818),
(#158819,#158820),(#158821,#158822),(#158823,#158824),(#158825,#158826),
(#158827,#158828),(#158829,#158830),(#158831,#158832),(#158833,#158834),
(#158835,#158836),(#158837,#158838),(#158839,#158840),(#158841,#158842),
(#158843,#158844),(#158845,#158846),(#158847,#158848),(#158849,#158850),
(#158851,#158852),(#158853,#158854),(#158855,#158856),(#158857,#158858),
(#158859,#158860),(#158861,#158862),(#158863,#158864),(#158865,#158866),
(#158867,#158868),(#158869,#158870),(#158871,#158872),(#158873,#158874),
(#158875,#158876),(#158877,#158878),(#158879,#158880),(#158881,#158882),
(#158883,#158884),(#158885,#158886),(#158887,#158888),(#158889,#158890),
(#158891,#158892),(#158893,#158894),(#158895,#158896),(#158897,#158898),
(#158899,#158900),(#158901,#158902),(#158903,#158904),(#158905,#158906),
(#158907,#158908),(#158909,#158910),(#158911,#158912),(#158913,#158914),
(#158915,#158916),(#158917,#158918),(#158919,#158920),(#158921,#158922),
(#158923,#158924),(#158925,#158926),(#158927,#158928),(#158929,#158930),
(#158931,#158932),(#158933,#158934),(#158935,#158936),(#158937,#158938),
(#158939,#158940),(#158941,#158942),(#158943,#158944),(#158945,#158946),
(#158947,#158948),(#158949,#158950),(#158951,#158952),(#158953,#158954),
(#158955,#158956),(#158957,#158958),(#158959,#158960),(#158961,#158962),
(#158963,#158964),(#158965,#158966),(#158967,#158968),(#158969,#158970),
(#158971,#158972),(#158973,#158974),(#158975,#158976),(#158977,#158978),
(#158979,#158980),(#158981,#158982),(#158983,#158984),(#158985,#158986),
(#158987,#158988),(#158989,#158990),(#158991,#158992),(#158993,#158994),
(#158995,#158996),(#158997,#158998),(#158999,#159000),(#159001,#159002),
(#159003,#159004),(#159005,#159006),(#159007,#159008),(#159009,#159010),
(#159011,#159012),(#159013,#159014),(#159015,#159016),(#159017,#159018),
(#159019,#159020),(#159021,#159022),(#159023,#159024),(#159025,#159026),
(#159027,#159028),(#159029,#159030),(#159031,#159032),(#159033,#159034),
(#159035,#159036),(#159037,#159038),(#159039,#159040),(#159041,#159042),
(#159043,#159044),(#159045,#159046),(#159047,#159048),(#159049,#159050),
(#159051,#159052),(#159053,#159054)),.UNSPECIFIED.,.F.,.F.,.F.)
B_SPLINE_SURFACE_WITH_KNOTS((6,1,1,1,1,1,1,1,1,1,1,1,1,1,1,1,1,1,1,1,1,
1,1,1,1,1,1,1,1,1,1,1,1,1,1,1,1,1,1,1,1,1,1,1,1,1,1,1,1,1,1,1,1,1,1,1,1,
1,1,1,1,1,1,1,1,1,1,1,1,1,1,1,1,1,1,1,1,1,1,1,1,1,1,1,1,1,1,1,1,1,1,1,1,
1,1,1,1,1,1,1,1,1,1,1,1,1,1,1,1,1,1,1,1,1,1,1,1,1,1,1,1,1,1,1,1,1,1,1,1,
1,1,1,1,1,1,1,1,1,1,1,1,1,1,1,1,1,1,1,1,1,1,1,1,1,1,1,1,1,1,1,1,1,1,1,1,
1,1,1,1,1,1,1,1,1,1,1,1,1,1,1,1,1,1,1,1,1,1,1,1,1,1,1,1,1,1,1,1,1,1,1,6),
(2,2),(-1.,-0.995000000000001,-0.990000000000001,-0.985000000000001,-0.980000000000001,
-0.975000000000001,-0.970000000000001,-0.965000000000001,-0.960000000000001,
-0.955000000000001,-0.950000000000001,-0.945000000000001,-0.940000000000001,
-0.935000000000001,-0.930000000000001,-0.925000000000001,-0.920000000000001,
-0.915000000000001,-0.910000000000001,-0.905000000000001,-0.900000000000001,
-0.895000000000001,-0.890000000000001,-0.885000000000001,-0.880000000000001,
-0.875000000000001,-0.870000000000001,-0.865000000000001,-0.860000000000001,
-0.855000000000001,-0.850000000000001,-0.845000000000001,-0.840000000000001,
-0.835000000000001,-0.830000000000001,-0.825000000000001,-0.820000000000001,
-0.815000000000001,-0.810000000000001,-0.805000000000001,-0.800000000000001,
-0.795000000000001,-0.790000000000001,-0.785000000000001,-0.780000000000001,
-0.775000000000001,-0.770000000000001,-0.765000000000001,-0.760000000000001,
-0.755000000000001,-0.750000000000001,-0.745000000000001,-0.740000000000001,
-0.735000000000001,-0.730000000000001,-0.725000000000001,-0.720000000000001,
-0.715000000000001,-0.710000000000001,-0.705000000000001,-0.700000000000001,
-0.695000000000001,-0.690000000000001,-0.685,-0.68,-0.675,-0.67,-0.665,
-0.66,-0.655,-0.65,-0.645,-0.64,-0.635,-0.63,-0.625,-0.62,-0.615,-0.61,
-0.605,-0.6,-0.595,-0.59,-0.585,-0.58,-0.575,-0.57,-0.565,-0.56,-0.555,
-0.55,-0.545,-0.54,-0.535,-0.53,-0.525,-0.52,-0.515,-0.51,-0.505,-0.5,-0.495,
-0.49,-0.485,-0.48,-0.475,-0.47,-0.465,-0.46,-0.455,-0.45,-0.445,-0.44,
-0.435,-0.43,-0.425,-0.42,-0.415,-0.41,-0.405,-0.4,-0.395,-0.39,-0.385,
-0.38,-0.375,-0.37,-0.365,-0.36,-0.355,-0.35,-0.345,-0.34,-0.335,-0.33,
-0.325,-0.32,-0.315,-0.31,-0.305,-0.3,-0.295,-0.29,-0.285,-0.28,-0.275,
-0.27,-0.265,-0.26,-0.255,-0.25,-0.245,-0.24,-0.235,-0.23,-0.225,-0.22,
-0.215,-0.21,-0.205,-0.2,-0.195,-0.19,-0.185,-0.18,-0.175,-0.17,-0.165,
-0.16,-0.155,-0.15,-0.145,-0.14,-0.135,-0.13,-0.125,-0.12,-0.115,-0.11,
-0.105,-0.1,-0.095,-0.09,-0.085,-0.08,-0.075,-0.07,-0.065,-0.06,-0.055,
-0.05,-0.045,-0.04,-0.035,-0.03,-0.025,-0.02,-0.015,-0.01,-0.005,0.),(0.,
1.2),.UNSPECIFIED.)
GEOMETRIC_REPRESENTATION_ITEM()
RATIONAL_B_SPLINE_SURFACE(((1.,1.),(1.,1.),(1.,1.),(1.,1.),(1.,1.),(1.,
1.),(1.,1.),(1.,1.),(1.,1.),(1.,1.),(1.,1.),(1.,1.),(1.,1.),(1.,1.),(1.,
1.),(1.,1.),(1.,1.),(1.,1.),(1.,1.),(1.,1.),(1.,1.),(1.,1.),(1.,1.),(1.,
1.),(1.,1.),(1.,1.),(1.,1.),(1.,1.),(1.,1.),(1.,1.),(1.,1.),(1.,1.),(1.,
1.),(1.,1.),(1.,1.),(1.,1.),(1.,1.),(1.,1.),(1.,1.),(1.,1.),(1.,1.),(1.,
1.),(1.,1.),(1.,1.),(1.,1.),(1.,1.),(1.,1.),(1.,1.),(1.,1.),(1.,1.),(1.,
1.),(1.,1.),(1.,1.),(1.,1.),(1.,1.),(1.,1.),(1.,1.),(1.,1.),(1.,1.),(1.,
1.),(1.,1.),(1.,1.),(1.,1.),(1.,1.),(1.,1.),(1.,1.),(1.,1.),(1.,1.),(1.,
1.),(1.,1.),(1.,1.),(1.,1.),(1.,1.),(1.,1.),(1.,1.),(1.,1.),(1.,1.),(1.,
1.),(1.,1.),(1.,1.),(1.,1.),(1.,1.),(1.,1.),(1.,1.),(1.,1.),(1.,1.),(1.,
1.),(1.,1.),(1.,1.),(1.,1.),(1.,1.),(1.,1.),(1.,1.),(1.,1.),(1.,1.),(1.,
1.),(1.,1.),(1.,1.),(1.,1.),(1.,1.),(1.,1.),(1.,1.),(1.,1.),(1.,1.),(1.,
1.),(1.,1.),(1.,1.),(1.,1.),(1.,1.),(1.,1.),(1.,1.),(1.,1.),(1.,1.),(1.,
1.),(1.,1.),(1.,1.),(1.,1.),(1.,1.),(1.,1.),(1.,1.),(1.,1.),(1.,1.),(1.,
1.),(1.,1.),(1.,1.),(1.,1.),(1.,1.),(1.,1.),(1.,1.),(1.,1.),(1.,1.),(1.,
1.),(1.,1.),(1.,1.),(1.,1.),(1.,1.),(1.,1.),(1.,1.),(1.,1.),(1.,1.),(1.,
1.),(1.,1.),(1.,1.),(1.,1.),(1.,1.),(1.,1.),(1.,1.),(1.,1.),(1.,1.),(1.,
1.),(1.,1.),(1.,1.),(1.,1.),(1.,1.),(1.,1.),(1.,1.),(1.,1.),(1.,1.),(1.,
1.),(1.,1.),(1.,1.),(1.,1.),(1.,1.),(1.,1.),(1.,1.),(1.,1.),(1.,1.),(1.,
1.),(1.,1.),(1.,1.),(1.,1.),(1.,1.),(1.,1.),(1.,1.),(1.,1.),(1.,1.),(1.,
1.),(1.,1.),(1.,1.),(1.,1.),(1.,1.),(1.,1.),(1.,1.),(1.,1.),(1.,1.),(1.,
1.),(1.,1.),(1.,1.),(1.,1.),(1.,1.),(1.,1.),(1.,1.),(1.,1.),(1.,1.),(1.,
1.),(1.,1.),(1.,1.),(1.,1.),(1.,1.),(1.,1.),(1.,1.),(1.,1.),(1.,1.),(1.,
1.),(1.,1.)))
REPRESENTATION_ITEM('')
SURFACE()
);
#1008=(
BOUNDED_SURFACE()
B_SPLINE_SURFACE(5,1,((#159446,#159447),(#159448,#159449),(#159450,#159451),
(#159452,#159453),(#159454,#159455),(#159456,#159457),(#159458,#159459),
(#159460,#159461),(#159462,#159463),(#159464,#159465),(#159466,#159467),
(#159468,#159469),(#159470,#159471),(#159472,#159473),(#159474,#159475),
(#159476,#159477),(#159478,#159479),(#159480,#159481),(#159482,#159483),
(#159484,#159485),(#159486,#159487),(#159488,#159489),(#159490,#159491),
(#159492,#159493),(#159494,#159495),(#159496,#159497),(#159498,#159499),
(#159500,#159501),(#159502,#159503),(#159504,#159505),(#159506,#159507),
(#159508,#159509),(#159510,#159511),(#159512,#159513),(#159514,#159515),
(#159516,#159517),(#159518,#159519),(#159520,#159521),(#159522,#159523),
(#159524,#159525),(#159526,#159527),(#159528,#159529),(#159530,#159531),
(#159532,#159533),(#159534,#159535),(#159536,#159537),(#159538,#159539),
(#159540,#159541),(#159542,#159543),(#159544,#159545),(#159546,#159547),
(#159548,#159549),(#159550,#159551),(#159552,#159553),(#159554,#159555),
(#159556,#159557),(#159558,#159559),(#159560,#159561),(#159562,#159563),
(#159564,#159565),(#159566,#159567),(#159568,#159569),(#159570,#159571),
(#159572,#159573),(#159574,#159575),(#159576,#159577),(#159578,#159579),
(#159580,#159581),(#159582,#159583),(#159584,#159585),(#159586,#159587),
(#159588,#159589),(#159590,#159591),(#159592,#159593),(#159594,#159595),
(#159596,#159597),(#159598,#159599),(#159600,#159601),(#159602,#159603),
(#159604,#159605),(#159606,#159607),(#159608,#159609),(#159610,#159611),
(#159612,#159613),(#159614,#159615),(#159616,#159617),(#159618,#159619),
(#159620,#159621),(#159622,#159623),(#159624,#159625),(#159626,#159627),
(#159628,#159629),(#159630,#159631),(#159632,#159633),(#159634,#159635),
(#159636,#159637),(#159638,#159639),(#159640,#159641),(#159642,#159643),
(#159644,#159645),(#159646,#159647),(#159648,#159649),(#159650,#159651),
(#159652,#159653),(#159654,#159655),(#159656,#159657),(#159658,#159659),
(#159660,#159661),(#159662,#159663),(#159664,#159665),(#159666,#159667),
(#159668,#159669),(#159670,#159671),(#159672,#159673),(#159674,#159675),
(#159676,#159677),(#159678,#159679),(#159680,#159681),(#159682,#159683),
(#159684,#159685),(#159686,#159687),(#159688,#159689),(#159690,#159691),
(#159692,#159693),(#159694,#159695),(#159696,#159697),(#159698,#159699),
(#159700,#159701),(#159702,#159703),(#159704,#159705),(#159706,#159707),
(#159708,#159709),(#159710,#159711),(#159712,#159713),(#159714,#159715),
(#159716,#159717),(#159718,#159719),(#159720,#159721),(#159722,#159723),
(#159724,#159725),(#159726,#159727),(#159728,#159729),(#159730,#159731),
(#159732,#159733),(#159734,#159735),(#159736,#159737),(#159738,#159739),
(#159740,#159741),(#159742,#159743),(#159744,#159745),(#159746,#159747),
(#159748,#159749),(#159750,#159751),(#159752,#159753),(#159754,#159755),
(#159756,#159757),(#159758,#159759),(#159760,#159761),(#159762,#159763),
(#159764,#159765),(#159766,#159767),(#159768,#159769),(#159770,#159771),
(#159772,#159773),(#159774,#159775),(#159776,#159777),(#159778,#159779),
(#159780,#159781),(#159782,#159783),(#159784,#159785),(#159786,#159787),
(#159788,#159789),(#159790,#159791),(#159792,#159793),(#159794,#159795),
(#159796,#159797),(#159798,#159799),(#159800,#159801),(#159802,#159803),
(#159804,#159805),(#159806,#159807),(#159808,#159809),(#159810,#159811),
(#159812,#159813),(#159814,#159815),(#159816,#159817),(#159818,#159819),
(#159820,#159821),(#159822,#159823),(#159824,#159825),(#159826,#159827),
(#159828,#159829),(#159830,#159831),(#159832,#159833),(#159834,#159835),
(#159836,#159837),(#159838,#159839),(#159840,#159841),(#159842,#159843),
(#159844,#159845),(#159846,#159847),(#159848,#159849),(#159850,#159851),
(#159852,#159853),(#159854,#159855)),.UNSPECIFIED.,.F.,.F.,.F.)
B_SPLINE_SURFACE_WITH_KNOTS((6,1,1,1,1,1,1,1,1,1,1,1,1,1,1,1,1,1,1,1,1,
1,1,1,1,1,1,1,1,1,1,1,1,1,1,1,1,1,1,1,1,1,1,1,1,1,1,1,1,1,1,1,1,1,1,1,1,
1,1,1,1,1,1,1,1,1,1,1,1,1,1,1,1,1,1,1,1,1,1,1,1,1,1,1,1,1,1,1,1,1,1,1,1,
1,1,1,1,1,1,1,1,1,1,1,1,1,1,1,1,1,1,1,1,1,1,1,1,1,1,1,1,1,1,1,1,1,1,1,1,
1,1,1,1,1,1,1,1,1,1,1,1,1,1,1,1,1,1,1,1,1,1,1,1,1,1,1,1,1,1,1,1,1,1,1,1,
1,1,1,1,1,1,1,1,1,1,1,1,1,1,1,1,1,1,1,1,1,1,1,1,1,1,1,1,1,1,1,1,1,1,1,6),
(2,2),(-1.,-0.995000000000001,-0.990000000000001,-0.985000000000001,-0.980000000000001,
-0.975000000000001,-0.970000000000001,-0.965000000000001,-0.960000000000001,
-0.955000000000001,-0.950000000000001,-0.945000000000001,-0.940000000000001,
-0.935000000000001,-0.930000000000001,-0.925000000000001,-0.920000000000001,
-0.915000000000001,-0.910000000000001,-0.905000000000001,-0.900000000000001,
-0.895000000000001,-0.890000000000001,-0.885000000000001,-0.880000000000001,
-0.875000000000001,-0.870000000000001,-0.865000000000001,-0.860000000000001,
-0.855000000000001,-0.850000000000001,-0.845000000000001,-0.840000000000001,
-0.835000000000001,-0.830000000000001,-0.825000000000001,-0.820000000000001,
-0.815000000000001,-0.810000000000001,-0.805000000000001,-0.800000000000001,
-0.795000000000001,-0.790000000000001,-0.785000000000001,-0.780000000000001,
-0.775000000000001,-0.770000000000001,-0.765000000000001,-0.760000000000001,
-0.755000000000001,-0.750000000000001,-0.745000000000001,-0.740000000000001,
-0.735000000000001,-0.730000000000001,-0.725000000000001,-0.720000000000001,
-0.715000000000001,-0.710000000000001,-0.705000000000001,-0.700000000000001,
-0.695000000000001,-0.690000000000001,-0.685,-0.68,-0.675,-0.67,-0.665,
-0.66,-0.655,-0.65,-0.645,-0.64,-0.635,-0.63,-0.625,-0.62,-0.615,-0.61,
-0.605,-0.6,-0.595,-0.59,-0.585,-0.58,-0.575,-0.57,-0.565,-0.56,-0.555,
-0.55,-0.545,-0.54,-0.535,-0.53,-0.525,-0.52,-0.515,-0.51,-0.505,-0.5,-0.495,
-0.49,-0.485,-0.48,-0.475,-0.47,-0.465,-0.46,-0.455,-0.45,-0.445,-0.44,
-0.435,-0.43,-0.425,-0.42,-0.415,-0.41,-0.405,-0.4,-0.395,-0.39,-0.385,
-0.38,-0.375,-0.37,-0.365,-0.36,-0.355,-0.35,-0.345,-0.34,-0.335,-0.33,
-0.325,-0.32,-0.315,-0.31,-0.305,-0.3,-0.295,-0.29,-0.285,-0.28,-0.275,
-0.27,-0.265,-0.26,-0.255,-0.25,-0.245,-0.24,-0.235,-0.23,-0.225,-0.22,
-0.215,-0.21,-0.205,-0.2,-0.195,-0.19,-0.185,-0.18,-0.175,-0.17,-0.165,
-0.16,-0.155,-0.15,-0.145,-0.14,-0.135,-0.13,-0.125,-0.12,-0.115,-0.11,
-0.105,-0.1,-0.095,-0.09,-0.085,-0.08,-0.075,-0.07,-0.065,-0.06,-0.055,
-0.05,-0.045,-0.04,-0.035,-0.03,-0.025,-0.02,-0.015,-0.01,-0.005,0.),(0.,
1.2),.UNSPECIFIED.)
GEOMETRIC_REPRESENTATION_ITEM()
RATIONAL_B_SPLINE_SURFACE(((1.,1.),(1.,1.),(1.,1.),(1.,1.),(1.,1.),(1.,
1.),(1.,1.),(1.,1.),(1.,1.),(1.,1.),(1.,1.),(1.,1.),(1.,1.),(1.,1.),(1.,
1.),(1.,1.),(1.,1.),(1.,1.),(1.,1.),(1.,1.),(1.,1.),(1.,1.),(1.,1.),(1.,
1.),(1.,1.),(1.,1.),(1.,1.),(1.,1.),(1.,1.),(1.,1.),(1.,1.),(1.,1.),(1.,
1.),(1.,1.),(1.,1.),(1.,1.),(1.,1.),(1.,1.),(1.,1.),(1.,1.),(1.,1.),(1.,
1.),(1.,1.),(1.,1.),(1.,1.),(1.,1.),(1.,1.),(1.,1.),(1.,1.),(1.,1.),(1.,
1.),(1.,1.),(1.,1.),(1.,1.),(1.,1.),(1.,1.),(1.,1.),(1.,1.),(1.,1.),(1.,
1.),(1.,1.),(1.,1.),(1.,1.),(1.,1.),(1.,1.),(1.,1.),(1.,1.),(1.,1.),(1.,
1.),(1.,1.),(1.,1.),(1.,1.),(1.,1.),(1.,1.),(1.,1.),(1.,1.),(1.,1.),(1.,
1.),(1.,1.),(1.,1.),(1.,1.),(1.,1.),(1.,1.),(1.,1.),(1.,1.),(1.,1.),(1.,
1.),(1.,1.),(1.,1.),(1.,1.),(1.,1.),(1.,1.),(1.,1.),(1.,1.),(1.,1.),(1.,
1.),(1.,1.),(1.,1.),(1.,1.),(1.,1.),(1.,1.),(1.,1.),(1.,1.),(1.,1.),(1.,
1.),(1.,1.),(1.,1.),(1.,1.),(1.,1.),(1.,1.),(1.,1.),(1.,1.),(1.,1.),(1.,
1.),(1.,1.),(1.,1.),(1.,1.),(1.,1.),(1.,1.),(1.,1.),(1.,1.),(1.,1.),(1.,
1.),(1.,1.),(1.,1.),(1.,1.),(1.,1.),(1.,1.),(1.,1.),(1.,1.),(1.,1.),(1.,
1.),(1.,1.),(1.,1.),(1.,1.),(1.,1.),(1.,1.),(1.,1.),(1.,1.),(1.,1.),(1.,
1.),(1.,1.),(1.,1.),(1.,1.),(1.,1.),(1.,1.),(1.,1.),(1.,1.),(1.,1.),(1.,
1.),(1.,1.),(1.,1.),(1.,1.),(1.,1.),(1.,1.),(1.,1.),(1.,1.),(1.,1.),(1.,
1.),(1.,1.),(1.,1.),(1.,1.),(1.,1.),(1.,1.),(1.,1.),(1.,1.),(1.,1.),(1.,
1.),(1.,1.),(1.,1.),(1.,1.),(1.,1.),(1.,1.),(1.,1.),(1.,1.),(1.,1.),(1.,
1.),(1.,1.),(1.,1.),(1.,1.),(1.,1.),(1.,1.),(1.,1.),(1.,1.),(1.,1.),(1.,
1.),(1.,1.),(1.,1.),(1.,1.),(1.,1.),(1.,1.),(1.,1.),(1.,1.),(1.,1.),(1.,
1.),(1.,1.),(1.,1.),(1.,1.),(1.,1.),(1.,1.),(1.,1.),(1.,1.),(1.,1.),(1.,
1.),(1.,1.)))
REPRESENTATION_ITEM('')
SURFACE()
);
#1009=(
BOUNDED_SURFACE()
B_SPLINE_SURFACE(5,1,((#160247,#160248),(#160249,#160250),(#160251,#160252),
(#160253,#160254),(#160255,#160256),(#160257,#160258),(#160259,#160260),
(#160261,#160262),(#160263,#160264),(#160265,#160266),(#160267,#160268),
(#160269,#160270),(#160271,#160272),(#160273,#160274),(#160275,#160276),
(#160277,#160278),(#160279,#160280),(#160281,#160282),(#160283,#160284),
(#160285,#160286),(#160287,#160288),(#160289,#160290),(#160291,#160292),
(#160293,#160294),(#160295,#160296),(#160297,#160298),(#160299,#160300),
(#160301,#160302),(#160303,#160304),(#160305,#160306),(#160307,#160308),
(#160309,#160310),(#160311,#160312),(#160313,#160314),(#160315,#160316),
(#160317,#160318),(#160319,#160320),(#160321,#160322),(#160323,#160324),
(#160325,#160326),(#160327,#160328),(#160329,#160330),(#160331,#160332),
(#160333,#160334),(#160335,#160336),(#160337,#160338),(#160339,#160340),
(#160341,#160342),(#160343,#160344),(#160345,#160346),(#160347,#160348),
(#160349,#160350),(#160351,#160352),(#160353,#160354),(#160355,#160356),
(#160357,#160358),(#160359,#160360),(#160361,#160362),(#160363,#160364),
(#160365,#160366),(#160367,#160368),(#160369,#160370),(#160371,#160372),
(#160373,#160374),(#160375,#160376),(#160377,#160378),(#160379,#160380),
(#160381,#160382),(#160383,#160384),(#160385,#160386),(#160387,#160388),
(#160389,#160390),(#160391,#160392),(#160393,#160394),(#160395,#160396),
(#160397,#160398),(#160399,#160400),(#160401,#160402),(#160403,#160404),
(#160405,#160406),(#160407,#160408),(#160409,#160410),(#160411,#160412),
(#160413,#160414),(#160415,#160416),(#160417,#160418),(#160419,#160420),
(#160421,#160422),(#160423,#160424),(#160425,#160426),(#160427,#160428),
(#160429,#160430),(#160431,#160432),(#160433,#160434),(#160435,#160436),
(#160437,#160438),(#160439,#160440),(#160441,#160442),(#160443,#160444),
(#160445,#160446),(#160447,#160448),(#160449,#160450),(#160451,#160452),
(#160453,#160454),(#160455,#160456),(#160457,#160458),(#160459,#160460),
(#160461,#160462),(#160463,#160464),(#160465,#160466),(#160467,#160468),
(#160469,#160470),(#160471,#160472),(#160473,#160474),(#160475,#160476),
(#160477,#160478),(#160479,#160480),(#160481,#160482),(#160483,#160484),
(#160485,#160486),(#160487,#160488),(#160489,#160490),(#160491,#160492),
(#160493,#160494),(#160495,#160496),(#160497,#160498),(#160499,#160500),
(#160501,#160502),(#160503,#160504),(#160505,#160506),(#160507,#160508),
(#160509,#160510),(#160511,#160512),(#160513,#160514),(#160515,#160516),
(#160517,#160518),(#160519,#160520),(#160521,#160522),(#160523,#160524),
(#160525,#160526),(#160527,#160528),(#160529,#160530),(#160531,#160532),
(#160533,#160534),(#160535,#160536),(#160537,#160538),(#160539,#160540),
(#160541,#160542),(#160543,#160544),(#160545,#160546),(#160547,#160548),
(#160549,#160550),(#160551,#160552),(#160553,#160554),(#160555,#160556),
(#160557,#160558),(#160559,#160560),(#160561,#160562),(#160563,#160564),
(#160565,#160566),(#160567,#160568),(#160569,#160570),(#160571,#160572),
(#160573,#160574),(#160575,#160576),(#160577,#160578),(#160579,#160580),
(#160581,#160582),(#160583,#160584),(#160585,#160586),(#160587,#160588),
(#160589,#160590),(#160591,#160592),(#160593,#160594),(#160595,#160596),
(#160597,#160598),(#160599,#160600),(#160601,#160602),(#160603,#160604),
(#160605,#160606),(#160607,#160608),(#160609,#160610),(#160611,#160612),
(#160613,#160614),(#160615,#160616),(#160617,#160618),(#160619,#160620),
(#160621,#160622),(#160623,#160624),(#160625,#160626),(#160627,#160628),
(#160629,#160630),(#160631,#160632),(#160633,#160634),(#160635,#160636),
(#160637,#160638),(#160639,#160640),(#160641,#160642),(#160643,#160644),
(#160645,#160646),(#160647,#160648),(#160649,#160650),(#160651,#160652),
(#160653,#160654),(#160655,#160656)),.UNSPECIFIED.,.F.,.F.,.F.)
B_SPLINE_SURFACE_WITH_KNOTS((6,1,1,1,1,1,1,1,1,1,1,1,1,1,1,1,1,1,1,1,1,
1,1,1,1,1,1,1,1,1,1,1,1,1,1,1,1,1,1,1,1,1,1,1,1,1,1,1,1,1,1,1,1,1,1,1,1,
1,1,1,1,1,1,1,1,1,1,1,1,1,1,1,1,1,1,1,1,1,1,1,1,1,1,1,1,1,1,1,1,1,1,1,1,
1,1,1,1,1,1,1,1,1,1,1,1,1,1,1,1,1,1,1,1,1,1,1,1,1,1,1,1,1,1,1,1,1,1,1,1,
1,1,1,1,1,1,1,1,1,1,1,1,1,1,1,1,1,1,1,1,1,1,1,1,1,1,1,1,1,1,1,1,1,1,1,1,
1,1,1,1,1,1,1,1,1,1,1,1,1,1,1,1,1,1,1,1,1,1,1,1,1,1,1,1,1,1,1,1,1,1,1,6),
(2,2),(-1.,-0.995000000000001,-0.990000000000001,-0.985000000000001,-0.980000000000001,
-0.975000000000001,-0.970000000000001,-0.965000000000001,-0.960000000000001,
-0.955000000000001,-0.950000000000001,-0.945000000000001,-0.940000000000001,
-0.935000000000001,-0.930000000000001,-0.925000000000001,-0.920000000000001,
-0.915000000000001,-0.910000000000001,-0.905000000000001,-0.900000000000001,
-0.895000000000001,-0.890000000000001,-0.885000000000001,-0.880000000000001,
-0.875000000000001,-0.870000000000001,-0.865000000000001,-0.860000000000001,
-0.855000000000001,-0.850000000000001,-0.845000000000001,-0.840000000000001,
-0.835000000000001,-0.830000000000001,-0.825000000000001,-0.820000000000001,
-0.815000000000001,-0.810000000000001,-0.805000000000001,-0.800000000000001,
-0.795000000000001,-0.790000000000001,-0.785000000000001,-0.780000000000001,
-0.775000000000001,-0.770000000000001,-0.765000000000001,-0.760000000000001,
-0.755000000000001,-0.750000000000001,-0.745000000000001,-0.740000000000001,
-0.735000000000001,-0.730000000000001,-0.725000000000001,-0.720000000000001,
-0.715000000000001,-0.710000000000001,-0.705000000000001,-0.700000000000001,
-0.695000000000001,-0.690000000000001,-0.685,-0.68,-0.675,-0.67,-0.665,
-0.66,-0.655,-0.65,-0.645,-0.64,-0.635,-0.63,-0.625,-0.62,-0.615,-0.61,
-0.605,-0.6,-0.595,-0.59,-0.585,-0.58,-0.575,-0.57,-0.565,-0.56,-0.555,
-0.55,-0.545,-0.54,-0.535,-0.53,-0.525,-0.52,-0.515,-0.51,-0.505,-0.5,-0.495,
-0.49,-0.485,-0.48,-0.475,-0.47,-0.465,-0.46,-0.455,-0.45,-0.445,-0.44,
-0.435,-0.43,-0.425,-0.42,-0.415,-0.41,-0.405,-0.4,-0.395,-0.39,-0.385,
-0.38,-0.375,-0.37,-0.365,-0.36,-0.355,-0.35,-0.345,-0.34,-0.335,-0.33,
-0.325,-0.32,-0.315,-0.31,-0.305,-0.3,-0.295,-0.29,-0.285,-0.28,-0.275,
-0.27,-0.265,-0.26,-0.255,-0.25,-0.245,-0.24,-0.235,-0.23,-0.225,-0.22,
-0.215,-0.21,-0.205,-0.2,-0.195,-0.19,-0.185,-0.18,-0.175,-0.17,-0.165,
-0.16,-0.155,-0.15,-0.145,-0.14,-0.135,-0.13,-0.125,-0.12,-0.115,-0.11,
-0.105,-0.1,-0.095,-0.09,-0.085,-0.08,-0.075,-0.07,-0.065,-0.06,-0.055,
-0.05,-0.045,-0.04,-0.035,-0.03,-0.025,-0.02,-0.015,-0.01,-0.005,0.),(0.,
1.2),.UNSPECIFIED.)
GEOMETRIC_REPRESENTATION_ITEM()
RATIONAL_B_SPLINE_SURFACE(((1.,1.),(1.,1.),(1.,1.),(1.,1.),(1.,1.),(1.,
1.),(1.,1.),(1.,1.),(1.,1.),(1.,1.),(1.,1.),(1.,1.),(1.,1.),(1.,1.),(1.,
1.),(1.,1.),(1.,1.),(1.,1.),(1.,1.),(1.,1.),(1.,1.),(1.,1.),(1.,1.),(1.,
1.),(1.,1.),(1.,1.),(1.,1.),(1.,1.),(1.,1.),(1.,1.),(1.,1.),(1.,1.),(1.,
1.),(1.,1.),(1.,1.),(1.,1.),(1.,1.),(1.,1.),(1.,1.),(1.,1.),(1.,1.),(1.,
1.),(1.,1.),(1.,1.),(1.,1.),(1.,1.),(1.,1.),(1.,1.),(1.,1.),(1.,1.),(1.,
1.),(1.,1.),(1.,1.),(1.,1.),(1.,1.),(1.,1.),(1.,1.),(1.,1.),(1.,1.),(1.,
1.),(1.,1.),(1.,1.),(1.,1.),(1.,1.),(1.,1.),(1.,1.),(1.,1.),(1.,1.),(1.,
1.),(1.,1.),(1.,1.),(1.,1.),(1.,1.),(1.,1.),(1.,1.),(1.,1.),(1.,1.),(1.,
1.),(1.,1.),(1.,1.),(1.,1.),(1.,1.),(1.,1.),(1.,1.),(1.,1.),(1.,1.),(1.,
1.),(1.,1.),(1.,1.),(1.,1.),(1.,1.),(1.,1.),(1.,1.),(1.,1.),(1.,1.),(1.,
1.),(1.,1.),(1.,1.),(1.,1.),(1.,1.),(1.,1.),(1.,1.),(1.,1.),(1.,1.),(1.,
1.),(1.,1.),(1.,1.),(1.,1.),(1.,1.),(1.,1.),(1.,1.),(1.,1.),(1.,1.),(1.,
1.),(1.,1.),(1.,1.),(1.,1.),(1.,1.),(1.,1.),(1.,1.),(1.,1.),(1.,1.),(1.,
1.),(1.,1.),(1.,1.),(1.,1.),(1.,1.),(1.,1.),(1.,1.),(1.,1.),(1.,1.),(1.,
1.),(1.,1.),(1.,1.),(1.,1.),(1.,1.),(1.,1.),(1.,1.),(1.,1.),(1.,1.),(1.,
1.),(1.,1.),(1.,1.),(1.,1.),(1.,1.),(1.,1.),(1.,1.),(1.,1.),(1.,1.),(1.,
1.),(1.,1.),(1.,1.),(1.,1.),(1.,1.),(1.,1.),(1.,1.),(1.,1.),(1.,1.),(1.,
1.),(1.,1.),(1.,1.),(1.,1.),(1.,1.),(1.,1.),(1.,1.),(1.,1.),(1.,1.),(1.,
1.),(1.,1.),(1.,1.),(1.,1.),(1.,1.),(1.,1.),(1.,1.),(1.,1.),(1.,1.),(1.,
1.),(1.,1.),(1.,1.),(1.,1.),(1.,1.),(1.,1.),(1.,1.),(1.,1.),(1.,1.),(1.,
1.),(1.,1.),(1.,1.),(1.,1.),(1.,1.),(1.,1.),(1.,1.),(1.,1.),(1.,1.),(1.,
1.),(1.,1.),(1.,1.),(1.,1.),(1.,1.),(1.,1.),(1.,1.),(1.,1.),(1.,1.),(1.,
1.),(1.,1.)))
REPRESENTATION_ITEM('')
SURFACE()
);
#1010=(
BOUNDED_SURFACE()
B_SPLINE_SURFACE(5,1,((#161048,#161049),(#161050,#161051),(#161052,#161053),
(#161054,#161055),(#161056,#161057),(#161058,#161059),(#161060,#161061),
(#161062,#161063),(#161064,#161065),(#161066,#161067),(#161068,#161069),
(#161070,#161071),(#161072,#161073),(#161074,#161075),(#161076,#161077),
(#161078,#161079),(#161080,#161081),(#161082,#161083),(#161084,#161085),
(#161086,#161087),(#161088,#161089),(#161090,#161091),(#161092,#161093),
(#161094,#161095),(#161096,#161097),(#161098,#161099),(#161100,#161101),
(#161102,#161103),(#161104,#161105),(#161106,#161107),(#161108,#161109),
(#161110,#161111),(#161112,#161113),(#161114,#161115),(#161116,#161117),
(#161118,#161119),(#161120,#161121),(#161122,#161123),(#161124,#161125),
(#161126,#161127),(#161128,#161129),(#161130,#161131),(#161132,#161133),
(#161134,#161135),(#161136,#161137),(#161138,#161139),(#161140,#161141),
(#161142,#161143),(#161144,#161145),(#161146,#161147),(#161148,#161149),
(#161150,#161151),(#161152,#161153),(#161154,#161155),(#161156,#161157),
(#161158,#161159),(#161160,#161161),(#161162,#161163),(#161164,#161165),
(#161166,#161167),(#161168,#161169),(#161170,#161171),(#161172,#161173),
(#161174,#161175),(#161176,#161177),(#161178,#161179),(#161180,#161181),
(#161182,#161183),(#161184,#161185),(#161186,#161187),(#161188,#161189),
(#161190,#161191),(#161192,#161193),(#161194,#161195),(#161196,#161197),
(#161198,#161199),(#161200,#161201),(#161202,#161203),(#161204,#161205),
(#161206,#161207),(#161208,#161209),(#161210,#161211),(#161212,#161213),
(#161214,#161215),(#161216,#161217),(#161218,#161219),(#161220,#161221),
(#161222,#161223),(#161224,#161225),(#161226,#161227),(#161228,#161229),
(#161230,#161231),(#161232,#161233),(#161234,#161235),(#161236,#161237),
(#161238,#161239),(#161240,#161241),(#161242,#161243),(#161244,#161245),
(#161246,#161247),(#161248,#161249),(#161250,#161251),(#161252,#161253),
(#161254,#161255),(#161256,#161257),(#161258,#161259),(#161260,#161261),
(#161262,#161263),(#161264,#161265),(#161266,#161267),(#161268,#161269),
(#161270,#161271),(#161272,#161273),(#161274,#161275),(#161276,#161277),
(#161278,#161279),(#161280,#161281),(#161282,#161283),(#161284,#161285),
(#161286,#161287),(#161288,#161289),(#161290,#161291),(#161292,#161293),
(#161294,#161295),(#161296,#161297),(#161298,#161299),(#161300,#161301),
(#161302,#161303),(#161304,#161305),(#161306,#161307),(#161308,#161309),
(#161310,#161311),(#161312,#161313),(#161314,#161315),(#161316,#161317),
(#161318,#161319),(#161320,#161321),(#161322,#161323),(#161324,#161325),
(#161326,#161327),(#161328,#161329),(#161330,#161331),(#161332,#161333),
(#161334,#161335),(#161336,#161337),(#161338,#161339),(#161340,#161341),
(#161342,#161343),(#161344,#161345),(#161346,#161347),(#161348,#161349),
(#161350,#161351),(#161352,#161353),(#161354,#161355),(#161356,#161357),
(#161358,#161359),(#161360,#161361),(#161362,#161363),(#161364,#161365),
(#161366,#161367),(#161368,#161369),(#161370,#161371),(#161372,#161373),
(#161374,#161375),(#161376,#161377),(#161378,#161379),(#161380,#161381),
(#161382,#161383),(#161384,#161385),(#161386,#161387),(#161388,#161389),
(#161390,#161391),(#161392,#161393),(#161394,#161395),(#161396,#161397),
(#161398,#161399),(#161400,#161401),(#161402,#161403),(#161404,#161405),
(#161406,#161407),(#161408,#161409),(#161410,#161411),(#161412,#161413),
(#161414,#161415),(#161416,#161417),(#161418,#161419),(#161420,#161421),
(#161422,#161423),(#161424,#161425),(#161426,#161427),(#161428,#161429),
(#161430,#161431),(#161432,#161433),(#161434,#161435),(#161436,#161437),
(#161438,#161439),(#161440,#161441),(#161442,#161443),(#161444,#161445),
(#161446,#161447),(#161448,#161449),(#161450,#161451),(#161452,#161453),
(#161454,#161455),(#161456,#161457)),.UNSPECIFIED.,.F.,.F.,.F.)
B_SPLINE_SURFACE_WITH_KNOTS((6,1,1,1,1,1,1,1,1,1,1,1,1,1,1,1,1,1,1,1,1,
1,1,1,1,1,1,1,1,1,1,1,1,1,1,1,1,1,1,1,1,1,1,1,1,1,1,1,1,1,1,1,1,1,1,1,1,
1,1,1,1,1,1,1,1,1,1,1,1,1,1,1,1,1,1,1,1,1,1,1,1,1,1,1,1,1,1,1,1,1,1,1,1,
1,1,1,1,1,1,1,1,1,1,1,1,1,1,1,1,1,1,1,1,1,1,1,1,1,1,1,1,1,1,1,1,1,1,1,1,
1,1,1,1,1,1,1,1,1,1,1,1,1,1,1,1,1,1,1,1,1,1,1,1,1,1,1,1,1,1,1,1,1,1,1,1,
1,1,1,1,1,1,1,1,1,1,1,1,1,1,1,1,1,1,1,1,1,1,1,1,1,1,1,1,1,1,1,1,1,1,1,6),
(2,2),(-1.,-0.995000000000001,-0.990000000000001,-0.985000000000001,-0.980000000000001,
-0.975000000000001,-0.970000000000001,-0.965000000000001,-0.960000000000001,
-0.955000000000001,-0.950000000000001,-0.945000000000001,-0.940000000000001,
-0.935000000000001,-0.930000000000001,-0.925000000000001,-0.920000000000001,
-0.915000000000001,-0.910000000000001,-0.905000000000001,-0.900000000000001,
-0.895000000000001,-0.890000000000001,-0.885000000000001,-0.880000000000001,
-0.875000000000001,-0.870000000000001,-0.865000000000001,-0.860000000000001,
-0.855000000000001,-0.850000000000001,-0.845000000000001,-0.840000000000001,
-0.835000000000001,-0.830000000000001,-0.825000000000001,-0.820000000000001,
-0.815000000000001,-0.810000000000001,-0.805000000000001,-0.800000000000001,
-0.795000000000001,-0.790000000000001,-0.785000000000001,-0.780000000000001,
-0.775000000000001,-0.770000000000001,-0.765000000000001,-0.760000000000001,
-0.755000000000001,-0.750000000000001,-0.745000000000001,-0.740000000000001,
-0.735000000000001,-0.730000000000001,-0.725000000000001,-0.720000000000001,
-0.715000000000001,-0.710000000000001,-0.705000000000001,-0.700000000000001,
-0.695000000000001,-0.690000000000001,-0.685,-0.68,-0.675,-0.67,-0.665,
-0.66,-0.655,-0.65,-0.645,-0.64,-0.635,-0.63,-0.625,-0.62,-0.615,-0.61,
-0.605,-0.6,-0.595,-0.59,-0.585,-0.58,-0.575,-0.57,-0.565,-0.56,-0.555,
-0.55,-0.545,-0.54,-0.535,-0.53,-0.525,-0.52,-0.515,-0.51,-0.505,-0.5,-0.495,
-0.49,-0.485,-0.48,-0.475,-0.47,-0.465,-0.46,-0.455,-0.45,-0.445,-0.44,
-0.435,-0.43,-0.425,-0.42,-0.415,-0.41,-0.405,-0.4,-0.395,-0.39,-0.385,
-0.38,-0.375,-0.37,-0.365,-0.36,-0.355,-0.35,-0.345,-0.34,-0.335,-0.33,
-0.325,-0.32,-0.315,-0.31,-0.305,-0.3,-0.295,-0.29,-0.285,-0.28,-0.275,
-0.27,-0.265,-0.26,-0.255,-0.25,-0.245,-0.24,-0.235,-0.23,-0.225,-0.22,
-0.215,-0.21,-0.205,-0.2,-0.195,-0.19,-0.185,-0.18,-0.175,-0.17,-0.165,
-0.16,-0.155,-0.15,-0.145,-0.14,-0.135,-0.13,-0.125,-0.12,-0.115,-0.11,
-0.105,-0.1,-0.095,-0.09,-0.085,-0.08,-0.075,-0.07,-0.065,-0.06,-0.055,
-0.05,-0.045,-0.04,-0.035,-0.03,-0.025,-0.02,-0.015,-0.01,-0.005,0.),(0.,
1.2),.UNSPECIFIED.)
GEOMETRIC_REPRESENTATION_ITEM()
RATIONAL_B_SPLINE_SURFACE(((1.,1.),(1.,1.),(1.,1.),(1.,1.),(1.,1.),(1.,
1.),(1.,1.),(1.,1.),(1.,1.),(1.,1.),(1.,1.),(1.,1.),(1.,1.),(1.,1.),(1.,
1.),(1.,1.),(1.,1.),(1.,1.),(1.,1.),(1.,1.),(1.,1.),(1.,1.),(1.,1.),(1.,
1.),(1.,1.),(1.,1.),(1.,1.),(1.,1.),(1.,1.),(1.,1.),(1.,1.),(1.,1.),(1.,
1.),(1.,1.),(1.,1.),(1.,1.),(1.,1.),(1.,1.),(1.,1.),(1.,1.),(1.,1.),(1.,
1.),(1.,1.),(1.,1.),(1.,1.),(1.,1.),(1.,1.),(1.,1.),(1.,1.),(1.,1.),(1.,
1.),(1.,1.),(1.,1.),(1.,1.),(1.,1.),(1.,1.),(1.,1.),(1.,1.),(1.,1.),(1.,
1.),(1.,1.),(1.,1.),(1.,1.),(1.,1.),(1.,1.),(1.,1.),(1.,1.),(1.,1.),(1.,
1.),(1.,1.),(1.,1.),(1.,1.),(1.,1.),(1.,1.),(1.,1.),(1.,1.),(1.,1.),(1.,
1.),(1.,1.),(1.,1.),(1.,1.),(1.,1.),(1.,1.),(1.,1.),(1.,1.),(1.,1.),(1.,
1.),(1.,1.),(1.,1.),(1.,1.),(1.,1.),(1.,1.),(1.,1.),(1.,1.),(1.,1.),(1.,
1.),(1.,1.),(1.,1.),(1.,1.),(1.,1.),(1.,1.),(1.,1.),(1.,1.),(1.,1.),(1.,
1.),(1.,1.),(1.,1.),(1.,1.),(1.,1.),(1.,1.),(1.,1.),(1.,1.),(1.,1.),(1.,
1.),(1.,1.),(1.,1.),(1.,1.),(1.,1.),(1.,1.),(1.,1.),(1.,1.),(1.,1.),(1.,
1.),(1.,1.),(1.,1.),(1.,1.),(1.,1.),(1.,1.),(1.,1.),(1.,1.),(1.,1.),(1.,
1.),(1.,1.),(1.,1.),(1.,1.),(1.,1.),(1.,1.),(1.,1.),(1.,1.),(1.,1.),(1.,
1.),(1.,1.),(1.,1.),(1.,1.),(1.,1.),(1.,1.),(1.,1.),(1.,1.),(1.,1.),(1.,
1.),(1.,1.),(1.,1.),(1.,1.),(1.,1.),(1.,1.),(1.,1.),(1.,1.),(1.,1.),(1.,
1.),(1.,1.),(1.,1.),(1.,1.),(1.,1.),(1.,1.),(1.,1.),(1.,1.),(1.,1.),(1.,
1.),(1.,1.),(1.,1.),(1.,1.),(1.,1.),(1.,1.),(1.,1.),(1.,1.),(1.,1.),(1.,
1.),(1.,1.),(1.,1.),(1.,1.),(1.,1.),(1.,1.),(1.,1.),(1.,1.),(1.,1.),(1.,
1.),(1.,1.),(1.,1.),(1.,1.),(1.,1.),(1.,1.),(1.,1.),(1.,1.),(1.,1.),(1.,
1.),(1.,1.),(1.,1.),(1.,1.),(1.,1.),(1.,1.),(1.,1.),(1.,1.),(1.,1.),(1.,
1.),(1.,1.)))
REPRESENTATION_ITEM('')
SURFACE()
);
#1011=(
BOUNDED_SURFACE()
B_SPLINE_SURFACE(5,1,((#161849,#161850),(#161851,#161852),(#161853,#161854),
(#161855,#161856),(#161857,#161858),(#161859,#161860),(#161861,#161862),
(#161863,#161864),(#161865,#161866),(#161867,#161868),(#161869,#161870),
(#161871,#161872),(#161873,#161874),(#161875,#161876),(#161877,#161878),
(#161879,#161880),(#161881,#161882),(#161883,#161884),(#161885,#161886),
(#161887,#161888),(#161889,#161890),(#161891,#161892),(#161893,#161894),
(#161895,#161896),(#161897,#161898),(#161899,#161900),(#161901,#161902),
(#161903,#161904),(#161905,#161906),(#161907,#161908),(#161909,#161910),
(#161911,#161912),(#161913,#161914),(#161915,#161916),(#161917,#161918),
(#161919,#161920),(#161921,#161922),(#161923,#161924),(#161925,#161926),
(#161927,#161928),(#161929,#161930),(#161931,#161932),(#161933,#161934),
(#161935,#161936),(#161937,#161938),(#161939,#161940),(#161941,#161942),
(#161943,#161944),(#161945,#161946),(#161947,#161948),(#161949,#161950),
(#161951,#161952),(#161953,#161954),(#161955,#161956),(#161957,#161958),
(#161959,#161960),(#161961,#161962),(#161963,#161964),(#161965,#161966),
(#161967,#161968),(#161969,#161970),(#161971,#161972),(#161973,#161974),
(#161975,#161976),(#161977,#161978),(#161979,#161980),(#161981,#161982),
(#161983,#161984),(#161985,#161986),(#161987,#161988),(#161989,#161990),
(#161991,#161992),(#161993,#161994),(#161995,#161996),(#161997,#161998),
(#161999,#162000),(#162001,#162002),(#162003,#162004),(#162005,#162006),
(#162007,#162008),(#162009,#162010),(#162011,#162012),(#162013,#162014),
(#162015,#162016),(#162017,#162018),(#162019,#162020),(#162021,#162022),
(#162023,#162024),(#162025,#162026),(#162027,#162028),(#162029,#162030),
(#162031,#162032),(#162033,#162034),(#162035,#162036),(#162037,#162038),
(#162039,#162040),(#162041,#162042),(#162043,#162044),(#162045,#162046),
(#162047,#162048),(#162049,#162050),(#162051,#162052),(#162053,#162054),
(#162055,#162056),(#162057,#162058),(#162059,#162060),(#162061,#162062),
(#162063,#162064),(#162065,#162066),(#162067,#162068),(#162069,#162070),
(#162071,#162072),(#162073,#162074),(#162075,#162076),(#162077,#162078),
(#162079,#162080),(#162081,#162082),(#162083,#162084),(#162085,#162086),
(#162087,#162088),(#162089,#162090),(#162091,#162092),(#162093,#162094),
(#162095,#162096),(#162097,#162098),(#162099,#162100),(#162101,#162102),
(#162103,#162104),(#162105,#162106),(#162107,#162108),(#162109,#162110),
(#162111,#162112),(#162113,#162114),(#162115,#162116),(#162117,#162118),
(#162119,#162120),(#162121,#162122),(#162123,#162124),(#162125,#162126),
(#162127,#162128),(#162129,#162130),(#162131,#162132),(#162133,#162134),
(#162135,#162136),(#162137,#162138),(#162139,#162140),(#162141,#162142),
(#162143,#162144),(#162145,#162146),(#162147,#162148),(#162149,#162150),
(#162151,#162152),(#162153,#162154),(#162155,#162156),(#162157,#162158),
(#162159,#162160),(#162161,#162162),(#162163,#162164),(#162165,#162166),
(#162167,#162168),(#162169,#162170),(#162171,#162172),(#162173,#162174),
(#162175,#162176),(#162177,#162178),(#162179,#162180),(#162181,#162182),
(#162183,#162184),(#162185,#162186),(#162187,#162188),(#162189,#162190),
(#162191,#162192),(#162193,#162194),(#162195,#162196),(#162197,#162198),
(#162199,#162200),(#162201,#162202),(#162203,#162204),(#162205,#162206),
(#162207,#162208),(#162209,#162210),(#162211,#162212),(#162213,#162214),
(#162215,#162216),(#162217,#162218),(#162219,#162220),(#162221,#162222),
(#162223,#162224),(#162225,#162226),(#162227,#162228),(#162229,#162230),
(#162231,#162232),(#162233,#162234),(#162235,#162236),(#162237,#162238),
(#162239,#162240),(#162241,#162242),(#162243,#162244),(#162245,#162246),
(#162247,#162248),(#162249,#162250),(#162251,#162252),(#162253,#162254),
(#162255,#162256),(#162257,#162258)),.UNSPECIFIED.,.F.,.F.,.F.)
B_SPLINE_SURFACE_WITH_KNOTS((6,1,1,1,1,1,1,1,1,1,1,1,1,1,1,1,1,1,1,1,1,
1,1,1,1,1,1,1,1,1,1,1,1,1,1,1,1,1,1,1,1,1,1,1,1,1,1,1,1,1,1,1,1,1,1,1,1,
1,1,1,1,1,1,1,1,1,1,1,1,1,1,1,1,1,1,1,1,1,1,1,1,1,1,1,1,1,1,1,1,1,1,1,1,
1,1,1,1,1,1,1,1,1,1,1,1,1,1,1,1,1,1,1,1,1,1,1,1,1,1,1,1,1,1,1,1,1,1,1,1,
1,1,1,1,1,1,1,1,1,1,1,1,1,1,1,1,1,1,1,1,1,1,1,1,1,1,1,1,1,1,1,1,1,1,1,1,
1,1,1,1,1,1,1,1,1,1,1,1,1,1,1,1,1,1,1,1,1,1,1,1,1,1,1,1,1,1,1,1,1,1,1,6),
(2,2),(-1.,-0.995000000000001,-0.990000000000001,-0.985000000000001,-0.980000000000001,
-0.975000000000001,-0.970000000000001,-0.965000000000001,-0.960000000000001,
-0.955000000000001,-0.950000000000001,-0.945000000000001,-0.940000000000001,
-0.935000000000001,-0.930000000000001,-0.925000000000001,-0.920000000000001,
-0.915000000000001,-0.910000000000001,-0.905000000000001,-0.900000000000001,
-0.895000000000001,-0.890000000000001,-0.885000000000001,-0.880000000000001,
-0.875000000000001,-0.870000000000001,-0.865000000000001,-0.860000000000001,
-0.855000000000001,-0.850000000000001,-0.845000000000001,-0.840000000000001,
-0.835000000000001,-0.830000000000001,-0.825000000000001,-0.820000000000001,
-0.815000000000001,-0.810000000000001,-0.805000000000001,-0.800000000000001,
-0.795000000000001,-0.790000000000001,-0.785000000000001,-0.780000000000001,
-0.775000000000001,-0.770000000000001,-0.765000000000001,-0.760000000000001,
-0.755000000000001,-0.750000000000001,-0.745000000000001,-0.740000000000001,
-0.735000000000001,-0.730000000000001,-0.725000000000001,-0.720000000000001,
-0.715000000000001,-0.710000000000001,-0.705000000000001,-0.700000000000001,
-0.695000000000001,-0.690000000000001,-0.685,-0.68,-0.675,-0.67,-0.665,
-0.66,-0.655,-0.65,-0.645,-0.64,-0.635,-0.63,-0.625,-0.62,-0.615,-0.61,
-0.605,-0.6,-0.595,-0.59,-0.585,-0.58,-0.575,-0.57,-0.565,-0.56,-0.555,
-0.55,-0.545,-0.54,-0.535,-0.53,-0.525,-0.52,-0.515,-0.51,-0.505,-0.5,-0.495,
-0.49,-0.485,-0.48,-0.475,-0.47,-0.465,-0.46,-0.455,-0.45,-0.445,-0.44,
-0.435,-0.43,-0.425,-0.42,-0.415,-0.41,-0.405,-0.4,-0.395,-0.39,-0.385,
-0.38,-0.375,-0.37,-0.365,-0.36,-0.355,-0.35,-0.345,-0.34,-0.335,-0.33,
-0.325,-0.32,-0.315,-0.31,-0.305,-0.3,-0.295,-0.29,-0.285,-0.28,-0.275,
-0.27,-0.265,-0.26,-0.255,-0.25,-0.245,-0.24,-0.235,-0.23,-0.225,-0.22,
-0.215,-0.21,-0.205,-0.2,-0.195,-0.19,-0.185,-0.18,-0.175,-0.17,-0.165,
-0.16,-0.155,-0.15,-0.145,-0.14,-0.135,-0.13,-0.125,-0.12,-0.115,-0.11,
-0.105,-0.1,-0.095,-0.09,-0.085,-0.08,-0.075,-0.07,-0.065,-0.06,-0.055,
-0.05,-0.045,-0.04,-0.035,-0.03,-0.025,-0.02,-0.015,-0.01,-0.005,0.),(0.,
1.2),.UNSPECIFIED.)
GEOMETRIC_REPRESENTATION_ITEM()
RATIONAL_B_SPLINE_SURFACE(((1.,1.),(1.,1.),(1.,1.),(1.,1.),(1.,1.),(1.,
1.),(1.,1.),(1.,1.),(1.,1.),(1.,1.),(1.,1.),(1.,1.),(1.,1.),(1.,1.),(1.,
1.),(1.,1.),(1.,1.),(1.,1.),(1.,1.),(1.,1.),(1.,1.),(1.,1.),(1.,1.),(1.,
1.),(1.,1.),(1.,1.),(1.,1.),(1.,1.),(1.,1.),(1.,1.),(1.,1.),(1.,1.),(1.,
1.),(1.,1.),(1.,1.),(1.,1.),(1.,1.),(1.,1.),(1.,1.),(1.,1.),(1.,1.),(1.,
1.),(1.,1.),(1.,1.),(1.,1.),(1.,1.),(1.,1.),(1.,1.),(1.,1.),(1.,1.),(1.,
1.),(1.,1.),(1.,1.),(1.,1.),(1.,1.),(1.,1.),(1.,1.),(1.,1.),(1.,1.),(1.,
1.),(1.,1.),(1.,1.),(1.,1.),(1.,1.),(1.,1.),(1.,1.),(1.,1.),(1.,1.),(1.,
1.),(1.,1.),(1.,1.),(1.,1.),(1.,1.),(1.,1.),(1.,1.),(1.,1.),(1.,1.),(1.,
1.),(1.,1.),(1.,1.),(1.,1.),(1.,1.),(1.,1.),(1.,1.),(1.,1.),(1.,1.),(1.,
1.),(1.,1.),(1.,1.),(1.,1.),(1.,1.),(1.,1.),(1.,1.),(1.,1.),(1.,1.),(1.,
1.),(1.,1.),(1.,1.),(1.,1.),(1.,1.),(1.,1.),(1.,1.),(1.,1.),(1.,1.),(1.,
1.),(1.,1.),(1.,1.),(1.,1.),(1.,1.),(1.,1.),(1.,1.),(1.,1.),(1.,1.),(1.,
1.),(1.,1.),(1.,1.),(1.,1.),(1.,1.),(1.,1.),(1.,1.),(1.,1.),(1.,1.),(1.,
1.),(1.,1.),(1.,1.),(1.,1.),(1.,1.),(1.,1.),(1.,1.),(1.,1.),(1.,1.),(1.,
1.),(1.,1.),(1.,1.),(1.,1.),(1.,1.),(1.,1.),(1.,1.),(1.,1.),(1.,1.),(1.,
1.),(1.,1.),(1.,1.),(1.,1.),(1.,1.),(1.,1.),(1.,1.),(1.,1.),(1.,1.),(1.,
1.),(1.,1.),(1.,1.),(1.,1.),(1.,1.),(1.,1.),(1.,1.),(1.,1.),(1.,1.),(1.,
1.),(1.,1.),(1.,1.),(1.,1.),(1.,1.),(1.,1.),(1.,1.),(1.,1.),(1.,1.),(1.,
1.),(1.,1.),(1.,1.),(1.,1.),(1.,1.),(1.,1.),(1.,1.),(1.,1.),(1.,1.),(1.,
1.),(1.,1.),(1.,1.),(1.,1.),(1.,1.),(1.,1.),(1.,1.),(1.,1.),(1.,1.),(1.,
1.),(1.,1.),(1.,1.),(1.,1.),(1.,1.),(1.,1.),(1.,1.),(1.,1.),(1.,1.),(1.,
1.),(1.,1.),(1.,1.),(1.,1.),(1.,1.),(1.,1.),(1.,1.),(1.,1.),(1.,1.),(1.,
1.),(1.,1.)))
REPRESENTATION_ITEM('')
SURFACE()
);
#1012=(
BOUNDED_SURFACE()
B_SPLINE_SURFACE(5,1,((#162650,#162651),(#162652,#162653),(#162654,#162655),
(#162656,#162657),(#162658,#162659),(#162660,#162661),(#162662,#162663),
(#162664,#162665),(#162666,#162667),(#162668,#162669),(#162670,#162671),
(#162672,#162673),(#162674,#162675),(#162676,#162677),(#162678,#162679),
(#162680,#162681),(#162682,#162683),(#162684,#162685),(#162686,#162687),
(#162688,#162689),(#162690,#162691),(#162692,#162693),(#162694,#162695),
(#162696,#162697),(#162698,#162699),(#162700,#162701),(#162702,#162703),
(#162704,#162705),(#162706,#162707),(#162708,#162709),(#162710,#162711),
(#162712,#162713),(#162714,#162715),(#162716,#162717),(#162718,#162719),
(#162720,#162721),(#162722,#162723),(#162724,#162725),(#162726,#162727),
(#162728,#162729),(#162730,#162731),(#162732,#162733),(#162734,#162735),
(#162736,#162737),(#162738,#162739),(#162740,#162741),(#162742,#162743),
(#162744,#162745),(#162746,#162747),(#162748,#162749),(#162750,#162751),
(#162752,#162753),(#162754,#162755),(#162756,#162757),(#162758,#162759),
(#162760,#162761),(#162762,#162763),(#162764,#162765),(#162766,#162767),
(#162768,#162769),(#162770,#162771),(#162772,#162773),(#162774,#162775),
(#162776,#162777),(#162778,#162779),(#162780,#162781),(#162782,#162783),
(#162784,#162785),(#162786,#162787),(#162788,#162789),(#162790,#162791),
(#162792,#162793),(#162794,#162795),(#162796,#162797),(#162798,#162799),
(#162800,#162801),(#162802,#162803),(#162804,#162805),(#162806,#162807),
(#162808,#162809),(#162810,#162811),(#162812,#162813),(#162814,#162815),
(#162816,#162817),(#162818,#162819),(#162820,#162821),(#162822,#162823),
(#162824,#162825),(#162826,#162827),(#162828,#162829),(#162830,#162831),
(#162832,#162833),(#162834,#162835),(#162836,#162837),(#162838,#162839),
(#162840,#162841),(#162842,#162843),(#162844,#162845),(#162846,#162847),
(#162848,#162849),(#162850,#162851),(#162852,#162853),(#162854,#162855),
(#162856,#162857),(#162858,#162859),(#162860,#162861),(#162862,#162863),
(#162864,#162865),(#162866,#162867),(#162868,#162869),(#162870,#162871),
(#162872,#162873),(#162874,#162875),(#162876,#162877),(#162878,#162879),
(#162880,#162881),(#162882,#162883),(#162884,#162885),(#162886,#162887),
(#162888,#162889),(#162890,#162891),(#162892,#162893),(#162894,#162895),
(#162896,#162897),(#162898,#162899),(#162900,#162901),(#162902,#162903),
(#162904,#162905),(#162906,#162907),(#162908,#162909),(#162910,#162911),
(#162912,#162913),(#162914,#162915),(#162916,#162917),(#162918,#162919),
(#162920,#162921),(#162922,#162923),(#162924,#162925),(#162926,#162927),
(#162928,#162929),(#162930,#162931),(#162932,#162933),(#162934,#162935),
(#162936,#162937),(#162938,#162939),(#162940,#162941),(#162942,#162943),
(#162944,#162945),(#162946,#162947),(#162948,#162949),(#162950,#162951),
(#162952,#162953),(#162954,#162955),(#162956,#162957),(#162958,#162959),
(#162960,#162961),(#162962,#162963),(#162964,#162965),(#162966,#162967),
(#162968,#162969),(#162970,#162971),(#162972,#162973),(#162974,#162975),
(#162976,#162977),(#162978,#162979),(#162980,#162981),(#162982,#162983),
(#162984,#162985),(#162986,#162987),(#162988,#162989),(#162990,#162991),
(#162992,#162993),(#162994,#162995),(#162996,#162997),(#162998,#162999),
(#163000,#163001),(#163002,#163003),(#163004,#163005),(#163006,#163007),
(#163008,#163009),(#163010,#163011),(#163012,#163013),(#163014,#163015),
(#163016,#163017),(#163018,#163019),(#163020,#163021),(#163022,#163023),
(#163024,#163025),(#163026,#163027),(#163028,#163029),(#163030,#163031),
(#163032,#163033),(#163034,#163035),(#163036,#163037),(#163038,#163039),
(#163040,#163041),(#163042,#163043),(#163044,#163045),(#163046,#163047),
(#163048,#163049),(#163050,#163051),(#163052,#163053),(#163054,#163055),
(#163056,#163057),(#163058,#163059)),.UNSPECIFIED.,.F.,.F.,.F.)
B_SPLINE_SURFACE_WITH_KNOTS((6,1,1,1,1,1,1,1,1,1,1,1,1,1,1,1,1,1,1,1,1,
1,1,1,1,1,1,1,1,1,1,1,1,1,1,1,1,1,1,1,1,1,1,1,1,1,1,1,1,1,1,1,1,1,1,1,1,
1,1,1,1,1,1,1,1,1,1,1,1,1,1,1,1,1,1,1,1,1,1,1,1,1,1,1,1,1,1,1,1,1,1,1,1,
1,1,1,1,1,1,1,1,1,1,1,1,1,1,1,1,1,1,1,1,1,1,1,1,1,1,1,1,1,1,1,1,1,1,1,1,
1,1,1,1,1,1,1,1,1,1,1,1,1,1,1,1,1,1,1,1,1,1,1,1,1,1,1,1,1,1,1,1,1,1,1,1,
1,1,1,1,1,1,1,1,1,1,1,1,1,1,1,1,1,1,1,1,1,1,1,1,1,1,1,1,1,1,1,1,1,1,1,6),
(2,2),(-1.,-0.995000000000001,-0.990000000000001,-0.985000000000001,-0.980000000000001,
-0.975000000000001,-0.970000000000001,-0.965000000000001,-0.960000000000001,
-0.955000000000001,-0.950000000000001,-0.945000000000001,-0.940000000000001,
-0.935000000000001,-0.930000000000001,-0.925000000000001,-0.920000000000001,
-0.915000000000001,-0.910000000000001,-0.905000000000001,-0.900000000000001,
-0.895000000000001,-0.890000000000001,-0.885000000000001,-0.880000000000001,
-0.875000000000001,-0.870000000000001,-0.865000000000001,-0.860000000000001,
-0.855000000000001,-0.850000000000001,-0.845000000000001,-0.840000000000001,
-0.835000000000001,-0.830000000000001,-0.825000000000001,-0.820000000000001,
-0.815000000000001,-0.810000000000001,-0.805000000000001,-0.800000000000001,
-0.795000000000001,-0.790000000000001,-0.785000000000001,-0.780000000000001,
-0.775000000000001,-0.770000000000001,-0.765000000000001,-0.760000000000001,
-0.755000000000001,-0.750000000000001,-0.745000000000001,-0.740000000000001,
-0.735000000000001,-0.730000000000001,-0.725000000000001,-0.720000000000001,
-0.715000000000001,-0.710000000000001,-0.705000000000001,-0.700000000000001,
-0.695000000000001,-0.690000000000001,-0.685,-0.68,-0.675,-0.67,-0.665,
-0.66,-0.655,-0.65,-0.645,-0.64,-0.635,-0.63,-0.625,-0.62,-0.615,-0.61,
-0.605,-0.6,-0.595,-0.59,-0.585,-0.58,-0.575,-0.57,-0.565,-0.56,-0.555,
-0.55,-0.545,-0.54,-0.535,-0.53,-0.525,-0.52,-0.515,-0.51,-0.505,-0.5,-0.495,
-0.49,-0.485,-0.48,-0.475,-0.47,-0.465,-0.46,-0.455,-0.45,-0.445,-0.44,
-0.435,-0.43,-0.425,-0.42,-0.415,-0.41,-0.405,-0.4,-0.395,-0.39,-0.385,
-0.38,-0.375,-0.37,-0.365,-0.36,-0.355,-0.35,-0.345,-0.34,-0.335,-0.33,
-0.325,-0.32,-0.315,-0.31,-0.305,-0.3,-0.295,-0.29,-0.285,-0.28,-0.275,
-0.27,-0.265,-0.26,-0.255,-0.25,-0.245,-0.24,-0.235,-0.23,-0.225,-0.22,
-0.215,-0.21,-0.205,-0.2,-0.195,-0.19,-0.185,-0.18,-0.175,-0.17,-0.165,
-0.16,-0.155,-0.15,-0.145,-0.14,-0.135,-0.13,-0.125,-0.12,-0.115,-0.11,
-0.105,-0.1,-0.095,-0.09,-0.085,-0.08,-0.075,-0.07,-0.065,-0.06,-0.055,
-0.05,-0.045,-0.04,-0.035,-0.03,-0.025,-0.02,-0.015,-0.01,-0.005,0.),(0.,
1.2),.UNSPECIFIED.)
GEOMETRIC_REPRESENTATION_ITEM()
RATIONAL_B_SPLINE_SURFACE(((1.,1.),(1.,1.),(1.,1.),(1.,1.),(1.,1.),(1.,
1.),(1.,1.),(1.,1.),(1.,1.),(1.,1.),(1.,1.),(1.,1.),(1.,1.),(1.,1.),(1.,
1.),(1.,1.),(1.,1.),(1.,1.),(1.,1.),(1.,1.),(1.,1.),(1.,1.),(1.,1.),(1.,
1.),(1.,1.),(1.,1.),(1.,1.),(1.,1.),(1.,1.),(1.,1.),(1.,1.),(1.,1.),(1.,
1.),(1.,1.),(1.,1.),(1.,1.),(1.,1.),(1.,1.),(1.,1.),(1.,1.),(1.,1.),(1.,
1.),(1.,1.),(1.,1.),(1.,1.),(1.,1.),(1.,1.),(1.,1.),(1.,1.),(1.,1.),(1.,
1.),(1.,1.),(1.,1.),(1.,1.),(1.,1.),(1.,1.),(1.,1.),(1.,1.),(1.,1.),(1.,
1.),(1.,1.),(1.,1.),(1.,1.),(1.,1.),(1.,1.),(1.,1.),(1.,1.),(1.,1.),(1.,
1.),(1.,1.),(1.,1.),(1.,1.),(1.,1.),(1.,1.),(1.,1.),(1.,1.),(1.,1.),(1.,
1.),(1.,1.),(1.,1.),(1.,1.),(1.,1.),(1.,1.),(1.,1.),(1.,1.),(1.,1.),(1.,
1.),(1.,1.),(1.,1.),(1.,1.),(1.,1.),(1.,1.),(1.,1.),(1.,1.),(1.,1.),(1.,
1.),(1.,1.),(1.,1.),(1.,1.),(1.,1.),(1.,1.),(1.,1.),(1.,1.),(1.,1.),(1.,
1.),(1.,1.),(1.,1.),(1.,1.),(1.,1.),(1.,1.),(1.,1.),(1.,1.),(1.,1.),(1.,
1.),(1.,1.),(1.,1.),(1.,1.),(1.,1.),(1.,1.),(1.,1.),(1.,1.),(1.,1.),(1.,
1.),(1.,1.),(1.,1.),(1.,1.),(1.,1.),(1.,1.),(1.,1.),(1.,1.),(1.,1.),(1.,
1.),(1.,1.),(1.,1.),(1.,1.),(1.,1.),(1.,1.),(1.,1.),(1.,1.),(1.,1.),(1.,
1.),(1.,1.),(1.,1.),(1.,1.),(1.,1.),(1.,1.),(1.,1.),(1.,1.),(1.,1.),(1.,
1.),(1.,1.),(1.,1.),(1.,1.),(1.,1.),(1.,1.),(1.,1.),(1.,1.),(1.,1.),(1.,
1.),(1.,1.),(1.,1.),(1.,1.),(1.,1.),(1.,1.),(1.,1.),(1.,1.),(1.,1.),(1.,
1.),(1.,1.),(1.,1.),(1.,1.),(1.,1.),(1.,1.),(1.,1.),(1.,1.),(1.,1.),(1.,
1.),(1.,1.),(1.,1.),(1.,1.),(1.,1.),(1.,1.),(1.,1.),(1.,1.),(1.,1.),(1.,
1.),(1.,1.),(1.,1.),(1.,1.),(1.,1.),(1.,1.),(1.,1.),(1.,1.),(1.,1.),(1.,
1.),(1.,1.),(1.,1.),(1.,1.),(1.,1.),(1.,1.),(1.,1.),(1.,1.),(1.,1.),(1.,
1.),(1.,1.)))
REPRESENTATION_ITEM('')
SURFACE()
);
#1013=(
BOUNDED_SURFACE()
B_SPLINE_SURFACE(5,1,((#163451,#163452),(#163453,#163454),(#163455,#163456),
(#163457,#163458),(#163459,#163460),(#163461,#163462),(#163463,#163464),
(#163465,#163466),(#163467,#163468),(#163469,#163470),(#163471,#163472),
(#163473,#163474),(#163475,#163476),(#163477,#163478),(#163479,#163480),
(#163481,#163482),(#163483,#163484),(#163485,#163486),(#163487,#163488),
(#163489,#163490),(#163491,#163492),(#163493,#163494),(#163495,#163496),
(#163497,#163498),(#163499,#163500),(#163501,#163502),(#163503,#163504),
(#163505,#163506),(#163507,#163508),(#163509,#163510),(#163511,#163512),
(#163513,#163514),(#163515,#163516),(#163517,#163518),(#163519,#163520),
(#163521,#163522),(#163523,#163524),(#163525,#163526),(#163527,#163528),
(#163529,#163530),(#163531,#163532),(#163533,#163534),(#163535,#163536),
(#163537,#163538),(#163539,#163540),(#163541,#163542),(#163543,#163544),
(#163545,#163546),(#163547,#163548),(#163549,#163550),(#163551,#163552),
(#163553,#163554),(#163555,#163556),(#163557,#163558),(#163559,#163560),
(#163561,#163562),(#163563,#163564),(#163565,#163566),(#163567,#163568),
(#163569,#163570),(#163571,#163572),(#163573,#163574),(#163575,#163576),
(#163577,#163578),(#163579,#163580),(#163581,#163582),(#163583,#163584),
(#163585,#163586),(#163587,#163588),(#163589,#163590),(#163591,#163592),
(#163593,#163594),(#163595,#163596),(#163597,#163598),(#163599,#163600),
(#163601,#163602),(#163603,#163604),(#163605,#163606),(#163607,#163608),
(#163609,#163610),(#163611,#163612),(#163613,#163614),(#163615,#163616),
(#163617,#163618),(#163619,#163620),(#163621,#163622),(#163623,#163624),
(#163625,#163626),(#163627,#163628),(#163629,#163630),(#163631,#163632),
(#163633,#163634),(#163635,#163636),(#163637,#163638),(#163639,#163640),
(#163641,#163642),(#163643,#163644),(#163645,#163646),(#163647,#163648),
(#163649,#163650),(#163651,#163652),(#163653,#163654),(#163655,#163656),
(#163657,#163658),(#163659,#163660),(#163661,#163662),(#163663,#163664),
(#163665,#163666),(#163667,#163668),(#163669,#163670),(#163671,#163672),
(#163673,#163674),(#163675,#163676),(#163677,#163678),(#163679,#163680),
(#163681,#163682),(#163683,#163684),(#163685,#163686),(#163687,#163688),
(#163689,#163690),(#163691,#163692),(#163693,#163694),(#163695,#163696),
(#163697,#163698),(#163699,#163700),(#163701,#163702),(#163703,#163704),
(#163705,#163706),(#163707,#163708),(#163709,#163710),(#163711,#163712),
(#163713,#163714),(#163715,#163716),(#163717,#163718),(#163719,#163720),
(#163721,#163722),(#163723,#163724),(#163725,#163726),(#163727,#163728),
(#163729,#163730),(#163731,#163732),(#163733,#163734),(#163735,#163736),
(#163737,#163738),(#163739,#163740),(#163741,#163742),(#163743,#163744),
(#163745,#163746),(#163747,#163748),(#163749,#163750),(#163751,#163752),
(#163753,#163754),(#163755,#163756),(#163757,#163758),(#163759,#163760),
(#163761,#163762),(#163763,#163764),(#163765,#163766),(#163767,#163768),
(#163769,#163770),(#163771,#163772),(#163773,#163774),(#163775,#163776),
(#163777,#163778),(#163779,#163780),(#163781,#163782),(#163783,#163784),
(#163785,#163786),(#163787,#163788),(#163789,#163790),(#163791,#163792),
(#163793,#163794),(#163795,#163796),(#163797,#163798),(#163799,#163800),
(#163801,#163802),(#163803,#163804),(#163805,#163806),(#163807,#163808),
(#163809,#163810),(#163811,#163812),(#163813,#163814),(#163815,#163816),
(#163817,#163818),(#163819,#163820),(#163821,#163822),(#163823,#163824),
(#163825,#163826),(#163827,#163828),(#163829,#163830),(#163831,#163832),
(#163833,#163834),(#163835,#163836),(#163837,#163838),(#163839,#163840),
(#163841,#163842),(#163843,#163844),(#163845,#163846),(#163847,#163848),
(#163849,#163850),(#163851,#163852),(#163853,#163854),(#163855,#163856),
(#163857,#163858),(#163859,#163860)),.UNSPECIFIED.,.F.,.F.,.F.)
B_SPLINE_SURFACE_WITH_KNOTS((6,1,1,1,1,1,1,1,1,1,1,1,1,1,1,1,1,1,1,1,1,
1,1,1,1,1,1,1,1,1,1,1,1,1,1,1,1,1,1,1,1,1,1,1,1,1,1,1,1,1,1,1,1,1,1,1,1,
1,1,1,1,1,1,1,1,1,1,1,1,1,1,1,1,1,1,1,1,1,1,1,1,1,1,1,1,1,1,1,1,1,1,1,1,
1,1,1,1,1,1,1,1,1,1,1,1,1,1,1,1,1,1,1,1,1,1,1,1,1,1,1,1,1,1,1,1,1,1,1,1,
1,1,1,1,1,1,1,1,1,1,1,1,1,1,1,1,1,1,1,1,1,1,1,1,1,1,1,1,1,1,1,1,1,1,1,1,
1,1,1,1,1,1,1,1,1,1,1,1,1,1,1,1,1,1,1,1,1,1,1,1,1,1,1,1,1,1,1,1,1,1,1,6),
(2,2),(-1.,-0.995000000000001,-0.990000000000001,-0.985000000000001,-0.980000000000001,
-0.975000000000001,-0.970000000000001,-0.965000000000001,-0.960000000000001,
-0.955000000000001,-0.950000000000001,-0.945000000000001,-0.940000000000001,
-0.935000000000001,-0.930000000000001,-0.925000000000001,-0.920000000000001,
-0.915000000000001,-0.910000000000001,-0.905000000000001,-0.900000000000001,
-0.895000000000001,-0.890000000000001,-0.885000000000001,-0.880000000000001,
-0.875000000000001,-0.870000000000001,-0.865000000000001,-0.860000000000001,
-0.855000000000001,-0.850000000000001,-0.845000000000001,-0.840000000000001,
-0.835000000000001,-0.830000000000001,-0.825000000000001,-0.820000000000001,
-0.815000000000001,-0.810000000000001,-0.805000000000001,-0.800000000000001,
-0.795000000000001,-0.790000000000001,-0.785000000000001,-0.780000000000001,
-0.775000000000001,-0.770000000000001,-0.765000000000001,-0.760000000000001,
-0.755000000000001,-0.750000000000001,-0.745000000000001,-0.740000000000001,
-0.735000000000001,-0.730000000000001,-0.725000000000001,-0.720000000000001,
-0.715000000000001,-0.710000000000001,-0.705000000000001,-0.700000000000001,
-0.695000000000001,-0.690000000000001,-0.685,-0.68,-0.675,-0.67,-0.665,
-0.66,-0.655,-0.65,-0.645,-0.64,-0.635,-0.63,-0.625,-0.62,-0.615,-0.61,
-0.605,-0.6,-0.595,-0.59,-0.585,-0.58,-0.575,-0.57,-0.565,-0.56,-0.555,
-0.55,-0.545,-0.54,-0.535,-0.53,-0.525,-0.52,-0.515,-0.51,-0.505,-0.5,-0.495,
-0.49,-0.485,-0.48,-0.475,-0.47,-0.465,-0.46,-0.455,-0.45,-0.445,-0.44,
-0.435,-0.43,-0.425,-0.42,-0.415,-0.41,-0.405,-0.4,-0.395,-0.39,-0.385,
-0.38,-0.375,-0.37,-0.365,-0.36,-0.355,-0.35,-0.345,-0.34,-0.335,-0.33,
-0.325,-0.32,-0.315,-0.31,-0.305,-0.3,-0.295,-0.29,-0.285,-0.28,-0.275,
-0.27,-0.265,-0.26,-0.255,-0.25,-0.245,-0.24,-0.235,-0.23,-0.225,-0.22,
-0.215,-0.21,-0.205,-0.2,-0.195,-0.19,-0.185,-0.18,-0.175,-0.17,-0.165,
-0.16,-0.155,-0.15,-0.145,-0.14,-0.135,-0.13,-0.125,-0.12,-0.115,-0.11,
-0.105,-0.1,-0.095,-0.09,-0.085,-0.08,-0.075,-0.07,-0.065,-0.06,-0.055,
-0.05,-0.045,-0.04,-0.035,-0.03,-0.025,-0.02,-0.015,-0.01,-0.005,0.),(0.,
1.2),.UNSPECIFIED.)
GEOMETRIC_REPRESENTATION_ITEM()
RATIONAL_B_SPLINE_SURFACE(((1.,1.),(1.,1.),(1.,1.),(1.,1.),(1.,1.),(1.,
1.),(1.,1.),(1.,1.),(1.,1.),(1.,1.),(1.,1.),(1.,1.),(1.,1.),(1.,1.),(1.,
1.),(1.,1.),(1.,1.),(1.,1.),(1.,1.),(1.,1.),(1.,1.),(1.,1.),(1.,1.),(1.,
1.),(1.,1.),(1.,1.),(1.,1.),(1.,1.),(1.,1.),(1.,1.),(1.,1.),(1.,1.),(1.,
1.),(1.,1.),(1.,1.),(1.,1.),(1.,1.),(1.,1.),(1.,1.),(1.,1.),(1.,1.),(1.,
1.),(1.,1.),(1.,1.),(1.,1.),(1.,1.),(1.,1.),(1.,1.),(1.,1.),(1.,1.),(1.,
1.),(1.,1.),(1.,1.),(1.,1.),(1.,1.),(1.,1.),(1.,1.),(1.,1.),(1.,1.),(1.,
1.),(1.,1.),(1.,1.),(1.,1.),(1.,1.),(1.,1.),(1.,1.),(1.,1.),(1.,1.),(1.,
1.),(1.,1.),(1.,1.),(1.,1.),(1.,1.),(1.,1.),(1.,1.),(1.,1.),(1.,1.),(1.,
1.),(1.,1.),(1.,1.),(1.,1.),(1.,1.),(1.,1.),(1.,1.),(1.,1.),(1.,1.),(1.,
1.),(1.,1.),(1.,1.),(1.,1.),(1.,1.),(1.,1.),(1.,1.),(1.,1.),(1.,1.),(1.,
1.),(1.,1.),(1.,1.),(1.,1.),(1.,1.),(1.,1.),(1.,1.),(1.,1.),(1.,1.),(1.,
1.),(1.,1.),(1.,1.),(1.,1.),(1.,1.),(1.,1.),(1.,1.),(1.,1.),(1.,1.),(1.,
1.),(1.,1.),(1.,1.),(1.,1.),(1.,1.),(1.,1.),(1.,1.),(1.,1.),(1.,1.),(1.,
1.),(1.,1.),(1.,1.),(1.,1.),(1.,1.),(1.,1.),(1.,1.),(1.,1.),(1.,1.),(1.,
1.),(1.,1.),(1.,1.),(1.,1.),(1.,1.),(1.,1.),(1.,1.),(1.,1.),(1.,1.),(1.,
1.),(1.,1.),(1.,1.),(1.,1.),(1.,1.),(1.,1.),(1.,1.),(1.,1.),(1.,1.),(1.,
1.),(1.,1.),(1.,1.),(1.,1.),(1.,1.),(1.,1.),(1.,1.),(1.,1.),(1.,1.),(1.,
1.),(1.,1.),(1.,1.),(1.,1.),(1.,1.),(1.,1.),(1.,1.),(1.,1.),(1.,1.),(1.,
1.),(1.,1.),(1.,1.),(1.,1.),(1.,1.),(1.,1.),(1.,1.),(1.,1.),(1.,1.),(1.,
1.),(1.,1.),(1.,1.),(1.,1.),(1.,1.),(1.,1.),(1.,1.),(1.,1.),(1.,1.),(1.,
1.),(1.,1.),(1.,1.),(1.,1.),(1.,1.),(1.,1.),(1.,1.),(1.,1.),(1.,1.),(1.,
1.),(1.,1.),(1.,1.),(1.,1.),(1.,1.),(1.,1.),(1.,1.),(1.,1.),(1.,1.),(1.,
1.),(1.,1.)))
REPRESENTATION_ITEM('')
SURFACE()
);
#1014=(
BOUNDED_SURFACE()
B_SPLINE_SURFACE(5,1,((#164252,#164253),(#164254,#164255),(#164256,#164257),
(#164258,#164259),(#164260,#164261),(#164262,#164263),(#164264,#164265),
(#164266,#164267),(#164268,#164269),(#164270,#164271),(#164272,#164273),
(#164274,#164275),(#164276,#164277),(#164278,#164279),(#164280,#164281),
(#164282,#164283),(#164284,#164285),(#164286,#164287),(#164288,#164289),
(#164290,#164291),(#164292,#164293),(#164294,#164295),(#164296,#164297),
(#164298,#164299),(#164300,#164301),(#164302,#164303),(#164304,#164305),
(#164306,#164307),(#164308,#164309),(#164310,#164311),(#164312,#164313),
(#164314,#164315),(#164316,#164317),(#164318,#164319),(#164320,#164321),
(#164322,#164323),(#164324,#164325),(#164326,#164327),(#164328,#164329),
(#164330,#164331),(#164332,#164333),(#164334,#164335),(#164336,#164337),
(#164338,#164339),(#164340,#164341),(#164342,#164343),(#164344,#164345),
(#164346,#164347),(#164348,#164349),(#164350,#164351),(#164352,#164353),
(#164354,#164355),(#164356,#164357),(#164358,#164359),(#164360,#164361),
(#164362,#164363),(#164364,#164365),(#164366,#164367),(#164368,#164369),
(#164370,#164371),(#164372,#164373),(#164374,#164375),(#164376,#164377),
(#164378,#164379),(#164380,#164381),(#164382,#164383),(#164384,#164385),
(#164386,#164387),(#164388,#164389),(#164390,#164391),(#164392,#164393),
(#164394,#164395),(#164396,#164397),(#164398,#164399),(#164400,#164401),
(#164402,#164403),(#164404,#164405),(#164406,#164407),(#164408,#164409),
(#164410,#164411),(#164412,#164413),(#164414,#164415),(#164416,#164417),
(#164418,#164419),(#164420,#164421),(#164422,#164423),(#164424,#164425),
(#164426,#164427),(#164428,#164429),(#164430,#164431),(#164432,#164433),
(#164434,#164435),(#164436,#164437),(#164438,#164439),(#164440,#164441),
(#164442,#164443),(#164444,#164445),(#164446,#164447),(#164448,#164449),
(#164450,#164451),(#164452,#164453),(#164454,#164455),(#164456,#164457),
(#164458,#164459),(#164460,#164461),(#164462,#164463),(#164464,#164465),
(#164466,#164467),(#164468,#164469),(#164470,#164471),(#164472,#164473),
(#164474,#164475),(#164476,#164477),(#164478,#164479),(#164480,#164481),
(#164482,#164483),(#164484,#164485),(#164486,#164487),(#164488,#164489),
(#164490,#164491),(#164492,#164493),(#164494,#164495),(#164496,#164497),
(#164498,#164499),(#164500,#164501),(#164502,#164503),(#164504,#164505),
(#164506,#164507),(#164508,#164509),(#164510,#164511),(#164512,#164513),
(#164514,#164515),(#164516,#164517),(#164518,#164519),(#164520,#164521),
(#164522,#164523),(#164524,#164525),(#164526,#164527),(#164528,#164529),
(#164530,#164531),(#164532,#164533),(#164534,#164535),(#164536,#164537),
(#164538,#164539),(#164540,#164541),(#164542,#164543),(#164544,#164545),
(#164546,#164547),(#164548,#164549),(#164550,#164551),(#164552,#164553),
(#164554,#164555),(#164556,#164557),(#164558,#164559),(#164560,#164561),
(#164562,#164563),(#164564,#164565),(#164566,#164567),(#164568,#164569),
(#164570,#164571),(#164572,#164573),(#164574,#164575),(#164576,#164577),
(#164578,#164579),(#164580,#164581),(#164582,#164583),(#164584,#164585),
(#164586,#164587),(#164588,#164589),(#164590,#164591),(#164592,#164593),
(#164594,#164595),(#164596,#164597),(#164598,#164599),(#164600,#164601),
(#164602,#164603),(#164604,#164605),(#164606,#164607),(#164608,#164609),
(#164610,#164611),(#164612,#164613),(#164614,#164615),(#164616,#164617),
(#164618,#164619),(#164620,#164621),(#164622,#164623),(#164624,#164625),
(#164626,#164627),(#164628,#164629),(#164630,#164631),(#164632,#164633),
(#164634,#164635),(#164636,#164637),(#164638,#164639),(#164640,#164641),
(#164642,#164643),(#164644,#164645),(#164646,#164647),(#164648,#164649),
(#164650,#164651),(#164652,#164653),(#164654,#164655),(#164656,#164657),
(#164658,#164659),(#164660,#164661)),.UNSPECIFIED.,.F.,.F.,.F.)
B_SPLINE_SURFACE_WITH_KNOTS((6,1,1,1,1,1,1,1,1,1,1,1,1,1,1,1,1,1,1,1,1,
1,1,1,1,1,1,1,1,1,1,1,1,1,1,1,1,1,1,1,1,1,1,1,1,1,1,1,1,1,1,1,1,1,1,1,1,
1,1,1,1,1,1,1,1,1,1,1,1,1,1,1,1,1,1,1,1,1,1,1,1,1,1,1,1,1,1,1,1,1,1,1,1,
1,1,1,1,1,1,1,1,1,1,1,1,1,1,1,1,1,1,1,1,1,1,1,1,1,1,1,1,1,1,1,1,1,1,1,1,
1,1,1,1,1,1,1,1,1,1,1,1,1,1,1,1,1,1,1,1,1,1,1,1,1,1,1,1,1,1,1,1,1,1,1,1,
1,1,1,1,1,1,1,1,1,1,1,1,1,1,1,1,1,1,1,1,1,1,1,1,1,1,1,1,1,1,1,1,1,1,1,6),
(2,2),(-1.,-0.995000000000001,-0.990000000000001,-0.985000000000001,-0.980000000000001,
-0.975000000000001,-0.970000000000001,-0.965000000000001,-0.960000000000001,
-0.955000000000001,-0.950000000000001,-0.945000000000001,-0.940000000000001,
-0.935000000000001,-0.930000000000001,-0.925000000000001,-0.920000000000001,
-0.915000000000001,-0.910000000000001,-0.905000000000001,-0.900000000000001,
-0.895000000000001,-0.890000000000001,-0.885000000000001,-0.880000000000001,
-0.875000000000001,-0.870000000000001,-0.865000000000001,-0.860000000000001,
-0.855000000000001,-0.850000000000001,-0.845000000000001,-0.840000000000001,
-0.835000000000001,-0.830000000000001,-0.825000000000001,-0.820000000000001,
-0.815000000000001,-0.810000000000001,-0.805000000000001,-0.800000000000001,
-0.795000000000001,-0.790000000000001,-0.785000000000001,-0.780000000000001,
-0.775000000000001,-0.770000000000001,-0.765000000000001,-0.760000000000001,
-0.755000000000001,-0.750000000000001,-0.745000000000001,-0.740000000000001,
-0.735000000000001,-0.730000000000001,-0.725000000000001,-0.720000000000001,
-0.715000000000001,-0.710000000000001,-0.705000000000001,-0.700000000000001,
-0.695000000000001,-0.690000000000001,-0.685,-0.68,-0.675,-0.67,-0.665,
-0.66,-0.655,-0.65,-0.645,-0.64,-0.635,-0.63,-0.625,-0.62,-0.615,-0.61,
-0.605,-0.6,-0.595,-0.59,-0.585,-0.58,-0.575,-0.57,-0.565,-0.56,-0.555,
-0.55,-0.545,-0.54,-0.535,-0.53,-0.525,-0.52,-0.515,-0.51,-0.505,-0.5,-0.495,
-0.49,-0.485,-0.48,-0.475,-0.47,-0.465,-0.46,-0.455,-0.45,-0.445,-0.44,
-0.435,-0.43,-0.425,-0.42,-0.415,-0.41,-0.405,-0.4,-0.395,-0.39,-0.385,
-0.38,-0.375,-0.37,-0.365,-0.36,-0.355,-0.35,-0.345,-0.34,-0.335,-0.33,
-0.325,-0.32,-0.315,-0.31,-0.305,-0.3,-0.295,-0.29,-0.285,-0.28,-0.275,
-0.27,-0.265,-0.26,-0.255,-0.25,-0.245,-0.24,-0.235,-0.23,-0.225,-0.22,
-0.215,-0.21,-0.205,-0.2,-0.195,-0.19,-0.185,-0.18,-0.175,-0.17,-0.165,
-0.16,-0.155,-0.15,-0.145,-0.14,-0.135,-0.13,-0.125,-0.12,-0.115,-0.11,
-0.105,-0.1,-0.095,-0.09,-0.085,-0.08,-0.075,-0.07,-0.065,-0.06,-0.055,
-0.05,-0.045,-0.04,-0.035,-0.03,-0.025,-0.02,-0.015,-0.01,-0.005,0.),(0.,
1.2),.UNSPECIFIED.)
GEOMETRIC_REPRESENTATION_ITEM()
RATIONAL_B_SPLINE_SURFACE(((1.,1.),(1.,1.),(1.,1.),(1.,1.),(1.,1.),(1.,
1.),(1.,1.),(1.,1.),(1.,1.),(1.,1.),(1.,1.),(1.,1.),(1.,1.),(1.,1.),(1.,
1.),(1.,1.),(1.,1.),(1.,1.),(1.,1.),(1.,1.),(1.,1.),(1.,1.),(1.,1.),(1.,
1.),(1.,1.),(1.,1.),(1.,1.),(1.,1.),(1.,1.),(1.,1.),(1.,1.),(1.,1.),(1.,
1.),(1.,1.),(1.,1.),(1.,1.),(1.,1.),(1.,1.),(1.,1.),(1.,1.),(1.,1.),(1.,
1.),(1.,1.),(1.,1.),(1.,1.),(1.,1.),(1.,1.),(1.,1.),(1.,1.),(1.,1.),(1.,
1.),(1.,1.),(1.,1.),(1.,1.),(1.,1.),(1.,1.),(1.,1.),(1.,1.),(1.,1.),(1.,
1.),(1.,1.),(1.,1.),(1.,1.),(1.,1.),(1.,1.),(1.,1.),(1.,1.),(1.,1.),(1.,
1.),(1.,1.),(1.,1.),(1.,1.),(1.,1.),(1.,1.),(1.,1.),(1.,1.),(1.,1.),(1.,
1.),(1.,1.),(1.,1.),(1.,1.),(1.,1.),(1.,1.),(1.,1.),(1.,1.),(1.,1.),(1.,
1.),(1.,1.),(1.,1.),(1.,1.),(1.,1.),(1.,1.),(1.,1.),(1.,1.),(1.,1.),(1.,
1.),(1.,1.),(1.,1.),(1.,1.),(1.,1.),(1.,1.),(1.,1.),(1.,1.),(1.,1.),(1.,
1.),(1.,1.),(1.,1.),(1.,1.),(1.,1.),(1.,1.),(1.,1.),(1.,1.),(1.,1.),(1.,
1.),(1.,1.),(1.,1.),(1.,1.),(1.,1.),(1.,1.),(1.,1.),(1.,1.),(1.,1.),(1.,
1.),(1.,1.),(1.,1.),(1.,1.),(1.,1.),(1.,1.),(1.,1.),(1.,1.),(1.,1.),(1.,
1.),(1.,1.),(1.,1.),(1.,1.),(1.,1.),(1.,1.),(1.,1.),(1.,1.),(1.,1.),(1.,
1.),(1.,1.),(1.,1.),(1.,1.),(1.,1.),(1.,1.),(1.,1.),(1.,1.),(1.,1.),(1.,
1.),(1.,1.),(1.,1.),(1.,1.),(1.,1.),(1.,1.),(1.,1.),(1.,1.),(1.,1.),(1.,
1.),(1.,1.),(1.,1.),(1.,1.),(1.,1.),(1.,1.),(1.,1.),(1.,1.),(1.,1.),(1.,
1.),(1.,1.),(1.,1.),(1.,1.),(1.,1.),(1.,1.),(1.,1.),(1.,1.),(1.,1.),(1.,
1.),(1.,1.),(1.,1.),(1.,1.),(1.,1.),(1.,1.),(1.,1.),(1.,1.),(1.,1.),(1.,
1.),(1.,1.),(1.,1.),(1.,1.),(1.,1.),(1.,1.),(1.,1.),(1.,1.),(1.,1.),(1.,
1.),(1.,1.),(1.,1.),(1.,1.),(1.,1.),(1.,1.),(1.,1.),(1.,1.),(1.,1.),(1.,
1.),(1.,1.)))
REPRESENTATION_ITEM('')
SURFACE()
);
#1015=(
BOUNDED_SURFACE()
B_SPLINE_SURFACE(5,1,((#165053,#165054),(#165055,#165056),(#165057,#165058),
(#165059,#165060),(#165061,#165062),(#165063,#165064),(#165065,#165066),
(#165067,#165068),(#165069,#165070),(#165071,#165072),(#165073,#165074),
(#165075,#165076),(#165077,#165078),(#165079,#165080),(#165081,#165082),
(#165083,#165084),(#165085,#165086),(#165087,#165088),(#165089,#165090),
(#165091,#165092),(#165093,#165094),(#165095,#165096),(#165097,#165098),
(#165099,#165100),(#165101,#165102),(#165103,#165104),(#165105,#165106),
(#165107,#165108),(#165109,#165110),(#165111,#165112),(#165113,#165114),
(#165115,#165116),(#165117,#165118),(#165119,#165120),(#165121,#165122),
(#165123,#165124),(#165125,#165126),(#165127,#165128),(#165129,#165130),
(#165131,#165132),(#165133,#165134),(#165135,#165136),(#165137,#165138),
(#165139,#165140),(#165141,#165142),(#165143,#165144),(#165145,#165146),
(#165147,#165148),(#165149,#165150),(#165151,#165152),(#165153,#165154),
(#165155,#165156),(#165157,#165158),(#165159,#165160),(#165161,#165162),
(#165163,#165164),(#165165,#165166),(#165167,#165168),(#165169,#165170),
(#165171,#165172),(#165173,#165174),(#165175,#165176),(#165177,#165178),
(#165179,#165180),(#165181,#165182),(#165183,#165184),(#165185,#165186),
(#165187,#165188),(#165189,#165190),(#165191,#165192),(#165193,#165194),
(#165195,#165196),(#165197,#165198),(#165199,#165200),(#165201,#165202),
(#165203,#165204),(#165205,#165206),(#165207,#165208),(#165209,#165210),
(#165211,#165212),(#165213,#165214),(#165215,#165216),(#165217,#165218),
(#165219,#165220),(#165221,#165222),(#165223,#165224),(#165225,#165226),
(#165227,#165228),(#165229,#165230),(#165231,#165232),(#165233,#165234),
(#165235,#165236),(#165237,#165238),(#165239,#165240),(#165241,#165242),
(#165243,#165244),(#165245,#165246),(#165247,#165248),(#165249,#165250),
(#165251,#165252),(#165253,#165254),(#165255,#165256),(#165257,#165258),
(#165259,#165260),(#165261,#165262),(#165263,#165264),(#165265,#165266),
(#165267,#165268),(#165269,#165270),(#165271,#165272),(#165273,#165274),
(#165275,#165276),(#165277,#165278),(#165279,#165280),(#165281,#165282),
(#165283,#165284),(#165285,#165286),(#165287,#165288),(#165289,#165290),
(#165291,#165292),(#165293,#165294),(#165295,#165296),(#165297,#165298),
(#165299,#165300),(#165301,#165302),(#165303,#165304),(#165305,#165306),
(#165307,#165308),(#165309,#165310),(#165311,#165312),(#165313,#165314),
(#165315,#165316),(#165317,#165318),(#165319,#165320),(#165321,#165322),
(#165323,#165324),(#165325,#165326),(#165327,#165328),(#165329,#165330),
(#165331,#165332),(#165333,#165334),(#165335,#165336),(#165337,#165338),
(#165339,#165340),(#165341,#165342),(#165343,#165344),(#165345,#165346),
(#165347,#165348),(#165349,#165350),(#165351,#165352),(#165353,#165354),
(#165355,#165356),(#165357,#165358),(#165359,#165360),(#165361,#165362),
(#165363,#165364),(#165365,#165366),(#165367,#165368),(#165369,#165370),
(#165371,#165372),(#165373,#165374),(#165375,#165376),(#165377,#165378),
(#165379,#165380),(#165381,#165382),(#165383,#165384),(#165385,#165386),
(#165387,#165388),(#165389,#165390),(#165391,#165392),(#165393,#165394),
(#165395,#165396),(#165397,#165398),(#165399,#165400),(#165401,#165402),
(#165403,#165404),(#165405,#165406),(#165407,#165408),(#165409,#165410),
(#165411,#165412),(#165413,#165414),(#165415,#165416),(#165417,#165418),
(#165419,#165420),(#165421,#165422),(#165423,#165424),(#165425,#165426),
(#165427,#165428),(#165429,#165430),(#165431,#165432),(#165433,#165434),
(#165435,#165436),(#165437,#165438),(#165439,#165440),(#165441,#165442),
(#165443,#165444),(#165445,#165446),(#165447,#165448),(#165449,#165450),
(#165451,#165452),(#165453,#165454),(#165455,#165456),(#165457,#165458),
(#165459,#165460),(#165461,#165462)),.UNSPECIFIED.,.F.,.F.,.F.)
B_SPLINE_SURFACE_WITH_KNOTS((6,1,1,1,1,1,1,1,1,1,1,1,1,1,1,1,1,1,1,1,1,
1,1,1,1,1,1,1,1,1,1,1,1,1,1,1,1,1,1,1,1,1,1,1,1,1,1,1,1,1,1,1,1,1,1,1,1,
1,1,1,1,1,1,1,1,1,1,1,1,1,1,1,1,1,1,1,1,1,1,1,1,1,1,1,1,1,1,1,1,1,1,1,1,
1,1,1,1,1,1,1,1,1,1,1,1,1,1,1,1,1,1,1,1,1,1,1,1,1,1,1,1,1,1,1,1,1,1,1,1,
1,1,1,1,1,1,1,1,1,1,1,1,1,1,1,1,1,1,1,1,1,1,1,1,1,1,1,1,1,1,1,1,1,1,1,1,
1,1,1,1,1,1,1,1,1,1,1,1,1,1,1,1,1,1,1,1,1,1,1,1,1,1,1,1,1,1,1,1,1,1,1,6),
(2,2),(-1.,-0.995000000000001,-0.990000000000001,-0.985000000000001,-0.980000000000001,
-0.975000000000001,-0.970000000000001,-0.965000000000001,-0.960000000000001,
-0.955000000000001,-0.950000000000001,-0.945000000000001,-0.940000000000001,
-0.935000000000001,-0.930000000000001,-0.925000000000001,-0.920000000000001,
-0.915000000000001,-0.910000000000001,-0.905000000000001,-0.900000000000001,
-0.895000000000001,-0.890000000000001,-0.885000000000001,-0.880000000000001,
-0.875000000000001,-0.870000000000001,-0.865000000000001,-0.860000000000001,
-0.855000000000001,-0.850000000000001,-0.845000000000001,-0.840000000000001,
-0.835000000000001,-0.830000000000001,-0.825000000000001,-0.820000000000001,
-0.815000000000001,-0.810000000000001,-0.805000000000001,-0.800000000000001,
-0.795000000000001,-0.790000000000001,-0.785000000000001,-0.780000000000001,
-0.775000000000001,-0.770000000000001,-0.765000000000001,-0.760000000000001,
-0.755000000000001,-0.750000000000001,-0.745000000000001,-0.740000000000001,
-0.735000000000001,-0.730000000000001,-0.725000000000001,-0.720000000000001,
-0.715000000000001,-0.710000000000001,-0.705000000000001,-0.700000000000001,
-0.695000000000001,-0.690000000000001,-0.685,-0.68,-0.675,-0.67,-0.665,
-0.66,-0.655,-0.65,-0.645,-0.64,-0.635,-0.63,-0.625,-0.62,-0.615,-0.61,
-0.605,-0.6,-0.595,-0.59,-0.585,-0.58,-0.575,-0.57,-0.565,-0.56,-0.555,
-0.55,-0.545,-0.54,-0.535,-0.53,-0.525,-0.52,-0.515,-0.51,-0.505,-0.5,-0.495,
-0.49,-0.485,-0.48,-0.475,-0.47,-0.465,-0.46,-0.455,-0.45,-0.445,-0.44,
-0.435,-0.43,-0.425,-0.42,-0.415,-0.41,-0.405,-0.4,-0.395,-0.39,-0.385,
-0.38,-0.375,-0.37,-0.365,-0.36,-0.355,-0.35,-0.345,-0.34,-0.335,-0.33,
-0.325,-0.32,-0.315,-0.31,-0.305,-0.3,-0.295,-0.29,-0.285,-0.28,-0.275,
-0.27,-0.265,-0.26,-0.255,-0.25,-0.245,-0.24,-0.235,-0.23,-0.225,-0.22,
-0.215,-0.21,-0.205,-0.2,-0.195,-0.19,-0.185,-0.18,-0.175,-0.17,-0.165,
-0.16,-0.155,-0.15,-0.145,-0.14,-0.135,-0.13,-0.125,-0.12,-0.115,-0.11,
-0.105,-0.1,-0.095,-0.09,-0.085,-0.08,-0.075,-0.07,-0.065,-0.06,-0.055,
-0.05,-0.045,-0.04,-0.035,-0.03,-0.025,-0.02,-0.015,-0.01,-0.005,0.),(0.,
1.2),.UNSPECIFIED.)
GEOMETRIC_REPRESENTATION_ITEM()
RATIONAL_B_SPLINE_SURFACE(((1.,1.),(1.,1.),(1.,1.),(1.,1.),(1.,1.),(1.,
1.),(1.,1.),(1.,1.),(1.,1.),(1.,1.),(1.,1.),(1.,1.),(1.,1.),(1.,1.),(1.,
1.),(1.,1.),(1.,1.),(1.,1.),(1.,1.),(1.,1.),(1.,1.),(1.,1.),(1.,1.),(1.,
1.),(1.,1.),(1.,1.),(1.,1.),(1.,1.),(1.,1.),(1.,1.),(1.,1.),(1.,1.),(1.,
1.),(1.,1.),(1.,1.),(1.,1.),(1.,1.),(1.,1.),(1.,1.),(1.,1.),(1.,1.),(1.,
1.),(1.,1.),(1.,1.),(1.,1.),(1.,1.),(1.,1.),(1.,1.),(1.,1.),(1.,1.),(1.,
1.),(1.,1.),(1.,1.),(1.,1.),(1.,1.),(1.,1.),(1.,1.),(1.,1.),(1.,1.),(1.,
1.),(1.,1.),(1.,1.),(1.,1.),(1.,1.),(1.,1.),(1.,1.),(1.,1.),(1.,1.),(1.,
1.),(1.,1.),(1.,1.),(1.,1.),(1.,1.),(1.,1.),(1.,1.),(1.,1.),(1.,1.),(1.,
1.),(1.,1.),(1.,1.),(1.,1.),(1.,1.),(1.,1.),(1.,1.),(1.,1.),(1.,1.),(1.,
1.),(1.,1.),(1.,1.),(1.,1.),(1.,1.),(1.,1.),(1.,1.),(1.,1.),(1.,1.),(1.,
1.),(1.,1.),(1.,1.),(1.,1.),(1.,1.),(1.,1.),(1.,1.),(1.,1.),(1.,1.),(1.,
1.),(1.,1.),(1.,1.),(1.,1.),(1.,1.),(1.,1.),(1.,1.),(1.,1.),(1.,1.),(1.,
1.),(1.,1.),(1.,1.),(1.,1.),(1.,1.),(1.,1.),(1.,1.),(1.,1.),(1.,1.),(1.,
1.),(1.,1.),(1.,1.),(1.,1.),(1.,1.),(1.,1.),(1.,1.),(1.,1.),(1.,1.),(1.,
1.),(1.,1.),(1.,1.),(1.,1.),(1.,1.),(1.,1.),(1.,1.),(1.,1.),(1.,1.),(1.,
1.),(1.,1.),(1.,1.),(1.,1.),(1.,1.),(1.,1.),(1.,1.),(1.,1.),(1.,1.),(1.,
1.),(1.,1.),(1.,1.),(1.,1.),(1.,1.),(1.,1.),(1.,1.),(1.,1.),(1.,1.),(1.,
1.),(1.,1.),(1.,1.),(1.,1.),(1.,1.),(1.,1.),(1.,1.),(1.,1.),(1.,1.),(1.,
1.),(1.,1.),(1.,1.),(1.,1.),(1.,1.),(1.,1.),(1.,1.),(1.,1.),(1.,1.),(1.,
1.),(1.,1.),(1.,1.),(1.,1.),(1.,1.),(1.,1.),(1.,1.),(1.,1.),(1.,1.),(1.,
1.),(1.,1.),(1.,1.),(1.,1.),(1.,1.),(1.,1.),(1.,1.),(1.,1.),(1.,1.),(1.,
1.),(1.,1.),(1.,1.),(1.,1.),(1.,1.),(1.,1.),(1.,1.),(1.,1.),(1.,1.),(1.,
1.),(1.,1.)))
REPRESENTATION_ITEM('')
SURFACE()
);
#1016=(
BOUNDED_SURFACE()
B_SPLINE_SURFACE(5,1,((#165854,#165855),(#165856,#165857),(#165858,#165859),
(#165860,#165861),(#165862,#165863),(#165864,#165865),(#165866,#165867),
(#165868,#165869),(#165870,#165871),(#165872,#165873),(#165874,#165875),
(#165876,#165877),(#165878,#165879),(#165880,#165881),(#165882,#165883),
(#165884,#165885),(#165886,#165887),(#165888,#165889),(#165890,#165891),
(#165892,#165893),(#165894,#165895),(#165896,#165897),(#165898,#165899),
(#165900,#165901),(#165902,#165903),(#165904,#165905),(#165906,#165907),
(#165908,#165909),(#165910,#165911),(#165912,#165913),(#165914,#165915),
(#165916,#165917),(#165918,#165919),(#165920,#165921),(#165922,#165923),
(#165924,#165925),(#165926,#165927),(#165928,#165929),(#165930,#165931),
(#165932,#165933),(#165934,#165935),(#165936,#165937),(#165938,#165939),
(#165940,#165941),(#165942,#165943),(#165944,#165945),(#165946,#165947),
(#165948,#165949),(#165950,#165951),(#165952,#165953),(#165954,#165955),
(#165956,#165957),(#165958,#165959),(#165960,#165961),(#165962,#165963),
(#165964,#165965),(#165966,#165967),(#165968,#165969),(#165970,#165971),
(#165972,#165973),(#165974,#165975),(#165976,#165977),(#165978,#165979),
(#165980,#165981),(#165982,#165983),(#165984,#165985),(#165986,#165987),
(#165988,#165989),(#165990,#165991),(#165992,#165993),(#165994,#165995),
(#165996,#165997),(#165998,#165999),(#166000,#166001),(#166002,#166003),
(#166004,#166005),(#166006,#166007),(#166008,#166009),(#166010,#166011),
(#166012,#166013),(#166014,#166015),(#166016,#166017),(#166018,#166019),
(#166020,#166021),(#166022,#166023),(#166024,#166025),(#166026,#166027),
(#166028,#166029),(#166030,#166031),(#166032,#166033),(#166034,#166035),
(#166036,#166037),(#166038,#166039),(#166040,#166041),(#166042,#166043),
(#166044,#166045),(#166046,#166047),(#166048,#166049),(#166050,#166051),
(#166052,#166053),(#166054,#166055),(#166056,#166057),(#166058,#166059),
(#166060,#166061),(#166062,#166063),(#166064,#166065),(#166066,#166067),
(#166068,#166069),(#166070,#166071),(#166072,#166073),(#166074,#166075),
(#166076,#166077),(#166078,#166079),(#166080,#166081),(#166082,#166083),
(#166084,#166085),(#166086,#166087),(#166088,#166089),(#166090,#166091),
(#166092,#166093),(#166094,#166095),(#166096,#166097),(#166098,#166099),
(#166100,#166101),(#166102,#166103),(#166104,#166105),(#166106,#166107),
(#166108,#166109),(#166110,#166111),(#166112,#166113),(#166114,#166115),
(#166116,#166117),(#166118,#166119),(#166120,#166121),(#166122,#166123),
(#166124,#166125),(#166126,#166127),(#166128,#166129),(#166130,#166131),
(#166132,#166133),(#166134,#166135),(#166136,#166137),(#166138,#166139),
(#166140,#166141),(#166142,#166143),(#166144,#166145),(#166146,#166147),
(#166148,#166149),(#166150,#166151),(#166152,#166153),(#166154,#166155),
(#166156,#166157),(#166158,#166159),(#166160,#166161),(#166162,#166163),
(#166164,#166165),(#166166,#166167),(#166168,#166169),(#166170,#166171),
(#166172,#166173),(#166174,#166175),(#166176,#166177),(#166178,#166179),
(#166180,#166181),(#166182,#166183),(#166184,#166185),(#166186,#166187),
(#166188,#166189),(#166190,#166191),(#166192,#166193),(#166194,#166195),
(#166196,#166197),(#166198,#166199),(#166200,#166201),(#166202,#166203),
(#166204,#166205),(#166206,#166207),(#166208,#166209),(#166210,#166211),
(#166212,#166213),(#166214,#166215),(#166216,#166217),(#166218,#166219),
(#166220,#166221),(#166222,#166223),(#166224,#166225),(#166226,#166227),
(#166228,#166229),(#166230,#166231),(#166232,#166233),(#166234,#166235),
(#166236,#166237),(#166238,#166239),(#166240,#166241),(#166242,#166243),
(#166244,#166245),(#166246,#166247),(#166248,#166249),(#166250,#166251),
(#166252,#166253),(#166254,#166255),(#166256,#166257),(#166258,#166259),
(#166260,#166261),(#166262,#166263)),.UNSPECIFIED.,.F.,.F.,.F.)
B_SPLINE_SURFACE_WITH_KNOTS((6,1,1,1,1,1,1,1,1,1,1,1,1,1,1,1,1,1,1,1,1,
1,1,1,1,1,1,1,1,1,1,1,1,1,1,1,1,1,1,1,1,1,1,1,1,1,1,1,1,1,1,1,1,1,1,1,1,
1,1,1,1,1,1,1,1,1,1,1,1,1,1,1,1,1,1,1,1,1,1,1,1,1,1,1,1,1,1,1,1,1,1,1,1,
1,1,1,1,1,1,1,1,1,1,1,1,1,1,1,1,1,1,1,1,1,1,1,1,1,1,1,1,1,1,1,1,1,1,1,1,
1,1,1,1,1,1,1,1,1,1,1,1,1,1,1,1,1,1,1,1,1,1,1,1,1,1,1,1,1,1,1,1,1,1,1,1,
1,1,1,1,1,1,1,1,1,1,1,1,1,1,1,1,1,1,1,1,1,1,1,1,1,1,1,1,1,1,1,1,1,1,1,6),
(2,2),(-1.,-0.995000000000001,-0.990000000000001,-0.985000000000001,-0.980000000000001,
-0.975000000000001,-0.970000000000001,-0.965000000000001,-0.960000000000001,
-0.955000000000001,-0.950000000000001,-0.945000000000001,-0.940000000000001,
-0.935000000000001,-0.930000000000001,-0.925000000000001,-0.920000000000001,
-0.915000000000001,-0.910000000000001,-0.905000000000001,-0.900000000000001,
-0.895000000000001,-0.890000000000001,-0.885000000000001,-0.880000000000001,
-0.875000000000001,-0.870000000000001,-0.865000000000001,-0.860000000000001,
-0.855000000000001,-0.850000000000001,-0.845000000000001,-0.840000000000001,
-0.835000000000001,-0.830000000000001,-0.825000000000001,-0.820000000000001,
-0.815000000000001,-0.810000000000001,-0.805000000000001,-0.800000000000001,
-0.795000000000001,-0.790000000000001,-0.785000000000001,-0.780000000000001,
-0.775000000000001,-0.770000000000001,-0.765000000000001,-0.760000000000001,
-0.755000000000001,-0.750000000000001,-0.745000000000001,-0.740000000000001,
-0.735000000000001,-0.730000000000001,-0.725000000000001,-0.720000000000001,
-0.715000000000001,-0.710000000000001,-0.705000000000001,-0.700000000000001,
-0.695000000000001,-0.690000000000001,-0.685,-0.68,-0.675,-0.67,-0.665,
-0.66,-0.655,-0.65,-0.645,-0.64,-0.635,-0.63,-0.625,-0.62,-0.615,-0.61,
-0.605,-0.6,-0.595,-0.59,-0.585,-0.58,-0.575,-0.57,-0.565,-0.56,-0.555,
-0.55,-0.545,-0.54,-0.535,-0.53,-0.525,-0.52,-0.515,-0.51,-0.505,-0.5,-0.495,
-0.49,-0.485,-0.48,-0.475,-0.47,-0.465,-0.46,-0.455,-0.45,-0.445,-0.44,
-0.435,-0.43,-0.425,-0.42,-0.415,-0.41,-0.405,-0.4,-0.395,-0.39,-0.385,
-0.38,-0.375,-0.37,-0.365,-0.36,-0.355,-0.35,-0.345,-0.34,-0.335,-0.33,
-0.325,-0.32,-0.315,-0.31,-0.305,-0.3,-0.295,-0.29,-0.285,-0.28,-0.275,
-0.27,-0.265,-0.26,-0.255,-0.25,-0.245,-0.24,-0.235,-0.23,-0.225,-0.22,
-0.215,-0.21,-0.205,-0.2,-0.195,-0.19,-0.185,-0.18,-0.175,-0.17,-0.165,
-0.16,-0.155,-0.15,-0.145,-0.14,-0.135,-0.13,-0.125,-0.12,-0.115,-0.11,
-0.105,-0.1,-0.095,-0.09,-0.085,-0.08,-0.075,-0.07,-0.065,-0.06,-0.055,
-0.05,-0.045,-0.04,-0.035,-0.03,-0.025,-0.02,-0.015,-0.01,-0.005,0.),(0.,
1.2),.UNSPECIFIED.)
GEOMETRIC_REPRESENTATION_ITEM()
RATIONAL_B_SPLINE_SURFACE(((1.,1.),(1.,1.),(1.,1.),(1.,1.),(1.,1.),(1.,
1.),(1.,1.),(1.,1.),(1.,1.),(1.,1.),(1.,1.),(1.,1.),(1.,1.),(1.,1.),(1.,
1.),(1.,1.),(1.,1.),(1.,1.),(1.,1.),(1.,1.),(1.,1.),(1.,1.),(1.,1.),(1.,
1.),(1.,1.),(1.,1.),(1.,1.),(1.,1.),(1.,1.),(1.,1.),(1.,1.),(1.,1.),(1.,
1.),(1.,1.),(1.,1.),(1.,1.),(1.,1.),(1.,1.),(1.,1.),(1.,1.),(1.,1.),(1.,
1.),(1.,1.),(1.,1.),(1.,1.),(1.,1.),(1.,1.),(1.,1.),(1.,1.),(1.,1.),(1.,
1.),(1.,1.),(1.,1.),(1.,1.),(1.,1.),(1.,1.),(1.,1.),(1.,1.),(1.,1.),(1.,
1.),(1.,1.),(1.,1.),(1.,1.),(1.,1.),(1.,1.),(1.,1.),(1.,1.),(1.,1.),(1.,
1.),(1.,1.),(1.,1.),(1.,1.),(1.,1.),(1.,1.),(1.,1.),(1.,1.),(1.,1.),(1.,
1.),(1.,1.),(1.,1.),(1.,1.),(1.,1.),(1.,1.),(1.,1.),(1.,1.),(1.,1.),(1.,
1.),(1.,1.),(1.,1.),(1.,1.),(1.,1.),(1.,1.),(1.,1.),(1.,1.),(1.,1.),(1.,
1.),(1.,1.),(1.,1.),(1.,1.),(1.,1.),(1.,1.),(1.,1.),(1.,1.),(1.,1.),(1.,
1.),(1.,1.),(1.,1.),(1.,1.),(1.,1.),(1.,1.),(1.,1.),(1.,1.),(1.,1.),(1.,
1.),(1.,1.),(1.,1.),(1.,1.),(1.,1.),(1.,1.),(1.,1.),(1.,1.),(1.,1.),(1.,
1.),(1.,1.),(1.,1.),(1.,1.),(1.,1.),(1.,1.),(1.,1.),(1.,1.),(1.,1.),(1.,
1.),(1.,1.),(1.,1.),(1.,1.),(1.,1.),(1.,1.),(1.,1.),(1.,1.),(1.,1.),(1.,
1.),(1.,1.),(1.,1.),(1.,1.),(1.,1.),(1.,1.),(1.,1.),(1.,1.),(1.,1.),(1.,
1.),(1.,1.),(1.,1.),(1.,1.),(1.,1.),(1.,1.),(1.,1.),(1.,1.),(1.,1.),(1.,
1.),(1.,1.),(1.,1.),(1.,1.),(1.,1.),(1.,1.),(1.,1.),(1.,1.),(1.,1.),(1.,
1.),(1.,1.),(1.,1.),(1.,1.),(1.,1.),(1.,1.),(1.,1.),(1.,1.),(1.,1.),(1.,
1.),(1.,1.),(1.,1.),(1.,1.),(1.,1.),(1.,1.),(1.,1.),(1.,1.),(1.,1.),(1.,
1.),(1.,1.),(1.,1.),(1.,1.),(1.,1.),(1.,1.),(1.,1.),(1.,1.),(1.,1.),(1.,
1.),(1.,1.),(1.,1.),(1.,1.),(1.,1.),(1.,1.),(1.,1.),(1.,1.),(1.,1.),(1.,
1.),(1.,1.)))
REPRESENTATION_ITEM('')
SURFACE()
);
#1017=(
BOUNDED_SURFACE()
B_SPLINE_SURFACE(5,1,((#166655,#166656),(#166657,#166658),(#166659,#166660),
(#166661,#166662),(#166663,#166664),(#166665,#166666),(#166667,#166668),
(#166669,#166670),(#166671,#166672),(#166673,#166674),(#166675,#166676),
(#166677,#166678),(#166679,#166680),(#166681,#166682),(#166683,#166684),
(#166685,#166686),(#166687,#166688),(#166689,#166690),(#166691,#166692),
(#166693,#166694),(#166695,#166696),(#166697,#166698),(#166699,#166700),
(#166701,#166702),(#166703,#166704),(#166705,#166706),(#166707,#166708),
(#166709,#166710),(#166711,#166712),(#166713,#166714),(#166715,#166716),
(#166717,#166718),(#166719,#166720),(#166721,#166722),(#166723,#166724),
(#166725,#166726),(#166727,#166728),(#166729,#166730),(#166731,#166732),
(#166733,#166734),(#166735,#166736),(#166737,#166738),(#166739,#166740),
(#166741,#166742),(#166743,#166744),(#166745,#166746),(#166747,#166748),
(#166749,#166750),(#166751,#166752),(#166753,#166754),(#166755,#166756),
(#166757,#166758),(#166759,#166760),(#166761,#166762),(#166763,#166764),
(#166765,#166766),(#166767,#166768),(#166769,#166770),(#166771,#166772),
(#166773,#166774),(#166775,#166776),(#166777,#166778),(#166779,#166780),
(#166781,#166782),(#166783,#166784),(#166785,#166786),(#166787,#166788),
(#166789,#166790),(#166791,#166792),(#166793,#166794),(#166795,#166796),
(#166797,#166798),(#166799,#166800),(#166801,#166802),(#166803,#166804),
(#166805,#166806),(#166807,#166808),(#166809,#166810),(#166811,#166812),
(#166813,#166814),(#166815,#166816),(#166817,#166818),(#166819,#166820),
(#166821,#166822),(#166823,#166824),(#166825,#166826),(#166827,#166828),
(#166829,#166830),(#166831,#166832),(#166833,#166834),(#166835,#166836),
(#166837,#166838),(#166839,#166840),(#166841,#166842),(#166843,#166844),
(#166845,#166846),(#166847,#166848),(#166849,#166850),(#166851,#166852),
(#166853,#166854),(#166855,#166856),(#166857,#166858),(#166859,#166860),
(#166861,#166862),(#166863,#166864),(#166865,#166866),(#166867,#166868),
(#166869,#166870),(#166871,#166872),(#166873,#166874),(#166875,#166876),
(#166877,#166878),(#166879,#166880),(#166881,#166882),(#166883,#166884),
(#166885,#166886),(#166887,#166888),(#166889,#166890),(#166891,#166892),
(#166893,#166894),(#166895,#166896),(#166897,#166898),(#166899,#166900),
(#166901,#166902),(#166903,#166904),(#166905,#166906),(#166907,#166908),
(#166909,#166910),(#166911,#166912),(#166913,#166914),(#166915,#166916),
(#166917,#166918),(#166919,#166920),(#166921,#166922),(#166923,#166924),
(#166925,#166926),(#166927,#166928),(#166929,#166930),(#166931,#166932),
(#166933,#166934),(#166935,#166936),(#166937,#166938),(#166939,#166940),
(#166941,#166942),(#166943,#166944),(#166945,#166946),(#166947,#166948),
(#166949,#166950),(#166951,#166952),(#166953,#166954),(#166955,#166956),
(#166957,#166958),(#166959,#166960),(#166961,#166962),(#166963,#166964),
(#166965,#166966),(#166967,#166968),(#166969,#166970),(#166971,#166972),
(#166973,#166974),(#166975,#166976),(#166977,#166978),(#166979,#166980),
(#166981,#166982),(#166983,#166984),(#166985,#166986),(#166987,#166988),
(#166989,#166990),(#166991,#166992),(#166993,#166994),(#166995,#166996),
(#166997,#166998),(#166999,#167000),(#167001,#167002),(#167003,#167004),
(#167005,#167006),(#167007,#167008),(#167009,#167010),(#167011,#167012),
(#167013,#167014),(#167015,#167016),(#167017,#167018),(#167019,#167020),
(#167021,#167022),(#167023,#167024),(#167025,#167026),(#167027,#167028),
(#167029,#167030),(#167031,#167032),(#167033,#167034),(#167035,#167036),
(#167037,#167038),(#167039,#167040),(#167041,#167042),(#167043,#167044),
(#167045,#167046),(#167047,#167048),(#167049,#167050),(#167051,#167052),
(#167053,#167054),(#167055,#167056),(#167057,#167058),(#167059,#167060),
(#167061,#167062),(#167063,#167064)),.UNSPECIFIED.,.F.,.F.,.F.)
B_SPLINE_SURFACE_WITH_KNOTS((6,1,1,1,1,1,1,1,1,1,1,1,1,1,1,1,1,1,1,1,1,
1,1,1,1,1,1,1,1,1,1,1,1,1,1,1,1,1,1,1,1,1,1,1,1,1,1,1,1,1,1,1,1,1,1,1,1,
1,1,1,1,1,1,1,1,1,1,1,1,1,1,1,1,1,1,1,1,1,1,1,1,1,1,1,1,1,1,1,1,1,1,1,1,
1,1,1,1,1,1,1,1,1,1,1,1,1,1,1,1,1,1,1,1,1,1,1,1,1,1,1,1,1,1,1,1,1,1,1,1,
1,1,1,1,1,1,1,1,1,1,1,1,1,1,1,1,1,1,1,1,1,1,1,1,1,1,1,1,1,1,1,1,1,1,1,1,
1,1,1,1,1,1,1,1,1,1,1,1,1,1,1,1,1,1,1,1,1,1,1,1,1,1,1,1,1,1,1,1,1,1,1,6),
(2,2),(-1.,-0.995000000000001,-0.990000000000001,-0.985000000000001,-0.980000000000001,
-0.975000000000001,-0.970000000000001,-0.965000000000001,-0.960000000000001,
-0.955000000000001,-0.950000000000001,-0.945000000000001,-0.940000000000001,
-0.935000000000001,-0.930000000000001,-0.925000000000001,-0.920000000000001,
-0.915000000000001,-0.910000000000001,-0.905000000000001,-0.900000000000001,
-0.895000000000001,-0.890000000000001,-0.885000000000001,-0.880000000000001,
-0.875000000000001,-0.870000000000001,-0.865000000000001,-0.860000000000001,
-0.855000000000001,-0.850000000000001,-0.845000000000001,-0.840000000000001,
-0.835000000000001,-0.830000000000001,-0.825000000000001,-0.820000000000001,
-0.815000000000001,-0.810000000000001,-0.805000000000001,-0.800000000000001,
-0.795000000000001,-0.790000000000001,-0.785000000000001,-0.780000000000001,
-0.775000000000001,-0.770000000000001,-0.765000000000001,-0.760000000000001,
-0.755000000000001,-0.750000000000001,-0.745000000000001,-0.740000000000001,
-0.735000000000001,-0.730000000000001,-0.725000000000001,-0.720000000000001,
-0.715000000000001,-0.710000000000001,-0.705000000000001,-0.700000000000001,
-0.695000000000001,-0.690000000000001,-0.685,-0.68,-0.675,-0.67,-0.665,
-0.66,-0.655,-0.65,-0.645,-0.64,-0.635,-0.63,-0.625,-0.62,-0.615,-0.61,
-0.605,-0.6,-0.595,-0.59,-0.585,-0.58,-0.575,-0.57,-0.565,-0.56,-0.555,
-0.55,-0.545,-0.54,-0.535,-0.53,-0.525,-0.52,-0.515,-0.51,-0.505,-0.5,-0.495,
-0.49,-0.485,-0.48,-0.475,-0.47,-0.465,-0.46,-0.455,-0.45,-0.445,-0.44,
-0.435,-0.43,-0.425,-0.42,-0.415,-0.41,-0.405,-0.4,-0.395,-0.39,-0.385,
-0.38,-0.375,-0.37,-0.365,-0.36,-0.355,-0.35,-0.345,-0.34,-0.335,-0.33,
-0.325,-0.32,-0.315,-0.31,-0.305,-0.3,-0.295,-0.29,-0.285,-0.28,-0.275,
-0.27,-0.265,-0.26,-0.255,-0.25,-0.245,-0.24,-0.235,-0.23,-0.225,-0.22,
-0.215,-0.21,-0.205,-0.2,-0.195,-0.19,-0.185,-0.18,-0.175,-0.17,-0.165,
-0.16,-0.155,-0.15,-0.145,-0.14,-0.135,-0.13,-0.125,-0.12,-0.115,-0.11,
-0.105,-0.1,-0.095,-0.09,-0.085,-0.08,-0.075,-0.07,-0.065,-0.06,-0.055,
-0.05,-0.045,-0.04,-0.035,-0.03,-0.025,-0.02,-0.015,-0.01,-0.005,0.),(0.,
1.2),.UNSPECIFIED.)
GEOMETRIC_REPRESENTATION_ITEM()
RATIONAL_B_SPLINE_SURFACE(((1.,1.),(1.,1.),(1.,1.),(1.,1.),(1.,1.),(1.,
1.),(1.,1.),(1.,1.),(1.,1.),(1.,1.),(1.,1.),(1.,1.),(1.,1.),(1.,1.),(1.,
1.),(1.,1.),(1.,1.),(1.,1.),(1.,1.),(1.,1.),(1.,1.),(1.,1.),(1.,1.),(1.,
1.),(1.,1.),(1.,1.),(1.,1.),(1.,1.),(1.,1.),(1.,1.),(1.,1.),(1.,1.),(1.,
1.),(1.,1.),(1.,1.),(1.,1.),(1.,1.),(1.,1.),(1.,1.),(1.,1.),(1.,1.),(1.,
1.),(1.,1.),(1.,1.),(1.,1.),(1.,1.),(1.,1.),(1.,1.),(1.,1.),(1.,1.),(1.,
1.),(1.,1.),(1.,1.),(1.,1.),(1.,1.),(1.,1.),(1.,1.),(1.,1.),(1.,1.),(1.,
1.),(1.,1.),(1.,1.),(1.,1.),(1.,1.),(1.,1.),(1.,1.),(1.,1.),(1.,1.),(1.,
1.),(1.,1.),(1.,1.),(1.,1.),(1.,1.),(1.,1.),(1.,1.),(1.,1.),(1.,1.),(1.,
1.),(1.,1.),(1.,1.),(1.,1.),(1.,1.),(1.,1.),(1.,1.),(1.,1.),(1.,1.),(1.,
1.),(1.,1.),(1.,1.),(1.,1.),(1.,1.),(1.,1.),(1.,1.),(1.,1.),(1.,1.),(1.,
1.),(1.,1.),(1.,1.),(1.,1.),(1.,1.),(1.,1.),(1.,1.),(1.,1.),(1.,1.),(1.,
1.),(1.,1.),(1.,1.),(1.,1.),(1.,1.),(1.,1.),(1.,1.),(1.,1.),(1.,1.),(1.,
1.),(1.,1.),(1.,1.),(1.,1.),(1.,1.),(1.,1.),(1.,1.),(1.,1.),(1.,1.),(1.,
1.),(1.,1.),(1.,1.),(1.,1.),(1.,1.),(1.,1.),(1.,1.),(1.,1.),(1.,1.),(1.,
1.),(1.,1.),(1.,1.),(1.,1.),(1.,1.),(1.,1.),(1.,1.),(1.,1.),(1.,1.),(1.,
1.),(1.,1.),(1.,1.),(1.,1.),(1.,1.),(1.,1.),(1.,1.),(1.,1.),(1.,1.),(1.,
1.),(1.,1.),(1.,1.),(1.,1.),(1.,1.),(1.,1.),(1.,1.),(1.,1.),(1.,1.),(1.,
1.),(1.,1.),(1.,1.),(1.,1.),(1.,1.),(1.,1.),(1.,1.),(1.,1.),(1.,1.),(1.,
1.),(1.,1.),(1.,1.),(1.,1.),(1.,1.),(1.,1.),(1.,1.),(1.,1.),(1.,1.),(1.,
1.),(1.,1.),(1.,1.),(1.,1.),(1.,1.),(1.,1.),(1.,1.),(1.,1.),(1.,1.),(1.,
1.),(1.,1.),(1.,1.),(1.,1.),(1.,1.),(1.,1.),(1.,1.),(1.,1.),(1.,1.),(1.,
1.),(1.,1.),(1.,1.),(1.,1.),(1.,1.),(1.,1.),(1.,1.),(1.,1.),(1.,1.),(1.,
1.),(1.,1.)))
REPRESENTATION_ITEM('')
SURFACE()
);
#1018=(
BOUNDED_SURFACE()
B_SPLINE_SURFACE(5,1,((#167456,#167457),(#167458,#167459),(#167460,#167461),
(#167462,#167463),(#167464,#167465),(#167466,#167467),(#167468,#167469),
(#167470,#167471),(#167472,#167473),(#167474,#167475),(#167476,#167477),
(#167478,#167479),(#167480,#167481),(#167482,#167483),(#167484,#167485),
(#167486,#167487),(#167488,#167489),(#167490,#167491),(#167492,#167493),
(#167494,#167495),(#167496,#167497),(#167498,#167499),(#167500,#167501),
(#167502,#167503),(#167504,#167505),(#167506,#167507),(#167508,#167509),
(#167510,#167511),(#167512,#167513),(#167514,#167515),(#167516,#167517),
(#167518,#167519),(#167520,#167521),(#167522,#167523),(#167524,#167525),
(#167526,#167527),(#167528,#167529),(#167530,#167531),(#167532,#167533),
(#167534,#167535),(#167536,#167537),(#167538,#167539),(#167540,#167541),
(#167542,#167543),(#167544,#167545),(#167546,#167547),(#167548,#167549),
(#167550,#167551),(#167552,#167553),(#167554,#167555),(#167556,#167557),
(#167558,#167559),(#167560,#167561),(#167562,#167563),(#167564,#167565),
(#167566,#167567),(#167568,#167569),(#167570,#167571),(#167572,#167573),
(#167574,#167575),(#167576,#167577),(#167578,#167579),(#167580,#167581),
(#167582,#167583),(#167584,#167585),(#167586,#167587),(#167588,#167589),
(#167590,#167591),(#167592,#167593),(#167594,#167595),(#167596,#167597),
(#167598,#167599),(#167600,#167601),(#167602,#167603),(#167604,#167605),
(#167606,#167607),(#167608,#167609),(#167610,#167611),(#167612,#167613),
(#167614,#167615),(#167616,#167617),(#167618,#167619),(#167620,#167621),
(#167622,#167623),(#167624,#167625),(#167626,#167627),(#167628,#167629),
(#167630,#167631),(#167632,#167633),(#167634,#167635),(#167636,#167637),
(#167638,#167639),(#167640,#167641),(#167642,#167643),(#167644,#167645),
(#167646,#167647),(#167648,#167649),(#167650,#167651),(#167652,#167653),
(#167654,#167655),(#167656,#167657),(#167658,#167659),(#167660,#167661),
(#167662,#167663),(#167664,#167665),(#167666,#167667),(#167668,#167669),
(#167670,#167671),(#167672,#167673),(#167674,#167675),(#167676,#167677),
(#167678,#167679),(#167680,#167681),(#167682,#167683),(#167684,#167685),
(#167686,#167687),(#167688,#167689),(#167690,#167691),(#167692,#167693),
(#167694,#167695),(#167696,#167697),(#167698,#167699),(#167700,#167701),
(#167702,#167703),(#167704,#167705),(#167706,#167707),(#167708,#167709),
(#167710,#167711),(#167712,#167713),(#167714,#167715),(#167716,#167717),
(#167718,#167719),(#167720,#167721),(#167722,#167723),(#167724,#167725),
(#167726,#167727),(#167728,#167729),(#167730,#167731),(#167732,#167733),
(#167734,#167735),(#167736,#167737),(#167738,#167739),(#167740,#167741),
(#167742,#167743),(#167744,#167745),(#167746,#167747),(#167748,#167749),
(#167750,#167751),(#167752,#167753),(#167754,#167755),(#167756,#167757),
(#167758,#167759),(#167760,#167761),(#167762,#167763),(#167764,#167765),
(#167766,#167767),(#167768,#167769),(#167770,#167771),(#167772,#167773),
(#167774,#167775),(#167776,#167777),(#167778,#167779),(#167780,#167781),
(#167782,#167783),(#167784,#167785),(#167786,#167787),(#167788,#167789),
(#167790,#167791),(#167792,#167793),(#167794,#167795),(#167796,#167797),
(#167798,#167799),(#167800,#167801),(#167802,#167803),(#167804,#167805),
(#167806,#167807),(#167808,#167809),(#167810,#167811),(#167812,#167813),
(#167814,#167815),(#167816,#167817),(#167818,#167819),(#167820,#167821),
(#167822,#167823),(#167824,#167825),(#167826,#167827),(#167828,#167829),
(#167830,#167831),(#167832,#167833),(#167834,#167835),(#167836,#167837),
(#167838,#167839),(#167840,#167841),(#167842,#167843),(#167844,#167845),
(#167846,#167847),(#167848,#167849),(#167850,#167851),(#167852,#167853),
(#167854,#167855),(#167856,#167857),(#167858,#167859),(#167860,#167861),
(#167862,#167863),(#167864,#167865)),.UNSPECIFIED.,.F.,.F.,.F.)
B_SPLINE_SURFACE_WITH_KNOTS((6,1,1,1,1,1,1,1,1,1,1,1,1,1,1,1,1,1,1,1,1,
1,1,1,1,1,1,1,1,1,1,1,1,1,1,1,1,1,1,1,1,1,1,1,1,1,1,1,1,1,1,1,1,1,1,1,1,
1,1,1,1,1,1,1,1,1,1,1,1,1,1,1,1,1,1,1,1,1,1,1,1,1,1,1,1,1,1,1,1,1,1,1,1,
1,1,1,1,1,1,1,1,1,1,1,1,1,1,1,1,1,1,1,1,1,1,1,1,1,1,1,1,1,1,1,1,1,1,1,1,
1,1,1,1,1,1,1,1,1,1,1,1,1,1,1,1,1,1,1,1,1,1,1,1,1,1,1,1,1,1,1,1,1,1,1,1,
1,1,1,1,1,1,1,1,1,1,1,1,1,1,1,1,1,1,1,1,1,1,1,1,1,1,1,1,1,1,1,1,1,1,1,6),
(2,2),(-1.,-0.995000000000001,-0.990000000000001,-0.985000000000001,-0.980000000000001,
-0.975000000000001,-0.970000000000001,-0.965000000000001,-0.960000000000001,
-0.955000000000001,-0.950000000000001,-0.945000000000001,-0.940000000000001,
-0.935000000000001,-0.930000000000001,-0.925000000000001,-0.920000000000001,
-0.915000000000001,-0.910000000000001,-0.905000000000001,-0.900000000000001,
-0.895000000000001,-0.890000000000001,-0.885000000000001,-0.880000000000001,
-0.875000000000001,-0.870000000000001,-0.865000000000001,-0.860000000000001,
-0.855000000000001,-0.850000000000001,-0.845000000000001,-0.840000000000001,
-0.835000000000001,-0.830000000000001,-0.825000000000001,-0.820000000000001,
-0.815000000000001,-0.810000000000001,-0.805000000000001,-0.800000000000001,
-0.795000000000001,-0.790000000000001,-0.785000000000001,-0.780000000000001,
-0.775000000000001,-0.770000000000001,-0.765000000000001,-0.760000000000001,
-0.755000000000001,-0.750000000000001,-0.745000000000001,-0.740000000000001,
-0.735000000000001,-0.730000000000001,-0.725000000000001,-0.720000000000001,
-0.715000000000001,-0.710000000000001,-0.705000000000001,-0.700000000000001,
-0.695000000000001,-0.690000000000001,-0.685,-0.68,-0.675,-0.67,-0.665,
-0.66,-0.655,-0.65,-0.645,-0.64,-0.635,-0.63,-0.625,-0.62,-0.615,-0.61,
-0.605,-0.6,-0.595,-0.59,-0.585,-0.58,-0.575,-0.57,-0.565,-0.56,-0.555,
-0.55,-0.545,-0.54,-0.535,-0.53,-0.525,-0.52,-0.515,-0.51,-0.505,-0.5,-0.495,
-0.49,-0.485,-0.48,-0.475,-0.47,-0.465,-0.46,-0.455,-0.45,-0.445,-0.44,
-0.435,-0.43,-0.425,-0.42,-0.415,-0.41,-0.405,-0.4,-0.395,-0.39,-0.385,
-0.38,-0.375,-0.37,-0.365,-0.36,-0.355,-0.35,-0.345,-0.34,-0.335,-0.33,
-0.325,-0.32,-0.315,-0.31,-0.305,-0.3,-0.295,-0.29,-0.285,-0.28,-0.275,
-0.27,-0.265,-0.26,-0.255,-0.25,-0.245,-0.24,-0.235,-0.23,-0.225,-0.22,
-0.215,-0.21,-0.205,-0.2,-0.195,-0.19,-0.185,-0.18,-0.175,-0.17,-0.165,
-0.16,-0.155,-0.15,-0.145,-0.14,-0.135,-0.13,-0.125,-0.12,-0.115,-0.11,
-0.105,-0.1,-0.095,-0.09,-0.085,-0.08,-0.075,-0.07,-0.065,-0.06,-0.055,
-0.05,-0.045,-0.04,-0.035,-0.03,-0.025,-0.02,-0.015,-0.01,-0.005,0.),(0.,
1.2),.UNSPECIFIED.)
GEOMETRIC_REPRESENTATION_ITEM()
RATIONAL_B_SPLINE_SURFACE(((1.,1.),(1.,1.),(1.,1.),(1.,1.),(1.,1.),(1.,
1.),(1.,1.),(1.,1.),(1.,1.),(1.,1.),(1.,1.),(1.,1.),(1.,1.),(1.,1.),(1.,
1.),(1.,1.),(1.,1.),(1.,1.),(1.,1.),(1.,1.),(1.,1.),(1.,1.),(1.,1.),(1.,
1.),(1.,1.),(1.,1.),(1.,1.),(1.,1.),(1.,1.),(1.,1.),(1.,1.),(1.,1.),(1.,
1.),(1.,1.),(1.,1.),(1.,1.),(1.,1.),(1.,1.),(1.,1.),(1.,1.),(1.,1.),(1.,
1.),(1.,1.),(1.,1.),(1.,1.),(1.,1.),(1.,1.),(1.,1.),(1.,1.),(1.,1.),(1.,
1.),(1.,1.),(1.,1.),(1.,1.),(1.,1.),(1.,1.),(1.,1.),(1.,1.),(1.,1.),(1.,
1.),(1.,1.),(1.,1.),(1.,1.),(1.,1.),(1.,1.),(1.,1.),(1.,1.),(1.,1.),(1.,
1.),(1.,1.),(1.,1.),(1.,1.),(1.,1.),(1.,1.),(1.,1.),(1.,1.),(1.,1.),(1.,
1.),(1.,1.),(1.,1.),(1.,1.),(1.,1.),(1.,1.),(1.,1.),(1.,1.),(1.,1.),(1.,
1.),(1.,1.),(1.,1.),(1.,1.),(1.,1.),(1.,1.),(1.,1.),(1.,1.),(1.,1.),(1.,
1.),(1.,1.),(1.,1.),(1.,1.),(1.,1.),(1.,1.),(1.,1.),(1.,1.),(1.,1.),(1.,
1.),(1.,1.),(1.,1.),(1.,1.),(1.,1.),(1.,1.),(1.,1.),(1.,1.),(1.,1.),(1.,
1.),(1.,1.),(1.,1.),(1.,1.),(1.,1.),(1.,1.),(1.,1.),(1.,1.),(1.,1.),(1.,
1.),(1.,1.),(1.,1.),(1.,1.),(1.,1.),(1.,1.),(1.,1.),(1.,1.),(1.,1.),(1.,
1.),(1.,1.),(1.,1.),(1.,1.),(1.,1.),(1.,1.),(1.,1.),(1.,1.),(1.,1.),(1.,
1.),(1.,1.),(1.,1.),(1.,1.),(1.,1.),(1.,1.),(1.,1.),(1.,1.),(1.,1.),(1.,
1.),(1.,1.),(1.,1.),(1.,1.),(1.,1.),(1.,1.),(1.,1.),(1.,1.),(1.,1.),(1.,
1.),(1.,1.),(1.,1.),(1.,1.),(1.,1.),(1.,1.),(1.,1.),(1.,1.),(1.,1.),(1.,
1.),(1.,1.),(1.,1.),(1.,1.),(1.,1.),(1.,1.),(1.,1.),(1.,1.),(1.,1.),(1.,
1.),(1.,1.),(1.,1.),(1.,1.),(1.,1.),(1.,1.),(1.,1.),(1.,1.),(1.,1.),(1.,
1.),(1.,1.),(1.,1.),(1.,1.),(1.,1.),(1.,1.),(1.,1.),(1.,1.),(1.,1.),(1.,
1.),(1.,1.),(1.,1.),(1.,1.),(1.,1.),(1.,1.),(1.,1.),(1.,1.),(1.,1.),(1.,
1.),(1.,1.)))
REPRESENTATION_ITEM('')
SURFACE()
);
#1019=(
BOUNDED_SURFACE()
B_SPLINE_SURFACE(5,1,((#168257,#168258),(#168259,#168260),(#168261,#168262),
(#168263,#168264),(#168265,#168266),(#168267,#168268),(#168269,#168270),
(#168271,#168272),(#168273,#168274),(#168275,#168276),(#168277,#168278),
(#168279,#168280),(#168281,#168282),(#168283,#168284),(#168285,#168286),
(#168287,#168288),(#168289,#168290),(#168291,#168292),(#168293,#168294),
(#168295,#168296),(#168297,#168298),(#168299,#168300),(#168301,#168302),
(#168303,#168304),(#168305,#168306),(#168307,#168308),(#168309,#168310),
(#168311,#168312),(#168313,#168314),(#168315,#168316),(#168317,#168318),
(#168319,#168320),(#168321,#168322),(#168323,#168324),(#168325,#168326),
(#168327,#168328),(#168329,#168330),(#168331,#168332),(#168333,#168334),
(#168335,#168336),(#168337,#168338),(#168339,#168340),(#168341,#168342),
(#168343,#168344),(#168345,#168346),(#168347,#168348),(#168349,#168350),
(#168351,#168352),(#168353,#168354),(#168355,#168356),(#168357,#168358),
(#168359,#168360),(#168361,#168362),(#168363,#168364),(#168365,#168366),
(#168367,#168368),(#168369,#168370),(#168371,#168372),(#168373,#168374),
(#168375,#168376),(#168377,#168378),(#168379,#168380),(#168381,#168382),
(#168383,#168384),(#168385,#168386),(#168387,#168388),(#168389,#168390),
(#168391,#168392),(#168393,#168394),(#168395,#168396),(#168397,#168398),
(#168399,#168400),(#168401,#168402),(#168403,#168404),(#168405,#168406),
(#168407,#168408),(#168409,#168410),(#168411,#168412),(#168413,#168414),
(#168415,#168416),(#168417,#168418),(#168419,#168420),(#168421,#168422),
(#168423,#168424),(#168425,#168426),(#168427,#168428),(#168429,#168430),
(#168431,#168432),(#168433,#168434),(#168435,#168436),(#168437,#168438),
(#168439,#168440),(#168441,#168442),(#168443,#168444),(#168445,#168446),
(#168447,#168448),(#168449,#168450),(#168451,#168452),(#168453,#168454),
(#168455,#168456),(#168457,#168458),(#168459,#168460),(#168461,#168462),
(#168463,#168464),(#168465,#168466),(#168467,#168468),(#168469,#168470),
(#168471,#168472),(#168473,#168474),(#168475,#168476),(#168477,#168478),
(#168479,#168480),(#168481,#168482),(#168483,#168484),(#168485,#168486),
(#168487,#168488),(#168489,#168490),(#168491,#168492),(#168493,#168494),
(#168495,#168496),(#168497,#168498),(#168499,#168500),(#168501,#168502),
(#168503,#168504),(#168505,#168506),(#168507,#168508),(#168509,#168510),
(#168511,#168512),(#168513,#168514),(#168515,#168516),(#168517,#168518),
(#168519,#168520),(#168521,#168522),(#168523,#168524),(#168525,#168526),
(#168527,#168528),(#168529,#168530),(#168531,#168532),(#168533,#168534),
(#168535,#168536),(#168537,#168538),(#168539,#168540),(#168541,#168542),
(#168543,#168544),(#168545,#168546),(#168547,#168548),(#168549,#168550),
(#168551,#168552),(#168553,#168554),(#168555,#168556),(#168557,#168558),
(#168559,#168560),(#168561,#168562),(#168563,#168564),(#168565,#168566),
(#168567,#168568),(#168569,#168570),(#168571,#168572),(#168573,#168574),
(#168575,#168576),(#168577,#168578),(#168579,#168580),(#168581,#168582),
(#168583,#168584),(#168585,#168586),(#168587,#168588),(#168589,#168590),
(#168591,#168592),(#168593,#168594),(#168595,#168596),(#168597,#168598),
(#168599,#168600),(#168601,#168602),(#168603,#168604),(#168605,#168606),
(#168607,#168608),(#168609,#168610),(#168611,#168612),(#168613,#168614),
(#168615,#168616),(#168617,#168618),(#168619,#168620),(#168621,#168622),
(#168623,#168624),(#168625,#168626),(#168627,#168628),(#168629,#168630),
(#168631,#168632),(#168633,#168634),(#168635,#168636),(#168637,#168638),
(#168639,#168640),(#168641,#168642),(#168643,#168644),(#168645,#168646),
(#168647,#168648),(#168649,#168650),(#168651,#168652),(#168653,#168654),
(#168655,#168656),(#168657,#168658),(#168659,#168660),(#168661,#168662),
(#168663,#168664),(#168665,#168666)),.UNSPECIFIED.,.F.,.F.,.F.)
B_SPLINE_SURFACE_WITH_KNOTS((6,1,1,1,1,1,1,1,1,1,1,1,1,1,1,1,1,1,1,1,1,
1,1,1,1,1,1,1,1,1,1,1,1,1,1,1,1,1,1,1,1,1,1,1,1,1,1,1,1,1,1,1,1,1,1,1,1,
1,1,1,1,1,1,1,1,1,1,1,1,1,1,1,1,1,1,1,1,1,1,1,1,1,1,1,1,1,1,1,1,1,1,1,1,
1,1,1,1,1,1,1,1,1,1,1,1,1,1,1,1,1,1,1,1,1,1,1,1,1,1,1,1,1,1,1,1,1,1,1,1,
1,1,1,1,1,1,1,1,1,1,1,1,1,1,1,1,1,1,1,1,1,1,1,1,1,1,1,1,1,1,1,1,1,1,1,1,
1,1,1,1,1,1,1,1,1,1,1,1,1,1,1,1,1,1,1,1,1,1,1,1,1,1,1,1,1,1,1,1,1,1,1,6),
(2,2),(-1.,-0.995000000000001,-0.990000000000001,-0.985000000000001,-0.980000000000001,
-0.975000000000001,-0.970000000000001,-0.965000000000001,-0.960000000000001,
-0.955000000000001,-0.950000000000001,-0.945000000000001,-0.940000000000001,
-0.935000000000001,-0.930000000000001,-0.925000000000001,-0.920000000000001,
-0.915000000000001,-0.910000000000001,-0.905000000000001,-0.900000000000001,
-0.895000000000001,-0.890000000000001,-0.885000000000001,-0.880000000000001,
-0.875000000000001,-0.870000000000001,-0.865000000000001,-0.860000000000001,
-0.855000000000001,-0.850000000000001,-0.845000000000001,-0.840000000000001,
-0.835000000000001,-0.830000000000001,-0.825000000000001,-0.820000000000001,
-0.815000000000001,-0.810000000000001,-0.805000000000001,-0.800000000000001,
-0.795000000000001,-0.790000000000001,-0.785000000000001,-0.780000000000001,
-0.775000000000001,-0.770000000000001,-0.765000000000001,-0.760000000000001,
-0.755000000000001,-0.750000000000001,-0.745000000000001,-0.740000000000001,
-0.735000000000001,-0.730000000000001,-0.725000000000001,-0.720000000000001,
-0.715000000000001,-0.710000000000001,-0.705000000000001,-0.700000000000001,
-0.695000000000001,-0.690000000000001,-0.685,-0.68,-0.675,-0.67,-0.665,
-0.66,-0.655,-0.65,-0.645,-0.64,-0.635,-0.63,-0.625,-0.62,-0.615,-0.61,
-0.605,-0.6,-0.595,-0.59,-0.585,-0.58,-0.575,-0.57,-0.565,-0.56,-0.555,
-0.55,-0.545,-0.54,-0.535,-0.53,-0.525,-0.52,-0.515,-0.51,-0.505,-0.5,-0.495,
-0.49,-0.485,-0.48,-0.475,-0.47,-0.465,-0.46,-0.455,-0.45,-0.445,-0.44,
-0.435,-0.43,-0.425,-0.42,-0.415,-0.41,-0.405,-0.4,-0.395,-0.39,-0.385,
-0.38,-0.375,-0.37,-0.365,-0.36,-0.355,-0.35,-0.345,-0.34,-0.335,-0.33,
-0.325,-0.32,-0.315,-0.31,-0.305,-0.3,-0.295,-0.29,-0.285,-0.28,-0.275,
-0.27,-0.265,-0.26,-0.255,-0.25,-0.245,-0.24,-0.235,-0.23,-0.225,-0.22,
-0.215,-0.21,-0.205,-0.2,-0.195,-0.19,-0.185,-0.18,-0.175,-0.17,-0.165,
-0.16,-0.155,-0.15,-0.145,-0.14,-0.135,-0.13,-0.125,-0.12,-0.115,-0.11,
-0.105,-0.1,-0.095,-0.09,-0.085,-0.08,-0.075,-0.07,-0.065,-0.06,-0.055,
-0.05,-0.045,-0.04,-0.035,-0.03,-0.025,-0.02,-0.015,-0.01,-0.005,0.),(0.,
1.2),.UNSPECIFIED.)
GEOMETRIC_REPRESENTATION_ITEM()
RATIONAL_B_SPLINE_SURFACE(((1.,1.),(1.,1.),(1.,1.),(1.,1.),(1.,1.),(1.,
1.),(1.,1.),(1.,1.),(1.,1.),(1.,1.),(1.,1.),(1.,1.),(1.,1.),(1.,1.),(1.,
1.),(1.,1.),(1.,1.),(1.,1.),(1.,1.),(1.,1.),(1.,1.),(1.,1.),(1.,1.),(1.,
1.),(1.,1.),(1.,1.),(1.,1.),(1.,1.),(1.,1.),(1.,1.),(1.,1.),(1.,1.),(1.,
1.),(1.,1.),(1.,1.),(1.,1.),(1.,1.),(1.,1.),(1.,1.),(1.,1.),(1.,1.),(1.,
1.),(1.,1.),(1.,1.),(1.,1.),(1.,1.),(1.,1.),(1.,1.),(1.,1.),(1.,1.),(1.,
1.),(1.,1.),(1.,1.),(1.,1.),(1.,1.),(1.,1.),(1.,1.),(1.,1.),(1.,1.),(1.,
1.),(1.,1.),(1.,1.),(1.,1.),(1.,1.),(1.,1.),(1.,1.),(1.,1.),(1.,1.),(1.,
1.),(1.,1.),(1.,1.),(1.,1.),(1.,1.),(1.,1.),(1.,1.),(1.,1.),(1.,1.),(1.,
1.),(1.,1.),(1.,1.),(1.,1.),(1.,1.),(1.,1.),(1.,1.),(1.,1.),(1.,1.),(1.,
1.),(1.,1.),(1.,1.),(1.,1.),(1.,1.),(1.,1.),(1.,1.),(1.,1.),(1.,1.),(1.,
1.),(1.,1.),(1.,1.),(1.,1.),(1.,1.),(1.,1.),(1.,1.),(1.,1.),(1.,1.),(1.,
1.),(1.,1.),(1.,1.),(1.,1.),(1.,1.),(1.,1.),(1.,1.),(1.,1.),(1.,1.),(1.,
1.),(1.,1.),(1.,1.),(1.,1.),(1.,1.),(1.,1.),(1.,1.),(1.,1.),(1.,1.),(1.,
1.),(1.,1.),(1.,1.),(1.,1.),(1.,1.),(1.,1.),(1.,1.),(1.,1.),(1.,1.),(1.,
1.),(1.,1.),(1.,1.),(1.,1.),(1.,1.),(1.,1.),(1.,1.),(1.,1.),(1.,1.),(1.,
1.),(1.,1.),(1.,1.),(1.,1.),(1.,1.),(1.,1.),(1.,1.),(1.,1.),(1.,1.),(1.,
1.),(1.,1.),(1.,1.),(1.,1.),(1.,1.),(1.,1.),(1.,1.),(1.,1.),(1.,1.),(1.,
1.),(1.,1.),(1.,1.),(1.,1.),(1.,1.),(1.,1.),(1.,1.),(1.,1.),(1.,1.),(1.,
1.),(1.,1.),(1.,1.),(1.,1.),(1.,1.),(1.,1.),(1.,1.),(1.,1.),(1.,1.),(1.,
1.),(1.,1.),(1.,1.),(1.,1.),(1.,1.),(1.,1.),(1.,1.),(1.,1.),(1.,1.),(1.,
1.),(1.,1.),(1.,1.),(1.,1.),(1.,1.),(1.,1.),(1.,1.),(1.,1.),(1.,1.),(1.,
1.),(1.,1.),(1.,1.),(1.,1.),(1.,1.),(1.,1.),(1.,1.),(1.,1.),(1.,1.),(1.,
1.),(1.,1.)))
REPRESENTATION_ITEM('')
SURFACE()
);
#1020=(
BOUNDED_SURFACE()
B_SPLINE_SURFACE(5,1,((#169058,#169059),(#169060,#169061),(#169062,#169063),
(#169064,#169065),(#169066,#169067),(#169068,#169069),(#169070,#169071),
(#169072,#169073),(#169074,#169075),(#169076,#169077),(#169078,#169079),
(#169080,#169081),(#169082,#169083),(#169084,#169085),(#169086,#169087),
(#169088,#169089),(#169090,#169091),(#169092,#169093),(#169094,#169095),
(#169096,#169097),(#169098,#169099),(#169100,#169101),(#169102,#169103),
(#169104,#169105),(#169106,#169107),(#169108,#169109),(#169110,#169111),
(#169112,#169113),(#169114,#169115),(#169116,#169117),(#169118,#169119),
(#169120,#169121),(#169122,#169123),(#169124,#169125),(#169126,#169127),
(#169128,#169129),(#169130,#169131),(#169132,#169133),(#169134,#169135),
(#169136,#169137),(#169138,#169139),(#169140,#169141),(#169142,#169143),
(#169144,#169145),(#169146,#169147),(#169148,#169149),(#169150,#169151),
(#169152,#169153),(#169154,#169155),(#169156,#169157),(#169158,#169159),
(#169160,#169161),(#169162,#169163),(#169164,#169165),(#169166,#169167),
(#169168,#169169),(#169170,#169171),(#169172,#169173),(#169174,#169175),
(#169176,#169177),(#169178,#169179),(#169180,#169181),(#169182,#169183),
(#169184,#169185),(#169186,#169187),(#169188,#169189),(#169190,#169191),
(#169192,#169193),(#169194,#169195),(#169196,#169197),(#169198,#169199),
(#169200,#169201),(#169202,#169203),(#169204,#169205),(#169206,#169207),
(#169208,#169209),(#169210,#169211),(#169212,#169213),(#169214,#169215),
(#169216,#169217),(#169218,#169219),(#169220,#169221),(#169222,#169223),
(#169224,#169225),(#169226,#169227),(#169228,#169229),(#169230,#169231),
(#169232,#169233),(#169234,#169235),(#169236,#169237),(#169238,#169239),
(#169240,#169241),(#169242,#169243),(#169244,#169245),(#169246,#169247),
(#169248,#169249),(#169250,#169251),(#169252,#169253),(#169254,#169255),
(#169256,#169257),(#169258,#169259),(#169260,#169261),(#169262,#169263),
(#169264,#169265),(#169266,#169267),(#169268,#169269),(#169270,#169271),
(#169272,#169273),(#169274,#169275),(#169276,#169277),(#169278,#169279),
(#169280,#169281),(#169282,#169283),(#169284,#169285),(#169286,#169287),
(#169288,#169289),(#169290,#169291),(#169292,#169293),(#169294,#169295),
(#169296,#169297),(#169298,#169299),(#169300,#169301),(#169302,#169303),
(#169304,#169305),(#169306,#169307),(#169308,#169309),(#169310,#169311),
(#169312,#169313),(#169314,#169315),(#169316,#169317),(#169318,#169319),
(#169320,#169321),(#169322,#169323),(#169324,#169325),(#169326,#169327),
(#169328,#169329),(#169330,#169331),(#169332,#169333),(#169334,#169335),
(#169336,#169337),(#169338,#169339),(#169340,#169341),(#169342,#169343),
(#169344,#169345),(#169346,#169347),(#169348,#169349),(#169350,#169351),
(#169352,#169353),(#169354,#169355),(#169356,#169357),(#169358,#169359),
(#169360,#169361),(#169362,#169363),(#169364,#169365),(#169366,#169367),
(#169368,#169369),(#169370,#169371),(#169372,#169373),(#169374,#169375),
(#169376,#169377),(#169378,#169379),(#169380,#169381),(#169382,#169383),
(#169384,#169385),(#169386,#169387),(#169388,#169389),(#169390,#169391),
(#169392,#169393),(#169394,#169395),(#169396,#169397),(#169398,#169399),
(#169400,#169401),(#169402,#169403),(#169404,#169405),(#169406,#169407),
(#169408,#169409),(#169410,#169411),(#169412,#169413),(#169414,#169415),
(#169416,#169417),(#169418,#169419),(#169420,#169421),(#169422,#169423),
(#169424,#169425),(#169426,#169427),(#169428,#169429),(#169430,#169431),
(#169432,#169433),(#169434,#169435),(#169436,#169437),(#169438,#169439),
(#169440,#169441),(#169442,#169443),(#169444,#169445),(#169446,#169447),
(#169448,#169449),(#169450,#169451),(#169452,#169453),(#169454,#169455),
(#169456,#169457),(#169458,#169459),(#169460,#169461),(#169462,#169463),
(#169464,#169465),(#169466,#169467)),.UNSPECIFIED.,.F.,.F.,.F.)
B_SPLINE_SURFACE_WITH_KNOTS((6,1,1,1,1,1,1,1,1,1,1,1,1,1,1,1,1,1,1,1,1,
1,1,1,1,1,1,1,1,1,1,1,1,1,1,1,1,1,1,1,1,1,1,1,1,1,1,1,1,1,1,1,1,1,1,1,1,
1,1,1,1,1,1,1,1,1,1,1,1,1,1,1,1,1,1,1,1,1,1,1,1,1,1,1,1,1,1,1,1,1,1,1,1,
1,1,1,1,1,1,1,1,1,1,1,1,1,1,1,1,1,1,1,1,1,1,1,1,1,1,1,1,1,1,1,1,1,1,1,1,
1,1,1,1,1,1,1,1,1,1,1,1,1,1,1,1,1,1,1,1,1,1,1,1,1,1,1,1,1,1,1,1,1,1,1,1,
1,1,1,1,1,1,1,1,1,1,1,1,1,1,1,1,1,1,1,1,1,1,1,1,1,1,1,1,1,1,1,1,1,1,1,6),
(2,2),(-1.,-0.995000000000001,-0.990000000000001,-0.985000000000001,-0.980000000000001,
-0.975000000000001,-0.970000000000001,-0.965000000000001,-0.960000000000001,
-0.955000000000001,-0.950000000000001,-0.945000000000001,-0.940000000000001,
-0.935000000000001,-0.930000000000001,-0.925000000000001,-0.920000000000001,
-0.915000000000001,-0.910000000000001,-0.905000000000001,-0.900000000000001,
-0.895000000000001,-0.890000000000001,-0.885000000000001,-0.880000000000001,
-0.875000000000001,-0.870000000000001,-0.865000000000001,-0.860000000000001,
-0.855000000000001,-0.850000000000001,-0.845000000000001,-0.840000000000001,
-0.835000000000001,-0.830000000000001,-0.825000000000001,-0.820000000000001,
-0.815000000000001,-0.810000000000001,-0.805000000000001,-0.800000000000001,
-0.795000000000001,-0.790000000000001,-0.785000000000001,-0.780000000000001,
-0.775000000000001,-0.770000000000001,-0.765000000000001,-0.760000000000001,
-0.755000000000001,-0.750000000000001,-0.745000000000001,-0.740000000000001,
-0.735000000000001,-0.730000000000001,-0.725000000000001,-0.720000000000001,
-0.715000000000001,-0.710000000000001,-0.705000000000001,-0.700000000000001,
-0.695000000000001,-0.690000000000001,-0.685,-0.68,-0.675,-0.67,-0.665,
-0.66,-0.655,-0.65,-0.645,-0.64,-0.635,-0.63,-0.625,-0.62,-0.615,-0.61,
-0.605,-0.6,-0.595,-0.59,-0.585,-0.58,-0.575,-0.57,-0.565,-0.56,-0.555,
-0.55,-0.545,-0.54,-0.535,-0.53,-0.525,-0.52,-0.515,-0.51,-0.505,-0.5,-0.495,
-0.49,-0.485,-0.48,-0.475,-0.47,-0.465,-0.46,-0.455,-0.45,-0.445,-0.44,
-0.435,-0.43,-0.425,-0.42,-0.415,-0.41,-0.405,-0.4,-0.395,-0.39,-0.385,
-0.38,-0.375,-0.37,-0.365,-0.36,-0.355,-0.35,-0.345,-0.34,-0.335,-0.33,
-0.325,-0.32,-0.315,-0.31,-0.305,-0.3,-0.295,-0.29,-0.285,-0.28,-0.275,
-0.27,-0.265,-0.26,-0.255,-0.25,-0.245,-0.24,-0.235,-0.23,-0.225,-0.22,
-0.215,-0.21,-0.205,-0.2,-0.195,-0.19,-0.185,-0.18,-0.175,-0.17,-0.165,
-0.16,-0.155,-0.15,-0.145,-0.14,-0.135,-0.13,-0.125,-0.12,-0.115,-0.11,
-0.105,-0.1,-0.095,-0.09,-0.085,-0.08,-0.075,-0.07,-0.065,-0.06,-0.055,
-0.05,-0.045,-0.04,-0.035,-0.03,-0.025,-0.02,-0.015,-0.01,-0.005,0.),(0.,
1.2),.UNSPECIFIED.)
GEOMETRIC_REPRESENTATION_ITEM()
RATIONAL_B_SPLINE_SURFACE(((1.,1.),(1.,1.),(1.,1.),(1.,1.),(1.,1.),(1.,
1.),(1.,1.),(1.,1.),(1.,1.),(1.,1.),(1.,1.),(1.,1.),(1.,1.),(1.,1.),(1.,
1.),(1.,1.),(1.,1.),(1.,1.),(1.,1.),(1.,1.),(1.,1.),(1.,1.),(1.,1.),(1.,
1.),(1.,1.),(1.,1.),(1.,1.),(1.,1.),(1.,1.),(1.,1.),(1.,1.),(1.,1.),(1.,
1.),(1.,1.),(1.,1.),(1.,1.),(1.,1.),(1.,1.),(1.,1.),(1.,1.),(1.,1.),(1.,
1.),(1.,1.),(1.,1.),(1.,1.),(1.,1.),(1.,1.),(1.,1.),(1.,1.),(1.,1.),(1.,
1.),(1.,1.),(1.,1.),(1.,1.),(1.,1.),(1.,1.),(1.,1.),(1.,1.),(1.,1.),(1.,
1.),(1.,1.),(1.,1.),(1.,1.),(1.,1.),(1.,1.),(1.,1.),(1.,1.),(1.,1.),(1.,
1.),(1.,1.),(1.,1.),(1.,1.),(1.,1.),(1.,1.),(1.,1.),(1.,1.),(1.,1.),(1.,
1.),(1.,1.),(1.,1.),(1.,1.),(1.,1.),(1.,1.),(1.,1.),(1.,1.),(1.,1.),(1.,
1.),(1.,1.),(1.,1.),(1.,1.),(1.,1.),(1.,1.),(1.,1.),(1.,1.),(1.,1.),(1.,
1.),(1.,1.),(1.,1.),(1.,1.),(1.,1.),(1.,1.),(1.,1.),(1.,1.),(1.,1.),(1.,
1.),(1.,1.),(1.,1.),(1.,1.),(1.,1.),(1.,1.),(1.,1.),(1.,1.),(1.,1.),(1.,
1.),(1.,1.),(1.,1.),(1.,1.),(1.,1.),(1.,1.),(1.,1.),(1.,1.),(1.,1.),(1.,
1.),(1.,1.),(1.,1.),(1.,1.),(1.,1.),(1.,1.),(1.,1.),(1.,1.),(1.,1.),(1.,
1.),(1.,1.),(1.,1.),(1.,1.),(1.,1.),(1.,1.),(1.,1.),(1.,1.),(1.,1.),(1.,
1.),(1.,1.),(1.,1.),(1.,1.),(1.,1.),(1.,1.),(1.,1.),(1.,1.),(1.,1.),(1.,
1.),(1.,1.),(1.,1.),(1.,1.),(1.,1.),(1.,1.),(1.,1.),(1.,1.),(1.,1.),(1.,
1.),(1.,1.),(1.,1.),(1.,1.),(1.,1.),(1.,1.),(1.,1.),(1.,1.),(1.,1.),(1.,
1.),(1.,1.),(1.,1.),(1.,1.),(1.,1.),(1.,1.),(1.,1.),(1.,1.),(1.,1.),(1.,
1.),(1.,1.),(1.,1.),(1.,1.),(1.,1.),(1.,1.),(1.,1.),(1.,1.),(1.,1.),(1.,
1.),(1.,1.),(1.,1.),(1.,1.),(1.,1.),(1.,1.),(1.,1.),(1.,1.),(1.,1.),(1.,
1.),(1.,1.),(1.,1.),(1.,1.),(1.,1.),(1.,1.),(1.,1.),(1.,1.),(1.,1.),(1.,
1.),(1.,1.)))
REPRESENTATION_ITEM('')
SURFACE()
);
#1021=(
BOUNDED_SURFACE()
B_SPLINE_SURFACE(5,1,((#169859,#169860),(#169861,#169862),(#169863,#169864),
(#169865,#169866),(#169867,#169868),(#169869,#169870),(#169871,#169872),
(#169873,#169874),(#169875,#169876),(#169877,#169878),(#169879,#169880),
(#169881,#169882),(#169883,#169884),(#169885,#169886),(#169887,#169888),
(#169889,#169890),(#169891,#169892),(#169893,#169894),(#169895,#169896),
(#169897,#169898),(#169899,#169900),(#169901,#169902),(#169903,#169904),
(#169905,#169906),(#169907,#169908),(#169909,#169910),(#169911,#169912),
(#169913,#169914),(#169915,#169916),(#169917,#169918),(#169919,#169920),
(#169921,#169922),(#169923,#169924),(#169925,#169926),(#169927,#169928),
(#169929,#169930),(#169931,#169932),(#169933,#169934),(#169935,#169936),
(#169937,#169938),(#169939,#169940),(#169941,#169942),(#169943,#169944),
(#169945,#169946),(#169947,#169948),(#169949,#169950),(#169951,#169952),
(#169953,#169954),(#169955,#169956),(#169957,#169958),(#169959,#169960),
(#169961,#169962),(#169963,#169964),(#169965,#169966),(#169967,#169968),
(#169969,#169970),(#169971,#169972),(#169973,#169974),(#169975,#169976),
(#169977,#169978),(#169979,#169980),(#169981,#169982),(#169983,#169984),
(#169985,#169986),(#169987,#169988),(#169989,#169990),(#169991,#169992),
(#169993,#169994),(#169995,#169996),(#169997,#169998),(#169999,#170000),
(#170001,#170002),(#170003,#170004),(#170005,#170006),(#170007,#170008),
(#170009,#170010),(#170011,#170012),(#170013,#170014),(#170015,#170016),
(#170017,#170018),(#170019,#170020),(#170021,#170022),(#170023,#170024),
(#170025,#170026),(#170027,#170028),(#170029,#170030),(#170031,#170032),
(#170033,#170034),(#170035,#170036),(#170037,#170038),(#170039,#170040),
(#170041,#170042),(#170043,#170044),(#170045,#170046),(#170047,#170048),
(#170049,#170050),(#170051,#170052),(#170053,#170054),(#170055,#170056),
(#170057,#170058),(#170059,#170060),(#170061,#170062),(#170063,#170064),
(#170065,#170066),(#170067,#170068),(#170069,#170070),(#170071,#170072),
(#170073,#170074),(#170075,#170076),(#170077,#170078),(#170079,#170080),
(#170081,#170082),(#170083,#170084),(#170085,#170086),(#170087,#170088),
(#170089,#170090),(#170091,#170092),(#170093,#170094),(#170095,#170096),
(#170097,#170098),(#170099,#170100),(#170101,#170102),(#170103,#170104),
(#170105,#170106),(#170107,#170108),(#170109,#170110),(#170111,#170112),
(#170113,#170114),(#170115,#170116),(#170117,#170118),(#170119,#170120),
(#170121,#170122),(#170123,#170124),(#170125,#170126),(#170127,#170128),
(#170129,#170130),(#170131,#170132),(#170133,#170134),(#170135,#170136),
(#170137,#170138),(#170139,#170140),(#170141,#170142),(#170143,#170144),
(#170145,#170146),(#170147,#170148),(#170149,#170150),(#170151,#170152),
(#170153,#170154),(#170155,#170156),(#170157,#170158),(#170159,#170160),
(#170161,#170162),(#170163,#170164),(#170165,#170166),(#170167,#170168),
(#170169,#170170),(#170171,#170172),(#170173,#170174),(#170175,#170176),
(#170177,#170178),(#170179,#170180),(#170181,#170182),(#170183,#170184),
(#170185,#170186),(#170187,#170188),(#170189,#170190),(#170191,#170192),
(#170193,#170194),(#170195,#170196),(#170197,#170198),(#170199,#170200),
(#170201,#170202),(#170203,#170204),(#170205,#170206),(#170207,#170208),
(#170209,#170210),(#170211,#170212),(#170213,#170214),(#170215,#170216),
(#170217,#170218),(#170219,#170220),(#170221,#170222),(#170223,#170224),
(#170225,#170226),(#170227,#170228),(#170229,#170230),(#170231,#170232),
(#170233,#170234),(#170235,#170236),(#170237,#170238),(#170239,#170240),
(#170241,#170242),(#170243,#170244),(#170245,#170246),(#170247,#170248),
(#170249,#170250),(#170251,#170252),(#170253,#170254),(#170255,#170256),
(#170257,#170258),(#170259,#170260),(#170261,#170262),(#170263,#170264),
(#170265,#170266),(#170267,#170268)),.UNSPECIFIED.,.F.,.F.,.F.)
B_SPLINE_SURFACE_WITH_KNOTS((6,1,1,1,1,1,1,1,1,1,1,1,1,1,1,1,1,1,1,1,1,
1,1,1,1,1,1,1,1,1,1,1,1,1,1,1,1,1,1,1,1,1,1,1,1,1,1,1,1,1,1,1,1,1,1,1,1,
1,1,1,1,1,1,1,1,1,1,1,1,1,1,1,1,1,1,1,1,1,1,1,1,1,1,1,1,1,1,1,1,1,1,1,1,
1,1,1,1,1,1,1,1,1,1,1,1,1,1,1,1,1,1,1,1,1,1,1,1,1,1,1,1,1,1,1,1,1,1,1,1,
1,1,1,1,1,1,1,1,1,1,1,1,1,1,1,1,1,1,1,1,1,1,1,1,1,1,1,1,1,1,1,1,1,1,1,1,
1,1,1,1,1,1,1,1,1,1,1,1,1,1,1,1,1,1,1,1,1,1,1,1,1,1,1,1,1,1,1,1,1,1,1,6),
(2,2),(-1.,-0.995000000000001,-0.990000000000001,-0.985000000000001,-0.980000000000001,
-0.975000000000001,-0.970000000000001,-0.965000000000001,-0.960000000000001,
-0.955000000000001,-0.950000000000001,-0.945000000000001,-0.940000000000001,
-0.935000000000001,-0.930000000000001,-0.925000000000001,-0.920000000000001,
-0.915000000000001,-0.910000000000001,-0.905000000000001,-0.900000000000001,
-0.895000000000001,-0.890000000000001,-0.885000000000001,-0.880000000000001,
-0.875000000000001,-0.870000000000001,-0.865000000000001,-0.860000000000001,
-0.855000000000001,-0.850000000000001,-0.845000000000001,-0.840000000000001,
-0.835000000000001,-0.830000000000001,-0.825000000000001,-0.820000000000001,
-0.815000000000001,-0.810000000000001,-0.805000000000001,-0.800000000000001,
-0.795000000000001,-0.790000000000001,-0.785000000000001,-0.780000000000001,
-0.775000000000001,-0.770000000000001,-0.765000000000001,-0.760000000000001,
-0.755000000000001,-0.750000000000001,-0.745000000000001,-0.740000000000001,
-0.735000000000001,-0.730000000000001,-0.725000000000001,-0.720000000000001,
-0.715000000000001,-0.710000000000001,-0.705000000000001,-0.700000000000001,
-0.695000000000001,-0.690000000000001,-0.685,-0.68,-0.675,-0.67,-0.665,
-0.66,-0.655,-0.65,-0.645,-0.64,-0.635,-0.63,-0.625,-0.62,-0.615,-0.61,
-0.605,-0.6,-0.595,-0.59,-0.585,-0.58,-0.575,-0.57,-0.565,-0.56,-0.555,
-0.55,-0.545,-0.54,-0.535,-0.53,-0.525,-0.52,-0.515,-0.51,-0.505,-0.5,-0.495,
-0.49,-0.485,-0.48,-0.475,-0.47,-0.465,-0.46,-0.455,-0.45,-0.445,-0.44,
-0.435,-0.43,-0.425,-0.42,-0.415,-0.41,-0.405,-0.4,-0.395,-0.39,-0.385,
-0.38,-0.375,-0.37,-0.365,-0.36,-0.355,-0.35,-0.345,-0.34,-0.335,-0.33,
-0.325,-0.32,-0.315,-0.31,-0.305,-0.3,-0.295,-0.29,-0.285,-0.28,-0.275,
-0.27,-0.265,-0.26,-0.255,-0.25,-0.245,-0.24,-0.235,-0.23,-0.225,-0.22,
-0.215,-0.21,-0.205,-0.2,-0.195,-0.19,-0.185,-0.18,-0.175,-0.17,-0.165,
-0.16,-0.155,-0.15,-0.145,-0.14,-0.135,-0.13,-0.125,-0.12,-0.115,-0.11,
-0.105,-0.1,-0.095,-0.09,-0.085,-0.08,-0.075,-0.07,-0.065,-0.06,-0.055,
-0.05,-0.045,-0.04,-0.035,-0.03,-0.025,-0.02,-0.015,-0.01,-0.005,0.),(0.,
1.2),.UNSPECIFIED.)
GEOMETRIC_REPRESENTATION_ITEM()
RATIONAL_B_SPLINE_SURFACE(((1.,1.),(1.,1.),(1.,1.),(1.,1.),(1.,1.),(1.,
1.),(1.,1.),(1.,1.),(1.,1.),(1.,1.),(1.,1.),(1.,1.),(1.,1.),(1.,1.),(1.,
1.),(1.,1.),(1.,1.),(1.,1.),(1.,1.),(1.,1.),(1.,1.),(1.,1.),(1.,1.),(1.,
1.),(1.,1.),(1.,1.),(1.,1.),(1.,1.),(1.,1.),(1.,1.),(1.,1.),(1.,1.),(1.,
1.),(1.,1.),(1.,1.),(1.,1.),(1.,1.),(1.,1.),(1.,1.),(1.,1.),(1.,1.),(1.,
1.),(1.,1.),(1.,1.),(1.,1.),(1.,1.),(1.,1.),(1.,1.),(1.,1.),(1.,1.),(1.,
1.),(1.,1.),(1.,1.),(1.,1.),(1.,1.),(1.,1.),(1.,1.),(1.,1.),(1.,1.),(1.,
1.),(1.,1.),(1.,1.),(1.,1.),(1.,1.),(1.,1.),(1.,1.),(1.,1.),(1.,1.),(1.,
1.),(1.,1.),(1.,1.),(1.,1.),(1.,1.),(1.,1.),(1.,1.),(1.,1.),(1.,1.),(1.,
1.),(1.,1.),(1.,1.),(1.,1.),(1.,1.),(1.,1.),(1.,1.),(1.,1.),(1.,1.),(1.,
1.),(1.,1.),(1.,1.),(1.,1.),(1.,1.),(1.,1.),(1.,1.),(1.,1.),(1.,1.),(1.,
1.),(1.,1.),(1.,1.),(1.,1.),(1.,1.),(1.,1.),(1.,1.),(1.,1.),(1.,1.),(1.,
1.),(1.,1.),(1.,1.),(1.,1.),(1.,1.),(1.,1.),(1.,1.),(1.,1.),(1.,1.),(1.,
1.),(1.,1.),(1.,1.),(1.,1.),(1.,1.),(1.,1.),(1.,1.),(1.,1.),(1.,1.),(1.,
1.),(1.,1.),(1.,1.),(1.,1.),(1.,1.),(1.,1.),(1.,1.),(1.,1.),(1.,1.),(1.,
1.),(1.,1.),(1.,1.),(1.,1.),(1.,1.),(1.,1.),(1.,1.),(1.,1.),(1.,1.),(1.,
1.),(1.,1.),(1.,1.),(1.,1.),(1.,1.),(1.,1.),(1.,1.),(1.,1.),(1.,1.),(1.,
1.),(1.,1.),(1.,1.),(1.,1.),(1.,1.),(1.,1.),(1.,1.),(1.,1.),(1.,1.),(1.,
1.),(1.,1.),(1.,1.),(1.,1.),(1.,1.),(1.,1.),(1.,1.),(1.,1.),(1.,1.),(1.,
1.),(1.,1.),(1.,1.),(1.,1.),(1.,1.),(1.,1.),(1.,1.),(1.,1.),(1.,1.),(1.,
1.),(1.,1.),(1.,1.),(1.,1.),(1.,1.),(1.,1.),(1.,1.),(1.,1.),(1.,1.),(1.,
1.),(1.,1.),(1.,1.),(1.,1.),(1.,1.),(1.,1.),(1.,1.),(1.,1.),(1.,1.),(1.,
1.),(1.,1.),(1.,1.),(1.,1.),(1.,1.),(1.,1.),(1.,1.),(1.,1.),(1.,1.),(1.,
1.),(1.,1.)))
REPRESENTATION_ITEM('')
SURFACE()
);
#1022=(
BOUNDED_SURFACE()
B_SPLINE_SURFACE(5,1,((#170660,#170661),(#170662,#170663),(#170664,#170665),
(#170666,#170667),(#170668,#170669),(#170670,#170671),(#170672,#170673),
(#170674,#170675),(#170676,#170677),(#170678,#170679),(#170680,#170681),
(#170682,#170683),(#170684,#170685),(#170686,#170687),(#170688,#170689),
(#170690,#170691),(#170692,#170693),(#170694,#170695),(#170696,#170697),
(#170698,#170699),(#170700,#170701),(#170702,#170703),(#170704,#170705),
(#170706,#170707),(#170708,#170709),(#170710,#170711),(#170712,#170713),
(#170714,#170715),(#170716,#170717),(#170718,#170719),(#170720,#170721),
(#170722,#170723),(#170724,#170725),(#170726,#170727),(#170728,#170729),
(#170730,#170731),(#170732,#170733),(#170734,#170735),(#170736,#170737),
(#170738,#170739),(#170740,#170741),(#170742,#170743),(#170744,#170745),
(#170746,#170747),(#170748,#170749),(#170750,#170751),(#170752,#170753),
(#170754,#170755),(#170756,#170757),(#170758,#170759),(#170760,#170761),
(#170762,#170763),(#170764,#170765),(#170766,#170767),(#170768,#170769),
(#170770,#170771),(#170772,#170773),(#170774,#170775),(#170776,#170777),
(#170778,#170779),(#170780,#170781),(#170782,#170783),(#170784,#170785),
(#170786,#170787),(#170788,#170789),(#170790,#170791),(#170792,#170793),
(#170794,#170795),(#170796,#170797),(#170798,#170799),(#170800,#170801),
(#170802,#170803),(#170804,#170805),(#170806,#170807),(#170808,#170809),
(#170810,#170811),(#170812,#170813),(#170814,#170815),(#170816,#170817),
(#170818,#170819),(#170820,#170821),(#170822,#170823),(#170824,#170825),
(#170826,#170827),(#170828,#170829),(#170830,#170831),(#170832,#170833),
(#170834,#170835),(#170836,#170837),(#170838,#170839),(#170840,#170841),
(#170842,#170843),(#170844,#170845),(#170846,#170847),(#170848,#170849),
(#170850,#170851),(#170852,#170853),(#170854,#170855),(#170856,#170857),
(#170858,#170859),(#170860,#170861),(#170862,#170863),(#170864,#170865),
(#170866,#170867),(#170868,#170869),(#170870,#170871),(#170872,#170873),
(#170874,#170875),(#170876,#170877),(#170878,#170879),(#170880,#170881),
(#170882,#170883),(#170884,#170885),(#170886,#170887),(#170888,#170889),
(#170890,#170891),(#170892,#170893),(#170894,#170895),(#170896,#170897),
(#170898,#170899),(#170900,#170901),(#170902,#170903),(#170904,#170905),
(#170906,#170907),(#170908,#170909),(#170910,#170911),(#170912,#170913),
(#170914,#170915),(#170916,#170917),(#170918,#170919),(#170920,#170921),
(#170922,#170923),(#170924,#170925),(#170926,#170927),(#170928,#170929),
(#170930,#170931),(#170932,#170933),(#170934,#170935),(#170936,#170937),
(#170938,#170939),(#170940,#170941),(#170942,#170943),(#170944,#170945),
(#170946,#170947),(#170948,#170949),(#170950,#170951),(#170952,#170953),
(#170954,#170955),(#170956,#170957),(#170958,#170959),(#170960,#170961),
(#170962,#170963),(#170964,#170965),(#170966,#170967),(#170968,#170969),
(#170970,#170971),(#170972,#170973),(#170974,#170975),(#170976,#170977),
(#170978,#170979),(#170980,#170981),(#170982,#170983),(#170984,#170985),
(#170986,#170987),(#170988,#170989),(#170990,#170991),(#170992,#170993),
(#170994,#170995),(#170996,#170997),(#170998,#170999),(#171000,#171001),
(#171002,#171003),(#171004,#171005),(#171006,#171007),(#171008,#171009),
(#171010,#171011),(#171012,#171013),(#171014,#171015),(#171016,#171017),
(#171018,#171019),(#171020,#171021),(#171022,#171023),(#171024,#171025),
(#171026,#171027),(#171028,#171029),(#171030,#171031),(#171032,#171033),
(#171034,#171035),(#171036,#171037),(#171038,#171039),(#171040,#171041),
(#171042,#171043),(#171044,#171045),(#171046,#171047),(#171048,#171049),
(#171050,#171051),(#171052,#171053),(#171054,#171055),(#171056,#171057),
(#171058,#171059),(#171060,#171061),(#171062,#171063),(#171064,#171065),
(#171066,#171067),(#171068,#171069)),.UNSPECIFIED.,.F.,.F.,.F.)
B_SPLINE_SURFACE_WITH_KNOTS((6,1,1,1,1,1,1,1,1,1,1,1,1,1,1,1,1,1,1,1,1,
1,1,1,1,1,1,1,1,1,1,1,1,1,1,1,1,1,1,1,1,1,1,1,1,1,1,1,1,1,1,1,1,1,1,1,1,
1,1,1,1,1,1,1,1,1,1,1,1,1,1,1,1,1,1,1,1,1,1,1,1,1,1,1,1,1,1,1,1,1,1,1,1,
1,1,1,1,1,1,1,1,1,1,1,1,1,1,1,1,1,1,1,1,1,1,1,1,1,1,1,1,1,1,1,1,1,1,1,1,
1,1,1,1,1,1,1,1,1,1,1,1,1,1,1,1,1,1,1,1,1,1,1,1,1,1,1,1,1,1,1,1,1,1,1,1,
1,1,1,1,1,1,1,1,1,1,1,1,1,1,1,1,1,1,1,1,1,1,1,1,1,1,1,1,1,1,1,1,1,1,1,6),
(2,2),(-1.,-0.995000000000001,-0.990000000000001,-0.985000000000001,-0.980000000000001,
-0.975000000000001,-0.970000000000001,-0.965000000000001,-0.960000000000001,
-0.955000000000001,-0.950000000000001,-0.945000000000001,-0.940000000000001,
-0.935000000000001,-0.930000000000001,-0.925000000000001,-0.920000000000001,
-0.915000000000001,-0.910000000000001,-0.905000000000001,-0.900000000000001,
-0.895000000000001,-0.890000000000001,-0.885000000000001,-0.880000000000001,
-0.875000000000001,-0.870000000000001,-0.865000000000001,-0.860000000000001,
-0.855000000000001,-0.850000000000001,-0.845000000000001,-0.840000000000001,
-0.835000000000001,-0.830000000000001,-0.825000000000001,-0.820000000000001,
-0.815000000000001,-0.810000000000001,-0.805000000000001,-0.800000000000001,
-0.795000000000001,-0.790000000000001,-0.785000000000001,-0.780000000000001,
-0.775000000000001,-0.770000000000001,-0.765000000000001,-0.760000000000001,
-0.755000000000001,-0.750000000000001,-0.745000000000001,-0.740000000000001,
-0.735000000000001,-0.730000000000001,-0.725000000000001,-0.720000000000001,
-0.715000000000001,-0.710000000000001,-0.705000000000001,-0.700000000000001,
-0.695000000000001,-0.690000000000001,-0.685,-0.68,-0.675,-0.67,-0.665,
-0.66,-0.655,-0.65,-0.645,-0.64,-0.635,-0.63,-0.625,-0.62,-0.615,-0.61,
-0.605,-0.6,-0.595,-0.59,-0.585,-0.58,-0.575,-0.57,-0.565,-0.56,-0.555,
-0.55,-0.545,-0.54,-0.535,-0.53,-0.525,-0.52,-0.515,-0.51,-0.505,-0.5,-0.495,
-0.49,-0.485,-0.48,-0.475,-0.47,-0.465,-0.46,-0.455,-0.45,-0.445,-0.44,
-0.435,-0.43,-0.425,-0.42,-0.415,-0.41,-0.405,-0.4,-0.395,-0.39,-0.385,
-0.38,-0.375,-0.37,-0.365,-0.36,-0.355,-0.35,-0.345,-0.34,-0.335,-0.33,
-0.325,-0.32,-0.315,-0.31,-0.305,-0.3,-0.295,-0.29,-0.285,-0.28,-0.275,
-0.27,-0.265,-0.26,-0.255,-0.25,-0.245,-0.24,-0.235,-0.23,-0.225,-0.22,
-0.215,-0.21,-0.205,-0.2,-0.195,-0.19,-0.185,-0.18,-0.175,-0.17,-0.165,
-0.16,-0.155,-0.15,-0.145,-0.14,-0.135,-0.13,-0.125,-0.12,-0.115,-0.11,
-0.105,-0.1,-0.095,-0.09,-0.085,-0.08,-0.075,-0.07,-0.065,-0.06,-0.055,
-0.05,-0.045,-0.04,-0.035,-0.03,-0.025,-0.02,-0.015,-0.01,-0.005,0.),(0.,
1.2),.UNSPECIFIED.)
GEOMETRIC_REPRESENTATION_ITEM()
RATIONAL_B_SPLINE_SURFACE(((1.,1.),(1.,1.),(1.,1.),(1.,1.),(1.,1.),(1.,
1.),(1.,1.),(1.,1.),(1.,1.),(1.,1.),(1.,1.),(1.,1.),(1.,1.),(1.,1.),(1.,
1.),(1.,1.),(1.,1.),(1.,1.),(1.,1.),(1.,1.),(1.,1.),(1.,1.),(1.,1.),(1.,
1.),(1.,1.),(1.,1.),(1.,1.),(1.,1.),(1.,1.),(1.,1.),(1.,1.),(1.,1.),(1.,
1.),(1.,1.),(1.,1.),(1.,1.),(1.,1.),(1.,1.),(1.,1.),(1.,1.),(1.,1.),(1.,
1.),(1.,1.),(1.,1.),(1.,1.),(1.,1.),(1.,1.),(1.,1.),(1.,1.),(1.,1.),(1.,
1.),(1.,1.),(1.,1.),(1.,1.),(1.,1.),(1.,1.),(1.,1.),(1.,1.),(1.,1.),(1.,
1.),(1.,1.),(1.,1.),(1.,1.),(1.,1.),(1.,1.),(1.,1.),(1.,1.),(1.,1.),(1.,
1.),(1.,1.),(1.,1.),(1.,1.),(1.,1.),(1.,1.),(1.,1.),(1.,1.),(1.,1.),(1.,
1.),(1.,1.),(1.,1.),(1.,1.),(1.,1.),(1.,1.),(1.,1.),(1.,1.),(1.,1.),(1.,
1.),(1.,1.),(1.,1.),(1.,1.),(1.,1.),(1.,1.),(1.,1.),(1.,1.),(1.,1.),(1.,
1.),(1.,1.),(1.,1.),(1.,1.),(1.,1.),(1.,1.),(1.,1.),(1.,1.),(1.,1.),(1.,
1.),(1.,1.),(1.,1.),(1.,1.),(1.,1.),(1.,1.),(1.,1.),(1.,1.),(1.,1.),(1.,
1.),(1.,1.),(1.,1.),(1.,1.),(1.,1.),(1.,1.),(1.,1.),(1.,1.),(1.,1.),(1.,
1.),(1.,1.),(1.,1.),(1.,1.),(1.,1.),(1.,1.),(1.,1.),(1.,1.),(1.,1.),(1.,
1.),(1.,1.),(1.,1.),(1.,1.),(1.,1.),(1.,1.),(1.,1.),(1.,1.),(1.,1.),(1.,
1.),(1.,1.),(1.,1.),(1.,1.),(1.,1.),(1.,1.),(1.,1.),(1.,1.),(1.,1.),(1.,
1.),(1.,1.),(1.,1.),(1.,1.),(1.,1.),(1.,1.),(1.,1.),(1.,1.),(1.,1.),(1.,
1.),(1.,1.),(1.,1.),(1.,1.),(1.,1.),(1.,1.),(1.,1.),(1.,1.),(1.,1.),(1.,
1.),(1.,1.),(1.,1.),(1.,1.),(1.,1.),(1.,1.),(1.,1.),(1.,1.),(1.,1.),(1.,
1.),(1.,1.),(1.,1.),(1.,1.),(1.,1.),(1.,1.),(1.,1.),(1.,1.),(1.,1.),(1.,
1.),(1.,1.),(1.,1.),(1.,1.),(1.,1.),(1.,1.),(1.,1.),(1.,1.),(1.,1.),(1.,
1.),(1.,1.),(1.,1.),(1.,1.),(1.,1.),(1.,1.),(1.,1.),(1.,1.),(1.,1.),(1.,
1.),(1.,1.)))
REPRESENTATION_ITEM('')
SURFACE()
);
#1023=(
BOUNDED_SURFACE()
B_SPLINE_SURFACE(5,1,((#171461,#171462),(#171463,#171464),(#171465,#171466),
(#171467,#171468),(#171469,#171470),(#171471,#171472),(#171473,#171474),
(#171475,#171476),(#171477,#171478),(#171479,#171480),(#171481,#171482),
(#171483,#171484),(#171485,#171486),(#171487,#171488),(#171489,#171490),
(#171491,#171492),(#171493,#171494),(#171495,#171496),(#171497,#171498),
(#171499,#171500),(#171501,#171502),(#171503,#171504),(#171505,#171506),
(#171507,#171508),(#171509,#171510),(#171511,#171512),(#171513,#171514),
(#171515,#171516),(#171517,#171518),(#171519,#171520),(#171521,#171522),
(#171523,#171524),(#171525,#171526),(#171527,#171528),(#171529,#171530),
(#171531,#171532),(#171533,#171534),(#171535,#171536),(#171537,#171538),
(#171539,#171540),(#171541,#171542),(#171543,#171544),(#171545,#171546),
(#171547,#171548),(#171549,#171550),(#171551,#171552),(#171553,#171554),
(#171555,#171556),(#171557,#171558),(#171559,#171560),(#171561,#171562),
(#171563,#171564),(#171565,#171566),(#171567,#171568),(#171569,#171570),
(#171571,#171572),(#171573,#171574),(#171575,#171576),(#171577,#171578),
(#171579,#171580),(#171581,#171582),(#171583,#171584),(#171585,#171586),
(#171587,#171588),(#171589,#171590),(#171591,#171592),(#171593,#171594),
(#171595,#171596),(#171597,#171598),(#171599,#171600),(#171601,#171602),
(#171603,#171604),(#171605,#171606),(#171607,#171608),(#171609,#171610),
(#171611,#171612),(#171613,#171614),(#171615,#171616),(#171617,#171618),
(#171619,#171620),(#171621,#171622),(#171623,#171624),(#171625,#171626),
(#171627,#171628),(#171629,#171630),(#171631,#171632),(#171633,#171634),
(#171635,#171636),(#171637,#171638),(#171639,#171640),(#171641,#171642),
(#171643,#171644),(#171645,#171646),(#171647,#171648),(#171649,#171650),
(#171651,#171652),(#171653,#171654),(#171655,#171656),(#171657,#171658),
(#171659,#171660),(#171661,#171662),(#171663,#171664),(#171665,#171666),
(#171667,#171668),(#171669,#171670),(#171671,#171672),(#171673,#171674),
(#171675,#171676),(#171677,#171678),(#171679,#171680),(#171681,#171682),
(#171683,#171684),(#171685,#171686),(#171687,#171688),(#171689,#171690),
(#171691,#171692),(#171693,#171694),(#171695,#171696),(#171697,#171698),
(#171699,#171700),(#171701,#171702),(#171703,#171704),(#171705,#171706),
(#171707,#171708),(#171709,#171710),(#171711,#171712),(#171713,#171714),
(#171715,#171716),(#171717,#171718),(#171719,#171720),(#171721,#171722),
(#171723,#171724),(#171725,#171726),(#171727,#171728),(#171729,#171730),
(#171731,#171732),(#171733,#171734),(#171735,#171736),(#171737,#171738),
(#171739,#171740),(#171741,#171742),(#171743,#171744),(#171745,#171746),
(#171747,#171748),(#171749,#171750),(#171751,#171752),(#171753,#171754),
(#171755,#171756),(#171757,#171758),(#171759,#171760),(#171761,#171762),
(#171763,#171764),(#171765,#171766),(#171767,#171768),(#171769,#171770),
(#171771,#171772),(#171773,#171774),(#171775,#171776),(#171777,#171778),
(#171779,#171780),(#171781,#171782),(#171783,#171784),(#171785,#171786),
(#171787,#171788),(#171789,#171790),(#171791,#171792),(#171793,#171794),
(#171795,#171796),(#171797,#171798),(#171799,#171800),(#171801,#171802),
(#171803,#171804),(#171805,#171806),(#171807,#171808),(#171809,#171810),
(#171811,#171812),(#171813,#171814),(#171815,#171816),(#171817,#171818),
(#171819,#171820),(#171821,#171822),(#171823,#171824),(#171825,#171826),
(#171827,#171828),(#171829,#171830),(#171831,#171832),(#171833,#171834),
(#171835,#171836),(#171837,#171838),(#171839,#171840),(#171841,#171842),
(#171843,#171844),(#171845,#171846),(#171847,#171848),(#171849,#171850),
(#171851,#171852),(#171853,#171854),(#171855,#171856),(#171857,#171858),
(#171859,#171860),(#171861,#171862),(#171863,#171864),(#171865,#171866),
(#171867,#171868),(#171869,#171870)),.UNSPECIFIED.,.F.,.F.,.F.)
B_SPLINE_SURFACE_WITH_KNOTS((6,1,1,1,1,1,1,1,1,1,1,1,1,1,1,1,1,1,1,1,1,
1,1,1,1,1,1,1,1,1,1,1,1,1,1,1,1,1,1,1,1,1,1,1,1,1,1,1,1,1,1,1,1,1,1,1,1,
1,1,1,1,1,1,1,1,1,1,1,1,1,1,1,1,1,1,1,1,1,1,1,1,1,1,1,1,1,1,1,1,1,1,1,1,
1,1,1,1,1,1,1,1,1,1,1,1,1,1,1,1,1,1,1,1,1,1,1,1,1,1,1,1,1,1,1,1,1,1,1,1,
1,1,1,1,1,1,1,1,1,1,1,1,1,1,1,1,1,1,1,1,1,1,1,1,1,1,1,1,1,1,1,1,1,1,1,1,
1,1,1,1,1,1,1,1,1,1,1,1,1,1,1,1,1,1,1,1,1,1,1,1,1,1,1,1,1,1,1,1,1,1,1,6),
(2,2),(-1.,-0.995000000000001,-0.990000000000001,-0.985000000000001,-0.980000000000001,
-0.975000000000001,-0.970000000000001,-0.965000000000001,-0.960000000000001,
-0.955000000000001,-0.950000000000001,-0.945000000000001,-0.940000000000001,
-0.935000000000001,-0.930000000000001,-0.925000000000001,-0.920000000000001,
-0.915000000000001,-0.910000000000001,-0.905000000000001,-0.900000000000001,
-0.895000000000001,-0.890000000000001,-0.885000000000001,-0.880000000000001,
-0.875000000000001,-0.870000000000001,-0.865000000000001,-0.860000000000001,
-0.855000000000001,-0.850000000000001,-0.845000000000001,-0.840000000000001,
-0.835000000000001,-0.830000000000001,-0.825000000000001,-0.820000000000001,
-0.815000000000001,-0.810000000000001,-0.805000000000001,-0.800000000000001,
-0.795000000000001,-0.790000000000001,-0.785000000000001,-0.780000000000001,
-0.775000000000001,-0.770000000000001,-0.765000000000001,-0.760000000000001,
-0.755000000000001,-0.750000000000001,-0.745000000000001,-0.740000000000001,
-0.735000000000001,-0.730000000000001,-0.725000000000001,-0.720000000000001,
-0.715000000000001,-0.710000000000001,-0.705000000000001,-0.700000000000001,
-0.695000000000001,-0.690000000000001,-0.685,-0.68,-0.675,-0.67,-0.665,
-0.66,-0.655,-0.65,-0.645,-0.64,-0.635,-0.63,-0.625,-0.62,-0.615,-0.61,
-0.605,-0.6,-0.595,-0.59,-0.585,-0.58,-0.575,-0.57,-0.565,-0.56,-0.555,
-0.55,-0.545,-0.54,-0.535,-0.53,-0.525,-0.52,-0.515,-0.51,-0.505,-0.5,-0.495,
-0.49,-0.485,-0.48,-0.475,-0.47,-0.465,-0.46,-0.455,-0.45,-0.445,-0.44,
-0.435,-0.43,-0.425,-0.42,-0.415,-0.41,-0.405,-0.4,-0.395,-0.39,-0.385,
-0.38,-0.375,-0.37,-0.365,-0.36,-0.355,-0.35,-0.345,-0.34,-0.335,-0.33,
-0.325,-0.32,-0.315,-0.31,-0.305,-0.3,-0.295,-0.29,-0.285,-0.28,-0.275,
-0.27,-0.265,-0.26,-0.255,-0.25,-0.245,-0.24,-0.235,-0.23,-0.225,-0.22,
-0.215,-0.21,-0.205,-0.2,-0.195,-0.19,-0.185,-0.18,-0.175,-0.17,-0.165,
-0.16,-0.155,-0.15,-0.145,-0.14,-0.135,-0.13,-0.125,-0.12,-0.115,-0.11,
-0.105,-0.1,-0.095,-0.09,-0.085,-0.08,-0.075,-0.07,-0.065,-0.06,-0.055,
-0.05,-0.045,-0.04,-0.035,-0.03,-0.025,-0.02,-0.015,-0.01,-0.005,0.),(0.,
1.2),.UNSPECIFIED.)
GEOMETRIC_REPRESENTATION_ITEM()
RATIONAL_B_SPLINE_SURFACE(((1.,1.),(1.,1.),(1.,1.),(1.,1.),(1.,1.),(1.,
1.),(1.,1.),(1.,1.),(1.,1.),(1.,1.),(1.,1.),(1.,1.),(1.,1.),(1.,1.),(1.,
1.),(1.,1.),(1.,1.),(1.,1.),(1.,1.),(1.,1.),(1.,1.),(1.,1.),(1.,1.),(1.,
1.),(1.,1.),(1.,1.),(1.,1.),(1.,1.),(1.,1.),(1.,1.),(1.,1.),(1.,1.),(1.,
1.),(1.,1.),(1.,1.),(1.,1.),(1.,1.),(1.,1.),(1.,1.),(1.,1.),(1.,1.),(1.,
1.),(1.,1.),(1.,1.),(1.,1.),(1.,1.),(1.,1.),(1.,1.),(1.,1.),(1.,1.),(1.,
1.),(1.,1.),(1.,1.),(1.,1.),(1.,1.),(1.,1.),(1.,1.),(1.,1.),(1.,1.),(1.,
1.),(1.,1.),(1.,1.),(1.,1.),(1.,1.),(1.,1.),(1.,1.),(1.,1.),(1.,1.),(1.,
1.),(1.,1.),(1.,1.),(1.,1.),(1.,1.),(1.,1.),(1.,1.),(1.,1.),(1.,1.),(1.,
1.),(1.,1.),(1.,1.),(1.,1.),(1.,1.),(1.,1.),(1.,1.),(1.,1.),(1.,1.),(1.,
1.),(1.,1.),(1.,1.),(1.,1.),(1.,1.),(1.,1.),(1.,1.),(1.,1.),(1.,1.),(1.,
1.),(1.,1.),(1.,1.),(1.,1.),(1.,1.),(1.,1.),(1.,1.),(1.,1.),(1.,1.),(1.,
1.),(1.,1.),(1.,1.),(1.,1.),(1.,1.),(1.,1.),(1.,1.),(1.,1.),(1.,1.),(1.,
1.),(1.,1.),(1.,1.),(1.,1.),(1.,1.),(1.,1.),(1.,1.),(1.,1.),(1.,1.),(1.,
1.),(1.,1.),(1.,1.),(1.,1.),(1.,1.),(1.,1.),(1.,1.),(1.,1.),(1.,1.),(1.,
1.),(1.,1.),(1.,1.),(1.,1.),(1.,1.),(1.,1.),(1.,1.),(1.,1.),(1.,1.),(1.,
1.),(1.,1.),(1.,1.),(1.,1.),(1.,1.),(1.,1.),(1.,1.),(1.,1.),(1.,1.),(1.,
1.),(1.,1.),(1.,1.),(1.,1.),(1.,1.),(1.,1.),(1.,1.),(1.,1.),(1.,1.),(1.,
1.),(1.,1.),(1.,1.),(1.,1.),(1.,1.),(1.,1.),(1.,1.),(1.,1.),(1.,1.),(1.,
1.),(1.,1.),(1.,1.),(1.,1.),(1.,1.),(1.,1.),(1.,1.),(1.,1.),(1.,1.),(1.,
1.),(1.,1.),(1.,1.),(1.,1.),(1.,1.),(1.,1.),(1.,1.),(1.,1.),(1.,1.),(1.,
1.),(1.,1.),(1.,1.),(1.,1.),(1.,1.),(1.,1.),(1.,1.),(1.,1.),(1.,1.),(1.,
1.),(1.,1.),(1.,1.),(1.,1.),(1.,1.),(1.,1.),(1.,1.),(1.,1.),(1.,1.),(1.,
1.),(1.,1.)))
REPRESENTATION_ITEM('')
SURFACE()
);
#1024=(
BOUNDED_SURFACE()
B_SPLINE_SURFACE(5,1,((#172262,#172263),(#172264,#172265),(#172266,#172267),
(#172268,#172269),(#172270,#172271),(#172272,#172273),(#172274,#172275),
(#172276,#172277),(#172278,#172279),(#172280,#172281),(#172282,#172283),
(#172284,#172285),(#172286,#172287),(#172288,#172289),(#172290,#172291),
(#172292,#172293),(#172294,#172295),(#172296,#172297),(#172298,#172299),
(#172300,#172301),(#172302,#172303),(#172304,#172305),(#172306,#172307),
(#172308,#172309),(#172310,#172311),(#172312,#172313),(#172314,#172315),
(#172316,#172317),(#172318,#172319),(#172320,#172321),(#172322,#172323),
(#172324,#172325),(#172326,#172327),(#172328,#172329),(#172330,#172331),
(#172332,#172333),(#172334,#172335),(#172336,#172337),(#172338,#172339),
(#172340,#172341),(#172342,#172343),(#172344,#172345),(#172346,#172347),
(#172348,#172349),(#172350,#172351),(#172352,#172353),(#172354,#172355),
(#172356,#172357),(#172358,#172359),(#172360,#172361),(#172362,#172363),
(#172364,#172365),(#172366,#172367),(#172368,#172369),(#172370,#172371),
(#172372,#172373),(#172374,#172375),(#172376,#172377),(#172378,#172379),
(#172380,#172381),(#172382,#172383),(#172384,#172385),(#172386,#172387),
(#172388,#172389),(#172390,#172391),(#172392,#172393),(#172394,#172395),
(#172396,#172397),(#172398,#172399),(#172400,#172401),(#172402,#172403),
(#172404,#172405),(#172406,#172407),(#172408,#172409),(#172410,#172411),
(#172412,#172413),(#172414,#172415),(#172416,#172417),(#172418,#172419),
(#172420,#172421),(#172422,#172423),(#172424,#172425),(#172426,#172427),
(#172428,#172429),(#172430,#172431),(#172432,#172433),(#172434,#172435),
(#172436,#172437),(#172438,#172439),(#172440,#172441),(#172442,#172443),
(#172444,#172445),(#172446,#172447),(#172448,#172449),(#172450,#172451),
(#172452,#172453),(#172454,#172455),(#172456,#172457),(#172458,#172459),
(#172460,#172461),(#172462,#172463),(#172464,#172465),(#172466,#172467),
(#172468,#172469),(#172470,#172471),(#172472,#172473),(#172474,#172475),
(#172476,#172477),(#172478,#172479),(#172480,#172481),(#172482,#172483),
(#172484,#172485),(#172486,#172487),(#172488,#172489),(#172490,#172491),
(#172492,#172493),(#172494,#172495),(#172496,#172497),(#172498,#172499),
(#172500,#172501),(#172502,#172503),(#172504,#172505),(#172506,#172507),
(#172508,#172509),(#172510,#172511),(#172512,#172513),(#172514,#172515),
(#172516,#172517),(#172518,#172519),(#172520,#172521),(#172522,#172523),
(#172524,#172525),(#172526,#172527),(#172528,#172529),(#172530,#172531),
(#172532,#172533),(#172534,#172535),(#172536,#172537),(#172538,#172539),
(#172540,#172541),(#172542,#172543),(#172544,#172545),(#172546,#172547),
(#172548,#172549),(#172550,#172551),(#172552,#172553),(#172554,#172555),
(#172556,#172557),(#172558,#172559),(#172560,#172561),(#172562,#172563),
(#172564,#172565),(#172566,#172567),(#172568,#172569),(#172570,#172571),
(#172572,#172573),(#172574,#172575),(#172576,#172577),(#172578,#172579),
(#172580,#172581),(#172582,#172583),(#172584,#172585),(#172586,#172587),
(#172588,#172589),(#172590,#172591),(#172592,#172593),(#172594,#172595),
(#172596,#172597),(#172598,#172599),(#172600,#172601),(#172602,#172603),
(#172604,#172605),(#172606,#172607),(#172608,#172609),(#172610,#172611),
(#172612,#172613),(#172614,#172615),(#172616,#172617),(#172618,#172619),
(#172620,#172621),(#172622,#172623),(#172624,#172625),(#172626,#172627),
(#172628,#172629),(#172630,#172631),(#172632,#172633),(#172634,#172635),
(#172636,#172637),(#172638,#172639),(#172640,#172641),(#172642,#172643),
(#172644,#172645),(#172646,#172647),(#172648,#172649),(#172650,#172651),
(#172652,#172653),(#172654,#172655),(#172656,#172657),(#172658,#172659),
(#172660,#172661),(#172662,#172663),(#172664,#172665),(#172666,#172667),
(#172668,#172669),(#172670,#172671)),.UNSPECIFIED.,.F.,.F.,.F.)
B_SPLINE_SURFACE_WITH_KNOTS((6,1,1,1,1,1,1,1,1,1,1,1,1,1,1,1,1,1,1,1,1,
1,1,1,1,1,1,1,1,1,1,1,1,1,1,1,1,1,1,1,1,1,1,1,1,1,1,1,1,1,1,1,1,1,1,1,1,
1,1,1,1,1,1,1,1,1,1,1,1,1,1,1,1,1,1,1,1,1,1,1,1,1,1,1,1,1,1,1,1,1,1,1,1,
1,1,1,1,1,1,1,1,1,1,1,1,1,1,1,1,1,1,1,1,1,1,1,1,1,1,1,1,1,1,1,1,1,1,1,1,
1,1,1,1,1,1,1,1,1,1,1,1,1,1,1,1,1,1,1,1,1,1,1,1,1,1,1,1,1,1,1,1,1,1,1,1,
1,1,1,1,1,1,1,1,1,1,1,1,1,1,1,1,1,1,1,1,1,1,1,1,1,1,1,1,1,1,1,1,1,1,1,6),
(2,2),(-1.,-0.995000000000001,-0.990000000000001,-0.985000000000001,-0.980000000000001,
-0.975000000000001,-0.970000000000001,-0.965000000000001,-0.960000000000001,
-0.955000000000001,-0.950000000000001,-0.945000000000001,-0.940000000000001,
-0.935000000000001,-0.930000000000001,-0.925000000000001,-0.920000000000001,
-0.915000000000001,-0.910000000000001,-0.905000000000001,-0.900000000000001,
-0.895000000000001,-0.890000000000001,-0.885000000000001,-0.880000000000001,
-0.875000000000001,-0.870000000000001,-0.865000000000001,-0.860000000000001,
-0.855000000000001,-0.850000000000001,-0.845000000000001,-0.840000000000001,
-0.835000000000001,-0.830000000000001,-0.825000000000001,-0.820000000000001,
-0.815000000000001,-0.810000000000001,-0.805000000000001,-0.800000000000001,
-0.795000000000001,-0.790000000000001,-0.785000000000001,-0.780000000000001,
-0.775000000000001,-0.770000000000001,-0.765000000000001,-0.760000000000001,
-0.755000000000001,-0.750000000000001,-0.745000000000001,-0.740000000000001,
-0.735000000000001,-0.730000000000001,-0.725000000000001,-0.720000000000001,
-0.715000000000001,-0.710000000000001,-0.705000000000001,-0.700000000000001,
-0.695000000000001,-0.690000000000001,-0.685,-0.68,-0.675,-0.67,-0.665,
-0.66,-0.655,-0.65,-0.645,-0.64,-0.635,-0.63,-0.625,-0.62,-0.615,-0.61,
-0.605,-0.6,-0.595,-0.59,-0.585,-0.58,-0.575,-0.57,-0.565,-0.56,-0.555,
-0.55,-0.545,-0.54,-0.535,-0.53,-0.525,-0.52,-0.515,-0.51,-0.505,-0.5,-0.495,
-0.49,-0.485,-0.48,-0.475,-0.47,-0.465,-0.46,-0.455,-0.45,-0.445,-0.44,
-0.435,-0.43,-0.425,-0.42,-0.415,-0.41,-0.405,-0.4,-0.395,-0.39,-0.385,
-0.38,-0.375,-0.37,-0.365,-0.36,-0.355,-0.35,-0.345,-0.34,-0.335,-0.33,
-0.325,-0.32,-0.315,-0.31,-0.305,-0.3,-0.295,-0.29,-0.285,-0.28,-0.275,
-0.27,-0.265,-0.26,-0.255,-0.25,-0.245,-0.24,-0.235,-0.23,-0.225,-0.22,
-0.215,-0.21,-0.205,-0.2,-0.195,-0.19,-0.185,-0.18,-0.175,-0.17,-0.165,
-0.16,-0.155,-0.15,-0.145,-0.14,-0.135,-0.13,-0.125,-0.12,-0.115,-0.11,
-0.105,-0.1,-0.095,-0.09,-0.085,-0.08,-0.075,-0.07,-0.065,-0.06,-0.055,
-0.05,-0.045,-0.04,-0.035,-0.03,-0.025,-0.02,-0.015,-0.01,-0.005,0.),(0.,
1.2),.UNSPECIFIED.)
GEOMETRIC_REPRESENTATION_ITEM()
RATIONAL_B_SPLINE_SURFACE(((1.,1.),(1.,1.),(1.,1.),(1.,1.),(1.,1.),(1.,
1.),(1.,1.),(1.,1.),(1.,1.),(1.,1.),(1.,1.),(1.,1.),(1.,1.),(1.,1.),(1.,
1.),(1.,1.),(1.,1.),(1.,1.),(1.,1.),(1.,1.),(1.,1.),(1.,1.),(1.,1.),(1.,
1.),(1.,1.),(1.,1.),(1.,1.),(1.,1.),(1.,1.),(1.,1.),(1.,1.),(1.,1.),(1.,
1.),(1.,1.),(1.,1.),(1.,1.),(1.,1.),(1.,1.),(1.,1.),(1.,1.),(1.,1.),(1.,
1.),(1.,1.),(1.,1.),(1.,1.),(1.,1.),(1.,1.),(1.,1.),(1.,1.),(1.,1.),(1.,
1.),(1.,1.),(1.,1.),(1.,1.),(1.,1.),(1.,1.),(1.,1.),(1.,1.),(1.,1.),(1.,
1.),(1.,1.),(1.,1.),(1.,1.),(1.,1.),(1.,1.),(1.,1.),(1.,1.),(1.,1.),(1.,
1.),(1.,1.),(1.,1.),(1.,1.),(1.,1.),(1.,1.),(1.,1.),(1.,1.),(1.,1.),(1.,
1.),(1.,1.),(1.,1.),(1.,1.),(1.,1.),(1.,1.),(1.,1.),(1.,1.),(1.,1.),(1.,
1.),(1.,1.),(1.,1.),(1.,1.),(1.,1.),(1.,1.),(1.,1.),(1.,1.),(1.,1.),(1.,
1.),(1.,1.),(1.,1.),(1.,1.),(1.,1.),(1.,1.),(1.,1.),(1.,1.),(1.,1.),(1.,
1.),(1.,1.),(1.,1.),(1.,1.),(1.,1.),(1.,1.),(1.,1.),(1.,1.),(1.,1.),(1.,
1.),(1.,1.),(1.,1.),(1.,1.),(1.,1.),(1.,1.),(1.,1.),(1.,1.),(1.,1.),(1.,
1.),(1.,1.),(1.,1.),(1.,1.),(1.,1.),(1.,1.),(1.,1.),(1.,1.),(1.,1.),(1.,
1.),(1.,1.),(1.,1.),(1.,1.),(1.,1.),(1.,1.),(1.,1.),(1.,1.),(1.,1.),(1.,
1.),(1.,1.),(1.,1.),(1.,1.),(1.,1.),(1.,1.),(1.,1.),(1.,1.),(1.,1.),(1.,
1.),(1.,1.),(1.,1.),(1.,1.),(1.,1.),(1.,1.),(1.,1.),(1.,1.),(1.,1.),(1.,
1.),(1.,1.),(1.,1.),(1.,1.),(1.,1.),(1.,1.),(1.,1.),(1.,1.),(1.,1.),(1.,
1.),(1.,1.),(1.,1.),(1.,1.),(1.,1.),(1.,1.),(1.,1.),(1.,1.),(1.,1.),(1.,
1.),(1.,1.),(1.,1.),(1.,1.),(1.,1.),(1.,1.),(1.,1.),(1.,1.),(1.,1.),(1.,
1.),(1.,1.),(1.,1.),(1.,1.),(1.,1.),(1.,1.),(1.,1.),(1.,1.),(1.,1.),(1.,
1.),(1.,1.),(1.,1.),(1.,1.),(1.,1.),(1.,1.),(1.,1.),(1.,1.),(1.,1.),(1.,
1.),(1.,1.)))
REPRESENTATION_ITEM('')
SURFACE()
);
#1025=(
BOUNDED_SURFACE()
B_SPLINE_SURFACE(5,1,((#173328,#173329),(#173330,#173331),(#173332,#173333),
(#173334,#173335),(#173336,#173337),(#173338,#173339),(#173340,#173341),
(#173342,#173343),(#173344,#173345),(#173346,#173347),(#173348,#173349),
(#173350,#173351),(#173352,#173353),(#173354,#173355),(#173356,#173357),
(#173358,#173359),(#173360,#173361),(#173362,#173363),(#173364,#173365),
(#173366,#173367),(#173368,#173369),(#173370,#173371),(#173372,#173373),
(#173374,#173375),(#173376,#173377),(#173378,#173379),(#173380,#173381),
(#173382,#173383),(#173384,#173385),(#173386,#173387),(#173388,#173389),
(#173390,#173391),(#173392,#173393),(#173394,#173395),(#173396,#173397),
(#173398,#173399),(#173400,#173401),(#173402,#173403),(#173404,#173405),
(#173406,#173407),(#173408,#173409),(#173410,#173411),(#173412,#173413),
(#173414,#173415),(#173416,#173417),(#173418,#173419),(#173420,#173421),
(#173422,#173423),(#173424,#173425),(#173426,#173427),(#173428,#173429),
(#173430,#173431),(#173432,#173433),(#173434,#173435),(#173436,#173437),
(#173438,#173439),(#173440,#173441),(#173442,#173443),(#173444,#173445),
(#173446,#173447),(#173448,#173449),(#173450,#173451),(#173452,#173453),
(#173454,#173455),(#173456,#173457),(#173458,#173459),(#173460,#173461),
(#173462,#173463),(#173464,#173465),(#173466,#173467),(#173468,#173469),
(#173470,#173471),(#173472,#173473),(#173474,#173475),(#173476,#173477),
(#173478,#173479),(#173480,#173481),(#173482,#173483),(#173484,#173485),
(#173486,#173487),(#173488,#173489),(#173490,#173491),(#173492,#173493),
(#173494,#173495),(#173496,#173497),(#173498,#173499),(#173500,#173501),
(#173502,#173503),(#173504,#173505),(#173506,#173507),(#173508,#173509),
(#173510,#173511),(#173512,#173513),(#173514,#173515),(#173516,#173517),
(#173518,#173519),(#173520,#173521),(#173522,#173523),(#173524,#173525),
(#173526,#173527),(#173528,#173529),(#173530,#173531),(#173532,#173533),
(#173534,#173535),(#173536,#173537),(#173538,#173539),(#173540,#173541),
(#173542,#173543),(#173544,#173545),(#173546,#173547),(#173548,#173549),
(#173550,#173551),(#173552,#173553),(#173554,#173555),(#173556,#173557),
(#173558,#173559),(#173560,#173561),(#173562,#173563),(#173564,#173565),
(#173566,#173567),(#173568,#173569),(#173570,#173571),(#173572,#173573),
(#173574,#173575),(#173576,#173577),(#173578,#173579),(#173580,#173581),
(#173582,#173583),(#173584,#173585),(#173586,#173587),(#173588,#173589),
(#173590,#173591),(#173592,#173593),(#173594,#173595),(#173596,#173597),
(#173598,#173599),(#173600,#173601),(#173602,#173603),(#173604,#173605),
(#173606,#173607),(#173608,#173609),(#173610,#173611),(#173612,#173613),
(#173614,#173615),(#173616,#173617),(#173618,#173619),(#173620,#173621),
(#173622,#173623),(#173624,#173625),(#173626,#173627),(#173628,#173629),
(#173630,#173631),(#173632,#173633),(#173634,#173635),(#173636,#173637),
(#173638,#173639),(#173640,#173641),(#173642,#173643),(#173644,#173645),
(#173646,#173647),(#173648,#173649),(#173650,#173651),(#173652,#173653),
(#173654,#173655),(#173656,#173657),(#173658,#173659),(#173660,#173661),
(#173662,#173663),(#173664,#173665),(#173666,#173667),(#173668,#173669),
(#173670,#173671),(#173672,#173673),(#173674,#173675),(#173676,#173677),
(#173678,#173679),(#173680,#173681),(#173682,#173683),(#173684,#173685),
(#173686,#173687),(#173688,#173689),(#173690,#173691),(#173692,#173693),
(#173694,#173695),(#173696,#173697),(#173698,#173699),(#173700,#173701),
(#173702,#173703),(#173704,#173705),(#173706,#173707),(#173708,#173709),
(#173710,#173711),(#173712,#173713),(#173714,#173715),(#173716,#173717),
(#173718,#173719),(#173720,#173721),(#173722,#173723),(#173724,#173725),
(#173726,#173727),(#173728,#173729),(#173730,#173731),(#173732,#173733),
(#173734,#173735),(#173736,#173737)),.UNSPECIFIED.,.F.,.F.,.F.)
B_SPLINE_SURFACE_WITH_KNOTS((6,1,1,1,1,1,1,1,1,1,1,1,1,1,1,1,1,1,1,1,1,
1,1,1,1,1,1,1,1,1,1,1,1,1,1,1,1,1,1,1,1,1,1,1,1,1,1,1,1,1,1,1,1,1,1,1,1,
1,1,1,1,1,1,1,1,1,1,1,1,1,1,1,1,1,1,1,1,1,1,1,1,1,1,1,1,1,1,1,1,1,1,1,1,
1,1,1,1,1,1,1,1,1,1,1,1,1,1,1,1,1,1,1,1,1,1,1,1,1,1,1,1,1,1,1,1,1,1,1,1,
1,1,1,1,1,1,1,1,1,1,1,1,1,1,1,1,1,1,1,1,1,1,1,1,1,1,1,1,1,1,1,1,1,1,1,1,
1,1,1,1,1,1,1,1,1,1,1,1,1,1,1,1,1,1,1,1,1,1,1,1,1,1,1,1,1,1,1,1,1,1,1,6),
(2,2),(0.,0.005,0.01,0.015,0.02,0.025,0.03,0.035,0.04,0.045,0.05,0.055,
0.06,0.065,0.07,0.075,0.08,0.085,0.09,0.095,0.1,0.105,0.11,0.115,0.12,0.125,
0.13,0.135,0.14,0.145,0.15,0.155,0.16,0.165,0.17,0.175,0.18,0.185,0.19,
0.195,0.2,0.205,0.21,0.215,0.22,0.225,0.23,0.235,0.24,0.245,0.25,0.255,
0.26,0.265,0.27,0.275,0.28,0.285,0.29,0.295,0.3,0.305,0.31,0.315,0.32,0.325,
0.33,0.335,0.34,0.345,0.35,0.355,0.36,0.365,0.37,0.375,0.38,0.385,0.39,
0.395,0.4,0.405,0.41,0.415,0.42,0.425,0.43,0.435,0.44,0.445,0.45,0.455,
0.46,0.465,0.47,0.475,0.48,0.485,0.49,0.495,0.5,0.505,0.51,0.515,0.52,0.525,
0.53,0.535,0.54,0.545,0.55,0.555,0.56,0.565,0.57,0.575,0.58,0.585,0.59,
0.595,0.6,0.605,0.61,0.615,0.62,0.625,0.63,0.635,0.64,0.645,0.65,0.655,
0.66,0.665,0.67,0.675,0.68,0.685,0.690000000000001,0.695000000000001,0.700000000000001,
0.705000000000001,0.710000000000001,0.715000000000001,0.720000000000001,
0.725000000000001,0.730000000000001,0.735000000000001,0.740000000000001,
0.745000000000001,0.750000000000001,0.755000000000001,0.760000000000001,
0.765000000000001,0.770000000000001,0.775000000000001,0.780000000000001,
0.785000000000001,0.790000000000001,0.795000000000001,0.800000000000001,
0.805000000000001,0.810000000000001,0.815000000000001,0.820000000000001,
0.825000000000001,0.830000000000001,0.835000000000001,0.840000000000001,
0.845000000000001,0.850000000000001,0.855000000000001,0.860000000000001,
0.865000000000001,0.870000000000001,0.875000000000001,0.880000000000001,
0.885000000000001,0.890000000000001,0.895000000000001,0.900000000000001,
0.905000000000001,0.910000000000001,0.915000000000001,0.920000000000001,
0.925000000000001,0.930000000000001,0.935000000000001,0.940000000000001,
0.945000000000001,0.950000000000001,0.955000000000001,0.960000000000001,
0.965000000000001,0.970000000000001,0.975000000000001,0.980000000000001,
0.985000000000001,0.990000000000001,0.995000000000001,1.),(0.,1.2),
 .UNSPECIFIED.)
GEOMETRIC_REPRESENTATION_ITEM()
RATIONAL_B_SPLINE_SURFACE(((1.,1.),(1.,1.),(1.,1.),(1.,1.),(1.,1.),(1.,
1.),(1.,1.),(1.,1.),(1.,1.),(1.,1.),(1.,1.),(1.,1.),(1.,1.),(1.,1.),(1.,
1.),(1.,1.),(1.,1.),(1.,1.),(1.,1.),(1.,1.),(1.,1.),(1.,1.),(1.,1.),(1.,
1.),(1.,1.),(1.,1.),(1.,1.),(1.,1.),(1.,1.),(1.,1.),(1.,1.),(1.,1.),(1.,
1.),(1.,1.),(1.,1.),(1.,1.),(1.,1.),(1.,1.),(1.,1.),(1.,1.),(1.,1.),(1.,
1.),(1.,1.),(1.,1.),(1.,1.),(1.,1.),(1.,1.),(1.,1.),(1.,1.),(1.,1.),(1.,
1.),(1.,1.),(1.,1.),(1.,1.),(1.,1.),(1.,1.),(1.,1.),(1.,1.),(1.,1.),(1.,
1.),(1.,1.),(1.,1.),(1.,1.),(1.,1.),(1.,1.),(1.,1.),(1.,1.),(1.,1.),(1.,
1.),(1.,1.),(1.,1.),(1.,1.),(1.,1.),(1.,1.),(1.,1.),(1.,1.),(1.,1.),(1.,
1.),(1.,1.),(1.,1.),(1.,1.),(1.,1.),(1.,1.),(1.,1.),(1.,1.),(1.,1.),(1.,
1.),(1.,1.),(1.,1.),(1.,1.),(1.,1.),(1.,1.),(1.,1.),(1.,1.),(1.,1.),(1.,
1.),(1.,1.),(1.,1.),(1.,1.),(1.,1.),(1.,1.),(1.,1.),(1.,1.),(1.,1.),(1.,
1.),(1.,1.),(1.,1.),(1.,1.),(1.,1.),(1.,1.),(1.,1.),(1.,1.),(1.,1.),(1.,
1.),(1.,1.),(1.,1.),(1.,1.),(1.,1.),(1.,1.),(1.,1.),(1.,1.),(1.,1.),(1.,
1.),(1.,1.),(1.,1.),(1.,1.),(1.,1.),(1.,1.),(1.,1.),(1.,1.),(1.,1.),(1.,
1.),(1.,1.),(1.,1.),(1.,1.),(1.,1.),(1.,1.),(1.,1.),(1.,1.),(1.,1.),(1.,
1.),(1.,1.),(1.,1.),(1.,1.),(1.,1.),(1.,1.),(1.,1.),(1.,1.),(1.,1.),(1.,
1.),(1.,1.),(1.,1.),(1.,1.),(1.,1.),(1.,1.),(1.,1.),(1.,1.),(1.,1.),(1.,
1.),(1.,1.),(1.,1.),(1.,1.),(1.,1.),(1.,1.),(1.,1.),(1.,1.),(1.,1.),(1.,
1.),(1.,1.),(1.,1.),(1.,1.),(1.,1.),(1.,1.),(1.,1.),(1.,1.),(1.,1.),(1.,
1.),(1.,1.),(1.,1.),(1.,1.),(1.,1.),(1.,1.),(1.,1.),(1.,1.),(1.,1.),(1.,
1.),(1.,1.),(1.,1.),(1.,1.),(1.,1.),(1.,1.),(1.,1.),(1.,1.),(1.,1.),(1.,
1.),(1.,1.),(1.,1.),(1.,1.),(1.,1.),(1.,1.),(1.,1.),(1.,1.),(1.,1.),(1.,
1.),(1.,1.)))
REPRESENTATION_ITEM('')
SURFACE()
);
#1026=(
BOUNDED_SURFACE()
B_SPLINE_SURFACE(5,1,((#174175,#174176),(#174177,#174178),(#174179,#174180),
(#174181,#174182),(#174183,#174184),(#174185,#174186),(#174187,#174188),
(#174189,#174190),(#174191,#174192),(#174193,#174194),(#174195,#174196),
(#174197,#174198),(#174199,#174200),(#174201,#174202),(#174203,#174204),
(#174205,#174206),(#174207,#174208),(#174209,#174210),(#174211,#174212),
(#174213,#174214),(#174215,#174216),(#174217,#174218),(#174219,#174220),
(#174221,#174222),(#174223,#174224),(#174225,#174226),(#174227,#174228),
(#174229,#174230),(#174231,#174232),(#174233,#174234),(#174235,#174236),
(#174237,#174238),(#174239,#174240),(#174241,#174242),(#174243,#174244),
(#174245,#174246),(#174247,#174248),(#174249,#174250),(#174251,#174252),
(#174253,#174254),(#174255,#174256),(#174257,#174258),(#174259,#174260),
(#174261,#174262),(#174263,#174264),(#174265,#174266),(#174267,#174268),
(#174269,#174270),(#174271,#174272),(#174273,#174274),(#174275,#174276),
(#174277,#174278),(#174279,#174280),(#174281,#174282),(#174283,#174284),
(#174285,#174286),(#174287,#174288),(#174289,#174290),(#174291,#174292),
(#174293,#174294),(#174295,#174296),(#174297,#174298),(#174299,#174300),
(#174301,#174302),(#174303,#174304),(#174305,#174306),(#174307,#174308),
(#174309,#174310),(#174311,#174312),(#174313,#174314),(#174315,#174316),
(#174317,#174318),(#174319,#174320),(#174321,#174322),(#174323,#174324),
(#174325,#174326),(#174327,#174328),(#174329,#174330),(#174331,#174332),
(#174333,#174334),(#174335,#174336),(#174337,#174338),(#174339,#174340),
(#174341,#174342),(#174343,#174344),(#174345,#174346),(#174347,#174348),
(#174349,#174350),(#174351,#174352),(#174353,#174354),(#174355,#174356),
(#174357,#174358),(#174359,#174360),(#174361,#174362),(#174363,#174364),
(#174365,#174366),(#174367,#174368),(#174369,#174370),(#174371,#174372),
(#174373,#174374),(#174375,#174376),(#174377,#174378),(#174379,#174380),
(#174381,#174382),(#174383,#174384),(#174385,#174386),(#174387,#174388),
(#174389,#174390),(#174391,#174392),(#174393,#174394),(#174395,#174396),
(#174397,#174398),(#174399,#174400),(#174401,#174402),(#174403,#174404),
(#174405,#174406),(#174407,#174408),(#174409,#174410),(#174411,#174412),
(#174413,#174414),(#174415,#174416),(#174417,#174418),(#174419,#174420),
(#174421,#174422),(#174423,#174424),(#174425,#174426),(#174427,#174428),
(#174429,#174430),(#174431,#174432),(#174433,#174434),(#174435,#174436),
(#174437,#174438),(#174439,#174440),(#174441,#174442),(#174443,#174444),
(#174445,#174446),(#174447,#174448),(#174449,#174450),(#174451,#174452),
(#174453,#174454),(#174455,#174456),(#174457,#174458),(#174459,#174460),
(#174461,#174462),(#174463,#174464),(#174465,#174466),(#174467,#174468),
(#174469,#174470),(#174471,#174472),(#174473,#174474),(#174475,#174476),
(#174477,#174478),(#174479,#174480),(#174481,#174482),(#174483,#174484),
(#174485,#174486),(#174487,#174488),(#174489,#174490),(#174491,#174492),
(#174493,#174494),(#174495,#174496),(#174497,#174498),(#174499,#174500),
(#174501,#174502),(#174503,#174504),(#174505,#174506),(#174507,#174508),
(#174509,#174510),(#174511,#174512),(#174513,#174514),(#174515,#174516),
(#174517,#174518),(#174519,#174520),(#174521,#174522),(#174523,#174524),
(#174525,#174526),(#174527,#174528),(#174529,#174530),(#174531,#174532),
(#174533,#174534),(#174535,#174536),(#174537,#174538),(#174539,#174540),
(#174541,#174542),(#174543,#174544),(#174545,#174546),(#174547,#174548),
(#174549,#174550),(#174551,#174552),(#174553,#174554),(#174555,#174556),
(#174557,#174558),(#174559,#174560),(#174561,#174562),(#174563,#174564),
(#174565,#174566),(#174567,#174568),(#174569,#174570),(#174571,#174572),
(#174573,#174574),(#174575,#174576),(#174577,#174578),(#174579,#174580),
(#174581,#174582),(#174583,#174584)),.UNSPECIFIED.,.F.,.F.,.F.)
B_SPLINE_SURFACE_WITH_KNOTS((6,1,1,1,1,1,1,1,1,1,1,1,1,1,1,1,1,1,1,1,1,
1,1,1,1,1,1,1,1,1,1,1,1,1,1,1,1,1,1,1,1,1,1,1,1,1,1,1,1,1,1,1,1,1,1,1,1,
1,1,1,1,1,1,1,1,1,1,1,1,1,1,1,1,1,1,1,1,1,1,1,1,1,1,1,1,1,1,1,1,1,1,1,1,
1,1,1,1,1,1,1,1,1,1,1,1,1,1,1,1,1,1,1,1,1,1,1,1,1,1,1,1,1,1,1,1,1,1,1,1,
1,1,1,1,1,1,1,1,1,1,1,1,1,1,1,1,1,1,1,1,1,1,1,1,1,1,1,1,1,1,1,1,1,1,1,1,
1,1,1,1,1,1,1,1,1,1,1,1,1,1,1,1,1,1,1,1,1,1,1,1,1,1,1,1,1,1,1,1,1,1,1,6),
(2,2),(-1.,-0.995000000000001,-0.990000000000001,-0.985000000000001,-0.980000000000001,
-0.975000000000001,-0.970000000000001,-0.965000000000001,-0.960000000000001,
-0.955000000000001,-0.950000000000001,-0.945000000000001,-0.940000000000001,
-0.935000000000001,-0.930000000000001,-0.925000000000001,-0.920000000000001,
-0.915000000000001,-0.910000000000001,-0.905000000000001,-0.900000000000001,
-0.895000000000001,-0.890000000000001,-0.885000000000001,-0.880000000000001,
-0.875000000000001,-0.870000000000001,-0.865000000000001,-0.860000000000001,
-0.855000000000001,-0.850000000000001,-0.845000000000001,-0.840000000000001,
-0.835000000000001,-0.830000000000001,-0.825000000000001,-0.820000000000001,
-0.815000000000001,-0.810000000000001,-0.805000000000001,-0.800000000000001,
-0.795000000000001,-0.790000000000001,-0.785000000000001,-0.780000000000001,
-0.775000000000001,-0.770000000000001,-0.765000000000001,-0.760000000000001,
-0.755000000000001,-0.750000000000001,-0.745000000000001,-0.740000000000001,
-0.735000000000001,-0.730000000000001,-0.725000000000001,-0.720000000000001,
-0.715000000000001,-0.710000000000001,-0.705000000000001,-0.700000000000001,
-0.695000000000001,-0.690000000000001,-0.685,-0.68,-0.675,-0.67,-0.665,
-0.66,-0.655,-0.65,-0.645,-0.64,-0.635,-0.63,-0.625,-0.62,-0.615,-0.61,
-0.605,-0.6,-0.595,-0.59,-0.585,-0.58,-0.575,-0.57,-0.565,-0.56,-0.555,
-0.55,-0.545,-0.54,-0.535,-0.53,-0.525,-0.52,-0.515,-0.51,-0.505,-0.5,-0.495,
-0.49,-0.485,-0.48,-0.475,-0.47,-0.465,-0.46,-0.455,-0.45,-0.445,-0.44,
-0.435,-0.43,-0.425,-0.42,-0.415,-0.41,-0.405,-0.4,-0.395,-0.39,-0.385,
-0.38,-0.375,-0.37,-0.365,-0.36,-0.355,-0.35,-0.345,-0.34,-0.335,-0.33,
-0.325,-0.32,-0.315,-0.31,-0.305,-0.3,-0.295,-0.29,-0.285,-0.28,-0.275,
-0.27,-0.265,-0.26,-0.255,-0.25,-0.245,-0.24,-0.235,-0.23,-0.225,-0.22,
-0.215,-0.21,-0.205,-0.2,-0.195,-0.19,-0.185,-0.18,-0.175,-0.17,-0.165,
-0.16,-0.155,-0.15,-0.145,-0.14,-0.135,-0.13,-0.125,-0.12,-0.115,-0.11,
-0.105,-0.1,-0.095,-0.09,-0.085,-0.08,-0.075,-0.07,-0.065,-0.06,-0.055,
-0.05,-0.045,-0.04,-0.035,-0.03,-0.025,-0.02,-0.015,-0.01,-0.005,0.),(0.,
1.2),.UNSPECIFIED.)
GEOMETRIC_REPRESENTATION_ITEM()
RATIONAL_B_SPLINE_SURFACE(((1.,1.),(1.,1.),(1.,1.),(1.,1.),(1.,1.),(1.,
1.),(1.,1.),(1.,1.),(1.,1.),(1.,1.),(1.,1.),(1.,1.),(1.,1.),(1.,1.),(1.,
1.),(1.,1.),(1.,1.),(1.,1.),(1.,1.),(1.,1.),(1.,1.),(1.,1.),(1.,1.),(1.,
1.),(1.,1.),(1.,1.),(1.,1.),(1.,1.),(1.,1.),(1.,1.),(1.,1.),(1.,1.),(1.,
1.),(1.,1.),(1.,1.),(1.,1.),(1.,1.),(1.,1.),(1.,1.),(1.,1.),(1.,1.),(1.,
1.),(1.,1.),(1.,1.),(1.,1.),(1.,1.),(1.,1.),(1.,1.),(1.,1.),(1.,1.),(1.,
1.),(1.,1.),(1.,1.),(1.,1.),(1.,1.),(1.,1.),(1.,1.),(1.,1.),(1.,1.),(1.,
1.),(1.,1.),(1.,1.),(1.,1.),(1.,1.),(1.,1.),(1.,1.),(1.,1.),(1.,1.),(1.,
1.),(1.,1.),(1.,1.),(1.,1.),(1.,1.),(1.,1.),(1.,1.),(1.,1.),(1.,1.),(1.,
1.),(1.,1.),(1.,1.),(1.,1.),(1.,1.),(1.,1.),(1.,1.),(1.,1.),(1.,1.),(1.,
1.),(1.,1.),(1.,1.),(1.,1.),(1.,1.),(1.,1.),(1.,1.),(1.,1.),(1.,1.),(1.,
1.),(1.,1.),(1.,1.),(1.,1.),(1.,1.),(1.,1.),(1.,1.),(1.,1.),(1.,1.),(1.,
1.),(1.,1.),(1.,1.),(1.,1.),(1.,1.),(1.,1.),(1.,1.),(1.,1.),(1.,1.),(1.,
1.),(1.,1.),(1.,1.),(1.,1.),(1.,1.),(1.,1.),(1.,1.),(1.,1.),(1.,1.),(1.,
1.),(1.,1.),(1.,1.),(1.,1.),(1.,1.),(1.,1.),(1.,1.),(1.,1.),(1.,1.),(1.,
1.),(1.,1.),(1.,1.),(1.,1.),(1.,1.),(1.,1.),(1.,1.),(1.,1.),(1.,1.),(1.,
1.),(1.,1.),(1.,1.),(1.,1.),(1.,1.),(1.,1.),(1.,1.),(1.,1.),(1.,1.),(1.,
1.),(1.,1.),(1.,1.),(1.,1.),(1.,1.),(1.,1.),(1.,1.),(1.,1.),(1.,1.),(1.,
1.),(1.,1.),(1.,1.),(1.,1.),(1.,1.),(1.,1.),(1.,1.),(1.,1.),(1.,1.),(1.,
1.),(1.,1.),(1.,1.),(1.,1.),(1.,1.),(1.,1.),(1.,1.),(1.,1.),(1.,1.),(1.,
1.),(1.,1.),(1.,1.),(1.,1.),(1.,1.),(1.,1.),(1.,1.),(1.,1.),(1.,1.),(1.,
1.),(1.,1.),(1.,1.),(1.,1.),(1.,1.),(1.,1.),(1.,1.),(1.,1.),(1.,1.),(1.,
1.),(1.,1.),(1.,1.),(1.,1.),(1.,1.),(1.,1.),(1.,1.),(1.,1.),(1.,1.),(1.,
1.),(1.,1.)))
REPRESENTATION_ITEM('')
SURFACE()
);
#1127=SHAPE_REPRESENTATION_RELATIONSHIP('SRR','None',#259374,#1147);
#1147=ADVANCED_BREP_SHAPE_REPRESENTATION('',(#1187),#259208);
#1167=STYLED_ITEM('',(#259483),#1187);
#1187=MANIFOLD_SOLID_BREP('Gear blank',#25154);
#1276=FACE_BOUND('',#3923,.T.);
#1277=FACE_BOUND('',#3926,.T.);
#1278=FACE_BOUND('',#3927,.T.);
#1279=FACE_BOUND('',#3928,.T.);
#1280=FACE_BOUND('',#3930,.T.);
#1334=B_SPLINE_SURFACE_WITH_KNOTS('',3,3,((#52576,#52577,#52578,#52579),
(#52580,#52581,#52582,#52583),(#52584,#52585,#52586,#52587),(#52588,#52589,
#52590,#52591),(#52592,#52593,#52594,#52595)),.UNSPECIFIED.,.F.,.F.,.F.,
(4,1,4),(4,4),(0.,0.571428571428571,1.),(-2.77555756156289E-17,1.2),
 .UNSPECIFIED.);
#1335=B_SPLINE_SURFACE_WITH_KNOTS('',3,3,((#53423,#53424,#53425,#53426),
(#53427,#53428,#53429,#53430),(#53431,#53432,#53433,#53434),(#53435,#53436,
#53437,#53438),(#53439,#53440,#53441,#53442)),.UNSPECIFIED.,.F.,.F.,.F.,
(4,1,4),(4,4),(0.,0.571428571428571,1.),(0.,1.2),.UNSPECIFIED.);
#1336=B_SPLINE_SURFACE_WITH_KNOTS('',3,3,((#53472,#53473,#53474,#53475),
(#53476,#53477,#53478,#53479),(#53480,#53481,#53482,#53483),(#53484,#53485,
#53486,#53487),(#53488,#53489,#53490,#53491)),.UNSPECIFIED.,.F.,.F.,.F.,
(4,1,4),(4,4),(0.,0.571428571428571,1.),(9.71445146547012E-17,1.2),
 .UNSPECIFIED.);
#1337=B_SPLINE_SURFACE_WITH_KNOTS('',3,3,((#54319,#54320,#54321,#54322),
(#54323,#54324,#54325,#54326),(#54327,#54328,#54329,#54330),(#54331,#54332,
#54333,#54334),(#54335,#54336,#54337,#54338)),.UNSPECIFIED.,.F.,.F.,.F.,
(4,1,4),(4,4),(0.,0.571428571428571,1.),(-6.97125684381022E-36,1.2),
 .UNSPECIFIED.);
#1338=B_SPLINE_SURFACE_WITH_KNOTS('',3,3,((#54368,#54369,#54370,#54371),
(#54372,#54373,#54374,#54375),(#54376,#54377,#54378,#54379),(#54380,#54381,
#54382,#54383),(#54384,#54385,#54386,#54387)),.UNSPECIFIED.,.F.,.F.,.F.,
(4,1,4),(4,4),(0.,0.571428571428571,1.),(4.06042677328019E-17,1.2),
 .UNSPECIFIED.);
#1339=B_SPLINE_SURFACE_WITH_KNOTS('',3,3,((#55215,#55216,#55217,#55218),
(#55219,#55220,#55221,#55222),(#55223,#55224,#55225,#55226),(#55227,#55228,
#55229,#55230),(#55231,#55232,#55233,#55234)),.UNSPECIFIED.,.F.,.F.,.F.,
(4,1,4),(4,4),(0.,0.571428571428571,1.),(-8.32667268468868E-17,1.2),
 .UNSPECIFIED.);
#1340=B_SPLINE_SURFACE_WITH_KNOTS('',3,3,((#55264,#55265,#55266,#55267),
(#55268,#55269,#55270,#55271),(#55272,#55273,#55274,#55275),(#55276,#55277,
#55278,#55279),(#55280,#55281,#55282,#55283)),.UNSPECIFIED.,.F.,.F.,.F.,
(4,1,4),(4,4),(0.,0.571428571428571,1.),(9.71445146547012E-17,1.2),
 .UNSPECIFIED.);
#1341=B_SPLINE_SURFACE_WITH_KNOTS('',3,3,((#56111,#56112,#56113,#56114),
(#56115,#56116,#56117,#56118),(#56119,#56120,#56121,#56122),(#56123,#56124,
#56125,#56126),(#56127,#56128,#56129,#56130)),.UNSPECIFIED.,.F.,.F.,.F.,
(4,1,4),(4,4),(0.,0.571428571428571,1.),(2.77555756156289E-17,1.2),
 .UNSPECIFIED.);
#1342=B_SPLINE_SURFACE_WITH_KNOTS('',3,3,((#56160,#56161,#56162,#56163),
(#56164,#56165,#56166,#56167),(#56168,#56169,#56170,#56171),(#56172,#56173,
#56174,#56175),(#56176,#56177,#56178,#56179)),.UNSPECIFIED.,.F.,.F.,.F.,
(4,1,4),(4,4),(0.,0.571428571428571,1.),(1.66533453693773E-16,1.2),
 .UNSPECIFIED.);
#1343=B_SPLINE_SURFACE_WITH_KNOTS('',3,3,((#57007,#57008,#57009,#57010),
(#57011,#57012,#57013,#57014),(#57015,#57016,#57017,#57018),(#57019,#57020,
#57021,#57022),(#57023,#57024,#57025,#57026)),.UNSPECIFIED.,.F.,.F.,.F.,
(4,1,4),(4,4),(0.,0.571428571428571,1.),(-4.16333634234434E-17,1.2),
 .UNSPECIFIED.);
#1344=B_SPLINE_SURFACE_WITH_KNOTS('',3,3,((#57056,#57057,#57058,#57059),
(#57060,#57061,#57062,#57063),(#57064,#57065,#57066,#57067),(#57068,#57069,
#57070,#57071),(#57072,#57073,#57074,#57075)),.UNSPECIFIED.,.F.,.F.,.F.,
(4,1,4),(4,4),(0.,0.571428571428571,1.),(1.38777878078145E-16,1.2),
 .UNSPECIFIED.);
#1345=B_SPLINE_SURFACE_WITH_KNOTS('',3,3,((#57903,#57904,#57905,#57906),
(#57907,#57908,#57909,#57910),(#57911,#57912,#57913,#57914),(#57915,#57916,
#57917,#57918),(#57919,#57920,#57921,#57922)),.UNSPECIFIED.,.F.,.F.,.F.,
(4,1,4),(4,4),(0.,0.571428571428571,1.),(-8.43563892506861E-17,1.2),
 .UNSPECIFIED.);
#1346=B_SPLINE_SURFACE_WITH_KNOTS('',3,3,((#57952,#57953,#57954,#57955),
(#57956,#57957,#57958,#57959),(#57960,#57961,#57962,#57963),(#57964,#57965,
#57966,#57967),(#57968,#57969,#57970,#57971)),.UNSPECIFIED.,.F.,.F.,.F.,
(4,1,4),(4,4),(0.,0.571428571428571,1.),(1.66533453693773E-16,1.2),
 .UNSPECIFIED.);
#1347=B_SPLINE_SURFACE_WITH_KNOTS('',3,3,((#58799,#58800,#58801,#58802),
(#58803,#58804,#58805,#58806),(#58807,#58808,#58809,#58810),(#58811,#58812,
#58813,#58814),(#58815,#58816,#58817,#58818)),.UNSPECIFIED.,.F.,.F.,.F.,
(4,1,4),(4,4),(0.,0.571428571428571,1.),(2.77555756156289E-17,1.2),
 .UNSPECIFIED.);
#1348=B_SPLINE_SURFACE_WITH_KNOTS('',3,3,((#58848,#58849,#58850,#58851),
(#58852,#58853,#58854,#58855),(#58856,#58857,#58858,#58859),(#58860,#58861,
#58862,#58863),(#58864,#58865,#58866,#58867)),.UNSPECIFIED.,.F.,.F.,.F.,
(4,1,4),(4,4),(0.,0.571428571428571,1.),(-8.32667268468868E-17,1.2),
 .UNSPECIFIED.);
#1349=B_SPLINE_SURFACE_WITH_KNOTS('',3,3,((#59695,#59696,#59697,#59698),
(#59699,#59700,#59701,#59702),(#59703,#59704,#59705,#59706),(#59707,#59708,
#59709,#59710),(#59711,#59712,#59713,#59714)),.UNSPECIFIED.,.F.,.F.,.F.,
(4,1,4),(4,4),(0.,0.571428571428571,1.),(5.55111512312578E-17,1.2),
 .UNSPECIFIED.);
#1350=B_SPLINE_SURFACE_WITH_KNOTS('',3,3,((#59744,#59745,#59746,#59747),
(#59748,#59749,#59750,#59751),(#59752,#59753,#59754,#59755),(#59756,#59757,
#59758,#59759),(#59760,#59761,#59762,#59763)),.UNSPECIFIED.,.F.,.F.,.F.,
(4,1,4),(4,4),(0.,0.571428571428571,1.),(1.66533453693773E-16,1.2),
 .UNSPECIFIED.);
#1351=B_SPLINE_SURFACE_WITH_KNOTS('',3,3,((#60591,#60592,#60593,#60594),
(#60595,#60596,#60597,#60598),(#60599,#60600,#60601,#60602),(#60603,#60604,
#60605,#60606),(#60607,#60608,#60609,#60610)),.UNSPECIFIED.,.F.,.F.,.F.,
(4,1,4),(4,4),(0.,0.571428571428571,1.),(-8.9628248557339E-17,1.2),
 .UNSPECIFIED.);
#1352=B_SPLINE_SURFACE_WITH_KNOTS('',3,3,((#60640,#60641,#60642,#60643),
(#60644,#60645,#60646,#60647),(#60648,#60649,#60650,#60651),(#60652,#60653,
#60654,#60655),(#60656,#60657,#60658,#60659)),.UNSPECIFIED.,.F.,.F.,.F.,
(4,1,4),(4,4),(0.,0.571428571428571,1.),(8.0522471671843E-17,1.2),
 .UNSPECIFIED.);
#1353=B_SPLINE_SURFACE_WITH_KNOTS('',3,3,((#61487,#61488,#61489,#61490),
(#61491,#61492,#61493,#61494),(#61495,#61496,#61497,#61498),(#61499,#61500,
#61501,#61502),(#61503,#61504,#61505,#61506)),.UNSPECIFIED.,.F.,.F.,.F.,
(4,1,4),(4,4),(0.,0.571428571428571,1.),(-7.52391395153922E-36,1.2),
 .UNSPECIFIED.);
#1354=B_SPLINE_SURFACE_WITH_KNOTS('',3,3,((#61536,#61537,#61538,#61539),
(#61540,#61541,#61542,#61543),(#61544,#61545,#61546,#61547),(#61548,#61549,
#61550,#61551),(#61552,#61553,#61554,#61555)),.UNSPECIFIED.,.F.,.F.,.F.,
(4,1,4),(4,4),(0.,0.571428571428571,1.),(9.71445146547012E-17,1.2),
 .UNSPECIFIED.);
#1355=B_SPLINE_SURFACE_WITH_KNOTS('',3,3,((#62383,#62384,#62385,#62386),
(#62387,#62388,#62389,#62390),(#62391,#62392,#62393,#62394),(#62395,#62396,
#62397,#62398),(#62399,#62400,#62401,#62402)),.UNSPECIFIED.,.F.,.F.,.F.,
(4,1,4),(4,4),(0.,0.571428571428571,1.),(2.77555756156289E-17,1.2),
 .UNSPECIFIED.);
#1356=B_SPLINE_SURFACE_WITH_KNOTS('',3,3,((#62432,#62433,#62434,#62435),
(#62436,#62437,#62438,#62439),(#62440,#62441,#62442,#62443),(#62444,#62445,
#62446,#62447),(#62448,#62449,#62450,#62451)),.UNSPECIFIED.,.F.,.F.,.F.,
(4,1,4),(4,4),(0.,0.571428571428571,1.),(6.66446838640284E-17,1.2),
 .UNSPECIFIED.);
#1357=B_SPLINE_SURFACE_WITH_KNOTS('',3,3,((#63279,#63280,#63281,#63282),
(#63283,#63284,#63285,#63286),(#63287,#63288,#63289,#63290),(#63291,#63292,
#63293,#63294),(#63295,#63296,#63297,#63298)),.UNSPECIFIED.,.F.,.F.,.F.,
(4,1,4),(4,4),(0.,0.571428571428571,1.),(-4.16333634234434E-17,1.2),
 .UNSPECIFIED.);
#1358=B_SPLINE_SURFACE_WITH_KNOTS('',3,3,((#63328,#63329,#63330,#63331),
(#63332,#63333,#63334,#63335),(#63336,#63337,#63338,#63339),(#63340,#63341,
#63342,#63343),(#63344,#63345,#63346,#63347)),.UNSPECIFIED.,.F.,.F.,.F.,
(4,1,4),(4,4),(0.,0.571428571428571,1.),(0.,1.2),.UNSPECIFIED.);
#1359=B_SPLINE_SURFACE_WITH_KNOTS('',3,3,((#64175,#64176,#64177,#64178),
(#64179,#64180,#64181,#64182),(#64183,#64184,#64185,#64186),(#64187,#64188,
#64189,#64190),(#64191,#64192,#64193,#64194)),.UNSPECIFIED.,.F.,.F.,.F.,
(4,1,4),(4,4),(0.,0.571428571428571,1.),(2.77555756156289E-17,1.2),
 .UNSPECIFIED.);
#1360=B_SPLINE_SURFACE_WITH_KNOTS('',3,3,((#64224,#64225,#64226,#64227),
(#64228,#64229,#64230,#64231),(#64232,#64233,#64234,#64235),(#64236,#64237,
#64238,#64239),(#64240,#64241,#64242,#64243)),.UNSPECIFIED.,.F.,.F.,.F.,
(4,1,4),(4,4),(0.,0.571428571428571,1.),(9.71445146547012E-17,1.2),
 .UNSPECIFIED.);
#1361=B_SPLINE_SURFACE_WITH_KNOTS('',3,3,((#65071,#65072,#65073,#65074),
(#65075,#65076,#65077,#65078),(#65079,#65080,#65081,#65082),(#65083,#65084,
#65085,#65086),(#65087,#65088,#65089,#65090)),.UNSPECIFIED.,.F.,.F.,.F.,
(4,1,4),(4,4),(0.,0.571428571428571,1.),(-1.11022302462516E-16,1.2),
 .UNSPECIFIED.);
#1362=B_SPLINE_SURFACE_WITH_KNOTS('',3,3,((#65120,#65121,#65122,#65123),
(#65124,#65125,#65126,#65127),(#65128,#65129,#65130,#65131),(#65132,#65133,
#65134,#65135),(#65136,#65137,#65138,#65139)),.UNSPECIFIED.,.F.,.F.,.F.,
(4,1,4),(4,4),(0.,0.571428571428571,1.),(6.66446838640285E-17,1.2),
 .UNSPECIFIED.);
#1363=B_SPLINE_SURFACE_WITH_KNOTS('',3,3,((#65967,#65968,#65969,#65970),
(#65971,#65972,#65973,#65974),(#65975,#65976,#65977,#65978),(#65979,#65980,
#65981,#65982),(#65983,#65984,#65985,#65986)),.UNSPECIFIED.,.F.,.F.,.F.,
(4,1,4),(4,4),(0.,0.571428571428571,1.),(2.77555756156289E-17,1.2),
 .UNSPECIFIED.);
#1364=B_SPLINE_SURFACE_WITH_KNOTS('',3,3,((#66016,#66017,#66018,#66019),
(#66020,#66021,#66022,#66023),(#66024,#66025,#66026,#66027),(#66028,#66029,
#66030,#66031),(#66032,#66033,#66034,#66035)),.UNSPECIFIED.,.F.,.F.,.F.,
(4,1,4),(4,4),(0.,0.571428571428571,1.),(6.93889390390723E-17,1.2),
 .UNSPECIFIED.);
#1365=B_SPLINE_SURFACE_WITH_KNOTS('',3,3,((#66863,#66864,#66865,#66866),
(#66867,#66868,#66869,#66870),(#66871,#66872,#66873,#66874),(#66875,#66876,
#66877,#66878),(#66879,#66880,#66881,#66882)),.UNSPECIFIED.,.F.,.F.,.F.,
(4,1,4),(4,4),(0.,0.571428571428571,1.),(0.,1.2),.UNSPECIFIED.);
#1366=B_SPLINE_SURFACE_WITH_KNOTS('',3,3,((#66912,#66913,#66914,#66915),
(#66916,#66917,#66918,#66919),(#66920,#66921,#66922,#66923),(#66924,#66925,
#66926,#66927),(#66928,#66929,#66930,#66931)),.UNSPECIFIED.,.F.,.F.,.F.,
(4,1,4),(4,4),(0.,0.571428571428571,1.),(8.32667268468867E-17,1.2),
 .UNSPECIFIED.);
#1367=B_SPLINE_SURFACE_WITH_KNOTS('',3,3,((#67759,#67760,#67761,#67762),
(#67763,#67764,#67765,#67766),(#67767,#67768,#67769,#67770),(#67771,#67772,
#67773,#67774),(#67775,#67776,#67777,#67778)),.UNSPECIFIED.,.F.,.F.,.F.,
(4,1,4),(4,4),(0.,0.571428571428571,1.),(-5.55111512312578E-17,1.2),
 .UNSPECIFIED.);
#1368=B_SPLINE_SURFACE_WITH_KNOTS('',3,3,((#67808,#67809,#67810,#67811),
(#67812,#67813,#67814,#67815),(#67816,#67817,#67818,#67819),(#67820,#67821,
#67822,#67823),(#67824,#67825,#67826,#67827)),.UNSPECIFIED.,.F.,.F.,.F.,
(4,1,4),(4,4),(0.,0.571428571428571,1.),(0.,1.2),.UNSPECIFIED.);
#1369=B_SPLINE_SURFACE_WITH_KNOTS('',3,3,((#68655,#68656,#68657,#68658),
(#68659,#68660,#68661,#68662),(#68663,#68664,#68665,#68666),(#68667,#68668,
#68669,#68670),(#68671,#68672,#68673,#68674)),.UNSPECIFIED.,.F.,.F.,.F.,
(4,1,4),(4,4),(0.,0.571428571428571,1.),(-8.32667268468868E-17,1.2),
 .UNSPECIFIED.);
#1370=B_SPLINE_SURFACE_WITH_KNOTS('',3,3,((#68704,#68705,#68706,#68707),
(#68708,#68709,#68710,#68711),(#68712,#68713,#68714,#68715),(#68716,#68717,
#68718,#68719),(#68720,#68721,#68722,#68723)),.UNSPECIFIED.,.F.,.F.,.F.,
(4,1,4),(4,4),(0.,0.571428571428571,1.),(9.71445146547012E-17,1.2),
 .UNSPECIFIED.);
#1371=B_SPLINE_SURFACE_WITH_KNOTS('',3,3,((#69551,#69552,#69553,#69554),
(#69555,#69556,#69557,#69558),(#69559,#69560,#69561,#69562),(#69563,#69564,
#69565,#69566),(#69567,#69568,#69569,#69570)),.UNSPECIFIED.,.F.,.F.,.F.,
(4,1,4),(4,4),(0.,0.571428571428571,1.),(-2.74425517504386E-18,1.2),
 .UNSPECIFIED.);
#1372=B_SPLINE_SURFACE_WITH_KNOTS('',3,3,((#69600,#69601,#69602,#69603),
(#69604,#69605,#69606,#69607),(#69608,#69609,#69610,#69611),(#69612,#69613,
#69614,#69615),(#69616,#69617,#69618,#69619)),.UNSPECIFIED.,.F.,.F.,.F.,
(4,1,4),(4,4),(0.,0.571428571428571,1.),(8.0522471671843E-17,1.2),
 .UNSPECIFIED.);
#1373=B_SPLINE_SURFACE_WITH_KNOTS('',3,3,((#70447,#70448,#70449,#70450),
(#70451,#70452,#70453,#70454),(#70455,#70456,#70457,#70458),(#70459,#70460,
#70461,#70462),(#70463,#70464,#70465,#70466)),.UNSPECIFIED.,.F.,.F.,.F.,
(4,1,4),(4,4),(0.,0.571428571428571,1.),(-1.38777878078145E-16,1.2),
 .UNSPECIFIED.);
#1374=B_SPLINE_SURFACE_WITH_KNOTS('',3,3,((#70496,#70497,#70498,#70499),
(#70500,#70501,#70502,#70503),(#70504,#70505,#70506,#70507),(#70508,#70509,
#70510,#70511),(#70512,#70513,#70514,#70515)),.UNSPECIFIED.,.F.,.F.,.F.,
(4,1,4),(4,4),(0.,0.571428571428571,1.),(8.32667268468867E-17,1.2),
 .UNSPECIFIED.);
#1375=B_SPLINE_SURFACE_WITH_KNOTS('',3,3,((#71343,#71344,#71345,#71346),
(#71347,#71348,#71349,#71350),(#71351,#71352,#71353,#71354),(#71355,#71356,
#71357,#71358),(#71359,#71360,#71361,#71362)),.UNSPECIFIED.,.F.,.F.,.F.,
(4,1,4),(4,4),(0.,0.571428571428571,1.),(0.,1.2),.UNSPECIFIED.);
#1376=B_SPLINE_SURFACE_WITH_KNOTS('',3,3,((#71392,#71393,#71394,#71395),
(#71396,#71397,#71398,#71399),(#71400,#71401,#71402,#71403),(#71404,#71405,
#71406,#71407),(#71408,#71409,#71410,#71411)),.UNSPECIFIED.,.F.,.F.,.F.,
(4,1,4),(4,4),(0.,0.571428571428571,1.),(1.66533453693773E-16,1.2),
 .UNSPECIFIED.);
#1377=B_SPLINE_SURFACE_WITH_KNOTS('',3,3,((#72239,#72240,#72241,#72242),
(#72243,#72244,#72245,#72246),(#72247,#72248,#72249,#72250),(#72251,#72252,
#72253,#72254),(#72255,#72256,#72257,#72258)),.UNSPECIFIED.,.F.,.F.,.F.,
(4,1,4),(4,4),(0.,0.571428571428571,1.),(-1.38777878078145E-16,1.2),
 .UNSPECIFIED.);
#1378=B_SPLINE_SURFACE_WITH_KNOTS('',3,3,((#72288,#72289,#72290,#72291),
(#72292,#72293,#72294,#72295),(#72296,#72297,#72298,#72299),(#72300,#72301,
#72302,#72303),(#72304,#72305,#72306,#72307)),.UNSPECIFIED.,.F.,.F.,.F.,
(4,1,4),(4,4),(0.,0.571428571428571,1.),(-2.08166817117217E-17,1.2),
 .UNSPECIFIED.);
#1379=B_SPLINE_SURFACE_WITH_KNOTS('',3,3,((#73135,#73136,#73137,#73138),
(#73139,#73140,#73141,#73142),(#73143,#73144,#73145,#73146),(#73147,#73148,
#73149,#73150),(#73151,#73152,#73153,#73154)),.UNSPECIFIED.,.F.,.F.,.F.,
(4,1,4),(4,4),(0.,0.571428571428571,1.),(-8.32667268468868E-17,1.2),
 .UNSPECIFIED.);
#1380=B_SPLINE_SURFACE_WITH_KNOTS('',3,3,((#73184,#73185,#73186,#73187),
(#73188,#73189,#73190,#73191),(#73192,#73193,#73194,#73195),(#73196,#73197,
#73198,#73199),(#73200,#73201,#73202,#73203)),.UNSPECIFIED.,.F.,.F.,.F.,
(4,1,4),(4,4),(0.,0.571428571428571,1.),(1.38777878078145E-16,1.2),
 .UNSPECIFIED.);
#1381=B_SPLINE_SURFACE_WITH_KNOTS('',3,3,((#74031,#74032,#74033,#74034),
(#74035,#74036,#74037,#74038),(#74039,#74040,#74041,#74042),(#74043,#74044,
#74045,#74046),(#74047,#74048,#74049,#74050)),.UNSPECIFIED.,.F.,.F.,.F.,
(4,1,4),(4,4),(0.,0.571428571428571,1.),(-8.43563892506861E-17,1.2),
 .UNSPECIFIED.);
#1382=B_SPLINE_SURFACE_WITH_KNOTS('',3,3,((#74080,#74081,#74082,#74083),
(#74084,#74085,#74086,#74087),(#74088,#74089,#74090,#74091),(#74092,#74093,
#74094,#74095),(#74096,#74097,#74098,#74099)),.UNSPECIFIED.,.F.,.F.,.F.,
(4,1,4),(4,4),(0.,0.571428571428571,1.),(9.71445146547012E-17,1.2),
 .UNSPECIFIED.);
#1383=B_SPLINE_SURFACE_WITH_KNOTS('',3,3,((#74927,#74928,#74929,#74930),
(#74931,#74932,#74933,#74934),(#74935,#74936,#74937,#74938),(#74939,#74940,
#74941,#74942),(#74943,#74944,#74945,#74946)),.UNSPECIFIED.,.F.,.F.,.F.,
(4,1,4),(4,4),(0.,0.571428571428571,1.),(0.,1.2),.UNSPECIFIED.);
#1384=B_SPLINE_SURFACE_WITH_KNOTS('',3,3,((#74976,#74977,#74978,#74979),
(#74980,#74981,#74982,#74983),(#74984,#74985,#74986,#74987),(#74988,#74989,
#74990,#74991),(#74992,#74993,#74994,#74995)),.UNSPECIFIED.,.F.,.F.,.F.,
(4,1,4),(4,4),(0.,0.571428571428571,1.),(9.71445146547012E-17,1.2),
 .UNSPECIFIED.);
#1385=B_SPLINE_SURFACE_WITH_KNOTS('',3,3,((#75823,#75824,#75825,#75826),
(#75827,#75828,#75829,#75830),(#75831,#75832,#75833,#75834),(#75835,#75836,
#75837,#75838),(#75839,#75840,#75841,#75842)),.UNSPECIFIED.,.F.,.F.,.F.,
(4,1,4),(4,4),(0.,0.571428571428571,1.),(-1.49437708898837E-16,1.2),
 .UNSPECIFIED.);
#1386=B_SPLINE_SURFACE_WITH_KNOTS('',3,3,((#75872,#75873,#75874,#75875),
(#75876,#75877,#75878,#75879),(#75880,#75881,#75882,#75883),(#75884,#75885,
#75886,#75887),(#75888,#75889,#75890,#75891)),.UNSPECIFIED.,.F.,.F.,.F.,
(4,1,4),(4,4),(0.,0.571428571428571,1.),(9.71445146547012E-17,1.2),
 .UNSPECIFIED.);
#1387=B_SPLINE_SURFACE_WITH_KNOTS('',3,3,((#76719,#76720,#76721,#76722),
(#76723,#76724,#76725,#76726),(#76727,#76728,#76729,#76730),(#76731,#76732,
#76733,#76734),(#76735,#76736,#76737,#76738)),.UNSPECIFIED.,.F.,.F.,.F.,
(4,1,4),(4,4),(0.,0.571428571428571,1.),(0.,1.2),.UNSPECIFIED.);
#1388=B_SPLINE_SURFACE_WITH_KNOTS('',3,3,((#76768,#76769,#76770,#76771),
(#76772,#76773,#76774,#76775),(#76776,#76777,#76778,#76779),(#76780,#76781,
#76782,#76783),(#76784,#76785,#76786,#76787)),.UNSPECIFIED.,.F.,.F.,.F.,
(4,1,4),(4,4),(0.,0.571428571428571,1.),(1.66533453693773E-16,1.2),
 .UNSPECIFIED.);
#1389=B_SPLINE_SURFACE_WITH_KNOTS('',3,3,((#77615,#77616,#77617,#77618),
(#77619,#77620,#77621,#77622),(#77623,#77624,#77625,#77626),(#77627,#77628,
#77629,#77630),(#77631,#77632,#77633,#77634)),.UNSPECIFIED.,.F.,.F.,.F.,
(4,1,4),(4,4),(0.,0.571428571428571,1.),(-1.47525527564366E-17,1.2),
 .UNSPECIFIED.);
#1390=B_SPLINE_SURFACE_WITH_KNOTS('',3,3,((#77664,#77665,#77666,#77667),
(#77668,#77669,#77670,#77671),(#77672,#77673,#77674,#77675),(#77676,#77677,
#77678,#77679),(#77680,#77681,#77682,#77683)),.UNSPECIFIED.,.F.,.F.,.F.,
(4,1,4),(4,4),(0.,0.571428571428571,1.),(-8.32667268468867E-17,1.2),
 .UNSPECIFIED.);
#1391=B_SPLINE_SURFACE_WITH_KNOTS('',3,3,((#78511,#78512,#78513,#78514),
(#78515,#78516,#78517,#78518),(#78519,#78520,#78521,#78522),(#78523,#78524,
#78525,#78526),(#78527,#78528,#78529,#78530)),.UNSPECIFIED.,.F.,.F.,.F.,
(4,1,4),(4,4),(0.,0.571428571428571,1.),(2.77555756156289E-17,1.2),
 .UNSPECIFIED.);
#1392=B_SPLINE_SURFACE_WITH_KNOTS('',3,3,((#78560,#78561,#78562,#78563),
(#78564,#78565,#78566,#78567),(#78568,#78569,#78570,#78571),(#78572,#78573,
#78574,#78575),(#78576,#78577,#78578,#78579)),.UNSPECIFIED.,.F.,.F.,.F.,
(4,1,4),(4,4),(0.,0.571428571428571,1.),(9.44002594796574E-17,1.2),
 .UNSPECIFIED.);
#1393=B_SPLINE_SURFACE_WITH_KNOTS('',3,3,((#79407,#79408,#79409,#79410),
(#79411,#79412,#79413,#79414),(#79415,#79416,#79417,#79418),(#79419,#79420,
#79421,#79422),(#79423,#79424,#79425,#79426)),.UNSPECIFIED.,.F.,.F.,.F.,
(4,1,4),(4,4),(0.,0.571428571428571,1.),(0.,1.2),.UNSPECIFIED.);
#1394=B_SPLINE_SURFACE_WITH_KNOTS('',3,3,((#79456,#79457,#79458,#79459),
(#79460,#79461,#79462,#79463),(#79464,#79465,#79466,#79467),(#79468,#79469,
#79470,#79471),(#79472,#79473,#79474,#79475)),.UNSPECIFIED.,.F.,.F.,.F.,
(4,1,4),(4,4),(0.,0.571428571428571,1.),(1.66533453693773E-16,1.2),
 .UNSPECIFIED.);
#1395=B_SPLINE_SURFACE_WITH_KNOTS('',3,3,((#80303,#80304,#80305,#80306),
(#80307,#80308,#80309,#80310),(#80311,#80312,#80313,#80314),(#80315,#80316,
#80317,#80318),(#80319,#80320,#80321,#80322)),.UNSPECIFIED.,.F.,.F.,.F.,
(4,1,4),(4,4),(0.,0.571428571428571,1.),(-1.8224407144634E-16,1.2),
 .UNSPECIFIED.);
#1396=B_SPLINE_SURFACE_WITH_KNOTS('',3,3,((#80352,#80353,#80354,#80355),
(#80356,#80357,#80358,#80359),(#80360,#80361,#80362,#80363),(#80364,#80365,
#80366,#80367),(#80368,#80369,#80370,#80371)),.UNSPECIFIED.,.F.,.F.,.F.,
(4,1,4),(4,4),(0.,0.571428571428571,1.),(-1.8809784878858E-36,1.2),
 .UNSPECIFIED.);
#1397=B_SPLINE_SURFACE_WITH_KNOTS('',3,3,((#81199,#81200,#81201,#81202),
(#81203,#81204,#81205,#81206),(#81207,#81208,#81209,#81210),(#81211,#81212,
#81213,#81214),(#81215,#81216,#81217,#81218)),.UNSPECIFIED.,.F.,.F.,.F.,
(4,1,4),(4,4),(0.,0.571428571428571,1.),(-5.55111512312578E-17,1.2),
 .UNSPECIFIED.);
#1398=B_SPLINE_SURFACE_WITH_KNOTS('',3,3,((#81248,#81249,#81250,#81251),
(#81252,#81253,#81254,#81255),(#81256,#81257,#81258,#81259),(#81260,#81261,
#81262,#81263),(#81264,#81265,#81266,#81267)),.UNSPECIFIED.,.F.,.F.,.F.,
(4,1,4),(4,4),(0.,0.571428571428571,1.),(9.71445146547012E-17,1.2),
 .UNSPECIFIED.);
#1399=B_SPLINE_SURFACE_WITH_KNOTS('',3,3,((#82095,#82096,#82097,#82098),
(#82099,#82100,#82101,#82102),(#82103,#82104,#82105,#82106),(#82107,#82108,
#82109,#82110),(#82111,#82112,#82113,#82114)),.UNSPECIFIED.,.F.,.F.,.F.,
(4,1,4),(4,4),(0.,0.571428571428571,1.),(-8.32667268468867E-17,1.2),
 .UNSPECIFIED.);
#1400=B_SPLINE_SURFACE_WITH_KNOTS('',3,3,((#82144,#82145,#82146,#82147),
(#82148,#82149,#82150,#82151),(#82152,#82153,#82154,#82155),(#82156,#82157,
#82158,#82159),(#82160,#82161,#82162,#82163)),.UNSPECIFIED.,.F.,.F.,.F.,
(4,1,4),(4,4),(0.,0.571428571428571,1.),(0.,1.2),.UNSPECIFIED.);
#1401=B_SPLINE_SURFACE_WITH_KNOTS('',3,3,((#82991,#82992,#82993,#82994),
(#82995,#82996,#82997,#82998),(#82999,#83000,#83001,#83002),(#83003,#83004,
#83005,#83006),(#83007,#83008,#83009,#83010)),.UNSPECIFIED.,.F.,.F.,.F.,
(4,1,4),(4,4),(0.,0.571428571428571,1.),(0.,1.2),.UNSPECIFIED.);
#1402=B_SPLINE_SURFACE_WITH_KNOTS('',3,3,((#83040,#83041,#83042,#83043),
(#83044,#83045,#83046,#83047),(#83048,#83049,#83050,#83051),(#83052,#83053,
#83054,#83055),(#83056,#83057,#83058,#83059)),.UNSPECIFIED.,.F.,.F.,.F.,
(4,1,4),(4,4),(0.,0.571428571428571,1.),(9.71445146547012E-17,1.2),
 .UNSPECIFIED.);
#1403=B_SPLINE_SURFACE_WITH_KNOTS('',3,3,((#83887,#83888,#83889,#83890),
(#83891,#83892,#83893,#83894),(#83895,#83896,#83897,#83898),(#83899,#83900,
#83901,#83902),(#83903,#83904,#83905,#83906)),.UNSPECIFIED.,.F.,.F.,.F.,
(4,1,4),(4,4),(0.,0.571428571428571,1.),(-2.77555756156289E-17,1.2),
 .UNSPECIFIED.);
#1404=B_SPLINE_SURFACE_WITH_KNOTS('',3,3,((#83936,#83937,#83938,#83939),
(#83940,#83941,#83942,#83943),(#83944,#83945,#83946,#83947),(#83948,#83949,
#83950,#83951),(#83952,#83953,#83954,#83955)),.UNSPECIFIED.,.F.,.F.,.F.,
(4,1,4),(4,4),(0.,0.571428571428571,1.),(9.71445146547012E-17,1.2),
 .UNSPECIFIED.);
#1405=B_SPLINE_SURFACE_WITH_KNOTS('',3,3,((#84783,#84784,#84785,#84786),
(#84787,#84788,#84789,#84790),(#84791,#84792,#84793,#84794),(#84795,#84796,
#84797,#84798),(#84799,#84800,#84801,#84802)),.UNSPECIFIED.,.F.,.F.,.F.,
(4,1,4),(4,4),(0.,0.571428571428571,1.),(-9.71445146547012E-17,1.2),
 .UNSPECIFIED.);
#1406=B_SPLINE_SURFACE_WITH_KNOTS('',3,3,((#84832,#84833,#84834,#84835),
(#84836,#84837,#84838,#84839),(#84840,#84841,#84842,#84843),(#84844,#84845,
#84846,#84847),(#84848,#84849,#84850,#84851)),.UNSPECIFIED.,.F.,.F.,.F.,
(4,1,4),(4,4),(0.,0.571428571428571,1.),(3.88891082483996E-17,1.2),
 .UNSPECIFIED.);
#1407=B_SPLINE_SURFACE_WITH_KNOTS('',3,3,((#85679,#85680,#85681,#85682),
(#85683,#85684,#85685,#85686),(#85687,#85688,#85689,#85690),(#85691,#85692,
#85693,#85694),(#85695,#85696,#85697,#85698)),.UNSPECIFIED.,.F.,.F.,.F.,
(4,1,4),(4,4),(0.,0.571428571428571,1.),(-1.11022302462516E-16,1.2),
 .UNSPECIFIED.);
#1408=B_SPLINE_SURFACE_WITH_KNOTS('',3,3,((#85728,#85729,#85730,#85731),
(#85732,#85733,#85734,#85735),(#85736,#85737,#85738,#85739),(#85740,#85741,
#85742,#85743),(#85744,#85745,#85746,#85747)),.UNSPECIFIED.,.F.,.F.,.F.,
(4,1,4),(4,4),(0.,0.571428571428571,1.),(3.88891082483996E-17,1.2),
 .UNSPECIFIED.);
#1409=B_SPLINE_SURFACE_WITH_KNOTS('',3,3,((#86575,#86576,#86577,#86578),
(#86579,#86580,#86581,#86582),(#86583,#86584,#86585,#86586),(#86587,#86588,
#86589,#86590),(#86591,#86592,#86593,#86594)),.UNSPECIFIED.,.F.,.F.,.F.,
(4,1,4),(4,4),(0.,0.571428571428571,1.),(-1.8809784878848E-36,1.2),
 .UNSPECIFIED.);
#1410=B_SPLINE_SURFACE_WITH_KNOTS('',3,3,((#86624,#86625,#86626,#86627),
(#86628,#86629,#86630,#86631),(#86632,#86633,#86634,#86635),(#86636,#86637,
#86638,#86639),(#86640,#86641,#86642,#86643)),.UNSPECIFIED.,.F.,.F.,.F.,
(4,1,4),(4,4),(0.,0.571428571428571,1.),(-1.11022302462516E-16,1.2),
 .UNSPECIFIED.);
#1411=B_SPLINE_SURFACE_WITH_KNOTS('',3,3,((#87471,#87472,#87473,#87474),
(#87475,#87476,#87477,#87478),(#87479,#87480,#87481,#87482),(#87483,#87484,
#87485,#87486),(#87487,#87488,#87489,#87490)),.UNSPECIFIED.,.F.,.F.,.F.,
(4,1,4),(4,4),(0.,0.571428571428571,1.),(-8.32667268468867E-17,1.2),
 .UNSPECIFIED.);
#1412=B_SPLINE_SURFACE_WITH_KNOTS('',3,3,((#87520,#87521,#87522,#87523),
(#87524,#87525,#87526,#87527),(#87528,#87529,#87530,#87531),(#87532,#87533,
#87534,#87535),(#87536,#87537,#87538,#87539)),.UNSPECIFIED.,.F.,.F.,.F.,
(4,1,4),(4,4),(0.,0.571428571428571,1.),(9.71445146547012E-17,1.2),
 .UNSPECIFIED.);
#1413=B_SPLINE_SURFACE_WITH_KNOTS('',3,3,((#88367,#88368,#88369,#88370),
(#88371,#88372,#88373,#88374),(#88375,#88376,#88377,#88378),(#88379,#88380,
#88381,#88382),(#88383,#88384,#88385,#88386)),.UNSPECIFIED.,.F.,.F.,.F.,
(4,1,4),(4,4),(0.,0.571428571428571,1.),(2.77555756156289E-17,1.2),
 .UNSPECIFIED.);
#1414=B_SPLINE_SURFACE_WITH_KNOTS('',3,3,((#88416,#88417,#88418,#88419),
(#88420,#88421,#88422,#88423),(#88424,#88425,#88426,#88427),(#88428,#88429,
#88430,#88431),(#88432,#88433,#88434,#88435)),.UNSPECIFIED.,.F.,.F.,.F.,
(4,1,4),(4,4),(0.,0.571428571428571,1.),(-1.38777878078145E-16,1.2),
 .UNSPECIFIED.);
#1415=B_SPLINE_SURFACE_WITH_KNOTS('',3,3,((#89263,#89264,#89265,#89266),
(#89267,#89268,#89269,#89270),(#89271,#89272,#89273,#89274),(#89275,#89276,
#89277,#89278),(#89279,#89280,#89281,#89282)),.UNSPECIFIED.,.F.,.F.,.F.,
(4,1,4),(4,4),(0.,0.571428571428571,1.),(2.77555756156289E-17,1.2),
 .UNSPECIFIED.);
#1416=B_SPLINE_SURFACE_WITH_KNOTS('',3,3,((#89312,#89313,#89314,#89315),
(#89316,#89317,#89318,#89319),(#89320,#89321,#89322,#89323),(#89324,#89325,
#89326,#89327),(#89328,#89329,#89330,#89331)),.UNSPECIFIED.,.F.,.F.,.F.,
(4,1,4),(4,4),(0.,0.571428571428571,1.),(9.71445146547012E-17,1.2),
 .UNSPECIFIED.);
#1417=B_SPLINE_SURFACE_WITH_KNOTS('',3,3,((#90159,#90160,#90161,#90162),
(#90163,#90164,#90165,#90166),(#90167,#90168,#90169,#90170),(#90171,#90172,
#90173,#90174),(#90175,#90176,#90177,#90178)),.UNSPECIFIED.,.F.,.F.,.F.,
(4,1,4),(4,4),(0.,0.571428571428571,1.),(-7.5239139515392E-36,1.2),
 .UNSPECIFIED.);
#1418=B_SPLINE_SURFACE_WITH_KNOTS('',3,3,((#90208,#90209,#90210,#90211),
(#90212,#90213,#90214,#90215),(#90216,#90217,#90218,#90219),(#90220,#90221,
#90222,#90223),(#90224,#90225,#90226,#90227)),.UNSPECIFIED.,.F.,.F.,.F.,
(4,1,4),(4,4),(0.,0.571428571428571,1.),(8.05224716718429E-17,1.2),
 .UNSPECIFIED.);
#1419=B_SPLINE_SURFACE_WITH_KNOTS('',3,3,((#91055,#91056,#91057,#91058),
(#91059,#91060,#91061,#91062),(#91063,#91064,#91065,#91066),(#91067,#91068,
#91069,#91070),(#91071,#91072,#91073,#91074)),.UNSPECIFIED.,.F.,.F.,.F.,
(4,1,4),(4,4),(0.,0.571428571428571,1.),(0.,1.2),.UNSPECIFIED.);
#1420=B_SPLINE_SURFACE_WITH_KNOTS('',3,3,((#91104,#91105,#91106,#91107),
(#91108,#91109,#91110,#91111),(#91112,#91113,#91114,#91115),(#91116,#91117,
#91118,#91119),(#91120,#91121,#91122,#91123)),.UNSPECIFIED.,.F.,.F.,.F.,
(4,1,4),(4,4),(0.,0.571428571428571,1.),(9.71445146547012E-17,1.2),
 .UNSPECIFIED.);
#1421=B_SPLINE_SURFACE_WITH_KNOTS('',3,3,((#91951,#91952,#91953,#91954),
(#91955,#91956,#91957,#91958),(#91959,#91960,#91961,#91962),(#91963,#91964,
#91965,#91966),(#91967,#91968,#91969,#91970)),.UNSPECIFIED.,.F.,.F.,.F.,
(4,1,4),(4,4),(0.,0.571428571428571,1.),(-1.49437708898837E-16,1.2),
 .UNSPECIFIED.);
#1422=B_SPLINE_SURFACE_WITH_KNOTS('',3,3,((#92000,#92001,#92002,#92003),
(#92004,#92005,#92006,#92007),(#92008,#92009,#92010,#92011),(#92012,#92013,
#92014,#92015),(#92016,#92017,#92018,#92019)),.UNSPECIFIED.,.F.,.F.,.F.,
(4,1,4),(4,4),(0.,0.571428571428571,1.),(5.55111512312578E-17,1.2),
 .UNSPECIFIED.);
#1423=B_SPLINE_SURFACE_WITH_KNOTS('',3,3,((#92847,#92848,#92849,#92850),
(#92851,#92852,#92853,#92854),(#92855,#92856,#92857,#92858),(#92859,#92860,
#92861,#92862),(#92863,#92864,#92865,#92866)),.UNSPECIFIED.,.F.,.F.,.F.,
(4,1,4),(4,4),(0.,0.571428571428571,1.),(-8.32667268468867E-17,1.2),
 .UNSPECIFIED.);
#1424=B_SPLINE_SURFACE_WITH_KNOTS('',3,3,((#92896,#92897,#92898,#92899),
(#92900,#92901,#92902,#92903),(#92904,#92905,#92906,#92907),(#92908,#92909,
#92910,#92911),(#92912,#92913,#92914,#92915)),.UNSPECIFIED.,.F.,.F.,.F.,
(4,1,4),(4,4),(0.,0.571428571428571,1.),(9.71445146547012E-17,1.2),
 .UNSPECIFIED.);
#1425=B_SPLINE_SURFACE_WITH_KNOTS('',3,3,((#93743,#93744,#93745,#93746),
(#93747,#93748,#93749,#93750),(#93751,#93752,#93753,#93754),(#93755,#93756,
#93757,#93758),(#93759,#93760,#93761,#93762)),.UNSPECIFIED.,.F.,.F.,.F.,
(4,1,4),(4,4),(0.,0.571428571428571,1.),(-8.32667268468868E-17,1.2),
 .UNSPECIFIED.);
#1426=B_SPLINE_SURFACE_WITH_KNOTS('',3,3,((#93792,#93793,#93794,#93795),
(#93796,#93797,#93798,#93799),(#93800,#93801,#93802,#93803),(#93804,#93805,
#93806,#93807),(#93808,#93809,#93810,#93811)),.UNSPECIFIED.,.F.,.F.,.F.,
(4,1,4),(4,4),(0.,0.571428571428571,1.),(-8.32667268468867E-17,1.2),
 .UNSPECIFIED.);
#1427=B_SPLINE_SURFACE_WITH_KNOTS('',3,3,((#94639,#94640,#94641,#94642),
(#94643,#94644,#94645,#94646),(#94647,#94648,#94649,#94650),(#94651,#94652,
#94653,#94654),(#94655,#94656,#94657,#94658)),.UNSPECIFIED.,.F.,.F.,.F.,
(4,1,4),(4,4),(0.,0.571428571428571,1.),(2.77555756156289E-17,1.2),
 .UNSPECIFIED.);
#1428=B_SPLINE_SURFACE_WITH_KNOTS('',3,3,((#94688,#94689,#94690,#94691),
(#94692,#94693,#94694,#94695),(#94696,#94697,#94698,#94699),(#94700,#94701,
#94702,#94703),(#94704,#94705,#94706,#94707)),.UNSPECIFIED.,.F.,.F.,.F.,
(4,1,4),(4,4),(0.,0.571428571428571,1.),(8.32667268468867E-17,1.2),
 .UNSPECIFIED.);
#1429=B_SPLINE_SURFACE_WITH_KNOTS('',3,3,((#95535,#95536,#95537,#95538),
(#95539,#95540,#95541,#95542),(#95543,#95544,#95545,#95546),(#95547,#95548,
#95549,#95550),(#95551,#95552,#95553,#95554)),.UNSPECIFIED.,.F.,.F.,.F.,
(4,1,4),(4,4),(0.,0.571428571428571,1.),(2.77555756156289E-17,1.2),
 .UNSPECIFIED.);
#1430=B_SPLINE_SURFACE_WITH_KNOTS('',3,3,((#95584,#95585,#95586,#95587),
(#95588,#95589,#95590,#95591),(#95592,#95593,#95594,#95595),(#95596,#95597,
#95598,#95599),(#95600,#95601,#95602,#95603)),.UNSPECIFIED.,.F.,.F.,.F.,
(4,1,4),(4,4),(0.,0.571428571428571,1.),(5.55111512312578E-17,1.2),
 .UNSPECIFIED.);
#1431=B_SPLINE_SURFACE_WITH_KNOTS('',3,3,((#96431,#96432,#96433,#96434),
(#96435,#96436,#96437,#96438),(#96439,#96440,#96441,#96442),(#96443,#96444,
#96445,#96446),(#96447,#96448,#96449,#96450)),.UNSPECIFIED.,.F.,.F.,.F.,
(4,1,4),(4,4),(0.,0.571428571428571,1.),(-1.38777878078145E-16,1.2),
 .UNSPECIFIED.);
#1432=B_SPLINE_SURFACE_WITH_KNOTS('',3,3,((#96480,#96481,#96482,#96483),
(#96484,#96485,#96486,#96487),(#96488,#96489,#96490,#96491),(#96492,#96493,
#96494,#96495),(#96496,#96497,#96498,#96499)),.UNSPECIFIED.,.F.,.F.,.F.,
(4,1,4),(4,4),(0.,0.571428571428571,1.),(2.77555756156289E-17,1.2),
 .UNSPECIFIED.);
#1433=B_SPLINE_SURFACE_WITH_KNOTS('',3,3,((#97327,#97328,#97329,#97330),
(#97331,#97332,#97333,#97334),(#97335,#97336,#97337,#97338),(#97339,#97340,
#97341,#97342),(#97343,#97344,#97345,#97346)),.UNSPECIFIED.,.F.,.F.,.F.,
(4,1,4),(4,4),(0.,0.571428571428571,1.),(0.,1.2),.UNSPECIFIED.);
#1434=B_SPLINE_SURFACE_WITH_KNOTS('',3,3,((#97376,#97377,#97378,#97379),
(#97380,#97381,#97382,#97383),(#97384,#97385,#97386,#97387),(#97388,#97389,
#97390,#97391),(#97392,#97393,#97394,#97395)),.UNSPECIFIED.,.F.,.F.,.F.,
(4,1,4),(4,4),(0.,0.571428571428571,1.),(1.66533453693773E-16,1.2),
 .UNSPECIFIED.);
#1435=B_SPLINE_SURFACE_WITH_KNOTS('',3,3,((#98223,#98224,#98225,#98226),
(#98227,#98228,#98229,#98230),(#98231,#98232,#98233,#98234),(#98235,#98236,
#98237,#98238),(#98239,#98240,#98241,#98242)),.UNSPECIFIED.,.F.,.F.,.F.,
(4,1,4),(4,4),(0.,0.571428571428571,1.),(-8.32667268468867E-17,1.2),
 .UNSPECIFIED.);
#1436=B_SPLINE_SURFACE_WITH_KNOTS('',3,3,((#98272,#98273,#98274,#98275),
(#98276,#98277,#98278,#98279),(#98280,#98281,#98282,#98283),(#98284,#98285,
#98286,#98287),(#98288,#98289,#98290,#98291)),.UNSPECIFIED.,.F.,.F.,.F.,
(4,1,4),(4,4),(0.,0.571428571428571,1.),(9.71445146547012E-17,1.2),
 .UNSPECIFIED.);
#1437=B_SPLINE_SURFACE_WITH_KNOTS('',3,3,((#99119,#99120,#99121,#99122),
(#99123,#99124,#99125,#99126),(#99127,#99128,#99129,#99130),(#99131,#99132,
#99133,#99134),(#99135,#99136,#99137,#99138)),.UNSPECIFIED.,.F.,.F.,.F.,
(4,1,4),(4,4),(0.,0.571428571428571,1.),(-2.03133674691991E-35,1.2),
 .UNSPECIFIED.);
#1438=B_SPLINE_SURFACE_WITH_KNOTS('',3,3,((#99168,#99169,#99170,#99171),
(#99172,#99173,#99174,#99175),(#99176,#99177,#99178,#99179),(#99180,#99181,
#99182,#99183),(#99184,#99185,#99186,#99187)),.UNSPECIFIED.,.F.,.F.,.F.,
(4,1,4),(4,4),(0.,0.571428571428571,1.),(-1.83155496676632E-16,1.2),
 .UNSPECIFIED.);
#1439=B_SPLINE_SURFACE_WITH_KNOTS('',3,3,((#100015,#100016,#100017,#100018),
(#100019,#100020,#100021,#100022),(#100023,#100024,#100025,#100026),(#100027,
#100028,#100029,#100030),(#100031,#100032,#100033,#100034)),
 .UNSPECIFIED.,.F.,.F.,.F.,(4,1,4),(4,4),(0.,0.571428571428571,1.),(-1.38777878078145E-16,
1.2),.UNSPECIFIED.);
#1440=B_SPLINE_SURFACE_WITH_KNOTS('',3,3,((#100064,#100065,#100066,#100067),
(#100068,#100069,#100070,#100071),(#100072,#100073,#100074,#100075),(#100076,
#100077,#100078,#100079),(#100080,#100081,#100082,#100083)),
 .UNSPECIFIED.,.F.,.F.,.F.,(4,1,4),(4,4),(0.,0.571428571428571,1.),(1.66533453693773E-16,
1.2),.UNSPECIFIED.);
#1441=B_SPLINE_SURFACE_WITH_KNOTS('',3,3,((#100911,#100912,#100913,#100914),
(#100915,#100916,#100917,#100918),(#100919,#100920,#100921,#100922),(#100923,
#100924,#100925,#100926),(#100927,#100928,#100929,#100930)),
 .UNSPECIFIED.,.F.,.F.,.F.,(4,1,4),(4,4),(0.,0.571428571428571,1.),(0.,
1.2),.UNSPECIFIED.);
#1442=B_SPLINE_SURFACE_WITH_KNOTS('',3,3,((#100960,#100961,#100962,#100963),
(#100964,#100965,#100966,#100967),(#100968,#100969,#100970,#100971),(#100972,
#100973,#100974,#100975),(#100976,#100977,#100978,#100979)),
 .UNSPECIFIED.,.F.,.F.,.F.,(4,1,4),(4,4),(0.,0.571428571428571,1.),(-1.38777878078145E-16,
1.2),.UNSPECIFIED.);
#1443=B_SPLINE_SURFACE_WITH_KNOTS('',3,3,((#101807,#101808,#101809,#101810),
(#101811,#101812,#101813,#101814),(#101815,#101816,#101817,#101818),(#101819,
#101820,#101821,#101822),(#101823,#101824,#101825,#101826)),
 .UNSPECIFIED.,.F.,.F.,.F.,(4,1,4),(4,4),(0.,0.571428571428571,1.),(-1.88097848788491E-36,
1.2),.UNSPECIFIED.);
#1444=B_SPLINE_SURFACE_WITH_KNOTS('',3,3,((#101856,#101857,#101858,#101859),
(#101860,#101861,#101862,#101863),(#101864,#101865,#101866,#101867),(#101868,
#101869,#101870,#101871),(#101872,#101873,#101874,#101875)),
 .UNSPECIFIED.,.F.,.F.,.F.,(4,1,4),(4,4),(0.,0.571428571428571,1.),(2.77555756156289E-17,
1.2),.UNSPECIFIED.);
#1445=B_SPLINE_SURFACE_WITH_KNOTS('',3,3,((#102703,#102704,#102705,#102706),
(#102707,#102708,#102709,#102710),(#102711,#102712,#102713,#102714),(#102715,
#102716,#102717,#102718),(#102719,#102720,#102721,#102722)),
 .UNSPECIFIED.,.F.,.F.,.F.,(4,1,4),(4,4),(0.,0.571428571428571,1.),(-1.38777878078145E-16,
1.2),.UNSPECIFIED.);
#1446=B_SPLINE_SURFACE_WITH_KNOTS('',3,3,((#102752,#102753,#102754,#102755),
(#102756,#102757,#102758,#102759),(#102760,#102761,#102762,#102763),(#102764,
#102765,#102766,#102767),(#102768,#102769,#102770,#102771)),
 .UNSPECIFIED.,.F.,.F.,.F.,(4,1,4),(4,4),(0.,0.571428571428571,1.),(0.,
1.2),.UNSPECIFIED.);
#1447=B_SPLINE_SURFACE_WITH_KNOTS('',3,3,((#103599,#103600,#103601,#103602),
(#103603,#103604,#103605,#103606),(#103607,#103608,#103609,#103610),(#103611,
#103612,#103613,#103614),(#103615,#103616,#103617,#103618)),
 .UNSPECIFIED.,.F.,.F.,.F.,(4,1,4),(4,4),(0.,0.571428571428571,1.),(0.,
1.2),.UNSPECIFIED.);
#1448=B_SPLINE_SURFACE_WITH_KNOTS('',3,3,((#103648,#103649,#103650,#103651),
(#103652,#103653,#103654,#103655),(#103656,#103657,#103658,#103659),(#103660,
#103661,#103662,#103663),(#103664,#103665,#103666,#103667)),
 .UNSPECIFIED.,.F.,.F.,.F.,(4,1,4),(4,4),(0.,0.571428571428571,1.),(9.71445146547012E-17,
1.2),.UNSPECIFIED.);
#1449=B_SPLINE_SURFACE_WITH_KNOTS('',3,3,((#104495,#104496,#104497,#104498),
(#104499,#104500,#104501,#104502),(#104503,#104504,#104505,#104506),(#104507,
#104508,#104509,#104510),(#104511,#104512,#104513,#104514)),
 .UNSPECIFIED.,.F.,.F.,.F.,(4,1,4),(4,4),(0.,0.571428571428571,1.),(-5.55111512312578E-17,
1.2),.UNSPECIFIED.);
#1450=B_SPLINE_SURFACE_WITH_KNOTS('',3,3,((#104544,#104545,#104546,#104547),
(#104548,#104549,#104550,#104551),(#104552,#104553,#104554,#104555),(#104556,
#104557,#104558,#104559),(#104560,#104561,#104562,#104563)),
 .UNSPECIFIED.,.F.,.F.,.F.,(4,1,4),(4,4),(0.,0.571428571428571,1.),(9.71445146547012E-17,
1.2),.UNSPECIFIED.);
#1451=B_SPLINE_SURFACE_WITH_KNOTS('',3,3,((#105391,#105392,#105393,#105394),
(#105395,#105396,#105397,#105398),(#105399,#105400,#105401,#105402),(#105403,
#105404,#105405,#105406),(#105407,#105408,#105409,#105410)),
 .UNSPECIFIED.,.F.,.F.,.F.,(4,1,4),(4,4),(0.,0.571428571428571,1.),(-1.41402172924014E-16,
1.2),.UNSPECIFIED.);
#1452=B_SPLINE_SURFACE_WITH_KNOTS('',3,3,((#105440,#105441,#105442,#105443),
(#105444,#105445,#105446,#105447),(#105448,#105449,#105450,#105451),(#105452,
#105453,#105454,#105455),(#105456,#105457,#105458,#105459)),
 .UNSPECIFIED.,.F.,.F.,.F.,(4,1,4),(4,4),(0.,0.571428571428571,1.),(0.,
1.2),.UNSPECIFIED.);
#1453=B_SPLINE_SURFACE_WITH_KNOTS('',3,3,((#106287,#106288,#106289,#106290),
(#106291,#106292,#106293,#106294),(#106295,#106296,#106297,#106298),(#106299,
#106300,#106301,#106302),(#106303,#106304,#106305,#106306)),
 .UNSPECIFIED.,.F.,.F.,.F.,(4,1,4),(4,4),(0.,0.571428571428571,1.),(-1.11022302462516E-16,
1.2),.UNSPECIFIED.);
#1454=B_SPLINE_SURFACE_WITH_KNOTS('',3,3,((#106336,#106337,#106338,#106339),
(#106340,#106341,#106342,#106343),(#106344,#106345,#106346,#106347),(#106348,
#106349,#106350,#106351),(#106352,#106353,#106354,#106355)),
 .UNSPECIFIED.,.F.,.F.,.F.,(4,1,4),(4,4),(0.,0.571428571428571,1.),(1.38777878078145E-16,
1.2),.UNSPECIFIED.);
#1455=B_SPLINE_SURFACE_WITH_KNOTS('',3,3,((#107183,#107184,#107185,#107186),
(#107187,#107188,#107189,#107190),(#107191,#107192,#107193,#107194),(#107195,
#107196,#107197,#107198),(#107199,#107200,#107201,#107202)),
 .UNSPECIFIED.,.F.,.F.,.F.,(4,1,4),(4,4),(0.,0.571428571428571,1.),(2.77555756156289E-17,
1.2),.UNSPECIFIED.);
#1456=B_SPLINE_SURFACE_WITH_KNOTS('',3,3,((#107232,#107233,#107234,#107235),
(#107236,#107237,#107238,#107239),(#107240,#107241,#107242,#107243),(#107244,
#107245,#107246,#107247),(#107248,#107249,#107250,#107251)),
 .UNSPECIFIED.,.F.,.F.,.F.,(4,1,4),(4,4),(0.,0.571428571428571,1.),(0.,
1.2),.UNSPECIFIED.);
#1457=B_SPLINE_SURFACE_WITH_KNOTS('',3,3,((#108079,#108080,#108081,#108082),
(#108083,#108084,#108085,#108086),(#108087,#108088,#108089,#108090),(#108091,
#108092,#108093,#108094),(#108095,#108096,#108097,#108098)),
 .UNSPECIFIED.,.F.,.F.,.F.,(4,1,4),(4,4),(0.,0.571428571428571,1.),(2.77555756156289E-17,
1.2),.UNSPECIFIED.);
#1458=B_SPLINE_SURFACE_WITH_KNOTS('',3,3,((#108128,#108129,#108130,#108131),
(#108132,#108133,#108134,#108135),(#108136,#108137,#108138,#108139),(#108140,
#108141,#108142,#108143),(#108144,#108145,#108146,#108147)),
 .UNSPECIFIED.,.F.,.F.,.F.,(4,1,4),(4,4),(0.,0.571428571428571,1.),(5.55111512312578E-17,
1.2),.UNSPECIFIED.);
#1459=B_SPLINE_SURFACE_WITH_KNOTS('',3,3,((#108975,#108976,#108977,#108978),
(#108979,#108980,#108981,#108982),(#108983,#108984,#108985,#108986),(#108987,
#108988,#108989,#108990),(#108991,#108992,#108993,#108994)),
 .UNSPECIFIED.,.F.,.F.,.F.,(4,1,4),(4,4),(0.,0.571428571428571,1.),(-8.32667268468867E-17,
1.2),.UNSPECIFIED.);
#1460=B_SPLINE_SURFACE_WITH_KNOTS('',3,3,((#109024,#109025,#109026,#109027),
(#109028,#109029,#109030,#109031),(#109032,#109033,#109034,#109035),(#109036,
#109037,#109038,#109039),(#109040,#109041,#109042,#109043)),
 .UNSPECIFIED.,.F.,.F.,.F.,(4,1,4),(4,4),(0.,0.571428571428571,1.),(1.66533453693773E-16,
1.2),.UNSPECIFIED.);
#1461=B_SPLINE_SURFACE_WITH_KNOTS('',3,3,((#109871,#109872,#109873,#109874),
(#109875,#109876,#109877,#109878),(#109879,#109880,#109881,#109882),(#109883,
#109884,#109885,#109886),(#109887,#109888,#109889,#109890)),
 .UNSPECIFIED.,.F.,.F.,.F.,(4,1,4),(4,4),(0.,0.571428571428571,1.),(-1.47525527564366E-17,
1.2),.UNSPECIFIED.);
#1462=B_SPLINE_SURFACE_WITH_KNOTS('',3,3,((#109920,#109921,#109922,#109923),
(#109924,#109925,#109926,#109927),(#109928,#109929,#109930,#109931),(#109932,
#109933,#109934,#109935),(#109936,#109937,#109938,#109939)),
 .UNSPECIFIED.,.F.,.F.,.F.,(4,1,4),(4,4),(0.,0.571428571428571,1.),(9.71445146547012E-17,
1.2),.UNSPECIFIED.);
#1463=B_SPLINE_SURFACE_WITH_KNOTS('',3,3,((#110767,#110768,#110769,#110770),
(#110771,#110772,#110773,#110774),(#110775,#110776,#110777,#110778),(#110779,
#110780,#110781,#110782),(#110783,#110784,#110785,#110786)),
 .UNSPECIFIED.,.F.,.F.,.F.,(4,1,4),(4,4),(0.,0.571428571428571,1.),(2.77555756156289E-17,
1.2),.UNSPECIFIED.);
#1464=B_SPLINE_SURFACE_WITH_KNOTS('',3,3,((#110816,#110817,#110818,#110819),
(#110820,#110821,#110822,#110823),(#110824,#110825,#110826,#110827),(#110828,
#110829,#110830,#110831),(#110832,#110833,#110834,#110835)),
 .UNSPECIFIED.,.F.,.F.,.F.,(4,1,4),(4,4),(0.,0.571428571428571,1.),(0.,
1.2),.UNSPECIFIED.);
#1465=B_SPLINE_SURFACE_WITH_KNOTS('',3,3,((#111663,#111664,#111665,#111666),
(#111667,#111668,#111669,#111670),(#111671,#111672,#111673,#111674),(#111675,
#111676,#111677,#111678),(#111679,#111680,#111681,#111682)),
 .UNSPECIFIED.,.F.,.F.,.F.,(4,1,4),(4,4),(0.,0.571428571428571,1.),(-8.32667268468867E-17,
1.2),.UNSPECIFIED.);
#1466=B_SPLINE_SURFACE_WITH_KNOTS('',3,3,((#111712,#111713,#111714,#111715),
(#111716,#111717,#111718,#111719),(#111720,#111721,#111722,#111723),(#111724,
#111725,#111726,#111727),(#111728,#111729,#111730,#111731)),
 .UNSPECIFIED.,.F.,.F.,.F.,(4,1,4),(4,4),(0.,0.571428571428571,1.),(-5.63859161805989E-17,
1.2),.UNSPECIFIED.);
#1467=B_SPLINE_SURFACE_WITH_KNOTS('',3,3,((#112559,#112560,#112561,#112562),
(#112563,#112564,#112565,#112566),(#112567,#112568,#112569,#112570),(#112571,
#112572,#112573,#112574),(#112575,#112576,#112577,#112578)),
 .UNSPECIFIED.,.F.,.F.,.F.,(4,1,4),(4,4),(0.,0.571428571428571,1.),(-3.76195697576961E-36,
1.2),.UNSPECIFIED.);
#1468=B_SPLINE_SURFACE_WITH_KNOTS('',3,3,((#112608,#112609,#112610,#112611),
(#112612,#112613,#112614,#112615),(#112616,#112617,#112618,#112619),(#112620,
#112621,#112622,#112623),(#112624,#112625,#112626,#112627)),
 .UNSPECIFIED.,.F.,.F.,.F.,(4,1,4),(4,4),(0.,0.571428571428571,1.),(2.77555756156289E-17,
1.2),.UNSPECIFIED.);
#1469=B_SPLINE_SURFACE_WITH_KNOTS('',3,3,((#113455,#113456,#113457,#113458),
(#113459,#113460,#113461,#113462),(#113463,#113464,#113465,#113466),(#113467,
#113468,#113469,#113470),(#113471,#113472,#113473,#113474)),
 .UNSPECIFIED.,.F.,.F.,.F.,(4,1,4),(4,4),(0.,0.571428571428571,1.),(0.,
1.2),.UNSPECIFIED.);
#1470=B_SPLINE_SURFACE_WITH_KNOTS('',3,3,((#113504,#113505,#113506,#113507),
(#113508,#113509,#113510,#113511),(#113512,#113513,#113514,#113515),(#113516,
#113517,#113518,#113519),(#113520,#113521,#113522,#113523)),
 .UNSPECIFIED.,.F.,.F.,.F.,(4,1,4),(4,4),(0.,0.571428571428571,1.),(9.71445146547012E-17,
1.2),.UNSPECIFIED.);
#1471=B_SPLINE_SURFACE_WITH_KNOTS('',3,3,((#114351,#114352,#114353,#114354),
(#114355,#114356,#114357,#114358),(#114359,#114360,#114361,#114362),(#114363,
#114364,#114365,#114366),(#114367,#114368,#114369,#114370)),
 .UNSPECIFIED.,.F.,.F.,.F.,(4,1,4),(4,4),(0.,0.571428571428571,1.),(-6.03986977505924E-17,
1.2),.UNSPECIFIED.);
#1472=B_SPLINE_SURFACE_WITH_KNOTS('',3,3,((#114400,#114401,#114402,#114403),
(#114404,#114405,#114406,#114407),(#114408,#114409,#114410,#114411),(#114412,
#114413,#114414,#114415),(#114416,#114417,#114418,#114419)),
 .UNSPECIFIED.,.F.,.F.,.F.,(4,1,4),(4,4),(0.,0.571428571428571,1.),(9.71445146547012E-17,
1.2),.UNSPECIFIED.);
#1473=B_SPLINE_SURFACE_WITH_KNOTS('',3,3,((#115247,#115248,#115249,#115250),
(#115251,#115252,#115253,#115254),(#115255,#115256,#115257,#115258),(#115259,
#115260,#115261,#115262),(#115263,#115264,#115265,#115266)),
 .UNSPECIFIED.,.F.,.F.,.F.,(4,1,4),(4,4),(0.,0.571428571428571,1.),(2.77555756156289E-17,
1.2),.UNSPECIFIED.);
#1474=B_SPLINE_SURFACE_WITH_KNOTS('',3,3,((#115296,#115297,#115298,#115299),
(#115300,#115301,#115302,#115303),(#115304,#115305,#115306,#115307),(#115308,
#115309,#115310,#115311),(#115312,#115313,#115314,#115315)),
 .UNSPECIFIED.,.F.,.F.,.F.,(4,1,4),(4,4),(0.,0.571428571428571,1.),(0.,
1.2),.UNSPECIFIED.);
#1475=B_SPLINE_SURFACE_WITH_KNOTS('',3,3,((#116143,#116144,#116145,#116146),
(#116147,#116148,#116149,#116150),(#116151,#116152,#116153,#116154),(#116155,
#116156,#116157,#116158),(#116159,#116160,#116161,#116162)),
 .UNSPECIFIED.,.F.,.F.,.F.,(4,1,4),(4,4),(0.,0.571428571428571,1.),(-5.55111512312578E-17,
1.2),.UNSPECIFIED.);
#1476=B_SPLINE_SURFACE_WITH_KNOTS('',3,3,((#173282,#173283,#173284,#173285),
(#173286,#173287,#173288,#173289),(#173290,#173291,#173292,#173293),(#173294,
#173295,#173296,#173297),(#173298,#173299,#173300,#173301)),
 .UNSPECIFIED.,.F.,.F.,.F.,(4,1,4),(4,4),(0.,0.571428571428571,1.),(2.13940539033965E-17,
1.2),.UNSPECIFIED.);
#1477=B_SPLINE_SURFACE_WITH_KNOTS('',3,3,((#174126,#174127,#174128,#174129),
(#174130,#174131,#174132,#174133),(#174134,#174135,#174136,#174137),(#174138,
#174139,#174140,#174141),(#174142,#174143,#174144,#174145)),
 .UNSPECIFIED.,.F.,.F.,.F.,(4,1,4),(4,4),(0.,0.571428571428571,1.),(0.,
1.2),.UNSPECIFIED.);
#1526=PLANE('',#25867);
#1527=PLANE('',#25870);
#1528=PLANE('',#25873);
#1529=PLANE('',#25876);
#1530=PLANE('',#26306);
#1531=PLANE('',#26313);
#2064=FACE_OUTER_BOUND('',#3483,.T.);
#2065=FACE_OUTER_BOUND('',#3484,.T.);
#2066=FACE_OUTER_BOUND('',#3485,.T.);
#2067=FACE_OUTER_BOUND('',#3486,.T.);
#2068=FACE_OUTER_BOUND('',#3487,.T.);
#2069=FACE_OUTER_BOUND('',#3488,.T.);
#2070=FACE_OUTER_BOUND('',#3489,.T.);
#2071=FACE_OUTER_BOUND('',#3490,.T.);
#2072=FACE_OUTER_BOUND('',#3491,.T.);
#2073=FACE_OUTER_BOUND('',#3492,.T.);
#2074=FACE_OUTER_BOUND('',#3493,.T.);
#2075=FACE_OUTER_BOUND('',#3494,.T.);
#2076=FACE_OUTER_BOUND('',#3495,.T.);
#2077=FACE_OUTER_BOUND('',#3496,.T.);
#2078=FACE_OUTER_BOUND('',#3497,.T.);
#2079=FACE_OUTER_BOUND('',#3498,.T.);
#2080=FACE_OUTER_BOUND('',#3499,.T.);
#2081=FACE_OUTER_BOUND('',#3500,.T.);
#2082=FACE_OUTER_BOUND('',#3501,.T.);
#2083=FACE_OUTER_BOUND('',#3502,.T.);
#2084=FACE_OUTER_BOUND('',#3503,.T.);
#2085=FACE_OUTER_BOUND('',#3504,.T.);
#2086=FACE_OUTER_BOUND('',#3505,.T.);
#2087=FACE_OUTER_BOUND('',#3506,.T.);
#2088=FACE_OUTER_BOUND('',#3507,.T.);
#2089=FACE_OUTER_BOUND('',#3508,.T.);
#2090=FACE_OUTER_BOUND('',#3509,.T.);
#2091=FACE_OUTER_BOUND('',#3510,.T.);
#2092=FACE_OUTER_BOUND('',#3511,.T.);
#2093=FACE_OUTER_BOUND('',#3512,.T.);
#2094=FACE_OUTER_BOUND('',#3513,.T.);
#2095=FACE_OUTER_BOUND('',#3514,.T.);
#2096=FACE_OUTER_BOUND('',#3515,.T.);
#2097=FACE_OUTER_BOUND('',#3516,.T.);
#2098=FACE_OUTER_BOUND('',#3517,.T.);
#2099=FACE_OUTER_BOUND('',#3518,.T.);
#2100=FACE_OUTER_BOUND('',#3519,.T.);
#2101=FACE_OUTER_BOUND('',#3520,.T.);
#2102=FACE_OUTER_BOUND('',#3521,.T.);
#2103=FACE_OUTER_BOUND('',#3522,.T.);
#2104=FACE_OUTER_BOUND('',#3523,.T.);
#2105=FACE_OUTER_BOUND('',#3524,.T.);
#2106=FACE_OUTER_BOUND('',#3525,.T.);
#2107=FACE_OUTER_BOUND('',#3526,.T.);
#2108=FACE_OUTER_BOUND('',#3527,.T.);
#2109=FACE_OUTER_BOUND('',#3528,.T.);
#2110=FACE_OUTER_BOUND('',#3529,.T.);
#2111=FACE_OUTER_BOUND('',#3530,.T.);
#2112=FACE_OUTER_BOUND('',#3531,.T.);
#2113=FACE_OUTER_BOUND('',#3532,.T.);
#2114=FACE_OUTER_BOUND('',#3533,.T.);
#2115=FACE_OUTER_BOUND('',#3534,.T.);
#2116=FACE_OUTER_BOUND('',#3535,.T.);
#2117=FACE_OUTER_BOUND('',#3536,.T.);
#2118=FACE_OUTER_BOUND('',#3537,.T.);
#2119=FACE_OUTER_BOUND('',#3538,.T.);
#2120=FACE_OUTER_BOUND('',#3539,.T.);
#2121=FACE_OUTER_BOUND('',#3540,.T.);
#2122=FACE_OUTER_BOUND('',#3541,.T.);
#2123=FACE_OUTER_BOUND('',#3542,.T.);
#2124=FACE_OUTER_BOUND('',#3543,.T.);
#2125=FACE_OUTER_BOUND('',#3544,.T.);
#2126=FACE_OUTER_BOUND('',#3545,.T.);
#2127=FACE_OUTER_BOUND('',#3546,.T.);
#2128=FACE_OUTER_BOUND('',#3547,.T.);
#2129=FACE_OUTER_BOUND('',#3548,.T.);
#2130=FACE_OUTER_BOUND('',#3549,.T.);
#2131=FACE_OUTER_BOUND('',#3550,.T.);
#2132=FACE_OUTER_BOUND('',#3551,.T.);
#2133=FACE_OUTER_BOUND('',#3552,.T.);
#2134=FACE_OUTER_BOUND('',#3553,.T.);
#2135=FACE_OUTER_BOUND('',#3554,.T.);
#2136=FACE_OUTER_BOUND('',#3555,.T.);
#2137=FACE_OUTER_BOUND('',#3556,.T.);
#2138=FACE_OUTER_BOUND('',#3557,.T.);
#2139=FACE_OUTER_BOUND('',#3558,.T.);
#2140=FACE_OUTER_BOUND('',#3559,.T.);
#2141=FACE_OUTER_BOUND('',#3560,.T.);
#2142=FACE_OUTER_BOUND('',#3561,.T.);
#2143=FACE_OUTER_BOUND('',#3562,.T.);
#2144=FACE_OUTER_BOUND('',#3563,.T.);
#2145=FACE_OUTER_BOUND('',#3564,.T.);
#2146=FACE_OUTER_BOUND('',#3565,.T.);
#2147=FACE_OUTER_BOUND('',#3566,.T.);
#2148=FACE_OUTER_BOUND('',#3567,.T.);
#2149=FACE_OUTER_BOUND('',#3568,.T.);
#2150=FACE_OUTER_BOUND('',#3569,.T.);
#2151=FACE_OUTER_BOUND('',#3570,.T.);
#2152=FACE_OUTER_BOUND('',#3571,.T.);
#2153=FACE_OUTER_BOUND('',#3572,.T.);
#2154=FACE_OUTER_BOUND('',#3573,.T.);
#2155=FACE_OUTER_BOUND('',#3574,.T.);
#2156=FACE_OUTER_BOUND('',#3575,.T.);
#2157=FACE_OUTER_BOUND('',#3576,.T.);
#2158=FACE_OUTER_BOUND('',#3577,.T.);
#2159=FACE_OUTER_BOUND('',#3578,.T.);
#2160=FACE_OUTER_BOUND('',#3579,.T.);
#2161=FACE_OUTER_BOUND('',#3580,.T.);
#2162=FACE_OUTER_BOUND('',#3581,.T.);
#2163=FACE_OUTER_BOUND('',#3582,.T.);
#2164=FACE_OUTER_BOUND('',#3583,.T.);
#2165=FACE_OUTER_BOUND('',#3584,.T.);
#2166=FACE_OUTER_BOUND('',#3585,.T.);
#2167=FACE_OUTER_BOUND('',#3586,.T.);
#2168=FACE_OUTER_BOUND('',#3587,.T.);
#2169=FACE_OUTER_BOUND('',#3588,.T.);
#2170=FACE_OUTER_BOUND('',#3589,.T.);
#2171=FACE_OUTER_BOUND('',#3590,.T.);
#2172=FACE_OUTER_BOUND('',#3591,.T.);
#2173=FACE_OUTER_BOUND('',#3592,.T.);
#2174=FACE_OUTER_BOUND('',#3593,.T.);
#2175=FACE_OUTER_BOUND('',#3594,.T.);
#2176=FACE_OUTER_BOUND('',#3595,.T.);
#2177=FACE_OUTER_BOUND('',#3596,.T.);
#2178=FACE_OUTER_BOUND('',#3597,.T.);
#2179=FACE_OUTER_BOUND('',#3598,.T.);
#2180=FACE_OUTER_BOUND('',#3599,.T.);
#2181=FACE_OUTER_BOUND('',#3600,.T.);
#2182=FACE_OUTER_BOUND('',#3601,.T.);
#2183=FACE_OUTER_BOUND('',#3602,.T.);
#2184=FACE_OUTER_BOUND('',#3603,.T.);
#2185=FACE_OUTER_BOUND('',#3604,.T.);
#2186=FACE_OUTER_BOUND('',#3605,.T.);
#2187=FACE_OUTER_BOUND('',#3606,.T.);
#2188=FACE_OUTER_BOUND('',#3607,.T.);
#2189=FACE_OUTER_BOUND('',#3608,.T.);
#2190=FACE_OUTER_BOUND('',#3609,.T.);
#2191=FACE_OUTER_BOUND('',#3610,.T.);
#2192=FACE_OUTER_BOUND('',#3611,.T.);
#2193=FACE_OUTER_BOUND('',#3612,.T.);
#2194=FACE_OUTER_BOUND('',#3613,.T.);
#2195=FACE_OUTER_BOUND('',#3614,.T.);
#2196=FACE_OUTER_BOUND('',#3615,.T.);
#2197=FACE_OUTER_BOUND('',#3616,.T.);
#2198=FACE_OUTER_BOUND('',#3617,.T.);
#2199=FACE_OUTER_BOUND('',#3618,.T.);
#2200=FACE_OUTER_BOUND('',#3619,.T.);
#2201=FACE_OUTER_BOUND('',#3620,.T.);
#2202=FACE_OUTER_BOUND('',#3621,.T.);
#2203=FACE_OUTER_BOUND('',#3622,.T.);
#2204=FACE_OUTER_BOUND('',#3623,.T.);
#2205=FACE_OUTER_BOUND('',#3624,.T.);
#2206=FACE_OUTER_BOUND('',#3625,.T.);
#2207=FACE_OUTER_BOUND('',#3626,.T.);
#2208=FACE_OUTER_BOUND('',#3627,.T.);
#2209=FACE_OUTER_BOUND('',#3628,.T.);
#2210=FACE_OUTER_BOUND('',#3629,.T.);
#2211=FACE_OUTER_BOUND('',#3630,.T.);
#2212=FACE_OUTER_BOUND('',#3631,.T.);
#2213=FACE_OUTER_BOUND('',#3632,.T.);
#2214=FACE_OUTER_BOUND('',#3633,.T.);
#2215=FACE_OUTER_BOUND('',#3634,.T.);
#2216=FACE_OUTER_BOUND('',#3635,.T.);
#2217=FACE_OUTER_BOUND('',#3636,.T.);
#2218=FACE_OUTER_BOUND('',#3637,.T.);
#2219=FACE_OUTER_BOUND('',#3638,.T.);
#2220=FACE_OUTER_BOUND('',#3639,.T.);
#2221=FACE_OUTER_BOUND('',#3640,.T.);
#2222=FACE_OUTER_BOUND('',#3641,.T.);
#2223=FACE_OUTER_BOUND('',#3642,.T.);
#2224=FACE_OUTER_BOUND('',#3643,.T.);
#2225=FACE_OUTER_BOUND('',#3644,.T.);
#2226=FACE_OUTER_BOUND('',#3645,.T.);
#2227=FACE_OUTER_BOUND('',#3646,.T.);
#2228=FACE_OUTER_BOUND('',#3647,.T.);
#2229=FACE_OUTER_BOUND('',#3648,.T.);
#2230=FACE_OUTER_BOUND('',#3649,.T.);
#2231=FACE_OUTER_BOUND('',#3650,.T.);
#2232=FACE_OUTER_BOUND('',#3651,.T.);
#2233=FACE_OUTER_BOUND('',#3652,.T.);
#2234=FACE_OUTER_BOUND('',#3653,.T.);
#2235=FACE_OUTER_BOUND('',#3654,.T.);
#2236=FACE_OUTER_BOUND('',#3655,.T.);
#2237=FACE_OUTER_BOUND('',#3656,.T.);
#2238=FACE_OUTER_BOUND('',#3657,.T.);
#2239=FACE_OUTER_BOUND('',#3658,.T.);
#2240=FACE_OUTER_BOUND('',#3659,.T.);
#2241=FACE_OUTER_BOUND('',#3660,.T.);
#2242=FACE_OUTER_BOUND('',#3661,.T.);
#2243=FACE_OUTER_BOUND('',#3662,.T.);
#2244=FACE_OUTER_BOUND('',#3663,.T.);
#2245=FACE_OUTER_BOUND('',#3664,.T.);
#2246=FACE_OUTER_BOUND('',#3665,.T.);
#2247=FACE_OUTER_BOUND('',#3666,.T.);
#2248=FACE_OUTER_BOUND('',#3667,.T.);
#2249=FACE_OUTER_BOUND('',#3668,.T.);
#2250=FACE_OUTER_BOUND('',#3669,.T.);
#2251=FACE_OUTER_BOUND('',#3670,.T.);
#2252=FACE_OUTER_BOUND('',#3671,.T.);
#2253=FACE_OUTER_BOUND('',#3672,.T.);
#2254=FACE_OUTER_BOUND('',#3673,.T.);
#2255=FACE_OUTER_BOUND('',#3674,.T.);
#2256=FACE_OUTER_BOUND('',#3675,.T.);
#2257=FACE_OUTER_BOUND('',#3676,.T.);
#2258=FACE_OUTER_BOUND('',#3677,.T.);
#2259=FACE_OUTER_BOUND('',#3678,.T.);
#2260=FACE_OUTER_BOUND('',#3679,.T.);
#2261=FACE_OUTER_BOUND('',#3680,.T.);
#2262=FACE_OUTER_BOUND('',#3681,.T.);
#2263=FACE_OUTER_BOUND('',#3682,.T.);
#2264=FACE_OUTER_BOUND('',#3683,.T.);
#2265=FACE_OUTER_BOUND('',#3684,.T.);
#2266=FACE_OUTER_BOUND('',#3685,.T.);
#2267=FACE_OUTER_BOUND('',#3686,.T.);
#2268=FACE_OUTER_BOUND('',#3687,.T.);
#2269=FACE_OUTER_BOUND('',#3688,.T.);
#2270=FACE_OUTER_BOUND('',#3689,.T.);
#2271=FACE_OUTER_BOUND('',#3690,.T.);
#2272=FACE_OUTER_BOUND('',#3691,.T.);
#2273=FACE_OUTER_BOUND('',#3692,.T.);
#2274=FACE_OUTER_BOUND('',#3693,.T.);
#2275=FACE_OUTER_BOUND('',#3694,.T.);
#2276=FACE_OUTER_BOUND('',#3695,.T.);
#2277=FACE_OUTER_BOUND('',#3696,.T.);
#2278=FACE_OUTER_BOUND('',#3697,.T.);
#2279=FACE_OUTER_BOUND('',#3698,.T.);
#2280=FACE_OUTER_BOUND('',#3699,.T.);
#2281=FACE_OUTER_BOUND('',#3700,.T.);
#2282=FACE_OUTER_BOUND('',#3701,.T.);
#2283=FACE_OUTER_BOUND('',#3702,.T.);
#2284=FACE_OUTER_BOUND('',#3703,.T.);
#2285=FACE_OUTER_BOUND('',#3704,.T.);
#2286=FACE_OUTER_BOUND('',#3705,.T.);
#2287=FACE_OUTER_BOUND('',#3706,.T.);
#2288=FACE_OUTER_BOUND('',#3707,.T.);
#2289=FACE_OUTER_BOUND('',#3708,.T.);
#2290=FACE_OUTER_BOUND('',#3709,.T.);
#2291=FACE_OUTER_BOUND('',#3710,.T.);
#2292=FACE_OUTER_BOUND('',#3711,.T.);
#2293=FACE_OUTER_BOUND('',#3712,.T.);
#2294=FACE_OUTER_BOUND('',#3713,.T.);
#2295=FACE_OUTER_BOUND('',#3714,.T.);
#2296=FACE_OUTER_BOUND('',#3715,.T.);
#2297=FACE_OUTER_BOUND('',#3716,.T.);
#2298=FACE_OUTER_BOUND('',#3717,.T.);
#2299=FACE_OUTER_BOUND('',#3718,.T.);
#2300=FACE_OUTER_BOUND('',#3719,.T.);
#2301=FACE_OUTER_BOUND('',#3720,.T.);
#2302=FACE_OUTER_BOUND('',#3721,.T.);
#2303=FACE_OUTER_BOUND('',#3722,.T.);
#2304=FACE_OUTER_BOUND('',#3723,.T.);
#2305=FACE_OUTER_BOUND('',#3724,.T.);
#2306=FACE_OUTER_BOUND('',#3725,.T.);
#2307=FACE_OUTER_BOUND('',#3726,.T.);
#2308=FACE_OUTER_BOUND('',#3727,.T.);
#2309=FACE_OUTER_BOUND('',#3728,.T.);
#2310=FACE_OUTER_BOUND('',#3729,.T.);
#2311=FACE_OUTER_BOUND('',#3730,.T.);
#2312=FACE_OUTER_BOUND('',#3731,.T.);
#2313=FACE_OUTER_BOUND('',#3732,.T.);
#2314=FACE_OUTER_BOUND('',#3733,.T.);
#2315=FACE_OUTER_BOUND('',#3734,.T.);
#2316=FACE_OUTER_BOUND('',#3735,.T.);
#2317=FACE_OUTER_BOUND('',#3736,.T.);
#2318=FACE_OUTER_BOUND('',#3737,.T.);
#2319=FACE_OUTER_BOUND('',#3738,.T.);
#2320=FACE_OUTER_BOUND('',#3739,.T.);
#2321=FACE_OUTER_BOUND('',#3740,.T.);
#2322=FACE_OUTER_BOUND('',#3741,.T.);
#2323=FACE_OUTER_BOUND('',#3742,.T.);
#2324=FACE_OUTER_BOUND('',#3743,.T.);
#2325=FACE_OUTER_BOUND('',#3744,.T.);
#2326=FACE_OUTER_BOUND('',#3745,.T.);
#2327=FACE_OUTER_BOUND('',#3746,.T.);
#2328=FACE_OUTER_BOUND('',#3747,.T.);
#2329=FACE_OUTER_BOUND('',#3748,.T.);
#2330=FACE_OUTER_BOUND('',#3749,.T.);
#2331=FACE_OUTER_BOUND('',#3750,.T.);
#2332=FACE_OUTER_BOUND('',#3751,.T.);
#2333=FACE_OUTER_BOUND('',#3752,.T.);
#2334=FACE_OUTER_BOUND('',#3753,.T.);
#2335=FACE_OUTER_BOUND('',#3754,.T.);
#2336=FACE_OUTER_BOUND('',#3755,.T.);
#2337=FACE_OUTER_BOUND('',#3756,.T.);
#2338=FACE_OUTER_BOUND('',#3757,.T.);
#2339=FACE_OUTER_BOUND('',#3758,.T.);
#2340=FACE_OUTER_BOUND('',#3759,.T.);
#2341=FACE_OUTER_BOUND('',#3760,.T.);
#2342=FACE_OUTER_BOUND('',#3761,.T.);
#2343=FACE_OUTER_BOUND('',#3762,.T.);
#2344=FACE_OUTER_BOUND('',#3763,.T.);
#2345=FACE_OUTER_BOUND('',#3764,.T.);
#2346=FACE_OUTER_BOUND('',#3765,.T.);
#2347=FACE_OUTER_BOUND('',#3766,.T.);
#2348=FACE_OUTER_BOUND('',#3767,.T.);
#2349=FACE_OUTER_BOUND('',#3768,.T.);
#2350=FACE_OUTER_BOUND('',#3769,.T.);
#2351=FACE_OUTER_BOUND('',#3770,.T.);
#2352=FACE_OUTER_BOUND('',#3771,.T.);
#2353=FACE_OUTER_BOUND('',#3772,.T.);
#2354=FACE_OUTER_BOUND('',#3773,.T.);
#2355=FACE_OUTER_BOUND('',#3774,.T.);
#2356=FACE_OUTER_BOUND('',#3775,.T.);
#2357=FACE_OUTER_BOUND('',#3776,.T.);
#2358=FACE_OUTER_BOUND('',#3777,.T.);
#2359=FACE_OUTER_BOUND('',#3778,.T.);
#2360=FACE_OUTER_BOUND('',#3779,.T.);
#2361=FACE_OUTER_BOUND('',#3780,.T.);
#2362=FACE_OUTER_BOUND('',#3781,.T.);
#2363=FACE_OUTER_BOUND('',#3782,.T.);
#2364=FACE_OUTER_BOUND('',#3783,.T.);
#2365=FACE_OUTER_BOUND('',#3784,.T.);
#2366=FACE_OUTER_BOUND('',#3785,.T.);
#2367=FACE_OUTER_BOUND('',#3786,.T.);
#2368=FACE_OUTER_BOUND('',#3787,.T.);
#2369=FACE_OUTER_BOUND('',#3788,.T.);
#2370=FACE_OUTER_BOUND('',#3789,.T.);
#2371=FACE_OUTER_BOUND('',#3790,.T.);
#2372=FACE_OUTER_BOUND('',#3791,.T.);
#2373=FACE_OUTER_BOUND('',#3792,.T.);
#2374=FACE_OUTER_BOUND('',#3793,.T.);
#2375=FACE_OUTER_BOUND('',#3794,.T.);
#2376=FACE_OUTER_BOUND('',#3795,.T.);
#2377=FACE_OUTER_BOUND('',#3796,.T.);
#2378=FACE_OUTER_BOUND('',#3797,.T.);
#2379=FACE_OUTER_BOUND('',#3798,.T.);
#2380=FACE_OUTER_BOUND('',#3799,.T.);
#2381=FACE_OUTER_BOUND('',#3800,.T.);
#2382=FACE_OUTER_BOUND('',#3801,.T.);
#2383=FACE_OUTER_BOUND('',#3802,.T.);
#2384=FACE_OUTER_BOUND('',#3803,.T.);
#2385=FACE_OUTER_BOUND('',#3804,.T.);
#2386=FACE_OUTER_BOUND('',#3805,.T.);
#2387=FACE_OUTER_BOUND('',#3806,.T.);
#2388=FACE_OUTER_BOUND('',#3807,.T.);
#2389=FACE_OUTER_BOUND('',#3808,.T.);
#2390=FACE_OUTER_BOUND('',#3809,.T.);
#2391=FACE_OUTER_BOUND('',#3810,.T.);
#2392=FACE_OUTER_BOUND('',#3811,.T.);
#2393=FACE_OUTER_BOUND('',#3812,.T.);
#2394=FACE_OUTER_BOUND('',#3813,.T.);
#2395=FACE_OUTER_BOUND('',#3814,.T.);
#2396=FACE_OUTER_BOUND('',#3815,.T.);
#2397=FACE_OUTER_BOUND('',#3816,.T.);
#2398=FACE_OUTER_BOUND('',#3817,.T.);
#2399=FACE_OUTER_BOUND('',#3818,.T.);
#2400=FACE_OUTER_BOUND('',#3819,.T.);
#2401=FACE_OUTER_BOUND('',#3820,.T.);
#2402=FACE_OUTER_BOUND('',#3821,.T.);
#2403=FACE_OUTER_BOUND('',#3822,.T.);
#2404=FACE_OUTER_BOUND('',#3823,.T.);
#2405=FACE_OUTER_BOUND('',#3824,.T.);
#2406=FACE_OUTER_BOUND('',#3825,.T.);
#2407=FACE_OUTER_BOUND('',#3826,.T.);
#2408=FACE_OUTER_BOUND('',#3827,.T.);
#2409=FACE_OUTER_BOUND('',#3828,.T.);
#2410=FACE_OUTER_BOUND('',#3829,.T.);
#2411=FACE_OUTER_BOUND('',#3830,.T.);
#2412=FACE_OUTER_BOUND('',#3831,.T.);
#2413=FACE_OUTER_BOUND('',#3832,.T.);
#2414=FACE_OUTER_BOUND('',#3833,.T.);
#2415=FACE_OUTER_BOUND('',#3834,.T.);
#2416=FACE_OUTER_BOUND('',#3835,.T.);
#2417=FACE_OUTER_BOUND('',#3836,.T.);
#2418=FACE_OUTER_BOUND('',#3837,.T.);
#2419=FACE_OUTER_BOUND('',#3838,.T.);
#2420=FACE_OUTER_BOUND('',#3839,.T.);
#2421=FACE_OUTER_BOUND('',#3840,.T.);
#2422=FACE_OUTER_BOUND('',#3841,.T.);
#2423=FACE_OUTER_BOUND('',#3842,.T.);
#2424=FACE_OUTER_BOUND('',#3843,.T.);
#2425=FACE_OUTER_BOUND('',#3844,.T.);
#2426=FACE_OUTER_BOUND('',#3845,.T.);
#2427=FACE_OUTER_BOUND('',#3846,.T.);
#2428=FACE_OUTER_BOUND('',#3847,.T.);
#2429=FACE_OUTER_BOUND('',#3848,.T.);
#2430=FACE_OUTER_BOUND('',#3849,.T.);
#2431=FACE_OUTER_BOUND('',#3850,.T.);
#2432=FACE_OUTER_BOUND('',#3851,.T.);
#2433=FACE_OUTER_BOUND('',#3852,.T.);
#2434=FACE_OUTER_BOUND('',#3853,.T.);
#2435=FACE_OUTER_BOUND('',#3854,.T.);
#2436=FACE_OUTER_BOUND('',#3855,.T.);
#2437=FACE_OUTER_BOUND('',#3856,.T.);
#2438=FACE_OUTER_BOUND('',#3857,.T.);
#2439=FACE_OUTER_BOUND('',#3858,.T.);
#2440=FACE_OUTER_BOUND('',#3859,.T.);
#2441=FACE_OUTER_BOUND('',#3860,.T.);
#2442=FACE_OUTER_BOUND('',#3861,.T.);
#2443=FACE_OUTER_BOUND('',#3862,.T.);
#2444=FACE_OUTER_BOUND('',#3863,.T.);
#2445=FACE_OUTER_BOUND('',#3864,.T.);
#2446=FACE_OUTER_BOUND('',#3865,.T.);
#2447=FACE_OUTER_BOUND('',#3866,.T.);
#2448=FACE_OUTER_BOUND('',#3867,.T.);
#2449=FACE_OUTER_BOUND('',#3868,.T.);
#2450=FACE_OUTER_BOUND('',#3869,.T.);
#2451=FACE_OUTER_BOUND('',#3870,.T.);
#2452=FACE_OUTER_BOUND('',#3871,.T.);
#2453=FACE_OUTER_BOUND('',#3872,.T.);
#2454=FACE_OUTER_BOUND('',#3873,.T.);
#2455=FACE_OUTER_BOUND('',#3874,.T.);
#2456=FACE_OUTER_BOUND('',#3875,.T.);
#2457=FACE_OUTER_BOUND('',#3876,.T.);
#2458=FACE_OUTER_BOUND('',#3877,.T.);
#2459=FACE_OUTER_BOUND('',#3878,.T.);
#2460=FACE_OUTER_BOUND('',#3879,.T.);
#2461=FACE_OUTER_BOUND('',#3880,.T.);
#2462=FACE_OUTER_BOUND('',#3881,.T.);
#2463=FACE_OUTER_BOUND('',#3882,.T.);
#2464=FACE_OUTER_BOUND('',#3883,.T.);
#2465=FACE_OUTER_BOUND('',#3884,.T.);
#2466=FACE_OUTER_BOUND('',#3885,.T.);
#2467=FACE_OUTER_BOUND('',#3886,.T.);
#2468=FACE_OUTER_BOUND('',#3887,.T.);
#2469=FACE_OUTER_BOUND('',#3888,.T.);
#2470=FACE_OUTER_BOUND('',#3889,.T.);
#2471=FACE_OUTER_BOUND('',#3890,.T.);
#2472=FACE_OUTER_BOUND('',#3891,.T.);
#2473=FACE_OUTER_BOUND('',#3892,.T.);
#2474=FACE_OUTER_BOUND('',#3893,.T.);
#2475=FACE_OUTER_BOUND('',#3894,.T.);
#2476=FACE_OUTER_BOUND('',#3895,.T.);
#2477=FACE_OUTER_BOUND('',#3896,.T.);
#2478=FACE_OUTER_BOUND('',#3897,.T.);
#2479=FACE_OUTER_BOUND('',#3898,.T.);
#2480=FACE_OUTER_BOUND('',#3899,.T.);
#2481=FACE_OUTER_BOUND('',#3900,.T.);
#2482=FACE_OUTER_BOUND('',#3901,.T.);
#2483=FACE_OUTER_BOUND('',#3902,.T.);
#2484=FACE_OUTER_BOUND('',#3903,.T.);
#2485=FACE_OUTER_BOUND('',#3904,.T.);
#2486=FACE_OUTER_BOUND('',#3905,.T.);
#2487=FACE_OUTER_BOUND('',#3906,.T.);
#2488=FACE_OUTER_BOUND('',#3907,.T.);
#2489=FACE_OUTER_BOUND('',#3908,.T.);
#2490=FACE_OUTER_BOUND('',#3909,.T.);
#2491=FACE_OUTER_BOUND('',#3910,.T.);
#2492=FACE_OUTER_BOUND('',#3911,.T.);
#2493=FACE_OUTER_BOUND('',#3912,.T.);
#2494=FACE_OUTER_BOUND('',#3913,.T.);
#2495=FACE_OUTER_BOUND('',#3914,.T.);
#2496=FACE_OUTER_BOUND('',#3915,.T.);
#2497=FACE_OUTER_BOUND('',#3916,.T.);
#2498=FACE_OUTER_BOUND('',#3917,.T.);
#2499=FACE_OUTER_BOUND('',#3918,.T.);
#2500=FACE_OUTER_BOUND('',#3919,.T.);
#2501=FACE_OUTER_BOUND('',#3920,.T.);
#2502=FACE_OUTER_BOUND('',#3921,.T.);
#2503=FACE_OUTER_BOUND('',#3922,.T.);
#2504=FACE_OUTER_BOUND('',#3924,.T.);
#2505=FACE_OUTER_BOUND('',#3925,.T.);
#2506=FACE_OUTER_BOUND('',#3929,.T.);
#3483=EDGE_LOOP('',(#17502,#17503,#17504,#17505,#17506));
#3484=EDGE_LOOP('',(#17507));
#3485=EDGE_LOOP('',(#17508,#17509,#17510,#17511,#17512));
#3486=EDGE_LOOP('',(#17513));
#3487=EDGE_LOOP('',(#17514,#17515,#17516,#17517,#17518,#17519));
#3488=EDGE_LOOP('',(#17520));
#3489=EDGE_LOOP('',(#17521,#17522,#17523,#17524,#17525,#17526));
#3490=EDGE_LOOP('',(#17527));
#3491=EDGE_LOOP('',(#17528,#17529,#17530,#17531));
#3492=EDGE_LOOP('',(#17532,#17533,#17534,#17535));
#3493=EDGE_LOOP('',(#17536,#17537,#17538,#17539));
#3494=EDGE_LOOP('',(#17540,#17541,#17542,#17543));
#3495=EDGE_LOOP('',(#17544,#17545,#17546,#17547));
#3496=EDGE_LOOP('',(#17548,#17549,#17550,#17551));
#3497=EDGE_LOOP('',(#17552,#17553,#17554,#17555));
#3498=EDGE_LOOP('',(#17556,#17557,#17558,#17559));
#3499=EDGE_LOOP('',(#17560,#17561,#17562,#17563));
#3500=EDGE_LOOP('',(#17564,#17565,#17566,#17567));
#3501=EDGE_LOOP('',(#17568,#17569,#17570,#17571));
#3502=EDGE_LOOP('',(#17572,#17573,#17574,#17575));
#3503=EDGE_LOOP('',(#17576,#17577,#17578,#17579));
#3504=EDGE_LOOP('',(#17580,#17581,#17582,#17583));
#3505=EDGE_LOOP('',(#17584,#17585,#17586,#17587));
#3506=EDGE_LOOP('',(#17588,#17589,#17590,#17591));
#3507=EDGE_LOOP('',(#17592,#17593,#17594,#17595));
#3508=EDGE_LOOP('',(#17596,#17597,#17598,#17599));
#3509=EDGE_LOOP('',(#17600,#17601,#17602,#17603));
#3510=EDGE_LOOP('',(#17604,#17605,#17606,#17607));
#3511=EDGE_LOOP('',(#17608,#17609,#17610,#17611));
#3512=EDGE_LOOP('',(#17612,#17613,#17614,#17615));
#3513=EDGE_LOOP('',(#17616,#17617,#17618,#17619));
#3514=EDGE_LOOP('',(#17620,#17621,#17622,#17623));
#3515=EDGE_LOOP('',(#17624,#17625,#17626,#17627));
#3516=EDGE_LOOP('',(#17628,#17629,#17630,#17631));
#3517=EDGE_LOOP('',(#17632,#17633,#17634,#17635));
#3518=EDGE_LOOP('',(#17636,#17637,#17638,#17639));
#3519=EDGE_LOOP('',(#17640,#17641,#17642,#17643));
#3520=EDGE_LOOP('',(#17644,#17645,#17646,#17647));
#3521=EDGE_LOOP('',(#17648,#17649,#17650,#17651));
#3522=EDGE_LOOP('',(#17652,#17653,#17654,#17655));
#3523=EDGE_LOOP('',(#17656,#17657,#17658,#17659));
#3524=EDGE_LOOP('',(#17660,#17661,#17662,#17663));
#3525=EDGE_LOOP('',(#17664,#17665,#17666,#17667));
#3526=EDGE_LOOP('',(#17668,#17669,#17670,#17671));
#3527=EDGE_LOOP('',(#17672,#17673,#17674,#17675));
#3528=EDGE_LOOP('',(#17676,#17677,#17678,#17679));
#3529=EDGE_LOOP('',(#17680,#17681,#17682,#17683));
#3530=EDGE_LOOP('',(#17684,#17685,#17686,#17687));
#3531=EDGE_LOOP('',(#17688,#17689,#17690,#17691));
#3532=EDGE_LOOP('',(#17692,#17693,#17694,#17695));
#3533=EDGE_LOOP('',(#17696,#17697,#17698,#17699));
#3534=EDGE_LOOP('',(#17700,#17701,#17702,#17703));
#3535=EDGE_LOOP('',(#17704,#17705,#17706,#17707));
#3536=EDGE_LOOP('',(#17708,#17709,#17710,#17711));
#3537=EDGE_LOOP('',(#17712,#17713,#17714,#17715));
#3538=EDGE_LOOP('',(#17716,#17717,#17718,#17719));
#3539=EDGE_LOOP('',(#17720,#17721,#17722,#17723));
#3540=EDGE_LOOP('',(#17724,#17725,#17726,#17727));
#3541=EDGE_LOOP('',(#17728,#17729,#17730,#17731));
#3542=EDGE_LOOP('',(#17732,#17733,#17734,#17735));
#3543=EDGE_LOOP('',(#17736,#17737,#17738,#17739));
#3544=EDGE_LOOP('',(#17740,#17741,#17742,#17743));
#3545=EDGE_LOOP('',(#17744,#17745,#17746,#17747));
#3546=EDGE_LOOP('',(#17748,#17749,#17750,#17751));
#3547=EDGE_LOOP('',(#17752,#17753,#17754,#17755));
#3548=EDGE_LOOP('',(#17756,#17757,#17758,#17759));
#3549=EDGE_LOOP('',(#17760,#17761,#17762,#17763));
#3550=EDGE_LOOP('',(#17764,#17765,#17766,#17767));
#3551=EDGE_LOOP('',(#17768,#17769,#17770,#17771));
#3552=EDGE_LOOP('',(#17772,#17773,#17774,#17775));
#3553=EDGE_LOOP('',(#17776,#17777,#17778,#17779));
#3554=EDGE_LOOP('',(#17780,#17781,#17782,#17783));
#3555=EDGE_LOOP('',(#17784,#17785,#17786,#17787));
#3556=EDGE_LOOP('',(#17788,#17789,#17790,#17791));
#3557=EDGE_LOOP('',(#17792,#17793,#17794,#17795));
#3558=EDGE_LOOP('',(#17796,#17797,#17798,#17799));
#3559=EDGE_LOOP('',(#17800,#17801,#17802,#17803));
#3560=EDGE_LOOP('',(#17804,#17805,#17806,#17807));
#3561=EDGE_LOOP('',(#17808,#17809,#17810,#17811));
#3562=EDGE_LOOP('',(#17812,#17813,#17814,#17815));
#3563=EDGE_LOOP('',(#17816,#17817,#17818,#17819));
#3564=EDGE_LOOP('',(#17820,#17821,#17822,#17823));
#3565=EDGE_LOOP('',(#17824,#17825,#17826,#17827));
#3566=EDGE_LOOP('',(#17828,#17829,#17830,#17831));
#3567=EDGE_LOOP('',(#17832,#17833,#17834,#17835));
#3568=EDGE_LOOP('',(#17836,#17837,#17838,#17839));
#3569=EDGE_LOOP('',(#17840,#17841,#17842,#17843));
#3570=EDGE_LOOP('',(#17844,#17845,#17846,#17847));
#3571=EDGE_LOOP('',(#17848,#17849,#17850,#17851));
#3572=EDGE_LOOP('',(#17852,#17853,#17854,#17855));
#3573=EDGE_LOOP('',(#17856,#17857,#17858,#17859));
#3574=EDGE_LOOP('',(#17860,#17861,#17862,#17863));
#3575=EDGE_LOOP('',(#17864,#17865,#17866,#17867));
#3576=EDGE_LOOP('',(#17868,#17869,#17870,#17871));
#3577=EDGE_LOOP('',(#17872,#17873,#17874,#17875));
#3578=EDGE_LOOP('',(#17876,#17877,#17878,#17879));
#3579=EDGE_LOOP('',(#17880,#17881,#17882,#17883));
#3580=EDGE_LOOP('',(#17884,#17885,#17886,#17887));
#3581=EDGE_LOOP('',(#17888,#17889,#17890,#17891));
#3582=EDGE_LOOP('',(#17892,#17893,#17894,#17895));
#3583=EDGE_LOOP('',(#17896,#17897,#17898,#17899));
#3584=EDGE_LOOP('',(#17900,#17901,#17902,#17903));
#3585=EDGE_LOOP('',(#17904,#17905,#17906,#17907));
#3586=EDGE_LOOP('',(#17908,#17909,#17910,#17911));
#3587=EDGE_LOOP('',(#17912,#17913,#17914,#17915));
#3588=EDGE_LOOP('',(#17916,#17917,#17918,#17919));
#3589=EDGE_LOOP('',(#17920,#17921,#17922,#17923));
#3590=EDGE_LOOP('',(#17924,#17925,#17926,#17927));
#3591=EDGE_LOOP('',(#17928,#17929,#17930,#17931));
#3592=EDGE_LOOP('',(#17932,#17933,#17934,#17935));
#3593=EDGE_LOOP('',(#17936,#17937,#17938,#17939));
#3594=EDGE_LOOP('',(#17940,#17941,#17942,#17943));
#3595=EDGE_LOOP('',(#17944,#17945,#17946,#17947));
#3596=EDGE_LOOP('',(#17948,#17949,#17950,#17951));
#3597=EDGE_LOOP('',(#17952,#17953,#17954,#17955));
#3598=EDGE_LOOP('',(#17956,#17957,#17958,#17959));
#3599=EDGE_LOOP('',(#17960,#17961,#17962,#17963));
#3600=EDGE_LOOP('',(#17964,#17965,#17966,#17967));
#3601=EDGE_LOOP('',(#17968,#17969,#17970,#17971));
#3602=EDGE_LOOP('',(#17972,#17973,#17974,#17975));
#3603=EDGE_LOOP('',(#17976,#17977,#17978,#17979));
#3604=EDGE_LOOP('',(#17980,#17981,#17982,#17983));
#3605=EDGE_LOOP('',(#17984,#17985,#17986,#17987));
#3606=EDGE_LOOP('',(#17988,#17989,#17990,#17991));
#3607=EDGE_LOOP('',(#17992,#17993,#17994,#17995));
#3608=EDGE_LOOP('',(#17996,#17997,#17998,#17999));
#3609=EDGE_LOOP('',(#18000,#18001,#18002,#18003));
#3610=EDGE_LOOP('',(#18004,#18005,#18006,#18007));
#3611=EDGE_LOOP('',(#18008,#18009,#18010,#18011));
#3612=EDGE_LOOP('',(#18012,#18013,#18014,#18015));
#3613=EDGE_LOOP('',(#18016,#18017,#18018,#18019));
#3614=EDGE_LOOP('',(#18020,#18021,#18022,#18023));
#3615=EDGE_LOOP('',(#18024,#18025,#18026,#18027));
#3616=EDGE_LOOP('',(#18028,#18029,#18030,#18031));
#3617=EDGE_LOOP('',(#18032,#18033,#18034,#18035));
#3618=EDGE_LOOP('',(#18036,#18037,#18038,#18039));
#3619=EDGE_LOOP('',(#18040,#18041,#18042,#18043));
#3620=EDGE_LOOP('',(#18044,#18045,#18046,#18047));
#3621=EDGE_LOOP('',(#18048,#18049,#18050,#18051));
#3622=EDGE_LOOP('',(#18052,#18053,#18054,#18055));
#3623=EDGE_LOOP('',(#18056,#18057,#18058,#18059));
#3624=EDGE_LOOP('',(#18060,#18061,#18062,#18063));
#3625=EDGE_LOOP('',(#18064,#18065,#18066,#18067));
#3626=EDGE_LOOP('',(#18068,#18069,#18070,#18071));
#3627=EDGE_LOOP('',(#18072,#18073,#18074,#18075));
#3628=EDGE_LOOP('',(#18076,#18077,#18078,#18079));
#3629=EDGE_LOOP('',(#18080,#18081,#18082,#18083));
#3630=EDGE_LOOP('',(#18084,#18085,#18086,#18087));
#3631=EDGE_LOOP('',(#18088,#18089,#18090,#18091));
#3632=EDGE_LOOP('',(#18092,#18093,#18094,#18095));
#3633=EDGE_LOOP('',(#18096,#18097,#18098,#18099));
#3634=EDGE_LOOP('',(#18100,#18101,#18102,#18103));
#3635=EDGE_LOOP('',(#18104,#18105,#18106,#18107));
#3636=EDGE_LOOP('',(#18108,#18109,#18110,#18111));
#3637=EDGE_LOOP('',(#18112,#18113,#18114,#18115));
#3638=EDGE_LOOP('',(#18116,#18117,#18118,#18119));
#3639=EDGE_LOOP('',(#18120,#18121,#18122,#18123));
#3640=EDGE_LOOP('',(#18124,#18125,#18126,#18127));
#3641=EDGE_LOOP('',(#18128,#18129,#18130,#18131));
#3642=EDGE_LOOP('',(#18132,#18133,#18134,#18135));
#3643=EDGE_LOOP('',(#18136,#18137,#18138,#18139));
#3644=EDGE_LOOP('',(#18140,#18141,#18142,#18143));
#3645=EDGE_LOOP('',(#18144,#18145,#18146,#18147));
#3646=EDGE_LOOP('',(#18148,#18149,#18150,#18151));
#3647=EDGE_LOOP('',(#18152,#18153,#18154,#18155));
#3648=EDGE_LOOP('',(#18156,#18157,#18158,#18159));
#3649=EDGE_LOOP('',(#18160,#18161,#18162,#18163));
#3650=EDGE_LOOP('',(#18164,#18165,#18166,#18167));
#3651=EDGE_LOOP('',(#18168,#18169,#18170,#18171));
#3652=EDGE_LOOP('',(#18172,#18173,#18174,#18175));
#3653=EDGE_LOOP('',(#18176,#18177,#18178,#18179));
#3654=EDGE_LOOP('',(#18180,#18181,#18182,#18183));
#3655=EDGE_LOOP('',(#18184,#18185,#18186,#18187));
#3656=EDGE_LOOP('',(#18188,#18189,#18190,#18191));
#3657=EDGE_LOOP('',(#18192,#18193,#18194,#18195));
#3658=EDGE_LOOP('',(#18196,#18197,#18198,#18199));
#3659=EDGE_LOOP('',(#18200,#18201,#18202,#18203));
#3660=EDGE_LOOP('',(#18204,#18205,#18206,#18207));
#3661=EDGE_LOOP('',(#18208,#18209,#18210,#18211));
#3662=EDGE_LOOP('',(#18212,#18213,#18214,#18215));
#3663=EDGE_LOOP('',(#18216,#18217,#18218,#18219));
#3664=EDGE_LOOP('',(#18220,#18221,#18222,#18223));
#3665=EDGE_LOOP('',(#18224,#18225,#18226,#18227));
#3666=EDGE_LOOP('',(#18228,#18229,#18230,#18231));
#3667=EDGE_LOOP('',(#18232,#18233,#18234,#18235));
#3668=EDGE_LOOP('',(#18236,#18237,#18238,#18239));
#3669=EDGE_LOOP('',(#18240,#18241,#18242,#18243));
#3670=EDGE_LOOP('',(#18244,#18245,#18246,#18247));
#3671=EDGE_LOOP('',(#18248,#18249,#18250,#18251));
#3672=EDGE_LOOP('',(#18252,#18253,#18254,#18255));
#3673=EDGE_LOOP('',(#18256,#18257,#18258,#18259));
#3674=EDGE_LOOP('',(#18260,#18261,#18262,#18263));
#3675=EDGE_LOOP('',(#18264,#18265,#18266,#18267));
#3676=EDGE_LOOP('',(#18268,#18269,#18270,#18271));
#3677=EDGE_LOOP('',(#18272,#18273,#18274,#18275));
#3678=EDGE_LOOP('',(#18276,#18277,#18278,#18279));
#3679=EDGE_LOOP('',(#18280,#18281,#18282,#18283));
#3680=EDGE_LOOP('',(#18284,#18285,#18286,#18287));
#3681=EDGE_LOOP('',(#18288,#18289,#18290,#18291));
#3682=EDGE_LOOP('',(#18292,#18293,#18294,#18295));
#3683=EDGE_LOOP('',(#18296,#18297,#18298,#18299));
#3684=EDGE_LOOP('',(#18300,#18301,#18302,#18303));
#3685=EDGE_LOOP('',(#18304,#18305,#18306,#18307));
#3686=EDGE_LOOP('',(#18308,#18309,#18310,#18311));
#3687=EDGE_LOOP('',(#18312,#18313,#18314,#18315));
#3688=EDGE_LOOP('',(#18316,#18317,#18318,#18319));
#3689=EDGE_LOOP('',(#18320,#18321,#18322,#18323));
#3690=EDGE_LOOP('',(#18324,#18325,#18326,#18327));
#3691=EDGE_LOOP('',(#18328,#18329,#18330,#18331));
#3692=EDGE_LOOP('',(#18332,#18333,#18334,#18335));
#3693=EDGE_LOOP('',(#18336,#18337,#18338,#18339));
#3694=EDGE_LOOP('',(#18340,#18341,#18342,#18343));
#3695=EDGE_LOOP('',(#18344,#18345,#18346,#18347));
#3696=EDGE_LOOP('',(#18348,#18349,#18350,#18351));
#3697=EDGE_LOOP('',(#18352,#18353,#18354,#18355));
#3698=EDGE_LOOP('',(#18356,#18357,#18358,#18359));
#3699=EDGE_LOOP('',(#18360,#18361,#18362,#18363));
#3700=EDGE_LOOP('',(#18364,#18365,#18366,#18367));
#3701=EDGE_LOOP('',(#18368,#18369,#18370,#18371));
#3702=EDGE_LOOP('',(#18372,#18373,#18374,#18375));
#3703=EDGE_LOOP('',(#18376,#18377,#18378,#18379));
#3704=EDGE_LOOP('',(#18380,#18381,#18382,#18383));
#3705=EDGE_LOOP('',(#18384,#18385,#18386,#18387));
#3706=EDGE_LOOP('',(#18388,#18389,#18390,#18391));
#3707=EDGE_LOOP('',(#18392,#18393,#18394,#18395));
#3708=EDGE_LOOP('',(#18396,#18397,#18398,#18399));
#3709=EDGE_LOOP('',(#18400,#18401,#18402,#18403));
#3710=EDGE_LOOP('',(#18404,#18405,#18406,#18407));
#3711=EDGE_LOOP('',(#18408,#18409,#18410,#18411));
#3712=EDGE_LOOP('',(#18412,#18413,#18414,#18415));
#3713=EDGE_LOOP('',(#18416,#18417,#18418,#18419));
#3714=EDGE_LOOP('',(#18420,#18421,#18422,#18423));
#3715=EDGE_LOOP('',(#18424,#18425,#18426,#18427));
#3716=EDGE_LOOP('',(#18428,#18429,#18430,#18431));
#3717=EDGE_LOOP('',(#18432,#18433,#18434,#18435));
#3718=EDGE_LOOP('',(#18436,#18437,#18438,#18439));
#3719=EDGE_LOOP('',(#18440,#18441,#18442,#18443));
#3720=EDGE_LOOP('',(#18444,#18445,#18446,#18447));
#3721=EDGE_LOOP('',(#18448,#18449,#18450,#18451));
#3722=EDGE_LOOP('',(#18452,#18453,#18454,#18455));
#3723=EDGE_LOOP('',(#18456,#18457,#18458,#18459));
#3724=EDGE_LOOP('',(#18460,#18461,#18462,#18463));
#3725=EDGE_LOOP('',(#18464,#18465,#18466,#18467));
#3726=EDGE_LOOP('',(#18468,#18469,#18470,#18471));
#3727=EDGE_LOOP('',(#18472,#18473,#18474,#18475));
#3728=EDGE_LOOP('',(#18476,#18477,#18478,#18479));
#3729=EDGE_LOOP('',(#18480,#18481,#18482,#18483));
#3730=EDGE_LOOP('',(#18484,#18485,#18486,#18487));
#3731=EDGE_LOOP('',(#18488,#18489,#18490,#18491));
#3732=EDGE_LOOP('',(#18492,#18493,#18494,#18495));
#3733=EDGE_LOOP('',(#18496,#18497,#18498,#18499));
#3734=EDGE_LOOP('',(#18500,#18501,#18502,#18503));
#3735=EDGE_LOOP('',(#18504,#18505,#18506,#18507));
#3736=EDGE_LOOP('',(#18508,#18509,#18510,#18511));
#3737=EDGE_LOOP('',(#18512,#18513,#18514,#18515));
#3738=EDGE_LOOP('',(#18516,#18517,#18518,#18519));
#3739=EDGE_LOOP('',(#18520,#18521,#18522,#18523));
#3740=EDGE_LOOP('',(#18524,#18525,#18526,#18527));
#3741=EDGE_LOOP('',(#18528,#18529,#18530,#18531));
#3742=EDGE_LOOP('',(#18532,#18533,#18534,#18535));
#3743=EDGE_LOOP('',(#18536,#18537,#18538,#18539));
#3744=EDGE_LOOP('',(#18540,#18541,#18542,#18543));
#3745=EDGE_LOOP('',(#18544,#18545,#18546,#18547));
#3746=EDGE_LOOP('',(#18548,#18549,#18550,#18551));
#3747=EDGE_LOOP('',(#18552,#18553,#18554,#18555));
#3748=EDGE_LOOP('',(#18556,#18557,#18558,#18559));
#3749=EDGE_LOOP('',(#18560,#18561,#18562,#18563));
#3750=EDGE_LOOP('',(#18564,#18565,#18566,#18567));
#3751=EDGE_LOOP('',(#18568,#18569,#18570,#18571));
#3752=EDGE_LOOP('',(#18572,#18573,#18574,#18575));
#3753=EDGE_LOOP('',(#18576,#18577,#18578,#18579));
#3754=EDGE_LOOP('',(#18580,#18581,#18582,#18583));
#3755=EDGE_LOOP('',(#18584,#18585,#18586,#18587));
#3756=EDGE_LOOP('',(#18588,#18589,#18590,#18591));
#3757=EDGE_LOOP('',(#18592,#18593,#18594,#18595));
#3758=EDGE_LOOP('',(#18596,#18597,#18598,#18599));
#3759=EDGE_LOOP('',(#18600,#18601,#18602,#18603));
#3760=EDGE_LOOP('',(#18604,#18605,#18606,#18607));
#3761=EDGE_LOOP('',(#18608,#18609,#18610,#18611));
#3762=EDGE_LOOP('',(#18612,#18613,#18614,#18615));
#3763=EDGE_LOOP('',(#18616,#18617,#18618,#18619));
#3764=EDGE_LOOP('',(#18620,#18621,#18622,#18623));
#3765=EDGE_LOOP('',(#18624,#18625,#18626,#18627));
#3766=EDGE_LOOP('',(#18628,#18629,#18630,#18631));
#3767=EDGE_LOOP('',(#18632,#18633,#18634,#18635));
#3768=EDGE_LOOP('',(#18636,#18637,#18638,#18639));
#3769=EDGE_LOOP('',(#18640,#18641,#18642,#18643));
#3770=EDGE_LOOP('',(#18644,#18645,#18646,#18647));
#3771=EDGE_LOOP('',(#18648,#18649,#18650,#18651));
#3772=EDGE_LOOP('',(#18652,#18653,#18654,#18655));
#3773=EDGE_LOOP('',(#18656,#18657,#18658,#18659));
#3774=EDGE_LOOP('',(#18660,#18661,#18662,#18663));
#3775=EDGE_LOOP('',(#18664,#18665,#18666,#18667));
#3776=EDGE_LOOP('',(#18668,#18669,#18670,#18671));
#3777=EDGE_LOOP('',(#18672,#18673,#18674,#18675));
#3778=EDGE_LOOP('',(#18676,#18677,#18678,#18679));
#3779=EDGE_LOOP('',(#18680,#18681,#18682,#18683));
#3780=EDGE_LOOP('',(#18684,#18685,#18686,#18687));
#3781=EDGE_LOOP('',(#18688,#18689,#18690,#18691));
#3782=EDGE_LOOP('',(#18692,#18693,#18694,#18695));
#3783=EDGE_LOOP('',(#18696,#18697,#18698,#18699));
#3784=EDGE_LOOP('',(#18700,#18701,#18702,#18703));
#3785=EDGE_LOOP('',(#18704,#18705,#18706,#18707));
#3786=EDGE_LOOP('',(#18708,#18709,#18710,#18711));
#3787=EDGE_LOOP('',(#18712,#18713,#18714,#18715));
#3788=EDGE_LOOP('',(#18716,#18717,#18718,#18719));
#3789=EDGE_LOOP('',(#18720,#18721,#18722,#18723));
#3790=EDGE_LOOP('',(#18724,#18725,#18726,#18727));
#3791=EDGE_LOOP('',(#18728,#18729,#18730,#18731));
#3792=EDGE_LOOP('',(#18732,#18733,#18734,#18735));
#3793=EDGE_LOOP('',(#18736,#18737,#18738,#18739));
#3794=EDGE_LOOP('',(#18740,#18741,#18742,#18743));
#3795=EDGE_LOOP('',(#18744,#18745,#18746,#18747));
#3796=EDGE_LOOP('',(#18748,#18749,#18750,#18751));
#3797=EDGE_LOOP('',(#18752,#18753,#18754,#18755));
#3798=EDGE_LOOP('',(#18756,#18757,#18758,#18759));
#3799=EDGE_LOOP('',(#18760,#18761,#18762,#18763));
#3800=EDGE_LOOP('',(#18764,#18765,#18766,#18767));
#3801=EDGE_LOOP('',(#18768,#18769,#18770,#18771));
#3802=EDGE_LOOP('',(#18772,#18773,#18774,#18775));
#3803=EDGE_LOOP('',(#18776,#18777,#18778,#18779));
#3804=EDGE_LOOP('',(#18780,#18781,#18782,#18783));
#3805=EDGE_LOOP('',(#18784,#18785,#18786,#18787));
#3806=EDGE_LOOP('',(#18788,#18789,#18790,#18791));
#3807=EDGE_LOOP('',(#18792,#18793,#18794,#18795));
#3808=EDGE_LOOP('',(#18796,#18797,#18798,#18799));
#3809=EDGE_LOOP('',(#18800,#18801,#18802,#18803));
#3810=EDGE_LOOP('',(#18804,#18805,#18806,#18807));
#3811=EDGE_LOOP('',(#18808,#18809,#18810,#18811));
#3812=EDGE_LOOP('',(#18812,#18813,#18814,#18815));
#3813=EDGE_LOOP('',(#18816,#18817,#18818,#18819));
#3814=EDGE_LOOP('',(#18820,#18821,#18822,#18823));
#3815=EDGE_LOOP('',(#18824,#18825,#18826,#18827));
#3816=EDGE_LOOP('',(#18828,#18829,#18830,#18831));
#3817=EDGE_LOOP('',(#18832,#18833,#18834,#18835));
#3818=EDGE_LOOP('',(#18836,#18837,#18838,#18839));
#3819=EDGE_LOOP('',(#18840,#18841,#18842,#18843));
#3820=EDGE_LOOP('',(#18844,#18845,#18846,#18847));
#3821=EDGE_LOOP('',(#18848,#18849,#18850,#18851));
#3822=EDGE_LOOP('',(#18852,#18853,#18854,#18855));
#3823=EDGE_LOOP('',(#18856,#18857,#18858,#18859));
#3824=EDGE_LOOP('',(#18860,#18861,#18862,#18863));
#3825=EDGE_LOOP('',(#18864,#18865,#18866,#18867));
#3826=EDGE_LOOP('',(#18868,#18869,#18870,#18871));
#3827=EDGE_LOOP('',(#18872,#18873,#18874,#18875));
#3828=EDGE_LOOP('',(#18876,#18877,#18878,#18879));
#3829=EDGE_LOOP('',(#18880,#18881,#18882,#18883));
#3830=EDGE_LOOP('',(#18884,#18885,#18886,#18887));
#3831=EDGE_LOOP('',(#18888,#18889,#18890,#18891));
#3832=EDGE_LOOP('',(#18892,#18893,#18894,#18895));
#3833=EDGE_LOOP('',(#18896,#18897,#18898,#18899));
#3834=EDGE_LOOP('',(#18900,#18901,#18902,#18903));
#3835=EDGE_LOOP('',(#18904,#18905,#18906,#18907));
#3836=EDGE_LOOP('',(#18908,#18909,#18910,#18911));
#3837=EDGE_LOOP('',(#18912,#18913,#18914,#18915));
#3838=EDGE_LOOP('',(#18916,#18917,#18918,#18919));
#3839=EDGE_LOOP('',(#18920,#18921,#18922,#18923));
#3840=EDGE_LOOP('',(#18924,#18925,#18926,#18927));
#3841=EDGE_LOOP('',(#18928,#18929,#18930,#18931));
#3842=EDGE_LOOP('',(#18932,#18933,#18934,#18935));
#3843=EDGE_LOOP('',(#18936,#18937,#18938,#18939));
#3844=EDGE_LOOP('',(#18940,#18941,#18942,#18943));
#3845=EDGE_LOOP('',(#18944,#18945,#18946,#18947));
#3846=EDGE_LOOP('',(#18948,#18949,#18950,#18951));
#3847=EDGE_LOOP('',(#18952,#18953,#18954,#18955));
#3848=EDGE_LOOP('',(#18956,#18957,#18958,#18959));
#3849=EDGE_LOOP('',(#18960,#18961,#18962,#18963));
#3850=EDGE_LOOP('',(#18964,#18965,#18966,#18967));
#3851=EDGE_LOOP('',(#18968,#18969,#18970,#18971));
#3852=EDGE_LOOP('',(#18972,#18973,#18974,#18975));
#3853=EDGE_LOOP('',(#18976,#18977,#18978,#18979));
#3854=EDGE_LOOP('',(#18980,#18981,#18982,#18983));
#3855=EDGE_LOOP('',(#18984,#18985,#18986,#18987));
#3856=EDGE_LOOP('',(#18988,#18989,#18990,#18991));
#3857=EDGE_LOOP('',(#18992,#18993,#18994,#18995));
#3858=EDGE_LOOP('',(#18996,#18997,#18998,#18999));
#3859=EDGE_LOOP('',(#19000,#19001,#19002,#19003));
#3860=EDGE_LOOP('',(#19004,#19005,#19006,#19007));
#3861=EDGE_LOOP('',(#19008,#19009,#19010,#19011));
#3862=EDGE_LOOP('',(#19012,#19013,#19014,#19015));
#3863=EDGE_LOOP('',(#19016,#19017,#19018,#19019));
#3864=EDGE_LOOP('',(#19020,#19021,#19022,#19023));
#3865=EDGE_LOOP('',(#19024,#19025,#19026,#19027));
#3866=EDGE_LOOP('',(#19028,#19029,#19030,#19031));
#3867=EDGE_LOOP('',(#19032,#19033,#19034,#19035));
#3868=EDGE_LOOP('',(#19036,#19037,#19038,#19039));
#3869=EDGE_LOOP('',(#19040,#19041,#19042,#19043));
#3870=EDGE_LOOP('',(#19044,#19045,#19046,#19047));
#3871=EDGE_LOOP('',(#19048,#19049,#19050,#19051));
#3872=EDGE_LOOP('',(#19052,#19053,#19054,#19055));
#3873=EDGE_LOOP('',(#19056,#19057,#19058,#19059));
#3874=EDGE_LOOP('',(#19060,#19061,#19062,#19063));
#3875=EDGE_LOOP('',(#19064,#19065,#19066,#19067));
#3876=EDGE_LOOP('',(#19068,#19069,#19070,#19071));
#3877=EDGE_LOOP('',(#19072,#19073,#19074,#19075));
#3878=EDGE_LOOP('',(#19076,#19077,#19078,#19079));
#3879=EDGE_LOOP('',(#19080,#19081,#19082,#19083));
#3880=EDGE_LOOP('',(#19084,#19085,#19086,#19087));
#3881=EDGE_LOOP('',(#19088,#19089,#19090,#19091));
#3882=EDGE_LOOP('',(#19092,#19093,#19094,#19095));
#3883=EDGE_LOOP('',(#19096,#19097,#19098,#19099));
#3884=EDGE_LOOP('',(#19100,#19101,#19102,#19103));
#3885=EDGE_LOOP('',(#19104,#19105,#19106,#19107));
#3886=EDGE_LOOP('',(#19108,#19109,#19110,#19111));
#3887=EDGE_LOOP('',(#19112,#19113,#19114,#19115));
#3888=EDGE_LOOP('',(#19116,#19117,#19118,#19119));
#3889=EDGE_LOOP('',(#19120,#19121,#19122,#19123));
#3890=EDGE_LOOP('',(#19124,#19125,#19126,#19127));
#3891=EDGE_LOOP('',(#19128,#19129,#19130,#19131));
#3892=EDGE_LOOP('',(#19132,#19133,#19134,#19135));
#3893=EDGE_LOOP('',(#19136,#19137,#19138,#19139));
#3894=EDGE_LOOP('',(#19140,#19141,#19142,#19143));
#3895=EDGE_LOOP('',(#19144,#19145,#19146,#19147));
#3896=EDGE_LOOP('',(#19148,#19149,#19150,#19151));
#3897=EDGE_LOOP('',(#19152,#19153,#19154,#19155));
#3898=EDGE_LOOP('',(#19156,#19157,#19158,#19159));
#3899=EDGE_LOOP('',(#19160,#19161,#19162,#19163));
#3900=EDGE_LOOP('',(#19164,#19165,#19166,#19167));
#3901=EDGE_LOOP('',(#19168,#19169,#19170,#19171));
#3902=EDGE_LOOP('',(#19172,#19173,#19174,#19175));
#3903=EDGE_LOOP('',(#19176,#19177,#19178,#19179));
#3904=EDGE_LOOP('',(#19180,#19181,#19182,#19183));
#3905=EDGE_LOOP('',(#19184,#19185,#19186,#19187));
#3906=EDGE_LOOP('',(#19188,#19189,#19190,#19191));
#3907=EDGE_LOOP('',(#19192,#19193,#19194,#19195));
#3908=EDGE_LOOP('',(#19196,#19197,#19198,#19199));
#3909=EDGE_LOOP('',(#19200,#19201,#19202,#19203));
#3910=EDGE_LOOP('',(#19204,#19205,#19206,#19207));
#3911=EDGE_LOOP('',(#19208,#19209,#19210,#19211));
#3912=EDGE_LOOP('',(#19212,#19213,#19214,#19215));
#3913=EDGE_LOOP('',(#19216,#19217,#19218,#19219));
#3914=EDGE_LOOP('',(#19220,#19221,#19222,#19223));
#3915=EDGE_LOOP('',(#19224,#19225,#19226,#19227));
#3916=EDGE_LOOP('',(#19228,#19229,#19230,#19231));
#3917=EDGE_LOOP('',(#19232,#19233,#19234,#19235));
#3918=EDGE_LOOP('',(#19236,#19237,#19238,#19239));
#3919=EDGE_LOOP('',(#19240,#19241,#19242,#19243));
#3920=EDGE_LOOP('',(#19244,#19245,#19246,#19247));
#3921=EDGE_LOOP('',(#19248,#19249,#19250,#19251));
#3922=EDGE_LOOP('',(#19252));
#3923=EDGE_LOOP('',(#19253,#19254,#19255,#19256,#19257,#19258,#19259,#19260,
#19261,#19262,#19263,#19264,#19265,#19266,#19267,#19268,#19269,#19270,#19271,
#19272,#19273,#19274,#19275,#19276,#19277,#19278,#19279,#19280,#19281,#19282,
#19283,#19284,#19285,#19286,#19287,#19288,#19289,#19290,#19291,#19292,#19293,
#19294,#19295,#19296,#19297,#19298,#19299,#19300,#19301,#19302,#19303,#19304,
#19305,#19306,#19307,#19308,#19309,#19310,#19311,#19312,#19313,#19314,#19315,
#19316,#19317,#19318,#19319,#19320,#19321,#19322,#19323,#19324,#19325,#19326,
#19327,#19328,#19329,#19330,#19331,#19332,#19333,#19334,#19335,#19336,#19337,
#19338,#19339,#19340,#19341,#19342,#19343,#19344,#19345,#19346,#19347,#19348,
#19349,#19350,#19351,#19352,#19353,#19354,#19355,#19356,#19357,#19358,#19359,
#19360,#19361,#19362,#19363,#19364,#19365,#19366,#19367,#19368,#19369,#19370,
#19371,#19372,#19373,#19374,#19375,#19376,#19377,#19378,#19379,#19380,#19381,
#19382,#19383,#19384,#19385,#19386,#19387,#19388,#19389,#19390,#19391,#19392,
#19393,#19394,#19395,#19396,#19397,#19398,#19399,#19400,#19401,#19402,#19403,
#19404,#19405,#19406,#19407,#19408,#19409,#19410,#19411,#19412,#19413,#19414,
#19415,#19416,#19417,#19418,#19419,#19420,#19421,#19422,#19423,#19424,#19425,
#19426,#19427,#19428,#19429,#19430,#19431,#19432,#19433,#19434,#19435,#19436,
#19437,#19438,#19439,#19440,#19441,#19442,#19443,#19444,#19445,#19446,#19447,
#19448,#19449,#19450,#19451,#19452,#19453,#19454,#19455,#19456,#19457,#19458,
#19459,#19460,#19461,#19462,#19463,#19464,#19465,#19466,#19467,#19468,#19469,
#19470,#19471,#19472,#19473,#19474,#19475,#19476,#19477,#19478,#19479,#19480,
#19481,#19482,#19483,#19484,#19485,#19486,#19487,#19488,#19489,#19490,#19491,
#19492,#19493,#19494,#19495,#19496,#19497,#19498,#19499,#19500,#19501,#19502,
#19503,#19504,#19505,#19506,#19507,#19508,#19509,#19510,#19511,#19512,#19513,
#19514,#19515,#19516,#19517,#19518,#19519,#19520,#19521,#19522,#19523,#19524,
#19525,#19526,#19527,#19528,#19529,#19530,#19531,#19532,#19533,#19534,#19535,
#19536,#19537,#19538,#19539,#19540,#19541,#19542,#19543,#19544,#19545,#19546,
#19547,#19548,#19549,#19550,#19551,#19552,#19553,#19554,#19555,#19556,#19557,
#19558,#19559,#19560,#19561,#19562,#19563,#19564,#19565,#19566,#19567,#19568,
#19569,#19570,#19571,#19572,#19573,#19574,#19575,#19576,#19577,#19578,#19579,
#19580,#19581,#19582,#19583,#19584,#19585,#19586,#19587,#19588,#19589,#19590,
#19591,#19592,#19593,#19594,#19595,#19596,#19597,#19598,#19599,#19600,#19601,
#19602,#19603,#19604,#19605,#19606,#19607,#19608,#19609,#19610,#19611,#19612,
#19613,#19614,#19615,#19616,#19617,#19618,#19619,#19620,#19621,#19622,#19623,
#19624,#19625,#19626,#19627,#19628,#19629,#19630,#19631,#19632,#19633,#19634,
#19635,#19636,#19637,#19638,#19639,#19640,#19641,#19642,#19643,#19644,#19645,
#19646,#19647,#19648,#19649,#19650,#19651,#19652,#19653,#19654,#19655,#19656,
#19657,#19658,#19659,#19660,#19661,#19662,#19663,#19664,#19665,#19666,#19667,
#19668,#19669,#19670,#19671,#19672,#19673,#19674,#19675,#19676,#19677,#19678,
#19679,#19680,#19681,#19682,#19683,#19684));
#3924=EDGE_LOOP('',(#19685,#19686,#19687,#19688));
#3925=EDGE_LOOP('',(#19689,#19690,#19691,#19692,#19693,#19694,#19695,#19696,
#19697));
#3926=EDGE_LOOP('',(#19698,#19699));
#3927=EDGE_LOOP('',(#19700,#19701));
#3928=EDGE_LOOP('',(#19702,#19703,#19704));
#3929=EDGE_LOOP('',(#19705));
#3930=EDGE_LOOP('',(#19706,#19707,#19708,#19709,#19710,#19711,#19712,#19713,
#19714,#19715,#19716,#19717,#19718,#19719,#19720,#19721,#19722,#19723,#19724,
#19725,#19726,#19727,#19728,#19729,#19730,#19731,#19732,#19733,#19734,#19735,
#19736,#19737,#19738,#19739,#19740,#19741,#19742,#19743,#19744,#19745,#19746,
#19747,#19748,#19749,#19750,#19751,#19752,#19753,#19754,#19755,#19756,#19757,
#19758,#19759,#19760,#19761,#19762,#19763,#19764,#19765,#19766,#19767,#19768,
#19769,#19770,#19771,#19772,#19773,#19774,#19775,#19776,#19777,#19778,#19779,
#19780,#19781,#19782,#19783,#19784,#19785,#19786,#19787,#19788,#19789,#19790,
#19791,#19792,#19793,#19794,#19795,#19796,#19797,#19798,#19799,#19800,#19801,
#19802,#19803,#19804,#19805,#19806,#19807,#19808,#19809,#19810,#19811,#19812,
#19813,#19814,#19815,#19816,#19817,#19818,#19819,#19820,#19821,#19822,#19823,
#19824,#19825,#19826,#19827,#19828,#19829,#19830,#19831,#19832,#19833,#19834,
#19835,#19836,#19837,#19838,#19839,#19840,#19841,#19842,#19843,#19844,#19845,
#19846,#19847,#19848,#19849,#19850,#19851,#19852,#19853,#19854,#19855,#19856,
#19857,#19858,#19859,#19860,#19861,#19862,#19863,#19864,#19865,#19866,#19867,
#19868,#19869,#19870,#19871,#19872,#19873,#19874,#19875,#19876,#19877,#19878,
#19879,#19880,#19881,#19882,#19883,#19884,#19885,#19886,#19887,#19888,#19889,
#19890,#19891,#19892,#19893,#19894,#19895,#19896,#19897,#19898,#19899,#19900,
#19901,#19902,#19903,#19904,#19905,#19906,#19907,#19908,#19909,#19910,#19911,
#19912,#19913,#19914,#19915,#19916,#19917,#19918,#19919,#19920,#19921,#19922,
#19923,#19924,#19925,#19926,#19927,#19928,#19929,#19930,#19931,#19932,#19933,
#19934,#19935,#19936,#19937,#19938,#19939,#19940,#19941,#19942,#19943,#19944,
#19945,#19946,#19947,#19948,#19949,#19950,#19951,#19952,#19953,#19954,#19955,
#19956,#19957,#19958,#19959,#19960,#19961,#19962,#19963,#19964,#19965,#19966,
#19967,#19968,#19969,#19970,#19971,#19972,#19973,#19974,#19975,#19976,#19977,
#19978,#19979,#19980,#19981,#19982,#19983,#19984,#19985,#19986,#19987,#19988,
#19989,#19990,#19991,#19992,#19993,#19994,#19995,#19996,#19997,#19998,#19999,
#20000,#20001,#20002,#20003,#20004,#20005,#20006,#20007,#20008,#20009,#20010,
#20011,#20012,#20013,#20014,#20015,#20016,#20017,#20018,#20019,#20020,#20021,
#20022,#20023,#20024,#20025,#20026,#20027,#20028,#20029,#20030,#20031,#20032,
#20033,#20034,#20035,#20036,#20037,#20038,#20039,#20040,#20041,#20042,#20043,
#20044,#20045,#20046,#20047,#20048,#20049,#20050,#20051,#20052,#20053,#20054,
#20055,#20056,#20057,#20058,#20059,#20060,#20061,#20062,#20063,#20064,#20065,
#20066,#20067,#20068,#20069,#20070,#20071,#20072,#20073,#20074,#20075,#20076,
#20077,#20078,#20079,#20080,#20081,#20082,#20083,#20084,#20085,#20086,#20087,
#20088,#20089,#20090,#20091,#20092,#20093,#20094,#20095,#20096,#20097,#20098,
#20099,#20100,#20101,#20102,#20103,#20104,#20105,#20106,#20107,#20108,#20109,
#20110,#20111,#20112,#20113,#20114,#20115,#20116,#20117,#20118,#20119,#20120,
#20121,#20122,#20123,#20124,#20125,#20126,#20127,#20128,#20129,#20130,#20131,
#20132,#20133,#20134,#20135,#20136,#20137));
#4623=CIRCLE('',#25866,2.);
#4624=CIRCLE('',#25869,2.);
#4625=CIRCLE('',#25872,2.);
#4626=CIRCLE('',#25875,2.);
#4627=CIRCLE('',#25878,74.4999999996252);
#4628=CIRCLE('',#25879,74.4999999996252);
#4629=CIRCLE('',#25881,74.4999999996252);
#4630=CIRCLE('',#25882,74.4999999996252);
#4631=CIRCLE('',#25884,74.4999999996252);
#4632=CIRCLE('',#25885,74.4999999996252);
#4633=CIRCLE('',#25887,74.4999999996252);
#4634=CIRCLE('',#25888,74.4999999996252);
#4635=CIRCLE('',#25890,74.4999999996252);
#4636=CIRCLE('',#25891,74.4999999996252);
#4637=CIRCLE('',#25893,74.4999999996252);
#4638=CIRCLE('',#25894,74.4999999996252);
#4639=CIRCLE('',#25896,74.4999999996252);
#4640=CIRCLE('',#25897,74.4999999996252);
#4641=CIRCLE('',#25899,74.4999999996252);
#4642=CIRCLE('',#25900,74.4999999996252);
#4643=CIRCLE('',#25902,74.4999999996252);
#4644=CIRCLE('',#25903,74.4999999996252);
#4645=CIRCLE('',#25905,74.4999999996252);
#4646=CIRCLE('',#25906,74.4999999996252);
#4647=CIRCLE('',#25908,74.4999999996252);
#4648=CIRCLE('',#25909,74.4999999996252);
#4649=CIRCLE('',#25911,74.4999999996252);
#4650=CIRCLE('',#25912,74.4999999996252);
#4651=CIRCLE('',#25914,74.4999999996252);
#4652=CIRCLE('',#25915,74.4999999996252);
#4653=CIRCLE('',#25917,74.4999999996252);
#4654=CIRCLE('',#25918,74.4999999996252);
#4655=CIRCLE('',#25920,74.4999999996252);
#4656=CIRCLE('',#25921,74.4999999996252);
#4657=CIRCLE('',#25923,74.4999999996252);
#4658=CIRCLE('',#25924,74.4999999996252);
#4659=CIRCLE('',#25926,74.4999999996252);
#4660=CIRCLE('',#25927,74.4999999996252);
#4661=CIRCLE('',#25929,74.4999999996252);
#4662=CIRCLE('',#25930,74.4999999996252);
#4663=CIRCLE('',#25932,74.4999999996252);
#4664=CIRCLE('',#25933,74.4999999996252);
#4665=CIRCLE('',#25935,74.4999999996252);
#4666=CIRCLE('',#25936,74.4999999996252);
#4667=CIRCLE('',#25938,74.4999999996252);
#4668=CIRCLE('',#25939,74.4999999996252);
#4669=CIRCLE('',#25941,74.4999999996252);
#4670=CIRCLE('',#25942,74.4999999996252);
#4671=CIRCLE('',#25944,74.4999999996252);
#4672=CIRCLE('',#25945,74.4999999996252);
#4673=CIRCLE('',#25947,74.4999999996252);
#4674=CIRCLE('',#25948,74.4999999996252);
#4675=CIRCLE('',#25950,74.4999999996252);
#4676=CIRCLE('',#25951,74.4999999996252);
#4677=CIRCLE('',#25953,74.4999999996252);
#4678=CIRCLE('',#25954,74.4999999996252);
#4679=CIRCLE('',#25956,74.4999999996252);
#4680=CIRCLE('',#25957,74.4999999996252);
#4681=CIRCLE('',#25959,74.4999999996252);
#4682=CIRCLE('',#25960,74.4999999996252);
#4683=CIRCLE('',#25962,74.4999999996252);
#4684=CIRCLE('',#25963,74.4999999996252);
#4685=CIRCLE('',#25965,74.4999999996252);
#4686=CIRCLE('',#25966,74.4999999996252);
#4687=CIRCLE('',#25968,74.4999999996252);
#4688=CIRCLE('',#25969,74.4999999996252);
#4689=CIRCLE('',#25971,74.4999999996252);
#4690=CIRCLE('',#25972,74.4999999996252);
#4691=CIRCLE('',#25974,74.4999999996252);
#4692=CIRCLE('',#25975,74.4999999996252);
#4693=CIRCLE('',#25977,74.4999999996252);
#4694=CIRCLE('',#25978,74.4999999996252);
#4695=CIRCLE('',#25980,74.4999999996252);
#4696=CIRCLE('',#25981,74.4999999996252);
#4697=CIRCLE('',#25983,74.4999999996252);
#4698=CIRCLE('',#25984,74.4999999996252);
#4699=CIRCLE('',#25986,74.4999999996252);
#4700=CIRCLE('',#25987,74.4999999996252);
#4701=CIRCLE('',#25989,74.4999999996252);
#4702=CIRCLE('',#25990,74.4999999996252);
#4703=CIRCLE('',#25992,74.4999999996252);
#4704=CIRCLE('',#25993,74.4999999996252);
#4705=CIRCLE('',#25995,74.4999999996252);
#4706=CIRCLE('',#25996,74.4999999996252);
#4707=CIRCLE('',#25998,74.4999999996252);
#4708=CIRCLE('',#25999,74.4999999996252);
#4709=CIRCLE('',#26001,74.4999999996252);
#4710=CIRCLE('',#26002,74.4999999996252);
#4711=CIRCLE('',#26004,74.4999999996252);
#4712=CIRCLE('',#26005,74.4999999996252);
#4713=CIRCLE('',#26007,74.4999999996252);
#4714=CIRCLE('',#26008,74.4999999996252);
#4715=CIRCLE('',#26010,74.4999999996252);
#4716=CIRCLE('',#26011,74.4999999996252);
#4717=CIRCLE('',#26013,74.4999999996252);
#4718=CIRCLE('',#26014,74.4999999996252);
#4719=CIRCLE('',#26016,74.4999999996252);
#4720=CIRCLE('',#26017,74.4999999996252);
#4721=CIRCLE('',#26019,74.4999999996252);
#4722=CIRCLE('',#26020,74.4999999996252);
#4723=CIRCLE('',#26022,74.4999999996252);
#4724=CIRCLE('',#26023,74.4999999996252);
#4725=CIRCLE('',#26025,74.4999999996252);
#4726=CIRCLE('',#26026,74.4999999996252);
#4727=CIRCLE('',#26028,74.4999999996252);
#4728=CIRCLE('',#26029,74.4999999996252);
#4729=CIRCLE('',#26031,74.4999999996252);
#4730=CIRCLE('',#26032,74.4999999996252);
#4731=CIRCLE('',#26034,74.4999999996252);
#4732=CIRCLE('',#26035,74.4999999996252);
#4733=CIRCLE('',#26037,74.4999999996252);
#4734=CIRCLE('',#26038,74.4999999996252);
#4735=CIRCLE('',#26040,74.4999999996252);
#4736=CIRCLE('',#26041,74.4999999996252);
#4737=CIRCLE('',#26043,74.4999999996252);
#4738=CIRCLE('',#26044,74.4999999996252);
#4739=CIRCLE('',#26046,74.4999999996252);
#4740=CIRCLE('',#26047,74.4999999996252);
#4741=CIRCLE('',#26049,74.4999999996252);
#4742=CIRCLE('',#26050,74.4999999996252);
#4743=CIRCLE('',#26052,74.4999999996252);
#4744=CIRCLE('',#26053,74.4999999996252);
#4745=CIRCLE('',#26055,74.4999999996252);
#4746=CIRCLE('',#26056,74.4999999996252);
#4747=CIRCLE('',#26058,74.4999999996252);
#4748=CIRCLE('',#26059,74.4999999996252);
#4749=CIRCLE('',#26061,74.4999999996252);
#4750=CIRCLE('',#26062,74.4999999996252);
#4751=CIRCLE('',#26064,74.4999999996252);
#4752=CIRCLE('',#26065,74.4999999996252);
#4753=CIRCLE('',#26067,74.4999999996252);
#4754=CIRCLE('',#26068,74.4999999996252);
#4755=CIRCLE('',#26070,74.4999999996252);
#4756=CIRCLE('',#26071,74.4999999996252);
#4757=CIRCLE('',#26073,74.4999999996252);
#4758=CIRCLE('',#26074,74.4999999996252);
#4759=CIRCLE('',#26076,74.4999999996252);
#4760=CIRCLE('',#26077,74.4999999996252);
#4761=CIRCLE('',#26079,74.4999999996252);
#4762=CIRCLE('',#26080,74.4999999996252);
#4763=CIRCLE('',#26082,74.4999999996252);
#4764=CIRCLE('',#26083,74.4999999996252);
#4765=CIRCLE('',#26085,74.4999999996252);
#4766=CIRCLE('',#26086,74.4999999996252);
#4767=CIRCLE('',#26088,74.4999999996252);
#4768=CIRCLE('',#26089,74.4999999996252);
#4769=CIRCLE('',#26091,70.);
#4770=CIRCLE('',#26092,70.);
#4771=CIRCLE('',#26094,70.);
#4772=CIRCLE('',#26095,70.);
#4773=CIRCLE('',#26097,70.);
#4774=CIRCLE('',#26098,70.);
#4775=CIRCLE('',#26100,70.);
#4776=CIRCLE('',#26101,70.);
#4777=CIRCLE('',#26103,70.);
#4778=CIRCLE('',#26104,70.);
#4779=CIRCLE('',#26106,70.);
#4780=CIRCLE('',#26107,70.);
#4781=CIRCLE('',#26109,70.);
#4782=CIRCLE('',#26110,70.);
#4783=CIRCLE('',#26112,70.);
#4784=CIRCLE('',#26113,70.);
#4785=CIRCLE('',#26115,70.);
#4786=CIRCLE('',#26116,70.);
#4787=CIRCLE('',#26118,70.);
#4788=CIRCLE('',#26119,70.);
#4789=CIRCLE('',#26121,70.);
#4790=CIRCLE('',#26122,70.);
#4791=CIRCLE('',#26124,70.);
#4792=CIRCLE('',#26125,70.);
#4793=CIRCLE('',#26127,70.);
#4794=CIRCLE('',#26128,70.);
#4795=CIRCLE('',#26130,70.);
#4796=CIRCLE('',#26131,70.);
#4797=CIRCLE('',#26133,70.);
#4798=CIRCLE('',#26134,70.);
#4799=CIRCLE('',#26136,70.);
#4800=CIRCLE('',#26137,70.);
#4801=CIRCLE('',#26139,70.);
#4802=CIRCLE('',#26140,70.);
#4803=CIRCLE('',#26142,70.);
#4804=CIRCLE('',#26143,70.);
#4805=CIRCLE('',#26145,70.);
#4806=CIRCLE('',#26146,70.);
#4807=CIRCLE('',#26148,70.);
#4808=CIRCLE('',#26149,70.);
#4809=CIRCLE('',#26151,70.);
#4810=CIRCLE('',#26152,70.);
#4811=CIRCLE('',#26154,70.);
#4812=CIRCLE('',#26155,70.);
#4813=CIRCLE('',#26157,70.);
#4814=CIRCLE('',#26158,70.);
#4815=CIRCLE('',#26160,70.);
#4816=CIRCLE('',#26161,70.);
#4817=CIRCLE('',#26163,70.);
#4818=CIRCLE('',#26164,70.);
#4819=CIRCLE('',#26166,70.);
#4820=CIRCLE('',#26167,70.);
#4821=CIRCLE('',#26169,70.);
#4822=CIRCLE('',#26170,70.);
#4823=CIRCLE('',#26172,70.);
#4824=CIRCLE('',#26173,70.);
#4825=CIRCLE('',#26175,70.);
#4826=CIRCLE('',#26176,70.);
#4827=CIRCLE('',#26178,70.);
#4828=CIRCLE('',#26179,70.);
#4829=CIRCLE('',#26181,70.);
#4830=CIRCLE('',#26182,70.);
#4831=CIRCLE('',#26184,70.);
#4832=CIRCLE('',#26185,70.);
#4833=CIRCLE('',#26187,70.);
#4834=CIRCLE('',#26188,70.);
#4835=CIRCLE('',#26190,70.);
#4836=CIRCLE('',#26191,70.);
#4837=CIRCLE('',#26193,70.);
#4838=CIRCLE('',#26194,70.);
#4839=CIRCLE('',#26196,70.);
#4840=CIRCLE('',#26197,70.);
#4841=CIRCLE('',#26199,70.);
#4842=CIRCLE('',#26200,70.);
#4843=CIRCLE('',#26202,70.);
#4844=CIRCLE('',#26203,70.);
#4845=CIRCLE('',#26205,70.);
#4846=CIRCLE('',#26206,70.);
#4847=CIRCLE('',#26208,70.);
#4848=CIRCLE('',#26209,70.);
#4849=CIRCLE('',#26211,70.);
#4850=CIRCLE('',#26212,70.);
#4851=CIRCLE('',#26214,70.);
#4852=CIRCLE('',#26215,70.);
#4853=CIRCLE('',#26217,70.);
#4854=CIRCLE('',#26218,70.);
#4855=CIRCLE('',#26220,70.);
#4856=CIRCLE('',#26221,70.);
#4857=CIRCLE('',#26223,70.);
#4858=CIRCLE('',#26224,70.);
#4859=CIRCLE('',#26226,70.);
#4860=CIRCLE('',#26227,70.);
#4861=CIRCLE('',#26229,70.);
#4862=CIRCLE('',#26230,70.);
#4863=CIRCLE('',#26232,70.);
#4864=CIRCLE('',#26233,70.);
#4865=CIRCLE('',#26235,70.);
#4866=CIRCLE('',#26236,70.);
#4867=CIRCLE('',#26238,70.);
#4868=CIRCLE('',#26239,70.);
#4869=CIRCLE('',#26241,70.);
#4870=CIRCLE('',#26242,70.);
#4871=CIRCLE('',#26244,70.);
#4872=CIRCLE('',#26245,70.);
#4873=CIRCLE('',#26247,70.);
#4874=CIRCLE('',#26248,70.);
#4875=CIRCLE('',#26250,70.);
#4876=CIRCLE('',#26251,70.);
#4877=CIRCLE('',#26253,70.);
#4878=CIRCLE('',#26254,70.);
#4879=CIRCLE('',#26256,70.);
#4880=CIRCLE('',#26257,70.);
#4881=CIRCLE('',#26259,70.);
#4882=CIRCLE('',#26260,70.);
#4883=CIRCLE('',#26262,70.);
#4884=CIRCLE('',#26263,70.);
#4885=CIRCLE('',#26265,70.);
#4886=CIRCLE('',#26266,70.);
#4887=CIRCLE('',#26268,70.);
#4888=CIRCLE('',#26269,70.);
#4889=CIRCLE('',#26271,70.);
#4890=CIRCLE('',#26272,70.);
#4891=CIRCLE('',#26274,70.);
#4892=CIRCLE('',#26275,70.);
#4893=CIRCLE('',#26277,70.);
#4894=CIRCLE('',#26278,70.);
#4895=CIRCLE('',#26280,70.);
#4896=CIRCLE('',#26281,70.);
#4897=CIRCLE('',#26283,70.);
#4898=CIRCLE('',#26284,70.);
#4899=CIRCLE('',#26286,70.);
#4900=CIRCLE('',#26287,70.);
#4901=CIRCLE('',#26289,70.);
#4902=CIRCLE('',#26290,70.);
#4903=CIRCLE('',#26292,70.);
#4904=CIRCLE('',#26293,70.);
#4905=CIRCLE('',#26295,70.);
#4906=CIRCLE('',#26296,70.);
#4907=CIRCLE('',#26298,70.);
#4908=CIRCLE('',#26299,70.);
#4909=CIRCLE('',#26301,70.);
#4910=CIRCLE('',#26302,70.);
#4911=CIRCLE('',#26304,74.4999999996252);
#4912=CIRCLE('',#26305,74.4999999996252);
#4913=CIRCLE('',#26307,90.);
#4914=CIRCLE('',#26308,70.);
#4915=CIRCLE('',#26310,70.);
#4916=CIRCLE('',#26312,90.);
#5993=B_SPLINE_CURVE_WITH_KNOTS('',3,(#52399,#52400,#52401,#52402,#52403,
#52404,#52405,#52406,#52407,#52408,#52409,#52410,#52411,#52412,#52413,#52414,
#52415,#52416),.UNSPECIFIED.,.F.,.F.,(4,2,2,2,2,2,2,2,4),(0.301359994903926,
0.376699993319996,0.452039991736066,0.527379990771959,0.602719989807853,
0.678059988843746,0.753399987879639,0.828739986295709,0.904079984711779),
 .UNSPECIFIED.);
#5994=B_SPLINE_CURVE_WITH_KNOTS('',3,(#52420,#52421,#52422,#52423,#52424,
#52425,#52426,#52427,#52428,#52429,#52430,#52431,#52432,#52433,#52434,#52435,
#52436,#52437,#52438),.UNSPECIFIED.,.F.,.F.,(4,2,2,2,3,2,2,2,4),(0.904079984711779,
0.979419983127849,1.05475998154392,1.13009998057981,1.20543997961571,1.2807799786516,
1.35611997768749,1.43145997610356,1.50679997451963),.UNSPECIFIED.);
#5995=B_SPLINE_CURVE_WITH_KNOTS('',3,(#52443,#52444,#52445,#52446,#52447,
#52448,#52449,#52450,#52451,#52452,#52453,#52454,#52455,#52456,#52457,#52458,
#52459,#52460),.UNSPECIFIED.,.F.,.F.,(4,2,2,2,2,2,2,2,4),(0.301359994903926,
0.376699993319996,0.452039991736066,0.527379990771959,0.602719989807853,
0.678059988843746,0.753399987879639,0.828739986295709,0.904079984711779),
 .UNSPECIFIED.);
#5996=B_SPLINE_CURVE_WITH_KNOTS('',3,(#52461,#52462,#52463,#52464,#52465,
#52466,#52467,#52468,#52469,#52470,#52471,#52472,#52473,#52474,#52475,#52476,
#52477,#52478,#52479),.UNSPECIFIED.,.F.,.F.,(4,2,2,2,3,2,2,2,4),(0.904079984711779,
0.979419983127849,1.05475998154392,1.13009998057981,1.20543997961571,1.2807799786516,
1.35611997768749,1.43145997610356,1.50679997451963),.UNSPECIFIED.);
#5997=B_SPLINE_CURVE_WITH_KNOTS('',3,(#52487,#52488,#52489,#52490,#52491,
#52492,#52493,#52494,#52495,#52496,#52497,#52498,#52499,#52500,#52501,#52502,
#52503,#52504),.UNSPECIFIED.,.F.,.F.,(4,2,2,2,2,2,2,2,4),(0.301359994903926,
0.376699993319996,0.452039991736066,0.527379990771959,0.602719989807853,
0.678059988843746,0.753399987879639,0.828739986295709,0.904079984711779),
 .UNSPECIFIED.);
#5998=B_SPLINE_CURVE_WITH_KNOTS('',3,(#52506,#52507,#52508,#52509,#52510,
#52511,#52512,#52513,#52514,#52515),.UNSPECIFIED.,.F.,.F.,(4,2,2,2,4),(1.20543997961571,
1.2807799786516,1.35611997768749,1.43145997610356,1.50679997451963),
 .UNSPECIFIED.);
#5999=B_SPLINE_CURVE_WITH_KNOTS('',3,(#52519,#52520,#52521,#52522,#52523,
#52524,#52525,#52526,#52527,#52528),.UNSPECIFIED.,.F.,.F.,(4,2,2,2,4),(0.904079984711779,
0.979419983127849,1.05475998154392,1.13009998057981,1.20543997961571),
 .UNSPECIFIED.);
#6000=B_SPLINE_CURVE_WITH_KNOTS('',3,(#52533,#52534,#52535,#52536,#52537,
#52538,#52539,#52540,#52541,#52542,#52543,#52544,#52545,#52546,#52547,#52548,
#52549,#52550),.UNSPECIFIED.,.F.,.F.,(4,2,2,2,2,2,2,2,4),(0.301359994903926,
0.376699993319996,0.452039991736066,0.527379990771959,0.602719989807853,
0.678059988843746,0.753399987879639,0.828739986295709,0.904079984711779),
 .UNSPECIFIED.);
#6001=B_SPLINE_CURVE_WITH_KNOTS('',3,(#52552,#52553,#52554,#52555,#52556,
#52557,#52558,#52559,#52560,#52561),.UNSPECIFIED.,.F.,.F.,(4,2,2,2,4),(1.20543997961571,
1.2807799786516,1.35611997768749,1.43145997610356,1.50679997451963),
 .UNSPECIFIED.);
#6002=B_SPLINE_CURVE_WITH_KNOTS('',3,(#52565,#52566,#52567,#52568,#52569,
#52570,#52571,#52572,#52573,#52574),.UNSPECIFIED.,.F.,.F.,(4,2,2,2,4),(0.904079984711779,
0.979419983127849,1.05475998154392,1.13009998057981,1.20543997961571),
 .UNSPECIFIED.);
#6003=B_SPLINE_CURVE_WITH_KNOTS('',3,(#52598,#52599,#52600,#52601,#52602,
#52603,#52604),.UNSPECIFIED.,.F.,.F.,(4,3,4),(0.,0.0330660780484128,0.0578656365847224),
 .UNSPECIFIED.);
#6004=B_SPLINE_CURVE_WITH_KNOTS('',3,(#52606,#52607,#52608,#52609),
 .UNSPECIFIED.,.F.,.F.,(4,4),(-2.77555756156289E-17,1.2),.UNSPECIFIED.);
#6005=B_SPLINE_CURVE_WITH_KNOTS('',3,(#52611,#52612,#52613,#52614,#52615,
#52616,#52617),.UNSPECIFIED.,.F.,.F.,(4,3,4),(0.,0.0247995585363078,0.0578656365847182),
 .UNSPECIFIED.);
#6006=B_SPLINE_CURVE_WITH_KNOTS('',3,(#52618,#52619,#52620,#52621),
 .UNSPECIFIED.,.F.,.F.,(4,4),(-1.2,2.77555756156289E-17),.UNSPECIFIED.);
#6007=B_SPLINE_CURVE_WITH_KNOTS('',3,(#53445,#53446,#53447,#53448,#53449,
#53450,#53451),.UNSPECIFIED.,.F.,.F.,(4,3,4),(0.,0.033066078045883,0.0578656365802953),
 .UNSPECIFIED.);
#6008=B_SPLINE_CURVE_WITH_KNOTS('',3,(#53453,#53454,#53455,#53456),
 .UNSPECIFIED.,.F.,.F.,(4,4),(0.,1.2),.UNSPECIFIED.);
#6009=B_SPLINE_CURVE_WITH_KNOTS('',3,(#53458,#53459,#53460,#53461,#53462,
#53463,#53464),.UNSPECIFIED.,.F.,.F.,(4,3,4),(0.,0.0247995585344089,0.0578656365802874),
 .UNSPECIFIED.);
#6010=B_SPLINE_CURVE_WITH_KNOTS('',3,(#53465,#53466,#53467,#53468),
 .UNSPECIFIED.,.F.,.F.,(4,4),(-1.2,0.),.UNSPECIFIED.);
#6011=B_SPLINE_CURVE_WITH_KNOTS('',3,(#53494,#53495,#53496,#53497,#53498,
#53499,#53500),.UNSPECIFIED.,.F.,.F.,(4,3,4),(0.,0.033066078048414,0.0578656365847245),
 .UNSPECIFIED.);
#6012=B_SPLINE_CURVE_WITH_KNOTS('',3,(#53502,#53503,#53504,#53505),
 .UNSPECIFIED.,.F.,.F.,(4,4),(9.71445146547012E-17,1.2),.UNSPECIFIED.);
#6013=B_SPLINE_CURVE_WITH_KNOTS('',3,(#53507,#53508,#53509,#53510,#53511,
#53512,#53513),.UNSPECIFIED.,.F.,.F.,(4,3,4),(0.,0.02479955853631,0.0578656365847234),
 .UNSPECIFIED.);
#6014=B_SPLINE_CURVE_WITH_KNOTS('',3,(#53514,#53515,#53516,#53517),
 .UNSPECIFIED.,.F.,.F.,(4,4),(-1.2,-9.71445146547012E-17),.UNSPECIFIED.);
#6015=B_SPLINE_CURVE_WITH_KNOTS('',3,(#54341,#54342,#54343,#54344,#54345,
#54346,#54347),.UNSPECIFIED.,.F.,.F.,(4,3,4),(0.,0.033066078045845,0.0578656365802287),
 .UNSPECIFIED.);
#6016=B_SPLINE_CURVE_WITH_KNOTS('',3,(#54349,#54350,#54351,#54352),
 .UNSPECIFIED.,.F.,.F.,(4,4),(-6.97125684381022E-36,1.2),.UNSPECIFIED.);
#6017=B_SPLINE_CURVE_WITH_KNOTS('',3,(#54354,#54355,#54356,#54357,#54358,
#54359,#54360),.UNSPECIFIED.,.F.,.F.,(4,3,4),(0.,0.0247995585343863,0.0578656365802347),
 .UNSPECIFIED.);
#6018=B_SPLINE_CURVE_WITH_KNOTS('',3,(#54361,#54362,#54363,#54364),
 .UNSPECIFIED.,.F.,.F.,(4,4),(-1.2,6.97125684381022E-36),.UNSPECIFIED.);
#6019=B_SPLINE_CURVE_WITH_KNOTS('',3,(#54390,#54391,#54392,#54393,#54394,
#54395,#54396),.UNSPECIFIED.,.F.,.F.,(4,3,4),(0.,0.0330660780483976,0.0578656365846959),
 .UNSPECIFIED.);
#6020=B_SPLINE_CURVE_WITH_KNOTS('',3,(#54398,#54399,#54400,#54401),
 .UNSPECIFIED.,.F.,.F.,(4,4),(4.06042677328019E-17,1.2),.UNSPECIFIED.);
#6021=B_SPLINE_CURVE_WITH_KNOTS('',3,(#54403,#54404,#54405,#54406,#54407,
#54408,#54409),.UNSPECIFIED.,.F.,.F.,(4,3,4),(0.,0.0247995585363066,0.0578656365847153),
 .UNSPECIFIED.);
#6022=B_SPLINE_CURVE_WITH_KNOTS('',3,(#54410,#54411,#54412,#54413),
 .UNSPECIFIED.,.F.,.F.,(4,4),(-1.2,-4.06042677328019E-17),.UNSPECIFIED.);
#6023=B_SPLINE_CURVE_WITH_KNOTS('',3,(#55237,#55238,#55239,#55240,#55241,
#55242,#55243),.UNSPECIFIED.,.F.,.F.,(4,3,4),(0.,0.0330660780458488,0.0578656365802353),
 .UNSPECIFIED.);
#6024=B_SPLINE_CURVE_WITH_KNOTS('',3,(#55245,#55246,#55247,#55248),
 .UNSPECIFIED.,.F.,.F.,(4,4),(-8.32667268468868E-17,1.2),.UNSPECIFIED.);
#6025=B_SPLINE_CURVE_WITH_KNOTS('',3,(#55250,#55251,#55252,#55253,#55254,
#55255,#55256),.UNSPECIFIED.,.F.,.F.,(4,3,4),(0.,0.0247995585343919,0.0578656365802478),
 .UNSPECIFIED.);
#6026=B_SPLINE_CURVE_WITH_KNOTS('',3,(#55257,#55258,#55259,#55260),
 .UNSPECIFIED.,.F.,.F.,(4,4),(-1.2,8.32667268468868E-17),.UNSPECIFIED.);
#6027=B_SPLINE_CURVE_WITH_KNOTS('',3,(#55286,#55287,#55288,#55289,#55290,
#55291,#55292),.UNSPECIFIED.,.F.,.F.,(4,3,4),(0.,0.0330660780484025,0.0578656365847044),
 .UNSPECIFIED.);
#6028=B_SPLINE_CURVE_WITH_KNOTS('',3,(#55294,#55295,#55296,#55297),
 .UNSPECIFIED.,.F.,.F.,(4,4),(9.71445146547012E-17,1.2),.UNSPECIFIED.);
#6029=B_SPLINE_CURVE_WITH_KNOTS('',3,(#55299,#55300,#55301,#55302,#55303,
#55304,#55305),.UNSPECIFIED.,.F.,.F.,(4,3,4),(0.,0.024799558536305,0.0578656365847116),
 .UNSPECIFIED.);
#6030=B_SPLINE_CURVE_WITH_KNOTS('',3,(#55306,#55307,#55308,#55309),
 .UNSPECIFIED.,.F.,.F.,(4,4),(-1.2,-9.71445146547012E-17),.UNSPECIFIED.);
#6031=B_SPLINE_CURVE_WITH_KNOTS('',3,(#56133,#56134,#56135,#56136,#56137,
#56138,#56139),.UNSPECIFIED.,.F.,.F.,(4,3,4),(0.,0.0330660780458838,0.0578656365802966),
 .UNSPECIFIED.);
#6032=B_SPLINE_CURVE_WITH_KNOTS('',3,(#56141,#56142,#56143,#56144),
 .UNSPECIFIED.,.F.,.F.,(4,4),(2.77555756156289E-17,1.2),.UNSPECIFIED.);
#6033=B_SPLINE_CURVE_WITH_KNOTS('',3,(#56146,#56147,#56148,#56149,#56150,
#56151,#56152),.UNSPECIFIED.,.F.,.F.,(4,3,4),(0.,0.024799558534413,0.0578656365802969),
 .UNSPECIFIED.);
#6034=B_SPLINE_CURVE_WITH_KNOTS('',3,(#56153,#56154,#56155,#56156),
 .UNSPECIFIED.,.F.,.F.,(4,4),(-1.2,-2.77555756156289E-17),.UNSPECIFIED.);
#6035=B_SPLINE_CURVE_WITH_KNOTS('',3,(#56182,#56183,#56184,#56185,#56186,
#56187,#56188),.UNSPECIFIED.,.F.,.F.,(4,3,4),(0.,0.0330660780484225,0.0578656365847394),
 .UNSPECIFIED.);
#6036=B_SPLINE_CURVE_WITH_KNOTS('',3,(#56190,#56191,#56192,#56193),
 .UNSPECIFIED.,.F.,.F.,(4,4),(1.66533453693773E-16,1.2),.UNSPECIFIED.);
#6037=B_SPLINE_CURVE_WITH_KNOTS('',3,(#56195,#56196,#56197,#56198,#56199,
#56200,#56201),.UNSPECIFIED.,.F.,.F.,(4,3,4),(0.,0.0247995585363181,0.0578656365847422),
 .UNSPECIFIED.);
#6038=B_SPLINE_CURVE_WITH_KNOTS('',3,(#56202,#56203,#56204,#56205),
 .UNSPECIFIED.,.F.,.F.,(4,4),(-1.2,-1.66533453693773E-16),.UNSPECIFIED.);
#6039=B_SPLINE_CURVE_WITH_KNOTS('',3,(#57029,#57030,#57031,#57032,#57033,
#57034,#57035),.UNSPECIFIED.,.F.,.F.,(4,3,4),(0.,0.0330660780459141,0.0578656365803497),
 .UNSPECIFIED.);
#6040=B_SPLINE_CURVE_WITH_KNOTS('',3,(#57037,#57038,#57039,#57040),
 .UNSPECIFIED.,.F.,.F.,(4,4),(-4.16333634234434E-17,1.2),.UNSPECIFIED.);
#6041=B_SPLINE_CURVE_WITH_KNOTS('',3,(#57042,#57043,#57044,#57045,#57046,
#57047,#57048),.UNSPECIFIED.,.F.,.F.,(4,3,4),(0.,0.0247995585344146,0.0578656365803007),
 .UNSPECIFIED.);
#6042=B_SPLINE_CURVE_WITH_KNOTS('',3,(#57049,#57050,#57051,#57052),
 .UNSPECIFIED.,.F.,.F.,(4,4),(-1.2,4.16333634234434E-17),.UNSPECIFIED.);
#6043=B_SPLINE_CURVE_WITH_KNOTS('',3,(#57078,#57079,#57080,#57081,#57082,
#57083,#57084),.UNSPECIFIED.,.F.,.F.,(4,3,4),(0.,0.0330660780484257,0.057865636584745),
 .UNSPECIFIED.);
#6044=B_SPLINE_CURVE_WITH_KNOTS('',3,(#57086,#57087,#57088,#57089),
 .UNSPECIFIED.,.F.,.F.,(4,4),(1.38777878078145E-16,1.2),.UNSPECIFIED.);
#6045=B_SPLINE_CURVE_WITH_KNOTS('',3,(#57091,#57092,#57093,#57094,#57095,
#57096,#57097),.UNSPECIFIED.,.F.,.F.,(4,3,4),(0.,0.0247995585363191,0.0578656365847445),
 .UNSPECIFIED.);
#6046=B_SPLINE_CURVE_WITH_KNOTS('',3,(#57098,#57099,#57100,#57101),
 .UNSPECIFIED.,.F.,.F.,(4,4),(-1.2,-1.38777878078145E-16),.UNSPECIFIED.);
#6047=B_SPLINE_CURVE_WITH_KNOTS('',3,(#57925,#57926,#57927,#57928,#57929,
#57930,#57931),.UNSPECIFIED.,.F.,.F.,(4,3,4),(0.,0.0330660780458979,0.0578656365803213),
 .UNSPECIFIED.);
#6048=B_SPLINE_CURVE_WITH_KNOTS('',3,(#57933,#57934,#57935,#57936),
 .UNSPECIFIED.,.F.,.F.,(4,4),(-8.43563892506861E-17,1.2),.UNSPECIFIED.);
#6049=B_SPLINE_CURVE_WITH_KNOTS('',3,(#57938,#57939,#57940,#57941,#57942,
#57943,#57944),.UNSPECIFIED.,.F.,.F.,(4,3,4),(0.,0.0247995585344144,0.0578656365803003),
 .UNSPECIFIED.);
#6050=B_SPLINE_CURVE_WITH_KNOTS('',3,(#57945,#57946,#57947,#57948),
 .UNSPECIFIED.,.F.,.F.,(4,4),(-1.2,8.43563892506861E-17),.UNSPECIFIED.);
#6051=B_SPLINE_CURVE_WITH_KNOTS('',3,(#57974,#57975,#57976,#57977,#57978,
#57979,#57980),.UNSPECIFIED.,.F.,.F.,(4,3,4),(0.,0.0330660780484328,0.0578656365847574),
 .UNSPECIFIED.);
#6052=B_SPLINE_CURVE_WITH_KNOTS('',3,(#57982,#57983,#57984,#57985),
 .UNSPECIFIED.,.F.,.F.,(4,4),(1.66533453693773E-16,1.2),.UNSPECIFIED.);
#6053=B_SPLINE_CURVE_WITH_KNOTS('',3,(#57987,#57988,#57989,#57990,#57991,
#57992,#57993),.UNSPECIFIED.,.F.,.F.,(4,3,4),(0.,0.0247995585363196,0.0578656365847458),
 .UNSPECIFIED.);
#6054=B_SPLINE_CURVE_WITH_KNOTS('',3,(#57994,#57995,#57996,#57997),
 .UNSPECIFIED.,.F.,.F.,(4,4),(-1.2,-1.66533453693773E-16),.UNSPECIFIED.);
#6055=B_SPLINE_CURVE_WITH_KNOTS('',3,(#58821,#58822,#58823,#58824,#58825,
#58826,#58827),.UNSPECIFIED.,.F.,.F.,(4,3,4),(0.,0.0330660780458605,0.0578656365802559),
 .UNSPECIFIED.);
#6056=B_SPLINE_CURVE_WITH_KNOTS('',3,(#58829,#58830,#58831,#58832),
 .UNSPECIFIED.,.F.,.F.,(4,4),(2.77555756156289E-17,1.2),.UNSPECIFIED.);
#6057=B_SPLINE_CURVE_WITH_KNOTS('',3,(#58834,#58835,#58836,#58837,#58838,
#58839,#58840),.UNSPECIFIED.,.F.,.F.,(4,3,4),(0.,0.0247995585344011,0.0578656365802693),
 .UNSPECIFIED.);
#6058=B_SPLINE_CURVE_WITH_KNOTS('',3,(#58841,#58842,#58843,#58844),
 .UNSPECIFIED.,.F.,.F.,(4,4),(-1.2,-2.77555756156289E-17),.UNSPECIFIED.);
#6059=B_SPLINE_CURVE_WITH_KNOTS('',3,(#58870,#58871,#58872,#58873,#58874,
#58875,#58876),.UNSPECIFIED.,.F.,.F.,(4,3,4),(0.,0.0330660780484201,0.0578656365847351),
 .UNSPECIFIED.);
#6060=B_SPLINE_CURVE_WITH_KNOTS('',3,(#58878,#58879,#58880,#58881),
 .UNSPECIFIED.,.F.,.F.,(4,4),(-8.32667268468868E-17,1.2),.UNSPECIFIED.);
#6061=B_SPLINE_CURVE_WITH_KNOTS('',3,(#58883,#58884,#58885,#58886,#58887,
#58888,#58889),.UNSPECIFIED.,.F.,.F.,(4,3,4),(0.,0.0247995585363181,0.0578656365847421),
 .UNSPECIFIED.);
#6062=B_SPLINE_CURVE_WITH_KNOTS('',3,(#58890,#58891,#58892,#58893),
 .UNSPECIFIED.,.F.,.F.,(4,4),(-1.2,8.32667268468868E-17),.UNSPECIFIED.);
#6063=B_SPLINE_CURVE_WITH_KNOTS('',3,(#59717,#59718,#59719,#59720,#59721,
#59722,#59723),.UNSPECIFIED.,.F.,.F.,(4,3,4),(0.,0.0330660780458621,0.0578656365802586),
 .UNSPECIFIED.);
#6064=B_SPLINE_CURVE_WITH_KNOTS('',3,(#59725,#59726,#59727,#59728),
 .UNSPECIFIED.,.F.,.F.,(4,4),(5.55111512312578E-17,1.2),.UNSPECIFIED.);
#6065=B_SPLINE_CURVE_WITH_KNOTS('',3,(#59730,#59731,#59732,#59733,#59734,
#59735,#59736),.UNSPECIFIED.,.F.,.F.,(4,3,4),(0.,0.0247995585343903,0.057865636580244),
 .UNSPECIFIED.);
#6066=B_SPLINE_CURVE_WITH_KNOTS('',3,(#59737,#59738,#59739,#59740),
 .UNSPECIFIED.,.F.,.F.,(4,4),(-1.2,-5.55111512312578E-17),.UNSPECIFIED.);
#6067=B_SPLINE_CURVE_WITH_KNOTS('',3,(#59766,#59767,#59768,#59769,#59770,
#59771,#59772),.UNSPECIFIED.,.F.,.F.,(4,3,4),(0.,0.03306607804842,0.057865636584735),
 .UNSPECIFIED.);
#6068=B_SPLINE_CURVE_WITH_KNOTS('',3,(#59774,#59775,#59776,#59777),
 .UNSPECIFIED.,.F.,.F.,(4,4),(1.66533453693773E-16,1.2),.UNSPECIFIED.);
#6069=B_SPLINE_CURVE_WITH_KNOTS('',3,(#59779,#59780,#59781,#59782,#59783,
#59784,#59785),.UNSPECIFIED.,.F.,.F.,(4,3,4),(0.,0.0247995585363173,0.0578656365847403),
 .UNSPECIFIED.);
#6070=B_SPLINE_CURVE_WITH_KNOTS('',3,(#59786,#59787,#59788,#59789),
 .UNSPECIFIED.,.F.,.F.,(4,4),(-1.2,-1.66533453693773E-16),.UNSPECIFIED.);
#6071=B_SPLINE_CURVE_WITH_KNOTS('',3,(#60613,#60614,#60615,#60616,#60617,
#60618,#60619),.UNSPECIFIED.,.F.,.F.,(4,3,4),(0.,0.0330660780458358,0.0578656365802127),
 .UNSPECIFIED.);
#6072=B_SPLINE_CURVE_WITH_KNOTS('',3,(#60621,#60622,#60623,#60624),
 .UNSPECIFIED.,.F.,.F.,(4,4),(-8.9628248557339E-17,1.2),.UNSPECIFIED.);
#6073=B_SPLINE_CURVE_WITH_KNOTS('',3,(#60626,#60627,#60628,#60629,#60630,
#60631,#60632),.UNSPECIFIED.,.F.,.F.,(4,3,4),(0.,0.0247995585343798,0.0578656365802194),
 .UNSPECIFIED.);
#6074=B_SPLINE_CURVE_WITH_KNOTS('',3,(#60633,#60634,#60635,#60636),
 .UNSPECIFIED.,.F.,.F.,(4,4),(-1.2,8.9628248557339E-17),.UNSPECIFIED.);
#6075=B_SPLINE_CURVE_WITH_KNOTS('',3,(#60662,#60663,#60664,#60665,#60666,
#60667,#60668),.UNSPECIFIED.,.F.,.F.,(4,3,4),(0.,0.0330660780483891,0.057865636584681),
 .UNSPECIFIED.);
#6076=B_SPLINE_CURVE_WITH_KNOTS('',3,(#60670,#60671,#60672,#60673),
 .UNSPECIFIED.,.F.,.F.,(4,4),(8.0522471671843E-17,1.2),.UNSPECIFIED.);
#6077=B_SPLINE_CURVE_WITH_KNOTS('',3,(#60675,#60676,#60677,#60678,#60679,
#60680,#60681),.UNSPECIFIED.,.F.,.F.,(4,3,4),(0.,0.024799558536297,0.0578656365846929),
 .UNSPECIFIED.);
#6078=B_SPLINE_CURVE_WITH_KNOTS('',3,(#60682,#60683,#60684,#60685),
 .UNSPECIFIED.,.F.,.F.,(4,4),(-1.2,-8.0522471671843E-17),.UNSPECIFIED.);
#6079=B_SPLINE_CURVE_WITH_KNOTS('',3,(#61509,#61510,#61511,#61512,#61513,
#61514,#61515),.UNSPECIFIED.,.F.,.F.,(4,3,4),(0.,0.033066078045854,0.0578656365802446),
 .UNSPECIFIED.);
#6080=B_SPLINE_CURVE_WITH_KNOTS('',3,(#61517,#61518,#61519,#61520),
 .UNSPECIFIED.,.F.,.F.,(4,4),(-7.52391395153922E-36,1.2),.UNSPECIFIED.);
#6081=B_SPLINE_CURVE_WITH_KNOTS('',3,(#61522,#61523,#61524,#61525,#61526,
#61527,#61528),.UNSPECIFIED.,.F.,.F.,(4,3,4),(0.,0.0247995585343871,0.0578656365802365),
 .UNSPECIFIED.);
#6082=B_SPLINE_CURVE_WITH_KNOTS('',3,(#61529,#61530,#61531,#61532),
 .UNSPECIFIED.,.F.,.F.,(4,4),(-1.2,7.52391395153922E-36),.UNSPECIFIED.);
#6083=B_SPLINE_CURVE_WITH_KNOTS('',3,(#61558,#61559,#61560,#61561,#61562,
#61563,#61564),.UNSPECIFIED.,.F.,.F.,(4,3,4),(0.,0.0330660780484426,0.0578656365847746),
 .UNSPECIFIED.);
#6084=B_SPLINE_CURVE_WITH_KNOTS('',3,(#61566,#61567,#61568,#61569),
 .UNSPECIFIED.,.F.,.F.,(4,4),(9.71445146547012E-17,1.2),.UNSPECIFIED.);
#6085=B_SPLINE_CURVE_WITH_KNOTS('',3,(#61571,#61572,#61573,#61574,#61575,
#61576,#61577),.UNSPECIFIED.,.F.,.F.,(4,3,4),(0.,0.0247995585363433,0.0578656365848011),
 .UNSPECIFIED.);
#6086=B_SPLINE_CURVE_WITH_KNOTS('',3,(#61578,#61579,#61580,#61581),
 .UNSPECIFIED.,.F.,.F.,(4,4),(-1.2,-9.71445146547012E-17),.UNSPECIFIED.);
#6087=B_SPLINE_CURVE_WITH_KNOTS('',3,(#62405,#62406,#62407,#62408,#62409,
#62410,#62411),.UNSPECIFIED.,.F.,.F.,(4,3,4),(0.,0.0330660780458487,0.0578656365802352),
 .UNSPECIFIED.);
#6088=B_SPLINE_CURVE_WITH_KNOTS('',3,(#62413,#62414,#62415,#62416),
 .UNSPECIFIED.,.F.,.F.,(4,4),(2.77555756156289E-17,1.2),.UNSPECIFIED.);
#6089=B_SPLINE_CURVE_WITH_KNOTS('',3,(#62418,#62419,#62420,#62421,#62422,
#62423,#62424),.UNSPECIFIED.,.F.,.F.,(4,3,4),(0.,0.0247995585343886,0.05786563658024),
 .UNSPECIFIED.);
#6090=B_SPLINE_CURVE_WITH_KNOTS('',3,(#62425,#62426,#62427,#62428),
 .UNSPECIFIED.,.F.,.F.,(4,4),(-1.2,-2.77555756156289E-17),.UNSPECIFIED.);
#6091=B_SPLINE_CURVE_WITH_KNOTS('',3,(#62454,#62455,#62456,#62457,#62458,
#62459,#62460),.UNSPECIFIED.,.F.,.F.,(4,3,4),(0.,0.0330660780484585,0.0578656365848024),
 .UNSPECIFIED.);
#6092=B_SPLINE_CURVE_WITH_KNOTS('',3,(#62462,#62463,#62464,#62465),
 .UNSPECIFIED.,.F.,.F.,(4,4),(6.66446838640284E-17,1.2),.UNSPECIFIED.);
#6093=B_SPLINE_CURVE_WITH_KNOTS('',3,(#62467,#62468,#62469,#62470,#62471,
#62472,#62473),.UNSPECIFIED.,.F.,.F.,(4,3,4),(0.,0.0247995585363314,0.0578656365847732),
 .UNSPECIFIED.);
#6094=B_SPLINE_CURVE_WITH_KNOTS('',3,(#62474,#62475,#62476,#62477),
 .UNSPECIFIED.,.F.,.F.,(4,4),(-1.2,-6.66446838640284E-17),.UNSPECIFIED.);
#6095=B_SPLINE_CURVE_WITH_KNOTS('',3,(#63301,#63302,#63303,#63304,#63305,
#63306,#63307),.UNSPECIFIED.,.F.,.F.,(4,3,4),(0.,0.0330660780458707,0.0578656365802737),
 .UNSPECIFIED.);
#6096=B_SPLINE_CURVE_WITH_KNOTS('',3,(#63309,#63310,#63311,#63312),
 .UNSPECIFIED.,.F.,.F.,(4,4),(-4.16333634234434E-17,1.2),.UNSPECIFIED.);
#6097=B_SPLINE_CURVE_WITH_KNOTS('',3,(#63314,#63315,#63316,#63317,#63318,
#63319,#63320),.UNSPECIFIED.,.F.,.F.,(4,3,4),(0.,0.0247995585344061,0.057865636580281),
 .UNSPECIFIED.);
#6098=B_SPLINE_CURVE_WITH_KNOTS('',3,(#63321,#63322,#63323,#63324),
 .UNSPECIFIED.,.F.,.F.,(4,4),(-1.2,4.16333634234434E-17),.UNSPECIFIED.);
#6099=B_SPLINE_CURVE_WITH_KNOTS('',3,(#63350,#63351,#63352,#63353,#63354,
#63355,#63356),.UNSPECIFIED.,.F.,.F.,(4,3,4),(0.,0.0330660780484377,0.0578656365847659),
 .UNSPECIFIED.);
#6100=B_SPLINE_CURVE_WITH_KNOTS('',3,(#63358,#63359,#63360,#63361),
 .UNSPECIFIED.,.F.,.F.,(4,4),(0.,1.2),.UNSPECIFIED.);
#6101=B_SPLINE_CURVE_WITH_KNOTS('',3,(#63363,#63364,#63365,#63366,#63367,
#63368,#63369),.UNSPECIFIED.,.F.,.F.,(4,3,4),(0.,0.0247995585363214,0.0578656365847499),
 .UNSPECIFIED.);
#6102=B_SPLINE_CURVE_WITH_KNOTS('',3,(#63370,#63371,#63372,#63373),
 .UNSPECIFIED.,.F.,.F.,(4,4),(-1.2,0.),.UNSPECIFIED.);
#6103=B_SPLINE_CURVE_WITH_KNOTS('',3,(#64197,#64198,#64199,#64200,#64201,
#64202,#64203),.UNSPECIFIED.,.F.,.F.,(4,3,4),(0.,0.0330660780458375,0.0578656365802156),
 .UNSPECIFIED.);
#6104=B_SPLINE_CURVE_WITH_KNOTS('',3,(#64205,#64206,#64207,#64208),
 .UNSPECIFIED.,.F.,.F.,(4,4),(2.77555756156289E-17,1.2),.UNSPECIFIED.);
#6105=B_SPLINE_CURVE_WITH_KNOTS('',3,(#64210,#64211,#64212,#64213,#64214,
#64215,#64216),.UNSPECIFIED.,.F.,.F.,(4,3,4),(0.,0.0247995585344089,0.0578656365802873),
 .UNSPECIFIED.);
#6106=B_SPLINE_CURVE_WITH_KNOTS('',3,(#64217,#64218,#64219,#64220),
 .UNSPECIFIED.,.F.,.F.,(4,4),(-1.2,-2.77555756156289E-17),.UNSPECIFIED.);
#6107=B_SPLINE_CURVE_WITH_KNOTS('',3,(#64246,#64247,#64248,#64249,#64250,
#64251,#64252),.UNSPECIFIED.,.F.,.F.,(4,3,4),(0.,0.0330660780484158,0.0578656365847277),
 .UNSPECIFIED.);
#6108=B_SPLINE_CURVE_WITH_KNOTS('',3,(#64254,#64255,#64256,#64257),
 .UNSPECIFIED.,.F.,.F.,(4,4),(9.71445146547012E-17,1.2),.UNSPECIFIED.);
#6109=B_SPLINE_CURVE_WITH_KNOTS('',3,(#64259,#64260,#64261,#64262,#64263,
#64264,#64265),.UNSPECIFIED.,.F.,.F.,(4,3,4),(0.,0.024799558536314,0.0578656365847327),
 .UNSPECIFIED.);
#6110=B_SPLINE_CURVE_WITH_KNOTS('',3,(#64266,#64267,#64268,#64269),
 .UNSPECIFIED.,.F.,.F.,(4,4),(-1.2,-9.71445146547012E-17),.UNSPECIFIED.);
#6111=B_SPLINE_CURVE_WITH_KNOTS('',3,(#65093,#65094,#65095,#65096,#65097,
#65098,#65099),.UNSPECIFIED.,.F.,.F.,(4,3,4),(0.,0.0330660780458398,0.0578656365802196),
 .UNSPECIFIED.);
#6112=B_SPLINE_CURVE_WITH_KNOTS('',3,(#65101,#65102,#65103,#65104),
 .UNSPECIFIED.,.F.,.F.,(4,4),(-1.11022302462516E-16,1.2),.UNSPECIFIED.);
#6113=B_SPLINE_CURVE_WITH_KNOTS('',3,(#65106,#65107,#65108,#65109,#65110,
#65111,#65112),.UNSPECIFIED.,.F.,.F.,(4,3,4),(0.,0.0247995585343881,0.057865636580239),
 .UNSPECIFIED.);
#6114=B_SPLINE_CURVE_WITH_KNOTS('',3,(#65113,#65114,#65115,#65116),
 .UNSPECIFIED.,.F.,.F.,(4,4),(-1.2,1.11022302462516E-16),.UNSPECIFIED.);
#6115=B_SPLINE_CURVE_WITH_KNOTS('',3,(#65142,#65143,#65144,#65145,#65146,
#65147,#65148),.UNSPECIFIED.,.F.,.F.,(4,3,4),(0.,0.0330660780484092,0.0578656365847161),
 .UNSPECIFIED.);
#6116=B_SPLINE_CURVE_WITH_KNOTS('',3,(#65150,#65151,#65152,#65153),
 .UNSPECIFIED.,.F.,.F.,(4,4),(6.66446838640285E-17,1.2),.UNSPECIFIED.);
#6117=B_SPLINE_CURVE_WITH_KNOTS('',3,(#65155,#65156,#65157,#65158,#65159,
#65160,#65161),.UNSPECIFIED.,.F.,.F.,(4,3,4),(0.,0.0247995585363108,0.0578656365847252),
 .UNSPECIFIED.);
#6118=B_SPLINE_CURVE_WITH_KNOTS('',3,(#65162,#65163,#65164,#65165),
 .UNSPECIFIED.,.F.,.F.,(4,4),(-1.2,-6.66446838640285E-17),.UNSPECIFIED.);
#6119=B_SPLINE_CURVE_WITH_KNOTS('',3,(#65989,#65990,#65991,#65992,#65993,
#65994,#65995),.UNSPECIFIED.,.F.,.F.,(4,3,4),(0.,0.0330660780458506,0.0578656365802386),
 .UNSPECIFIED.);
#6120=B_SPLINE_CURVE_WITH_KNOTS('',3,(#65997,#65998,#65999,#66000),
 .UNSPECIFIED.,.F.,.F.,(4,4),(2.77555756156289E-17,1.2),.UNSPECIFIED.);
#6121=B_SPLINE_CURVE_WITH_KNOTS('',3,(#66002,#66003,#66004,#66005,#66006,
#66007,#66008),.UNSPECIFIED.,.F.,.F.,(4,3,4),(0.,0.024799558534388,0.0578656365802388),
 .UNSPECIFIED.);
#6122=B_SPLINE_CURVE_WITH_KNOTS('',3,(#66009,#66010,#66011,#66012),
 .UNSPECIFIED.,.F.,.F.,(4,4),(-1.2,-2.77555756156289E-17),.UNSPECIFIED.);
#6123=B_SPLINE_CURVE_WITH_KNOTS('',3,(#66038,#66039,#66040,#66041,#66042,
#66043,#66044),.UNSPECIFIED.,.F.,.F.,(4,3,4),(0.,0.0330660780484157,0.0578656365847274),
 .UNSPECIFIED.);
#6124=B_SPLINE_CURVE_WITH_KNOTS('',3,(#66046,#66047,#66048,#66049),
 .UNSPECIFIED.,.F.,.F.,(4,4),(6.93889390390723E-17,1.2),.UNSPECIFIED.);
#6125=B_SPLINE_CURVE_WITH_KNOTS('',3,(#66051,#66052,#66053,#66054,#66055,
#66056,#66057),.UNSPECIFIED.,.F.,.F.,(4,3,4),(0.,0.0247995585363113,0.0578656365847263),
 .UNSPECIFIED.);
#6126=B_SPLINE_CURVE_WITH_KNOTS('',3,(#66058,#66059,#66060,#66061),
 .UNSPECIFIED.,.F.,.F.,(4,4),(-1.2,-6.93889390390723E-17),.UNSPECIFIED.);
#6127=B_SPLINE_CURVE_WITH_KNOTS('',3,(#66885,#66886,#66887,#66888,#66889,
#66890,#66891),.UNSPECIFIED.,.F.,.F.,(4,3,4),(0.,0.0330660780458591,0.0578656365802535),
 .UNSPECIFIED.);
#6128=B_SPLINE_CURVE_WITH_KNOTS('',3,(#66893,#66894,#66895,#66896),
 .UNSPECIFIED.,.F.,.F.,(4,4),(0.,1.2),.UNSPECIFIED.);
#6129=B_SPLINE_CURVE_WITH_KNOTS('',3,(#66898,#66899,#66900,#66901,#66902,
#66903,#66904),.UNSPECIFIED.,.F.,.F.,(4,3,4),(0.,0.0247995585343995,0.0578656365802656),
 .UNSPECIFIED.);
#6130=B_SPLINE_CURVE_WITH_KNOTS('',3,(#66905,#66906,#66907,#66908),
 .UNSPECIFIED.,.F.,.F.,(4,4),(-1.2,0.),.UNSPECIFIED.);
#6131=B_SPLINE_CURVE_WITH_KNOTS('',3,(#66934,#66935,#66936,#66937,#66938,
#66939,#66940),.UNSPECIFIED.,.F.,.F.,(4,3,4),(0.,0.0330660780484159,0.0578656365847279),
 .UNSPECIFIED.);
#6132=B_SPLINE_CURVE_WITH_KNOTS('',3,(#66942,#66943,#66944,#66945),
 .UNSPECIFIED.,.F.,.F.,(4,4),(8.32667268468867E-17,1.2),.UNSPECIFIED.);
#6133=B_SPLINE_CURVE_WITH_KNOTS('',3,(#66947,#66948,#66949,#66950,#66951,
#66952,#66953),.UNSPECIFIED.,.F.,.F.,(4,3,4),(0.,0.0247995585363112,0.0578656365847262),
 .UNSPECIFIED.);
#6134=B_SPLINE_CURVE_WITH_KNOTS('',3,(#66954,#66955,#66956,#66957),
 .UNSPECIFIED.,.F.,.F.,(4,4),(-1.2,-8.32667268468867E-17),.UNSPECIFIED.);
#6135=B_SPLINE_CURVE_WITH_KNOTS('',3,(#67781,#67782,#67783,#67784,#67785,
#67786,#67787),.UNSPECIFIED.,.F.,.F.,(4,3,4),(0.,0.0330660780458738,0.0578656365802791),
 .UNSPECIFIED.);
#6136=B_SPLINE_CURVE_WITH_KNOTS('',3,(#67789,#67790,#67791,#67792),
 .UNSPECIFIED.,.F.,.F.,(4,4),(-5.55111512312578E-17,1.2),.UNSPECIFIED.);
#6137=B_SPLINE_CURVE_WITH_KNOTS('',3,(#67794,#67795,#67796,#67797,#67798,
#67799,#67800),.UNSPECIFIED.,.F.,.F.,(4,3,4),(0.,0.0247995585344049,0.0578656365802781),
 .UNSPECIFIED.);
#6138=B_SPLINE_CURVE_WITH_KNOTS('',3,(#67801,#67802,#67803,#67804),
 .UNSPECIFIED.,.F.,.F.,(4,4),(-1.2,5.55111512312578E-17),.UNSPECIFIED.);
#6139=B_SPLINE_CURVE_WITH_KNOTS('',3,(#67830,#67831,#67832,#67833,#67834,
#67835,#67836),.UNSPECIFIED.,.F.,.F.,(4,3,4),(0.,0.0330660780483935,0.0578656365846887),
 .UNSPECIFIED.);
#6140=B_SPLINE_CURVE_WITH_KNOTS('',3,(#67838,#67839,#67840,#67841),
 .UNSPECIFIED.,.F.,.F.,(4,4),(0.,1.2),.UNSPECIFIED.);
#6141=B_SPLINE_CURVE_WITH_KNOTS('',3,(#67843,#67844,#67845,#67846,#67847,
#67848,#67849),.UNSPECIFIED.,.F.,.F.,(4,3,4),(0.,0.0247995585363067,0.0578656365847155),
 .UNSPECIFIED.);
#6142=B_SPLINE_CURVE_WITH_KNOTS('',3,(#67850,#67851,#67852,#67853),
 .UNSPECIFIED.,.F.,.F.,(4,4),(-1.2,0.),.UNSPECIFIED.);
#6143=B_SPLINE_CURVE_WITH_KNOTS('',3,(#68677,#68678,#68679,#68680,#68681,
#68682,#68683),.UNSPECIFIED.,.F.,.F.,(4,3,4),(0.,0.0330660780458547,0.0578656365802457),
 .UNSPECIFIED.);
#6144=B_SPLINE_CURVE_WITH_KNOTS('',3,(#68685,#68686,#68687,#68688),
 .UNSPECIFIED.,.F.,.F.,(4,4),(-8.32667268468868E-17,1.2),.UNSPECIFIED.);
#6145=B_SPLINE_CURVE_WITH_KNOTS('',3,(#68690,#68691,#68692,#68693,#68694,
#68695,#68696),.UNSPECIFIED.,.F.,.F.,(4,3,4),(0.,0.0247995585343948,0.0578656365802546),
 .UNSPECIFIED.);
#6146=B_SPLINE_CURVE_WITH_KNOTS('',3,(#68697,#68698,#68699,#68700),
 .UNSPECIFIED.,.F.,.F.,(4,4),(-1.2,8.32667268468868E-17),.UNSPECIFIED.);
#6147=B_SPLINE_CURVE_WITH_KNOTS('',3,(#68726,#68727,#68728,#68729,#68730,
#68731,#68732),.UNSPECIFIED.,.F.,.F.,(4,3,4),(0.,0.0330660780484166,0.0578656365847291),
 .UNSPECIFIED.);
#6148=B_SPLINE_CURVE_WITH_KNOTS('',3,(#68734,#68735,#68736,#68737),
 .UNSPECIFIED.,.F.,.F.,(4,4),(9.71445146547012E-17,1.2),.UNSPECIFIED.);
#6149=B_SPLINE_CURVE_WITH_KNOTS('',3,(#68739,#68740,#68741,#68742,#68743,
#68744,#68745),.UNSPECIFIED.,.F.,.F.,(4,3,4),(0.,0.0247995585363142,0.0578656365847332),
 .UNSPECIFIED.);
#6150=B_SPLINE_CURVE_WITH_KNOTS('',3,(#68746,#68747,#68748,#68749),
 .UNSPECIFIED.,.F.,.F.,(4,4),(-1.2,-9.71445146547012E-17),.UNSPECIFIED.);
#6151=B_SPLINE_CURVE_WITH_KNOTS('',3,(#69573,#69574,#69575,#69576,#69577,
#69578,#69579),.UNSPECIFIED.,.F.,.F.,(4,3,4),(0.,0.0330660780458543,0.057865636580245),
 .UNSPECIFIED.);
#6152=B_SPLINE_CURVE_WITH_KNOTS('',3,(#69581,#69582,#69583,#69584),
 .UNSPECIFIED.,.F.,.F.,(4,4),(-2.74425517504386E-18,1.2),.UNSPECIFIED.);
#6153=B_SPLINE_CURVE_WITH_KNOTS('',3,(#69586,#69587,#69588,#69589,#69590,
#69591,#69592),.UNSPECIFIED.,.F.,.F.,(4,3,4),(0.,0.0247995585344,0.0578656365802666),
 .UNSPECIFIED.);
#6154=B_SPLINE_CURVE_WITH_KNOTS('',3,(#69593,#69594,#69595,#69596),
 .UNSPECIFIED.,.F.,.F.,(4,4),(-1.2,2.74425517504386E-18),.UNSPECIFIED.);
#6155=B_SPLINE_CURVE_WITH_KNOTS('',3,(#69622,#69623,#69624,#69625,#69626,
#69627,#69628),.UNSPECIFIED.,.F.,.F.,(4,3,4),(0.,0.033066078048411,0.0578656365847193),
 .UNSPECIFIED.);
#6156=B_SPLINE_CURVE_WITH_KNOTS('',3,(#69630,#69631,#69632,#69633),
 .UNSPECIFIED.,.F.,.F.,(4,4),(8.0522471671843E-17,1.2),.UNSPECIFIED.);
#6157=B_SPLINE_CURVE_WITH_KNOTS('',3,(#69635,#69636,#69637,#69638,#69639,
#69640,#69641),.UNSPECIFIED.,.F.,.F.,(4,3,4),(0.,0.0247995585363087,0.0578656365847204),
 .UNSPECIFIED.);
#6158=B_SPLINE_CURVE_WITH_KNOTS('',3,(#69642,#69643,#69644,#69645),
 .UNSPECIFIED.,.F.,.F.,(4,4),(-1.2,-8.0522471671843E-17),.UNSPECIFIED.);
#6159=B_SPLINE_CURVE_WITH_KNOTS('',3,(#70469,#70470,#70471,#70472,#70473,
#70474,#70475),.UNSPECIFIED.,.F.,.F.,(4,3,4),(0.,0.0330660780458236,0.0578656365801913),
 .UNSPECIFIED.);
#6160=B_SPLINE_CURVE_WITH_KNOTS('',3,(#70477,#70478,#70479,#70480),
 .UNSPECIFIED.,.F.,.F.,(4,4),(-1.38777878078145E-16,1.2),.UNSPECIFIED.);
#6161=B_SPLINE_CURVE_WITH_KNOTS('',3,(#70482,#70483,#70484,#70485,#70486,
#70487,#70488),.UNSPECIFIED.,.F.,.F.,(4,3,4),(0.,0.024799558534366,0.0578656365801874),
 .UNSPECIFIED.);
#6162=B_SPLINE_CURVE_WITH_KNOTS('',3,(#70489,#70490,#70491,#70492),
 .UNSPECIFIED.,.F.,.F.,(4,4),(-1.2,1.38777878078145E-16),.UNSPECIFIED.);
#6163=B_SPLINE_CURVE_WITH_KNOTS('',3,(#70518,#70519,#70520,#70521,#70522,
#70523,#70524),.UNSPECIFIED.,.F.,.F.,(4,3,4),(0.,0.0330660780484102,0.0578656365847179),
 .UNSPECIFIED.);
#6164=B_SPLINE_CURVE_WITH_KNOTS('',3,(#70526,#70527,#70528,#70529),
 .UNSPECIFIED.,.F.,.F.,(4,4),(8.32667268468867E-17,1.2),.UNSPECIFIED.);
#6165=B_SPLINE_CURVE_WITH_KNOTS('',3,(#70531,#70532,#70533,#70534,#70535,
#70536,#70537),.UNSPECIFIED.,.F.,.F.,(4,3,4),(0.,0.0247995585363082,0.057865636584719),
 .UNSPECIFIED.);
#6166=B_SPLINE_CURVE_WITH_KNOTS('',3,(#70538,#70539,#70540,#70541),
 .UNSPECIFIED.,.F.,.F.,(4,4),(-1.2,-8.32667268468867E-17),.UNSPECIFIED.);
#6167=B_SPLINE_CURVE_WITH_KNOTS('',3,(#71365,#71366,#71367,#71368,#71369,
#71370,#71371),.UNSPECIFIED.,.F.,.F.,(4,3,4),(0.,0.0330660780458722,0.0578656365802764),
 .UNSPECIFIED.);
#6168=B_SPLINE_CURVE_WITH_KNOTS('',3,(#71373,#71374,#71375,#71376),
 .UNSPECIFIED.,.F.,.F.,(4,4),(0.,1.2),.UNSPECIFIED.);
#6169=B_SPLINE_CURVE_WITH_KNOTS('',3,(#71378,#71379,#71380,#71381,#71382,
#71383,#71384),.UNSPECIFIED.,.F.,.F.,(4,3,4),(0.,0.0247995585344033,0.0578656365802744),
 .UNSPECIFIED.);
#6170=B_SPLINE_CURVE_WITH_KNOTS('',3,(#71385,#71386,#71387,#71388),
 .UNSPECIFIED.,.F.,.F.,(4,4),(-1.2,0.),.UNSPECIFIED.);
#6171=B_SPLINE_CURVE_WITH_KNOTS('',3,(#71414,#71415,#71416,#71417,#71418,
#71419,#71420),.UNSPECIFIED.,.F.,.F.,(4,3,4),(0.,0.0330660780484072,0.0578656365847127),
 .UNSPECIFIED.);
#6172=B_SPLINE_CURVE_WITH_KNOTS('',3,(#71422,#71423,#71424,#71425),
 .UNSPECIFIED.,.F.,.F.,(4,4),(1.66533453693773E-16,1.2),.UNSPECIFIED.);
#6173=B_SPLINE_CURVE_WITH_KNOTS('',3,(#71427,#71428,#71429,#71430,#71431,
#71432,#71433),.UNSPECIFIED.,.F.,.F.,(4,3,4),(0.,0.0247995585363061,0.0578656365847142),
 .UNSPECIFIED.);
#6174=B_SPLINE_CURVE_WITH_KNOTS('',3,(#71434,#71435,#71436,#71437),
 .UNSPECIFIED.,.F.,.F.,(4,4),(-1.2,-1.66533453693773E-16),.UNSPECIFIED.);
#6175=B_SPLINE_CURVE_WITH_KNOTS('',3,(#72261,#72262,#72263,#72264,#72265,
#72266,#72267),.UNSPECIFIED.,.F.,.F.,(4,3,4),(0.,0.033066078045837,0.0578656365802148),
 .UNSPECIFIED.);
#6176=B_SPLINE_CURVE_WITH_KNOTS('',3,(#72269,#72270,#72271,#72272),
 .UNSPECIFIED.,.F.,.F.,(4,4),(-1.38777878078145E-16,1.2),.UNSPECIFIED.);
#6177=B_SPLINE_CURVE_WITH_KNOTS('',3,(#72274,#72275,#72276,#72277,#72278,
#72279,#72280),.UNSPECIFIED.,.F.,.F.,(4,3,4),(0.,0.0247995585343889,0.0578656365802407),
 .UNSPECIFIED.);
#6178=B_SPLINE_CURVE_WITH_KNOTS('',3,(#72281,#72282,#72283,#72284),
 .UNSPECIFIED.,.F.,.F.,(4,4),(-1.2,1.38777878078145E-16),.UNSPECIFIED.);
#6179=B_SPLINE_CURVE_WITH_KNOTS('',3,(#72310,#72311,#72312,#72313,#72314,
#72315,#72316),.UNSPECIFIED.,.F.,.F.,(4,3,4),(0.,0.0330660780484256,0.0578656365847448),
 .UNSPECIFIED.);
#6180=B_SPLINE_CURVE_WITH_KNOTS('',3,(#72318,#72319,#72320,#72321),
 .UNSPECIFIED.,.F.,.F.,(4,4),(-2.08166817117217E-17,1.2),.UNSPECIFIED.);
#6181=B_SPLINE_CURVE_WITH_KNOTS('',3,(#72323,#72324,#72325,#72326,#72327,
#72328,#72329),.UNSPECIFIED.,.F.,.F.,(4,3,4),(0.,0.024799558536321,0.057865636584749),
 .UNSPECIFIED.);
#6182=B_SPLINE_CURVE_WITH_KNOTS('',3,(#72330,#72331,#72332,#72333),
 .UNSPECIFIED.,.F.,.F.,(4,4),(-1.2,2.08166817117217E-17),.UNSPECIFIED.);
#6183=B_SPLINE_CURVE_WITH_KNOTS('',3,(#73157,#73158,#73159,#73160,#73161,
#73162,#73163),.UNSPECIFIED.,.F.,.F.,(4,3,4),(0.,0.0330660780458522,0.0578656365802413),
 .UNSPECIFIED.);
#6184=B_SPLINE_CURVE_WITH_KNOTS('',3,(#73165,#73166,#73167,#73168),
 .UNSPECIFIED.,.F.,.F.,(4,4),(-8.32667268468868E-17,1.2),.UNSPECIFIED.);
#6185=B_SPLINE_CURVE_WITH_KNOTS('',3,(#73170,#73171,#73172,#73173,#73174,
#73175,#73176),.UNSPECIFIED.,.F.,.F.,(4,3,4),(0.,0.0247995585343892,0.0578656365802414),
 .UNSPECIFIED.);
#6186=B_SPLINE_CURVE_WITH_KNOTS('',3,(#73177,#73178,#73179,#73180),
 .UNSPECIFIED.,.F.,.F.,(4,4),(-1.2,8.32667268468868E-17),.UNSPECIFIED.);
#6187=B_SPLINE_CURVE_WITH_KNOTS('',3,(#73206,#73207,#73208,#73209,#73210,
#73211,#73212),.UNSPECIFIED.,.F.,.F.,(4,3,4),(0.,0.0330660780484257,0.057865636584745),
 .UNSPECIFIED.);
#6188=B_SPLINE_CURVE_WITH_KNOTS('',3,(#73214,#73215,#73216,#73217),
 .UNSPECIFIED.,.F.,.F.,(4,4),(1.38777878078145E-16,1.2),.UNSPECIFIED.);
#6189=B_SPLINE_CURVE_WITH_KNOTS('',3,(#73219,#73220,#73221,#73222,#73223,
#73224,#73225),.UNSPECIFIED.,.F.,.F.,(4,3,4),(0.,0.0247995585363191,0.0578656365847445),
 .UNSPECIFIED.);
#6190=B_SPLINE_CURVE_WITH_KNOTS('',3,(#73226,#73227,#73228,#73229),
 .UNSPECIFIED.,.F.,.F.,(4,4),(-1.2,-1.38777878078145E-16),.UNSPECIFIED.);
#6191=B_SPLINE_CURVE_WITH_KNOTS('',3,(#74053,#74054,#74055,#74056,#74057,
#74058,#74059),.UNSPECIFIED.,.F.,.F.,(4,3,4),(0.,0.0330660780458979,0.0578656365803213),
 .UNSPECIFIED.);
#6192=B_SPLINE_CURVE_WITH_KNOTS('',3,(#74061,#74062,#74063,#74064),
 .UNSPECIFIED.,.F.,.F.,(4,4),(-8.43563892506861E-17,1.2),.UNSPECIFIED.);
#6193=B_SPLINE_CURVE_WITH_KNOTS('',3,(#74066,#74067,#74068,#74069,#74070,
#74071,#74072),.UNSPECIFIED.,.F.,.F.,(4,3,4),(0.,0.0247995585344144,0.0578656365803003),
 .UNSPECIFIED.);
#6194=B_SPLINE_CURVE_WITH_KNOTS('',3,(#74073,#74074,#74075,#74076),
 .UNSPECIFIED.,.F.,.F.,(4,4),(-1.2,8.43563892506861E-17),.UNSPECIFIED.);
#6195=B_SPLINE_CURVE_WITH_KNOTS('',3,(#74102,#74103,#74104,#74105,#74106,
#74107,#74108),.UNSPECIFIED.,.F.,.F.,(4,3,4),(0.,0.033066078048418,0.0578656365847316),
 .UNSPECIFIED.);
#6196=B_SPLINE_CURVE_WITH_KNOTS('',3,(#74110,#74111,#74112,#74113),
 .UNSPECIFIED.,.F.,.F.,(4,4),(9.71445146547012E-17,1.2),.UNSPECIFIED.);
#6197=B_SPLINE_CURVE_WITH_KNOTS('',3,(#74115,#74116,#74117,#74118,#74119,
#74120,#74121),.UNSPECIFIED.,.F.,.F.,(4,3,4),(0.,0.0247995585363153,0.0578656365847356),
 .UNSPECIFIED.);
#6198=B_SPLINE_CURVE_WITH_KNOTS('',3,(#74122,#74123,#74124,#74125),
 .UNSPECIFIED.,.F.,.F.,(4,4),(-1.2,-9.71445146547012E-17),.UNSPECIFIED.);
#6199=B_SPLINE_CURVE_WITH_KNOTS('',3,(#74949,#74950,#74951,#74952,#74953,
#74954,#74955),.UNSPECIFIED.,.F.,.F.,(4,3,4),(0.,0.0330660780458051,0.0578656365801589),
 .UNSPECIFIED.);
#6200=B_SPLINE_CURVE_WITH_KNOTS('',3,(#74957,#74958,#74959,#74960),
 .UNSPECIFIED.,.F.,.F.,(4,4),(0.,1.2),.UNSPECIFIED.);
#6201=B_SPLINE_CURVE_WITH_KNOTS('',3,(#74962,#74963,#74964,#74965,#74966,
#74967,#74968),.UNSPECIFIED.,.F.,.F.,(4,3,4),(0.,0.0247995585343412,0.0578656365801295),
 .UNSPECIFIED.);
#6202=B_SPLINE_CURVE_WITH_KNOTS('',3,(#74969,#74970,#74971,#74972),
 .UNSPECIFIED.,.F.,.F.,(4,4),(-1.2,0.),.UNSPECIFIED.);
#6203=B_SPLINE_CURVE_WITH_KNOTS('',3,(#74998,#74999,#75000,#75001,#75002,
#75003,#75004),.UNSPECIFIED.,.F.,.F.,(4,3,4),(0.,0.03306607804841,0.0578656365847175),
 .UNSPECIFIED.);
#6204=B_SPLINE_CURVE_WITH_KNOTS('',3,(#75006,#75007,#75008,#75009),
 .UNSPECIFIED.,.F.,.F.,(4,4),(9.71445146547012E-17,1.2),.UNSPECIFIED.);
#6205=B_SPLINE_CURVE_WITH_KNOTS('',3,(#75011,#75012,#75013,#75014,#75015,
#75016,#75017),.UNSPECIFIED.,.F.,.F.,(4,3,4),(0.,0.0247995585363106,0.0578656365847246),
 .UNSPECIFIED.);
#6206=B_SPLINE_CURVE_WITH_KNOTS('',3,(#75018,#75019,#75020,#75021),
 .UNSPECIFIED.,.F.,.F.,(4,4),(-1.2,-9.71445146547012E-17),.UNSPECIFIED.);
#6207=B_SPLINE_CURVE_WITH_KNOTS('',3,(#75845,#75846,#75847,#75848,#75849,
#75850,#75851),.UNSPECIFIED.,.F.,.F.,(4,3,4),(0.,0.0330660780458883,0.0578656365803045),
 .UNSPECIFIED.);
#6208=B_SPLINE_CURVE_WITH_KNOTS('',3,(#75853,#75854,#75855,#75856),
 .UNSPECIFIED.,.F.,.F.,(4,4),(-1.49437708898837E-16,1.2),.UNSPECIFIED.);
#6209=B_SPLINE_CURVE_WITH_KNOTS('',3,(#75858,#75859,#75860,#75861,#75862,
#75863,#75864),.UNSPECIFIED.,.F.,.F.,(4,3,4),(0.,0.0247995585344198,0.0578656365803129),
 .UNSPECIFIED.);
#6210=B_SPLINE_CURVE_WITH_KNOTS('',3,(#75865,#75866,#75867,#75868),
 .UNSPECIFIED.,.F.,.F.,(4,4),(-1.2,1.49437708898837E-16),.UNSPECIFIED.);
#6211=B_SPLINE_CURVE_WITH_KNOTS('',3,(#75894,#75895,#75896,#75897,#75898,
#75899,#75900),.UNSPECIFIED.,.F.,.F.,(4,3,4),(0.,0.0330660780483754,0.057865636584657),
 .UNSPECIFIED.);
#6212=B_SPLINE_CURVE_WITH_KNOTS('',3,(#75902,#75903,#75904,#75905),
 .UNSPECIFIED.,.F.,.F.,(4,4),(9.71445146547012E-17,1.2),.UNSPECIFIED.);
#6213=B_SPLINE_CURVE_WITH_KNOTS('',3,(#75907,#75908,#75909,#75910,#75911,
#75912,#75913),.UNSPECIFIED.,.F.,.F.,(4,3,4),(0.,0.0247995585362854,0.057865636584666),
 .UNSPECIFIED.);
#6214=B_SPLINE_CURVE_WITH_KNOTS('',3,(#75914,#75915,#75916,#75917),
 .UNSPECIFIED.,.F.,.F.,(4,4),(-1.2,-9.71445146547012E-17),.UNSPECIFIED.);
#6215=B_SPLINE_CURVE_WITH_KNOTS('',3,(#76741,#76742,#76743,#76744,#76745,
#76746,#76747),.UNSPECIFIED.,.F.,.F.,(4,3,4),(0.,0.0330660780458802,0.0578656365802904),
 .UNSPECIFIED.);
#6216=B_SPLINE_CURVE_WITH_KNOTS('',3,(#76749,#76750,#76751,#76752),
 .UNSPECIFIED.,.F.,.F.,(4,4),(0.,1.2),.UNSPECIFIED.);
#6217=B_SPLINE_CURVE_WITH_KNOTS('',3,(#76754,#76755,#76756,#76757,#76758,
#76759,#76760),.UNSPECIFIED.,.F.,.F.,(4,3,4),(0.,0.0247995585344145,0.0578656365803004),
 .UNSPECIFIED.);
#6218=B_SPLINE_CURVE_WITH_KNOTS('',3,(#76761,#76762,#76763,#76764),
 .UNSPECIFIED.,.F.,.F.,(4,4),(-1.2,0.),.UNSPECIFIED.);
#6219=B_SPLINE_CURVE_WITH_KNOTS('',3,(#76790,#76791,#76792,#76793,#76794,
#76795,#76796),.UNSPECIFIED.,.F.,.F.,(4,3,4),(0.,0.033066078048439,0.0578656365847682),
 .UNSPECIFIED.);
#6220=B_SPLINE_CURVE_WITH_KNOTS('',3,(#76798,#76799,#76800,#76801),
 .UNSPECIFIED.,.F.,.F.,(4,4),(1.66533453693773E-16,1.2),.UNSPECIFIED.);
#6221=B_SPLINE_CURVE_WITH_KNOTS('',3,(#76803,#76804,#76805,#76806,#76807,
#76808,#76809),.UNSPECIFIED.,.F.,.F.,(4,3,4),(0.,0.0247995585363292,0.0578656365847682),
 .UNSPECIFIED.);
#6222=B_SPLINE_CURVE_WITH_KNOTS('',3,(#76810,#76811,#76812,#76813),
 .UNSPECIFIED.,.F.,.F.,(4,4),(-1.2,-1.66533453693773E-16),.UNSPECIFIED.);
#6223=B_SPLINE_CURVE_WITH_KNOTS('',3,(#77637,#77638,#77639,#77640,#77641,
#77642,#77643),.UNSPECIFIED.,.F.,.F.,(4,3,4),(0.,0.033066078045871,0.0578656365802742),
 .UNSPECIFIED.);
#6224=B_SPLINE_CURVE_WITH_KNOTS('',3,(#77645,#77646,#77647,#77648),
 .UNSPECIFIED.,.F.,.F.,(4,4),(-1.47525527564366E-17,1.2),.UNSPECIFIED.);
#6225=B_SPLINE_CURVE_WITH_KNOTS('',3,(#77650,#77651,#77652,#77653,#77654,
#77655,#77656),.UNSPECIFIED.,.F.,.F.,(4,3,4),(0.,0.0247995585344122,0.057865636580295),
 .UNSPECIFIED.);
#6226=B_SPLINE_CURVE_WITH_KNOTS('',3,(#77657,#77658,#77659,#77660),
 .UNSPECIFIED.,.F.,.F.,(4,4),(-1.2,1.47525527564366E-17),.UNSPECIFIED.);
#6227=B_SPLINE_CURVE_WITH_KNOTS('',3,(#77686,#77687,#77688,#77689,#77690,
#77691,#77692),.UNSPECIFIED.,.F.,.F.,(4,3,4),(0.,0.0330660780484519,0.0578656365847908),
 .UNSPECIFIED.);
#6228=B_SPLINE_CURVE_WITH_KNOTS('',3,(#77694,#77695,#77696,#77697),
 .UNSPECIFIED.,.F.,.F.,(4,4),(-8.32667268468867E-17,1.2),.UNSPECIFIED.);
#6229=B_SPLINE_CURVE_WITH_KNOTS('',3,(#77699,#77700,#77701,#77702,#77703,
#77704,#77705),.UNSPECIFIED.,.F.,.F.,(4,3,4),(0.,0.0247995585363362,0.0578656365847844),
 .UNSPECIFIED.);
#6230=B_SPLINE_CURVE_WITH_KNOTS('',3,(#77706,#77707,#77708,#77709),
 .UNSPECIFIED.,.F.,.F.,(4,4),(-1.2,8.32667268468867E-17),.UNSPECIFIED.);
#6231=B_SPLINE_CURVE_WITH_KNOTS('',3,(#78533,#78534,#78535,#78536,#78537,
#78538,#78539),.UNSPECIFIED.,.F.,.F.,(4,3,4),(0.,0.0330660780458195,0.0578656365801842),
 .UNSPECIFIED.);
#6232=B_SPLINE_CURVE_WITH_KNOTS('',3,(#78541,#78542,#78543,#78544),
 .UNSPECIFIED.,.F.,.F.,(4,4),(2.77555756156289E-17,1.2),.UNSPECIFIED.);
#6233=B_SPLINE_CURVE_WITH_KNOTS('',3,(#78546,#78547,#78548,#78549,#78550,
#78551,#78552),.UNSPECIFIED.,.F.,.F.,(4,3,4),(0.,0.024799558534367,0.0578656365801897),
 .UNSPECIFIED.);
#6234=B_SPLINE_CURVE_WITH_KNOTS('',3,(#78553,#78554,#78555,#78556),
 .UNSPECIFIED.,.F.,.F.,(4,4),(-1.2,-2.77555756156289E-17),.UNSPECIFIED.);
#6235=B_SPLINE_CURVE_WITH_KNOTS('',3,(#78582,#78583,#78584,#78585,#78586,
#78587,#78588),.UNSPECIFIED.,.F.,.F.,(4,3,4),(0.,0.0330660780484703,0.057865636584823),
 .UNSPECIFIED.);
#6236=B_SPLINE_CURVE_WITH_KNOTS('',3,(#78590,#78591,#78592,#78593),
 .UNSPECIFIED.,.F.,.F.,(4,4),(9.44002594796574E-17,1.2),.UNSPECIFIED.);
#6237=B_SPLINE_CURVE_WITH_KNOTS('',3,(#78595,#78596,#78597,#78598,#78599,
#78600,#78601),.UNSPECIFIED.,.F.,.F.,(4,3,4),(0.,0.0247995585363458,0.0578656365848069),
 .UNSPECIFIED.);
#6238=B_SPLINE_CURVE_WITH_KNOTS('',3,(#78602,#78603,#78604,#78605),
 .UNSPECIFIED.,.F.,.F.,(4,4),(-1.2,-9.44002594796574E-17),.UNSPECIFIED.);
#6239=B_SPLINE_CURVE_WITH_KNOTS('',3,(#79429,#79430,#79431,#79432,#79433,
#79434,#79435),.UNSPECIFIED.,.F.,.F.,(4,3,4),(0.,0.0330660780458513,0.0578656365802398),
 .UNSPECIFIED.);
#6240=B_SPLINE_CURVE_WITH_KNOTS('',3,(#79437,#79438,#79439,#79440),
 .UNSPECIFIED.,.F.,.F.,(4,4),(0.,1.2),.UNSPECIFIED.);
#6241=B_SPLINE_CURVE_WITH_KNOTS('',3,(#79442,#79443,#79444,#79445,#79446,
#79447,#79448),.UNSPECIFIED.,.F.,.F.,(4,3,4),(0.,0.0247995585343902,0.0578656365802439),
 .UNSPECIFIED.);
#6242=B_SPLINE_CURVE_WITH_KNOTS('',3,(#79449,#79450,#79451,#79452),
 .UNSPECIFIED.,.F.,.F.,(4,4),(-1.2,0.),.UNSPECIFIED.);
#6243=B_SPLINE_CURVE_WITH_KNOTS('',3,(#79478,#79479,#79480,#79481,#79482,
#79483,#79484),.UNSPECIFIED.,.F.,.F.,(4,3,4),(0.,0.0330660780484092,0.0578656365847161),
 .UNSPECIFIED.);
#6244=B_SPLINE_CURVE_WITH_KNOTS('',3,(#79486,#79487,#79488,#79489),
 .UNSPECIFIED.,.F.,.F.,(4,4),(1.66533453693773E-16,1.2),.UNSPECIFIED.);
#6245=B_SPLINE_CURVE_WITH_KNOTS('',3,(#79491,#79492,#79493,#79494,#79495,
#79496,#79497),.UNSPECIFIED.,.F.,.F.,(4,3,4),(0.,0.0247995585363076,0.0578656365847178),
 .UNSPECIFIED.);
#6246=B_SPLINE_CURVE_WITH_KNOTS('',3,(#79498,#79499,#79500,#79501),
 .UNSPECIFIED.,.F.,.F.,(4,4),(-1.2,-1.66533453693773E-16),.UNSPECIFIED.);
#6247=B_SPLINE_CURVE_WITH_KNOTS('',3,(#80325,#80326,#80327,#80328,#80329,
#80330,#80331),.UNSPECIFIED.,.F.,.F.,(4,3,4),(0.,0.033066078045864,0.0578656365802619),
 .UNSPECIFIED.);
#6248=B_SPLINE_CURVE_WITH_KNOTS('',3,(#80333,#80334,#80335,#80336),
 .UNSPECIFIED.,.F.,.F.,(4,4),(-1.8224407144634E-16,1.2),.UNSPECIFIED.);
#6249=B_SPLINE_CURVE_WITH_KNOTS('',3,(#80338,#80339,#80340,#80341,#80342,
#80343,#80344),.UNSPECIFIED.,.F.,.F.,(4,3,4),(0.,0.0247995585343939,0.0578656365802525),
 .UNSPECIFIED.);
#6250=B_SPLINE_CURVE_WITH_KNOTS('',3,(#80345,#80346,#80347,#80348),
 .UNSPECIFIED.,.F.,.F.,(4,4),(-1.2,1.8224407144634E-16),.UNSPECIFIED.);
#6251=B_SPLINE_CURVE_WITH_KNOTS('',3,(#80374,#80375,#80376,#80377,#80378,
#80379,#80380),.UNSPECIFIED.,.F.,.F.,(4,3,4),(0.,0.0330660780484494,0.0578656365847864),
 .UNSPECIFIED.);
#6252=B_SPLINE_CURVE_WITH_KNOTS('',3,(#80382,#80383,#80384,#80385),
 .UNSPECIFIED.,.F.,.F.,(4,4),(-1.8809784878858E-36,1.2),.UNSPECIFIED.);
#6253=B_SPLINE_CURVE_WITH_KNOTS('',3,(#80387,#80388,#80389,#80390,#80391,
#80392,#80393),.UNSPECIFIED.,.F.,.F.,(4,3,4),(0.,0.0247995585363297,0.0578656365847694),
 .UNSPECIFIED.);
#6254=B_SPLINE_CURVE_WITH_KNOTS('',3,(#80394,#80395,#80396,#80397),
 .UNSPECIFIED.,.F.,.F.,(4,4),(-1.2,1.8809784878858E-36),.UNSPECIFIED.);
#6255=B_SPLINE_CURVE_WITH_KNOTS('',3,(#81221,#81222,#81223,#81224,#81225,
#81226,#81227),.UNSPECIFIED.,.F.,.F.,(4,3,4),(0.,0.033066078045872,0.0578656365802761),
 .UNSPECIFIED.);
#6256=B_SPLINE_CURVE_WITH_KNOTS('',3,(#81229,#81230,#81231,#81232),
 .UNSPECIFIED.,.F.,.F.,(4,4),(-5.55111512312578E-17,1.2),.UNSPECIFIED.);
#6257=B_SPLINE_CURVE_WITH_KNOTS('',3,(#81234,#81235,#81236,#81237,#81238,
#81239,#81240),.UNSPECIFIED.,.F.,.F.,(4,3,4),(0.,0.0247995585344019,0.0578656365802711),
 .UNSPECIFIED.);
#6258=B_SPLINE_CURVE_WITH_KNOTS('',3,(#81241,#81242,#81243,#81244),
 .UNSPECIFIED.,.F.,.F.,(4,4),(-1.2,5.55111512312578E-17),.UNSPECIFIED.);
#6259=B_SPLINE_CURVE_WITH_KNOTS('',3,(#81270,#81271,#81272,#81273,#81274,
#81275,#81276),.UNSPECIFIED.,.F.,.F.,(4,3,4),(0.,0.0330660780483919,0.0578656365846859),
 .UNSPECIFIED.);
#6260=B_SPLINE_CURVE_WITH_KNOTS('',3,(#81278,#81279,#81280,#81281),
 .UNSPECIFIED.,.F.,.F.,(4,4),(9.71445146547012E-17,1.2),.UNSPECIFIED.);
#6261=B_SPLINE_CURVE_WITH_KNOTS('',3,(#81283,#81284,#81285,#81286,#81287,
#81288,#81289),.UNSPECIFIED.,.F.,.F.,(4,3,4),(0.,0.0247995585363007,0.0578656365847015),
 .UNSPECIFIED.);
#6262=B_SPLINE_CURVE_WITH_KNOTS('',3,(#81290,#81291,#81292,#81293),
 .UNSPECIFIED.,.F.,.F.,(4,4),(-1.2,-9.71445146547012E-17),.UNSPECIFIED.);
#6263=B_SPLINE_CURVE_WITH_KNOTS('',3,(#82117,#82118,#82119,#82120,#82121,
#82122,#82123),.UNSPECIFIED.,.F.,.F.,(4,3,4),(0.,0.03306607804585,0.0578656365802375),
 .UNSPECIFIED.);
#6264=B_SPLINE_CURVE_WITH_KNOTS('',3,(#82125,#82126,#82127,#82128),
 .UNSPECIFIED.,.F.,.F.,(4,4),(-8.32667268468867E-17,1.2),.UNSPECIFIED.);
#6265=B_SPLINE_CURVE_WITH_KNOTS('',3,(#82130,#82131,#82132,#82133,#82134,
#82135,#82136),.UNSPECIFIED.,.F.,.F.,(4,3,4),(0.,0.0247995585343902,0.0578656365802437),
 .UNSPECIFIED.);
#6266=B_SPLINE_CURVE_WITH_KNOTS('',3,(#82137,#82138,#82139,#82140),
 .UNSPECIFIED.,.F.,.F.,(4,4),(-1.2,8.32667268468867E-17),.UNSPECIFIED.);
#6267=B_SPLINE_CURVE_WITH_KNOTS('',3,(#82166,#82167,#82168,#82169,#82170,
#82171,#82172),.UNSPECIFIED.,.F.,.F.,(4,3,4),(0.,0.0330660780483826,0.0578656365846695),
 .UNSPECIFIED.);
#6268=B_SPLINE_CURVE_WITH_KNOTS('',3,(#82174,#82175,#82176,#82177),
 .UNSPECIFIED.,.F.,.F.,(4,4),(0.,1.2),.UNSPECIFIED.);
#6269=B_SPLINE_CURVE_WITH_KNOTS('',3,(#82179,#82180,#82181,#82182,#82183,
#82184,#82185),.UNSPECIFIED.,.F.,.F.,(4,3,4),(0.,0.0247995585362904,0.0578656365846775),
 .UNSPECIFIED.);
#6270=B_SPLINE_CURVE_WITH_KNOTS('',3,(#82186,#82187,#82188,#82189),
 .UNSPECIFIED.,.F.,.F.,(4,4),(-1.2,0.),.UNSPECIFIED.);
#6271=B_SPLINE_CURVE_WITH_KNOTS('',3,(#83013,#83014,#83015,#83016,#83017,
#83018,#83019),.UNSPECIFIED.,.F.,.F.,(4,3,4),(0.,0.0330660780458701,0.0578656365802727),
 .UNSPECIFIED.);
#6272=B_SPLINE_CURVE_WITH_KNOTS('',3,(#83021,#83022,#83023,#83024),
 .UNSPECIFIED.,.F.,.F.,(4,4),(0.,1.2),.UNSPECIFIED.);
#6273=B_SPLINE_CURVE_WITH_KNOTS('',3,(#83026,#83027,#83028,#83029,#83030,
#83031,#83032),.UNSPECIFIED.,.F.,.F.,(4,3,4),(0.,0.0247995585344047,0.0578656365802776),
 .UNSPECIFIED.);
#6274=B_SPLINE_CURVE_WITH_KNOTS('',3,(#83033,#83034,#83035,#83036),
 .UNSPECIFIED.,.F.,.F.,(4,4),(-1.2,0.),.UNSPECIFIED.);
#6275=B_SPLINE_CURVE_WITH_KNOTS('',3,(#83062,#83063,#83064,#83065,#83066,
#83067,#83068),.UNSPECIFIED.,.F.,.F.,(4,3,4),(0.,0.0330660780484355,0.0578656365847621),
 .UNSPECIFIED.);
#6276=B_SPLINE_CURVE_WITH_KNOTS('',3,(#83070,#83071,#83072,#83073),
 .UNSPECIFIED.,.F.,.F.,(4,4),(9.71445146547012E-17,1.2),.UNSPECIFIED.);
#6277=B_SPLINE_CURVE_WITH_KNOTS('',3,(#83075,#83076,#83077,#83078,#83079,
#83080,#83081),.UNSPECIFIED.,.F.,.F.,(4,3,4),(0.,0.0247995585363203,0.0578656365847474),
 .UNSPECIFIED.);
#6278=B_SPLINE_CURVE_WITH_KNOTS('',3,(#83082,#83083,#83084,#83085),
 .UNSPECIFIED.,.F.,.F.,(4,4),(-1.2,-9.71445146547012E-17),.UNSPECIFIED.);
#6279=B_SPLINE_CURVE_WITH_KNOTS('',3,(#83909,#83910,#83911,#83912,#83913,
#83914,#83915),.UNSPECIFIED.,.F.,.F.,(4,3,4),(0.,0.0330660780458469,0.057865636580232),
 .UNSPECIFIED.);
#6280=B_SPLINE_CURVE_WITH_KNOTS('',3,(#83917,#83918,#83919,#83920),
 .UNSPECIFIED.,.F.,.F.,(4,4),(-2.77555756156289E-17,1.2),.UNSPECIFIED.);
#6281=B_SPLINE_CURVE_WITH_KNOTS('',3,(#83922,#83923,#83924,#83925,#83926,
#83927,#83928),.UNSPECIFIED.,.F.,.F.,(4,3,4),(0.,0.0247995585343852,0.0578656365802322),
 .UNSPECIFIED.);
#6282=B_SPLINE_CURVE_WITH_KNOTS('',3,(#83929,#83930,#83931,#83932),
 .UNSPECIFIED.,.F.,.F.,(4,4),(-1.2,2.77555756156289E-17),.UNSPECIFIED.);
#6283=B_SPLINE_CURVE_WITH_KNOTS('',3,(#83958,#83959,#83960,#83961,#83962,
#83963,#83964),.UNSPECIFIED.,.F.,.F.,(4,3,4),(0.,0.0330660780484186,0.0578656365847326),
 .UNSPECIFIED.);
#6284=B_SPLINE_CURVE_WITH_KNOTS('',3,(#83966,#83967,#83968,#83969),
 .UNSPECIFIED.,.F.,.F.,(4,4),(9.71445146547012E-17,1.2),.UNSPECIFIED.);
#6285=B_SPLINE_CURVE_WITH_KNOTS('',3,(#83971,#83972,#83973,#83974,#83975,
#83976,#83977),.UNSPECIFIED.,.F.,.F.,(4,3,4),(0.,0.0247995585363121,0.0578656365847283),
 .UNSPECIFIED.);
#6286=B_SPLINE_CURVE_WITH_KNOTS('',3,(#83978,#83979,#83980,#83981),
 .UNSPECIFIED.,.F.,.F.,(4,4),(-1.2,-9.71445146547012E-17),.UNSPECIFIED.);
#6287=B_SPLINE_CURVE_WITH_KNOTS('',3,(#84805,#84806,#84807,#84808,#84809,
#84810,#84811),.UNSPECIFIED.,.F.,.F.,(4,3,4),(0.,0.0330660780458515,0.05786563658024),
 .UNSPECIFIED.);
#6288=B_SPLINE_CURVE_WITH_KNOTS('',3,(#84813,#84814,#84815,#84816),
 .UNSPECIFIED.,.F.,.F.,(4,4),(-9.71445146547012E-17,1.2),.UNSPECIFIED.);
#6289=B_SPLINE_CURVE_WITH_KNOTS('',3,(#84818,#84819,#84820,#84821,#84822,
#84823,#84824),.UNSPECIFIED.,.F.,.F.,(4,3,4),(0.,0.0247995585343902,0.0578656365802438),
 .UNSPECIFIED.);
#6290=B_SPLINE_CURVE_WITH_KNOTS('',3,(#84825,#84826,#84827,#84828),
 .UNSPECIFIED.,.F.,.F.,(4,4),(-1.2,9.71445146547012E-17),.UNSPECIFIED.);
#6291=B_SPLINE_CURVE_WITH_KNOTS('',3,(#84854,#84855,#84856,#84857,#84858,
#84859,#84860),.UNSPECIFIED.,.F.,.F.,(4,3,4),(0.,0.0330660780484054,0.0578656365847094),
 .UNSPECIFIED.);
#6292=B_SPLINE_CURVE_WITH_KNOTS('',3,(#84862,#84863,#84864,#84865),
 .UNSPECIFIED.,.F.,.F.,(4,4),(3.88891082483996E-17,1.2),.UNSPECIFIED.);
#6293=B_SPLINE_CURVE_WITH_KNOTS('',3,(#84867,#84868,#84869,#84870,#84871,
#84872,#84873),.UNSPECIFIED.,.F.,.F.,(4,3,4),(0.,0.0247995585363042,0.0578656365847097),
 .UNSPECIFIED.);
#6294=B_SPLINE_CURVE_WITH_KNOTS('',3,(#84874,#84875,#84876,#84877),
 .UNSPECIFIED.,.F.,.F.,(4,4),(-1.2,-3.88891082483996E-17),.UNSPECIFIED.);
#6295=B_SPLINE_CURVE_WITH_KNOTS('',3,(#85701,#85702,#85703,#85704,#85705,
#85706,#85707),.UNSPECIFIED.,.F.,.F.,(4,3,4),(0.,0.0330660780458555,0.0578656365802471),
 .UNSPECIFIED.);
#6296=B_SPLINE_CURVE_WITH_KNOTS('',3,(#85709,#85710,#85711,#85712),
 .UNSPECIFIED.,.F.,.F.,(4,4),(-1.11022302462516E-16,1.2),.UNSPECIFIED.);
#6297=B_SPLINE_CURVE_WITH_KNOTS('',3,(#85714,#85715,#85716,#85717,#85718,
#85719,#85720),.UNSPECIFIED.,.F.,.F.,(4,3,4),(0.,0.0247995585343896,0.0578656365802423),
 .UNSPECIFIED.);
#6298=B_SPLINE_CURVE_WITH_KNOTS('',3,(#85721,#85722,#85723,#85724),
 .UNSPECIFIED.,.F.,.F.,(4,4),(-1.2,1.11022302462516E-16),.UNSPECIFIED.);
#6299=B_SPLINE_CURVE_WITH_KNOTS('',3,(#85750,#85751,#85752,#85753,#85754,
#85755,#85756),.UNSPECIFIED.,.F.,.F.,(4,3,4),(0.,0.0330660780484363,0.0578656365847635),
 .UNSPECIFIED.);
#6300=B_SPLINE_CURVE_WITH_KNOTS('',3,(#85758,#85759,#85760,#85761),
 .UNSPECIFIED.,.F.,.F.,(4,4),(3.88891082483996E-17,1.2),.UNSPECIFIED.);
#6301=B_SPLINE_CURVE_WITH_KNOTS('',3,(#85763,#85764,#85765,#85766,#85767,
#85768,#85769),.UNSPECIFIED.,.F.,.F.,(4,3,4),(0.,0.0247995585363172,0.05786563658474),
 .UNSPECIFIED.);
#6302=B_SPLINE_CURVE_WITH_KNOTS('',3,(#85770,#85771,#85772,#85773),
 .UNSPECIFIED.,.F.,.F.,(4,4),(-1.2,-3.88891082483996E-17),.UNSPECIFIED.);
#6303=B_SPLINE_CURVE_WITH_KNOTS('',3,(#86597,#86598,#86599,#86600,#86601,
#86602,#86603),.UNSPECIFIED.,.F.,.F.,(4,3,4),(0.,0.033066078045885,0.0578656365802987),
 .UNSPECIFIED.);
#6304=B_SPLINE_CURVE_WITH_KNOTS('',3,(#86605,#86606,#86607,#86608),
 .UNSPECIFIED.,.F.,.F.,(4,4),(-1.8809784878848E-36,1.2),.UNSPECIFIED.);
#6305=B_SPLINE_CURVE_WITH_KNOTS('',3,(#86610,#86611,#86612,#86613,#86614,
#86615,#86616),.UNSPECIFIED.,.F.,.F.,(4,3,4),(0.,0.0247995585344127,0.0578656365802964),
 .UNSPECIFIED.);
#6306=B_SPLINE_CURVE_WITH_KNOTS('',3,(#86617,#86618,#86619,#86620),
 .UNSPECIFIED.,.F.,.F.,(4,4),(-1.2,1.8809784878848E-36),.UNSPECIFIED.);
#6307=B_SPLINE_CURVE_WITH_KNOTS('',3,(#86646,#86647,#86648,#86649,#86650,
#86651,#86652),.UNSPECIFIED.,.F.,.F.,(4,3,4),(0.,0.0330660780484386,0.0578656365847676),
 .UNSPECIFIED.);
#6308=B_SPLINE_CURVE_WITH_KNOTS('',3,(#86654,#86655,#86656,#86657),
 .UNSPECIFIED.,.F.,.F.,(4,4),(-1.11022302462516E-16,1.2),.UNSPECIFIED.);
#6309=B_SPLINE_CURVE_WITH_KNOTS('',3,(#86659,#86660,#86661,#86662,#86663,
#86664,#86665),.UNSPECIFIED.,.F.,.F.,(4,3,4),(0.,0.024799558536317,0.0578656365847397),
 .UNSPECIFIED.);
#6310=B_SPLINE_CURVE_WITH_KNOTS('',3,(#86666,#86667,#86668,#86669),
 .UNSPECIFIED.,.F.,.F.,(4,4),(-1.2,1.11022302462516E-16),.UNSPECIFIED.);
#6311=B_SPLINE_CURVE_WITH_KNOTS('',3,(#87493,#87494,#87495,#87496,#87497,
#87498,#87499),.UNSPECIFIED.,.F.,.F.,(4,3,4),(0.,0.0330660780458761,0.0578656365802832),
 .UNSPECIFIED.);
#6312=B_SPLINE_CURVE_WITH_KNOTS('',3,(#87501,#87502,#87503,#87504),
 .UNSPECIFIED.,.F.,.F.,(4,4),(-8.32667268468867E-17,1.2),.UNSPECIFIED.);
#6313=B_SPLINE_CURVE_WITH_KNOTS('',3,(#87506,#87507,#87508,#87509,#87510,
#87511,#87512),.UNSPECIFIED.,.F.,.F.,(4,3,4),(0.,0.0247995585344117,0.0578656365802939),
 .UNSPECIFIED.);
#6314=B_SPLINE_CURVE_WITH_KNOTS('',3,(#87513,#87514,#87515,#87516),
 .UNSPECIFIED.,.F.,.F.,(4,4),(-1.2,8.32667268468867E-17),.UNSPECIFIED.);
#6315=B_SPLINE_CURVE_WITH_KNOTS('',3,(#87542,#87543,#87544,#87545,#87546,
#87547,#87548),.UNSPECIFIED.,.F.,.F.,(4,3,4),(0.,0.0330660780484119,0.0578656365847208),
 .UNSPECIFIED.);
#6316=B_SPLINE_CURVE_WITH_KNOTS('',3,(#87550,#87551,#87552,#87553),
 .UNSPECIFIED.,.F.,.F.,(4,4),(9.71445146547012E-17,1.2),.UNSPECIFIED.);
#6317=B_SPLINE_CURVE_WITH_KNOTS('',3,(#87555,#87556,#87557,#87558,#87559,
#87560,#87561),.UNSPECIFIED.,.F.,.F.,(4,3,4),(0.,0.0247995585363125,0.0578656365847292),
 .UNSPECIFIED.);
#6318=B_SPLINE_CURVE_WITH_KNOTS('',3,(#87562,#87563,#87564,#87565),
 .UNSPECIFIED.,.F.,.F.,(4,4),(-1.2,-9.71445146547012E-17),.UNSPECIFIED.);
#6319=B_SPLINE_CURVE_WITH_KNOTS('',3,(#88389,#88390,#88391,#88392,#88393,
#88394,#88395),.UNSPECIFIED.,.F.,.F.,(4,3,4),(0.,0.033066078045965,0.0578656365804388),
 .UNSPECIFIED.);
#6320=B_SPLINE_CURVE_WITH_KNOTS('',3,(#88397,#88398,#88399,#88400),
 .UNSPECIFIED.,.F.,.F.,(4,4),(2.77555756156289E-17,1.2),.UNSPECIFIED.);
#6321=B_SPLINE_CURVE_WITH_KNOTS('',3,(#88402,#88403,#88404,#88405,#88406,
#88407,#88408),.UNSPECIFIED.,.F.,.F.,(4,3,4),(0.,0.024799558534469,0.0578656365804277),
 .UNSPECIFIED.);
#6322=B_SPLINE_CURVE_WITH_KNOTS('',3,(#88409,#88410,#88411,#88412),
 .UNSPECIFIED.,.F.,.F.,(4,4),(-1.2,-2.77555756156289E-17),.UNSPECIFIED.);
#6323=B_SPLINE_CURVE_WITH_KNOTS('',3,(#88438,#88439,#88440,#88441,#88442,
#88443,#88444),.UNSPECIFIED.,.F.,.F.,(4,3,4),(0.,0.0330660780484208,0.0578656365847365),
 .UNSPECIFIED.);
#6324=B_SPLINE_CURVE_WITH_KNOTS('',3,(#88446,#88447,#88448,#88449),
 .UNSPECIFIED.,.F.,.F.,(4,4),(-1.38777878078145E-16,1.2),.UNSPECIFIED.);
#6325=B_SPLINE_CURVE_WITH_KNOTS('',3,(#88451,#88452,#88453,#88454,#88455,
#88456,#88457),.UNSPECIFIED.,.F.,.F.,(4,3,4),(0.,0.0247995585363145,0.0578656365847338),
 .UNSPECIFIED.);
#6326=B_SPLINE_CURVE_WITH_KNOTS('',3,(#88458,#88459,#88460,#88461),
 .UNSPECIFIED.,.F.,.F.,(4,4),(-1.2,1.38777878078145E-16),.UNSPECIFIED.);
#6327=B_SPLINE_CURVE_WITH_KNOTS('',3,(#89285,#89286,#89287,#89288,#89289,
#89290,#89291),.UNSPECIFIED.,.F.,.F.,(4,3,4),(0.,0.0330660780458555,0.0578656365802471),
 .UNSPECIFIED.);
#6328=B_SPLINE_CURVE_WITH_KNOTS('',3,(#89293,#89294,#89295,#89296),
 .UNSPECIFIED.,.F.,.F.,(4,4),(2.77555756156289E-17,1.2),.UNSPECIFIED.);
#6329=B_SPLINE_CURVE_WITH_KNOTS('',3,(#89298,#89299,#89300,#89301,#89302,
#89303,#89304),.UNSPECIFIED.,.F.,.F.,(4,3,4),(0.,0.0247995585343909,0.0578656365802454),
 .UNSPECIFIED.);
#6330=B_SPLINE_CURVE_WITH_KNOTS('',3,(#89305,#89306,#89307,#89308),
 .UNSPECIFIED.,.F.,.F.,(4,4),(-1.2,-2.77555756156289E-17),.UNSPECIFIED.);
#6331=B_SPLINE_CURVE_WITH_KNOTS('',3,(#89334,#89335,#89336,#89337,#89338,
#89339,#89340),.UNSPECIFIED.,.F.,.F.,(4,3,4),(0.,0.0330660780484046,0.0578656365847081),
 .UNSPECIFIED.);
#6332=B_SPLINE_CURVE_WITH_KNOTS('',3,(#89342,#89343,#89344,#89345),
 .UNSPECIFIED.,.F.,.F.,(4,4),(9.71445146547012E-17,1.2),.UNSPECIFIED.);
#6333=B_SPLINE_CURVE_WITH_KNOTS('',3,(#89347,#89348,#89349,#89350,#89351,
#89352,#89353),.UNSPECIFIED.,.F.,.F.,(4,3,4),(0.,0.0247995585363076,0.0578656365847176),
 .UNSPECIFIED.);
#6334=B_SPLINE_CURVE_WITH_KNOTS('',3,(#89354,#89355,#89356,#89357),
 .UNSPECIFIED.,.F.,.F.,(4,4),(-1.2,-9.71445146547012E-17),.UNSPECIFIED.);
#6335=B_SPLINE_CURVE_WITH_KNOTS('',3,(#90181,#90182,#90183,#90184,#90185,
#90186,#90187),.UNSPECIFIED.,.F.,.F.,(4,3,4),(0.,0.0330660780458503,0.057865636580238),
 .UNSPECIFIED.);
#6336=B_SPLINE_CURVE_WITH_KNOTS('',3,(#90189,#90190,#90191,#90192),
 .UNSPECIFIED.,.F.,.F.,(4,4),(-7.5239139515392E-36,1.2),.UNSPECIFIED.);
#6337=B_SPLINE_CURVE_WITH_KNOTS('',3,(#90194,#90195,#90196,#90197,#90198,
#90199,#90200),.UNSPECIFIED.,.F.,.F.,(4,3,4),(0.,0.0247995585343863,0.0578656365802348),
 .UNSPECIFIED.);
#6338=B_SPLINE_CURVE_WITH_KNOTS('',3,(#90201,#90202,#90203,#90204),
 .UNSPECIFIED.,.F.,.F.,(4,4),(-1.2,7.5239139515392E-36),.UNSPECIFIED.);
#6339=B_SPLINE_CURVE_WITH_KNOTS('',3,(#90230,#90231,#90232,#90233,#90234,
#90235,#90236),.UNSPECIFIED.,.F.,.F.,(4,3,4),(0.,0.0330660780483922,0.0578656365846863),
 .UNSPECIFIED.);
#6340=B_SPLINE_CURVE_WITH_KNOTS('',3,(#90238,#90239,#90240,#90241),
 .UNSPECIFIED.,.F.,.F.,(4,4),(8.05224716718429E-17,1.2),.UNSPECIFIED.);
#6341=B_SPLINE_CURVE_WITH_KNOTS('',3,(#90243,#90244,#90245,#90246,#90247,
#90248,#90249),.UNSPECIFIED.,.F.,.F.,(4,3,4),(0.,0.0247995585363117,0.0578656365847273),
 .UNSPECIFIED.);
#6342=B_SPLINE_CURVE_WITH_KNOTS('',3,(#90250,#90251,#90252,#90253),
 .UNSPECIFIED.,.F.,.F.,(4,4),(-1.2,-8.05224716718429E-17),.UNSPECIFIED.);
#6343=B_SPLINE_CURVE_WITH_KNOTS('',3,(#91077,#91078,#91079,#91080,#91081,
#91082,#91083),.UNSPECIFIED.,.F.,.F.,(4,3,4),(0.,0.0330660780458931,0.057865636580313),
 .UNSPECIFIED.);
#6344=B_SPLINE_CURVE_WITH_KNOTS('',3,(#91085,#91086,#91087,#91088),
 .UNSPECIFIED.,.F.,.F.,(4,4),(0.,1.2),.UNSPECIFIED.);
#6345=B_SPLINE_CURVE_WITH_KNOTS('',3,(#91090,#91091,#91092,#91093,#91094,
#91095,#91096),.UNSPECIFIED.,.F.,.F.,(4,3,4),(0.,0.0247995585344171,0.0578656365803065),
 .UNSPECIFIED.);
#6346=B_SPLINE_CURVE_WITH_KNOTS('',3,(#91097,#91098,#91099,#91100),
 .UNSPECIFIED.,.F.,.F.,(4,4),(-1.2,0.),.UNSPECIFIED.);
#6347=B_SPLINE_CURVE_WITH_KNOTS('',3,(#91126,#91127,#91128,#91129,#91130,
#91131,#91132),.UNSPECIFIED.,.F.,.F.,(4,3,4),(0.,0.03306607804841,0.0578656365847175),
 .UNSPECIFIED.);
#6348=B_SPLINE_CURVE_WITH_KNOTS('',3,(#91134,#91135,#91136,#91137),
 .UNSPECIFIED.,.F.,.F.,(4,4),(9.71445146547012E-17,1.2),.UNSPECIFIED.);
#6349=B_SPLINE_CURVE_WITH_KNOTS('',3,(#91139,#91140,#91141,#91142,#91143,
#91144,#91145),.UNSPECIFIED.,.F.,.F.,(4,3,4),(0.,0.0247995585363106,0.0578656365847246),
 .UNSPECIFIED.);
#6350=B_SPLINE_CURVE_WITH_KNOTS('',3,(#91146,#91147,#91148,#91149),
 .UNSPECIFIED.,.F.,.F.,(4,4),(-1.2,-9.71445146547012E-17),.UNSPECIFIED.);
#6351=B_SPLINE_CURVE_WITH_KNOTS('',3,(#91973,#91974,#91975,#91976,#91977,
#91978,#91979),.UNSPECIFIED.,.F.,.F.,(4,3,4),(0.,0.0330660780458883,0.0578656365803045),
 .UNSPECIFIED.);
#6352=B_SPLINE_CURVE_WITH_KNOTS('',3,(#91981,#91982,#91983,#91984),
 .UNSPECIFIED.,.F.,.F.,(4,4),(-1.49437708898837E-16,1.2),.UNSPECIFIED.);
#6353=B_SPLINE_CURVE_WITH_KNOTS('',3,(#91986,#91987,#91988,#91989,#91990,
#91991,#91992),.UNSPECIFIED.,.F.,.F.,(4,3,4),(0.,0.0247995585344198,0.0578656365803129),
 .UNSPECIFIED.);
#6354=B_SPLINE_CURVE_WITH_KNOTS('',3,(#91993,#91994,#91995,#91996),
 .UNSPECIFIED.,.F.,.F.,(4,4),(-1.2,1.49437708898837E-16),.UNSPECIFIED.);
#6355=B_SPLINE_CURVE_WITH_KNOTS('',3,(#92022,#92023,#92024,#92025,#92026,
#92027,#92028),.UNSPECIFIED.,.F.,.F.,(4,3,4),(0.,0.0330660780483646,0.057865636584638),
 .UNSPECIFIED.);
#6356=B_SPLINE_CURVE_WITH_KNOTS('',3,(#92030,#92031,#92032,#92033),
 .UNSPECIFIED.,.F.,.F.,(4,4),(5.55111512312578E-17,1.2),.UNSPECIFIED.);
#6357=B_SPLINE_CURVE_WITH_KNOTS('',3,(#92035,#92036,#92037,#92038,#92039,
#92040,#92041),.UNSPECIFIED.,.F.,.F.,(4,3,4),(0.,0.0247995585362812,0.057865636584656),
 .UNSPECIFIED.);
#6358=B_SPLINE_CURVE_WITH_KNOTS('',3,(#92042,#92043,#92044,#92045),
 .UNSPECIFIED.,.F.,.F.,(4,4),(-1.2,-5.55111512312578E-17),.UNSPECIFIED.);
#6359=B_SPLINE_CURVE_WITH_KNOTS('',3,(#92869,#92870,#92871,#92872,#92873,
#92874,#92875),.UNSPECIFIED.,.F.,.F.,(4,3,4),(0.,0.0330660780458722,0.0578656365802764),
 .UNSPECIFIED.);
#6360=B_SPLINE_CURVE_WITH_KNOTS('',3,(#92877,#92878,#92879,#92880),
 .UNSPECIFIED.,.F.,.F.,(4,4),(-8.32667268468867E-17,1.2),.UNSPECIFIED.);
#6361=B_SPLINE_CURVE_WITH_KNOTS('',3,(#92882,#92883,#92884,#92885,#92886,
#92887,#92888),.UNSPECIFIED.,.F.,.F.,(4,3,4),(0.,0.0247995585344042,0.0578656365802765),
 .UNSPECIFIED.);
#6362=B_SPLINE_CURVE_WITH_KNOTS('',3,(#92889,#92890,#92891,#92892),
 .UNSPECIFIED.,.F.,.F.,(4,4),(-1.2,8.32667268468867E-17),.UNSPECIFIED.);
#6363=B_SPLINE_CURVE_WITH_KNOTS('',3,(#92918,#92919,#92920,#92921,#92922,
#92923,#92924),.UNSPECIFIED.,.F.,.F.,(4,3,4),(0.,0.0330660780483716,0.0578656365846503),
 .UNSPECIFIED.);
#6364=B_SPLINE_CURVE_WITH_KNOTS('',3,(#92926,#92927,#92928,#92929),
 .UNSPECIFIED.,.F.,.F.,(4,4),(9.71445146547012E-17,1.2),.UNSPECIFIED.);
#6365=B_SPLINE_CURVE_WITH_KNOTS('',3,(#92931,#92932,#92933,#92934,#92935,
#92936,#92937),.UNSPECIFIED.,.F.,.F.,(4,3,4),(0.,0.0247995585362986,0.0578656365846968),
 .UNSPECIFIED.);
#6366=B_SPLINE_CURVE_WITH_KNOTS('',3,(#92938,#92939,#92940,#92941),
 .UNSPECIFIED.,.F.,.F.,(4,4),(-1.2,-9.71445146547012E-17),.UNSPECIFIED.);
#6367=B_SPLINE_CURVE_WITH_KNOTS('',3,(#93765,#93766,#93767,#93768,#93769,
#93770,#93771),.UNSPECIFIED.,.F.,.F.,(4,3,4),(0.,0.0330660780458217,0.057865636580188),
 .UNSPECIFIED.);
#6368=B_SPLINE_CURVE_WITH_KNOTS('',3,(#93773,#93774,#93775,#93776),
 .UNSPECIFIED.,.F.,.F.,(4,4),(-8.32667268468868E-17,1.2),.UNSPECIFIED.);
#6369=B_SPLINE_CURVE_WITH_KNOTS('',3,(#93778,#93779,#93780,#93781,#93782,
#93783,#93784),.UNSPECIFIED.,.F.,.F.,(4,3,4),(0.,0.0247995585343724,0.0578656365802022),
 .UNSPECIFIED.);
#6370=B_SPLINE_CURVE_WITH_KNOTS('',3,(#93785,#93786,#93787,#93788),
 .UNSPECIFIED.,.F.,.F.,(4,4),(-1.2,8.32667268468868E-17),.UNSPECIFIED.);
#6371=B_SPLINE_CURVE_WITH_KNOTS('',3,(#93814,#93815,#93816,#93817,#93818,
#93819,#93820),.UNSPECIFIED.,.F.,.F.,(4,3,4),(0.,0.0330660780484519,0.0578656365847908),
 .UNSPECIFIED.);
#6372=B_SPLINE_CURVE_WITH_KNOTS('',3,(#93822,#93823,#93824,#93825),
 .UNSPECIFIED.,.F.,.F.,(4,4),(-8.32667268468867E-17,1.2),.UNSPECIFIED.);
#6373=B_SPLINE_CURVE_WITH_KNOTS('',3,(#93827,#93828,#93829,#93830,#93831,
#93832,#93833),.UNSPECIFIED.,.F.,.F.,(4,3,4),(0.,0.0247995585363362,0.0578656365847844),
 .UNSPECIFIED.);
#6374=B_SPLINE_CURVE_WITH_KNOTS('',3,(#93834,#93835,#93836,#93837),
 .UNSPECIFIED.,.F.,.F.,(4,4),(-1.2,8.32667268468867E-17),.UNSPECIFIED.);
#6375=B_SPLINE_CURVE_WITH_KNOTS('',3,(#94661,#94662,#94663,#94664,#94665,
#94666,#94667),.UNSPECIFIED.,.F.,.F.,(4,3,4),(0.,0.0330660780458195,0.0578656365801842),
 .UNSPECIFIED.);
#6376=B_SPLINE_CURVE_WITH_KNOTS('',3,(#94669,#94670,#94671,#94672),
 .UNSPECIFIED.,.F.,.F.,(4,4),(2.77555756156289E-17,1.2),.UNSPECIFIED.);
#6377=B_SPLINE_CURVE_WITH_KNOTS('',3,(#94674,#94675,#94676,#94677,#94678,
#94679,#94680),.UNSPECIFIED.,.F.,.F.,(4,3,4),(0.,0.024799558534367,0.0578656365801897),
 .UNSPECIFIED.);
#6378=B_SPLINE_CURVE_WITH_KNOTS('',3,(#94681,#94682,#94683,#94684),
 .UNSPECIFIED.,.F.,.F.,(4,4),(-1.2,-2.77555756156289E-17),.UNSPECIFIED.);
#6379=B_SPLINE_CURVE_WITH_KNOTS('',3,(#94710,#94711,#94712,#94713,#94714,
#94715,#94716),.UNSPECIFIED.,.F.,.F.,(4,3,4),(0.,0.0330660780484102,0.0578656365847178),
 .UNSPECIFIED.);
#6380=B_SPLINE_CURVE_WITH_KNOTS('',3,(#94718,#94719,#94720,#94721),
 .UNSPECIFIED.,.F.,.F.,(4,4),(8.32667268468867E-17,1.2),.UNSPECIFIED.);
#6381=B_SPLINE_CURVE_WITH_KNOTS('',3,(#94723,#94724,#94725,#94726,#94727,
#94728,#94729),.UNSPECIFIED.,.F.,.F.,(4,3,4),(0.,0.0247995585363047,0.057865636584711),
 .UNSPECIFIED.);
#6382=B_SPLINE_CURVE_WITH_KNOTS('',3,(#94730,#94731,#94732,#94733),
 .UNSPECIFIED.,.F.,.F.,(4,4),(-1.2,-8.32667268468867E-17),.UNSPECIFIED.);
#6383=B_SPLINE_CURVE_WITH_KNOTS('',3,(#95557,#95558,#95559,#95560,#95561,
#95562,#95563),.UNSPECIFIED.,.F.,.F.,(4,3,4),(0.,0.033066078045887,0.0578656365803023),
 .UNSPECIFIED.);
#6384=B_SPLINE_CURVE_WITH_KNOTS('',3,(#95565,#95566,#95567,#95568),
 .UNSPECIFIED.,.F.,.F.,(4,4),(2.77555756156289E-17,1.2),.UNSPECIFIED.);
#6385=B_SPLINE_CURVE_WITH_KNOTS('',3,(#95570,#95571,#95572,#95573,#95574,
#95575,#95576),.UNSPECIFIED.,.F.,.F.,(4,3,4),(0.,0.0247995585344129,0.0578656365802968),
 .UNSPECIFIED.);
#6386=B_SPLINE_CURVE_WITH_KNOTS('',3,(#95577,#95578,#95579,#95580),
 .UNSPECIFIED.,.F.,.F.,(4,4),(-1.2,-2.77555756156289E-17),.UNSPECIFIED.);
#6387=B_SPLINE_CURVE_WITH_KNOTS('',3,(#95606,#95607,#95608,#95609,#95610,
#95611,#95612),.UNSPECIFIED.,.F.,.F.,(4,3,4),(0.,0.0330660780484079,0.0578656365847137),
 .UNSPECIFIED.);
#6388=B_SPLINE_CURVE_WITH_KNOTS('',3,(#95614,#95615,#95616,#95617),
 .UNSPECIFIED.,.F.,.F.,(4,4),(5.55111512312578E-17,1.2),.UNSPECIFIED.);
#6389=B_SPLINE_CURVE_WITH_KNOTS('',3,(#95619,#95620,#95621,#95622,#95623,
#95624,#95625),.UNSPECIFIED.,.F.,.F.,(4,3,4),(0.,0.0247995585363057,0.0578656365847134),
 .UNSPECIFIED.);
#6390=B_SPLINE_CURVE_WITH_KNOTS('',3,(#95626,#95627,#95628,#95629),
 .UNSPECIFIED.,.F.,.F.,(4,4),(-1.2,-5.55111512312578E-17),.UNSPECIFIED.);
#6391=B_SPLINE_CURVE_WITH_KNOTS('',3,(#96453,#96454,#96455,#96456,#96457,
#96458,#96459),.UNSPECIFIED.,.F.,.F.,(4,3,4),(0.,0.0330660780458631,0.0578656365802604),
 .UNSPECIFIED.);
#6392=B_SPLINE_CURVE_WITH_KNOTS('',3,(#96461,#96462,#96463,#96464),
 .UNSPECIFIED.,.F.,.F.,(4,4),(-1.38777878078145E-16,1.2),.UNSPECIFIED.);
#6393=B_SPLINE_CURVE_WITH_KNOTS('',3,(#96466,#96467,#96468,#96469,#96470,
#96471,#96472),.UNSPECIFIED.,.F.,.F.,(4,3,4),(0.,0.0247995585343987,0.0578656365802637),
 .UNSPECIFIED.);
#6394=B_SPLINE_CURVE_WITH_KNOTS('',3,(#96473,#96474,#96475,#96476),
 .UNSPECIFIED.,.F.,.F.,(4,4),(-1.2,1.38777878078145E-16),.UNSPECIFIED.);
#6395=B_SPLINE_CURVE_WITH_KNOTS('',3,(#96502,#96503,#96504,#96505,#96506,
#96507,#96508),.UNSPECIFIED.,.F.,.F.,(4,3,4),(0.,0.0330660780483721,0.0578656365846511),
 .UNSPECIFIED.);
#6396=B_SPLINE_CURVE_WITH_KNOTS('',3,(#96510,#96511,#96512,#96513),
 .UNSPECIFIED.,.F.,.F.,(4,4),(2.77555756156289E-17,1.2),.UNSPECIFIED.);
#6397=B_SPLINE_CURVE_WITH_KNOTS('',3,(#96515,#96516,#96517,#96518,#96519,
#96520,#96521),.UNSPECIFIED.,.F.,.F.,(4,3,4),(0.,0.0247995585362904,0.0578656365846776),
 .UNSPECIFIED.);
#6398=B_SPLINE_CURVE_WITH_KNOTS('',3,(#96522,#96523,#96524,#96525),
 .UNSPECIFIED.,.F.,.F.,(4,4),(-1.2,-2.77555756156289E-17),.UNSPECIFIED.);
#6399=B_SPLINE_CURVE_WITH_KNOTS('',3,(#97349,#97350,#97351,#97352,#97353,
#97354,#97355),.UNSPECIFIED.,.F.,.F.,(4,3,4),(0.,0.0330660780458673,0.0578656365802679),
 .UNSPECIFIED.);
#6400=B_SPLINE_CURVE_WITH_KNOTS('',3,(#97357,#97358,#97359,#97360),
 .UNSPECIFIED.,.F.,.F.,(4,4),(0.,1.2),.UNSPECIFIED.);
#6401=B_SPLINE_CURVE_WITH_KNOTS('',3,(#97362,#97363,#97364,#97365,#97366,
#97367,#97368),.UNSPECIFIED.,.F.,.F.,(4,3,4),(0.,0.0247995585344041,0.0578656365802761),
 .UNSPECIFIED.);
#6402=B_SPLINE_CURVE_WITH_KNOTS('',3,(#97369,#97370,#97371,#97372),
 .UNSPECIFIED.,.F.,.F.,(4,4),(-1.2,0.),.UNSPECIFIED.);
#6403=B_SPLINE_CURVE_WITH_KNOTS('',3,(#97398,#97399,#97400,#97401,#97402,
#97403,#97404),.UNSPECIFIED.,.F.,.F.,(4,3,4),(0.,0.0330660780484141,0.0578656365847246),
 .UNSPECIFIED.);
#6404=B_SPLINE_CURVE_WITH_KNOTS('',3,(#97406,#97407,#97408,#97409),
 .UNSPECIFIED.,.F.,.F.,(4,4),(1.66533453693773E-16,1.2),.UNSPECIFIED.);
#6405=B_SPLINE_CURVE_WITH_KNOTS('',3,(#97411,#97412,#97413,#97414,#97415,
#97416,#97417),.UNSPECIFIED.,.F.,.F.,(4,3,4),(0.,0.024799558536313,0.0578656365847304),
 .UNSPECIFIED.);
#6406=B_SPLINE_CURVE_WITH_KNOTS('',3,(#97418,#97419,#97420,#97421),
 .UNSPECIFIED.,.F.,.F.,(4,4),(-1.2,-1.66533453693773E-16),.UNSPECIFIED.);
#6407=B_SPLINE_CURVE_WITH_KNOTS('',3,(#98245,#98246,#98247,#98248,#98249,
#98250,#98251),.UNSPECIFIED.,.F.,.F.,(4,3,4),(0.,0.0330660780458716,0.0578656365802753),
 .UNSPECIFIED.);
#6408=B_SPLINE_CURVE_WITH_KNOTS('',3,(#98253,#98254,#98255,#98256),
 .UNSPECIFIED.,.F.,.F.,(4,4),(-8.32667268468867E-17,1.2),.UNSPECIFIED.);
#6409=B_SPLINE_CURVE_WITH_KNOTS('',3,(#98258,#98259,#98260,#98261,#98262,
#98263,#98264),.UNSPECIFIED.,.F.,.F.,(4,3,4),(0.,0.0247995585344033,0.0578656365802743),
 .UNSPECIFIED.);
#6410=B_SPLINE_CURVE_WITH_KNOTS('',3,(#98265,#98266,#98267,#98268),
 .UNSPECIFIED.,.F.,.F.,(4,4),(-1.2,8.32667268468867E-17),.UNSPECIFIED.);
#6411=B_SPLINE_CURVE_WITH_KNOTS('',3,(#98294,#98295,#98296,#98297,#98298,
#98299,#98300),.UNSPECIFIED.,.F.,.F.,(4,3,4),(0.,0.0330660780484192,0.0578656365847337),
 .UNSPECIFIED.);
#6412=B_SPLINE_CURVE_WITH_KNOTS('',3,(#98302,#98303,#98304,#98305),
 .UNSPECIFIED.,.F.,.F.,(4,4),(9.71445146547012E-17,1.2),.UNSPECIFIED.);
#6413=B_SPLINE_CURVE_WITH_KNOTS('',3,(#98307,#98308,#98309,#98310,#98311,
#98312,#98313),.UNSPECIFIED.,.F.,.F.,(4,3,4),(0.,0.0247995585363099,0.0578656365847232),
 .UNSPECIFIED.);
#6414=B_SPLINE_CURVE_WITH_KNOTS('',3,(#98314,#98315,#98316,#98317),
 .UNSPECIFIED.,.F.,.F.,(4,4),(-1.2,-9.71445146547012E-17),.UNSPECIFIED.);
#6415=B_SPLINE_CURVE_WITH_KNOTS('',3,(#99141,#99142,#99143,#99144,#99145,
#99146,#99147),.UNSPECIFIED.,.F.,.F.,(4,3,4),(0.,0.0330660780458584,0.0578656365802523),
 .UNSPECIFIED.);
#6416=B_SPLINE_CURVE_WITH_KNOTS('',3,(#99149,#99150,#99151,#99152),
 .UNSPECIFIED.,.F.,.F.,(4,4),(-2.03133674691991E-35,1.2),.UNSPECIFIED.);
#6417=B_SPLINE_CURVE_WITH_KNOTS('',3,(#99154,#99155,#99156,#99157,#99158,
#99159,#99160),.UNSPECIFIED.,.F.,.F.,(4,3,4),(0.,0.0247995585343932,0.0578656365802508),
 .UNSPECIFIED.);
#6418=B_SPLINE_CURVE_WITH_KNOTS('',3,(#99161,#99162,#99163,#99164),
 .UNSPECIFIED.,.F.,.F.,(4,4),(-1.2,2.03133674691991E-35),.UNSPECIFIED.);
#6419=B_SPLINE_CURVE_WITH_KNOTS('',3,(#99190,#99191,#99192,#99193,#99194,
#99195,#99196),.UNSPECIFIED.,.F.,.F.,(4,3,4),(0.,0.033066078048434,0.0578656365847594),
 .UNSPECIFIED.);
#6420=B_SPLINE_CURVE_WITH_KNOTS('',3,(#99198,#99199,#99200,#99201),
 .UNSPECIFIED.,.F.,.F.,(4,4),(-1.83155496676632E-16,1.2),.UNSPECIFIED.);
#6421=B_SPLINE_CURVE_WITH_KNOTS('',3,(#99203,#99204,#99205,#99206,#99207,
#99208,#99209),.UNSPECIFIED.,.F.,.F.,(4,3,4),(0.,0.0247995585363058,0.0578656365847137),
 .UNSPECIFIED.);
#6422=B_SPLINE_CURVE_WITH_KNOTS('',3,(#99210,#99211,#99212,#99213),
 .UNSPECIFIED.,.F.,.F.,(4,4),(-1.2,1.83155496676632E-16),.UNSPECIFIED.);
#6423=B_SPLINE_CURVE_WITH_KNOTS('',3,(#100037,#100038,#100039,#100040,#100041,
#100042,#100043),.UNSPECIFIED.,.F.,.F.,(4,3,4),(0.,0.0330660780458696,0.0578656365802718),
 .UNSPECIFIED.);
#6424=B_SPLINE_CURVE_WITH_KNOTS('',3,(#100045,#100046,#100047,#100048),
 .UNSPECIFIED.,.F.,.F.,(4,4),(-1.38777878078145E-16,1.2),.UNSPECIFIED.);
#6425=B_SPLINE_CURVE_WITH_KNOTS('',3,(#100050,#100051,#100052,#100053,#100054,
#100055,#100056),.UNSPECIFIED.,.F.,.F.,(4,3,4),(0.,0.0247995585343985,0.0578656365802632),
 .UNSPECIFIED.);
#6426=B_SPLINE_CURVE_WITH_KNOTS('',3,(#100057,#100058,#100059,#100060),
 .UNSPECIFIED.,.F.,.F.,(4,4),(-1.2,1.38777878078145E-16),.UNSPECIFIED.);
#6427=B_SPLINE_CURVE_WITH_KNOTS('',3,(#100086,#100087,#100088,#100089,#100090,
#100091,#100092),.UNSPECIFIED.,.F.,.F.,(4,3,4),(0.,0.0330660780483983,0.0578656365846971),
 .UNSPECIFIED.);
#6428=B_SPLINE_CURVE_WITH_KNOTS('',3,(#100094,#100095,#100096,#100097),
 .UNSPECIFIED.,.F.,.F.,(4,4),(1.66533453693773E-16,1.2),.UNSPECIFIED.);
#6429=B_SPLINE_CURVE_WITH_KNOTS('',3,(#100099,#100100,#100101,#100102,#100103,
#100104,#100105),.UNSPECIFIED.,.F.,.F.,(4,3,4),(0.,0.0247995585362993,0.0578656365846983),
 .UNSPECIFIED.);
#6430=B_SPLINE_CURVE_WITH_KNOTS('',3,(#100106,#100107,#100108,#100109),
 .UNSPECIFIED.,.F.,.F.,(4,4),(-1.2,-1.66533453693773E-16),.UNSPECIFIED.);
#6431=B_SPLINE_CURVE_WITH_KNOTS('',3,(#100933,#100934,#100935,#100936,#100937,
#100938,#100939),.UNSPECIFIED.,.F.,.F.,(4,3,4),(0.,0.0330660780458496,0.0578656365802369),
 .UNSPECIFIED.);
#6432=B_SPLINE_CURVE_WITH_KNOTS('',3,(#100941,#100942,#100943,#100944),
 .UNSPECIFIED.,.F.,.F.,(4,4),(0.,1.2),.UNSPECIFIED.);
#6433=B_SPLINE_CURVE_WITH_KNOTS('',3,(#100946,#100947,#100948,#100949,#100950,
#100951,#100952),.UNSPECIFIED.,.F.,.F.,(4,3,4),(0.,0.0247995585343804,0.0578656365802209),
 .UNSPECIFIED.);
#6434=B_SPLINE_CURVE_WITH_KNOTS('',3,(#100953,#100954,#100955,#100956),
 .UNSPECIFIED.,.F.,.F.,(4,4),(-1.2,0.),.UNSPECIFIED.);
#6435=B_SPLINE_CURVE_WITH_KNOTS('',3,(#100982,#100983,#100984,#100985,#100986,
#100987,#100988),.UNSPECIFIED.,.F.,.F.,(4,3,4),(0.,0.0330660780484024,0.0578656365847041),
 .UNSPECIFIED.);
#6436=B_SPLINE_CURVE_WITH_KNOTS('',3,(#100990,#100991,#100992,#100993),
 .UNSPECIFIED.,.F.,.F.,(4,4),(-1.38777878078145E-16,1.2),.UNSPECIFIED.);
#6437=B_SPLINE_CURVE_WITH_KNOTS('',3,(#100995,#100996,#100997,#100998,#100999,
#101000,#101001),.UNSPECIFIED.,.F.,.F.,(4,3,4),(0.,0.0247995585362999,0.0578656365846998),
 .UNSPECIFIED.);
#6438=B_SPLINE_CURVE_WITH_KNOTS('',3,(#101002,#101003,#101004,#101005),
 .UNSPECIFIED.,.F.,.F.,(4,4),(-1.2,1.38777878078145E-16),.UNSPECIFIED.);
#6439=B_SPLINE_CURVE_WITH_KNOTS('',3,(#101829,#101830,#101831,#101832,#101833,
#101834,#101835),.UNSPECIFIED.,.F.,.F.,(4,3,4),(0.,0.033066078045876,0.057865636580283),
 .UNSPECIFIED.);
#6440=B_SPLINE_CURVE_WITH_KNOTS('',3,(#101837,#101838,#101839,#101840),
 .UNSPECIFIED.,.F.,.F.,(4,4),(-1.88097848788491E-36,1.2),.UNSPECIFIED.);
#6441=B_SPLINE_CURVE_WITH_KNOTS('',3,(#101842,#101843,#101844,#101845,#101846,
#101847,#101848),.UNSPECIFIED.,.F.,.F.,(4,3,4),(0.,0.0247995585344058,0.0578656365802801),
 .UNSPECIFIED.);
#6442=B_SPLINE_CURVE_WITH_KNOTS('',3,(#101849,#101850,#101851,#101852),
 .UNSPECIFIED.,.F.,.F.,(4,4),(-1.2,1.88097848788491E-36),.UNSPECIFIED.);
#6443=B_SPLINE_CURVE_WITH_KNOTS('',3,(#101878,#101879,#101880,#101881,#101882,
#101883,#101884),.UNSPECIFIED.,.F.,.F.,(4,3,4),(0.,0.0330660780484209,0.0578656365847367),
 .UNSPECIFIED.);
#6444=B_SPLINE_CURVE_WITH_KNOTS('',3,(#101886,#101887,#101888,#101889),
 .UNSPECIFIED.,.F.,.F.,(4,4),(2.77555756156289E-17,1.2),.UNSPECIFIED.);
#6445=B_SPLINE_CURVE_WITH_KNOTS('',3,(#101891,#101892,#101893,#101894,#101895,
#101896,#101897),.UNSPECIFIED.,.F.,.F.,(4,3,4),(0.,0.0247995585363132,0.0578656365847308),
 .UNSPECIFIED.);
#6446=B_SPLINE_CURVE_WITH_KNOTS('',3,(#101898,#101899,#101900,#101901),
 .UNSPECIFIED.,.F.,.F.,(4,4),(-1.2,-2.77555756156289E-17),.UNSPECIFIED.);
#6447=B_SPLINE_CURVE_WITH_KNOTS('',3,(#102725,#102726,#102727,#102728,#102729,
#102730,#102731),.UNSPECIFIED.,.F.,.F.,(4,3,4),(0.,0.0330660780458869,0.0578656365803021),
 .UNSPECIFIED.);
#6448=B_SPLINE_CURVE_WITH_KNOTS('',3,(#102733,#102734,#102735,#102736),
 .UNSPECIFIED.,.F.,.F.,(4,4),(-1.38777878078145E-16,1.2),.UNSPECIFIED.);
#6449=B_SPLINE_CURVE_WITH_KNOTS('',3,(#102738,#102739,#102740,#102741,#102742,
#102743,#102744),.UNSPECIFIED.,.F.,.F.,(4,3,4),(0.,0.0247995585344142,0.0578656365802999),
 .UNSPECIFIED.);
#6450=B_SPLINE_CURVE_WITH_KNOTS('',3,(#102745,#102746,#102747,#102748),
 .UNSPECIFIED.,.F.,.F.,(4,4),(-1.2,1.38777878078145E-16),.UNSPECIFIED.);
#6451=B_SPLINE_CURVE_WITH_KNOTS('',3,(#102774,#102775,#102776,#102777,#102778,
#102779,#102780),.UNSPECIFIED.,.F.,.F.,(4,3,4),(0.,0.0330660780484272,0.0578656365847475),
 .UNSPECIFIED.);
#6452=B_SPLINE_CURVE_WITH_KNOTS('',3,(#102782,#102783,#102784,#102785),
 .UNSPECIFIED.,.F.,.F.,(4,4),(0.,1.2),.UNSPECIFIED.);
#6453=B_SPLINE_CURVE_WITH_KNOTS('',3,(#102787,#102788,#102789,#102790,#102791,
#102792,#102793),.UNSPECIFIED.,.F.,.F.,(4,3,4),(0.,0.0247995585363195,0.0578656365847456),
 .UNSPECIFIED.);
#6454=B_SPLINE_CURVE_WITH_KNOTS('',3,(#102794,#102795,#102796,#102797),
 .UNSPECIFIED.,.F.,.F.,(4,4),(-1.2,0.),.UNSPECIFIED.);
#6455=B_SPLINE_CURVE_WITH_KNOTS('',3,(#103621,#103622,#103623,#103624,#103625,
#103626,#103627),.UNSPECIFIED.,.F.,.F.,(4,3,4),(0.,0.0330660780458254,0.0578656365801945),
 .UNSPECIFIED.);
#6456=B_SPLINE_CURVE_WITH_KNOTS('',3,(#103629,#103630,#103631,#103632),
 .UNSPECIFIED.,.F.,.F.,(4,4),(0.,1.2),.UNSPECIFIED.);
#6457=B_SPLINE_CURVE_WITH_KNOTS('',3,(#103634,#103635,#103636,#103637,#103638,
#103639,#103640),.UNSPECIFIED.,.F.,.F.,(4,3,4),(0.,0.0247995585343927,0.0578656365802495),
 .UNSPECIFIED.);
#6458=B_SPLINE_CURVE_WITH_KNOTS('',3,(#103641,#103642,#103643,#103644),
 .UNSPECIFIED.,.F.,.F.,(4,4),(-1.2,0.),.UNSPECIFIED.);
#6459=B_SPLINE_CURVE_WITH_KNOTS('',3,(#103670,#103671,#103672,#103673,#103674,
#103675,#103676),.UNSPECIFIED.,.F.,.F.,(4,3,4),(0.,0.0330660780484286,0.05786563658475),
 .UNSPECIFIED.);
#6460=B_SPLINE_CURVE_WITH_KNOTS('',3,(#103678,#103679,#103680,#103681),
 .UNSPECIFIED.,.F.,.F.,(4,4),(9.71445146547012E-17,1.2),.UNSPECIFIED.);
#6461=B_SPLINE_CURVE_WITH_KNOTS('',3,(#103683,#103684,#103685,#103686,#103687,
#103688,#103689),.UNSPECIFIED.,.F.,.F.,(4,3,4),(0.,0.024799558536323,0.0578656365847537),
 .UNSPECIFIED.);
#6462=B_SPLINE_CURVE_WITH_KNOTS('',3,(#103690,#103691,#103692,#103693),
 .UNSPECIFIED.,.F.,.F.,(4,4),(-1.2,-9.71445146547012E-17),.UNSPECIFIED.);
#6463=B_SPLINE_CURVE_WITH_KNOTS('',3,(#104517,#104518,#104519,#104520,#104521,
#104522,#104523),.UNSPECIFIED.,.F.,.F.,(4,3,4),(0.,0.0330660780458335,0.0578656365802087),
 .UNSPECIFIED.);
#6464=B_SPLINE_CURVE_WITH_KNOTS('',3,(#104525,#104526,#104527,#104528),
 .UNSPECIFIED.,.F.,.F.,(4,4),(-5.55111512312578E-17,1.2),.UNSPECIFIED.);
#6465=B_SPLINE_CURVE_WITH_KNOTS('',3,(#104530,#104531,#104532,#104533,#104534,
#104535,#104536),.UNSPECIFIED.,.F.,.F.,(4,3,4),(0.,0.0247995585343757,0.0578656365802101),
 .UNSPECIFIED.);
#6466=B_SPLINE_CURVE_WITH_KNOTS('',3,(#104537,#104538,#104539,#104540),
 .UNSPECIFIED.,.F.,.F.,(4,4),(-1.2,5.55111512312578E-17),.UNSPECIFIED.);
#6467=B_SPLINE_CURVE_WITH_KNOTS('',3,(#104566,#104567,#104568,#104569,#104570,
#104571,#104572),.UNSPECIFIED.,.F.,.F.,(4,3,4),(0.,0.0330660780484165,0.0578656365847288),
 .UNSPECIFIED.);
#6468=B_SPLINE_CURVE_WITH_KNOTS('',3,(#104574,#104575,#104576,#104577),
 .UNSPECIFIED.,.F.,.F.,(4,4),(9.71445146547012E-17,1.2),.UNSPECIFIED.);
#6469=B_SPLINE_CURVE_WITH_KNOTS('',3,(#104579,#104580,#104581,#104582,#104583,
#104584,#104585),.UNSPECIFIED.,.F.,.F.,(4,3,4),(0.,0.0247995585363161,0.0578656365847375),
 .UNSPECIFIED.);
#6470=B_SPLINE_CURVE_WITH_KNOTS('',3,(#104586,#104587,#104588,#104589),
 .UNSPECIFIED.,.F.,.F.,(4,4),(-1.2,-9.71445146547012E-17),.UNSPECIFIED.);
#6471=B_SPLINE_CURVE_WITH_KNOTS('',3,(#105413,#105414,#105415,#105416,#105417,
#105418,#105419),.UNSPECIFIED.,.F.,.F.,(4,3,4),(0.,0.0330660780458765,0.0578656365802839),
 .UNSPECIFIED.);
#6472=B_SPLINE_CURVE_WITH_KNOTS('',3,(#105421,#105422,#105423,#105424),
 .UNSPECIFIED.,.F.,.F.,(4,4),(-1.41402172924014E-16,1.2),.UNSPECIFIED.);
#6473=B_SPLINE_CURVE_WITH_KNOTS('',3,(#105426,#105427,#105428,#105429,#105430,
#105431,#105432),.UNSPECIFIED.,.F.,.F.,(4,3,4),(0.,0.0247995585344063,0.0578656365802813),
 .UNSPECIFIED.);
#6474=B_SPLINE_CURVE_WITH_KNOTS('',3,(#105433,#105434,#105435,#105436),
 .UNSPECIFIED.,.F.,.F.,(4,4),(-1.2,1.41402172924014E-16),.UNSPECIFIED.);
#6475=B_SPLINE_CURVE_WITH_KNOTS('',3,(#105462,#105463,#105464,#105465,#105466,
#105467,#105468),.UNSPECIFIED.,.F.,.F.,(4,3,4),(0.,0.0330660780484353,0.0578656365847618),
 .UNSPECIFIED.);
#6476=B_SPLINE_CURVE_WITH_KNOTS('',3,(#105470,#105471,#105472,#105473),
 .UNSPECIFIED.,.F.,.F.,(4,4),(0.,1.2),.UNSPECIFIED.);
#6477=B_SPLINE_CURVE_WITH_KNOTS('',3,(#105475,#105476,#105477,#105478,#105479,
#105480,#105481),.UNSPECIFIED.,.F.,.F.,(4,3,4),(0.,0.0247995585363296,0.057865636584769),
 .UNSPECIFIED.);
#6478=B_SPLINE_CURVE_WITH_KNOTS('',3,(#105482,#105483,#105484,#105485),
 .UNSPECIFIED.,.F.,.F.,(4,4),(-1.2,0.),.UNSPECIFIED.);
#6479=B_SPLINE_CURVE_WITH_KNOTS('',3,(#106309,#106310,#106311,#106312,#106313,
#106314,#106315),.UNSPECIFIED.,.F.,.F.,(4,3,4),(0.,0.0330660780458757,0.0578656365802824),
 .UNSPECIFIED.);
#6480=B_SPLINE_CURVE_WITH_KNOTS('',3,(#106317,#106318,#106319,#106320),
 .UNSPECIFIED.,.F.,.F.,(4,4),(-1.11022302462516E-16,1.2),.UNSPECIFIED.);
#6481=B_SPLINE_CURVE_WITH_KNOTS('',3,(#106322,#106323,#106324,#106325,#106326,
#106327,#106328),.UNSPECIFIED.,.F.,.F.,(4,3,4),(0.,0.0247995585344084,0.0578656365802862),
 .UNSPECIFIED.);
#6482=B_SPLINE_CURVE_WITH_KNOTS('',3,(#106329,#106330,#106331,#106332),
 .UNSPECIFIED.,.F.,.F.,(4,4),(-1.2,1.11022302462516E-16),.UNSPECIFIED.);
#6483=B_SPLINE_CURVE_WITH_KNOTS('',3,(#106358,#106359,#106360,#106361,#106362,
#106363,#106364),.UNSPECIFIED.,.F.,.F.,(4,3,4),(0.,0.0330660780484577,0.057865636584801),
 .UNSPECIFIED.);
#6484=B_SPLINE_CURVE_WITH_KNOTS('',3,(#106366,#106367,#106368,#106369),
 .UNSPECIFIED.,.F.,.F.,(4,4),(1.38777878078145E-16,1.2),.UNSPECIFIED.);
#6485=B_SPLINE_CURVE_WITH_KNOTS('',3,(#106371,#106372,#106373,#106374,#106375,
#106376,#106377),.UNSPECIFIED.,.F.,.F.,(4,3,4),(0.,0.0247995585363564,0.0578656365848316),
 .UNSPECIFIED.);
#6486=B_SPLINE_CURVE_WITH_KNOTS('',3,(#106378,#106379,#106380,#106381),
 .UNSPECIFIED.,.F.,.F.,(4,4),(-1.2,-1.38777878078145E-16),.UNSPECIFIED.);
#6487=B_SPLINE_CURVE_WITH_KNOTS('',3,(#107205,#107206,#107207,#107208,#107209,
#107210,#107211),.UNSPECIFIED.,.F.,.F.,(4,3,4),(0.,0.0330660780458936,0.0578656365803137),
 .UNSPECIFIED.);
#6488=B_SPLINE_CURVE_WITH_KNOTS('',3,(#107213,#107214,#107215,#107216),
 .UNSPECIFIED.,.F.,.F.,(4,4),(2.77555756156289E-17,1.2),.UNSPECIFIED.);
#6489=B_SPLINE_CURVE_WITH_KNOTS('',3,(#107218,#107219,#107220,#107221,#107222,
#107223,#107224),.UNSPECIFIED.,.F.,.F.,(4,3,4),(0.,0.0247995585344178,0.0578656365803083),
 .UNSPECIFIED.);
#6490=B_SPLINE_CURVE_WITH_KNOTS('',3,(#107225,#107226,#107227,#107228),
 .UNSPECIFIED.,.F.,.F.,(4,4),(-1.2,-2.77555756156289E-17),.UNSPECIFIED.);
#6491=B_SPLINE_CURVE_WITH_KNOTS('',3,(#107254,#107255,#107256,#107257,#107258,
#107259,#107260),.UNSPECIFIED.,.F.,.F.,(4,3,4),(0.,0.0330660780484244,0.0578656365847427),
 .UNSPECIFIED.);
#6492=B_SPLINE_CURVE_WITH_KNOTS('',3,(#107262,#107263,#107264,#107265),
 .UNSPECIFIED.,.F.,.F.,(4,4),(0.,1.2),.UNSPECIFIED.);
#6493=B_SPLINE_CURVE_WITH_KNOTS('',3,(#107267,#107268,#107269,#107270,#107271,
#107272,#107273),.UNSPECIFIED.,.F.,.F.,(4,3,4),(0.,0.0247995585363162,0.0578656365847378),
 .UNSPECIFIED.);
#6494=B_SPLINE_CURVE_WITH_KNOTS('',3,(#107274,#107275,#107276,#107277),
 .UNSPECIFIED.,.F.,.F.,(4,4),(-1.2,0.),.UNSPECIFIED.);
#6495=B_SPLINE_CURVE_WITH_KNOTS('',3,(#108101,#108102,#108103,#108104,#108105,
#108106,#108107),.UNSPECIFIED.,.F.,.F.,(4,3,4),(0.,0.0330660780458305,0.0578656365802034),
 .UNSPECIFIED.);
#6496=B_SPLINE_CURVE_WITH_KNOTS('',3,(#108109,#108110,#108111,#108112),
 .UNSPECIFIED.,.F.,.F.,(4,4),(2.77555756156289E-17,1.2),.UNSPECIFIED.);
#6497=B_SPLINE_CURVE_WITH_KNOTS('',3,(#108114,#108115,#108116,#108117,#108118,
#108119,#108120),.UNSPECIFIED.,.F.,.F.,(4,3,4),(0.,0.0247995585343651,0.0578656365801852),
 .UNSPECIFIED.);
#6498=B_SPLINE_CURVE_WITH_KNOTS('',3,(#108121,#108122,#108123,#108124),
 .UNSPECIFIED.,.F.,.F.,(4,4),(-1.2,-2.77555756156289E-17),.UNSPECIFIED.);
#6499=B_SPLINE_CURVE_WITH_KNOTS('',3,(#108150,#108151,#108152,#108153,#108154,
#108155,#108156),.UNSPECIFIED.,.F.,.F.,(4,3,4),(0.,0.0330660780483646,0.057865636584638),
 .UNSPECIFIED.);
#6500=B_SPLINE_CURVE_WITH_KNOTS('',3,(#108158,#108159,#108160,#108161),
 .UNSPECIFIED.,.F.,.F.,(4,4),(5.55111512312578E-17,1.2),.UNSPECIFIED.);
#6501=B_SPLINE_CURVE_WITH_KNOTS('',3,(#108163,#108164,#108165,#108166,#108167,
#108168,#108169),.UNSPECIFIED.,.F.,.F.,(4,3,4),(0.,0.0247995585362812,0.057865636584656),
 .UNSPECIFIED.);
#6502=B_SPLINE_CURVE_WITH_KNOTS('',3,(#108170,#108171,#108172,#108173),
 .UNSPECIFIED.,.F.,.F.,(4,4),(-1.2,-5.55111512312578E-17),.UNSPECIFIED.);
#6503=B_SPLINE_CURVE_WITH_KNOTS('',3,(#108997,#108998,#108999,#109000,#109001,
#109002,#109003),.UNSPECIFIED.,.F.,.F.,(4,3,4),(0.,0.0330660780458722,0.0578656365802764),
 .UNSPECIFIED.);
#6504=B_SPLINE_CURVE_WITH_KNOTS('',3,(#109005,#109006,#109007,#109008),
 .UNSPECIFIED.,.F.,.F.,(4,4),(-8.32667268468867E-17,1.2),.UNSPECIFIED.);
#6505=B_SPLINE_CURVE_WITH_KNOTS('',3,(#109010,#109011,#109012,#109013,#109014,
#109015,#109016),.UNSPECIFIED.,.F.,.F.,(4,3,4),(0.,0.0247995585344042,0.0578656365802765),
 .UNSPECIFIED.);
#6506=B_SPLINE_CURVE_WITH_KNOTS('',3,(#109017,#109018,#109019,#109020),
 .UNSPECIFIED.,.F.,.F.,(4,4),(-1.2,8.32667268468867E-17),.UNSPECIFIED.);
#6507=B_SPLINE_CURVE_WITH_KNOTS('',3,(#109046,#109047,#109048,#109049,#109050,
#109051,#109052),.UNSPECIFIED.,.F.,.F.,(4,3,4),(0.,0.033066078048439,0.0578656365847682),
 .UNSPECIFIED.);
#6508=B_SPLINE_CURVE_WITH_KNOTS('',3,(#109054,#109055,#109056,#109057),
 .UNSPECIFIED.,.F.,.F.,(4,4),(1.66533453693773E-16,1.2),.UNSPECIFIED.);
#6509=B_SPLINE_CURVE_WITH_KNOTS('',3,(#109059,#109060,#109061,#109062,#109063,
#109064,#109065),.UNSPECIFIED.,.F.,.F.,(4,3,4),(0.,0.0247995585363292,0.0578656365847682),
 .UNSPECIFIED.);
#6510=B_SPLINE_CURVE_WITH_KNOTS('',3,(#109066,#109067,#109068,#109069),
 .UNSPECIFIED.,.F.,.F.,(4,4),(-1.2,-1.66533453693773E-16),.UNSPECIFIED.);
#6511=B_SPLINE_CURVE_WITH_KNOTS('',3,(#109893,#109894,#109895,#109896,#109897,
#109898,#109899),.UNSPECIFIED.,.F.,.F.,(4,3,4),(0.,0.033066078045871,0.0578656365802742),
 .UNSPECIFIED.);
#6512=B_SPLINE_CURVE_WITH_KNOTS('',3,(#109901,#109902,#109903,#109904),
 .UNSPECIFIED.,.F.,.F.,(4,4),(-1.47525527564366E-17,1.2),.UNSPECIFIED.);
#6513=B_SPLINE_CURVE_WITH_KNOTS('',3,(#109906,#109907,#109908,#109909,#109910,
#109911,#109912),.UNSPECIFIED.,.F.,.F.,(4,3,4),(0.,0.0247995585344122,0.057865636580295),
 .UNSPECIFIED.);
#6514=B_SPLINE_CURVE_WITH_KNOTS('',3,(#109913,#109914,#109915,#109916),
 .UNSPECIFIED.,.F.,.F.,(4,4),(-1.2,1.47525527564366E-17),.UNSPECIFIED.);
#6515=B_SPLINE_CURVE_WITH_KNOTS('',3,(#109942,#109943,#109944,#109945,#109946,
#109947,#109948),.UNSPECIFIED.,.F.,.F.,(4,3,4),(0.,0.0330660780484426,0.0578656365847746),
 .UNSPECIFIED.);
#6516=B_SPLINE_CURVE_WITH_KNOTS('',3,(#109950,#109951,#109952,#109953),
 .UNSPECIFIED.,.F.,.F.,(4,4),(9.71445146547012E-17,1.2),.UNSPECIFIED.);
#6517=B_SPLINE_CURVE_WITH_KNOTS('',3,(#109955,#109956,#109957,#109958,#109959,
#109960,#109961),.UNSPECIFIED.,.F.,.F.,(4,3,4),(0.,0.0247995585363433,0.0578656365848011),
 .UNSPECIFIED.);
#6518=B_SPLINE_CURVE_WITH_KNOTS('',3,(#109962,#109963,#109964,#109965),
 .UNSPECIFIED.,.F.,.F.,(4,4),(-1.2,-9.71445146547012E-17),.UNSPECIFIED.);
#6519=B_SPLINE_CURVE_WITH_KNOTS('',3,(#110789,#110790,#110791,#110792,#110793,
#110794,#110795),.UNSPECIFIED.,.F.,.F.,(4,3,4),(0.,0.0330660780458487,0.0578656365802352),
 .UNSPECIFIED.);
#6520=B_SPLINE_CURVE_WITH_KNOTS('',3,(#110797,#110798,#110799,#110800),
 .UNSPECIFIED.,.F.,.F.,(4,4),(2.77555756156289E-17,1.2),.UNSPECIFIED.);
#6521=B_SPLINE_CURVE_WITH_KNOTS('',3,(#110802,#110803,#110804,#110805,#110806,
#110807,#110808),.UNSPECIFIED.,.F.,.F.,(4,3,4),(0.,0.0247995585343886,0.05786563658024),
 .UNSPECIFIED.);
#6522=B_SPLINE_CURVE_WITH_KNOTS('',3,(#110809,#110810,#110811,#110812),
 .UNSPECIFIED.,.F.,.F.,(4,4),(-1.2,-2.77555756156289E-17),.UNSPECIFIED.);
#6523=B_SPLINE_CURVE_WITH_KNOTS('',3,(#110838,#110839,#110840,#110841,#110842,
#110843,#110844),.UNSPECIFIED.,.F.,.F.,(4,3,4),(0.,0.0330660780484081,0.0578656365847142),
 .UNSPECIFIED.);
#6524=B_SPLINE_CURVE_WITH_KNOTS('',3,(#110846,#110847,#110848,#110849),
 .UNSPECIFIED.,.F.,.F.,(4,4),(0.,1.2),.UNSPECIFIED.);
#6525=B_SPLINE_CURVE_WITH_KNOTS('',3,(#110851,#110852,#110853,#110854,#110855,
#110856,#110857),.UNSPECIFIED.,.F.,.F.,(4,3,4),(0.,0.0247995585363053,0.0578656365847123),
 .UNSPECIFIED.);
#6526=B_SPLINE_CURVE_WITH_KNOTS('',3,(#110858,#110859,#110860,#110861),
 .UNSPECIFIED.,.F.,.F.,(4,4),(-1.2,0.),.UNSPECIFIED.);
#6527=B_SPLINE_CURVE_WITH_KNOTS('',3,(#111685,#111686,#111687,#111688,#111689,
#111690,#111691),.UNSPECIFIED.,.F.,.F.,(4,3,4),(0.,0.0330660780458939,0.0578656365803143),
 .UNSPECIFIED.);
#6528=B_SPLINE_CURVE_WITH_KNOTS('',3,(#111693,#111694,#111695,#111696),
 .UNSPECIFIED.,.F.,.F.,(4,4),(-8.32667268468867E-17,1.2),.UNSPECIFIED.);
#6529=B_SPLINE_CURVE_WITH_KNOTS('',3,(#111698,#111699,#111700,#111701,#111702,
#111703,#111704),.UNSPECIFIED.,.F.,.F.,(4,3,4),(0.,0.0247995585344063,0.0578656365802814),
 .UNSPECIFIED.);
#6530=B_SPLINE_CURVE_WITH_KNOTS('',3,(#111705,#111706,#111707,#111708),
 .UNSPECIFIED.,.F.,.F.,(4,4),(-1.2,8.32667268468867E-17),.UNSPECIFIED.);
#6531=B_SPLINE_CURVE_WITH_KNOTS('',3,(#111734,#111735,#111736,#111737,#111738,
#111739,#111740),.UNSPECIFIED.,.F.,.F.,(4,3,4),(0.,0.0330660780483969,0.0578656365846947),
 .UNSPECIFIED.);
#6532=B_SPLINE_CURVE_WITH_KNOTS('',3,(#111742,#111743,#111744,#111745),
 .UNSPECIFIED.,.F.,.F.,(4,4),(-5.63859161805989E-17,1.2),.UNSPECIFIED.);
#6533=B_SPLINE_CURVE_WITH_KNOTS('',3,(#111747,#111748,#111749,#111750,#111751,
#111752,#111753),.UNSPECIFIED.,.F.,.F.,(4,3,4),(0.,0.0247995585362953,0.0578656365846891),
 .UNSPECIFIED.);
#6534=B_SPLINE_CURVE_WITH_KNOTS('',3,(#111754,#111755,#111756,#111757),
 .UNSPECIFIED.,.F.,.F.,(4,4),(-1.2,5.63859161805989E-17),.UNSPECIFIED.);
#6535=B_SPLINE_CURVE_WITH_KNOTS('',3,(#112581,#112582,#112583,#112584,#112585,
#112586,#112587),.UNSPECIFIED.,.F.,.F.,(4,3,4),(0.,0.0330660780458488,0.0578656365802353),
 .UNSPECIFIED.);
#6536=B_SPLINE_CURVE_WITH_KNOTS('',3,(#112589,#112590,#112591,#112592),
 .UNSPECIFIED.,.F.,.F.,(4,4),(-3.76195697576961E-36,1.2),.UNSPECIFIED.);
#6537=B_SPLINE_CURVE_WITH_KNOTS('',3,(#112594,#112595,#112596,#112597,#112598,
#112599,#112600),.UNSPECIFIED.,.F.,.F.,(4,3,4),(0.,0.0247995585344019,0.0578656365802711),
 .UNSPECIFIED.);
#6538=B_SPLINE_CURVE_WITH_KNOTS('',3,(#112601,#112602,#112603,#112604),
 .UNSPECIFIED.,.F.,.F.,(4,4),(-1.2,3.76195697576961E-36),.UNSPECIFIED.);
#6539=B_SPLINE_CURVE_WITH_KNOTS('',3,(#112630,#112631,#112632,#112633,#112634,
#112635,#112636),.UNSPECIFIED.,.F.,.F.,(4,3,4),(0.,0.0330660780483721,0.0578656365846511),
 .UNSPECIFIED.);
#6540=B_SPLINE_CURVE_WITH_KNOTS('',3,(#112638,#112639,#112640,#112641),
 .UNSPECIFIED.,.F.,.F.,(4,4),(2.77555756156289E-17,1.2),.UNSPECIFIED.);
#6541=B_SPLINE_CURVE_WITH_KNOTS('',3,(#112643,#112644,#112645,#112646,#112647,
#112648,#112649),.UNSPECIFIED.,.F.,.F.,(4,3,4),(0.,0.0247995585362904,0.0578656365846776),
 .UNSPECIFIED.);
#6542=B_SPLINE_CURVE_WITH_KNOTS('',3,(#112650,#112651,#112652,#112653),
 .UNSPECIFIED.,.F.,.F.,(4,4),(-1.2,-2.77555756156289E-17),.UNSPECIFIED.);
#6543=B_SPLINE_CURVE_WITH_KNOTS('',3,(#113477,#113478,#113479,#113480,#113481,
#113482,#113483),.UNSPECIFIED.,.F.,.F.,(4,3,4),(0.,0.0330660780458673,0.0578656365802679),
 .UNSPECIFIED.);
#6544=B_SPLINE_CURVE_WITH_KNOTS('',3,(#113485,#113486,#113487,#113488),
 .UNSPECIFIED.,.F.,.F.,(4,4),(0.,1.2),.UNSPECIFIED.);
#6545=B_SPLINE_CURVE_WITH_KNOTS('',3,(#113490,#113491,#113492,#113493,#113494,
#113495,#113496),.UNSPECIFIED.,.F.,.F.,(4,3,4),(0.,0.0247995585344041,0.0578656365802761),
 .UNSPECIFIED.);
#6546=B_SPLINE_CURVE_WITH_KNOTS('',3,(#113497,#113498,#113499,#113500),
 .UNSPECIFIED.,.F.,.F.,(4,4),(-1.2,0.),.UNSPECIFIED.);
#6547=B_SPLINE_CURVE_WITH_KNOTS('',3,(#113526,#113527,#113528,#113529,#113530,
#113531,#113532),.UNSPECIFIED.,.F.,.F.,(4,3,4),(0.,0.0330660780484096,0.0578656365847167),
 .UNSPECIFIED.);
#6548=B_SPLINE_CURVE_WITH_KNOTS('',3,(#113534,#113535,#113536,#113537),
 .UNSPECIFIED.,.F.,.F.,(4,4),(9.71445146547012E-17,1.2),.UNSPECIFIED.);
#6549=B_SPLINE_CURVE_WITH_KNOTS('',3,(#113539,#113540,#113541,#113542,#113543,
#113544,#113545),.UNSPECIFIED.,.F.,.F.,(4,3,4),(0.,0.0247995585363052,0.0578656365847121),
 .UNSPECIFIED.);
#6550=B_SPLINE_CURVE_WITH_KNOTS('',3,(#113546,#113547,#113548,#113549),
 .UNSPECIFIED.,.F.,.F.,(4,4),(-1.2,-9.71445146547012E-17),.UNSPECIFIED.);
#6551=B_SPLINE_CURVE_WITH_KNOTS('',3,(#114373,#114374,#114375,#114376,#114377,
#114378,#114379),.UNSPECIFIED.,.F.,.F.,(4,3,4),(0.,0.0330660780458525,0.0578656365802419),
 .UNSPECIFIED.);
#6552=B_SPLINE_CURVE_WITH_KNOTS('',3,(#114381,#114382,#114383,#114384),
 .UNSPECIFIED.,.F.,.F.,(4,4),(-6.03986977505924E-17,1.2),.UNSPECIFIED.);
#6553=B_SPLINE_CURVE_WITH_KNOTS('',3,(#114386,#114387,#114388,#114389,#114390,
#114391,#114392),.UNSPECIFIED.,.F.,.F.,(4,3,4),(0.,0.0247995585343901,0.0578656365802435),
 .UNSPECIFIED.);
#6554=B_SPLINE_CURVE_WITH_KNOTS('',3,(#114393,#114394,#114395,#114396),
 .UNSPECIFIED.,.F.,.F.,(4,4),(-1.2,6.03986977505924E-17),.UNSPECIFIED.);
#6555=B_SPLINE_CURVE_WITH_KNOTS('',3,(#114422,#114423,#114424,#114425,#114426,
#114427,#114428),.UNSPECIFIED.,.F.,.F.,(4,3,4),(0.,0.0330660780484176,0.0578656365847307),
 .UNSPECIFIED.);
#6556=B_SPLINE_CURVE_WITH_KNOTS('',3,(#114430,#114431,#114432,#114433),
 .UNSPECIFIED.,.F.,.F.,(4,4),(9.71445146547012E-17,1.2),.UNSPECIFIED.);
#6557=B_SPLINE_CURVE_WITH_KNOTS('',3,(#114435,#114436,#114437,#114438,#114439,
#114440,#114441),.UNSPECIFIED.,.F.,.F.,(4,3,4),(0.,0.0247995585363079,0.0578656365847185),
 .UNSPECIFIED.);
#6558=B_SPLINE_CURVE_WITH_KNOTS('',3,(#114442,#114443,#114444,#114445),
 .UNSPECIFIED.,.F.,.F.,(4,4),(-1.2,-9.71445146547012E-17),.UNSPECIFIED.);
#6559=B_SPLINE_CURVE_WITH_KNOTS('',3,(#115269,#115270,#115271,#115272,#115273,
#115274,#115275),.UNSPECIFIED.,.F.,.F.,(4,3,4),(0.,0.0330660780458678,0.0578656365802686),
 .UNSPECIFIED.);
#6560=B_SPLINE_CURVE_WITH_KNOTS('',3,(#115277,#115278,#115279,#115280),
 .UNSPECIFIED.,.F.,.F.,(4,4),(2.77555756156289E-17,1.2),.UNSPECIFIED.);
#6561=B_SPLINE_CURVE_WITH_KNOTS('',3,(#115282,#115283,#115284,#115285,#115286,
#115287,#115288),.UNSPECIFIED.,.F.,.F.,(4,3,4),(0.,0.0247995585344011,0.0578656365802693),
 .UNSPECIFIED.);
#6562=B_SPLINE_CURVE_WITH_KNOTS('',3,(#115289,#115290,#115291,#115292),
 .UNSPECIFIED.,.F.,.F.,(4,4),(-1.2,-2.77555756156289E-17),.UNSPECIFIED.);
#6563=B_SPLINE_CURVE_WITH_KNOTS('',3,(#115318,#115319,#115320,#115321,#115322,
#115323,#115324),.UNSPECIFIED.,.F.,.F.,(4,3,4),(0.,0.033066078048387,0.0578656365846772),
 .UNSPECIFIED.);
#6564=B_SPLINE_CURVE_WITH_KNOTS('',3,(#115326,#115327,#115328,#115329),
 .UNSPECIFIED.,.F.,.F.,(4,4),(0.,1.2),.UNSPECIFIED.);
#6565=B_SPLINE_CURVE_WITH_KNOTS('',3,(#115331,#115332,#115333,#115334,#115335,
#115336,#115337),.UNSPECIFIED.,.F.,.F.,(4,3,4),(0.,0.024799558536296,0.0578656365846907),
 .UNSPECIFIED.);
#6566=B_SPLINE_CURVE_WITH_KNOTS('',3,(#115338,#115339,#115340,#115341),
 .UNSPECIFIED.,.F.,.F.,(4,4),(-1.2,0.),.UNSPECIFIED.);
#6567=B_SPLINE_CURVE_WITH_KNOTS('',3,(#116165,#116166,#116167,#116168,#116169,
#116170,#116171),.UNSPECIFIED.,.F.,.F.,(4,3,4),(0.,0.0330660780458588,0.0578656365802528),
 .UNSPECIFIED.);
#6568=B_SPLINE_CURVE_WITH_KNOTS('',3,(#116173,#116174,#116175,#116176),
 .UNSPECIFIED.,.F.,.F.,(4,4),(-5.55111512312578E-17,1.2),.UNSPECIFIED.);
#6569=B_SPLINE_CURVE_WITH_KNOTS('',3,(#116178,#116179,#116180,#116181,#116182,
#116183,#116184),.UNSPECIFIED.,.F.,.F.,(4,3,4),(0.,0.0247995585343981,0.0578656365802622),
 .UNSPECIFIED.);
#6570=B_SPLINE_CURVE_WITH_KNOTS('',3,(#116185,#116186,#116187,#116188),
 .UNSPECIFIED.,.F.,.F.,(4,4),(-1.2,5.55111512312578E-17),.UNSPECIFIED.);
#6571=B_SPLINE_CURVE_WITH_KNOTS('',3,(#173304,#173305,#173306,#173307,#173308,
#173309,#173310),.UNSPECIFIED.,.F.,.F.,(4,3,4),(0.,0.0330660780484233,0.0578656365847407),
 .UNSPECIFIED.);
#6572=B_SPLINE_CURVE_WITH_KNOTS('',3,(#173312,#173313,#173314,#173315),
 .UNSPECIFIED.,.F.,.F.,(4,4),(2.13940539033965E-17,1.2),.UNSPECIFIED.);
#6573=B_SPLINE_CURVE_WITH_KNOTS('',3,(#173317,#173318,#173319,#173320,#173321,
#173322,#173323),.UNSPECIFIED.,.F.,.F.,(4,3,4),(0.,0.0247995585363121,0.0578656365847283),
 .UNSPECIFIED.);
#6574=B_SPLINE_CURVE_WITH_KNOTS('',3,(#173324,#173325,#173326,#173327),
 .UNSPECIFIED.,.F.,.F.,(4,4),(-1.2,-2.13940539033965E-17),.UNSPECIFIED.);
#6575=B_SPLINE_CURVE_WITH_KNOTS('',3,(#174148,#174149,#174150,#174151,#174152,
#174153,#174154),.UNSPECIFIED.,.F.,.F.,(4,3,4),(0.,0.0330660780458505,0.0578656365802384),
 .UNSPECIFIED.);
#6576=B_SPLINE_CURVE_WITH_KNOTS('',3,(#174156,#174157,#174158,#174159),
 .UNSPECIFIED.,.F.,.F.,(4,4),(0.,1.2),.UNSPECIFIED.);
#6577=B_SPLINE_CURVE_WITH_KNOTS('',3,(#174161,#174162,#174163,#174164,#174165,
#174166,#174167),.UNSPECIFIED.,.F.,.F.,(4,3,4),(0.,0.024799558534381,0.0578656365802222),
 .UNSPECIFIED.);
#6578=B_SPLINE_CURVE_WITH_KNOTS('',3,(#174168,#174169,#174170,#174171),
 .UNSPECIFIED.,.F.,.F.,(4,4),(-1.2,0.),.UNSPECIFIED.);
#6980=LINE('',#52418,#8165);
#6981=LINE('',#52481,#8166);
#6982=LINE('',#52517,#8167);
#6983=LINE('',#52563,#8168);
#6984=LINE('',#53228,#8169);
#6985=LINE('',#54124,#8170);
#6986=LINE('',#55020,#8171);
#6987=LINE('',#55916,#8172);
#6988=LINE('',#56812,#8173);
#6989=LINE('',#57708,#8174);
#6990=LINE('',#58604,#8175);
#6991=LINE('',#59500,#8176);
#6992=LINE('',#60396,#8177);
#6993=LINE('',#61292,#8178);
#6994=LINE('',#62188,#8179);
#6995=LINE('',#63084,#8180);
#6996=LINE('',#63980,#8181);
#6997=LINE('',#64876,#8182);
#6998=LINE('',#65772,#8183);
#6999=LINE('',#66668,#8184);
#7000=LINE('',#67564,#8185);
#7001=LINE('',#68460,#8186);
#7002=LINE('',#69356,#8187);
#7003=LINE('',#70252,#8188);
#7004=LINE('',#71148,#8189);
#7005=LINE('',#72044,#8190);
#7006=LINE('',#72940,#8191);
#7007=LINE('',#73836,#8192);
#7008=LINE('',#74732,#8193);
#7009=LINE('',#75628,#8194);
#7010=LINE('',#76524,#8195);
#7011=LINE('',#77420,#8196);
#7012=LINE('',#78316,#8197);
#7013=LINE('',#79212,#8198);
#7014=LINE('',#80108,#8199);
#7015=LINE('',#81004,#8200);
#7016=LINE('',#81900,#8201);
#7017=LINE('',#82796,#8202);
#7018=LINE('',#83692,#8203);
#7019=LINE('',#84588,#8204);
#7020=LINE('',#85484,#8205);
#7021=LINE('',#86380,#8206);
#7022=LINE('',#87276,#8207);
#7023=LINE('',#88172,#8208);
#7024=LINE('',#89068,#8209);
#7025=LINE('',#89964,#8210);
#7026=LINE('',#90860,#8211);
#7027=LINE('',#91756,#8212);
#7028=LINE('',#92652,#8213);
#7029=LINE('',#93548,#8214);
#7030=LINE('',#94444,#8215);
#7031=LINE('',#95340,#8216);
#7032=LINE('',#96236,#8217);
#7033=LINE('',#97132,#8218);
#7034=LINE('',#98028,#8219);
#7035=LINE('',#98924,#8220);
#7036=LINE('',#99820,#8221);
#7037=LINE('',#100716,#8222);
#7038=LINE('',#101612,#8223);
#7039=LINE('',#102508,#8224);
#7040=LINE('',#103404,#8225);
#7041=LINE('',#104300,#8226);
#7042=LINE('',#105196,#8227);
#7043=LINE('',#106092,#8228);
#7044=LINE('',#106988,#8229);
#7045=LINE('',#107884,#8230);
#7046=LINE('',#108780,#8231);
#7047=LINE('',#109676,#8232);
#7048=LINE('',#110572,#8233);
#7049=LINE('',#111468,#8234);
#7050=LINE('',#112364,#8235);
#7051=LINE('',#113260,#8236);
#7052=LINE('',#114156,#8237);
#7053=LINE('',#115052,#8238);
#7054=LINE('',#115948,#8239);
#7055=LINE('',#116798,#8240);
#7056=LINE('',#117599,#8241);
#7057=LINE('',#118400,#8242);
#7058=LINE('',#119201,#8243);
#7059=LINE('',#120002,#8244);
#7060=LINE('',#120803,#8245);
#7061=LINE('',#121604,#8246);
#7062=LINE('',#122405,#8247);
#7063=LINE('',#123206,#8248);
#7064=LINE('',#124007,#8249);
#7065=LINE('',#124808,#8250);
#7066=LINE('',#125609,#8251);
#7067=LINE('',#126410,#8252);
#7068=LINE('',#127211,#8253);
#7069=LINE('',#128012,#8254);
#7070=LINE('',#128813,#8255);
#7071=LINE('',#129614,#8256);
#7072=LINE('',#130415,#8257);
#7073=LINE('',#131216,#8258);
#7074=LINE('',#132017,#8259);
#7075=LINE('',#132818,#8260);
#7076=LINE('',#133619,#8261);
#7077=LINE('',#134420,#8262);
#7078=LINE('',#135221,#8263);
#7079=LINE('',#136022,#8264);
#7080=LINE('',#136823,#8265);
#7081=LINE('',#137624,#8266);
#7082=LINE('',#138425,#8267);
#7083=LINE('',#139226,#8268);
#7084=LINE('',#140027,#8269);
#7085=LINE('',#140828,#8270);
#7086=LINE('',#141629,#8271);
#7087=LINE('',#142430,#8272);
#7088=LINE('',#143231,#8273);
#7089=LINE('',#144032,#8274);
#7090=LINE('',#144833,#8275);
#7091=LINE('',#145634,#8276);
#7092=LINE('',#146435,#8277);
#7093=LINE('',#147236,#8278);
#7094=LINE('',#148037,#8279);
#7095=LINE('',#148838,#8280);
#7096=LINE('',#149639,#8281);
#7097=LINE('',#150440,#8282);
#7098=LINE('',#151241,#8283);
#7099=LINE('',#152042,#8284);
#7100=LINE('',#152843,#8285);
#7101=LINE('',#153644,#8286);
#7102=LINE('',#154445,#8287);
#7103=LINE('',#155246,#8288);
#7104=LINE('',#156047,#8289);
#7105=LINE('',#156848,#8290);
#7106=LINE('',#157649,#8291);
#7107=LINE('',#158450,#8292);
#7108=LINE('',#159251,#8293);
#7109=LINE('',#160052,#8294);
#7110=LINE('',#160853,#8295);
#7111=LINE('',#161654,#8296);
#7112=LINE('',#162455,#8297);
#7113=LINE('',#163256,#8298);
#7114=LINE('',#164057,#8299);
#7115=LINE('',#164858,#8300);
#7116=LINE('',#165659,#8301);
#7117=LINE('',#166460,#8302);
#7118=LINE('',#167261,#8303);
#7119=LINE('',#168062,#8304);
#7120=LINE('',#168863,#8305);
#7121=LINE('',#169664,#8306);
#7122=LINE('',#170465,#8307);
#7123=LINE('',#171266,#8308);
#7124=LINE('',#172067,#8309);
#7125=LINE('',#172868,#8310);
#7126=LINE('',#173067,#8311);
#7127=LINE('',#173280,#8312);
#7128=LINE('',#174980,#8313);
#7129=LINE('',#174982,#8314);
#8165=VECTOR('',#28597,2.);
#8166=VECTOR('',#28604,2.);
#8167=VECTOR('',#28611,2.);
#8168=VECTOR('',#28618,2.);
#8169=VECTOR('',#28623,10.);
#8170=VECTOR('',#28630,10.);
#8171=VECTOR('',#28637,10.);
#8172=VECTOR('',#28644,10.);
#8173=VECTOR('',#28651,10.);
#8174=VECTOR('',#28658,10.);
#8175=VECTOR('',#28665,10.);
#8176=VECTOR('',#28672,10.);
#8177=VECTOR('',#28679,10.);
#8178=VECTOR('',#28686,10.);
#8179=VECTOR('',#28693,10.);
#8180=VECTOR('',#28700,10.);
#8181=VECTOR('',#28707,10.);
#8182=VECTOR('',#28714,10.);
#8183=VECTOR('',#28721,10.);
#8184=VECTOR('',#28728,10.);
#8185=VECTOR('',#28735,10.);
#8186=VECTOR('',#28742,10.);
#8187=VECTOR('',#28749,10.);
#8188=VECTOR('',#28756,10.);
#8189=VECTOR('',#28763,10.);
#8190=VECTOR('',#28770,10.);
#8191=VECTOR('',#28777,10.);
#8192=VECTOR('',#28784,10.);
#8193=VECTOR('',#28791,10.);
#8194=VECTOR('',#28798,10.);
#8195=VECTOR('',#28805,10.);
#8196=VECTOR('',#28812,10.);
#8197=VECTOR('',#28819,10.);
#8198=VECTOR('',#28826,10.);
#8199=VECTOR('',#28833,10.);
#8200=VECTOR('',#28840,10.);
#8201=VECTOR('',#28847,10.);
#8202=VECTOR('',#28854,10.);
#8203=VECTOR('',#28861,10.);
#8204=VECTOR('',#28868,10.);
#8205=VECTOR('',#28875,10.);
#8206=VECTOR('',#28882,10.);
#8207=VECTOR('',#28889,10.);
#8208=VECTOR('',#28896,10.);
#8209=VECTOR('',#28903,10.);
#8210=VECTOR('',#28910,10.);
#8211=VECTOR('',#28917,10.);
#8212=VECTOR('',#28924,10.);
#8213=VECTOR('',#28931,10.);
#8214=VECTOR('',#28938,10.);
#8215=VECTOR('',#28945,10.);
#8216=VECTOR('',#28952,10.);
#8217=VECTOR('',#28959,10.);
#8218=VECTOR('',#28966,10.);
#8219=VECTOR('',#28973,10.);
#8220=VECTOR('',#28980,10.);
#8221=VECTOR('',#28987,10.);
#8222=VECTOR('',#28994,10.);
#8223=VECTOR('',#29001,10.);
#8224=VECTOR('',#29008,10.);
#8225=VECTOR('',#29015,10.);
#8226=VECTOR('',#29022,10.);
#8227=VECTOR('',#29029,10.);
#8228=VECTOR('',#29036,10.);
#8229=VECTOR('',#29043,10.);
#8230=VECTOR('',#29050,10.);
#8231=VECTOR('',#29057,10.);
#8232=VECTOR('',#29064,10.);
#8233=VECTOR('',#29071,10.);
#8234=VECTOR('',#29078,10.);
#8235=VECTOR('',#29085,10.);
#8236=VECTOR('',#29092,10.);
#8237=VECTOR('',#29099,10.);
#8238=VECTOR('',#29106,10.);
#8239=VECTOR('',#29113,10.);
#8240=VECTOR('',#29120,10.);
#8241=VECTOR('',#29121,10.);
#8242=VECTOR('',#29122,10.);
#8243=VECTOR('',#29123,10.);
#8244=VECTOR('',#29124,10.);
#8245=VECTOR('',#29125,10.);
#8246=VECTOR('',#29126,10.);
#8247=VECTOR('',#29127,10.);
#8248=VECTOR('',#29128,10.);
#8249=VECTOR('',#29129,10.);
#8250=VECTOR('',#29130,10.);
#8251=VECTOR('',#29131,10.);
#8252=VECTOR('',#29132,10.);
#8253=VECTOR('',#29133,10.);
#8254=VECTOR('',#29134,10.);
#8255=VECTOR('',#29135,10.);
#8256=VECTOR('',#29136,10.);
#8257=VECTOR('',#29137,10.);
#8258=VECTOR('',#29138,10.);
#8259=VECTOR('',#29139,10.);
#8260=VECTOR('',#29140,10.);
#8261=VECTOR('',#29141,10.);
#8262=VECTOR('',#29142,10.);
#8263=VECTOR('',#29143,10.);
#8264=VECTOR('',#29144,10.);
#8265=VECTOR('',#29145,10.);
#8266=VECTOR('',#29146,10.);
#8267=VECTOR('',#29147,10.);
#8268=VECTOR('',#29148,10.);
#8269=VECTOR('',#29149,10.);
#8270=VECTOR('',#29150,10.);
#8271=VECTOR('',#29151,10.);
#8272=VECTOR('',#29152,10.);
#8273=VECTOR('',#29153,10.);
#8274=VECTOR('',#29154,10.);
#8275=VECTOR('',#29155,10.);
#8276=VECTOR('',#29156,10.);
#8277=VECTOR('',#29157,10.);
#8278=VECTOR('',#29158,10.);
#8279=VECTOR('',#29159,10.);
#8280=VECTOR('',#29160,10.);
#8281=VECTOR('',#29161,10.);
#8282=VECTOR('',#29162,10.);
#8283=VECTOR('',#29163,10.);
#8284=VECTOR('',#29164,10.);
#8285=VECTOR('',#29165,10.);
#8286=VECTOR('',#29166,10.);
#8287=VECTOR('',#29167,10.);
#8288=VECTOR('',#29168,10.);
#8289=VECTOR('',#29169,10.);
#8290=VECTOR('',#29170,10.);
#8291=VECTOR('',#29171,10.);
#8292=VECTOR('',#29172,10.);
#8293=VECTOR('',#29173,10.);
#8294=VECTOR('',#29174,10.);
#8295=VECTOR('',#29175,10.);
#8296=VECTOR('',#29176,10.);
#8297=VECTOR('',#29177,10.);
#8298=VECTOR('',#29178,10.);
#8299=VECTOR('',#29179,10.);
#8300=VECTOR('',#29180,10.);
#8301=VECTOR('',#29181,10.);
#8302=VECTOR('',#29182,10.);
#8303=VECTOR('',#29183,10.);
#8304=VECTOR('',#29184,10.);
#8305=VECTOR('',#29185,10.);
#8306=VECTOR('',#29186,10.);
#8307=VECTOR('',#29187,10.);
#8308=VECTOR('',#29188,10.);
#8309=VECTOR('',#29189,10.);
#8310=VECTOR('',#29190,10.);
#8311=VECTOR('',#29195,10.);
#8312=VECTOR('',#29616,10.);
#8313=VECTOR('',#29637,90.);
#8314=VECTOR('',#29638,90.);
#9737=VERTEX_POINT('',#52397);
#9738=VERTEX_POINT('',#52398);
#9739=VERTEX_POINT('',#52417);
#9740=VERTEX_POINT('',#52441);
#9741=VERTEX_POINT('',#52442);
#9742=VERTEX_POINT('',#52480);
#9743=VERTEX_POINT('',#52485);
#9744=VERTEX_POINT('',#52486);
#9745=VERTEX_POINT('',#52505);
#9746=VERTEX_POINT('',#52516);
#9747=VERTEX_POINT('',#52531);
#9748=VERTEX_POINT('',#52532);
#9749=VERTEX_POINT('',#52551);
#9750=VERTEX_POINT('',#52562);
#9751=VERTEX_POINT('',#52596);
#9752=VERTEX_POINT('',#52597);
#9753=VERTEX_POINT('',#52605);
#9754=VERTEX_POINT('',#52610);
#9755=VERTEX_POINT('',#53032);
#9756=VERTEX_POINT('',#53227);
#9757=VERTEX_POINT('',#53443);
#9758=VERTEX_POINT('',#53444);
#9759=VERTEX_POINT('',#53452);
#9760=VERTEX_POINT('',#53457);
#9761=VERTEX_POINT('',#53492);
#9762=VERTEX_POINT('',#53493);
#9763=VERTEX_POINT('',#53501);
#9764=VERTEX_POINT('',#53506);
#9765=VERTEX_POINT('',#53928);
#9766=VERTEX_POINT('',#54123);
#9767=VERTEX_POINT('',#54339);
#9768=VERTEX_POINT('',#54340);
#9769=VERTEX_POINT('',#54348);
#9770=VERTEX_POINT('',#54353);
#9771=VERTEX_POINT('',#54388);
#9772=VERTEX_POINT('',#54389);
#9773=VERTEX_POINT('',#54397);
#9774=VERTEX_POINT('',#54402);
#9775=VERTEX_POINT('',#54824);
#9776=VERTEX_POINT('',#55019);
#9777=VERTEX_POINT('',#55235);
#9778=VERTEX_POINT('',#55236);
#9779=VERTEX_POINT('',#55244);
#9780=VERTEX_POINT('',#55249);
#9781=VERTEX_POINT('',#55284);
#9782=VERTEX_POINT('',#55285);
#9783=VERTEX_POINT('',#55293);
#9784=VERTEX_POINT('',#55298);
#9785=VERTEX_POINT('',#55720);
#9786=VERTEX_POINT('',#55915);
#9787=VERTEX_POINT('',#56131);
#9788=VERTEX_POINT('',#56132);
#9789=VERTEX_POINT('',#56140);
#9790=VERTEX_POINT('',#56145);
#9791=VERTEX_POINT('',#56180);
#9792=VERTEX_POINT('',#56181);
#9793=VERTEX_POINT('',#56189);
#9794=VERTEX_POINT('',#56194);
#9795=VERTEX_POINT('',#56616);
#9796=VERTEX_POINT('',#56811);
#9797=VERTEX_POINT('',#57027);
#9798=VERTEX_POINT('',#57028);
#9799=VERTEX_POINT('',#57036);
#9800=VERTEX_POINT('',#57041);
#9801=VERTEX_POINT('',#57076);
#9802=VERTEX_POINT('',#57077);
#9803=VERTEX_POINT('',#57085);
#9804=VERTEX_POINT('',#57090);
#9805=VERTEX_POINT('',#57512);
#9806=VERTEX_POINT('',#57707);
#9807=VERTEX_POINT('',#57923);
#9808=VERTEX_POINT('',#57924);
#9809=VERTEX_POINT('',#57932);
#9810=VERTEX_POINT('',#57937);
#9811=VERTEX_POINT('',#57972);
#9812=VERTEX_POINT('',#57973);
#9813=VERTEX_POINT('',#57981);
#9814=VERTEX_POINT('',#57986);
#9815=VERTEX_POINT('',#58408);
#9816=VERTEX_POINT('',#58603);
#9817=VERTEX_POINT('',#58819);
#9818=VERTEX_POINT('',#58820);
#9819=VERTEX_POINT('',#58828);
#9820=VERTEX_POINT('',#58833);
#9821=VERTEX_POINT('',#58868);
#9822=VERTEX_POINT('',#58869);
#9823=VERTEX_POINT('',#58877);
#9824=VERTEX_POINT('',#58882);
#9825=VERTEX_POINT('',#59304);
#9826=VERTEX_POINT('',#59499);
#9827=VERTEX_POINT('',#59715);
#9828=VERTEX_POINT('',#59716);
#9829=VERTEX_POINT('',#59724);
#9830=VERTEX_POINT('',#59729);
#9831=VERTEX_POINT('',#59764);
#9832=VERTEX_POINT('',#59765);
#9833=VERTEX_POINT('',#59773);
#9834=VERTEX_POINT('',#59778);
#9835=VERTEX_POINT('',#60200);
#9836=VERTEX_POINT('',#60395);
#9837=VERTEX_POINT('',#60611);
#9838=VERTEX_POINT('',#60612);
#9839=VERTEX_POINT('',#60620);
#9840=VERTEX_POINT('',#60625);
#9841=VERTEX_POINT('',#60660);
#9842=VERTEX_POINT('',#60661);
#9843=VERTEX_POINT('',#60669);
#9844=VERTEX_POINT('',#60674);
#9845=VERTEX_POINT('',#61096);
#9846=VERTEX_POINT('',#61291);
#9847=VERTEX_POINT('',#61507);
#9848=VERTEX_POINT('',#61508);
#9849=VERTEX_POINT('',#61516);
#9850=VERTEX_POINT('',#61521);
#9851=VERTEX_POINT('',#61556);
#9852=VERTEX_POINT('',#61557);
#9853=VERTEX_POINT('',#61565);
#9854=VERTEX_POINT('',#61570);
#9855=VERTEX_POINT('',#61992);
#9856=VERTEX_POINT('',#62187);
#9857=VERTEX_POINT('',#62403);
#9858=VERTEX_POINT('',#62404);
#9859=VERTEX_POINT('',#62412);
#9860=VERTEX_POINT('',#62417);
#9861=VERTEX_POINT('',#62452);
#9862=VERTEX_POINT('',#62453);
#9863=VERTEX_POINT('',#62461);
#9864=VERTEX_POINT('',#62466);
#9865=VERTEX_POINT('',#62888);
#9866=VERTEX_POINT('',#63083);
#9867=VERTEX_POINT('',#63299);
#9868=VERTEX_POINT('',#63300);
#9869=VERTEX_POINT('',#63308);
#9870=VERTEX_POINT('',#63313);
#9871=VERTEX_POINT('',#63348);
#9872=VERTEX_POINT('',#63349);
#9873=VERTEX_POINT('',#63357);
#9874=VERTEX_POINT('',#63362);
#9875=VERTEX_POINT('',#63784);
#9876=VERTEX_POINT('',#63979);
#9877=VERTEX_POINT('',#64195);
#9878=VERTEX_POINT('',#64196);
#9879=VERTEX_POINT('',#64204);
#9880=VERTEX_POINT('',#64209);
#9881=VERTEX_POINT('',#64244);
#9882=VERTEX_POINT('',#64245);
#9883=VERTEX_POINT('',#64253);
#9884=VERTEX_POINT('',#64258);
#9885=VERTEX_POINT('',#64680);
#9886=VERTEX_POINT('',#64875);
#9887=VERTEX_POINT('',#65091);
#9888=VERTEX_POINT('',#65092);
#9889=VERTEX_POINT('',#65100);
#9890=VERTEX_POINT('',#65105);
#9891=VERTEX_POINT('',#65140);
#9892=VERTEX_POINT('',#65141);
#9893=VERTEX_POINT('',#65149);
#9894=VERTEX_POINT('',#65154);
#9895=VERTEX_POINT('',#65576);
#9896=VERTEX_POINT('',#65771);
#9897=VERTEX_POINT('',#65987);
#9898=VERTEX_POINT('',#65988);
#9899=VERTEX_POINT('',#65996);
#9900=VERTEX_POINT('',#66001);
#9901=VERTEX_POINT('',#66036);
#9902=VERTEX_POINT('',#66037);
#9903=VERTEX_POINT('',#66045);
#9904=VERTEX_POINT('',#66050);
#9905=VERTEX_POINT('',#66472);
#9906=VERTEX_POINT('',#66667);
#9907=VERTEX_POINT('',#66883);
#9908=VERTEX_POINT('',#66884);
#9909=VERTEX_POINT('',#66892);
#9910=VERTEX_POINT('',#66897);
#9911=VERTEX_POINT('',#66932);
#9912=VERTEX_POINT('',#66933);
#9913=VERTEX_POINT('',#66941);
#9914=VERTEX_POINT('',#66946);
#9915=VERTEX_POINT('',#67368);
#9916=VERTEX_POINT('',#67563);
#9917=VERTEX_POINT('',#67779);
#9918=VERTEX_POINT('',#67780);
#9919=VERTEX_POINT('',#67788);
#9920=VERTEX_POINT('',#67793);
#9921=VERTEX_POINT('',#67828);
#9922=VERTEX_POINT('',#67829);
#9923=VERTEX_POINT('',#67837);
#9924=VERTEX_POINT('',#67842);
#9925=VERTEX_POINT('',#68264);
#9926=VERTEX_POINT('',#68459);
#9927=VERTEX_POINT('',#68675);
#9928=VERTEX_POINT('',#68676);
#9929=VERTEX_POINT('',#68684);
#9930=VERTEX_POINT('',#68689);
#9931=VERTEX_POINT('',#68724);
#9932=VERTEX_POINT('',#68725);
#9933=VERTEX_POINT('',#68733);
#9934=VERTEX_POINT('',#68738);
#9935=VERTEX_POINT('',#69160);
#9936=VERTEX_POINT('',#69355);
#9937=VERTEX_POINT('',#69571);
#9938=VERTEX_POINT('',#69572);
#9939=VERTEX_POINT('',#69580);
#9940=VERTEX_POINT('',#69585);
#9941=VERTEX_POINT('',#69620);
#9942=VERTEX_POINT('',#69621);
#9943=VERTEX_POINT('',#69629);
#9944=VERTEX_POINT('',#69634);
#9945=VERTEX_POINT('',#70056);
#9946=VERTEX_POINT('',#70251);
#9947=VERTEX_POINT('',#70467);
#9948=VERTEX_POINT('',#70468);
#9949=VERTEX_POINT('',#70476);
#9950=VERTEX_POINT('',#70481);
#9951=VERTEX_POINT('',#70516);
#9952=VERTEX_POINT('',#70517);
#9953=VERTEX_POINT('',#70525);
#9954=VERTEX_POINT('',#70530);
#9955=VERTEX_POINT('',#70952);
#9956=VERTEX_POINT('',#71147);
#9957=VERTEX_POINT('',#71363);
#9958=VERTEX_POINT('',#71364);
#9959=VERTEX_POINT('',#71372);
#9960=VERTEX_POINT('',#71377);
#9961=VERTEX_POINT('',#71412);
#9962=VERTEX_POINT('',#71413);
#9963=VERTEX_POINT('',#71421);
#9964=VERTEX_POINT('',#71426);
#9965=VERTEX_POINT('',#71848);
#9966=VERTEX_POINT('',#72043);
#9967=VERTEX_POINT('',#72259);
#9968=VERTEX_POINT('',#72260);
#9969=VERTEX_POINT('',#72268);
#9970=VERTEX_POINT('',#72273);
#9971=VERTEX_POINT('',#72308);
#9972=VERTEX_POINT('',#72309);
#9973=VERTEX_POINT('',#72317);
#9974=VERTEX_POINT('',#72322);
#9975=VERTEX_POINT('',#72744);
#9976=VERTEX_POINT('',#72939);
#9977=VERTEX_POINT('',#73155);
#9978=VERTEX_POINT('',#73156);
#9979=VERTEX_POINT('',#73164);
#9980=VERTEX_POINT('',#73169);
#9981=VERTEX_POINT('',#73204);
#9982=VERTEX_POINT('',#73205);
#9983=VERTEX_POINT('',#73213);
#9984=VERTEX_POINT('',#73218);
#9985=VERTEX_POINT('',#73640);
#9986=VERTEX_POINT('',#73835);
#9987=VERTEX_POINT('',#74051);
#9988=VERTEX_POINT('',#74052);
#9989=VERTEX_POINT('',#74060);
#9990=VERTEX_POINT('',#74065);
#9991=VERTEX_POINT('',#74100);
#9992=VERTEX_POINT('',#74101);
#9993=VERTEX_POINT('',#74109);
#9994=VERTEX_POINT('',#74114);
#9995=VERTEX_POINT('',#74536);
#9996=VERTEX_POINT('',#74731);
#9997=VERTEX_POINT('',#74947);
#9998=VERTEX_POINT('',#74948);
#9999=VERTEX_POINT('',#74956);
#10000=VERTEX_POINT('',#74961);
#10001=VERTEX_POINT('',#74996);
#10002=VERTEX_POINT('',#74997);
#10003=VERTEX_POINT('',#75005);
#10004=VERTEX_POINT('',#75010);
#10005=VERTEX_POINT('',#75432);
#10006=VERTEX_POINT('',#75627);
#10007=VERTEX_POINT('',#75843);
#10008=VERTEX_POINT('',#75844);
#10009=VERTEX_POINT('',#75852);
#10010=VERTEX_POINT('',#75857);
#10011=VERTEX_POINT('',#75892);
#10012=VERTEX_POINT('',#75893);
#10013=VERTEX_POINT('',#75901);
#10014=VERTEX_POINT('',#75906);
#10015=VERTEX_POINT('',#76328);
#10016=VERTEX_POINT('',#76523);
#10017=VERTEX_POINT('',#76739);
#10018=VERTEX_POINT('',#76740);
#10019=VERTEX_POINT('',#76748);
#10020=VERTEX_POINT('',#76753);
#10021=VERTEX_POINT('',#76788);
#10022=VERTEX_POINT('',#76789);
#10023=VERTEX_POINT('',#76797);
#10024=VERTEX_POINT('',#76802);
#10025=VERTEX_POINT('',#77224);
#10026=VERTEX_POINT('',#77419);
#10027=VERTEX_POINT('',#77635);
#10028=VERTEX_POINT('',#77636);
#10029=VERTEX_POINT('',#77644);
#10030=VERTEX_POINT('',#77649);
#10031=VERTEX_POINT('',#77684);
#10032=VERTEX_POINT('',#77685);
#10033=VERTEX_POINT('',#77693);
#10034=VERTEX_POINT('',#77698);
#10035=VERTEX_POINT('',#78120);
#10036=VERTEX_POINT('',#78315);
#10037=VERTEX_POINT('',#78531);
#10038=VERTEX_POINT('',#78532);
#10039=VERTEX_POINT('',#78540);
#10040=VERTEX_POINT('',#78545);
#10041=VERTEX_POINT('',#78580);
#10042=VERTEX_POINT('',#78581);
#10043=VERTEX_POINT('',#78589);
#10044=VERTEX_POINT('',#78594);
#10045=VERTEX_POINT('',#79016);
#10046=VERTEX_POINT('',#79211);
#10047=VERTEX_POINT('',#79427);
#10048=VERTEX_POINT('',#79428);
#10049=VERTEX_POINT('',#79436);
#10050=VERTEX_POINT('',#79441);
#10051=VERTEX_POINT('',#79476);
#10052=VERTEX_POINT('',#79477);
#10053=VERTEX_POINT('',#79485);
#10054=VERTEX_POINT('',#79490);
#10055=VERTEX_POINT('',#79912);
#10056=VERTEX_POINT('',#80107);
#10057=VERTEX_POINT('',#80323);
#10058=VERTEX_POINT('',#80324);
#10059=VERTEX_POINT('',#80332);
#10060=VERTEX_POINT('',#80337);
#10061=VERTEX_POINT('',#80372);
#10062=VERTEX_POINT('',#80373);
#10063=VERTEX_POINT('',#80381);
#10064=VERTEX_POINT('',#80386);
#10065=VERTEX_POINT('',#80808);
#10066=VERTEX_POINT('',#81003);
#10067=VERTEX_POINT('',#81219);
#10068=VERTEX_POINT('',#81220);
#10069=VERTEX_POINT('',#81228);
#10070=VERTEX_POINT('',#81233);
#10071=VERTEX_POINT('',#81268);
#10072=VERTEX_POINT('',#81269);
#10073=VERTEX_POINT('',#81277);
#10074=VERTEX_POINT('',#81282);
#10075=VERTEX_POINT('',#81704);
#10076=VERTEX_POINT('',#81899);
#10077=VERTEX_POINT('',#82115);
#10078=VERTEX_POINT('',#82116);
#10079=VERTEX_POINT('',#82124);
#10080=VERTEX_POINT('',#82129);
#10081=VERTEX_POINT('',#82164);
#10082=VERTEX_POINT('',#82165);
#10083=VERTEX_POINT('',#82173);
#10084=VERTEX_POINT('',#82178);
#10085=VERTEX_POINT('',#82600);
#10086=VERTEX_POINT('',#82795);
#10087=VERTEX_POINT('',#83011);
#10088=VERTEX_POINT('',#83012);
#10089=VERTEX_POINT('',#83020);
#10090=VERTEX_POINT('',#83025);
#10091=VERTEX_POINT('',#83060);
#10092=VERTEX_POINT('',#83061);
#10093=VERTEX_POINT('',#83069);
#10094=VERTEX_POINT('',#83074);
#10095=VERTEX_POINT('',#83496);
#10096=VERTEX_POINT('',#83691);
#10097=VERTEX_POINT('',#83907);
#10098=VERTEX_POINT('',#83908);
#10099=VERTEX_POINT('',#83916);
#10100=VERTEX_POINT('',#83921);
#10101=VERTEX_POINT('',#83956);
#10102=VERTEX_POINT('',#83957);
#10103=VERTEX_POINT('',#83965);
#10104=VERTEX_POINT('',#83970);
#10105=VERTEX_POINT('',#84392);
#10106=VERTEX_POINT('',#84587);
#10107=VERTEX_POINT('',#84803);
#10108=VERTEX_POINT('',#84804);
#10109=VERTEX_POINT('',#84812);
#10110=VERTEX_POINT('',#84817);
#10111=VERTEX_POINT('',#84852);
#10112=VERTEX_POINT('',#84853);
#10113=VERTEX_POINT('',#84861);
#10114=VERTEX_POINT('',#84866);
#10115=VERTEX_POINT('',#85288);
#10116=VERTEX_POINT('',#85483);
#10117=VERTEX_POINT('',#85699);
#10118=VERTEX_POINT('',#85700);
#10119=VERTEX_POINT('',#85708);
#10120=VERTEX_POINT('',#85713);
#10121=VERTEX_POINT('',#85748);
#10122=VERTEX_POINT('',#85749);
#10123=VERTEX_POINT('',#85757);
#10124=VERTEX_POINT('',#85762);
#10125=VERTEX_POINT('',#86184);
#10126=VERTEX_POINT('',#86379);
#10127=VERTEX_POINT('',#86595);
#10128=VERTEX_POINT('',#86596);
#10129=VERTEX_POINT('',#86604);
#10130=VERTEX_POINT('',#86609);
#10131=VERTEX_POINT('',#86644);
#10132=VERTEX_POINT('',#86645);
#10133=VERTEX_POINT('',#86653);
#10134=VERTEX_POINT('',#86658);
#10135=VERTEX_POINT('',#87080);
#10136=VERTEX_POINT('',#87275);
#10137=VERTEX_POINT('',#87491);
#10138=VERTEX_POINT('',#87492);
#10139=VERTEX_POINT('',#87500);
#10140=VERTEX_POINT('',#87505);
#10141=VERTEX_POINT('',#87540);
#10142=VERTEX_POINT('',#87541);
#10143=VERTEX_POINT('',#87549);
#10144=VERTEX_POINT('',#87554);
#10145=VERTEX_POINT('',#87976);
#10146=VERTEX_POINT('',#88171);
#10147=VERTEX_POINT('',#88387);
#10148=VERTEX_POINT('',#88388);
#10149=VERTEX_POINT('',#88396);
#10150=VERTEX_POINT('',#88401);
#10151=VERTEX_POINT('',#88436);
#10152=VERTEX_POINT('',#88437);
#10153=VERTEX_POINT('',#88445);
#10154=VERTEX_POINT('',#88450);
#10155=VERTEX_POINT('',#88872);
#10156=VERTEX_POINT('',#89067);
#10157=VERTEX_POINT('',#89283);
#10158=VERTEX_POINT('',#89284);
#10159=VERTEX_POINT('',#89292);
#10160=VERTEX_POINT('',#89297);
#10161=VERTEX_POINT('',#89332);
#10162=VERTEX_POINT('',#89333);
#10163=VERTEX_POINT('',#89341);
#10164=VERTEX_POINT('',#89346);
#10165=VERTEX_POINT('',#89768);
#10166=VERTEX_POINT('',#89963);
#10167=VERTEX_POINT('',#90179);
#10168=VERTEX_POINT('',#90180);
#10169=VERTEX_POINT('',#90188);
#10170=VERTEX_POINT('',#90193);
#10171=VERTEX_POINT('',#90228);
#10172=VERTEX_POINT('',#90229);
#10173=VERTEX_POINT('',#90237);
#10174=VERTEX_POINT('',#90242);
#10175=VERTEX_POINT('',#90664);
#10176=VERTEX_POINT('',#90859);
#10177=VERTEX_POINT('',#91075);
#10178=VERTEX_POINT('',#91076);
#10179=VERTEX_POINT('',#91084);
#10180=VERTEX_POINT('',#91089);
#10181=VERTEX_POINT('',#91124);
#10182=VERTEX_POINT('',#91125);
#10183=VERTEX_POINT('',#91133);
#10184=VERTEX_POINT('',#91138);
#10185=VERTEX_POINT('',#91560);
#10186=VERTEX_POINT('',#91755);
#10187=VERTEX_POINT('',#91971);
#10188=VERTEX_POINT('',#91972);
#10189=VERTEX_POINT('',#91980);
#10190=VERTEX_POINT('',#91985);
#10191=VERTEX_POINT('',#92020);
#10192=VERTEX_POINT('',#92021);
#10193=VERTEX_POINT('',#92029);
#10194=VERTEX_POINT('',#92034);
#10195=VERTEX_POINT('',#92456);
#10196=VERTEX_POINT('',#92651);
#10197=VERTEX_POINT('',#92867);
#10198=VERTEX_POINT('',#92868);
#10199=VERTEX_POINT('',#92876);
#10200=VERTEX_POINT('',#92881);
#10201=VERTEX_POINT('',#92916);
#10202=VERTEX_POINT('',#92917);
#10203=VERTEX_POINT('',#92925);
#10204=VERTEX_POINT('',#92930);
#10205=VERTEX_POINT('',#93352);
#10206=VERTEX_POINT('',#93547);
#10207=VERTEX_POINT('',#93763);
#10208=VERTEX_POINT('',#93764);
#10209=VERTEX_POINT('',#93772);
#10210=VERTEX_POINT('',#93777);
#10211=VERTEX_POINT('',#93812);
#10212=VERTEX_POINT('',#93813);
#10213=VERTEX_POINT('',#93821);
#10214=VERTEX_POINT('',#93826);
#10215=VERTEX_POINT('',#94248);
#10216=VERTEX_POINT('',#94443);
#10217=VERTEX_POINT('',#94659);
#10218=VERTEX_POINT('',#94660);
#10219=VERTEX_POINT('',#94668);
#10220=VERTEX_POINT('',#94673);
#10221=VERTEX_POINT('',#94708);
#10222=VERTEX_POINT('',#94709);
#10223=VERTEX_POINT('',#94717);
#10224=VERTEX_POINT('',#94722);
#10225=VERTEX_POINT('',#95144);
#10226=VERTEX_POINT('',#95339);
#10227=VERTEX_POINT('',#95555);
#10228=VERTEX_POINT('',#95556);
#10229=VERTEX_POINT('',#95564);
#10230=VERTEX_POINT('',#95569);
#10231=VERTEX_POINT('',#95604);
#10232=VERTEX_POINT('',#95605);
#10233=VERTEX_POINT('',#95613);
#10234=VERTEX_POINT('',#95618);
#10235=VERTEX_POINT('',#96040);
#10236=VERTEX_POINT('',#96235);
#10237=VERTEX_POINT('',#96451);
#10238=VERTEX_POINT('',#96452);
#10239=VERTEX_POINT('',#96460);
#10240=VERTEX_POINT('',#96465);
#10241=VERTEX_POINT('',#96500);
#10242=VERTEX_POINT('',#96501);
#10243=VERTEX_POINT('',#96509);
#10244=VERTEX_POINT('',#96514);
#10245=VERTEX_POINT('',#96936);
#10246=VERTEX_POINT('',#97131);
#10247=VERTEX_POINT('',#97347);
#10248=VERTEX_POINT('',#97348);
#10249=VERTEX_POINT('',#97356);
#10250=VERTEX_POINT('',#97361);
#10251=VERTEX_POINT('',#97396);
#10252=VERTEX_POINT('',#97397);
#10253=VERTEX_POINT('',#97405);
#10254=VERTEX_POINT('',#97410);
#10255=VERTEX_POINT('',#97832);
#10256=VERTEX_POINT('',#98027);
#10257=VERTEX_POINT('',#98243);
#10258=VERTEX_POINT('',#98244);
#10259=VERTEX_POINT('',#98252);
#10260=VERTEX_POINT('',#98257);
#10261=VERTEX_POINT('',#98292);
#10262=VERTEX_POINT('',#98293);
#10263=VERTEX_POINT('',#98301);
#10264=VERTEX_POINT('',#98306);
#10265=VERTEX_POINT('',#98728);
#10266=VERTEX_POINT('',#98923);
#10267=VERTEX_POINT('',#99139);
#10268=VERTEX_POINT('',#99140);
#10269=VERTEX_POINT('',#99148);
#10270=VERTEX_POINT('',#99153);
#10271=VERTEX_POINT('',#99188);
#10272=VERTEX_POINT('',#99189);
#10273=VERTEX_POINT('',#99197);
#10274=VERTEX_POINT('',#99202);
#10275=VERTEX_POINT('',#99624);
#10276=VERTEX_POINT('',#99819);
#10277=VERTEX_POINT('',#100035);
#10278=VERTEX_POINT('',#100036);
#10279=VERTEX_POINT('',#100044);
#10280=VERTEX_POINT('',#100049);
#10281=VERTEX_POINT('',#100084);
#10282=VERTEX_POINT('',#100085);
#10283=VERTEX_POINT('',#100093);
#10284=VERTEX_POINT('',#100098);
#10285=VERTEX_POINT('',#100520);
#10286=VERTEX_POINT('',#100715);
#10287=VERTEX_POINT('',#100931);
#10288=VERTEX_POINT('',#100932);
#10289=VERTEX_POINT('',#100940);
#10290=VERTEX_POINT('',#100945);
#10291=VERTEX_POINT('',#100980);
#10292=VERTEX_POINT('',#100981);
#10293=VERTEX_POINT('',#100989);
#10294=VERTEX_POINT('',#100994);
#10295=VERTEX_POINT('',#101416);
#10296=VERTEX_POINT('',#101611);
#10297=VERTEX_POINT('',#101827);
#10298=VERTEX_POINT('',#101828);
#10299=VERTEX_POINT('',#101836);
#10300=VERTEX_POINT('',#101841);
#10301=VERTEX_POINT('',#101876);
#10302=VERTEX_POINT('',#101877);
#10303=VERTEX_POINT('',#101885);
#10304=VERTEX_POINT('',#101890);
#10305=VERTEX_POINT('',#102312);
#10306=VERTEX_POINT('',#102507);
#10307=VERTEX_POINT('',#102723);
#10308=VERTEX_POINT('',#102724);
#10309=VERTEX_POINT('',#102732);
#10310=VERTEX_POINT('',#102737);
#10311=VERTEX_POINT('',#102772);
#10312=VERTEX_POINT('',#102773);
#10313=VERTEX_POINT('',#102781);
#10314=VERTEX_POINT('',#102786);
#10315=VERTEX_POINT('',#103208);
#10316=VERTEX_POINT('',#103403);
#10317=VERTEX_POINT('',#103619);
#10318=VERTEX_POINT('',#103620);
#10319=VERTEX_POINT('',#103628);
#10320=VERTEX_POINT('',#103633);
#10321=VERTEX_POINT('',#103668);
#10322=VERTEX_POINT('',#103669);
#10323=VERTEX_POINT('',#103677);
#10324=VERTEX_POINT('',#103682);
#10325=VERTEX_POINT('',#104104);
#10326=VERTEX_POINT('',#104299);
#10327=VERTEX_POINT('',#104515);
#10328=VERTEX_POINT('',#104516);
#10329=VERTEX_POINT('',#104524);
#10330=VERTEX_POINT('',#104529);
#10331=VERTEX_POINT('',#104564);
#10332=VERTEX_POINT('',#104565);
#10333=VERTEX_POINT('',#104573);
#10334=VERTEX_POINT('',#104578);
#10335=VERTEX_POINT('',#105000);
#10336=VERTEX_POINT('',#105195);
#10337=VERTEX_POINT('',#105411);
#10338=VERTEX_POINT('',#105412);
#10339=VERTEX_POINT('',#105420);
#10340=VERTEX_POINT('',#105425);
#10341=VERTEX_POINT('',#105460);
#10342=VERTEX_POINT('',#105461);
#10343=VERTEX_POINT('',#105469);
#10344=VERTEX_POINT('',#105474);
#10345=VERTEX_POINT('',#105896);
#10346=VERTEX_POINT('',#106091);
#10347=VERTEX_POINT('',#106307);
#10348=VERTEX_POINT('',#106308);
#10349=VERTEX_POINT('',#106316);
#10350=VERTEX_POINT('',#106321);
#10351=VERTEX_POINT('',#106356);
#10352=VERTEX_POINT('',#106357);
#10353=VERTEX_POINT('',#106365);
#10354=VERTEX_POINT('',#106370);
#10355=VERTEX_POINT('',#106792);
#10356=VERTEX_POINT('',#106987);
#10357=VERTEX_POINT('',#107203);
#10358=VERTEX_POINT('',#107204);
#10359=VERTEX_POINT('',#107212);
#10360=VERTEX_POINT('',#107217);
#10361=VERTEX_POINT('',#107252);
#10362=VERTEX_POINT('',#107253);
#10363=VERTEX_POINT('',#107261);
#10364=VERTEX_POINT('',#107266);
#10365=VERTEX_POINT('',#107688);
#10366=VERTEX_POINT('',#107883);
#10367=VERTEX_POINT('',#108099);
#10368=VERTEX_POINT('',#108100);
#10369=VERTEX_POINT('',#108108);
#10370=VERTEX_POINT('',#108113);
#10371=VERTEX_POINT('',#108148);
#10372=VERTEX_POINT('',#108149);
#10373=VERTEX_POINT('',#108157);
#10374=VERTEX_POINT('',#108162);
#10375=VERTEX_POINT('',#108584);
#10376=VERTEX_POINT('',#108779);
#10377=VERTEX_POINT('',#108995);
#10378=VERTEX_POINT('',#108996);
#10379=VERTEX_POINT('',#109004);
#10380=VERTEX_POINT('',#109009);
#10381=VERTEX_POINT('',#109044);
#10382=VERTEX_POINT('',#109045);
#10383=VERTEX_POINT('',#109053);
#10384=VERTEX_POINT('',#109058);
#10385=VERTEX_POINT('',#109480);
#10386=VERTEX_POINT('',#109675);
#10387=VERTEX_POINT('',#109891);
#10388=VERTEX_POINT('',#109892);
#10389=VERTEX_POINT('',#109900);
#10390=VERTEX_POINT('',#109905);
#10391=VERTEX_POINT('',#109940);
#10392=VERTEX_POINT('',#109941);
#10393=VERTEX_POINT('',#109949);
#10394=VERTEX_POINT('',#109954);
#10395=VERTEX_POINT('',#110376);
#10396=VERTEX_POINT('',#110571);
#10397=VERTEX_POINT('',#110787);
#10398=VERTEX_POINT('',#110788);
#10399=VERTEX_POINT('',#110796);
#10400=VERTEX_POINT('',#110801);
#10401=VERTEX_POINT('',#110836);
#10402=VERTEX_POINT('',#110837);
#10403=VERTEX_POINT('',#110845);
#10404=VERTEX_POINT('',#110850);
#10405=VERTEX_POINT('',#111272);
#10406=VERTEX_POINT('',#111467);
#10407=VERTEX_POINT('',#111683);
#10408=VERTEX_POINT('',#111684);
#10409=VERTEX_POINT('',#111692);
#10410=VERTEX_POINT('',#111697);
#10411=VERTEX_POINT('',#111732);
#10412=VERTEX_POINT('',#111733);
#10413=VERTEX_POINT('',#111741);
#10414=VERTEX_POINT('',#111746);
#10415=VERTEX_POINT('',#112168);
#10416=VERTEX_POINT('',#112363);
#10417=VERTEX_POINT('',#112579);
#10418=VERTEX_POINT('',#112580);
#10419=VERTEX_POINT('',#112588);
#10420=VERTEX_POINT('',#112593);
#10421=VERTEX_POINT('',#112628);
#10422=VERTEX_POINT('',#112629);
#10423=VERTEX_POINT('',#112637);
#10424=VERTEX_POINT('',#112642);
#10425=VERTEX_POINT('',#113064);
#10426=VERTEX_POINT('',#113259);
#10427=VERTEX_POINT('',#113475);
#10428=VERTEX_POINT('',#113476);
#10429=VERTEX_POINT('',#113484);
#10430=VERTEX_POINT('',#113489);
#10431=VERTEX_POINT('',#113524);
#10432=VERTEX_POINT('',#113525);
#10433=VERTEX_POINT('',#113533);
#10434=VERTEX_POINT('',#113538);
#10435=VERTEX_POINT('',#113960);
#10436=VERTEX_POINT('',#114155);
#10437=VERTEX_POINT('',#114371);
#10438=VERTEX_POINT('',#114372);
#10439=VERTEX_POINT('',#114380);
#10440=VERTEX_POINT('',#114385);
#10441=VERTEX_POINT('',#114420);
#10442=VERTEX_POINT('',#114421);
#10443=VERTEX_POINT('',#114429);
#10444=VERTEX_POINT('',#114434);
#10445=VERTEX_POINT('',#114856);
#10446=VERTEX_POINT('',#115051);
#10447=VERTEX_POINT('',#115267);
#10448=VERTEX_POINT('',#115268);
#10449=VERTEX_POINT('',#115276);
#10450=VERTEX_POINT('',#115281);
#10451=VERTEX_POINT('',#115316);
#10452=VERTEX_POINT('',#115317);
#10453=VERTEX_POINT('',#115325);
#10454=VERTEX_POINT('',#115330);
#10455=VERTEX_POINT('',#115752);
#10456=VERTEX_POINT('',#115947);
#10457=VERTEX_POINT('',#116163);
#10458=VERTEX_POINT('',#116164);
#10459=VERTEX_POINT('',#116172);
#10460=VERTEX_POINT('',#116177);
#10461=VERTEX_POINT('',#116602);
#10462=VERTEX_POINT('',#116797);
#10463=VERTEX_POINT('',#117403);
#10464=VERTEX_POINT('',#117598);
#10465=VERTEX_POINT('',#118204);
#10466=VERTEX_POINT('',#118399);
#10467=VERTEX_POINT('',#119005);
#10468=VERTEX_POINT('',#119200);
#10469=VERTEX_POINT('',#119806);
#10470=VERTEX_POINT('',#120001);
#10471=VERTEX_POINT('',#120607);
#10472=VERTEX_POINT('',#120802);
#10473=VERTEX_POINT('',#121408);
#10474=VERTEX_POINT('',#121603);
#10475=VERTEX_POINT('',#122209);
#10476=VERTEX_POINT('',#122404);
#10477=VERTEX_POINT('',#123010);
#10478=VERTEX_POINT('',#123205);
#10479=VERTEX_POINT('',#123811);
#10480=VERTEX_POINT('',#124006);
#10481=VERTEX_POINT('',#124612);
#10482=VERTEX_POINT('',#124807);
#10483=VERTEX_POINT('',#125413);
#10484=VERTEX_POINT('',#125608);
#10485=VERTEX_POINT('',#126214);
#10486=VERTEX_POINT('',#126409);
#10487=VERTEX_POINT('',#127015);
#10488=VERTEX_POINT('',#127210);
#10489=VERTEX_POINT('',#127816);
#10490=VERTEX_POINT('',#128011);
#10491=VERTEX_POINT('',#128617);
#10492=VERTEX_POINT('',#128812);
#10493=VERTEX_POINT('',#129418);
#10494=VERTEX_POINT('',#129613);
#10495=VERTEX_POINT('',#130219);
#10496=VERTEX_POINT('',#130414);
#10497=VERTEX_POINT('',#131020);
#10498=VERTEX_POINT('',#131215);
#10499=VERTEX_POINT('',#131821);
#10500=VERTEX_POINT('',#132016);
#10501=VERTEX_POINT('',#132622);
#10502=VERTEX_POINT('',#132817);
#10503=VERTEX_POINT('',#133423);
#10504=VERTEX_POINT('',#133618);
#10505=VERTEX_POINT('',#134224);
#10506=VERTEX_POINT('',#134419);
#10507=VERTEX_POINT('',#135025);
#10508=VERTEX_POINT('',#135220);
#10509=VERTEX_POINT('',#135826);
#10510=VERTEX_POINT('',#136021);
#10511=VERTEX_POINT('',#136627);
#10512=VERTEX_POINT('',#136822);
#10513=VERTEX_POINT('',#137428);
#10514=VERTEX_POINT('',#137623);
#10515=VERTEX_POINT('',#138229);
#10516=VERTEX_POINT('',#138424);
#10517=VERTEX_POINT('',#139030);
#10518=VERTEX_POINT('',#139225);
#10519=VERTEX_POINT('',#139831);
#10520=VERTEX_POINT('',#140026);
#10521=VERTEX_POINT('',#140632);
#10522=VERTEX_POINT('',#140827);
#10523=VERTEX_POINT('',#141433);
#10524=VERTEX_POINT('',#141628);
#10525=VERTEX_POINT('',#142234);
#10526=VERTEX_POINT('',#142429);
#10527=VERTEX_POINT('',#143035);
#10528=VERTEX_POINT('',#143230);
#10529=VERTEX_POINT('',#143836);
#10530=VERTEX_POINT('',#144031);
#10531=VERTEX_POINT('',#144637);
#10532=VERTEX_POINT('',#144832);
#10533=VERTEX_POINT('',#145438);
#10534=VERTEX_POINT('',#145633);
#10535=VERTEX_POINT('',#146239);
#10536=VERTEX_POINT('',#146434);
#10537=VERTEX_POINT('',#147040);
#10538=VERTEX_POINT('',#147235);
#10539=VERTEX_POINT('',#147841);
#10540=VERTEX_POINT('',#148036);
#10541=VERTEX_POINT('',#148642);
#10542=VERTEX_POINT('',#148837);
#10543=VERTEX_POINT('',#149443);
#10544=VERTEX_POINT('',#149638);
#10545=VERTEX_POINT('',#150244);
#10546=VERTEX_POINT('',#150439);
#10547=VERTEX_POINT('',#151045);
#10548=VERTEX_POINT('',#151240);
#10549=VERTEX_POINT('',#151846);
#10550=VERTEX_POINT('',#152041);
#10551=VERTEX_POINT('',#152647);
#10552=VERTEX_POINT('',#152842);
#10553=VERTEX_POINT('',#153448);
#10554=VERTEX_POINT('',#153643);
#10555=VERTEX_POINT('',#154249);
#10556=VERTEX_POINT('',#154444);
#10557=VERTEX_POINT('',#155050);
#10558=VERTEX_POINT('',#155245);
#10559=VERTEX_POINT('',#155851);
#10560=VERTEX_POINT('',#156046);
#10561=VERTEX_POINT('',#156652);
#10562=VERTEX_POINT('',#156847);
#10563=VERTEX_POINT('',#157453);
#10564=VERTEX_POINT('',#157648);
#10565=VERTEX_POINT('',#158254);
#10566=VERTEX_POINT('',#158449);
#10567=VERTEX_POINT('',#159055);
#10568=VERTEX_POINT('',#159250);
#10569=VERTEX_POINT('',#159856);
#10570=VERTEX_POINT('',#160051);
#10571=VERTEX_POINT('',#160657);
#10572=VERTEX_POINT('',#160852);
#10573=VERTEX_POINT('',#161458);
#10574=VERTEX_POINT('',#161653);
#10575=VERTEX_POINT('',#162259);
#10576=VERTEX_POINT('',#162454);
#10577=VERTEX_POINT('',#163060);
#10578=VERTEX_POINT('',#163255);
#10579=VERTEX_POINT('',#163861);
#10580=VERTEX_POINT('',#164056);
#10581=VERTEX_POINT('',#164662);
#10582=VERTEX_POINT('',#164857);
#10583=VERTEX_POINT('',#165463);
#10584=VERTEX_POINT('',#165658);
#10585=VERTEX_POINT('',#166264);
#10586=VERTEX_POINT('',#166459);
#10587=VERTEX_POINT('',#167065);
#10588=VERTEX_POINT('',#167260);
#10589=VERTEX_POINT('',#167866);
#10590=VERTEX_POINT('',#168061);
#10591=VERTEX_POINT('',#168667);
#10592=VERTEX_POINT('',#168862);
#10593=VERTEX_POINT('',#169468);
#10594=VERTEX_POINT('',#169663);
#10595=VERTEX_POINT('',#170269);
#10596=VERTEX_POINT('',#170464);
#10597=VERTEX_POINT('',#171070);
#10598=VERTEX_POINT('',#171265);
#10599=VERTEX_POINT('',#171871);
#10600=VERTEX_POINT('',#172066);
#10601=VERTEX_POINT('',#172672);
#10602=VERTEX_POINT('',#172867);
#10603=VERTEX_POINT('',#173064);
#10604=VERTEX_POINT('',#173066);
#10605=VERTEX_POINT('',#173277);
#10606=VERTEX_POINT('',#173279);
#10607=VERTEX_POINT('',#173302);
#10608=VERTEX_POINT('',#173303);
#10609=VERTEX_POINT('',#173311);
#10610=VERTEX_POINT('',#173316);
#10611=VERTEX_POINT('',#174146);
#10612=VERTEX_POINT('',#174147);
#10613=VERTEX_POINT('',#174155);
#10614=VERTEX_POINT('',#174160);
#10615=VERTEX_POINT('',#174974);
#10616=VERTEX_POINT('',#174981);
#12636=EDGE_CURVE('',#9737,#9738,#5993,.T.);
#12637=EDGE_CURVE('',#9737,#9739,#6980,.T.);
#12638=EDGE_CURVE('',#9739,#9739,#4623,.T.);
#12639=EDGE_CURVE('',#9738,#9737,#5994,.T.);
#12640=EDGE_CURVE('',#9740,#9741,#5995,.T.);
#12641=EDGE_CURVE('',#9741,#9740,#5996,.T.);
#12642=EDGE_CURVE('',#9741,#9742,#6981,.T.);
#12643=EDGE_CURVE('',#9742,#9742,#4624,.T.);
#12644=EDGE_CURVE('',#9743,#9744,#5997,.T.);
#12645=EDGE_CURVE('',#9745,#9743,#5998,.T.);
#12646=EDGE_CURVE('',#9745,#9746,#6982,.T.);
#12647=EDGE_CURVE('',#9746,#9746,#4625,.T.);
#12648=EDGE_CURVE('',#9744,#9745,#5999,.T.);
#12649=EDGE_CURVE('',#9747,#9748,#6000,.T.);
#12650=EDGE_CURVE('',#9749,#9747,#6001,.T.);
#12651=EDGE_CURVE('',#9749,#9750,#6983,.T.);
#12652=EDGE_CURVE('',#9750,#9750,#4626,.T.);
#12653=EDGE_CURVE('',#9748,#9749,#6002,.T.);
#12654=EDGE_CURVE('',#9751,#9752,#6003,.T.);
#12655=EDGE_CURVE('',#9752,#9753,#6004,.T.);
#12656=EDGE_CURVE('',#9753,#9754,#6005,.T.);
#12657=EDGE_CURVE('',#9754,#9751,#6006,.T.);
#12658=EDGE_CURVE('',#9755,#9752,#403,.T.);
#12659=EDGE_CURVE('',#9756,#9755,#6984,.T.);
#12660=EDGE_CURVE('',#9753,#9756,#404,.T.);
#12661=EDGE_CURVE('',#9757,#9758,#6007,.T.);
#12662=EDGE_CURVE('',#9758,#9759,#6008,.T.);
#12663=EDGE_CURVE('',#9759,#9760,#6009,.T.);
#12664=EDGE_CURVE('',#9760,#9757,#6010,.T.);
#12665=EDGE_CURVE('',#9759,#9754,#4627,.T.);
#12666=EDGE_CURVE('',#9751,#9758,#4628,.T.);
#12667=EDGE_CURVE('',#9761,#9762,#6011,.T.);
#12668=EDGE_CURVE('',#9762,#9763,#6012,.T.);
#12669=EDGE_CURVE('',#9763,#9764,#6013,.T.);
#12670=EDGE_CURVE('',#9764,#9761,#6014,.T.);
#12671=EDGE_CURVE('',#9765,#9762,#405,.T.);
#12672=EDGE_CURVE('',#9766,#9765,#6985,.T.);
#12673=EDGE_CURVE('',#9763,#9766,#406,.T.);
#12674=EDGE_CURVE('',#9767,#9768,#6015,.T.);
#12675=EDGE_CURVE('',#9768,#9769,#6016,.T.);
#12676=EDGE_CURVE('',#9769,#9770,#6017,.T.);
#12677=EDGE_CURVE('',#9770,#9767,#6018,.T.);
#12678=EDGE_CURVE('',#9769,#9764,#4629,.T.);
#12679=EDGE_CURVE('',#9761,#9768,#4630,.T.);
#12680=EDGE_CURVE('',#9771,#9772,#6019,.T.);
#12681=EDGE_CURVE('',#9772,#9773,#6020,.T.);
#12682=EDGE_CURVE('',#9773,#9774,#6021,.T.);
#12683=EDGE_CURVE('',#9774,#9771,#6022,.T.);
#12684=EDGE_CURVE('',#9775,#9772,#407,.T.);
#12685=EDGE_CURVE('',#9776,#9775,#6986,.T.);
#12686=EDGE_CURVE('',#9773,#9776,#408,.T.);
#12687=EDGE_CURVE('',#9777,#9778,#6023,.T.);
#12688=EDGE_CURVE('',#9778,#9779,#6024,.T.);
#12689=EDGE_CURVE('',#9779,#9780,#6025,.T.);
#12690=EDGE_CURVE('',#9780,#9777,#6026,.T.);
#12691=EDGE_CURVE('',#9779,#9774,#4631,.T.);
#12692=EDGE_CURVE('',#9771,#9778,#4632,.T.);
#12693=EDGE_CURVE('',#9781,#9782,#6027,.T.);
#12694=EDGE_CURVE('',#9782,#9783,#6028,.T.);
#12695=EDGE_CURVE('',#9783,#9784,#6029,.T.);
#12696=EDGE_CURVE('',#9784,#9781,#6030,.T.);
#12697=EDGE_CURVE('',#9785,#9782,#409,.T.);
#12698=EDGE_CURVE('',#9786,#9785,#6987,.T.);
#12699=EDGE_CURVE('',#9783,#9786,#410,.T.);
#12700=EDGE_CURVE('',#9787,#9788,#6031,.T.);
#12701=EDGE_CURVE('',#9788,#9789,#6032,.T.);
#12702=EDGE_CURVE('',#9789,#9790,#6033,.T.);
#12703=EDGE_CURVE('',#9790,#9787,#6034,.T.);
#12704=EDGE_CURVE('',#9789,#9784,#4633,.T.);
#12705=EDGE_CURVE('',#9781,#9788,#4634,.T.);
#12706=EDGE_CURVE('',#9791,#9792,#6035,.T.);
#12707=EDGE_CURVE('',#9792,#9793,#6036,.T.);
#12708=EDGE_CURVE('',#9793,#9794,#6037,.T.);
#12709=EDGE_CURVE('',#9794,#9791,#6038,.T.);
#12710=EDGE_CURVE('',#9795,#9792,#411,.T.);
#12711=EDGE_CURVE('',#9796,#9795,#6988,.T.);
#12712=EDGE_CURVE('',#9793,#9796,#412,.T.);
#12713=EDGE_CURVE('',#9797,#9798,#6039,.T.);
#12714=EDGE_CURVE('',#9798,#9799,#6040,.T.);
#12715=EDGE_CURVE('',#9799,#9800,#6041,.T.);
#12716=EDGE_CURVE('',#9800,#9797,#6042,.T.);
#12717=EDGE_CURVE('',#9799,#9794,#4635,.T.);
#12718=EDGE_CURVE('',#9791,#9798,#4636,.T.);
#12719=EDGE_CURVE('',#9801,#9802,#6043,.T.);
#12720=EDGE_CURVE('',#9802,#9803,#6044,.T.);
#12721=EDGE_CURVE('',#9803,#9804,#6045,.T.);
#12722=EDGE_CURVE('',#9804,#9801,#6046,.T.);
#12723=EDGE_CURVE('',#9805,#9802,#413,.T.);
#12724=EDGE_CURVE('',#9806,#9805,#6989,.T.);
#12725=EDGE_CURVE('',#9803,#9806,#414,.T.);
#12726=EDGE_CURVE('',#9807,#9808,#6047,.T.);
#12727=EDGE_CURVE('',#9808,#9809,#6048,.T.);
#12728=EDGE_CURVE('',#9809,#9810,#6049,.T.);
#12729=EDGE_CURVE('',#9810,#9807,#6050,.T.);
#12730=EDGE_CURVE('',#9809,#9804,#4637,.T.);
#12731=EDGE_CURVE('',#9801,#9808,#4638,.T.);
#12732=EDGE_CURVE('',#9811,#9812,#6051,.T.);
#12733=EDGE_CURVE('',#9812,#9813,#6052,.T.);
#12734=EDGE_CURVE('',#9813,#9814,#6053,.T.);
#12735=EDGE_CURVE('',#9814,#9811,#6054,.T.);
#12736=EDGE_CURVE('',#9815,#9812,#415,.T.);
#12737=EDGE_CURVE('',#9816,#9815,#6990,.T.);
#12738=EDGE_CURVE('',#9813,#9816,#416,.T.);
#12739=EDGE_CURVE('',#9817,#9818,#6055,.T.);
#12740=EDGE_CURVE('',#9818,#9819,#6056,.T.);
#12741=EDGE_CURVE('',#9819,#9820,#6057,.T.);
#12742=EDGE_CURVE('',#9820,#9817,#6058,.T.);
#12743=EDGE_CURVE('',#9819,#9814,#4639,.T.);
#12744=EDGE_CURVE('',#9811,#9818,#4640,.T.);
#12745=EDGE_CURVE('',#9821,#9822,#6059,.T.);
#12746=EDGE_CURVE('',#9822,#9823,#6060,.T.);
#12747=EDGE_CURVE('',#9823,#9824,#6061,.T.);
#12748=EDGE_CURVE('',#9824,#9821,#6062,.T.);
#12749=EDGE_CURVE('',#9825,#9822,#417,.T.);
#12750=EDGE_CURVE('',#9826,#9825,#6991,.T.);
#12751=EDGE_CURVE('',#9823,#9826,#418,.T.);
#12752=EDGE_CURVE('',#9827,#9828,#6063,.T.);
#12753=EDGE_CURVE('',#9828,#9829,#6064,.T.);
#12754=EDGE_CURVE('',#9829,#9830,#6065,.T.);
#12755=EDGE_CURVE('',#9830,#9827,#6066,.T.);
#12756=EDGE_CURVE('',#9829,#9824,#4641,.T.);
#12757=EDGE_CURVE('',#9821,#9828,#4642,.T.);
#12758=EDGE_CURVE('',#9831,#9832,#6067,.T.);
#12759=EDGE_CURVE('',#9832,#9833,#6068,.T.);
#12760=EDGE_CURVE('',#9833,#9834,#6069,.T.);
#12761=EDGE_CURVE('',#9834,#9831,#6070,.T.);
#12762=EDGE_CURVE('',#9835,#9832,#419,.T.);
#12763=EDGE_CURVE('',#9836,#9835,#6992,.T.);
#12764=EDGE_CURVE('',#9833,#9836,#420,.T.);
#12765=EDGE_CURVE('',#9837,#9838,#6071,.T.);
#12766=EDGE_CURVE('',#9838,#9839,#6072,.T.);
#12767=EDGE_CURVE('',#9839,#9840,#6073,.T.);
#12768=EDGE_CURVE('',#9840,#9837,#6074,.T.);
#12769=EDGE_CURVE('',#9839,#9834,#4643,.T.);
#12770=EDGE_CURVE('',#9831,#9838,#4644,.T.);
#12771=EDGE_CURVE('',#9841,#9842,#6075,.T.);
#12772=EDGE_CURVE('',#9842,#9843,#6076,.T.);
#12773=EDGE_CURVE('',#9843,#9844,#6077,.T.);
#12774=EDGE_CURVE('',#9844,#9841,#6078,.T.);
#12775=EDGE_CURVE('',#9845,#9842,#421,.T.);
#12776=EDGE_CURVE('',#9846,#9845,#6993,.T.);
#12777=EDGE_CURVE('',#9843,#9846,#422,.T.);
#12778=EDGE_CURVE('',#9847,#9848,#6079,.T.);
#12779=EDGE_CURVE('',#9848,#9849,#6080,.T.);
#12780=EDGE_CURVE('',#9849,#9850,#6081,.T.);
#12781=EDGE_CURVE('',#9850,#9847,#6082,.T.);
#12782=EDGE_CURVE('',#9849,#9844,#4645,.T.);
#12783=EDGE_CURVE('',#9841,#9848,#4646,.T.);
#12784=EDGE_CURVE('',#9851,#9852,#6083,.T.);
#12785=EDGE_CURVE('',#9852,#9853,#6084,.T.);
#12786=EDGE_CURVE('',#9853,#9854,#6085,.T.);
#12787=EDGE_CURVE('',#9854,#9851,#6086,.T.);
#12788=EDGE_CURVE('',#9855,#9852,#423,.T.);
#12789=EDGE_CURVE('',#9856,#9855,#6994,.T.);
#12790=EDGE_CURVE('',#9853,#9856,#424,.T.);
#12791=EDGE_CURVE('',#9857,#9858,#6087,.T.);
#12792=EDGE_CURVE('',#9858,#9859,#6088,.T.);
#12793=EDGE_CURVE('',#9859,#9860,#6089,.T.);
#12794=EDGE_CURVE('',#9860,#9857,#6090,.T.);
#12795=EDGE_CURVE('',#9859,#9854,#4647,.T.);
#12796=EDGE_CURVE('',#9851,#9858,#4648,.T.);
#12797=EDGE_CURVE('',#9861,#9862,#6091,.T.);
#12798=EDGE_CURVE('',#9862,#9863,#6092,.T.);
#12799=EDGE_CURVE('',#9863,#9864,#6093,.T.);
#12800=EDGE_CURVE('',#9864,#9861,#6094,.T.);
#12801=EDGE_CURVE('',#9865,#9862,#425,.T.);
#12802=EDGE_CURVE('',#9866,#9865,#6995,.T.);
#12803=EDGE_CURVE('',#9863,#9866,#426,.T.);
#12804=EDGE_CURVE('',#9867,#9868,#6095,.T.);
#12805=EDGE_CURVE('',#9868,#9869,#6096,.T.);
#12806=EDGE_CURVE('',#9869,#9870,#6097,.T.);
#12807=EDGE_CURVE('',#9870,#9867,#6098,.T.);
#12808=EDGE_CURVE('',#9869,#9864,#4649,.T.);
#12809=EDGE_CURVE('',#9861,#9868,#4650,.T.);
#12810=EDGE_CURVE('',#9871,#9872,#6099,.T.);
#12811=EDGE_CURVE('',#9872,#9873,#6100,.T.);
#12812=EDGE_CURVE('',#9873,#9874,#6101,.T.);
#12813=EDGE_CURVE('',#9874,#9871,#6102,.T.);
#12814=EDGE_CURVE('',#9875,#9872,#427,.T.);
#12815=EDGE_CURVE('',#9876,#9875,#6996,.T.);
#12816=EDGE_CURVE('',#9873,#9876,#428,.T.);
#12817=EDGE_CURVE('',#9877,#9878,#6103,.T.);
#12818=EDGE_CURVE('',#9878,#9879,#6104,.T.);
#12819=EDGE_CURVE('',#9879,#9880,#6105,.T.);
#12820=EDGE_CURVE('',#9880,#9877,#6106,.T.);
#12821=EDGE_CURVE('',#9879,#9874,#4651,.T.);
#12822=EDGE_CURVE('',#9871,#9878,#4652,.T.);
#12823=EDGE_CURVE('',#9881,#9882,#6107,.T.);
#12824=EDGE_CURVE('',#9882,#9883,#6108,.T.);
#12825=EDGE_CURVE('',#9883,#9884,#6109,.T.);
#12826=EDGE_CURVE('',#9884,#9881,#6110,.T.);
#12827=EDGE_CURVE('',#9885,#9882,#429,.T.);
#12828=EDGE_CURVE('',#9886,#9885,#6997,.T.);
#12829=EDGE_CURVE('',#9883,#9886,#430,.T.);
#12830=EDGE_CURVE('',#9887,#9888,#6111,.T.);
#12831=EDGE_CURVE('',#9888,#9889,#6112,.T.);
#12832=EDGE_CURVE('',#9889,#9890,#6113,.T.);
#12833=EDGE_CURVE('',#9890,#9887,#6114,.T.);
#12834=EDGE_CURVE('',#9889,#9884,#4653,.T.);
#12835=EDGE_CURVE('',#9881,#9888,#4654,.T.);
#12836=EDGE_CURVE('',#9891,#9892,#6115,.T.);
#12837=EDGE_CURVE('',#9892,#9893,#6116,.T.);
#12838=EDGE_CURVE('',#9893,#9894,#6117,.T.);
#12839=EDGE_CURVE('',#9894,#9891,#6118,.T.);
#12840=EDGE_CURVE('',#9895,#9892,#431,.T.);
#12841=EDGE_CURVE('',#9896,#9895,#6998,.T.);
#12842=EDGE_CURVE('',#9893,#9896,#432,.T.);
#12843=EDGE_CURVE('',#9897,#9898,#6119,.T.);
#12844=EDGE_CURVE('',#9898,#9899,#6120,.T.);
#12845=EDGE_CURVE('',#9899,#9900,#6121,.T.);
#12846=EDGE_CURVE('',#9900,#9897,#6122,.T.);
#12847=EDGE_CURVE('',#9899,#9894,#4655,.T.);
#12848=EDGE_CURVE('',#9891,#9898,#4656,.T.);
#12849=EDGE_CURVE('',#9901,#9902,#6123,.T.);
#12850=EDGE_CURVE('',#9902,#9903,#6124,.T.);
#12851=EDGE_CURVE('',#9903,#9904,#6125,.T.);
#12852=EDGE_CURVE('',#9904,#9901,#6126,.T.);
#12853=EDGE_CURVE('',#9905,#9902,#433,.T.);
#12854=EDGE_CURVE('',#9906,#9905,#6999,.T.);
#12855=EDGE_CURVE('',#9903,#9906,#434,.T.);
#12856=EDGE_CURVE('',#9907,#9908,#6127,.T.);
#12857=EDGE_CURVE('',#9908,#9909,#6128,.T.);
#12858=EDGE_CURVE('',#9909,#9910,#6129,.T.);
#12859=EDGE_CURVE('',#9910,#9907,#6130,.T.);
#12860=EDGE_CURVE('',#9909,#9904,#4657,.T.);
#12861=EDGE_CURVE('',#9901,#9908,#4658,.T.);
#12862=EDGE_CURVE('',#9911,#9912,#6131,.T.);
#12863=EDGE_CURVE('',#9912,#9913,#6132,.T.);
#12864=EDGE_CURVE('',#9913,#9914,#6133,.T.);
#12865=EDGE_CURVE('',#9914,#9911,#6134,.T.);
#12866=EDGE_CURVE('',#9915,#9912,#435,.T.);
#12867=EDGE_CURVE('',#9916,#9915,#7000,.T.);
#12868=EDGE_CURVE('',#9913,#9916,#436,.T.);
#12869=EDGE_CURVE('',#9917,#9918,#6135,.T.);
#12870=EDGE_CURVE('',#9918,#9919,#6136,.T.);
#12871=EDGE_CURVE('',#9919,#9920,#6137,.T.);
#12872=EDGE_CURVE('',#9920,#9917,#6138,.T.);
#12873=EDGE_CURVE('',#9919,#9914,#4659,.T.);
#12874=EDGE_CURVE('',#9911,#9918,#4660,.T.);
#12875=EDGE_CURVE('',#9921,#9922,#6139,.T.);
#12876=EDGE_CURVE('',#9922,#9923,#6140,.T.);
#12877=EDGE_CURVE('',#9923,#9924,#6141,.T.);
#12878=EDGE_CURVE('',#9924,#9921,#6142,.T.);
#12879=EDGE_CURVE('',#9925,#9922,#437,.T.);
#12880=EDGE_CURVE('',#9926,#9925,#7001,.T.);
#12881=EDGE_CURVE('',#9923,#9926,#438,.T.);
#12882=EDGE_CURVE('',#9927,#9928,#6143,.T.);
#12883=EDGE_CURVE('',#9928,#9929,#6144,.T.);
#12884=EDGE_CURVE('',#9929,#9930,#6145,.T.);
#12885=EDGE_CURVE('',#9930,#9927,#6146,.T.);
#12886=EDGE_CURVE('',#9929,#9924,#4661,.T.);
#12887=EDGE_CURVE('',#9921,#9928,#4662,.T.);
#12888=EDGE_CURVE('',#9931,#9932,#6147,.T.);
#12889=EDGE_CURVE('',#9932,#9933,#6148,.T.);
#12890=EDGE_CURVE('',#9933,#9934,#6149,.T.);
#12891=EDGE_CURVE('',#9934,#9931,#6150,.T.);
#12892=EDGE_CURVE('',#9935,#9932,#439,.T.);
#12893=EDGE_CURVE('',#9936,#9935,#7002,.T.);
#12894=EDGE_CURVE('',#9933,#9936,#440,.T.);
#12895=EDGE_CURVE('',#9937,#9938,#6151,.T.);
#12896=EDGE_CURVE('',#9938,#9939,#6152,.T.);
#12897=EDGE_CURVE('',#9939,#9940,#6153,.T.);
#12898=EDGE_CURVE('',#9940,#9937,#6154,.T.);
#12899=EDGE_CURVE('',#9939,#9934,#4663,.T.);
#12900=EDGE_CURVE('',#9931,#9938,#4664,.T.);
#12901=EDGE_CURVE('',#9941,#9942,#6155,.T.);
#12902=EDGE_CURVE('',#9942,#9943,#6156,.T.);
#12903=EDGE_CURVE('',#9943,#9944,#6157,.T.);
#12904=EDGE_CURVE('',#9944,#9941,#6158,.T.);
#12905=EDGE_CURVE('',#9945,#9942,#441,.T.);
#12906=EDGE_CURVE('',#9946,#9945,#7003,.T.);
#12907=EDGE_CURVE('',#9943,#9946,#442,.T.);
#12908=EDGE_CURVE('',#9947,#9948,#6159,.T.);
#12909=EDGE_CURVE('',#9948,#9949,#6160,.T.);
#12910=EDGE_CURVE('',#9949,#9950,#6161,.T.);
#12911=EDGE_CURVE('',#9950,#9947,#6162,.T.);
#12912=EDGE_CURVE('',#9949,#9944,#4665,.T.);
#12913=EDGE_CURVE('',#9941,#9948,#4666,.T.);
#12914=EDGE_CURVE('',#9951,#9952,#6163,.T.);
#12915=EDGE_CURVE('',#9952,#9953,#6164,.T.);
#12916=EDGE_CURVE('',#9953,#9954,#6165,.T.);
#12917=EDGE_CURVE('',#9954,#9951,#6166,.T.);
#12918=EDGE_CURVE('',#9955,#9952,#443,.T.);
#12919=EDGE_CURVE('',#9956,#9955,#7004,.T.);
#12920=EDGE_CURVE('',#9953,#9956,#444,.T.);
#12921=EDGE_CURVE('',#9957,#9958,#6167,.T.);
#12922=EDGE_CURVE('',#9958,#9959,#6168,.T.);
#12923=EDGE_CURVE('',#9959,#9960,#6169,.T.);
#12924=EDGE_CURVE('',#9960,#9957,#6170,.T.);
#12925=EDGE_CURVE('',#9959,#9954,#4667,.T.);
#12926=EDGE_CURVE('',#9951,#9958,#4668,.T.);
#12927=EDGE_CURVE('',#9961,#9962,#6171,.T.);
#12928=EDGE_CURVE('',#9962,#9963,#6172,.T.);
#12929=EDGE_CURVE('',#9963,#9964,#6173,.T.);
#12930=EDGE_CURVE('',#9964,#9961,#6174,.T.);
#12931=EDGE_CURVE('',#9965,#9962,#445,.T.);
#12932=EDGE_CURVE('',#9966,#9965,#7005,.T.);
#12933=EDGE_CURVE('',#9963,#9966,#446,.T.);
#12934=EDGE_CURVE('',#9967,#9968,#6175,.T.);
#12935=EDGE_CURVE('',#9968,#9969,#6176,.T.);
#12936=EDGE_CURVE('',#9969,#9970,#6177,.T.);
#12937=EDGE_CURVE('',#9970,#9967,#6178,.T.);
#12938=EDGE_CURVE('',#9969,#9964,#4669,.T.);
#12939=EDGE_CURVE('',#9961,#9968,#4670,.T.);
#12940=EDGE_CURVE('',#9971,#9972,#6179,.T.);
#12941=EDGE_CURVE('',#9972,#9973,#6180,.T.);
#12942=EDGE_CURVE('',#9973,#9974,#6181,.T.);
#12943=EDGE_CURVE('',#9974,#9971,#6182,.T.);
#12944=EDGE_CURVE('',#9975,#9972,#447,.T.);
#12945=EDGE_CURVE('',#9976,#9975,#7006,.T.);
#12946=EDGE_CURVE('',#9973,#9976,#448,.T.);
#12947=EDGE_CURVE('',#9977,#9978,#6183,.T.);
#12948=EDGE_CURVE('',#9978,#9979,#6184,.T.);
#12949=EDGE_CURVE('',#9979,#9980,#6185,.T.);
#12950=EDGE_CURVE('',#9980,#9977,#6186,.T.);
#12951=EDGE_CURVE('',#9979,#9974,#4671,.T.);
#12952=EDGE_CURVE('',#9971,#9978,#4672,.T.);
#12953=EDGE_CURVE('',#9981,#9982,#6187,.T.);
#12954=EDGE_CURVE('',#9982,#9983,#6188,.T.);
#12955=EDGE_CURVE('',#9983,#9984,#6189,.T.);
#12956=EDGE_CURVE('',#9984,#9981,#6190,.T.);
#12957=EDGE_CURVE('',#9985,#9982,#449,.T.);
#12958=EDGE_CURVE('',#9986,#9985,#7007,.T.);
#12959=EDGE_CURVE('',#9983,#9986,#450,.T.);
#12960=EDGE_CURVE('',#9987,#9988,#6191,.T.);
#12961=EDGE_CURVE('',#9988,#9989,#6192,.T.);
#12962=EDGE_CURVE('',#9989,#9990,#6193,.T.);
#12963=EDGE_CURVE('',#9990,#9987,#6194,.T.);
#12964=EDGE_CURVE('',#9989,#9984,#4673,.T.);
#12965=EDGE_CURVE('',#9981,#9988,#4674,.T.);
#12966=EDGE_CURVE('',#9991,#9992,#6195,.T.);
#12967=EDGE_CURVE('',#9992,#9993,#6196,.T.);
#12968=EDGE_CURVE('',#9993,#9994,#6197,.T.);
#12969=EDGE_CURVE('',#9994,#9991,#6198,.T.);
#12970=EDGE_CURVE('',#9995,#9992,#451,.T.);
#12971=EDGE_CURVE('',#9996,#9995,#7008,.T.);
#12972=EDGE_CURVE('',#9993,#9996,#452,.T.);
#12973=EDGE_CURVE('',#9997,#9998,#6199,.T.);
#12974=EDGE_CURVE('',#9998,#9999,#6200,.T.);
#12975=EDGE_CURVE('',#9999,#10000,#6201,.T.);
#12976=EDGE_CURVE('',#10000,#9997,#6202,.T.);
#12977=EDGE_CURVE('',#9999,#9994,#4675,.T.);
#12978=EDGE_CURVE('',#9991,#9998,#4676,.T.);
#12979=EDGE_CURVE('',#10001,#10002,#6203,.T.);
#12980=EDGE_CURVE('',#10002,#10003,#6204,.T.);
#12981=EDGE_CURVE('',#10003,#10004,#6205,.T.);
#12982=EDGE_CURVE('',#10004,#10001,#6206,.T.);
#12983=EDGE_CURVE('',#10005,#10002,#453,.T.);
#12984=EDGE_CURVE('',#10006,#10005,#7009,.T.);
#12985=EDGE_CURVE('',#10003,#10006,#454,.T.);
#12986=EDGE_CURVE('',#10007,#10008,#6207,.T.);
#12987=EDGE_CURVE('',#10008,#10009,#6208,.T.);
#12988=EDGE_CURVE('',#10009,#10010,#6209,.T.);
#12989=EDGE_CURVE('',#10010,#10007,#6210,.T.);
#12990=EDGE_CURVE('',#10009,#10004,#4677,.T.);
#12991=EDGE_CURVE('',#10001,#10008,#4678,.T.);
#12992=EDGE_CURVE('',#10011,#10012,#6211,.T.);
#12993=EDGE_CURVE('',#10012,#10013,#6212,.T.);
#12994=EDGE_CURVE('',#10013,#10014,#6213,.T.);
#12995=EDGE_CURVE('',#10014,#10011,#6214,.T.);
#12996=EDGE_CURVE('',#10015,#10012,#455,.T.);
#12997=EDGE_CURVE('',#10016,#10015,#7010,.T.);
#12998=EDGE_CURVE('',#10013,#10016,#456,.T.);
#12999=EDGE_CURVE('',#10017,#10018,#6215,.T.);
#13000=EDGE_CURVE('',#10018,#10019,#6216,.T.);
#13001=EDGE_CURVE('',#10019,#10020,#6217,.T.);
#13002=EDGE_CURVE('',#10020,#10017,#6218,.T.);
#13003=EDGE_CURVE('',#10019,#10014,#4679,.T.);
#13004=EDGE_CURVE('',#10011,#10018,#4680,.T.);
#13005=EDGE_CURVE('',#10021,#10022,#6219,.T.);
#13006=EDGE_CURVE('',#10022,#10023,#6220,.T.);
#13007=EDGE_CURVE('',#10023,#10024,#6221,.T.);
#13008=EDGE_CURVE('',#10024,#10021,#6222,.T.);
#13009=EDGE_CURVE('',#10025,#10022,#457,.T.);
#13010=EDGE_CURVE('',#10026,#10025,#7011,.T.);
#13011=EDGE_CURVE('',#10023,#10026,#458,.T.);
#13012=EDGE_CURVE('',#10027,#10028,#6223,.T.);
#13013=EDGE_CURVE('',#10028,#10029,#6224,.T.);
#13014=EDGE_CURVE('',#10029,#10030,#6225,.T.);
#13015=EDGE_CURVE('',#10030,#10027,#6226,.T.);
#13016=EDGE_CURVE('',#10029,#10024,#4681,.T.);
#13017=EDGE_CURVE('',#10021,#10028,#4682,.T.);
#13018=EDGE_CURVE('',#10031,#10032,#6227,.T.);
#13019=EDGE_CURVE('',#10032,#10033,#6228,.T.);
#13020=EDGE_CURVE('',#10033,#10034,#6229,.T.);
#13021=EDGE_CURVE('',#10034,#10031,#6230,.T.);
#13022=EDGE_CURVE('',#10035,#10032,#459,.T.);
#13023=EDGE_CURVE('',#10036,#10035,#7012,.T.);
#13024=EDGE_CURVE('',#10033,#10036,#460,.T.);
#13025=EDGE_CURVE('',#10037,#10038,#6231,.T.);
#13026=EDGE_CURVE('',#10038,#10039,#6232,.T.);
#13027=EDGE_CURVE('',#10039,#10040,#6233,.T.);
#13028=EDGE_CURVE('',#10040,#10037,#6234,.T.);
#13029=EDGE_CURVE('',#10039,#10034,#4683,.T.);
#13030=EDGE_CURVE('',#10031,#10038,#4684,.T.);
#13031=EDGE_CURVE('',#10041,#10042,#6235,.T.);
#13032=EDGE_CURVE('',#10042,#10043,#6236,.T.);
#13033=EDGE_CURVE('',#10043,#10044,#6237,.T.);
#13034=EDGE_CURVE('',#10044,#10041,#6238,.T.);
#13035=EDGE_CURVE('',#10045,#10042,#461,.T.);
#13036=EDGE_CURVE('',#10046,#10045,#7013,.T.);
#13037=EDGE_CURVE('',#10043,#10046,#462,.T.);
#13038=EDGE_CURVE('',#10047,#10048,#6239,.T.);
#13039=EDGE_CURVE('',#10048,#10049,#6240,.T.);
#13040=EDGE_CURVE('',#10049,#10050,#6241,.T.);
#13041=EDGE_CURVE('',#10050,#10047,#6242,.T.);
#13042=EDGE_CURVE('',#10049,#10044,#4685,.T.);
#13043=EDGE_CURVE('',#10041,#10048,#4686,.T.);
#13044=EDGE_CURVE('',#10051,#10052,#6243,.T.);
#13045=EDGE_CURVE('',#10052,#10053,#6244,.T.);
#13046=EDGE_CURVE('',#10053,#10054,#6245,.T.);
#13047=EDGE_CURVE('',#10054,#10051,#6246,.T.);
#13048=EDGE_CURVE('',#10055,#10052,#463,.T.);
#13049=EDGE_CURVE('',#10056,#10055,#7014,.T.);
#13050=EDGE_CURVE('',#10053,#10056,#464,.T.);
#13051=EDGE_CURVE('',#10057,#10058,#6247,.T.);
#13052=EDGE_CURVE('',#10058,#10059,#6248,.T.);
#13053=EDGE_CURVE('',#10059,#10060,#6249,.T.);
#13054=EDGE_CURVE('',#10060,#10057,#6250,.T.);
#13055=EDGE_CURVE('',#10059,#10054,#4687,.T.);
#13056=EDGE_CURVE('',#10051,#10058,#4688,.T.);
#13057=EDGE_CURVE('',#10061,#10062,#6251,.T.);
#13058=EDGE_CURVE('',#10062,#10063,#6252,.T.);
#13059=EDGE_CURVE('',#10063,#10064,#6253,.T.);
#13060=EDGE_CURVE('',#10064,#10061,#6254,.T.);
#13061=EDGE_CURVE('',#10065,#10062,#465,.T.);
#13062=EDGE_CURVE('',#10066,#10065,#7015,.T.);
#13063=EDGE_CURVE('',#10063,#10066,#466,.T.);
#13064=EDGE_CURVE('',#10067,#10068,#6255,.T.);
#13065=EDGE_CURVE('',#10068,#10069,#6256,.T.);
#13066=EDGE_CURVE('',#10069,#10070,#6257,.T.);
#13067=EDGE_CURVE('',#10070,#10067,#6258,.T.);
#13068=EDGE_CURVE('',#10069,#10064,#4689,.T.);
#13069=EDGE_CURVE('',#10061,#10068,#4690,.T.);
#13070=EDGE_CURVE('',#10071,#10072,#6259,.T.);
#13071=EDGE_CURVE('',#10072,#10073,#6260,.T.);
#13072=EDGE_CURVE('',#10073,#10074,#6261,.T.);
#13073=EDGE_CURVE('',#10074,#10071,#6262,.T.);
#13074=EDGE_CURVE('',#10075,#10072,#467,.T.);
#13075=EDGE_CURVE('',#10076,#10075,#7016,.T.);
#13076=EDGE_CURVE('',#10073,#10076,#468,.T.);
#13077=EDGE_CURVE('',#10077,#10078,#6263,.T.);
#13078=EDGE_CURVE('',#10078,#10079,#6264,.T.);
#13079=EDGE_CURVE('',#10079,#10080,#6265,.T.);
#13080=EDGE_CURVE('',#10080,#10077,#6266,.T.);
#13081=EDGE_CURVE('',#10079,#10074,#4691,.T.);
#13082=EDGE_CURVE('',#10071,#10078,#4692,.T.);
#13083=EDGE_CURVE('',#10081,#10082,#6267,.T.);
#13084=EDGE_CURVE('',#10082,#10083,#6268,.T.);
#13085=EDGE_CURVE('',#10083,#10084,#6269,.T.);
#13086=EDGE_CURVE('',#10084,#10081,#6270,.T.);
#13087=EDGE_CURVE('',#10085,#10082,#469,.T.);
#13088=EDGE_CURVE('',#10086,#10085,#7017,.T.);
#13089=EDGE_CURVE('',#10083,#10086,#470,.T.);
#13090=EDGE_CURVE('',#10087,#10088,#6271,.T.);
#13091=EDGE_CURVE('',#10088,#10089,#6272,.T.);
#13092=EDGE_CURVE('',#10089,#10090,#6273,.T.);
#13093=EDGE_CURVE('',#10090,#10087,#6274,.T.);
#13094=EDGE_CURVE('',#10089,#10084,#4693,.T.);
#13095=EDGE_CURVE('',#10081,#10088,#4694,.T.);
#13096=EDGE_CURVE('',#10091,#10092,#6275,.T.);
#13097=EDGE_CURVE('',#10092,#10093,#6276,.T.);
#13098=EDGE_CURVE('',#10093,#10094,#6277,.T.);
#13099=EDGE_CURVE('',#10094,#10091,#6278,.T.);
#13100=EDGE_CURVE('',#10095,#10092,#471,.T.);
#13101=EDGE_CURVE('',#10096,#10095,#7018,.T.);
#13102=EDGE_CURVE('',#10093,#10096,#472,.T.);
#13103=EDGE_CURVE('',#10097,#10098,#6279,.T.);
#13104=EDGE_CURVE('',#10098,#10099,#6280,.T.);
#13105=EDGE_CURVE('',#10099,#10100,#6281,.T.);
#13106=EDGE_CURVE('',#10100,#10097,#6282,.T.);
#13107=EDGE_CURVE('',#10099,#10094,#4695,.T.);
#13108=EDGE_CURVE('',#10091,#10098,#4696,.T.);
#13109=EDGE_CURVE('',#10101,#10102,#6283,.T.);
#13110=EDGE_CURVE('',#10102,#10103,#6284,.T.);
#13111=EDGE_CURVE('',#10103,#10104,#6285,.T.);
#13112=EDGE_CURVE('',#10104,#10101,#6286,.T.);
#13113=EDGE_CURVE('',#10105,#10102,#473,.T.);
#13114=EDGE_CURVE('',#10106,#10105,#7019,.T.);
#13115=EDGE_CURVE('',#10103,#10106,#474,.T.);
#13116=EDGE_CURVE('',#10107,#10108,#6287,.T.);
#13117=EDGE_CURVE('',#10108,#10109,#6288,.T.);
#13118=EDGE_CURVE('',#10109,#10110,#6289,.T.);
#13119=EDGE_CURVE('',#10110,#10107,#6290,.T.);
#13120=EDGE_CURVE('',#10109,#10104,#4697,.T.);
#13121=EDGE_CURVE('',#10101,#10108,#4698,.T.);
#13122=EDGE_CURVE('',#10111,#10112,#6291,.T.);
#13123=EDGE_CURVE('',#10112,#10113,#6292,.T.);
#13124=EDGE_CURVE('',#10113,#10114,#6293,.T.);
#13125=EDGE_CURVE('',#10114,#10111,#6294,.T.);
#13126=EDGE_CURVE('',#10115,#10112,#475,.T.);
#13127=EDGE_CURVE('',#10116,#10115,#7020,.T.);
#13128=EDGE_CURVE('',#10113,#10116,#476,.T.);
#13129=EDGE_CURVE('',#10117,#10118,#6295,.T.);
#13130=EDGE_CURVE('',#10118,#10119,#6296,.T.);
#13131=EDGE_CURVE('',#10119,#10120,#6297,.T.);
#13132=EDGE_CURVE('',#10120,#10117,#6298,.T.);
#13133=EDGE_CURVE('',#10119,#10114,#4699,.T.);
#13134=EDGE_CURVE('',#10111,#10118,#4700,.T.);
#13135=EDGE_CURVE('',#10121,#10122,#6299,.T.);
#13136=EDGE_CURVE('',#10122,#10123,#6300,.T.);
#13137=EDGE_CURVE('',#10123,#10124,#6301,.T.);
#13138=EDGE_CURVE('',#10124,#10121,#6302,.T.);
#13139=EDGE_CURVE('',#10125,#10122,#477,.T.);
#13140=EDGE_CURVE('',#10126,#10125,#7021,.T.);
#13141=EDGE_CURVE('',#10123,#10126,#478,.T.);
#13142=EDGE_CURVE('',#10127,#10128,#6303,.T.);
#13143=EDGE_CURVE('',#10128,#10129,#6304,.T.);
#13144=EDGE_CURVE('',#10129,#10130,#6305,.T.);
#13145=EDGE_CURVE('',#10130,#10127,#6306,.T.);
#13146=EDGE_CURVE('',#10129,#10124,#4701,.T.);
#13147=EDGE_CURVE('',#10121,#10128,#4702,.T.);
#13148=EDGE_CURVE('',#10131,#10132,#6307,.T.);
#13149=EDGE_CURVE('',#10132,#10133,#6308,.T.);
#13150=EDGE_CURVE('',#10133,#10134,#6309,.T.);
#13151=EDGE_CURVE('',#10134,#10131,#6310,.T.);
#13152=EDGE_CURVE('',#10135,#10132,#479,.T.);
#13153=EDGE_CURVE('',#10136,#10135,#7022,.T.);
#13154=EDGE_CURVE('',#10133,#10136,#480,.T.);
#13155=EDGE_CURVE('',#10137,#10138,#6311,.T.);
#13156=EDGE_CURVE('',#10138,#10139,#6312,.T.);
#13157=EDGE_CURVE('',#10139,#10140,#6313,.T.);
#13158=EDGE_CURVE('',#10140,#10137,#6314,.T.);
#13159=EDGE_CURVE('',#10139,#10134,#4703,.T.);
#13160=EDGE_CURVE('',#10131,#10138,#4704,.T.);
#13161=EDGE_CURVE('',#10141,#10142,#6315,.T.);
#13162=EDGE_CURVE('',#10142,#10143,#6316,.T.);
#13163=EDGE_CURVE('',#10143,#10144,#6317,.T.);
#13164=EDGE_CURVE('',#10144,#10141,#6318,.T.);
#13165=EDGE_CURVE('',#10145,#10142,#481,.T.);
#13166=EDGE_CURVE('',#10146,#10145,#7023,.T.);
#13167=EDGE_CURVE('',#10143,#10146,#482,.T.);
#13168=EDGE_CURVE('',#10147,#10148,#6319,.T.);
#13169=EDGE_CURVE('',#10148,#10149,#6320,.T.);
#13170=EDGE_CURVE('',#10149,#10150,#6321,.T.);
#13171=EDGE_CURVE('',#10150,#10147,#6322,.T.);
#13172=EDGE_CURVE('',#10149,#10144,#4705,.T.);
#13173=EDGE_CURVE('',#10141,#10148,#4706,.T.);
#13174=EDGE_CURVE('',#10151,#10152,#6323,.T.);
#13175=EDGE_CURVE('',#10152,#10153,#6324,.T.);
#13176=EDGE_CURVE('',#10153,#10154,#6325,.T.);
#13177=EDGE_CURVE('',#10154,#10151,#6326,.T.);
#13178=EDGE_CURVE('',#10155,#10152,#483,.T.);
#13179=EDGE_CURVE('',#10156,#10155,#7024,.T.);
#13180=EDGE_CURVE('',#10153,#10156,#484,.T.);
#13181=EDGE_CURVE('',#10157,#10158,#6327,.T.);
#13182=EDGE_CURVE('',#10158,#10159,#6328,.T.);
#13183=EDGE_CURVE('',#10159,#10160,#6329,.T.);
#13184=EDGE_CURVE('',#10160,#10157,#6330,.T.);
#13185=EDGE_CURVE('',#10159,#10154,#4707,.T.);
#13186=EDGE_CURVE('',#10151,#10158,#4708,.T.);
#13187=EDGE_CURVE('',#10161,#10162,#6331,.T.);
#13188=EDGE_CURVE('',#10162,#10163,#6332,.T.);
#13189=EDGE_CURVE('',#10163,#10164,#6333,.T.);
#13190=EDGE_CURVE('',#10164,#10161,#6334,.T.);
#13191=EDGE_CURVE('',#10165,#10162,#485,.T.);
#13192=EDGE_CURVE('',#10166,#10165,#7025,.T.);
#13193=EDGE_CURVE('',#10163,#10166,#486,.T.);
#13194=EDGE_CURVE('',#10167,#10168,#6335,.T.);
#13195=EDGE_CURVE('',#10168,#10169,#6336,.T.);
#13196=EDGE_CURVE('',#10169,#10170,#6337,.T.);
#13197=EDGE_CURVE('',#10170,#10167,#6338,.T.);
#13198=EDGE_CURVE('',#10169,#10164,#4709,.T.);
#13199=EDGE_CURVE('',#10161,#10168,#4710,.T.);
#13200=EDGE_CURVE('',#10171,#10172,#6339,.T.);
#13201=EDGE_CURVE('',#10172,#10173,#6340,.T.);
#13202=EDGE_CURVE('',#10173,#10174,#6341,.T.);
#13203=EDGE_CURVE('',#10174,#10171,#6342,.T.);
#13204=EDGE_CURVE('',#10175,#10172,#487,.T.);
#13205=EDGE_CURVE('',#10176,#10175,#7026,.T.);
#13206=EDGE_CURVE('',#10173,#10176,#488,.T.);
#13207=EDGE_CURVE('',#10177,#10178,#6343,.T.);
#13208=EDGE_CURVE('',#10178,#10179,#6344,.T.);
#13209=EDGE_CURVE('',#10179,#10180,#6345,.T.);
#13210=EDGE_CURVE('',#10180,#10177,#6346,.T.);
#13211=EDGE_CURVE('',#10179,#10174,#4711,.T.);
#13212=EDGE_CURVE('',#10171,#10178,#4712,.T.);
#13213=EDGE_CURVE('',#10181,#10182,#6347,.T.);
#13214=EDGE_CURVE('',#10182,#10183,#6348,.T.);
#13215=EDGE_CURVE('',#10183,#10184,#6349,.T.);
#13216=EDGE_CURVE('',#10184,#10181,#6350,.T.);
#13217=EDGE_CURVE('',#10185,#10182,#489,.T.);
#13218=EDGE_CURVE('',#10186,#10185,#7027,.T.);
#13219=EDGE_CURVE('',#10183,#10186,#490,.T.);
#13220=EDGE_CURVE('',#10187,#10188,#6351,.T.);
#13221=EDGE_CURVE('',#10188,#10189,#6352,.T.);
#13222=EDGE_CURVE('',#10189,#10190,#6353,.T.);
#13223=EDGE_CURVE('',#10190,#10187,#6354,.T.);
#13224=EDGE_CURVE('',#10189,#10184,#4713,.T.);
#13225=EDGE_CURVE('',#10181,#10188,#4714,.T.);
#13226=EDGE_CURVE('',#10191,#10192,#6355,.T.);
#13227=EDGE_CURVE('',#10192,#10193,#6356,.T.);
#13228=EDGE_CURVE('',#10193,#10194,#6357,.T.);
#13229=EDGE_CURVE('',#10194,#10191,#6358,.T.);
#13230=EDGE_CURVE('',#10195,#10192,#491,.T.);
#13231=EDGE_CURVE('',#10196,#10195,#7028,.T.);
#13232=EDGE_CURVE('',#10193,#10196,#492,.T.);
#13233=EDGE_CURVE('',#10197,#10198,#6359,.T.);
#13234=EDGE_CURVE('',#10198,#10199,#6360,.T.);
#13235=EDGE_CURVE('',#10199,#10200,#6361,.T.);
#13236=EDGE_CURVE('',#10200,#10197,#6362,.T.);
#13237=EDGE_CURVE('',#10199,#10194,#4715,.T.);
#13238=EDGE_CURVE('',#10191,#10198,#4716,.T.);
#13239=EDGE_CURVE('',#10201,#10202,#6363,.T.);
#13240=EDGE_CURVE('',#10202,#10203,#6364,.T.);
#13241=EDGE_CURVE('',#10203,#10204,#6365,.T.);
#13242=EDGE_CURVE('',#10204,#10201,#6366,.T.);
#13243=EDGE_CURVE('',#10205,#10202,#493,.T.);
#13244=EDGE_CURVE('',#10206,#10205,#7029,.T.);
#13245=EDGE_CURVE('',#10203,#10206,#494,.T.);
#13246=EDGE_CURVE('',#10207,#10208,#6367,.T.);
#13247=EDGE_CURVE('',#10208,#10209,#6368,.T.);
#13248=EDGE_CURVE('',#10209,#10210,#6369,.T.);
#13249=EDGE_CURVE('',#10210,#10207,#6370,.T.);
#13250=EDGE_CURVE('',#10209,#10204,#4717,.T.);
#13251=EDGE_CURVE('',#10201,#10208,#4718,.T.);
#13252=EDGE_CURVE('',#10211,#10212,#6371,.T.);
#13253=EDGE_CURVE('',#10212,#10213,#6372,.T.);
#13254=EDGE_CURVE('',#10213,#10214,#6373,.T.);
#13255=EDGE_CURVE('',#10214,#10211,#6374,.T.);
#13256=EDGE_CURVE('',#10215,#10212,#495,.T.);
#13257=EDGE_CURVE('',#10216,#10215,#7030,.T.);
#13258=EDGE_CURVE('',#10213,#10216,#496,.T.);
#13259=EDGE_CURVE('',#10217,#10218,#6375,.T.);
#13260=EDGE_CURVE('',#10218,#10219,#6376,.T.);
#13261=EDGE_CURVE('',#10219,#10220,#6377,.T.);
#13262=EDGE_CURVE('',#10220,#10217,#6378,.T.);
#13263=EDGE_CURVE('',#10219,#10214,#4719,.T.);
#13264=EDGE_CURVE('',#10211,#10218,#4720,.T.);
#13265=EDGE_CURVE('',#10221,#10222,#6379,.T.);
#13266=EDGE_CURVE('',#10222,#10223,#6380,.T.);
#13267=EDGE_CURVE('',#10223,#10224,#6381,.T.);
#13268=EDGE_CURVE('',#10224,#10221,#6382,.T.);
#13269=EDGE_CURVE('',#10225,#10222,#497,.T.);
#13270=EDGE_CURVE('',#10226,#10225,#7031,.T.);
#13271=EDGE_CURVE('',#10223,#10226,#498,.T.);
#13272=EDGE_CURVE('',#10227,#10228,#6383,.T.);
#13273=EDGE_CURVE('',#10228,#10229,#6384,.T.);
#13274=EDGE_CURVE('',#10229,#10230,#6385,.T.);
#13275=EDGE_CURVE('',#10230,#10227,#6386,.T.);
#13276=EDGE_CURVE('',#10229,#10224,#4721,.T.);
#13277=EDGE_CURVE('',#10221,#10228,#4722,.T.);
#13278=EDGE_CURVE('',#10231,#10232,#6387,.T.);
#13279=EDGE_CURVE('',#10232,#10233,#6388,.T.);
#13280=EDGE_CURVE('',#10233,#10234,#6389,.T.);
#13281=EDGE_CURVE('',#10234,#10231,#6390,.T.);
#13282=EDGE_CURVE('',#10235,#10232,#499,.T.);
#13283=EDGE_CURVE('',#10236,#10235,#7032,.T.);
#13284=EDGE_CURVE('',#10233,#10236,#500,.T.);
#13285=EDGE_CURVE('',#10237,#10238,#6391,.T.);
#13286=EDGE_CURVE('',#10238,#10239,#6392,.T.);
#13287=EDGE_CURVE('',#10239,#10240,#6393,.T.);
#13288=EDGE_CURVE('',#10240,#10237,#6394,.T.);
#13289=EDGE_CURVE('',#10239,#10234,#4723,.T.);
#13290=EDGE_CURVE('',#10231,#10238,#4724,.T.);
#13291=EDGE_CURVE('',#10241,#10242,#6395,.T.);
#13292=EDGE_CURVE('',#10242,#10243,#6396,.T.);
#13293=EDGE_CURVE('',#10243,#10244,#6397,.T.);
#13294=EDGE_CURVE('',#10244,#10241,#6398,.T.);
#13295=EDGE_CURVE('',#10245,#10242,#501,.T.);
#13296=EDGE_CURVE('',#10246,#10245,#7033,.T.);
#13297=EDGE_CURVE('',#10243,#10246,#502,.T.);
#13298=EDGE_CURVE('',#10247,#10248,#6399,.T.);
#13299=EDGE_CURVE('',#10248,#10249,#6400,.T.);
#13300=EDGE_CURVE('',#10249,#10250,#6401,.T.);
#13301=EDGE_CURVE('',#10250,#10247,#6402,.T.);
#13302=EDGE_CURVE('',#10249,#10244,#4725,.T.);
#13303=EDGE_CURVE('',#10241,#10248,#4726,.T.);
#13304=EDGE_CURVE('',#10251,#10252,#6403,.T.);
#13305=EDGE_CURVE('',#10252,#10253,#6404,.T.);
#13306=EDGE_CURVE('',#10253,#10254,#6405,.T.);
#13307=EDGE_CURVE('',#10254,#10251,#6406,.T.);
#13308=EDGE_CURVE('',#10255,#10252,#503,.T.);
#13309=EDGE_CURVE('',#10256,#10255,#7034,.T.);
#13310=EDGE_CURVE('',#10253,#10256,#504,.T.);
#13311=EDGE_CURVE('',#10257,#10258,#6407,.T.);
#13312=EDGE_CURVE('',#10258,#10259,#6408,.T.);
#13313=EDGE_CURVE('',#10259,#10260,#6409,.T.);
#13314=EDGE_CURVE('',#10260,#10257,#6410,.T.);
#13315=EDGE_CURVE('',#10259,#10254,#4727,.T.);
#13316=EDGE_CURVE('',#10251,#10258,#4728,.T.);
#13317=EDGE_CURVE('',#10261,#10262,#6411,.T.);
#13318=EDGE_CURVE('',#10262,#10263,#6412,.T.);
#13319=EDGE_CURVE('',#10263,#10264,#6413,.T.);
#13320=EDGE_CURVE('',#10264,#10261,#6414,.T.);
#13321=EDGE_CURVE('',#10265,#10262,#505,.T.);
#13322=EDGE_CURVE('',#10266,#10265,#7035,.T.);
#13323=EDGE_CURVE('',#10263,#10266,#506,.T.);
#13324=EDGE_CURVE('',#10267,#10268,#6415,.T.);
#13325=EDGE_CURVE('',#10268,#10269,#6416,.T.);
#13326=EDGE_CURVE('',#10269,#10270,#6417,.T.);
#13327=EDGE_CURVE('',#10270,#10267,#6418,.T.);
#13328=EDGE_CURVE('',#10269,#10264,#4729,.T.);
#13329=EDGE_CURVE('',#10261,#10268,#4730,.T.);
#13330=EDGE_CURVE('',#10271,#10272,#6419,.T.);
#13331=EDGE_CURVE('',#10272,#10273,#6420,.T.);
#13332=EDGE_CURVE('',#10273,#10274,#6421,.T.);
#13333=EDGE_CURVE('',#10274,#10271,#6422,.T.);
#13334=EDGE_CURVE('',#10275,#10272,#507,.T.);
#13335=EDGE_CURVE('',#10276,#10275,#7036,.T.);
#13336=EDGE_CURVE('',#10273,#10276,#508,.T.);
#13337=EDGE_CURVE('',#10277,#10278,#6423,.T.);
#13338=EDGE_CURVE('',#10278,#10279,#6424,.T.);
#13339=EDGE_CURVE('',#10279,#10280,#6425,.T.);
#13340=EDGE_CURVE('',#10280,#10277,#6426,.T.);
#13341=EDGE_CURVE('',#10279,#10274,#4731,.T.);
#13342=EDGE_CURVE('',#10271,#10278,#4732,.T.);
#13343=EDGE_CURVE('',#10281,#10282,#6427,.T.);
#13344=EDGE_CURVE('',#10282,#10283,#6428,.T.);
#13345=EDGE_CURVE('',#10283,#10284,#6429,.T.);
#13346=EDGE_CURVE('',#10284,#10281,#6430,.T.);
#13347=EDGE_CURVE('',#10285,#10282,#509,.T.);
#13348=EDGE_CURVE('',#10286,#10285,#7037,.T.);
#13349=EDGE_CURVE('',#10283,#10286,#510,.T.);
#13350=EDGE_CURVE('',#10287,#10288,#6431,.T.);
#13351=EDGE_CURVE('',#10288,#10289,#6432,.T.);
#13352=EDGE_CURVE('',#10289,#10290,#6433,.T.);
#13353=EDGE_CURVE('',#10290,#10287,#6434,.T.);
#13354=EDGE_CURVE('',#10289,#10284,#4733,.T.);
#13355=EDGE_CURVE('',#10281,#10288,#4734,.T.);
#13356=EDGE_CURVE('',#10291,#10292,#6435,.T.);
#13357=EDGE_CURVE('',#10292,#10293,#6436,.T.);
#13358=EDGE_CURVE('',#10293,#10294,#6437,.T.);
#13359=EDGE_CURVE('',#10294,#10291,#6438,.T.);
#13360=EDGE_CURVE('',#10295,#10292,#511,.T.);
#13361=EDGE_CURVE('',#10296,#10295,#7038,.T.);
#13362=EDGE_CURVE('',#10293,#10296,#512,.T.);
#13363=EDGE_CURVE('',#10297,#10298,#6439,.T.);
#13364=EDGE_CURVE('',#10298,#10299,#6440,.T.);
#13365=EDGE_CURVE('',#10299,#10300,#6441,.T.);
#13366=EDGE_CURVE('',#10300,#10297,#6442,.T.);
#13367=EDGE_CURVE('',#10299,#10294,#4735,.T.);
#13368=EDGE_CURVE('',#10291,#10298,#4736,.T.);
#13369=EDGE_CURVE('',#10301,#10302,#6443,.T.);
#13370=EDGE_CURVE('',#10302,#10303,#6444,.T.);
#13371=EDGE_CURVE('',#10303,#10304,#6445,.T.);
#13372=EDGE_CURVE('',#10304,#10301,#6446,.T.);
#13373=EDGE_CURVE('',#10305,#10302,#513,.T.);
#13374=EDGE_CURVE('',#10306,#10305,#7039,.T.);
#13375=EDGE_CURVE('',#10303,#10306,#514,.T.);
#13376=EDGE_CURVE('',#10307,#10308,#6447,.T.);
#13377=EDGE_CURVE('',#10308,#10309,#6448,.T.);
#13378=EDGE_CURVE('',#10309,#10310,#6449,.T.);
#13379=EDGE_CURVE('',#10310,#10307,#6450,.T.);
#13380=EDGE_CURVE('',#10309,#10304,#4737,.T.);
#13381=EDGE_CURVE('',#10301,#10308,#4738,.T.);
#13382=EDGE_CURVE('',#10311,#10312,#6451,.T.);
#13383=EDGE_CURVE('',#10312,#10313,#6452,.T.);
#13384=EDGE_CURVE('',#10313,#10314,#6453,.T.);
#13385=EDGE_CURVE('',#10314,#10311,#6454,.T.);
#13386=EDGE_CURVE('',#10315,#10312,#515,.T.);
#13387=EDGE_CURVE('',#10316,#10315,#7040,.T.);
#13388=EDGE_CURVE('',#10313,#10316,#516,.T.);
#13389=EDGE_CURVE('',#10317,#10318,#6455,.T.);
#13390=EDGE_CURVE('',#10318,#10319,#6456,.T.);
#13391=EDGE_CURVE('',#10319,#10320,#6457,.T.);
#13392=EDGE_CURVE('',#10320,#10317,#6458,.T.);
#13393=EDGE_CURVE('',#10319,#10314,#4739,.T.);
#13394=EDGE_CURVE('',#10311,#10318,#4740,.T.);
#13395=EDGE_CURVE('',#10321,#10322,#6459,.T.);
#13396=EDGE_CURVE('',#10322,#10323,#6460,.T.);
#13397=EDGE_CURVE('',#10323,#10324,#6461,.T.);
#13398=EDGE_CURVE('',#10324,#10321,#6462,.T.);
#13399=EDGE_CURVE('',#10325,#10322,#517,.T.);
#13400=EDGE_CURVE('',#10326,#10325,#7041,.T.);
#13401=EDGE_CURVE('',#10323,#10326,#518,.T.);
#13402=EDGE_CURVE('',#10327,#10328,#6463,.T.);
#13403=EDGE_CURVE('',#10328,#10329,#6464,.T.);
#13404=EDGE_CURVE('',#10329,#10330,#6465,.T.);
#13405=EDGE_CURVE('',#10330,#10327,#6466,.T.);
#13406=EDGE_CURVE('',#10329,#10324,#4741,.T.);
#13407=EDGE_CURVE('',#10321,#10328,#4742,.T.);
#13408=EDGE_CURVE('',#10331,#10332,#6467,.T.);
#13409=EDGE_CURVE('',#10332,#10333,#6468,.T.);
#13410=EDGE_CURVE('',#10333,#10334,#6469,.T.);
#13411=EDGE_CURVE('',#10334,#10331,#6470,.T.);
#13412=EDGE_CURVE('',#10335,#10332,#519,.T.);
#13413=EDGE_CURVE('',#10336,#10335,#7042,.T.);
#13414=EDGE_CURVE('',#10333,#10336,#520,.T.);
#13415=EDGE_CURVE('',#10337,#10338,#6471,.T.);
#13416=EDGE_CURVE('',#10338,#10339,#6472,.T.);
#13417=EDGE_CURVE('',#10339,#10340,#6473,.T.);
#13418=EDGE_CURVE('',#10340,#10337,#6474,.T.);
#13419=EDGE_CURVE('',#10339,#10334,#4743,.T.);
#13420=EDGE_CURVE('',#10331,#10338,#4744,.T.);
#13421=EDGE_CURVE('',#10341,#10342,#6475,.T.);
#13422=EDGE_CURVE('',#10342,#10343,#6476,.T.);
#13423=EDGE_CURVE('',#10343,#10344,#6477,.T.);
#13424=EDGE_CURVE('',#10344,#10341,#6478,.T.);
#13425=EDGE_CURVE('',#10345,#10342,#521,.T.);
#13426=EDGE_CURVE('',#10346,#10345,#7043,.T.);
#13427=EDGE_CURVE('',#10343,#10346,#522,.T.);
#13428=EDGE_CURVE('',#10347,#10348,#6479,.T.);
#13429=EDGE_CURVE('',#10348,#10349,#6480,.T.);
#13430=EDGE_CURVE('',#10349,#10350,#6481,.T.);
#13431=EDGE_CURVE('',#10350,#10347,#6482,.T.);
#13432=EDGE_CURVE('',#10349,#10344,#4745,.T.);
#13433=EDGE_CURVE('',#10341,#10348,#4746,.T.);
#13434=EDGE_CURVE('',#10351,#10352,#6483,.T.);
#13435=EDGE_CURVE('',#10352,#10353,#6484,.T.);
#13436=EDGE_CURVE('',#10353,#10354,#6485,.T.);
#13437=EDGE_CURVE('',#10354,#10351,#6486,.T.);
#13438=EDGE_CURVE('',#10355,#10352,#523,.T.);
#13439=EDGE_CURVE('',#10356,#10355,#7044,.T.);
#13440=EDGE_CURVE('',#10353,#10356,#524,.T.);
#13441=EDGE_CURVE('',#10357,#10358,#6487,.T.);
#13442=EDGE_CURVE('',#10358,#10359,#6488,.T.);
#13443=EDGE_CURVE('',#10359,#10360,#6489,.T.);
#13444=EDGE_CURVE('',#10360,#10357,#6490,.T.);
#13445=EDGE_CURVE('',#10359,#10354,#4747,.T.);
#13446=EDGE_CURVE('',#10351,#10358,#4748,.T.);
#13447=EDGE_CURVE('',#10361,#10362,#6491,.T.);
#13448=EDGE_CURVE('',#10362,#10363,#6492,.T.);
#13449=EDGE_CURVE('',#10363,#10364,#6493,.T.);
#13450=EDGE_CURVE('',#10364,#10361,#6494,.T.);
#13451=EDGE_CURVE('',#10365,#10362,#525,.T.);
#13452=EDGE_CURVE('',#10366,#10365,#7045,.T.);
#13453=EDGE_CURVE('',#10363,#10366,#526,.T.);
#13454=EDGE_CURVE('',#10367,#10368,#6495,.T.);
#13455=EDGE_CURVE('',#10368,#10369,#6496,.T.);
#13456=EDGE_CURVE('',#10369,#10370,#6497,.T.);
#13457=EDGE_CURVE('',#10370,#10367,#6498,.T.);
#13458=EDGE_CURVE('',#10369,#10364,#4749,.T.);
#13459=EDGE_CURVE('',#10361,#10368,#4750,.T.);
#13460=EDGE_CURVE('',#10371,#10372,#6499,.T.);
#13461=EDGE_CURVE('',#10372,#10373,#6500,.T.);
#13462=EDGE_CURVE('',#10373,#10374,#6501,.T.);
#13463=EDGE_CURVE('',#10374,#10371,#6502,.T.);
#13464=EDGE_CURVE('',#10375,#10372,#527,.T.);
#13465=EDGE_CURVE('',#10376,#10375,#7046,.T.);
#13466=EDGE_CURVE('',#10373,#10376,#528,.T.);
#13467=EDGE_CURVE('',#10377,#10378,#6503,.T.);
#13468=EDGE_CURVE('',#10378,#10379,#6504,.T.);
#13469=EDGE_CURVE('',#10379,#10380,#6505,.T.);
#13470=EDGE_CURVE('',#10380,#10377,#6506,.T.);
#13471=EDGE_CURVE('',#10379,#10374,#4751,.T.);
#13472=EDGE_CURVE('',#10371,#10378,#4752,.T.);
#13473=EDGE_CURVE('',#10381,#10382,#6507,.T.);
#13474=EDGE_CURVE('',#10382,#10383,#6508,.T.);
#13475=EDGE_CURVE('',#10383,#10384,#6509,.T.);
#13476=EDGE_CURVE('',#10384,#10381,#6510,.T.);
#13477=EDGE_CURVE('',#10385,#10382,#529,.T.);
#13478=EDGE_CURVE('',#10386,#10385,#7047,.T.);
#13479=EDGE_CURVE('',#10383,#10386,#530,.T.);
#13480=EDGE_CURVE('',#10387,#10388,#6511,.T.);
#13481=EDGE_CURVE('',#10388,#10389,#6512,.T.);
#13482=EDGE_CURVE('',#10389,#10390,#6513,.T.);
#13483=EDGE_CURVE('',#10390,#10387,#6514,.T.);
#13484=EDGE_CURVE('',#10389,#10384,#4753,.T.);
#13485=EDGE_CURVE('',#10381,#10388,#4754,.T.);
#13486=EDGE_CURVE('',#10391,#10392,#6515,.T.);
#13487=EDGE_CURVE('',#10392,#10393,#6516,.T.);
#13488=EDGE_CURVE('',#10393,#10394,#6517,.T.);
#13489=EDGE_CURVE('',#10394,#10391,#6518,.T.);
#13490=EDGE_CURVE('',#10395,#10392,#531,.T.);
#13491=EDGE_CURVE('',#10396,#10395,#7048,.T.);
#13492=EDGE_CURVE('',#10393,#10396,#532,.T.);
#13493=EDGE_CURVE('',#10397,#10398,#6519,.T.);
#13494=EDGE_CURVE('',#10398,#10399,#6520,.T.);
#13495=EDGE_CURVE('',#10399,#10400,#6521,.T.);
#13496=EDGE_CURVE('',#10400,#10397,#6522,.T.);
#13497=EDGE_CURVE('',#10399,#10394,#4755,.T.);
#13498=EDGE_CURVE('',#10391,#10398,#4756,.T.);
#13499=EDGE_CURVE('',#10401,#10402,#6523,.T.);
#13500=EDGE_CURVE('',#10402,#10403,#6524,.T.);
#13501=EDGE_CURVE('',#10403,#10404,#6525,.T.);
#13502=EDGE_CURVE('',#10404,#10401,#6526,.T.);
#13503=EDGE_CURVE('',#10405,#10402,#533,.T.);
#13504=EDGE_CURVE('',#10406,#10405,#7049,.T.);
#13505=EDGE_CURVE('',#10403,#10406,#534,.T.);
#13506=EDGE_CURVE('',#10407,#10408,#6527,.T.);
#13507=EDGE_CURVE('',#10408,#10409,#6528,.T.);
#13508=EDGE_CURVE('',#10409,#10410,#6529,.T.);
#13509=EDGE_CURVE('',#10410,#10407,#6530,.T.);
#13510=EDGE_CURVE('',#10409,#10404,#4757,.T.);
#13511=EDGE_CURVE('',#10401,#10408,#4758,.T.);
#13512=EDGE_CURVE('',#10411,#10412,#6531,.T.);
#13513=EDGE_CURVE('',#10412,#10413,#6532,.T.);
#13514=EDGE_CURVE('',#10413,#10414,#6533,.T.);
#13515=EDGE_CURVE('',#10414,#10411,#6534,.T.);
#13516=EDGE_CURVE('',#10415,#10412,#535,.T.);
#13517=EDGE_CURVE('',#10416,#10415,#7050,.T.);
#13518=EDGE_CURVE('',#10413,#10416,#536,.T.);
#13519=EDGE_CURVE('',#10417,#10418,#6535,.T.);
#13520=EDGE_CURVE('',#10418,#10419,#6536,.T.);
#13521=EDGE_CURVE('',#10419,#10420,#6537,.T.);
#13522=EDGE_CURVE('',#10420,#10417,#6538,.T.);
#13523=EDGE_CURVE('',#10419,#10414,#4759,.T.);
#13524=EDGE_CURVE('',#10411,#10418,#4760,.T.);
#13525=EDGE_CURVE('',#10421,#10422,#6539,.T.);
#13526=EDGE_CURVE('',#10422,#10423,#6540,.T.);
#13527=EDGE_CURVE('',#10423,#10424,#6541,.T.);
#13528=EDGE_CURVE('',#10424,#10421,#6542,.T.);
#13529=EDGE_CURVE('',#10425,#10422,#537,.T.);
#13530=EDGE_CURVE('',#10426,#10425,#7051,.T.);
#13531=EDGE_CURVE('',#10423,#10426,#538,.T.);
#13532=EDGE_CURVE('',#10427,#10428,#6543,.T.);
#13533=EDGE_CURVE('',#10428,#10429,#6544,.T.);
#13534=EDGE_CURVE('',#10429,#10430,#6545,.T.);
#13535=EDGE_CURVE('',#10430,#10427,#6546,.T.);
#13536=EDGE_CURVE('',#10429,#10424,#4761,.T.);
#13537=EDGE_CURVE('',#10421,#10428,#4762,.T.);
#13538=EDGE_CURVE('',#10431,#10432,#6547,.T.);
#13539=EDGE_CURVE('',#10432,#10433,#6548,.T.);
#13540=EDGE_CURVE('',#10433,#10434,#6549,.T.);
#13541=EDGE_CURVE('',#10434,#10431,#6550,.T.);
#13542=EDGE_CURVE('',#10435,#10432,#539,.T.);
#13543=EDGE_CURVE('',#10436,#10435,#7052,.T.);
#13544=EDGE_CURVE('',#10433,#10436,#540,.T.);
#13545=EDGE_CURVE('',#10437,#10438,#6551,.T.);
#13546=EDGE_CURVE('',#10438,#10439,#6552,.T.);
#13547=EDGE_CURVE('',#10439,#10440,#6553,.T.);
#13548=EDGE_CURVE('',#10440,#10437,#6554,.T.);
#13549=EDGE_CURVE('',#10439,#10434,#4763,.T.);
#13550=EDGE_CURVE('',#10431,#10438,#4764,.T.);
#13551=EDGE_CURVE('',#10441,#10442,#6555,.T.);
#13552=EDGE_CURVE('',#10442,#10443,#6556,.T.);
#13553=EDGE_CURVE('',#10443,#10444,#6557,.T.);
#13554=EDGE_CURVE('',#10444,#10441,#6558,.T.);
#13555=EDGE_CURVE('',#10445,#10442,#541,.T.);
#13556=EDGE_CURVE('',#10446,#10445,#7053,.T.);
#13557=EDGE_CURVE('',#10443,#10446,#542,.T.);
#13558=EDGE_CURVE('',#10447,#10448,#6559,.T.);
#13559=EDGE_CURVE('',#10448,#10449,#6560,.T.);
#13560=EDGE_CURVE('',#10449,#10450,#6561,.T.);
#13561=EDGE_CURVE('',#10450,#10447,#6562,.T.);
#13562=EDGE_CURVE('',#10449,#10444,#4765,.T.);
#13563=EDGE_CURVE('',#10441,#10448,#4766,.T.);
#13564=EDGE_CURVE('',#10451,#10452,#6563,.T.);
#13565=EDGE_CURVE('',#10452,#10453,#6564,.T.);
#13566=EDGE_CURVE('',#10453,#10454,#6565,.T.);
#13567=EDGE_CURVE('',#10454,#10451,#6566,.T.);
#13568=EDGE_CURVE('',#10455,#10452,#543,.T.);
#13569=EDGE_CURVE('',#10456,#10455,#7054,.T.);
#13570=EDGE_CURVE('',#10453,#10456,#544,.T.);
#13571=EDGE_CURVE('',#10457,#10458,#6567,.T.);
#13572=EDGE_CURVE('',#10458,#10459,#6568,.T.);
#13573=EDGE_CURVE('',#10459,#10460,#6569,.T.);
#13574=EDGE_CURVE('',#10460,#10457,#6570,.T.);
#13575=EDGE_CURVE('',#10459,#10454,#4767,.T.);
#13576=EDGE_CURVE('',#10451,#10458,#4768,.T.);
#13577=EDGE_CURVE('',#10461,#9760,#545,.T.);
#13578=EDGE_CURVE('',#10462,#10461,#7055,.T.);
#13579=EDGE_CURVE('',#9757,#10462,#546,.T.);
#13580=EDGE_CURVE('',#10463,#9770,#547,.T.);
#13581=EDGE_CURVE('',#10464,#10463,#7056,.T.);
#13582=EDGE_CURVE('',#9767,#10464,#548,.T.);
#13583=EDGE_CURVE('',#10465,#9780,#549,.T.);
#13584=EDGE_CURVE('',#10466,#10465,#7057,.T.);
#13585=EDGE_CURVE('',#9777,#10466,#550,.T.);
#13586=EDGE_CURVE('',#10467,#9790,#551,.T.);
#13587=EDGE_CURVE('',#10468,#10467,#7058,.T.);
#13588=EDGE_CURVE('',#9787,#10468,#552,.T.);
#13589=EDGE_CURVE('',#10469,#9800,#553,.T.);
#13590=EDGE_CURVE('',#10470,#10469,#7059,.T.);
#13591=EDGE_CURVE('',#9797,#10470,#554,.T.);
#13592=EDGE_CURVE('',#10471,#9810,#555,.T.);
#13593=EDGE_CURVE('',#10472,#10471,#7060,.T.);
#13594=EDGE_CURVE('',#9807,#10472,#556,.T.);
#13595=EDGE_CURVE('',#10473,#9820,#557,.T.);
#13596=EDGE_CURVE('',#10474,#10473,#7061,.T.);
#13597=EDGE_CURVE('',#9817,#10474,#558,.T.);
#13598=EDGE_CURVE('',#10475,#9830,#559,.T.);
#13599=EDGE_CURVE('',#10476,#10475,#7062,.T.);
#13600=EDGE_CURVE('',#9827,#10476,#560,.T.);
#13601=EDGE_CURVE('',#10477,#9840,#561,.T.);
#13602=EDGE_CURVE('',#10478,#10477,#7063,.T.);
#13603=EDGE_CURVE('',#9837,#10478,#562,.T.);
#13604=EDGE_CURVE('',#10479,#9850,#563,.T.);
#13605=EDGE_CURVE('',#10480,#10479,#7064,.T.);
#13606=EDGE_CURVE('',#9847,#10480,#564,.T.);
#13607=EDGE_CURVE('',#10481,#9860,#565,.T.);
#13608=EDGE_CURVE('',#10482,#10481,#7065,.T.);
#13609=EDGE_CURVE('',#9857,#10482,#566,.T.);
#13610=EDGE_CURVE('',#10483,#9870,#567,.T.);
#13611=EDGE_CURVE('',#10484,#10483,#7066,.T.);
#13612=EDGE_CURVE('',#9867,#10484,#568,.T.);
#13613=EDGE_CURVE('',#10485,#9880,#569,.T.);
#13614=EDGE_CURVE('',#10486,#10485,#7067,.T.);
#13615=EDGE_CURVE('',#9877,#10486,#570,.T.);
#13616=EDGE_CURVE('',#10487,#9890,#571,.T.);
#13617=EDGE_CURVE('',#10488,#10487,#7068,.T.);
#13618=EDGE_CURVE('',#9887,#10488,#572,.T.);
#13619=EDGE_CURVE('',#10489,#9900,#573,.T.);
#13620=EDGE_CURVE('',#10490,#10489,#7069,.T.);
#13621=EDGE_CURVE('',#9897,#10490,#574,.T.);
#13622=EDGE_CURVE('',#10491,#9910,#575,.T.);
#13623=EDGE_CURVE('',#10492,#10491,#7070,.T.);
#13624=EDGE_CURVE('',#9907,#10492,#576,.T.);
#13625=EDGE_CURVE('',#10493,#9920,#577,.T.);
#13626=EDGE_CURVE('',#10494,#10493,#7071,.T.);
#13627=EDGE_CURVE('',#9917,#10494,#578,.T.);
#13628=EDGE_CURVE('',#10495,#9930,#579,.T.);
#13629=EDGE_CURVE('',#10496,#10495,#7072,.T.);
#13630=EDGE_CURVE('',#9927,#10496,#580,.T.);
#13631=EDGE_CURVE('',#10497,#9940,#581,.T.);
#13632=EDGE_CURVE('',#10498,#10497,#7073,.T.);
#13633=EDGE_CURVE('',#9937,#10498,#582,.T.);
#13634=EDGE_CURVE('',#10499,#9950,#583,.T.);
#13635=EDGE_CURVE('',#10500,#10499,#7074,.T.);
#13636=EDGE_CURVE('',#9947,#10500,#584,.T.);
#13637=EDGE_CURVE('',#10501,#9960,#585,.T.);
#13638=EDGE_CURVE('',#10502,#10501,#7075,.T.);
#13639=EDGE_CURVE('',#9957,#10502,#586,.T.);
#13640=EDGE_CURVE('',#10503,#9970,#587,.T.);
#13641=EDGE_CURVE('',#10504,#10503,#7076,.T.);
#13642=EDGE_CURVE('',#9967,#10504,#588,.T.);
#13643=EDGE_CURVE('',#10505,#9980,#589,.T.);
#13644=EDGE_CURVE('',#10506,#10505,#7077,.T.);
#13645=EDGE_CURVE('',#9977,#10506,#590,.T.);
#13646=EDGE_CURVE('',#10507,#9990,#591,.T.);
#13647=EDGE_CURVE('',#10508,#10507,#7078,.T.);
#13648=EDGE_CURVE('',#9987,#10508,#592,.T.);
#13649=EDGE_CURVE('',#10509,#10000,#593,.T.);
#13650=EDGE_CURVE('',#10510,#10509,#7079,.T.);
#13651=EDGE_CURVE('',#9997,#10510,#594,.T.);
#13652=EDGE_CURVE('',#10511,#10010,#595,.T.);
#13653=EDGE_CURVE('',#10512,#10511,#7080,.T.);
#13654=EDGE_CURVE('',#10007,#10512,#596,.T.);
#13655=EDGE_CURVE('',#10513,#10020,#597,.T.);
#13656=EDGE_CURVE('',#10514,#10513,#7081,.T.);
#13657=EDGE_CURVE('',#10017,#10514,#598,.T.);
#13658=EDGE_CURVE('',#10515,#10030,#599,.T.);
#13659=EDGE_CURVE('',#10516,#10515,#7082,.T.);
#13660=EDGE_CURVE('',#10027,#10516,#600,.T.);
#13661=EDGE_CURVE('',#10517,#10040,#601,.T.);
#13662=EDGE_CURVE('',#10518,#10517,#7083,.T.);
#13663=EDGE_CURVE('',#10037,#10518,#602,.T.);
#13664=EDGE_CURVE('',#10519,#10050,#603,.T.);
#13665=EDGE_CURVE('',#10520,#10519,#7084,.T.);
#13666=EDGE_CURVE('',#10047,#10520,#604,.T.);
#13667=EDGE_CURVE('',#10521,#10060,#605,.T.);
#13668=EDGE_CURVE('',#10522,#10521,#7085,.T.);
#13669=EDGE_CURVE('',#10057,#10522,#606,.T.);
#13670=EDGE_CURVE('',#10523,#10070,#607,.T.);
#13671=EDGE_CURVE('',#10524,#10523,#7086,.T.);
#13672=EDGE_CURVE('',#10067,#10524,#608,.T.);
#13673=EDGE_CURVE('',#10525,#10080,#609,.T.);
#13674=EDGE_CURVE('',#10526,#10525,#7087,.T.);
#13675=EDGE_CURVE('',#10077,#10526,#610,.T.);
#13676=EDGE_CURVE('',#10527,#10090,#611,.T.);
#13677=EDGE_CURVE('',#10528,#10527,#7088,.T.);
#13678=EDGE_CURVE('',#10087,#10528,#612,.T.);
#13679=EDGE_CURVE('',#10529,#10100,#613,.T.);
#13680=EDGE_CURVE('',#10530,#10529,#7089,.T.);
#13681=EDGE_CURVE('',#10097,#10530,#614,.T.);
#13682=EDGE_CURVE('',#10531,#10110,#615,.T.);
#13683=EDGE_CURVE('',#10532,#10531,#7090,.T.);
#13684=EDGE_CURVE('',#10107,#10532,#616,.T.);
#13685=EDGE_CURVE('',#10533,#10120,#617,.T.);
#13686=EDGE_CURVE('',#10534,#10533,#7091,.T.);
#13687=EDGE_CURVE('',#10117,#10534,#618,.T.);
#13688=EDGE_CURVE('',#10535,#10130,#619,.T.);
#13689=EDGE_CURVE('',#10536,#10535,#7092,.T.);
#13690=EDGE_CURVE('',#10127,#10536,#620,.T.);
#13691=EDGE_CURVE('',#10537,#10140,#621,.T.);
#13692=EDGE_CURVE('',#10538,#10537,#7093,.T.);
#13693=EDGE_CURVE('',#10137,#10538,#622,.T.);
#13694=EDGE_CURVE('',#10539,#10150,#623,.T.);
#13695=EDGE_CURVE('',#10540,#10539,#7094,.T.);
#13696=EDGE_CURVE('',#10147,#10540,#624,.T.);
#13697=EDGE_CURVE('',#10541,#10160,#625,.T.);
#13698=EDGE_CURVE('',#10542,#10541,#7095,.T.);
#13699=EDGE_CURVE('',#10157,#10542,#626,.T.);
#13700=EDGE_CURVE('',#10543,#10170,#627,.T.);
#13701=EDGE_CURVE('',#10544,#10543,#7096,.T.);
#13702=EDGE_CURVE('',#10167,#10544,#628,.T.);
#13703=EDGE_CURVE('',#10545,#10180,#629,.T.);
#13704=EDGE_CURVE('',#10546,#10545,#7097,.T.);
#13705=EDGE_CURVE('',#10177,#10546,#630,.T.);
#13706=EDGE_CURVE('',#10547,#10190,#631,.T.);
#13707=EDGE_CURVE('',#10548,#10547,#7098,.T.);
#13708=EDGE_CURVE('',#10187,#10548,#632,.T.);
#13709=EDGE_CURVE('',#10549,#10200,#633,.T.);
#13710=EDGE_CURVE('',#10550,#10549,#7099,.T.);
#13711=EDGE_CURVE('',#10197,#10550,#634,.T.);
#13712=EDGE_CURVE('',#10551,#10210,#635,.T.);
#13713=EDGE_CURVE('',#10552,#10551,#7100,.T.);
#13714=EDGE_CURVE('',#10207,#10552,#636,.T.);
#13715=EDGE_CURVE('',#10553,#10220,#637,.T.);
#13716=EDGE_CURVE('',#10554,#10553,#7101,.T.);
#13717=EDGE_CURVE('',#10217,#10554,#638,.T.);
#13718=EDGE_CURVE('',#10555,#10230,#639,.T.);
#13719=EDGE_CURVE('',#10556,#10555,#7102,.T.);
#13720=EDGE_CURVE('',#10227,#10556,#640,.T.);
#13721=EDGE_CURVE('',#10557,#10240,#641,.T.);
#13722=EDGE_CURVE('',#10558,#10557,#7103,.T.);
#13723=EDGE_CURVE('',#10237,#10558,#642,.T.);
#13724=EDGE_CURVE('',#10559,#10250,#643,.T.);
#13725=EDGE_CURVE('',#10560,#10559,#7104,.T.);
#13726=EDGE_CURVE('',#10247,#10560,#644,.T.);
#13727=EDGE_CURVE('',#10561,#10260,#645,.T.);
#13728=EDGE_CURVE('',#10562,#10561,#7105,.T.);
#13729=EDGE_CURVE('',#10257,#10562,#646,.T.);
#13730=EDGE_CURVE('',#10563,#10270,#647,.T.);
#13731=EDGE_CURVE('',#10564,#10563,#7106,.T.);
#13732=EDGE_CURVE('',#10267,#10564,#648,.T.);
#13733=EDGE_CURVE('',#10565,#10280,#649,.T.);
#13734=EDGE_CURVE('',#10566,#10565,#7107,.T.);
#13735=EDGE_CURVE('',#10277,#10566,#650,.T.);
#13736=EDGE_CURVE('',#10567,#10290,#651,.T.);
#13737=EDGE_CURVE('',#10568,#10567,#7108,.T.);
#13738=EDGE_CURVE('',#10287,#10568,#652,.T.);
#13739=EDGE_CURVE('',#10569,#10300,#653,.T.);
#13740=EDGE_CURVE('',#10570,#10569,#7109,.T.);
#13741=EDGE_CURVE('',#10297,#10570,#654,.T.);
#13742=EDGE_CURVE('',#10571,#10310,#655,.T.);
#13743=EDGE_CURVE('',#10572,#10571,#7110,.T.);
#13744=EDGE_CURVE('',#10307,#10572,#656,.T.);
#13745=EDGE_CURVE('',#10573,#10320,#657,.T.);
#13746=EDGE_CURVE('',#10574,#10573,#7111,.T.);
#13747=EDGE_CURVE('',#10317,#10574,#658,.T.);
#13748=EDGE_CURVE('',#10575,#10330,#659,.T.);
#13749=EDGE_CURVE('',#10576,#10575,#7112,.T.);
#13750=EDGE_CURVE('',#10327,#10576,#660,.T.);
#13751=EDGE_CURVE('',#10577,#10340,#661,.T.);
#13752=EDGE_CURVE('',#10578,#10577,#7113,.T.);
#13753=EDGE_CURVE('',#10337,#10578,#662,.T.);
#13754=EDGE_CURVE('',#10579,#10350,#663,.T.);
#13755=EDGE_CURVE('',#10580,#10579,#7114,.T.);
#13756=EDGE_CURVE('',#10347,#10580,#664,.T.);
#13757=EDGE_CURVE('',#10581,#10360,#665,.T.);
#13758=EDGE_CURVE('',#10582,#10581,#7115,.T.);
#13759=EDGE_CURVE('',#10357,#10582,#666,.T.);
#13760=EDGE_CURVE('',#10583,#10370,#667,.T.);
#13761=EDGE_CURVE('',#10584,#10583,#7116,.T.);
#13762=EDGE_CURVE('',#10367,#10584,#668,.T.);
#13763=EDGE_CURVE('',#10585,#10380,#669,.T.);
#13764=EDGE_CURVE('',#10586,#10585,#7117,.T.);
#13765=EDGE_CURVE('',#10377,#10586,#670,.T.);
#13766=EDGE_CURVE('',#10587,#10390,#671,.T.);
#13767=EDGE_CURVE('',#10588,#10587,#7118,.T.);
#13768=EDGE_CURVE('',#10387,#10588,#672,.T.);
#13769=EDGE_CURVE('',#10589,#10400,#673,.T.);
#13770=EDGE_CURVE('',#10590,#10589,#7119,.T.);
#13771=EDGE_CURVE('',#10397,#10590,#674,.T.);
#13772=EDGE_CURVE('',#10591,#10410,#675,.T.);
#13773=EDGE_CURVE('',#10592,#10591,#7120,.T.);
#13774=EDGE_CURVE('',#10407,#10592,#676,.T.);
#13775=EDGE_CURVE('',#10593,#10420,#677,.T.);
#13776=EDGE_CURVE('',#10594,#10593,#7121,.T.);
#13777=EDGE_CURVE('',#10417,#10594,#678,.T.);
#13778=EDGE_CURVE('',#10595,#10430,#679,.T.);
#13779=EDGE_CURVE('',#10596,#10595,#7122,.T.);
#13780=EDGE_CURVE('',#10427,#10596,#680,.T.);
#13781=EDGE_CURVE('',#10597,#10440,#681,.T.);
#13782=EDGE_CURVE('',#10598,#10597,#7123,.T.);
#13783=EDGE_CURVE('',#10437,#10598,#682,.T.);
#13784=EDGE_CURVE('',#10599,#10450,#683,.T.);
#13785=EDGE_CURVE('',#10600,#10599,#7124,.T.);
#13786=EDGE_CURVE('',#10447,#10600,#684,.T.);
#13787=EDGE_CURVE('',#10601,#10460,#685,.T.);
#13788=EDGE_CURVE('',#10602,#10601,#7125,.T.);
#13789=EDGE_CURVE('',#10457,#10602,#686,.T.);
#13790=EDGE_CURVE('',#10455,#10603,#4769,.T.);
#13791=EDGE_CURVE('',#10603,#10604,#7126,.T.);
#13792=EDGE_CURVE('',#10456,#10604,#4770,.T.);
#13793=EDGE_CURVE('',#10445,#10602,#4771,.T.);
#13794=EDGE_CURVE('',#10446,#10601,#4772,.T.);
#13795=EDGE_CURVE('',#10435,#10600,#4773,.T.);
#13796=EDGE_CURVE('',#10436,#10599,#4774,.T.);
#13797=EDGE_CURVE('',#10425,#10598,#4775,.T.);
#13798=EDGE_CURVE('',#10426,#10597,#4776,.T.);
#13799=EDGE_CURVE('',#10415,#10596,#4777,.T.);
#13800=EDGE_CURVE('',#10416,#10595,#4778,.T.);
#13801=EDGE_CURVE('',#10405,#10594,#4779,.T.);
#13802=EDGE_CURVE('',#10406,#10593,#4780,.T.);
#13803=EDGE_CURVE('',#10395,#10592,#4781,.T.);
#13804=EDGE_CURVE('',#10396,#10591,#4782,.T.);
#13805=EDGE_CURVE('',#10385,#10590,#4783,.T.);
#13806=EDGE_CURVE('',#10386,#10589,#4784,.T.);
#13807=EDGE_CURVE('',#10375,#10588,#4785,.T.);
#13808=EDGE_CURVE('',#10376,#10587,#4786,.T.);
#13809=EDGE_CURVE('',#10365,#10586,#4787,.T.);
#13810=EDGE_CURVE('',#10366,#10585,#4788,.T.);
#13811=EDGE_CURVE('',#10355,#10584,#4789,.T.);
#13812=EDGE_CURVE('',#10356,#10583,#4790,.T.);
#13813=EDGE_CURVE('',#10345,#10582,#4791,.T.);
#13814=EDGE_CURVE('',#10346,#10581,#4792,.T.);
#13815=EDGE_CURVE('',#10335,#10580,#4793,.T.);
#13816=EDGE_CURVE('',#10336,#10579,#4794,.T.);
#13817=EDGE_CURVE('',#10325,#10578,#4795,.T.);
#13818=EDGE_CURVE('',#10326,#10577,#4796,.T.);
#13819=EDGE_CURVE('',#10315,#10576,#4797,.T.);
#13820=EDGE_CURVE('',#10316,#10575,#4798,.T.);
#13821=EDGE_CURVE('',#10305,#10574,#4799,.T.);
#13822=EDGE_CURVE('',#10306,#10573,#4800,.T.);
#13823=EDGE_CURVE('',#10295,#10572,#4801,.T.);
#13824=EDGE_CURVE('',#10296,#10571,#4802,.T.);
#13825=EDGE_CURVE('',#10285,#10570,#4803,.T.);
#13826=EDGE_CURVE('',#10286,#10569,#4804,.T.);
#13827=EDGE_CURVE('',#10275,#10568,#4805,.T.);
#13828=EDGE_CURVE('',#10276,#10567,#4806,.T.);
#13829=EDGE_CURVE('',#10265,#10566,#4807,.T.);
#13830=EDGE_CURVE('',#10266,#10565,#4808,.T.);
#13831=EDGE_CURVE('',#10255,#10564,#4809,.T.);
#13832=EDGE_CURVE('',#10256,#10563,#4810,.T.);
#13833=EDGE_CURVE('',#10245,#10562,#4811,.T.);
#13834=EDGE_CURVE('',#10246,#10561,#4812,.T.);
#13835=EDGE_CURVE('',#10235,#10560,#4813,.T.);
#13836=EDGE_CURVE('',#10236,#10559,#4814,.T.);
#13837=EDGE_CURVE('',#10225,#10558,#4815,.T.);
#13838=EDGE_CURVE('',#10226,#10557,#4816,.T.);
#13839=EDGE_CURVE('',#10215,#10556,#4817,.T.);
#13840=EDGE_CURVE('',#10216,#10555,#4818,.T.);
#13841=EDGE_CURVE('',#10205,#10554,#4819,.T.);
#13842=EDGE_CURVE('',#10206,#10553,#4820,.T.);
#13843=EDGE_CURVE('',#10195,#10552,#4821,.T.);
#13844=EDGE_CURVE('',#10196,#10551,#4822,.T.);
#13845=EDGE_CURVE('',#10185,#10550,#4823,.T.);
#13846=EDGE_CURVE('',#10186,#10549,#4824,.T.);
#13847=EDGE_CURVE('',#10175,#10548,#4825,.T.);
#13848=EDGE_CURVE('',#10176,#10547,#4826,.T.);
#13849=EDGE_CURVE('',#10165,#10546,#4827,.T.);
#13850=EDGE_CURVE('',#10166,#10545,#4828,.T.);
#13851=EDGE_CURVE('',#10155,#10544,#4829,.T.);
#13852=EDGE_CURVE('',#10156,#10543,#4830,.T.);
#13853=EDGE_CURVE('',#10145,#10542,#4831,.T.);
#13854=EDGE_CURVE('',#10146,#10541,#4832,.T.);
#13855=EDGE_CURVE('',#10135,#10540,#4833,.T.);
#13856=EDGE_CURVE('',#10136,#10539,#4834,.T.);
#13857=EDGE_CURVE('',#10125,#10538,#4835,.T.);
#13858=EDGE_CURVE('',#10126,#10537,#4836,.T.);
#13859=EDGE_CURVE('',#10115,#10536,#4837,.T.);
#13860=EDGE_CURVE('',#10116,#10535,#4838,.T.);
#13861=EDGE_CURVE('',#10105,#10534,#4839,.T.);
#13862=EDGE_CURVE('',#10106,#10533,#4840,.T.);
#13863=EDGE_CURVE('',#10095,#10532,#4841,.T.);
#13864=EDGE_CURVE('',#10096,#10531,#4842,.T.);
#13865=EDGE_CURVE('',#10085,#10530,#4843,.T.);
#13866=EDGE_CURVE('',#10086,#10529,#4844,.T.);
#13867=EDGE_CURVE('',#10075,#10528,#4845,.T.);
#13868=EDGE_CURVE('',#10076,#10527,#4846,.T.);
#13869=EDGE_CURVE('',#10065,#10526,#4847,.T.);
#13870=EDGE_CURVE('',#10066,#10525,#4848,.T.);
#13871=EDGE_CURVE('',#10055,#10524,#4849,.T.);
#13872=EDGE_CURVE('',#10056,#10523,#4850,.T.);
#13873=EDGE_CURVE('',#10045,#10522,#4851,.T.);
#13874=EDGE_CURVE('',#10046,#10521,#4852,.T.);
#13875=EDGE_CURVE('',#10035,#10520,#4853,.T.);
#13876=EDGE_CURVE('',#10036,#10519,#4854,.T.);
#13877=EDGE_CURVE('',#10025,#10518,#4855,.T.);
#13878=EDGE_CURVE('',#10026,#10517,#4856,.T.);
#13879=EDGE_CURVE('',#10015,#10516,#4857,.T.);
#13880=EDGE_CURVE('',#10016,#10515,#4858,.T.);
#13881=EDGE_CURVE('',#10005,#10514,#4859,.T.);
#13882=EDGE_CURVE('',#10006,#10513,#4860,.T.);
#13883=EDGE_CURVE('',#9995,#10512,#4861,.T.);
#13884=EDGE_CURVE('',#9996,#10511,#4862,.T.);
#13885=EDGE_CURVE('',#9985,#10510,#4863,.T.);
#13886=EDGE_CURVE('',#9986,#10509,#4864,.T.);
#13887=EDGE_CURVE('',#9975,#10508,#4865,.T.);
#13888=EDGE_CURVE('',#9976,#10507,#4866,.T.);
#13889=EDGE_CURVE('',#9965,#10506,#4867,.T.);
#13890=EDGE_CURVE('',#9966,#10505,#4868,.T.);
#13891=EDGE_CURVE('',#9955,#10504,#4869,.T.);
#13892=EDGE_CURVE('',#9956,#10503,#4870,.T.);
#13893=EDGE_CURVE('',#9945,#10502,#4871,.T.);
#13894=EDGE_CURVE('',#9946,#10501,#4872,.T.);
#13895=EDGE_CURVE('',#9935,#10500,#4873,.T.);
#13896=EDGE_CURVE('',#9936,#10499,#4874,.T.);
#13897=EDGE_CURVE('',#9925,#10498,#4875,.T.);
#13898=EDGE_CURVE('',#9926,#10497,#4876,.T.);
#13899=EDGE_CURVE('',#9915,#10496,#4877,.T.);
#13900=EDGE_CURVE('',#9916,#10495,#4878,.T.);
#13901=EDGE_CURVE('',#9905,#10494,#4879,.T.);
#13902=EDGE_CURVE('',#9906,#10493,#4880,.T.);
#13903=EDGE_CURVE('',#9895,#10492,#4881,.T.);
#13904=EDGE_CURVE('',#9896,#10491,#4882,.T.);
#13905=EDGE_CURVE('',#9885,#10490,#4883,.T.);
#13906=EDGE_CURVE('',#9886,#10489,#4884,.T.);
#13907=EDGE_CURVE('',#9875,#10488,#4885,.T.);
#13908=EDGE_CURVE('',#9876,#10487,#4886,.T.);
#13909=EDGE_CURVE('',#9865,#10486,#4887,.T.);
#13910=EDGE_CURVE('',#9866,#10485,#4888,.T.);
#13911=EDGE_CURVE('',#9855,#10484,#4889,.T.);
#13912=EDGE_CURVE('',#9856,#10483,#4890,.T.);
#13913=EDGE_CURVE('',#9845,#10482,#4891,.T.);
#13914=EDGE_CURVE('',#9846,#10481,#4892,.T.);
#13915=EDGE_CURVE('',#9835,#10480,#4893,.T.);
#13916=EDGE_CURVE('',#9836,#10479,#4894,.T.);
#13917=EDGE_CURVE('',#9825,#10478,#4895,.T.);
#13918=EDGE_CURVE('',#9826,#10477,#4896,.T.);
#13919=EDGE_CURVE('',#9815,#10476,#4897,.T.);
#13920=EDGE_CURVE('',#9816,#10475,#4898,.T.);
#13921=EDGE_CURVE('',#9805,#10474,#4899,.T.);
#13922=EDGE_CURVE('',#9806,#10473,#4900,.T.);
#13923=EDGE_CURVE('',#9795,#10472,#4901,.T.);
#13924=EDGE_CURVE('',#9796,#10471,#4902,.T.);
#13925=EDGE_CURVE('',#9785,#10470,#4903,.T.);
#13926=EDGE_CURVE('',#9786,#10469,#4904,.T.);
#13927=EDGE_CURVE('',#9775,#10468,#4905,.T.);
#13928=EDGE_CURVE('',#9776,#10467,#4906,.T.);
#13929=EDGE_CURVE('',#9765,#10466,#4907,.T.);
#13930=EDGE_CURVE('',#9766,#10465,#4908,.T.);
#13931=EDGE_CURVE('',#10605,#10461,#4909,.T.);
#13932=EDGE_CURVE('',#10605,#10606,#7127,.T.);
#13933=EDGE_CURVE('',#10606,#10462,#4910,.T.);
#13934=EDGE_CURVE('',#10607,#10608,#6571,.T.);
#13935=EDGE_CURVE('',#10608,#10609,#6572,.T.);
#13936=EDGE_CURVE('',#10609,#10610,#6573,.T.);
#13937=EDGE_CURVE('',#10610,#10607,#6574,.T.);
#13938=EDGE_CURVE('',#10606,#10608,#687,.T.);
#13939=EDGE_CURVE('',#10609,#10605,#688,.T.);
#13940=EDGE_CURVE('',#10611,#10612,#6575,.T.);
#13941=EDGE_CURVE('',#10612,#10613,#6576,.T.);
#13942=EDGE_CURVE('',#10613,#10614,#6577,.T.);
#13943=EDGE_CURVE('',#10614,#10611,#6578,.T.);
#13944=EDGE_CURVE('',#10613,#10610,#4911,.T.);
#13945=EDGE_CURVE('',#10607,#10612,#4912,.T.);
#13946=EDGE_CURVE('',#10604,#10614,#689,.T.);
#13947=EDGE_CURVE('',#10611,#10603,#690,.T.);
#13948=EDGE_CURVE('',#10615,#10615,#4913,.T.);
#13949=EDGE_CURVE('',#9756,#10463,#4914,.T.);
#13950=EDGE_CURVE('',#9755,#10464,#4915,.T.);
#13951=EDGE_CURVE('',#10615,#9743,#7128,.T.);
#13952=EDGE_CURVE('',#9744,#10616,#7129,.T.);
#13953=EDGE_CURVE('',#10616,#10616,#4916,.T.);
#17502=ORIENTED_EDGE('',*,*,#12636,.F.);
#17503=ORIENTED_EDGE('',*,*,#12637,.T.);
#17504=ORIENTED_EDGE('',*,*,#12638,.T.);
#17505=ORIENTED_EDGE('',*,*,#12637,.F.);
#17506=ORIENTED_EDGE('',*,*,#12639,.F.);
#17507=ORIENTED_EDGE('',*,*,#12638,.F.);
#17508=ORIENTED_EDGE('',*,*,#12640,.F.);
#17509=ORIENTED_EDGE('',*,*,#12641,.F.);
#17510=ORIENTED_EDGE('',*,*,#12642,.T.);
#17511=ORIENTED_EDGE('',*,*,#12643,.T.);
#17512=ORIENTED_EDGE('',*,*,#12642,.F.);
#17513=ORIENTED_EDGE('',*,*,#12643,.F.);
#17514=ORIENTED_EDGE('',*,*,#12644,.F.);
#17515=ORIENTED_EDGE('',*,*,#12645,.F.);
#17516=ORIENTED_EDGE('',*,*,#12646,.T.);
#17517=ORIENTED_EDGE('',*,*,#12647,.T.);
#17518=ORIENTED_EDGE('',*,*,#12646,.F.);
#17519=ORIENTED_EDGE('',*,*,#12648,.F.);
#17520=ORIENTED_EDGE('',*,*,#12647,.F.);
#17521=ORIENTED_EDGE('',*,*,#12649,.F.);
#17522=ORIENTED_EDGE('',*,*,#12650,.F.);
#17523=ORIENTED_EDGE('',*,*,#12651,.T.);
#17524=ORIENTED_EDGE('',*,*,#12652,.T.);
#17525=ORIENTED_EDGE('',*,*,#12651,.F.);
#17526=ORIENTED_EDGE('',*,*,#12653,.F.);
#17527=ORIENTED_EDGE('',*,*,#12652,.F.);
#17528=ORIENTED_EDGE('',*,*,#12654,.T.);
#17529=ORIENTED_EDGE('',*,*,#12655,.T.);
#17530=ORIENTED_EDGE('',*,*,#12656,.T.);
#17531=ORIENTED_EDGE('',*,*,#12657,.T.);
#17532=ORIENTED_EDGE('',*,*,#12655,.F.);
#17533=ORIENTED_EDGE('',*,*,#12658,.F.);
#17534=ORIENTED_EDGE('',*,*,#12659,.F.);
#17535=ORIENTED_EDGE('',*,*,#12660,.F.);
#17536=ORIENTED_EDGE('',*,*,#12661,.T.);
#17537=ORIENTED_EDGE('',*,*,#12662,.T.);
#17538=ORIENTED_EDGE('',*,*,#12663,.T.);
#17539=ORIENTED_EDGE('',*,*,#12664,.T.);
#17540=ORIENTED_EDGE('',*,*,#12657,.F.);
#17541=ORIENTED_EDGE('',*,*,#12665,.F.);
#17542=ORIENTED_EDGE('',*,*,#12662,.F.);
#17543=ORIENTED_EDGE('',*,*,#12666,.F.);
#17544=ORIENTED_EDGE('',*,*,#12667,.T.);
#17545=ORIENTED_EDGE('',*,*,#12668,.T.);
#17546=ORIENTED_EDGE('',*,*,#12669,.T.);
#17547=ORIENTED_EDGE('',*,*,#12670,.T.);
#17548=ORIENTED_EDGE('',*,*,#12668,.F.);
#17549=ORIENTED_EDGE('',*,*,#12671,.F.);
#17550=ORIENTED_EDGE('',*,*,#12672,.F.);
#17551=ORIENTED_EDGE('',*,*,#12673,.F.);
#17552=ORIENTED_EDGE('',*,*,#12674,.T.);
#17553=ORIENTED_EDGE('',*,*,#12675,.T.);
#17554=ORIENTED_EDGE('',*,*,#12676,.T.);
#17555=ORIENTED_EDGE('',*,*,#12677,.T.);
#17556=ORIENTED_EDGE('',*,*,#12670,.F.);
#17557=ORIENTED_EDGE('',*,*,#12678,.F.);
#17558=ORIENTED_EDGE('',*,*,#12675,.F.);
#17559=ORIENTED_EDGE('',*,*,#12679,.F.);
#17560=ORIENTED_EDGE('',*,*,#12680,.T.);
#17561=ORIENTED_EDGE('',*,*,#12681,.T.);
#17562=ORIENTED_EDGE('',*,*,#12682,.T.);
#17563=ORIENTED_EDGE('',*,*,#12683,.T.);
#17564=ORIENTED_EDGE('',*,*,#12681,.F.);
#17565=ORIENTED_EDGE('',*,*,#12684,.F.);
#17566=ORIENTED_EDGE('',*,*,#12685,.F.);
#17567=ORIENTED_EDGE('',*,*,#12686,.F.);
#17568=ORIENTED_EDGE('',*,*,#12687,.T.);
#17569=ORIENTED_EDGE('',*,*,#12688,.T.);
#17570=ORIENTED_EDGE('',*,*,#12689,.T.);
#17571=ORIENTED_EDGE('',*,*,#12690,.T.);
#17572=ORIENTED_EDGE('',*,*,#12683,.F.);
#17573=ORIENTED_EDGE('',*,*,#12691,.F.);
#17574=ORIENTED_EDGE('',*,*,#12688,.F.);
#17575=ORIENTED_EDGE('',*,*,#12692,.F.);
#17576=ORIENTED_EDGE('',*,*,#12693,.T.);
#17577=ORIENTED_EDGE('',*,*,#12694,.T.);
#17578=ORIENTED_EDGE('',*,*,#12695,.T.);
#17579=ORIENTED_EDGE('',*,*,#12696,.T.);
#17580=ORIENTED_EDGE('',*,*,#12694,.F.);
#17581=ORIENTED_EDGE('',*,*,#12697,.F.);
#17582=ORIENTED_EDGE('',*,*,#12698,.F.);
#17583=ORIENTED_EDGE('',*,*,#12699,.F.);
#17584=ORIENTED_EDGE('',*,*,#12700,.T.);
#17585=ORIENTED_EDGE('',*,*,#12701,.T.);
#17586=ORIENTED_EDGE('',*,*,#12702,.T.);
#17587=ORIENTED_EDGE('',*,*,#12703,.T.);
#17588=ORIENTED_EDGE('',*,*,#12696,.F.);
#17589=ORIENTED_EDGE('',*,*,#12704,.F.);
#17590=ORIENTED_EDGE('',*,*,#12701,.F.);
#17591=ORIENTED_EDGE('',*,*,#12705,.F.);
#17592=ORIENTED_EDGE('',*,*,#12706,.T.);
#17593=ORIENTED_EDGE('',*,*,#12707,.T.);
#17594=ORIENTED_EDGE('',*,*,#12708,.T.);
#17595=ORIENTED_EDGE('',*,*,#12709,.T.);
#17596=ORIENTED_EDGE('',*,*,#12707,.F.);
#17597=ORIENTED_EDGE('',*,*,#12710,.F.);
#17598=ORIENTED_EDGE('',*,*,#12711,.F.);
#17599=ORIENTED_EDGE('',*,*,#12712,.F.);
#17600=ORIENTED_EDGE('',*,*,#12713,.T.);
#17601=ORIENTED_EDGE('',*,*,#12714,.T.);
#17602=ORIENTED_EDGE('',*,*,#12715,.T.);
#17603=ORIENTED_EDGE('',*,*,#12716,.T.);
#17604=ORIENTED_EDGE('',*,*,#12709,.F.);
#17605=ORIENTED_EDGE('',*,*,#12717,.F.);
#17606=ORIENTED_EDGE('',*,*,#12714,.F.);
#17607=ORIENTED_EDGE('',*,*,#12718,.F.);
#17608=ORIENTED_EDGE('',*,*,#12719,.T.);
#17609=ORIENTED_EDGE('',*,*,#12720,.T.);
#17610=ORIENTED_EDGE('',*,*,#12721,.T.);
#17611=ORIENTED_EDGE('',*,*,#12722,.T.);
#17612=ORIENTED_EDGE('',*,*,#12720,.F.);
#17613=ORIENTED_EDGE('',*,*,#12723,.F.);
#17614=ORIENTED_EDGE('',*,*,#12724,.F.);
#17615=ORIENTED_EDGE('',*,*,#12725,.F.);
#17616=ORIENTED_EDGE('',*,*,#12726,.T.);
#17617=ORIENTED_EDGE('',*,*,#12727,.T.);
#17618=ORIENTED_EDGE('',*,*,#12728,.T.);
#17619=ORIENTED_EDGE('',*,*,#12729,.T.);
#17620=ORIENTED_EDGE('',*,*,#12722,.F.);
#17621=ORIENTED_EDGE('',*,*,#12730,.F.);
#17622=ORIENTED_EDGE('',*,*,#12727,.F.);
#17623=ORIENTED_EDGE('',*,*,#12731,.F.);
#17624=ORIENTED_EDGE('',*,*,#12732,.T.);
#17625=ORIENTED_EDGE('',*,*,#12733,.T.);
#17626=ORIENTED_EDGE('',*,*,#12734,.T.);
#17627=ORIENTED_EDGE('',*,*,#12735,.T.);
#17628=ORIENTED_EDGE('',*,*,#12733,.F.);
#17629=ORIENTED_EDGE('',*,*,#12736,.F.);
#17630=ORIENTED_EDGE('',*,*,#12737,.F.);
#17631=ORIENTED_EDGE('',*,*,#12738,.F.);
#17632=ORIENTED_EDGE('',*,*,#12739,.T.);
#17633=ORIENTED_EDGE('',*,*,#12740,.T.);
#17634=ORIENTED_EDGE('',*,*,#12741,.T.);
#17635=ORIENTED_EDGE('',*,*,#12742,.T.);
#17636=ORIENTED_EDGE('',*,*,#12735,.F.);
#17637=ORIENTED_EDGE('',*,*,#12743,.F.);
#17638=ORIENTED_EDGE('',*,*,#12740,.F.);
#17639=ORIENTED_EDGE('',*,*,#12744,.F.);
#17640=ORIENTED_EDGE('',*,*,#12745,.T.);
#17641=ORIENTED_EDGE('',*,*,#12746,.T.);
#17642=ORIENTED_EDGE('',*,*,#12747,.T.);
#17643=ORIENTED_EDGE('',*,*,#12748,.T.);
#17644=ORIENTED_EDGE('',*,*,#12746,.F.);
#17645=ORIENTED_EDGE('',*,*,#12749,.F.);
#17646=ORIENTED_EDGE('',*,*,#12750,.F.);
#17647=ORIENTED_EDGE('',*,*,#12751,.F.);
#17648=ORIENTED_EDGE('',*,*,#12752,.T.);
#17649=ORIENTED_EDGE('',*,*,#12753,.T.);
#17650=ORIENTED_EDGE('',*,*,#12754,.T.);
#17651=ORIENTED_EDGE('',*,*,#12755,.T.);
#17652=ORIENTED_EDGE('',*,*,#12748,.F.);
#17653=ORIENTED_EDGE('',*,*,#12756,.F.);
#17654=ORIENTED_EDGE('',*,*,#12753,.F.);
#17655=ORIENTED_EDGE('',*,*,#12757,.F.);
#17656=ORIENTED_EDGE('',*,*,#12758,.T.);
#17657=ORIENTED_EDGE('',*,*,#12759,.T.);
#17658=ORIENTED_EDGE('',*,*,#12760,.T.);
#17659=ORIENTED_EDGE('',*,*,#12761,.T.);
#17660=ORIENTED_EDGE('',*,*,#12759,.F.);
#17661=ORIENTED_EDGE('',*,*,#12762,.F.);
#17662=ORIENTED_EDGE('',*,*,#12763,.F.);
#17663=ORIENTED_EDGE('',*,*,#12764,.F.);
#17664=ORIENTED_EDGE('',*,*,#12765,.T.);
#17665=ORIENTED_EDGE('',*,*,#12766,.T.);
#17666=ORIENTED_EDGE('',*,*,#12767,.T.);
#17667=ORIENTED_EDGE('',*,*,#12768,.T.);
#17668=ORIENTED_EDGE('',*,*,#12761,.F.);
#17669=ORIENTED_EDGE('',*,*,#12769,.F.);
#17670=ORIENTED_EDGE('',*,*,#12766,.F.);
#17671=ORIENTED_EDGE('',*,*,#12770,.F.);
#17672=ORIENTED_EDGE('',*,*,#12771,.T.);
#17673=ORIENTED_EDGE('',*,*,#12772,.T.);
#17674=ORIENTED_EDGE('',*,*,#12773,.T.);
#17675=ORIENTED_EDGE('',*,*,#12774,.T.);
#17676=ORIENTED_EDGE('',*,*,#12772,.F.);
#17677=ORIENTED_EDGE('',*,*,#12775,.F.);
#17678=ORIENTED_EDGE('',*,*,#12776,.F.);
#17679=ORIENTED_EDGE('',*,*,#12777,.F.);
#17680=ORIENTED_EDGE('',*,*,#12778,.T.);
#17681=ORIENTED_EDGE('',*,*,#12779,.T.);
#17682=ORIENTED_EDGE('',*,*,#12780,.T.);
#17683=ORIENTED_EDGE('',*,*,#12781,.T.);
#17684=ORIENTED_EDGE('',*,*,#12774,.F.);
#17685=ORIENTED_EDGE('',*,*,#12782,.F.);
#17686=ORIENTED_EDGE('',*,*,#12779,.F.);
#17687=ORIENTED_EDGE('',*,*,#12783,.F.);
#17688=ORIENTED_EDGE('',*,*,#12784,.T.);
#17689=ORIENTED_EDGE('',*,*,#12785,.T.);
#17690=ORIENTED_EDGE('',*,*,#12786,.T.);
#17691=ORIENTED_EDGE('',*,*,#12787,.T.);
#17692=ORIENTED_EDGE('',*,*,#12785,.F.);
#17693=ORIENTED_EDGE('',*,*,#12788,.F.);
#17694=ORIENTED_EDGE('',*,*,#12789,.F.);
#17695=ORIENTED_EDGE('',*,*,#12790,.F.);
#17696=ORIENTED_EDGE('',*,*,#12791,.T.);
#17697=ORIENTED_EDGE('',*,*,#12792,.T.);
#17698=ORIENTED_EDGE('',*,*,#12793,.T.);
#17699=ORIENTED_EDGE('',*,*,#12794,.T.);
#17700=ORIENTED_EDGE('',*,*,#12787,.F.);
#17701=ORIENTED_EDGE('',*,*,#12795,.F.);
#17702=ORIENTED_EDGE('',*,*,#12792,.F.);
#17703=ORIENTED_EDGE('',*,*,#12796,.F.);
#17704=ORIENTED_EDGE('',*,*,#12797,.T.);
#17705=ORIENTED_EDGE('',*,*,#12798,.T.);
#17706=ORIENTED_EDGE('',*,*,#12799,.T.);
#17707=ORIENTED_EDGE('',*,*,#12800,.T.);
#17708=ORIENTED_EDGE('',*,*,#12798,.F.);
#17709=ORIENTED_EDGE('',*,*,#12801,.F.);
#17710=ORIENTED_EDGE('',*,*,#12802,.F.);
#17711=ORIENTED_EDGE('',*,*,#12803,.F.);
#17712=ORIENTED_EDGE('',*,*,#12804,.T.);
#17713=ORIENTED_EDGE('',*,*,#12805,.T.);
#17714=ORIENTED_EDGE('',*,*,#12806,.T.);
#17715=ORIENTED_EDGE('',*,*,#12807,.T.);
#17716=ORIENTED_EDGE('',*,*,#12800,.F.);
#17717=ORIENTED_EDGE('',*,*,#12808,.F.);
#17718=ORIENTED_EDGE('',*,*,#12805,.F.);
#17719=ORIENTED_EDGE('',*,*,#12809,.F.);
#17720=ORIENTED_EDGE('',*,*,#12810,.T.);
#17721=ORIENTED_EDGE('',*,*,#12811,.T.);
#17722=ORIENTED_EDGE('',*,*,#12812,.T.);
#17723=ORIENTED_EDGE('',*,*,#12813,.T.);
#17724=ORIENTED_EDGE('',*,*,#12811,.F.);
#17725=ORIENTED_EDGE('',*,*,#12814,.F.);
#17726=ORIENTED_EDGE('',*,*,#12815,.F.);
#17727=ORIENTED_EDGE('',*,*,#12816,.F.);
#17728=ORIENTED_EDGE('',*,*,#12817,.T.);
#17729=ORIENTED_EDGE('',*,*,#12818,.T.);
#17730=ORIENTED_EDGE('',*,*,#12819,.T.);
#17731=ORIENTED_EDGE('',*,*,#12820,.T.);
#17732=ORIENTED_EDGE('',*,*,#12813,.F.);
#17733=ORIENTED_EDGE('',*,*,#12821,.F.);
#17734=ORIENTED_EDGE('',*,*,#12818,.F.);
#17735=ORIENTED_EDGE('',*,*,#12822,.F.);
#17736=ORIENTED_EDGE('',*,*,#12823,.T.);
#17737=ORIENTED_EDGE('',*,*,#12824,.T.);
#17738=ORIENTED_EDGE('',*,*,#12825,.T.);
#17739=ORIENTED_EDGE('',*,*,#12826,.T.);
#17740=ORIENTED_EDGE('',*,*,#12824,.F.);
#17741=ORIENTED_EDGE('',*,*,#12827,.F.);
#17742=ORIENTED_EDGE('',*,*,#12828,.F.);
#17743=ORIENTED_EDGE('',*,*,#12829,.F.);
#17744=ORIENTED_EDGE('',*,*,#12830,.T.);
#17745=ORIENTED_EDGE('',*,*,#12831,.T.);
#17746=ORIENTED_EDGE('',*,*,#12832,.T.);
#17747=ORIENTED_EDGE('',*,*,#12833,.T.);
#17748=ORIENTED_EDGE('',*,*,#12826,.F.);
#17749=ORIENTED_EDGE('',*,*,#12834,.F.);
#17750=ORIENTED_EDGE('',*,*,#12831,.F.);
#17751=ORIENTED_EDGE('',*,*,#12835,.F.);
#17752=ORIENTED_EDGE('',*,*,#12836,.T.);
#17753=ORIENTED_EDGE('',*,*,#12837,.T.);
#17754=ORIENTED_EDGE('',*,*,#12838,.T.);
#17755=ORIENTED_EDGE('',*,*,#12839,.T.);
#17756=ORIENTED_EDGE('',*,*,#12837,.F.);
#17757=ORIENTED_EDGE('',*,*,#12840,.F.);
#17758=ORIENTED_EDGE('',*,*,#12841,.F.);
#17759=ORIENTED_EDGE('',*,*,#12842,.F.);
#17760=ORIENTED_EDGE('',*,*,#12843,.T.);
#17761=ORIENTED_EDGE('',*,*,#12844,.T.);
#17762=ORIENTED_EDGE('',*,*,#12845,.T.);
#17763=ORIENTED_EDGE('',*,*,#12846,.T.);
#17764=ORIENTED_EDGE('',*,*,#12839,.F.);
#17765=ORIENTED_EDGE('',*,*,#12847,.F.);
#17766=ORIENTED_EDGE('',*,*,#12844,.F.);
#17767=ORIENTED_EDGE('',*,*,#12848,.F.);
#17768=ORIENTED_EDGE('',*,*,#12849,.T.);
#17769=ORIENTED_EDGE('',*,*,#12850,.T.);
#17770=ORIENTED_EDGE('',*,*,#12851,.T.);
#17771=ORIENTED_EDGE('',*,*,#12852,.T.);
#17772=ORIENTED_EDGE('',*,*,#12850,.F.);
#17773=ORIENTED_EDGE('',*,*,#12853,.F.);
#17774=ORIENTED_EDGE('',*,*,#12854,.F.);
#17775=ORIENTED_EDGE('',*,*,#12855,.F.);
#17776=ORIENTED_EDGE('',*,*,#12856,.T.);
#17777=ORIENTED_EDGE('',*,*,#12857,.T.);
#17778=ORIENTED_EDGE('',*,*,#12858,.T.);
#17779=ORIENTED_EDGE('',*,*,#12859,.T.);
#17780=ORIENTED_EDGE('',*,*,#12852,.F.);
#17781=ORIENTED_EDGE('',*,*,#12860,.F.);
#17782=ORIENTED_EDGE('',*,*,#12857,.F.);
#17783=ORIENTED_EDGE('',*,*,#12861,.F.);
#17784=ORIENTED_EDGE('',*,*,#12862,.T.);
#17785=ORIENTED_EDGE('',*,*,#12863,.T.);
#17786=ORIENTED_EDGE('',*,*,#12864,.T.);
#17787=ORIENTED_EDGE('',*,*,#12865,.T.);
#17788=ORIENTED_EDGE('',*,*,#12863,.F.);
#17789=ORIENTED_EDGE('',*,*,#12866,.F.);
#17790=ORIENTED_EDGE('',*,*,#12867,.F.);
#17791=ORIENTED_EDGE('',*,*,#12868,.F.);
#17792=ORIENTED_EDGE('',*,*,#12869,.T.);
#17793=ORIENTED_EDGE('',*,*,#12870,.T.);
#17794=ORIENTED_EDGE('',*,*,#12871,.T.);
#17795=ORIENTED_EDGE('',*,*,#12872,.T.);
#17796=ORIENTED_EDGE('',*,*,#12865,.F.);
#17797=ORIENTED_EDGE('',*,*,#12873,.F.);
#17798=ORIENTED_EDGE('',*,*,#12870,.F.);
#17799=ORIENTED_EDGE('',*,*,#12874,.F.);
#17800=ORIENTED_EDGE('',*,*,#12875,.T.);
#17801=ORIENTED_EDGE('',*,*,#12876,.T.);
#17802=ORIENTED_EDGE('',*,*,#12877,.T.);
#17803=ORIENTED_EDGE('',*,*,#12878,.T.);
#17804=ORIENTED_EDGE('',*,*,#12876,.F.);
#17805=ORIENTED_EDGE('',*,*,#12879,.F.);
#17806=ORIENTED_EDGE('',*,*,#12880,.F.);
#17807=ORIENTED_EDGE('',*,*,#12881,.F.);
#17808=ORIENTED_EDGE('',*,*,#12882,.T.);
#17809=ORIENTED_EDGE('',*,*,#12883,.T.);
#17810=ORIENTED_EDGE('',*,*,#12884,.T.);
#17811=ORIENTED_EDGE('',*,*,#12885,.T.);
#17812=ORIENTED_EDGE('',*,*,#12878,.F.);
#17813=ORIENTED_EDGE('',*,*,#12886,.F.);
#17814=ORIENTED_EDGE('',*,*,#12883,.F.);
#17815=ORIENTED_EDGE('',*,*,#12887,.F.);
#17816=ORIENTED_EDGE('',*,*,#12888,.T.);
#17817=ORIENTED_EDGE('',*,*,#12889,.T.);
#17818=ORIENTED_EDGE('',*,*,#12890,.T.);
#17819=ORIENTED_EDGE('',*,*,#12891,.T.);
#17820=ORIENTED_EDGE('',*,*,#12889,.F.);
#17821=ORIENTED_EDGE('',*,*,#12892,.F.);
#17822=ORIENTED_EDGE('',*,*,#12893,.F.);
#17823=ORIENTED_EDGE('',*,*,#12894,.F.);
#17824=ORIENTED_EDGE('',*,*,#12895,.T.);
#17825=ORIENTED_EDGE('',*,*,#12896,.T.);
#17826=ORIENTED_EDGE('',*,*,#12897,.T.);
#17827=ORIENTED_EDGE('',*,*,#12898,.T.);
#17828=ORIENTED_EDGE('',*,*,#12891,.F.);
#17829=ORIENTED_EDGE('',*,*,#12899,.F.);
#17830=ORIENTED_EDGE('',*,*,#12896,.F.);
#17831=ORIENTED_EDGE('',*,*,#12900,.F.);
#17832=ORIENTED_EDGE('',*,*,#12901,.T.);
#17833=ORIENTED_EDGE('',*,*,#12902,.T.);
#17834=ORIENTED_EDGE('',*,*,#12903,.T.);
#17835=ORIENTED_EDGE('',*,*,#12904,.T.);
#17836=ORIENTED_EDGE('',*,*,#12902,.F.);
#17837=ORIENTED_EDGE('',*,*,#12905,.F.);
#17838=ORIENTED_EDGE('',*,*,#12906,.F.);
#17839=ORIENTED_EDGE('',*,*,#12907,.F.);
#17840=ORIENTED_EDGE('',*,*,#12908,.T.);
#17841=ORIENTED_EDGE('',*,*,#12909,.T.);
#17842=ORIENTED_EDGE('',*,*,#12910,.T.);
#17843=ORIENTED_EDGE('',*,*,#12911,.T.);
#17844=ORIENTED_EDGE('',*,*,#12904,.F.);
#17845=ORIENTED_EDGE('',*,*,#12912,.F.);
#17846=ORIENTED_EDGE('',*,*,#12909,.F.);
#17847=ORIENTED_EDGE('',*,*,#12913,.F.);
#17848=ORIENTED_EDGE('',*,*,#12914,.T.);
#17849=ORIENTED_EDGE('',*,*,#12915,.T.);
#17850=ORIENTED_EDGE('',*,*,#12916,.T.);
#17851=ORIENTED_EDGE('',*,*,#12917,.T.);
#17852=ORIENTED_EDGE('',*,*,#12915,.F.);
#17853=ORIENTED_EDGE('',*,*,#12918,.F.);
#17854=ORIENTED_EDGE('',*,*,#12919,.F.);
#17855=ORIENTED_EDGE('',*,*,#12920,.F.);
#17856=ORIENTED_EDGE('',*,*,#12921,.T.);
#17857=ORIENTED_EDGE('',*,*,#12922,.T.);
#17858=ORIENTED_EDGE('',*,*,#12923,.T.);
#17859=ORIENTED_EDGE('',*,*,#12924,.T.);
#17860=ORIENTED_EDGE('',*,*,#12917,.F.);
#17861=ORIENTED_EDGE('',*,*,#12925,.F.);
#17862=ORIENTED_EDGE('',*,*,#12922,.F.);
#17863=ORIENTED_EDGE('',*,*,#12926,.F.);
#17864=ORIENTED_EDGE('',*,*,#12927,.T.);
#17865=ORIENTED_EDGE('',*,*,#12928,.T.);
#17866=ORIENTED_EDGE('',*,*,#12929,.T.);
#17867=ORIENTED_EDGE('',*,*,#12930,.T.);
#17868=ORIENTED_EDGE('',*,*,#12928,.F.);
#17869=ORIENTED_EDGE('',*,*,#12931,.F.);
#17870=ORIENTED_EDGE('',*,*,#12932,.F.);
#17871=ORIENTED_EDGE('',*,*,#12933,.F.);
#17872=ORIENTED_EDGE('',*,*,#12934,.T.);
#17873=ORIENTED_EDGE('',*,*,#12935,.T.);
#17874=ORIENTED_EDGE('',*,*,#12936,.T.);
#17875=ORIENTED_EDGE('',*,*,#12937,.T.);
#17876=ORIENTED_EDGE('',*,*,#12930,.F.);
#17877=ORIENTED_EDGE('',*,*,#12938,.F.);
#17878=ORIENTED_EDGE('',*,*,#12935,.F.);
#17879=ORIENTED_EDGE('',*,*,#12939,.F.);
#17880=ORIENTED_EDGE('',*,*,#12940,.T.);
#17881=ORIENTED_EDGE('',*,*,#12941,.T.);
#17882=ORIENTED_EDGE('',*,*,#12942,.T.);
#17883=ORIENTED_EDGE('',*,*,#12943,.T.);
#17884=ORIENTED_EDGE('',*,*,#12941,.F.);
#17885=ORIENTED_EDGE('',*,*,#12944,.F.);
#17886=ORIENTED_EDGE('',*,*,#12945,.F.);
#17887=ORIENTED_EDGE('',*,*,#12946,.F.);
#17888=ORIENTED_EDGE('',*,*,#12947,.T.);
#17889=ORIENTED_EDGE('',*,*,#12948,.T.);
#17890=ORIENTED_EDGE('',*,*,#12949,.T.);
#17891=ORIENTED_EDGE('',*,*,#12950,.T.);
#17892=ORIENTED_EDGE('',*,*,#12943,.F.);
#17893=ORIENTED_EDGE('',*,*,#12951,.F.);
#17894=ORIENTED_EDGE('',*,*,#12948,.F.);
#17895=ORIENTED_EDGE('',*,*,#12952,.F.);
#17896=ORIENTED_EDGE('',*,*,#12953,.T.);
#17897=ORIENTED_EDGE('',*,*,#12954,.T.);
#17898=ORIENTED_EDGE('',*,*,#12955,.T.);
#17899=ORIENTED_EDGE('',*,*,#12956,.T.);
#17900=ORIENTED_EDGE('',*,*,#12954,.F.);
#17901=ORIENTED_EDGE('',*,*,#12957,.F.);
#17902=ORIENTED_EDGE('',*,*,#12958,.F.);
#17903=ORIENTED_EDGE('',*,*,#12959,.F.);
#17904=ORIENTED_EDGE('',*,*,#12960,.T.);
#17905=ORIENTED_EDGE('',*,*,#12961,.T.);
#17906=ORIENTED_EDGE('',*,*,#12962,.T.);
#17907=ORIENTED_EDGE('',*,*,#12963,.T.);
#17908=ORIENTED_EDGE('',*,*,#12956,.F.);
#17909=ORIENTED_EDGE('',*,*,#12964,.F.);
#17910=ORIENTED_EDGE('',*,*,#12961,.F.);
#17911=ORIENTED_EDGE('',*,*,#12965,.F.);
#17912=ORIENTED_EDGE('',*,*,#12966,.T.);
#17913=ORIENTED_EDGE('',*,*,#12967,.T.);
#17914=ORIENTED_EDGE('',*,*,#12968,.T.);
#17915=ORIENTED_EDGE('',*,*,#12969,.T.);
#17916=ORIENTED_EDGE('',*,*,#12967,.F.);
#17917=ORIENTED_EDGE('',*,*,#12970,.F.);
#17918=ORIENTED_EDGE('',*,*,#12971,.F.);
#17919=ORIENTED_EDGE('',*,*,#12972,.F.);
#17920=ORIENTED_EDGE('',*,*,#12973,.T.);
#17921=ORIENTED_EDGE('',*,*,#12974,.T.);
#17922=ORIENTED_EDGE('',*,*,#12975,.T.);
#17923=ORIENTED_EDGE('',*,*,#12976,.T.);
#17924=ORIENTED_EDGE('',*,*,#12969,.F.);
#17925=ORIENTED_EDGE('',*,*,#12977,.F.);
#17926=ORIENTED_EDGE('',*,*,#12974,.F.);
#17927=ORIENTED_EDGE('',*,*,#12978,.F.);
#17928=ORIENTED_EDGE('',*,*,#12979,.T.);
#17929=ORIENTED_EDGE('',*,*,#12980,.T.);
#17930=ORIENTED_EDGE('',*,*,#12981,.T.);
#17931=ORIENTED_EDGE('',*,*,#12982,.T.);
#17932=ORIENTED_EDGE('',*,*,#12980,.F.);
#17933=ORIENTED_EDGE('',*,*,#12983,.F.);
#17934=ORIENTED_EDGE('',*,*,#12984,.F.);
#17935=ORIENTED_EDGE('',*,*,#12985,.F.);
#17936=ORIENTED_EDGE('',*,*,#12986,.T.);
#17937=ORIENTED_EDGE('',*,*,#12987,.T.);
#17938=ORIENTED_EDGE('',*,*,#12988,.T.);
#17939=ORIENTED_EDGE('',*,*,#12989,.T.);
#17940=ORIENTED_EDGE('',*,*,#12982,.F.);
#17941=ORIENTED_EDGE('',*,*,#12990,.F.);
#17942=ORIENTED_EDGE('',*,*,#12987,.F.);
#17943=ORIENTED_EDGE('',*,*,#12991,.F.);
#17944=ORIENTED_EDGE('',*,*,#12992,.T.);
#17945=ORIENTED_EDGE('',*,*,#12993,.T.);
#17946=ORIENTED_EDGE('',*,*,#12994,.T.);
#17947=ORIENTED_EDGE('',*,*,#12995,.T.);
#17948=ORIENTED_EDGE('',*,*,#12993,.F.);
#17949=ORIENTED_EDGE('',*,*,#12996,.F.);
#17950=ORIENTED_EDGE('',*,*,#12997,.F.);
#17951=ORIENTED_EDGE('',*,*,#12998,.F.);
#17952=ORIENTED_EDGE('',*,*,#12999,.T.);
#17953=ORIENTED_EDGE('',*,*,#13000,.T.);
#17954=ORIENTED_EDGE('',*,*,#13001,.T.);
#17955=ORIENTED_EDGE('',*,*,#13002,.T.);
#17956=ORIENTED_EDGE('',*,*,#12995,.F.);
#17957=ORIENTED_EDGE('',*,*,#13003,.F.);
#17958=ORIENTED_EDGE('',*,*,#13000,.F.);
#17959=ORIENTED_EDGE('',*,*,#13004,.F.);
#17960=ORIENTED_EDGE('',*,*,#13005,.T.);
#17961=ORIENTED_EDGE('',*,*,#13006,.T.);
#17962=ORIENTED_EDGE('',*,*,#13007,.T.);
#17963=ORIENTED_EDGE('',*,*,#13008,.T.);
#17964=ORIENTED_EDGE('',*,*,#13006,.F.);
#17965=ORIENTED_EDGE('',*,*,#13009,.F.);
#17966=ORIENTED_EDGE('',*,*,#13010,.F.);
#17967=ORIENTED_EDGE('',*,*,#13011,.F.);
#17968=ORIENTED_EDGE('',*,*,#13012,.T.);
#17969=ORIENTED_EDGE('',*,*,#13013,.T.);
#17970=ORIENTED_EDGE('',*,*,#13014,.T.);
#17971=ORIENTED_EDGE('',*,*,#13015,.T.);
#17972=ORIENTED_EDGE('',*,*,#13008,.F.);
#17973=ORIENTED_EDGE('',*,*,#13016,.F.);
#17974=ORIENTED_EDGE('',*,*,#13013,.F.);
#17975=ORIENTED_EDGE('',*,*,#13017,.F.);
#17976=ORIENTED_EDGE('',*,*,#13018,.T.);
#17977=ORIENTED_EDGE('',*,*,#13019,.T.);
#17978=ORIENTED_EDGE('',*,*,#13020,.T.);
#17979=ORIENTED_EDGE('',*,*,#13021,.T.);
#17980=ORIENTED_EDGE('',*,*,#13019,.F.);
#17981=ORIENTED_EDGE('',*,*,#13022,.F.);
#17982=ORIENTED_EDGE('',*,*,#13023,.F.);
#17983=ORIENTED_EDGE('',*,*,#13024,.F.);
#17984=ORIENTED_EDGE('',*,*,#13025,.T.);
#17985=ORIENTED_EDGE('',*,*,#13026,.T.);
#17986=ORIENTED_EDGE('',*,*,#13027,.T.);
#17987=ORIENTED_EDGE('',*,*,#13028,.T.);
#17988=ORIENTED_EDGE('',*,*,#13021,.F.);
#17989=ORIENTED_EDGE('',*,*,#13029,.F.);
#17990=ORIENTED_EDGE('',*,*,#13026,.F.);
#17991=ORIENTED_EDGE('',*,*,#13030,.F.);
#17992=ORIENTED_EDGE('',*,*,#13031,.T.);
#17993=ORIENTED_EDGE('',*,*,#13032,.T.);
#17994=ORIENTED_EDGE('',*,*,#13033,.T.);
#17995=ORIENTED_EDGE('',*,*,#13034,.T.);
#17996=ORIENTED_EDGE('',*,*,#13032,.F.);
#17997=ORIENTED_EDGE('',*,*,#13035,.F.);
#17998=ORIENTED_EDGE('',*,*,#13036,.F.);
#17999=ORIENTED_EDGE('',*,*,#13037,.F.);
#18000=ORIENTED_EDGE('',*,*,#13038,.T.);
#18001=ORIENTED_EDGE('',*,*,#13039,.T.);
#18002=ORIENTED_EDGE('',*,*,#13040,.T.);
#18003=ORIENTED_EDGE('',*,*,#13041,.T.);
#18004=ORIENTED_EDGE('',*,*,#13034,.F.);
#18005=ORIENTED_EDGE('',*,*,#13042,.F.);
#18006=ORIENTED_EDGE('',*,*,#13039,.F.);
#18007=ORIENTED_EDGE('',*,*,#13043,.F.);
#18008=ORIENTED_EDGE('',*,*,#13044,.T.);
#18009=ORIENTED_EDGE('',*,*,#13045,.T.);
#18010=ORIENTED_EDGE('',*,*,#13046,.T.);
#18011=ORIENTED_EDGE('',*,*,#13047,.T.);
#18012=ORIENTED_EDGE('',*,*,#13045,.F.);
#18013=ORIENTED_EDGE('',*,*,#13048,.F.);
#18014=ORIENTED_EDGE('',*,*,#13049,.F.);
#18015=ORIENTED_EDGE('',*,*,#13050,.F.);
#18016=ORIENTED_EDGE('',*,*,#13051,.T.);
#18017=ORIENTED_EDGE('',*,*,#13052,.T.);
#18018=ORIENTED_EDGE('',*,*,#13053,.T.);
#18019=ORIENTED_EDGE('',*,*,#13054,.T.);
#18020=ORIENTED_EDGE('',*,*,#13047,.F.);
#18021=ORIENTED_EDGE('',*,*,#13055,.F.);
#18022=ORIENTED_EDGE('',*,*,#13052,.F.);
#18023=ORIENTED_EDGE('',*,*,#13056,.F.);
#18024=ORIENTED_EDGE('',*,*,#13057,.T.);
#18025=ORIENTED_EDGE('',*,*,#13058,.T.);
#18026=ORIENTED_EDGE('',*,*,#13059,.T.);
#18027=ORIENTED_EDGE('',*,*,#13060,.T.);
#18028=ORIENTED_EDGE('',*,*,#13058,.F.);
#18029=ORIENTED_EDGE('',*,*,#13061,.F.);
#18030=ORIENTED_EDGE('',*,*,#13062,.F.);
#18031=ORIENTED_EDGE('',*,*,#13063,.F.);
#18032=ORIENTED_EDGE('',*,*,#13064,.T.);
#18033=ORIENTED_EDGE('',*,*,#13065,.T.);
#18034=ORIENTED_EDGE('',*,*,#13066,.T.);
#18035=ORIENTED_EDGE('',*,*,#13067,.T.);
#18036=ORIENTED_EDGE('',*,*,#13060,.F.);
#18037=ORIENTED_EDGE('',*,*,#13068,.F.);
#18038=ORIENTED_EDGE('',*,*,#13065,.F.);
#18039=ORIENTED_EDGE('',*,*,#13069,.F.);
#18040=ORIENTED_EDGE('',*,*,#13070,.T.);
#18041=ORIENTED_EDGE('',*,*,#13071,.T.);
#18042=ORIENTED_EDGE('',*,*,#13072,.T.);
#18043=ORIENTED_EDGE('',*,*,#13073,.T.);
#18044=ORIENTED_EDGE('',*,*,#13071,.F.);
#18045=ORIENTED_EDGE('',*,*,#13074,.F.);
#18046=ORIENTED_EDGE('',*,*,#13075,.F.);
#18047=ORIENTED_EDGE('',*,*,#13076,.F.);
#18048=ORIENTED_EDGE('',*,*,#13077,.T.);
#18049=ORIENTED_EDGE('',*,*,#13078,.T.);
#18050=ORIENTED_EDGE('',*,*,#13079,.T.);
#18051=ORIENTED_EDGE('',*,*,#13080,.T.);
#18052=ORIENTED_EDGE('',*,*,#13073,.F.);
#18053=ORIENTED_EDGE('',*,*,#13081,.F.);
#18054=ORIENTED_EDGE('',*,*,#13078,.F.);
#18055=ORIENTED_EDGE('',*,*,#13082,.F.);
#18056=ORIENTED_EDGE('',*,*,#13083,.T.);
#18057=ORIENTED_EDGE('',*,*,#13084,.T.);
#18058=ORIENTED_EDGE('',*,*,#13085,.T.);
#18059=ORIENTED_EDGE('',*,*,#13086,.T.);
#18060=ORIENTED_EDGE('',*,*,#13084,.F.);
#18061=ORIENTED_EDGE('',*,*,#13087,.F.);
#18062=ORIENTED_EDGE('',*,*,#13088,.F.);
#18063=ORIENTED_EDGE('',*,*,#13089,.F.);
#18064=ORIENTED_EDGE('',*,*,#13090,.T.);
#18065=ORIENTED_EDGE('',*,*,#13091,.T.);
#18066=ORIENTED_EDGE('',*,*,#13092,.T.);
#18067=ORIENTED_EDGE('',*,*,#13093,.T.);
#18068=ORIENTED_EDGE('',*,*,#13086,.F.);
#18069=ORIENTED_EDGE('',*,*,#13094,.F.);
#18070=ORIENTED_EDGE('',*,*,#13091,.F.);
#18071=ORIENTED_EDGE('',*,*,#13095,.F.);
#18072=ORIENTED_EDGE('',*,*,#13096,.T.);
#18073=ORIENTED_EDGE('',*,*,#13097,.T.);
#18074=ORIENTED_EDGE('',*,*,#13098,.T.);
#18075=ORIENTED_EDGE('',*,*,#13099,.T.);
#18076=ORIENTED_EDGE('',*,*,#13097,.F.);
#18077=ORIENTED_EDGE('',*,*,#13100,.F.);
#18078=ORIENTED_EDGE('',*,*,#13101,.F.);
#18079=ORIENTED_EDGE('',*,*,#13102,.F.);
#18080=ORIENTED_EDGE('',*,*,#13103,.T.);
#18081=ORIENTED_EDGE('',*,*,#13104,.T.);
#18082=ORIENTED_EDGE('',*,*,#13105,.T.);
#18083=ORIENTED_EDGE('',*,*,#13106,.T.);
#18084=ORIENTED_EDGE('',*,*,#13099,.F.);
#18085=ORIENTED_EDGE('',*,*,#13107,.F.);
#18086=ORIENTED_EDGE('',*,*,#13104,.F.);
#18087=ORIENTED_EDGE('',*,*,#13108,.F.);
#18088=ORIENTED_EDGE('',*,*,#13109,.T.);
#18089=ORIENTED_EDGE('',*,*,#13110,.T.);
#18090=ORIENTED_EDGE('',*,*,#13111,.T.);
#18091=ORIENTED_EDGE('',*,*,#13112,.T.);
#18092=ORIENTED_EDGE('',*,*,#13110,.F.);
#18093=ORIENTED_EDGE('',*,*,#13113,.F.);
#18094=ORIENTED_EDGE('',*,*,#13114,.F.);
#18095=ORIENTED_EDGE('',*,*,#13115,.F.);
#18096=ORIENTED_EDGE('',*,*,#13116,.T.);
#18097=ORIENTED_EDGE('',*,*,#13117,.T.);
#18098=ORIENTED_EDGE('',*,*,#13118,.T.);
#18099=ORIENTED_EDGE('',*,*,#13119,.T.);
#18100=ORIENTED_EDGE('',*,*,#13112,.F.);
#18101=ORIENTED_EDGE('',*,*,#13120,.F.);
#18102=ORIENTED_EDGE('',*,*,#13117,.F.);
#18103=ORIENTED_EDGE('',*,*,#13121,.F.);
#18104=ORIENTED_EDGE('',*,*,#13122,.T.);
#18105=ORIENTED_EDGE('',*,*,#13123,.T.);
#18106=ORIENTED_EDGE('',*,*,#13124,.T.);
#18107=ORIENTED_EDGE('',*,*,#13125,.T.);
#18108=ORIENTED_EDGE('',*,*,#13123,.F.);
#18109=ORIENTED_EDGE('',*,*,#13126,.F.);
#18110=ORIENTED_EDGE('',*,*,#13127,.F.);
#18111=ORIENTED_EDGE('',*,*,#13128,.F.);
#18112=ORIENTED_EDGE('',*,*,#13129,.T.);
#18113=ORIENTED_EDGE('',*,*,#13130,.T.);
#18114=ORIENTED_EDGE('',*,*,#13131,.T.);
#18115=ORIENTED_EDGE('',*,*,#13132,.T.);
#18116=ORIENTED_EDGE('',*,*,#13125,.F.);
#18117=ORIENTED_EDGE('',*,*,#13133,.F.);
#18118=ORIENTED_EDGE('',*,*,#13130,.F.);
#18119=ORIENTED_EDGE('',*,*,#13134,.F.);
#18120=ORIENTED_EDGE('',*,*,#13135,.T.);
#18121=ORIENTED_EDGE('',*,*,#13136,.T.);
#18122=ORIENTED_EDGE('',*,*,#13137,.T.);
#18123=ORIENTED_EDGE('',*,*,#13138,.T.);
#18124=ORIENTED_EDGE('',*,*,#13136,.F.);
#18125=ORIENTED_EDGE('',*,*,#13139,.F.);
#18126=ORIENTED_EDGE('',*,*,#13140,.F.);
#18127=ORIENTED_EDGE('',*,*,#13141,.F.);
#18128=ORIENTED_EDGE('',*,*,#13142,.T.);
#18129=ORIENTED_EDGE('',*,*,#13143,.T.);
#18130=ORIENTED_EDGE('',*,*,#13144,.T.);
#18131=ORIENTED_EDGE('',*,*,#13145,.T.);
#18132=ORIENTED_EDGE('',*,*,#13138,.F.);
#18133=ORIENTED_EDGE('',*,*,#13146,.F.);
#18134=ORIENTED_EDGE('',*,*,#13143,.F.);
#18135=ORIENTED_EDGE('',*,*,#13147,.F.);
#18136=ORIENTED_EDGE('',*,*,#13148,.T.);
#18137=ORIENTED_EDGE('',*,*,#13149,.T.);
#18138=ORIENTED_EDGE('',*,*,#13150,.T.);
#18139=ORIENTED_EDGE('',*,*,#13151,.T.);
#18140=ORIENTED_EDGE('',*,*,#13149,.F.);
#18141=ORIENTED_EDGE('',*,*,#13152,.F.);
#18142=ORIENTED_EDGE('',*,*,#13153,.F.);
#18143=ORIENTED_EDGE('',*,*,#13154,.F.);
#18144=ORIENTED_EDGE('',*,*,#13155,.T.);
#18145=ORIENTED_EDGE('',*,*,#13156,.T.);
#18146=ORIENTED_EDGE('',*,*,#13157,.T.);
#18147=ORIENTED_EDGE('',*,*,#13158,.T.);
#18148=ORIENTED_EDGE('',*,*,#13151,.F.);
#18149=ORIENTED_EDGE('',*,*,#13159,.F.);
#18150=ORIENTED_EDGE('',*,*,#13156,.F.);
#18151=ORIENTED_EDGE('',*,*,#13160,.F.);
#18152=ORIENTED_EDGE('',*,*,#13161,.T.);
#18153=ORIENTED_EDGE('',*,*,#13162,.T.);
#18154=ORIENTED_EDGE('',*,*,#13163,.T.);
#18155=ORIENTED_EDGE('',*,*,#13164,.T.);
#18156=ORIENTED_EDGE('',*,*,#13162,.F.);
#18157=ORIENTED_EDGE('',*,*,#13165,.F.);
#18158=ORIENTED_EDGE('',*,*,#13166,.F.);
#18159=ORIENTED_EDGE('',*,*,#13167,.F.);
#18160=ORIENTED_EDGE('',*,*,#13168,.T.);
#18161=ORIENTED_EDGE('',*,*,#13169,.T.);
#18162=ORIENTED_EDGE('',*,*,#13170,.T.);
#18163=ORIENTED_EDGE('',*,*,#13171,.T.);
#18164=ORIENTED_EDGE('',*,*,#13164,.F.);
#18165=ORIENTED_EDGE('',*,*,#13172,.F.);
#18166=ORIENTED_EDGE('',*,*,#13169,.F.);
#18167=ORIENTED_EDGE('',*,*,#13173,.F.);
#18168=ORIENTED_EDGE('',*,*,#13174,.T.);
#18169=ORIENTED_EDGE('',*,*,#13175,.T.);
#18170=ORIENTED_EDGE('',*,*,#13176,.T.);
#18171=ORIENTED_EDGE('',*,*,#13177,.T.);
#18172=ORIENTED_EDGE('',*,*,#13175,.F.);
#18173=ORIENTED_EDGE('',*,*,#13178,.F.);
#18174=ORIENTED_EDGE('',*,*,#13179,.F.);
#18175=ORIENTED_EDGE('',*,*,#13180,.F.);
#18176=ORIENTED_EDGE('',*,*,#13181,.T.);
#18177=ORIENTED_EDGE('',*,*,#13182,.T.);
#18178=ORIENTED_EDGE('',*,*,#13183,.T.);
#18179=ORIENTED_EDGE('',*,*,#13184,.T.);
#18180=ORIENTED_EDGE('',*,*,#13177,.F.);
#18181=ORIENTED_EDGE('',*,*,#13185,.F.);
#18182=ORIENTED_EDGE('',*,*,#13182,.F.);
#18183=ORIENTED_EDGE('',*,*,#13186,.F.);
#18184=ORIENTED_EDGE('',*,*,#13187,.T.);
#18185=ORIENTED_EDGE('',*,*,#13188,.T.);
#18186=ORIENTED_EDGE('',*,*,#13189,.T.);
#18187=ORIENTED_EDGE('',*,*,#13190,.T.);
#18188=ORIENTED_EDGE('',*,*,#13188,.F.);
#18189=ORIENTED_EDGE('',*,*,#13191,.F.);
#18190=ORIENTED_EDGE('',*,*,#13192,.F.);
#18191=ORIENTED_EDGE('',*,*,#13193,.F.);
#18192=ORIENTED_EDGE('',*,*,#13194,.T.);
#18193=ORIENTED_EDGE('',*,*,#13195,.T.);
#18194=ORIENTED_EDGE('',*,*,#13196,.T.);
#18195=ORIENTED_EDGE('',*,*,#13197,.T.);
#18196=ORIENTED_EDGE('',*,*,#13190,.F.);
#18197=ORIENTED_EDGE('',*,*,#13198,.F.);
#18198=ORIENTED_EDGE('',*,*,#13195,.F.);
#18199=ORIENTED_EDGE('',*,*,#13199,.F.);
#18200=ORIENTED_EDGE('',*,*,#13200,.T.);
#18201=ORIENTED_EDGE('',*,*,#13201,.T.);
#18202=ORIENTED_EDGE('',*,*,#13202,.T.);
#18203=ORIENTED_EDGE('',*,*,#13203,.T.);
#18204=ORIENTED_EDGE('',*,*,#13201,.F.);
#18205=ORIENTED_EDGE('',*,*,#13204,.F.);
#18206=ORIENTED_EDGE('',*,*,#13205,.F.);
#18207=ORIENTED_EDGE('',*,*,#13206,.F.);
#18208=ORIENTED_EDGE('',*,*,#13207,.T.);
#18209=ORIENTED_EDGE('',*,*,#13208,.T.);
#18210=ORIENTED_EDGE('',*,*,#13209,.T.);
#18211=ORIENTED_EDGE('',*,*,#13210,.T.);
#18212=ORIENTED_EDGE('',*,*,#13203,.F.);
#18213=ORIENTED_EDGE('',*,*,#13211,.F.);
#18214=ORIENTED_EDGE('',*,*,#13208,.F.);
#18215=ORIENTED_EDGE('',*,*,#13212,.F.);
#18216=ORIENTED_EDGE('',*,*,#13213,.T.);
#18217=ORIENTED_EDGE('',*,*,#13214,.T.);
#18218=ORIENTED_EDGE('',*,*,#13215,.T.);
#18219=ORIENTED_EDGE('',*,*,#13216,.T.);
#18220=ORIENTED_EDGE('',*,*,#13214,.F.);
#18221=ORIENTED_EDGE('',*,*,#13217,.F.);
#18222=ORIENTED_EDGE('',*,*,#13218,.F.);
#18223=ORIENTED_EDGE('',*,*,#13219,.F.);
#18224=ORIENTED_EDGE('',*,*,#13220,.T.);
#18225=ORIENTED_EDGE('',*,*,#13221,.T.);
#18226=ORIENTED_EDGE('',*,*,#13222,.T.);
#18227=ORIENTED_EDGE('',*,*,#13223,.T.);
#18228=ORIENTED_EDGE('',*,*,#13216,.F.);
#18229=ORIENTED_EDGE('',*,*,#13224,.F.);
#18230=ORIENTED_EDGE('',*,*,#13221,.F.);
#18231=ORIENTED_EDGE('',*,*,#13225,.F.);
#18232=ORIENTED_EDGE('',*,*,#13226,.T.);
#18233=ORIENTED_EDGE('',*,*,#13227,.T.);
#18234=ORIENTED_EDGE('',*,*,#13228,.T.);
#18235=ORIENTED_EDGE('',*,*,#13229,.T.);
#18236=ORIENTED_EDGE('',*,*,#13227,.F.);
#18237=ORIENTED_EDGE('',*,*,#13230,.F.);
#18238=ORIENTED_EDGE('',*,*,#13231,.F.);
#18239=ORIENTED_EDGE('',*,*,#13232,.F.);
#18240=ORIENTED_EDGE('',*,*,#13233,.T.);
#18241=ORIENTED_EDGE('',*,*,#13234,.T.);
#18242=ORIENTED_EDGE('',*,*,#13235,.T.);
#18243=ORIENTED_EDGE('',*,*,#13236,.T.);
#18244=ORIENTED_EDGE('',*,*,#13229,.F.);
#18245=ORIENTED_EDGE('',*,*,#13237,.F.);
#18246=ORIENTED_EDGE('',*,*,#13234,.F.);
#18247=ORIENTED_EDGE('',*,*,#13238,.F.);
#18248=ORIENTED_EDGE('',*,*,#13239,.T.);
#18249=ORIENTED_EDGE('',*,*,#13240,.T.);
#18250=ORIENTED_EDGE('',*,*,#13241,.T.);
#18251=ORIENTED_EDGE('',*,*,#13242,.T.);
#18252=ORIENTED_EDGE('',*,*,#13240,.F.);
#18253=ORIENTED_EDGE('',*,*,#13243,.F.);
#18254=ORIENTED_EDGE('',*,*,#13244,.F.);
#18255=ORIENTED_EDGE('',*,*,#13245,.F.);
#18256=ORIENTED_EDGE('',*,*,#13246,.T.);
#18257=ORIENTED_EDGE('',*,*,#13247,.T.);
#18258=ORIENTED_EDGE('',*,*,#13248,.T.);
#18259=ORIENTED_EDGE('',*,*,#13249,.T.);
#18260=ORIENTED_EDGE('',*,*,#13242,.F.);
#18261=ORIENTED_EDGE('',*,*,#13250,.F.);
#18262=ORIENTED_EDGE('',*,*,#13247,.F.);
#18263=ORIENTED_EDGE('',*,*,#13251,.F.);
#18264=ORIENTED_EDGE('',*,*,#13252,.T.);
#18265=ORIENTED_EDGE('',*,*,#13253,.T.);
#18266=ORIENTED_EDGE('',*,*,#13254,.T.);
#18267=ORIENTED_EDGE('',*,*,#13255,.T.);
#18268=ORIENTED_EDGE('',*,*,#13253,.F.);
#18269=ORIENTED_EDGE('',*,*,#13256,.F.);
#18270=ORIENTED_EDGE('',*,*,#13257,.F.);
#18271=ORIENTED_EDGE('',*,*,#13258,.F.);
#18272=ORIENTED_EDGE('',*,*,#13259,.T.);
#18273=ORIENTED_EDGE('',*,*,#13260,.T.);
#18274=ORIENTED_EDGE('',*,*,#13261,.T.);
#18275=ORIENTED_EDGE('',*,*,#13262,.T.);
#18276=ORIENTED_EDGE('',*,*,#13255,.F.);
#18277=ORIENTED_EDGE('',*,*,#13263,.F.);
#18278=ORIENTED_EDGE('',*,*,#13260,.F.);
#18279=ORIENTED_EDGE('',*,*,#13264,.F.);
#18280=ORIENTED_EDGE('',*,*,#13265,.T.);
#18281=ORIENTED_EDGE('',*,*,#13266,.T.);
#18282=ORIENTED_EDGE('',*,*,#13267,.T.);
#18283=ORIENTED_EDGE('',*,*,#13268,.T.);
#18284=ORIENTED_EDGE('',*,*,#13266,.F.);
#18285=ORIENTED_EDGE('',*,*,#13269,.F.);
#18286=ORIENTED_EDGE('',*,*,#13270,.F.);
#18287=ORIENTED_EDGE('',*,*,#13271,.F.);
#18288=ORIENTED_EDGE('',*,*,#13272,.T.);
#18289=ORIENTED_EDGE('',*,*,#13273,.T.);
#18290=ORIENTED_EDGE('',*,*,#13274,.T.);
#18291=ORIENTED_EDGE('',*,*,#13275,.T.);
#18292=ORIENTED_EDGE('',*,*,#13268,.F.);
#18293=ORIENTED_EDGE('',*,*,#13276,.F.);
#18294=ORIENTED_EDGE('',*,*,#13273,.F.);
#18295=ORIENTED_EDGE('',*,*,#13277,.F.);
#18296=ORIENTED_EDGE('',*,*,#13278,.T.);
#18297=ORIENTED_EDGE('',*,*,#13279,.T.);
#18298=ORIENTED_EDGE('',*,*,#13280,.T.);
#18299=ORIENTED_EDGE('',*,*,#13281,.T.);
#18300=ORIENTED_EDGE('',*,*,#13279,.F.);
#18301=ORIENTED_EDGE('',*,*,#13282,.F.);
#18302=ORIENTED_EDGE('',*,*,#13283,.F.);
#18303=ORIENTED_EDGE('',*,*,#13284,.F.);
#18304=ORIENTED_EDGE('',*,*,#13285,.T.);
#18305=ORIENTED_EDGE('',*,*,#13286,.T.);
#18306=ORIENTED_EDGE('',*,*,#13287,.T.);
#18307=ORIENTED_EDGE('',*,*,#13288,.T.);
#18308=ORIENTED_EDGE('',*,*,#13281,.F.);
#18309=ORIENTED_EDGE('',*,*,#13289,.F.);
#18310=ORIENTED_EDGE('',*,*,#13286,.F.);
#18311=ORIENTED_EDGE('',*,*,#13290,.F.);
#18312=ORIENTED_EDGE('',*,*,#13291,.T.);
#18313=ORIENTED_EDGE('',*,*,#13292,.T.);
#18314=ORIENTED_EDGE('',*,*,#13293,.T.);
#18315=ORIENTED_EDGE('',*,*,#13294,.T.);
#18316=ORIENTED_EDGE('',*,*,#13292,.F.);
#18317=ORIENTED_EDGE('',*,*,#13295,.F.);
#18318=ORIENTED_EDGE('',*,*,#13296,.F.);
#18319=ORIENTED_EDGE('',*,*,#13297,.F.);
#18320=ORIENTED_EDGE('',*,*,#13298,.T.);
#18321=ORIENTED_EDGE('',*,*,#13299,.T.);
#18322=ORIENTED_EDGE('',*,*,#13300,.T.);
#18323=ORIENTED_EDGE('',*,*,#13301,.T.);
#18324=ORIENTED_EDGE('',*,*,#13294,.F.);
#18325=ORIENTED_EDGE('',*,*,#13302,.F.);
#18326=ORIENTED_EDGE('',*,*,#13299,.F.);
#18327=ORIENTED_EDGE('',*,*,#13303,.F.);
#18328=ORIENTED_EDGE('',*,*,#13304,.T.);
#18329=ORIENTED_EDGE('',*,*,#13305,.T.);
#18330=ORIENTED_EDGE('',*,*,#13306,.T.);
#18331=ORIENTED_EDGE('',*,*,#13307,.T.);
#18332=ORIENTED_EDGE('',*,*,#13305,.F.);
#18333=ORIENTED_EDGE('',*,*,#13308,.F.);
#18334=ORIENTED_EDGE('',*,*,#13309,.F.);
#18335=ORIENTED_EDGE('',*,*,#13310,.F.);
#18336=ORIENTED_EDGE('',*,*,#13311,.T.);
#18337=ORIENTED_EDGE('',*,*,#13312,.T.);
#18338=ORIENTED_EDGE('',*,*,#13313,.T.);
#18339=ORIENTED_EDGE('',*,*,#13314,.T.);
#18340=ORIENTED_EDGE('',*,*,#13307,.F.);
#18341=ORIENTED_EDGE('',*,*,#13315,.F.);
#18342=ORIENTED_EDGE('',*,*,#13312,.F.);
#18343=ORIENTED_EDGE('',*,*,#13316,.F.);
#18344=ORIENTED_EDGE('',*,*,#13317,.T.);
#18345=ORIENTED_EDGE('',*,*,#13318,.T.);
#18346=ORIENTED_EDGE('',*,*,#13319,.T.);
#18347=ORIENTED_EDGE('',*,*,#13320,.T.);
#18348=ORIENTED_EDGE('',*,*,#13318,.F.);
#18349=ORIENTED_EDGE('',*,*,#13321,.F.);
#18350=ORIENTED_EDGE('',*,*,#13322,.F.);
#18351=ORIENTED_EDGE('',*,*,#13323,.F.);
#18352=ORIENTED_EDGE('',*,*,#13324,.T.);
#18353=ORIENTED_EDGE('',*,*,#13325,.T.);
#18354=ORIENTED_EDGE('',*,*,#13326,.T.);
#18355=ORIENTED_EDGE('',*,*,#13327,.T.);
#18356=ORIENTED_EDGE('',*,*,#13320,.F.);
#18357=ORIENTED_EDGE('',*,*,#13328,.F.);
#18358=ORIENTED_EDGE('',*,*,#13325,.F.);
#18359=ORIENTED_EDGE('',*,*,#13329,.F.);
#18360=ORIENTED_EDGE('',*,*,#13330,.T.);
#18361=ORIENTED_EDGE('',*,*,#13331,.T.);
#18362=ORIENTED_EDGE('',*,*,#13332,.T.);
#18363=ORIENTED_EDGE('',*,*,#13333,.T.);
#18364=ORIENTED_EDGE('',*,*,#13331,.F.);
#18365=ORIENTED_EDGE('',*,*,#13334,.F.);
#18366=ORIENTED_EDGE('',*,*,#13335,.F.);
#18367=ORIENTED_EDGE('',*,*,#13336,.F.);
#18368=ORIENTED_EDGE('',*,*,#13337,.T.);
#18369=ORIENTED_EDGE('',*,*,#13338,.T.);
#18370=ORIENTED_EDGE('',*,*,#13339,.T.);
#18371=ORIENTED_EDGE('',*,*,#13340,.T.);
#18372=ORIENTED_EDGE('',*,*,#13333,.F.);
#18373=ORIENTED_EDGE('',*,*,#13341,.F.);
#18374=ORIENTED_EDGE('',*,*,#13338,.F.);
#18375=ORIENTED_EDGE('',*,*,#13342,.F.);
#18376=ORIENTED_EDGE('',*,*,#13343,.T.);
#18377=ORIENTED_EDGE('',*,*,#13344,.T.);
#18378=ORIENTED_EDGE('',*,*,#13345,.T.);
#18379=ORIENTED_EDGE('',*,*,#13346,.T.);
#18380=ORIENTED_EDGE('',*,*,#13344,.F.);
#18381=ORIENTED_EDGE('',*,*,#13347,.F.);
#18382=ORIENTED_EDGE('',*,*,#13348,.F.);
#18383=ORIENTED_EDGE('',*,*,#13349,.F.);
#18384=ORIENTED_EDGE('',*,*,#13350,.T.);
#18385=ORIENTED_EDGE('',*,*,#13351,.T.);
#18386=ORIENTED_EDGE('',*,*,#13352,.T.);
#18387=ORIENTED_EDGE('',*,*,#13353,.T.);
#18388=ORIENTED_EDGE('',*,*,#13346,.F.);
#18389=ORIENTED_EDGE('',*,*,#13354,.F.);
#18390=ORIENTED_EDGE('',*,*,#13351,.F.);
#18391=ORIENTED_EDGE('',*,*,#13355,.F.);
#18392=ORIENTED_EDGE('',*,*,#13356,.T.);
#18393=ORIENTED_EDGE('',*,*,#13357,.T.);
#18394=ORIENTED_EDGE('',*,*,#13358,.T.);
#18395=ORIENTED_EDGE('',*,*,#13359,.T.);
#18396=ORIENTED_EDGE('',*,*,#13357,.F.);
#18397=ORIENTED_EDGE('',*,*,#13360,.F.);
#18398=ORIENTED_EDGE('',*,*,#13361,.F.);
#18399=ORIENTED_EDGE('',*,*,#13362,.F.);
#18400=ORIENTED_EDGE('',*,*,#13363,.T.);
#18401=ORIENTED_EDGE('',*,*,#13364,.T.);
#18402=ORIENTED_EDGE('',*,*,#13365,.T.);
#18403=ORIENTED_EDGE('',*,*,#13366,.T.);
#18404=ORIENTED_EDGE('',*,*,#13359,.F.);
#18405=ORIENTED_EDGE('',*,*,#13367,.F.);
#18406=ORIENTED_EDGE('',*,*,#13364,.F.);
#18407=ORIENTED_EDGE('',*,*,#13368,.F.);
#18408=ORIENTED_EDGE('',*,*,#13369,.T.);
#18409=ORIENTED_EDGE('',*,*,#13370,.T.);
#18410=ORIENTED_EDGE('',*,*,#13371,.T.);
#18411=ORIENTED_EDGE('',*,*,#13372,.T.);
#18412=ORIENTED_EDGE('',*,*,#13370,.F.);
#18413=ORIENTED_EDGE('',*,*,#13373,.F.);
#18414=ORIENTED_EDGE('',*,*,#13374,.F.);
#18415=ORIENTED_EDGE('',*,*,#13375,.F.);
#18416=ORIENTED_EDGE('',*,*,#13376,.T.);
#18417=ORIENTED_EDGE('',*,*,#13377,.T.);
#18418=ORIENTED_EDGE('',*,*,#13378,.T.);
#18419=ORIENTED_EDGE('',*,*,#13379,.T.);
#18420=ORIENTED_EDGE('',*,*,#13372,.F.);
#18421=ORIENTED_EDGE('',*,*,#13380,.F.);
#18422=ORIENTED_EDGE('',*,*,#13377,.F.);
#18423=ORIENTED_EDGE('',*,*,#13381,.F.);
#18424=ORIENTED_EDGE('',*,*,#13382,.T.);
#18425=ORIENTED_EDGE('',*,*,#13383,.T.);
#18426=ORIENTED_EDGE('',*,*,#13384,.T.);
#18427=ORIENTED_EDGE('',*,*,#13385,.T.);
#18428=ORIENTED_EDGE('',*,*,#13383,.F.);
#18429=ORIENTED_EDGE('',*,*,#13386,.F.);
#18430=ORIENTED_EDGE('',*,*,#13387,.F.);
#18431=ORIENTED_EDGE('',*,*,#13388,.F.);
#18432=ORIENTED_EDGE('',*,*,#13389,.T.);
#18433=ORIENTED_EDGE('',*,*,#13390,.T.);
#18434=ORIENTED_EDGE('',*,*,#13391,.T.);
#18435=ORIENTED_EDGE('',*,*,#13392,.T.);
#18436=ORIENTED_EDGE('',*,*,#13385,.F.);
#18437=ORIENTED_EDGE('',*,*,#13393,.F.);
#18438=ORIENTED_EDGE('',*,*,#13390,.F.);
#18439=ORIENTED_EDGE('',*,*,#13394,.F.);
#18440=ORIENTED_EDGE('',*,*,#13395,.T.);
#18441=ORIENTED_EDGE('',*,*,#13396,.T.);
#18442=ORIENTED_EDGE('',*,*,#13397,.T.);
#18443=ORIENTED_EDGE('',*,*,#13398,.T.);
#18444=ORIENTED_EDGE('',*,*,#13396,.F.);
#18445=ORIENTED_EDGE('',*,*,#13399,.F.);
#18446=ORIENTED_EDGE('',*,*,#13400,.F.);
#18447=ORIENTED_EDGE('',*,*,#13401,.F.);
#18448=ORIENTED_EDGE('',*,*,#13402,.T.);
#18449=ORIENTED_EDGE('',*,*,#13403,.T.);
#18450=ORIENTED_EDGE('',*,*,#13404,.T.);
#18451=ORIENTED_EDGE('',*,*,#13405,.T.);
#18452=ORIENTED_EDGE('',*,*,#13398,.F.);
#18453=ORIENTED_EDGE('',*,*,#13406,.F.);
#18454=ORIENTED_EDGE('',*,*,#13403,.F.);
#18455=ORIENTED_EDGE('',*,*,#13407,.F.);
#18456=ORIENTED_EDGE('',*,*,#13408,.T.);
#18457=ORIENTED_EDGE('',*,*,#13409,.T.);
#18458=ORIENTED_EDGE('',*,*,#13410,.T.);
#18459=ORIENTED_EDGE('',*,*,#13411,.T.);
#18460=ORIENTED_EDGE('',*,*,#13409,.F.);
#18461=ORIENTED_EDGE('',*,*,#13412,.F.);
#18462=ORIENTED_EDGE('',*,*,#13413,.F.);
#18463=ORIENTED_EDGE('',*,*,#13414,.F.);
#18464=ORIENTED_EDGE('',*,*,#13415,.T.);
#18465=ORIENTED_EDGE('',*,*,#13416,.T.);
#18466=ORIENTED_EDGE('',*,*,#13417,.T.);
#18467=ORIENTED_EDGE('',*,*,#13418,.T.);
#18468=ORIENTED_EDGE('',*,*,#13411,.F.);
#18469=ORIENTED_EDGE('',*,*,#13419,.F.);
#18470=ORIENTED_EDGE('',*,*,#13416,.F.);
#18471=ORIENTED_EDGE('',*,*,#13420,.F.);
#18472=ORIENTED_EDGE('',*,*,#13421,.T.);
#18473=ORIENTED_EDGE('',*,*,#13422,.T.);
#18474=ORIENTED_EDGE('',*,*,#13423,.T.);
#18475=ORIENTED_EDGE('',*,*,#13424,.T.);
#18476=ORIENTED_EDGE('',*,*,#13422,.F.);
#18477=ORIENTED_EDGE('',*,*,#13425,.F.);
#18478=ORIENTED_EDGE('',*,*,#13426,.F.);
#18479=ORIENTED_EDGE('',*,*,#13427,.F.);
#18480=ORIENTED_EDGE('',*,*,#13428,.T.);
#18481=ORIENTED_EDGE('',*,*,#13429,.T.);
#18482=ORIENTED_EDGE('',*,*,#13430,.T.);
#18483=ORIENTED_EDGE('',*,*,#13431,.T.);
#18484=ORIENTED_EDGE('',*,*,#13424,.F.);
#18485=ORIENTED_EDGE('',*,*,#13432,.F.);
#18486=ORIENTED_EDGE('',*,*,#13429,.F.);
#18487=ORIENTED_EDGE('',*,*,#13433,.F.);
#18488=ORIENTED_EDGE('',*,*,#13434,.T.);
#18489=ORIENTED_EDGE('',*,*,#13435,.T.);
#18490=ORIENTED_EDGE('',*,*,#13436,.T.);
#18491=ORIENTED_EDGE('',*,*,#13437,.T.);
#18492=ORIENTED_EDGE('',*,*,#13435,.F.);
#18493=ORIENTED_EDGE('',*,*,#13438,.F.);
#18494=ORIENTED_EDGE('',*,*,#13439,.F.);
#18495=ORIENTED_EDGE('',*,*,#13440,.F.);
#18496=ORIENTED_EDGE('',*,*,#13441,.T.);
#18497=ORIENTED_EDGE('',*,*,#13442,.T.);
#18498=ORIENTED_EDGE('',*,*,#13443,.T.);
#18499=ORIENTED_EDGE('',*,*,#13444,.T.);
#18500=ORIENTED_EDGE('',*,*,#13437,.F.);
#18501=ORIENTED_EDGE('',*,*,#13445,.F.);
#18502=ORIENTED_EDGE('',*,*,#13442,.F.);
#18503=ORIENTED_EDGE('',*,*,#13446,.F.);
#18504=ORIENTED_EDGE('',*,*,#13447,.T.);
#18505=ORIENTED_EDGE('',*,*,#13448,.T.);
#18506=ORIENTED_EDGE('',*,*,#13449,.T.);
#18507=ORIENTED_EDGE('',*,*,#13450,.T.);
#18508=ORIENTED_EDGE('',*,*,#13448,.F.);
#18509=ORIENTED_EDGE('',*,*,#13451,.F.);
#18510=ORIENTED_EDGE('',*,*,#13452,.F.);
#18511=ORIENTED_EDGE('',*,*,#13453,.F.);
#18512=ORIENTED_EDGE('',*,*,#13454,.T.);
#18513=ORIENTED_EDGE('',*,*,#13455,.T.);
#18514=ORIENTED_EDGE('',*,*,#13456,.T.);
#18515=ORIENTED_EDGE('',*,*,#13457,.T.);
#18516=ORIENTED_EDGE('',*,*,#13450,.F.);
#18517=ORIENTED_EDGE('',*,*,#13458,.F.);
#18518=ORIENTED_EDGE('',*,*,#13455,.F.);
#18519=ORIENTED_EDGE('',*,*,#13459,.F.);
#18520=ORIENTED_EDGE('',*,*,#13460,.T.);
#18521=ORIENTED_EDGE('',*,*,#13461,.T.);
#18522=ORIENTED_EDGE('',*,*,#13462,.T.);
#18523=ORIENTED_EDGE('',*,*,#13463,.T.);
#18524=ORIENTED_EDGE('',*,*,#13461,.F.);
#18525=ORIENTED_EDGE('',*,*,#13464,.F.);
#18526=ORIENTED_EDGE('',*,*,#13465,.F.);
#18527=ORIENTED_EDGE('',*,*,#13466,.F.);
#18528=ORIENTED_EDGE('',*,*,#13467,.T.);
#18529=ORIENTED_EDGE('',*,*,#13468,.T.);
#18530=ORIENTED_EDGE('',*,*,#13469,.T.);
#18531=ORIENTED_EDGE('',*,*,#13470,.T.);
#18532=ORIENTED_EDGE('',*,*,#13463,.F.);
#18533=ORIENTED_EDGE('',*,*,#13471,.F.);
#18534=ORIENTED_EDGE('',*,*,#13468,.F.);
#18535=ORIENTED_EDGE('',*,*,#13472,.F.);
#18536=ORIENTED_EDGE('',*,*,#13473,.T.);
#18537=ORIENTED_EDGE('',*,*,#13474,.T.);
#18538=ORIENTED_EDGE('',*,*,#13475,.T.);
#18539=ORIENTED_EDGE('',*,*,#13476,.T.);
#18540=ORIENTED_EDGE('',*,*,#13474,.F.);
#18541=ORIENTED_EDGE('',*,*,#13477,.F.);
#18542=ORIENTED_EDGE('',*,*,#13478,.F.);
#18543=ORIENTED_EDGE('',*,*,#13479,.F.);
#18544=ORIENTED_EDGE('',*,*,#13480,.T.);
#18545=ORIENTED_EDGE('',*,*,#13481,.T.);
#18546=ORIENTED_EDGE('',*,*,#13482,.T.);
#18547=ORIENTED_EDGE('',*,*,#13483,.T.);
#18548=ORIENTED_EDGE('',*,*,#13476,.F.);
#18549=ORIENTED_EDGE('',*,*,#13484,.F.);
#18550=ORIENTED_EDGE('',*,*,#13481,.F.);
#18551=ORIENTED_EDGE('',*,*,#13485,.F.);
#18552=ORIENTED_EDGE('',*,*,#13486,.T.);
#18553=ORIENTED_EDGE('',*,*,#13487,.T.);
#18554=ORIENTED_EDGE('',*,*,#13488,.T.);
#18555=ORIENTED_EDGE('',*,*,#13489,.T.);
#18556=ORIENTED_EDGE('',*,*,#13487,.F.);
#18557=ORIENTED_EDGE('',*,*,#13490,.F.);
#18558=ORIENTED_EDGE('',*,*,#13491,.F.);
#18559=ORIENTED_EDGE('',*,*,#13492,.F.);
#18560=ORIENTED_EDGE('',*,*,#13493,.T.);
#18561=ORIENTED_EDGE('',*,*,#13494,.T.);
#18562=ORIENTED_EDGE('',*,*,#13495,.T.);
#18563=ORIENTED_EDGE('',*,*,#13496,.T.);
#18564=ORIENTED_EDGE('',*,*,#13489,.F.);
#18565=ORIENTED_EDGE('',*,*,#13497,.F.);
#18566=ORIENTED_EDGE('',*,*,#13494,.F.);
#18567=ORIENTED_EDGE('',*,*,#13498,.F.);
#18568=ORIENTED_EDGE('',*,*,#13499,.T.);
#18569=ORIENTED_EDGE('',*,*,#13500,.T.);
#18570=ORIENTED_EDGE('',*,*,#13501,.T.);
#18571=ORIENTED_EDGE('',*,*,#13502,.T.);
#18572=ORIENTED_EDGE('',*,*,#13500,.F.);
#18573=ORIENTED_EDGE('',*,*,#13503,.F.);
#18574=ORIENTED_EDGE('',*,*,#13504,.F.);
#18575=ORIENTED_EDGE('',*,*,#13505,.F.);
#18576=ORIENTED_EDGE('',*,*,#13506,.T.);
#18577=ORIENTED_EDGE('',*,*,#13507,.T.);
#18578=ORIENTED_EDGE('',*,*,#13508,.T.);
#18579=ORIENTED_EDGE('',*,*,#13509,.T.);
#18580=ORIENTED_EDGE('',*,*,#13502,.F.);
#18581=ORIENTED_EDGE('',*,*,#13510,.F.);
#18582=ORIENTED_EDGE('',*,*,#13507,.F.);
#18583=ORIENTED_EDGE('',*,*,#13511,.F.);
#18584=ORIENTED_EDGE('',*,*,#13512,.T.);
#18585=ORIENTED_EDGE('',*,*,#13513,.T.);
#18586=ORIENTED_EDGE('',*,*,#13514,.T.);
#18587=ORIENTED_EDGE('',*,*,#13515,.T.);
#18588=ORIENTED_EDGE('',*,*,#13513,.F.);
#18589=ORIENTED_EDGE('',*,*,#13516,.F.);
#18590=ORIENTED_EDGE('',*,*,#13517,.F.);
#18591=ORIENTED_EDGE('',*,*,#13518,.F.);
#18592=ORIENTED_EDGE('',*,*,#13519,.T.);
#18593=ORIENTED_EDGE('',*,*,#13520,.T.);
#18594=ORIENTED_EDGE('',*,*,#13521,.T.);
#18595=ORIENTED_EDGE('',*,*,#13522,.T.);
#18596=ORIENTED_EDGE('',*,*,#13515,.F.);
#18597=ORIENTED_EDGE('',*,*,#13523,.F.);
#18598=ORIENTED_EDGE('',*,*,#13520,.F.);
#18599=ORIENTED_EDGE('',*,*,#13524,.F.);
#18600=ORIENTED_EDGE('',*,*,#13525,.T.);
#18601=ORIENTED_EDGE('',*,*,#13526,.T.);
#18602=ORIENTED_EDGE('',*,*,#13527,.T.);
#18603=ORIENTED_EDGE('',*,*,#13528,.T.);
#18604=ORIENTED_EDGE('',*,*,#13526,.F.);
#18605=ORIENTED_EDGE('',*,*,#13529,.F.);
#18606=ORIENTED_EDGE('',*,*,#13530,.F.);
#18607=ORIENTED_EDGE('',*,*,#13531,.F.);
#18608=ORIENTED_EDGE('',*,*,#13532,.T.);
#18609=ORIENTED_EDGE('',*,*,#13533,.T.);
#18610=ORIENTED_EDGE('',*,*,#13534,.T.);
#18611=ORIENTED_EDGE('',*,*,#13535,.T.);
#18612=ORIENTED_EDGE('',*,*,#13528,.F.);
#18613=ORIENTED_EDGE('',*,*,#13536,.F.);
#18614=ORIENTED_EDGE('',*,*,#13533,.F.);
#18615=ORIENTED_EDGE('',*,*,#13537,.F.);
#18616=ORIENTED_EDGE('',*,*,#13538,.T.);
#18617=ORIENTED_EDGE('',*,*,#13539,.T.);
#18618=ORIENTED_EDGE('',*,*,#13540,.T.);
#18619=ORIENTED_EDGE('',*,*,#13541,.T.);
#18620=ORIENTED_EDGE('',*,*,#13539,.F.);
#18621=ORIENTED_EDGE('',*,*,#13542,.F.);
#18622=ORIENTED_EDGE('',*,*,#13543,.F.);
#18623=ORIENTED_EDGE('',*,*,#13544,.F.);
#18624=ORIENTED_EDGE('',*,*,#13545,.T.);
#18625=ORIENTED_EDGE('',*,*,#13546,.T.);
#18626=ORIENTED_EDGE('',*,*,#13547,.T.);
#18627=ORIENTED_EDGE('',*,*,#13548,.T.);
#18628=ORIENTED_EDGE('',*,*,#13541,.F.);
#18629=ORIENTED_EDGE('',*,*,#13549,.F.);
#18630=ORIENTED_EDGE('',*,*,#13546,.F.);
#18631=ORIENTED_EDGE('',*,*,#13550,.F.);
#18632=ORIENTED_EDGE('',*,*,#13551,.T.);
#18633=ORIENTED_EDGE('',*,*,#13552,.T.);
#18634=ORIENTED_EDGE('',*,*,#13553,.T.);
#18635=ORIENTED_EDGE('',*,*,#13554,.T.);
#18636=ORIENTED_EDGE('',*,*,#13552,.F.);
#18637=ORIENTED_EDGE('',*,*,#13555,.F.);
#18638=ORIENTED_EDGE('',*,*,#13556,.F.);
#18639=ORIENTED_EDGE('',*,*,#13557,.F.);
#18640=ORIENTED_EDGE('',*,*,#13558,.T.);
#18641=ORIENTED_EDGE('',*,*,#13559,.T.);
#18642=ORIENTED_EDGE('',*,*,#13560,.T.);
#18643=ORIENTED_EDGE('',*,*,#13561,.T.);
#18644=ORIENTED_EDGE('',*,*,#13554,.F.);
#18645=ORIENTED_EDGE('',*,*,#13562,.F.);
#18646=ORIENTED_EDGE('',*,*,#13559,.F.);
#18647=ORIENTED_EDGE('',*,*,#13563,.F.);
#18648=ORIENTED_EDGE('',*,*,#13564,.T.);
#18649=ORIENTED_EDGE('',*,*,#13565,.T.);
#18650=ORIENTED_EDGE('',*,*,#13566,.T.);
#18651=ORIENTED_EDGE('',*,*,#13567,.T.);
#18652=ORIENTED_EDGE('',*,*,#13565,.F.);
#18653=ORIENTED_EDGE('',*,*,#13568,.F.);
#18654=ORIENTED_EDGE('',*,*,#13569,.F.);
#18655=ORIENTED_EDGE('',*,*,#13570,.F.);
#18656=ORIENTED_EDGE('',*,*,#13571,.T.);
#18657=ORIENTED_EDGE('',*,*,#13572,.T.);
#18658=ORIENTED_EDGE('',*,*,#13573,.T.);
#18659=ORIENTED_EDGE('',*,*,#13574,.T.);
#18660=ORIENTED_EDGE('',*,*,#13567,.F.);
#18661=ORIENTED_EDGE('',*,*,#13575,.F.);
#18662=ORIENTED_EDGE('',*,*,#13572,.F.);
#18663=ORIENTED_EDGE('',*,*,#13576,.F.);
#18664=ORIENTED_EDGE('',*,*,#12664,.F.);
#18665=ORIENTED_EDGE('',*,*,#13577,.F.);
#18666=ORIENTED_EDGE('',*,*,#13578,.F.);
#18667=ORIENTED_EDGE('',*,*,#13579,.F.);
#18668=ORIENTED_EDGE('',*,*,#12677,.F.);
#18669=ORIENTED_EDGE('',*,*,#13580,.F.);
#18670=ORIENTED_EDGE('',*,*,#13581,.F.);
#18671=ORIENTED_EDGE('',*,*,#13582,.F.);
#18672=ORIENTED_EDGE('',*,*,#12690,.F.);
#18673=ORIENTED_EDGE('',*,*,#13583,.F.);
#18674=ORIENTED_EDGE('',*,*,#13584,.F.);
#18675=ORIENTED_EDGE('',*,*,#13585,.F.);
#18676=ORIENTED_EDGE('',*,*,#12703,.F.);
#18677=ORIENTED_EDGE('',*,*,#13586,.F.);
#18678=ORIENTED_EDGE('',*,*,#13587,.F.);
#18679=ORIENTED_EDGE('',*,*,#13588,.F.);
#18680=ORIENTED_EDGE('',*,*,#12716,.F.);
#18681=ORIENTED_EDGE('',*,*,#13589,.F.);
#18682=ORIENTED_EDGE('',*,*,#13590,.F.);
#18683=ORIENTED_EDGE('',*,*,#13591,.F.);
#18684=ORIENTED_EDGE('',*,*,#12729,.F.);
#18685=ORIENTED_EDGE('',*,*,#13592,.F.);
#18686=ORIENTED_EDGE('',*,*,#13593,.F.);
#18687=ORIENTED_EDGE('',*,*,#13594,.F.);
#18688=ORIENTED_EDGE('',*,*,#12742,.F.);
#18689=ORIENTED_EDGE('',*,*,#13595,.F.);
#18690=ORIENTED_EDGE('',*,*,#13596,.F.);
#18691=ORIENTED_EDGE('',*,*,#13597,.F.);
#18692=ORIENTED_EDGE('',*,*,#12755,.F.);
#18693=ORIENTED_EDGE('',*,*,#13598,.F.);
#18694=ORIENTED_EDGE('',*,*,#13599,.F.);
#18695=ORIENTED_EDGE('',*,*,#13600,.F.);
#18696=ORIENTED_EDGE('',*,*,#12768,.F.);
#18697=ORIENTED_EDGE('',*,*,#13601,.F.);
#18698=ORIENTED_EDGE('',*,*,#13602,.F.);
#18699=ORIENTED_EDGE('',*,*,#13603,.F.);
#18700=ORIENTED_EDGE('',*,*,#12781,.F.);
#18701=ORIENTED_EDGE('',*,*,#13604,.F.);
#18702=ORIENTED_EDGE('',*,*,#13605,.F.);
#18703=ORIENTED_EDGE('',*,*,#13606,.F.);
#18704=ORIENTED_EDGE('',*,*,#12794,.F.);
#18705=ORIENTED_EDGE('',*,*,#13607,.F.);
#18706=ORIENTED_EDGE('',*,*,#13608,.F.);
#18707=ORIENTED_EDGE('',*,*,#13609,.F.);
#18708=ORIENTED_EDGE('',*,*,#12807,.F.);
#18709=ORIENTED_EDGE('',*,*,#13610,.F.);
#18710=ORIENTED_EDGE('',*,*,#13611,.F.);
#18711=ORIENTED_EDGE('',*,*,#13612,.F.);
#18712=ORIENTED_EDGE('',*,*,#12820,.F.);
#18713=ORIENTED_EDGE('',*,*,#13613,.F.);
#18714=ORIENTED_EDGE('',*,*,#13614,.F.);
#18715=ORIENTED_EDGE('',*,*,#13615,.F.);
#18716=ORIENTED_EDGE('',*,*,#12833,.F.);
#18717=ORIENTED_EDGE('',*,*,#13616,.F.);
#18718=ORIENTED_EDGE('',*,*,#13617,.F.);
#18719=ORIENTED_EDGE('',*,*,#13618,.F.);
#18720=ORIENTED_EDGE('',*,*,#12846,.F.);
#18721=ORIENTED_EDGE('',*,*,#13619,.F.);
#18722=ORIENTED_EDGE('',*,*,#13620,.F.);
#18723=ORIENTED_EDGE('',*,*,#13621,.F.);
#18724=ORIENTED_EDGE('',*,*,#12859,.F.);
#18725=ORIENTED_EDGE('',*,*,#13622,.F.);
#18726=ORIENTED_EDGE('',*,*,#13623,.F.);
#18727=ORIENTED_EDGE('',*,*,#13624,.F.);
#18728=ORIENTED_EDGE('',*,*,#12872,.F.);
#18729=ORIENTED_EDGE('',*,*,#13625,.F.);
#18730=ORIENTED_EDGE('',*,*,#13626,.F.);
#18731=ORIENTED_EDGE('',*,*,#13627,.F.);
#18732=ORIENTED_EDGE('',*,*,#12885,.F.);
#18733=ORIENTED_EDGE('',*,*,#13628,.F.);
#18734=ORIENTED_EDGE('',*,*,#13629,.F.);
#18735=ORIENTED_EDGE('',*,*,#13630,.F.);
#18736=ORIENTED_EDGE('',*,*,#12898,.F.);
#18737=ORIENTED_EDGE('',*,*,#13631,.F.);
#18738=ORIENTED_EDGE('',*,*,#13632,.F.);
#18739=ORIENTED_EDGE('',*,*,#13633,.F.);
#18740=ORIENTED_EDGE('',*,*,#12911,.F.);
#18741=ORIENTED_EDGE('',*,*,#13634,.F.);
#18742=ORIENTED_EDGE('',*,*,#13635,.F.);
#18743=ORIENTED_EDGE('',*,*,#13636,.F.);
#18744=ORIENTED_EDGE('',*,*,#12924,.F.);
#18745=ORIENTED_EDGE('',*,*,#13637,.F.);
#18746=ORIENTED_EDGE('',*,*,#13638,.F.);
#18747=ORIENTED_EDGE('',*,*,#13639,.F.);
#18748=ORIENTED_EDGE('',*,*,#12937,.F.);
#18749=ORIENTED_EDGE('',*,*,#13640,.F.);
#18750=ORIENTED_EDGE('',*,*,#13641,.F.);
#18751=ORIENTED_EDGE('',*,*,#13642,.F.);
#18752=ORIENTED_EDGE('',*,*,#12950,.F.);
#18753=ORIENTED_EDGE('',*,*,#13643,.F.);
#18754=ORIENTED_EDGE('',*,*,#13644,.F.);
#18755=ORIENTED_EDGE('',*,*,#13645,.F.);
#18756=ORIENTED_EDGE('',*,*,#12963,.F.);
#18757=ORIENTED_EDGE('',*,*,#13646,.F.);
#18758=ORIENTED_EDGE('',*,*,#13647,.F.);
#18759=ORIENTED_EDGE('',*,*,#13648,.F.);
#18760=ORIENTED_EDGE('',*,*,#12976,.F.);
#18761=ORIENTED_EDGE('',*,*,#13649,.F.);
#18762=ORIENTED_EDGE('',*,*,#13650,.F.);
#18763=ORIENTED_EDGE('',*,*,#13651,.F.);
#18764=ORIENTED_EDGE('',*,*,#12989,.F.);
#18765=ORIENTED_EDGE('',*,*,#13652,.F.);
#18766=ORIENTED_EDGE('',*,*,#13653,.F.);
#18767=ORIENTED_EDGE('',*,*,#13654,.F.);
#18768=ORIENTED_EDGE('',*,*,#13002,.F.);
#18769=ORIENTED_EDGE('',*,*,#13655,.F.);
#18770=ORIENTED_EDGE('',*,*,#13656,.F.);
#18771=ORIENTED_EDGE('',*,*,#13657,.F.);
#18772=ORIENTED_EDGE('',*,*,#13015,.F.);
#18773=ORIENTED_EDGE('',*,*,#13658,.F.);
#18774=ORIENTED_EDGE('',*,*,#13659,.F.);
#18775=ORIENTED_EDGE('',*,*,#13660,.F.);
#18776=ORIENTED_EDGE('',*,*,#13028,.F.);
#18777=ORIENTED_EDGE('',*,*,#13661,.F.);
#18778=ORIENTED_EDGE('',*,*,#13662,.F.);
#18779=ORIENTED_EDGE('',*,*,#13663,.F.);
#18780=ORIENTED_EDGE('',*,*,#13041,.F.);
#18781=ORIENTED_EDGE('',*,*,#13664,.F.);
#18782=ORIENTED_EDGE('',*,*,#13665,.F.);
#18783=ORIENTED_EDGE('',*,*,#13666,.F.);
#18784=ORIENTED_EDGE('',*,*,#13054,.F.);
#18785=ORIENTED_EDGE('',*,*,#13667,.F.);
#18786=ORIENTED_EDGE('',*,*,#13668,.F.);
#18787=ORIENTED_EDGE('',*,*,#13669,.F.);
#18788=ORIENTED_EDGE('',*,*,#13067,.F.);
#18789=ORIENTED_EDGE('',*,*,#13670,.F.);
#18790=ORIENTED_EDGE('',*,*,#13671,.F.);
#18791=ORIENTED_EDGE('',*,*,#13672,.F.);
#18792=ORIENTED_EDGE('',*,*,#13080,.F.);
#18793=ORIENTED_EDGE('',*,*,#13673,.F.);
#18794=ORIENTED_EDGE('',*,*,#13674,.F.);
#18795=ORIENTED_EDGE('',*,*,#13675,.F.);
#18796=ORIENTED_EDGE('',*,*,#13093,.F.);
#18797=ORIENTED_EDGE('',*,*,#13676,.F.);
#18798=ORIENTED_EDGE('',*,*,#13677,.F.);
#18799=ORIENTED_EDGE('',*,*,#13678,.F.);
#18800=ORIENTED_EDGE('',*,*,#13106,.F.);
#18801=ORIENTED_EDGE('',*,*,#13679,.F.);
#18802=ORIENTED_EDGE('',*,*,#13680,.F.);
#18803=ORIENTED_EDGE('',*,*,#13681,.F.);
#18804=ORIENTED_EDGE('',*,*,#13119,.F.);
#18805=ORIENTED_EDGE('',*,*,#13682,.F.);
#18806=ORIENTED_EDGE('',*,*,#13683,.F.);
#18807=ORIENTED_EDGE('',*,*,#13684,.F.);
#18808=ORIENTED_EDGE('',*,*,#13132,.F.);
#18809=ORIENTED_EDGE('',*,*,#13685,.F.);
#18810=ORIENTED_EDGE('',*,*,#13686,.F.);
#18811=ORIENTED_EDGE('',*,*,#13687,.F.);
#18812=ORIENTED_EDGE('',*,*,#13145,.F.);
#18813=ORIENTED_EDGE('',*,*,#13688,.F.);
#18814=ORIENTED_EDGE('',*,*,#13689,.F.);
#18815=ORIENTED_EDGE('',*,*,#13690,.F.);
#18816=ORIENTED_EDGE('',*,*,#13158,.F.);
#18817=ORIENTED_EDGE('',*,*,#13691,.F.);
#18818=ORIENTED_EDGE('',*,*,#13692,.F.);
#18819=ORIENTED_EDGE('',*,*,#13693,.F.);
#18820=ORIENTED_EDGE('',*,*,#13171,.F.);
#18821=ORIENTED_EDGE('',*,*,#13694,.F.);
#18822=ORIENTED_EDGE('',*,*,#13695,.F.);
#18823=ORIENTED_EDGE('',*,*,#13696,.F.);
#18824=ORIENTED_EDGE('',*,*,#13184,.F.);
#18825=ORIENTED_EDGE('',*,*,#13697,.F.);
#18826=ORIENTED_EDGE('',*,*,#13698,.F.);
#18827=ORIENTED_EDGE('',*,*,#13699,.F.);
#18828=ORIENTED_EDGE('',*,*,#13197,.F.);
#18829=ORIENTED_EDGE('',*,*,#13700,.F.);
#18830=ORIENTED_EDGE('',*,*,#13701,.F.);
#18831=ORIENTED_EDGE('',*,*,#13702,.F.);
#18832=ORIENTED_EDGE('',*,*,#13210,.F.);
#18833=ORIENTED_EDGE('',*,*,#13703,.F.);
#18834=ORIENTED_EDGE('',*,*,#13704,.F.);
#18835=ORIENTED_EDGE('',*,*,#13705,.F.);
#18836=ORIENTED_EDGE('',*,*,#13223,.F.);
#18837=ORIENTED_EDGE('',*,*,#13706,.F.);
#18838=ORIENTED_EDGE('',*,*,#13707,.F.);
#18839=ORIENTED_EDGE('',*,*,#13708,.F.);
#18840=ORIENTED_EDGE('',*,*,#13236,.F.);
#18841=ORIENTED_EDGE('',*,*,#13709,.F.);
#18842=ORIENTED_EDGE('',*,*,#13710,.F.);
#18843=ORIENTED_EDGE('',*,*,#13711,.F.);
#18844=ORIENTED_EDGE('',*,*,#13249,.F.);
#18845=ORIENTED_EDGE('',*,*,#13712,.F.);
#18846=ORIENTED_EDGE('',*,*,#13713,.F.);
#18847=ORIENTED_EDGE('',*,*,#13714,.F.);
#18848=ORIENTED_EDGE('',*,*,#13262,.F.);
#18849=ORIENTED_EDGE('',*,*,#13715,.F.);
#18850=ORIENTED_EDGE('',*,*,#13716,.F.);
#18851=ORIENTED_EDGE('',*,*,#13717,.F.);
#18852=ORIENTED_EDGE('',*,*,#13275,.F.);
#18853=ORIENTED_EDGE('',*,*,#13718,.F.);
#18854=ORIENTED_EDGE('',*,*,#13719,.F.);
#18855=ORIENTED_EDGE('',*,*,#13720,.F.);
#18856=ORIENTED_EDGE('',*,*,#13288,.F.);
#18857=ORIENTED_EDGE('',*,*,#13721,.F.);
#18858=ORIENTED_EDGE('',*,*,#13722,.F.);
#18859=ORIENTED_EDGE('',*,*,#13723,.F.);
#18860=ORIENTED_EDGE('',*,*,#13301,.F.);
#18861=ORIENTED_EDGE('',*,*,#13724,.F.);
#18862=ORIENTED_EDGE('',*,*,#13725,.F.);
#18863=ORIENTED_EDGE('',*,*,#13726,.F.);
#18864=ORIENTED_EDGE('',*,*,#13314,.F.);
#18865=ORIENTED_EDGE('',*,*,#13727,.F.);
#18866=ORIENTED_EDGE('',*,*,#13728,.F.);
#18867=ORIENTED_EDGE('',*,*,#13729,.F.);
#18868=ORIENTED_EDGE('',*,*,#13327,.F.);
#18869=ORIENTED_EDGE('',*,*,#13730,.F.);
#18870=ORIENTED_EDGE('',*,*,#13731,.F.);
#18871=ORIENTED_EDGE('',*,*,#13732,.F.);
#18872=ORIENTED_EDGE('',*,*,#13340,.F.);
#18873=ORIENTED_EDGE('',*,*,#13733,.F.);
#18874=ORIENTED_EDGE('',*,*,#13734,.F.);
#18875=ORIENTED_EDGE('',*,*,#13735,.F.);
#18876=ORIENTED_EDGE('',*,*,#13353,.F.);
#18877=ORIENTED_EDGE('',*,*,#13736,.F.);
#18878=ORIENTED_EDGE('',*,*,#13737,.F.);
#18879=ORIENTED_EDGE('',*,*,#13738,.F.);
#18880=ORIENTED_EDGE('',*,*,#13366,.F.);
#18881=ORIENTED_EDGE('',*,*,#13739,.F.);
#18882=ORIENTED_EDGE('',*,*,#13740,.F.);
#18883=ORIENTED_EDGE('',*,*,#13741,.F.);
#18884=ORIENTED_EDGE('',*,*,#13379,.F.);
#18885=ORIENTED_EDGE('',*,*,#13742,.F.);
#18886=ORIENTED_EDGE('',*,*,#13743,.F.);
#18887=ORIENTED_EDGE('',*,*,#13744,.F.);
#18888=ORIENTED_EDGE('',*,*,#13392,.F.);
#18889=ORIENTED_EDGE('',*,*,#13745,.F.);
#18890=ORIENTED_EDGE('',*,*,#13746,.F.);
#18891=ORIENTED_EDGE('',*,*,#13747,.F.);
#18892=ORIENTED_EDGE('',*,*,#13405,.F.);
#18893=ORIENTED_EDGE('',*,*,#13748,.F.);
#18894=ORIENTED_EDGE('',*,*,#13749,.F.);
#18895=ORIENTED_EDGE('',*,*,#13750,.F.);
#18896=ORIENTED_EDGE('',*,*,#13418,.F.);
#18897=ORIENTED_EDGE('',*,*,#13751,.F.);
#18898=ORIENTED_EDGE('',*,*,#13752,.F.);
#18899=ORIENTED_EDGE('',*,*,#13753,.F.);
#18900=ORIENTED_EDGE('',*,*,#13431,.F.);
#18901=ORIENTED_EDGE('',*,*,#13754,.F.);
#18902=ORIENTED_EDGE('',*,*,#13755,.F.);
#18903=ORIENTED_EDGE('',*,*,#13756,.F.);
#18904=ORIENTED_EDGE('',*,*,#13444,.F.);
#18905=ORIENTED_EDGE('',*,*,#13757,.F.);
#18906=ORIENTED_EDGE('',*,*,#13758,.F.);
#18907=ORIENTED_EDGE('',*,*,#13759,.F.);
#18908=ORIENTED_EDGE('',*,*,#13457,.F.);
#18909=ORIENTED_EDGE('',*,*,#13760,.F.);
#18910=ORIENTED_EDGE('',*,*,#13761,.F.);
#18911=ORIENTED_EDGE('',*,*,#13762,.F.);
#18912=ORIENTED_EDGE('',*,*,#13470,.F.);
#18913=ORIENTED_EDGE('',*,*,#13763,.F.);
#18914=ORIENTED_EDGE('',*,*,#13764,.F.);
#18915=ORIENTED_EDGE('',*,*,#13765,.F.);
#18916=ORIENTED_EDGE('',*,*,#13483,.F.);
#18917=ORIENTED_EDGE('',*,*,#13766,.F.);
#18918=ORIENTED_EDGE('',*,*,#13767,.F.);
#18919=ORIENTED_EDGE('',*,*,#13768,.F.);
#18920=ORIENTED_EDGE('',*,*,#13496,.F.);
#18921=ORIENTED_EDGE('',*,*,#13769,.F.);
#18922=ORIENTED_EDGE('',*,*,#13770,.F.);
#18923=ORIENTED_EDGE('',*,*,#13771,.F.);
#18924=ORIENTED_EDGE('',*,*,#13509,.F.);
#18925=ORIENTED_EDGE('',*,*,#13772,.F.);
#18926=ORIENTED_EDGE('',*,*,#13773,.F.);
#18927=ORIENTED_EDGE('',*,*,#13774,.F.);
#18928=ORIENTED_EDGE('',*,*,#13522,.F.);
#18929=ORIENTED_EDGE('',*,*,#13775,.F.);
#18930=ORIENTED_EDGE('',*,*,#13776,.F.);
#18931=ORIENTED_EDGE('',*,*,#13777,.F.);
#18932=ORIENTED_EDGE('',*,*,#13535,.F.);
#18933=ORIENTED_EDGE('',*,*,#13778,.F.);
#18934=ORIENTED_EDGE('',*,*,#13779,.F.);
#18935=ORIENTED_EDGE('',*,*,#13780,.F.);
#18936=ORIENTED_EDGE('',*,*,#13548,.F.);
#18937=ORIENTED_EDGE('',*,*,#13781,.F.);
#18938=ORIENTED_EDGE('',*,*,#13782,.F.);
#18939=ORIENTED_EDGE('',*,*,#13783,.F.);
#18940=ORIENTED_EDGE('',*,*,#13561,.F.);
#18941=ORIENTED_EDGE('',*,*,#13784,.F.);
#18942=ORIENTED_EDGE('',*,*,#13785,.F.);
#18943=ORIENTED_EDGE('',*,*,#13786,.F.);
#18944=ORIENTED_EDGE('',*,*,#13574,.F.);
#18945=ORIENTED_EDGE('',*,*,#13787,.F.);
#18946=ORIENTED_EDGE('',*,*,#13788,.F.);
#18947=ORIENTED_EDGE('',*,*,#13789,.F.);
#18948=ORIENTED_EDGE('',*,*,#13569,.T.);
#18949=ORIENTED_EDGE('',*,*,#13790,.T.);
#18950=ORIENTED_EDGE('',*,*,#13791,.T.);
#18951=ORIENTED_EDGE('',*,*,#13792,.F.);
#18952=ORIENTED_EDGE('',*,*,#13556,.T.);
#18953=ORIENTED_EDGE('',*,*,#13793,.T.);
#18954=ORIENTED_EDGE('',*,*,#13788,.T.);
#18955=ORIENTED_EDGE('',*,*,#13794,.F.);
#18956=ORIENTED_EDGE('',*,*,#13543,.T.);
#18957=ORIENTED_EDGE('',*,*,#13795,.T.);
#18958=ORIENTED_EDGE('',*,*,#13785,.T.);
#18959=ORIENTED_EDGE('',*,*,#13796,.F.);
#18960=ORIENTED_EDGE('',*,*,#13530,.T.);
#18961=ORIENTED_EDGE('',*,*,#13797,.T.);
#18962=ORIENTED_EDGE('',*,*,#13782,.T.);
#18963=ORIENTED_EDGE('',*,*,#13798,.F.);
#18964=ORIENTED_EDGE('',*,*,#13517,.T.);
#18965=ORIENTED_EDGE('',*,*,#13799,.T.);
#18966=ORIENTED_EDGE('',*,*,#13779,.T.);
#18967=ORIENTED_EDGE('',*,*,#13800,.F.);
#18968=ORIENTED_EDGE('',*,*,#13504,.T.);
#18969=ORIENTED_EDGE('',*,*,#13801,.T.);
#18970=ORIENTED_EDGE('',*,*,#13776,.T.);
#18971=ORIENTED_EDGE('',*,*,#13802,.F.);
#18972=ORIENTED_EDGE('',*,*,#13491,.T.);
#18973=ORIENTED_EDGE('',*,*,#13803,.T.);
#18974=ORIENTED_EDGE('',*,*,#13773,.T.);
#18975=ORIENTED_EDGE('',*,*,#13804,.F.);
#18976=ORIENTED_EDGE('',*,*,#13478,.T.);
#18977=ORIENTED_EDGE('',*,*,#13805,.T.);
#18978=ORIENTED_EDGE('',*,*,#13770,.T.);
#18979=ORIENTED_EDGE('',*,*,#13806,.F.);
#18980=ORIENTED_EDGE('',*,*,#13465,.T.);
#18981=ORIENTED_EDGE('',*,*,#13807,.T.);
#18982=ORIENTED_EDGE('',*,*,#13767,.T.);
#18983=ORIENTED_EDGE('',*,*,#13808,.F.);
#18984=ORIENTED_EDGE('',*,*,#13452,.T.);
#18985=ORIENTED_EDGE('',*,*,#13809,.T.);
#18986=ORIENTED_EDGE('',*,*,#13764,.T.);
#18987=ORIENTED_EDGE('',*,*,#13810,.F.);
#18988=ORIENTED_EDGE('',*,*,#13439,.T.);
#18989=ORIENTED_EDGE('',*,*,#13811,.T.);
#18990=ORIENTED_EDGE('',*,*,#13761,.T.);
#18991=ORIENTED_EDGE('',*,*,#13812,.F.);
#18992=ORIENTED_EDGE('',*,*,#13426,.T.);
#18993=ORIENTED_EDGE('',*,*,#13813,.T.);
#18994=ORIENTED_EDGE('',*,*,#13758,.T.);
#18995=ORIENTED_EDGE('',*,*,#13814,.F.);
#18996=ORIENTED_EDGE('',*,*,#13413,.T.);
#18997=ORIENTED_EDGE('',*,*,#13815,.T.);
#18998=ORIENTED_EDGE('',*,*,#13755,.T.);
#18999=ORIENTED_EDGE('',*,*,#13816,.F.);
#19000=ORIENTED_EDGE('',*,*,#13400,.T.);
#19001=ORIENTED_EDGE('',*,*,#13817,.T.);
#19002=ORIENTED_EDGE('',*,*,#13752,.T.);
#19003=ORIENTED_EDGE('',*,*,#13818,.F.);
#19004=ORIENTED_EDGE('',*,*,#13387,.T.);
#19005=ORIENTED_EDGE('',*,*,#13819,.T.);
#19006=ORIENTED_EDGE('',*,*,#13749,.T.);
#19007=ORIENTED_EDGE('',*,*,#13820,.F.);
#19008=ORIENTED_EDGE('',*,*,#13374,.T.);
#19009=ORIENTED_EDGE('',*,*,#13821,.T.);
#19010=ORIENTED_EDGE('',*,*,#13746,.T.);
#19011=ORIENTED_EDGE('',*,*,#13822,.F.);
#19012=ORIENTED_EDGE('',*,*,#13361,.T.);
#19013=ORIENTED_EDGE('',*,*,#13823,.T.);
#19014=ORIENTED_EDGE('',*,*,#13743,.T.);
#19015=ORIENTED_EDGE('',*,*,#13824,.F.);
#19016=ORIENTED_EDGE('',*,*,#13348,.T.);
#19017=ORIENTED_EDGE('',*,*,#13825,.T.);
#19018=ORIENTED_EDGE('',*,*,#13740,.T.);
#19019=ORIENTED_EDGE('',*,*,#13826,.F.);
#19020=ORIENTED_EDGE('',*,*,#13335,.T.);
#19021=ORIENTED_EDGE('',*,*,#13827,.T.);
#19022=ORIENTED_EDGE('',*,*,#13737,.T.);
#19023=ORIENTED_EDGE('',*,*,#13828,.F.);
#19024=ORIENTED_EDGE('',*,*,#13322,.T.);
#19025=ORIENTED_EDGE('',*,*,#13829,.T.);
#19026=ORIENTED_EDGE('',*,*,#13734,.T.);
#19027=ORIENTED_EDGE('',*,*,#13830,.F.);
#19028=ORIENTED_EDGE('',*,*,#13309,.T.);
#19029=ORIENTED_EDGE('',*,*,#13831,.T.);
#19030=ORIENTED_EDGE('',*,*,#13731,.T.);
#19031=ORIENTED_EDGE('',*,*,#13832,.F.);
#19032=ORIENTED_EDGE('',*,*,#13296,.T.);
#19033=ORIENTED_EDGE('',*,*,#13833,.T.);
#19034=ORIENTED_EDGE('',*,*,#13728,.T.);
#19035=ORIENTED_EDGE('',*,*,#13834,.F.);
#19036=ORIENTED_EDGE('',*,*,#13283,.T.);
#19037=ORIENTED_EDGE('',*,*,#13835,.T.);
#19038=ORIENTED_EDGE('',*,*,#13725,.T.);
#19039=ORIENTED_EDGE('',*,*,#13836,.F.);
#19040=ORIENTED_EDGE('',*,*,#13270,.T.);
#19041=ORIENTED_EDGE('',*,*,#13837,.T.);
#19042=ORIENTED_EDGE('',*,*,#13722,.T.);
#19043=ORIENTED_EDGE('',*,*,#13838,.F.);
#19044=ORIENTED_EDGE('',*,*,#13257,.T.);
#19045=ORIENTED_EDGE('',*,*,#13839,.T.);
#19046=ORIENTED_EDGE('',*,*,#13719,.T.);
#19047=ORIENTED_EDGE('',*,*,#13840,.F.);
#19048=ORIENTED_EDGE('',*,*,#13244,.T.);
#19049=ORIENTED_EDGE('',*,*,#13841,.T.);
#19050=ORIENTED_EDGE('',*,*,#13716,.T.);
#19051=ORIENTED_EDGE('',*,*,#13842,.F.);
#19052=ORIENTED_EDGE('',*,*,#13231,.T.);
#19053=ORIENTED_EDGE('',*,*,#13843,.T.);
#19054=ORIENTED_EDGE('',*,*,#13713,.T.);
#19055=ORIENTED_EDGE('',*,*,#13844,.F.);
#19056=ORIENTED_EDGE('',*,*,#13218,.T.);
#19057=ORIENTED_EDGE('',*,*,#13845,.T.);
#19058=ORIENTED_EDGE('',*,*,#13710,.T.);
#19059=ORIENTED_EDGE('',*,*,#13846,.F.);
#19060=ORIENTED_EDGE('',*,*,#13205,.T.);
#19061=ORIENTED_EDGE('',*,*,#13847,.T.);
#19062=ORIENTED_EDGE('',*,*,#13707,.T.);
#19063=ORIENTED_EDGE('',*,*,#13848,.F.);
#19064=ORIENTED_EDGE('',*,*,#13192,.T.);
#19065=ORIENTED_EDGE('',*,*,#13849,.T.);
#19066=ORIENTED_EDGE('',*,*,#13704,.T.);
#19067=ORIENTED_EDGE('',*,*,#13850,.F.);
#19068=ORIENTED_EDGE('',*,*,#13179,.T.);
#19069=ORIENTED_EDGE('',*,*,#13851,.T.);
#19070=ORIENTED_EDGE('',*,*,#13701,.T.);
#19071=ORIENTED_EDGE('',*,*,#13852,.F.);
#19072=ORIENTED_EDGE('',*,*,#13166,.T.);
#19073=ORIENTED_EDGE('',*,*,#13853,.T.);
#19074=ORIENTED_EDGE('',*,*,#13698,.T.);
#19075=ORIENTED_EDGE('',*,*,#13854,.F.);
#19076=ORIENTED_EDGE('',*,*,#13153,.T.);
#19077=ORIENTED_EDGE('',*,*,#13855,.T.);
#19078=ORIENTED_EDGE('',*,*,#13695,.T.);
#19079=ORIENTED_EDGE('',*,*,#13856,.F.);
#19080=ORIENTED_EDGE('',*,*,#13140,.T.);
#19081=ORIENTED_EDGE('',*,*,#13857,.T.);
#19082=ORIENTED_EDGE('',*,*,#13692,.T.);
#19083=ORIENTED_EDGE('',*,*,#13858,.F.);
#19084=ORIENTED_EDGE('',*,*,#13127,.T.);
#19085=ORIENTED_EDGE('',*,*,#13859,.T.);
#19086=ORIENTED_EDGE('',*,*,#13689,.T.);
#19087=ORIENTED_EDGE('',*,*,#13860,.F.);
#19088=ORIENTED_EDGE('',*,*,#13114,.T.);
#19089=ORIENTED_EDGE('',*,*,#13861,.T.);
#19090=ORIENTED_EDGE('',*,*,#13686,.T.);
#19091=ORIENTED_EDGE('',*,*,#13862,.F.);
#19092=ORIENTED_EDGE('',*,*,#13101,.T.);
#19093=ORIENTED_EDGE('',*,*,#13863,.T.);
#19094=ORIENTED_EDGE('',*,*,#13683,.T.);
#19095=ORIENTED_EDGE('',*,*,#13864,.F.);
#19096=ORIENTED_EDGE('',*,*,#13088,.T.);
#19097=ORIENTED_EDGE('',*,*,#13865,.T.);
#19098=ORIENTED_EDGE('',*,*,#13680,.T.);
#19099=ORIENTED_EDGE('',*,*,#13866,.F.);
#19100=ORIENTED_EDGE('',*,*,#13075,.T.);
#19101=ORIENTED_EDGE('',*,*,#13867,.T.);
#19102=ORIENTED_EDGE('',*,*,#13677,.T.);
#19103=ORIENTED_EDGE('',*,*,#13868,.F.);
#19104=ORIENTED_EDGE('',*,*,#13062,.T.);
#19105=ORIENTED_EDGE('',*,*,#13869,.T.);
#19106=ORIENTED_EDGE('',*,*,#13674,.T.);
#19107=ORIENTED_EDGE('',*,*,#13870,.F.);
#19108=ORIENTED_EDGE('',*,*,#13049,.T.);
#19109=ORIENTED_EDGE('',*,*,#13871,.T.);
#19110=ORIENTED_EDGE('',*,*,#13671,.T.);
#19111=ORIENTED_EDGE('',*,*,#13872,.F.);
#19112=ORIENTED_EDGE('',*,*,#13036,.T.);
#19113=ORIENTED_EDGE('',*,*,#13873,.T.);
#19114=ORIENTED_EDGE('',*,*,#13668,.T.);
#19115=ORIENTED_EDGE('',*,*,#13874,.F.);
#19116=ORIENTED_EDGE('',*,*,#13023,.T.);
#19117=ORIENTED_EDGE('',*,*,#13875,.T.);
#19118=ORIENTED_EDGE('',*,*,#13665,.T.);
#19119=ORIENTED_EDGE('',*,*,#13876,.F.);
#19120=ORIENTED_EDGE('',*,*,#13010,.T.);
#19121=ORIENTED_EDGE('',*,*,#13877,.T.);
#19122=ORIENTED_EDGE('',*,*,#13662,.T.);
#19123=ORIENTED_EDGE('',*,*,#13878,.F.);
#19124=ORIENTED_EDGE('',*,*,#12997,.T.);
#19125=ORIENTED_EDGE('',*,*,#13879,.T.);
#19126=ORIENTED_EDGE('',*,*,#13659,.T.);
#19127=ORIENTED_EDGE('',*,*,#13880,.F.);
#19128=ORIENTED_EDGE('',*,*,#12984,.T.);
#19129=ORIENTED_EDGE('',*,*,#13881,.T.);
#19130=ORIENTED_EDGE('',*,*,#13656,.T.);
#19131=ORIENTED_EDGE('',*,*,#13882,.F.);
#19132=ORIENTED_EDGE('',*,*,#12971,.T.);
#19133=ORIENTED_EDGE('',*,*,#13883,.T.);
#19134=ORIENTED_EDGE('',*,*,#13653,.T.);
#19135=ORIENTED_EDGE('',*,*,#13884,.F.);
#19136=ORIENTED_EDGE('',*,*,#12958,.T.);
#19137=ORIENTED_EDGE('',*,*,#13885,.T.);
#19138=ORIENTED_EDGE('',*,*,#13650,.T.);
#19139=ORIENTED_EDGE('',*,*,#13886,.F.);
#19140=ORIENTED_EDGE('',*,*,#12945,.T.);
#19141=ORIENTED_EDGE('',*,*,#13887,.T.);
#19142=ORIENTED_EDGE('',*,*,#13647,.T.);
#19143=ORIENTED_EDGE('',*,*,#13888,.F.);
#19144=ORIENTED_EDGE('',*,*,#12932,.T.);
#19145=ORIENTED_EDGE('',*,*,#13889,.T.);
#19146=ORIENTED_EDGE('',*,*,#13644,.T.);
#19147=ORIENTED_EDGE('',*,*,#13890,.F.);
#19148=ORIENTED_EDGE('',*,*,#12919,.T.);
#19149=ORIENTED_EDGE('',*,*,#13891,.T.);
#19150=ORIENTED_EDGE('',*,*,#13641,.T.);
#19151=ORIENTED_EDGE('',*,*,#13892,.F.);
#19152=ORIENTED_EDGE('',*,*,#12906,.T.);
#19153=ORIENTED_EDGE('',*,*,#13893,.T.);
#19154=ORIENTED_EDGE('',*,*,#13638,.T.);
#19155=ORIENTED_EDGE('',*,*,#13894,.F.);
#19156=ORIENTED_EDGE('',*,*,#12893,.T.);
#19157=ORIENTED_EDGE('',*,*,#13895,.T.);
#19158=ORIENTED_EDGE('',*,*,#13635,.T.);
#19159=ORIENTED_EDGE('',*,*,#13896,.F.);
#19160=ORIENTED_EDGE('',*,*,#12880,.T.);
#19161=ORIENTED_EDGE('',*,*,#13897,.T.);
#19162=ORIENTED_EDGE('',*,*,#13632,.T.);
#19163=ORIENTED_EDGE('',*,*,#13898,.F.);
#19164=ORIENTED_EDGE('',*,*,#12867,.T.);
#19165=ORIENTED_EDGE('',*,*,#13899,.T.);
#19166=ORIENTED_EDGE('',*,*,#13629,.T.);
#19167=ORIENTED_EDGE('',*,*,#13900,.F.);
#19168=ORIENTED_EDGE('',*,*,#12854,.T.);
#19169=ORIENTED_EDGE('',*,*,#13901,.T.);
#19170=ORIENTED_EDGE('',*,*,#13626,.T.);
#19171=ORIENTED_EDGE('',*,*,#13902,.F.);
#19172=ORIENTED_EDGE('',*,*,#12841,.T.);
#19173=ORIENTED_EDGE('',*,*,#13903,.T.);
#19174=ORIENTED_EDGE('',*,*,#13623,.T.);
#19175=ORIENTED_EDGE('',*,*,#13904,.F.);
#19176=ORIENTED_EDGE('',*,*,#12828,.T.);
#19177=ORIENTED_EDGE('',*,*,#13905,.T.);
#19178=ORIENTED_EDGE('',*,*,#13620,.T.);
#19179=ORIENTED_EDGE('',*,*,#13906,.F.);
#19180=ORIENTED_EDGE('',*,*,#12815,.T.);
#19181=ORIENTED_EDGE('',*,*,#13907,.T.);
#19182=ORIENTED_EDGE('',*,*,#13617,.T.);
#19183=ORIENTED_EDGE('',*,*,#13908,.F.);
#19184=ORIENTED_EDGE('',*,*,#12802,.T.);
#19185=ORIENTED_EDGE('',*,*,#13909,.T.);
#19186=ORIENTED_EDGE('',*,*,#13614,.T.);
#19187=ORIENTED_EDGE('',*,*,#13910,.F.);
#19188=ORIENTED_EDGE('',*,*,#12789,.T.);
#19189=ORIENTED_EDGE('',*,*,#13911,.T.);
#19190=ORIENTED_EDGE('',*,*,#13611,.T.);
#19191=ORIENTED_EDGE('',*,*,#13912,.F.);
#19192=ORIENTED_EDGE('',*,*,#12776,.T.);
#19193=ORIENTED_EDGE('',*,*,#13913,.T.);
#19194=ORIENTED_EDGE('',*,*,#13608,.T.);
#19195=ORIENTED_EDGE('',*,*,#13914,.F.);
#19196=ORIENTED_EDGE('',*,*,#12763,.T.);
#19197=ORIENTED_EDGE('',*,*,#13915,.T.);
#19198=ORIENTED_EDGE('',*,*,#13605,.T.);
#19199=ORIENTED_EDGE('',*,*,#13916,.F.);
#19200=ORIENTED_EDGE('',*,*,#12750,.T.);
#19201=ORIENTED_EDGE('',*,*,#13917,.T.);
#19202=ORIENTED_EDGE('',*,*,#13602,.T.);
#19203=ORIENTED_EDGE('',*,*,#13918,.F.);
#19204=ORIENTED_EDGE('',*,*,#12737,.T.);
#19205=ORIENTED_EDGE('',*,*,#13919,.T.);
#19206=ORIENTED_EDGE('',*,*,#13599,.T.);
#19207=ORIENTED_EDGE('',*,*,#13920,.F.);
#19208=ORIENTED_EDGE('',*,*,#12724,.T.);
#19209=ORIENTED_EDGE('',*,*,#13921,.T.);
#19210=ORIENTED_EDGE('',*,*,#13596,.T.);
#19211=ORIENTED_EDGE('',*,*,#13922,.F.);
#19212=ORIENTED_EDGE('',*,*,#12711,.T.);
#19213=ORIENTED_EDGE('',*,*,#13923,.T.);
#19214=ORIENTED_EDGE('',*,*,#13593,.T.);
#19215=ORIENTED_EDGE('',*,*,#13924,.F.);
#19216=ORIENTED_EDGE('',*,*,#12698,.T.);
#19217=ORIENTED_EDGE('',*,*,#13925,.T.);
#19218=ORIENTED_EDGE('',*,*,#13590,.T.);
#19219=ORIENTED_EDGE('',*,*,#13926,.F.);
#19220=ORIENTED_EDGE('',*,*,#12685,.T.);
#19221=ORIENTED_EDGE('',*,*,#13927,.T.);
#19222=ORIENTED_EDGE('',*,*,#13587,.T.);
#19223=ORIENTED_EDGE('',*,*,#13928,.F.);
#19224=ORIENTED_EDGE('',*,*,#12672,.T.);
#19225=ORIENTED_EDGE('',*,*,#13929,.T.);
#19226=ORIENTED_EDGE('',*,*,#13584,.T.);
#19227=ORIENTED_EDGE('',*,*,#13930,.F.);
#19228=ORIENTED_EDGE('',*,*,#13578,.T.);
#19229=ORIENTED_EDGE('',*,*,#13931,.F.);
#19230=ORIENTED_EDGE('',*,*,#13932,.T.);
#19231=ORIENTED_EDGE('',*,*,#13933,.T.);
#19232=ORIENTED_EDGE('',*,*,#13934,.T.);
#19233=ORIENTED_EDGE('',*,*,#13935,.T.);
#19234=ORIENTED_EDGE('',*,*,#13936,.T.);
#19235=ORIENTED_EDGE('',*,*,#13937,.T.);
#19236=ORIENTED_EDGE('',*,*,#13935,.F.);
#19237=ORIENTED_EDGE('',*,*,#13938,.F.);
#19238=ORIENTED_EDGE('',*,*,#13932,.F.);
#19239=ORIENTED_EDGE('',*,*,#13939,.F.);
#19240=ORIENTED_EDGE('',*,*,#13940,.T.);
#19241=ORIENTED_EDGE('',*,*,#13941,.T.);
#19242=ORIENTED_EDGE('',*,*,#13942,.T.);
#19243=ORIENTED_EDGE('',*,*,#13943,.T.);
#19244=ORIENTED_EDGE('',*,*,#13937,.F.);
#19245=ORIENTED_EDGE('',*,*,#13944,.F.);
#19246=ORIENTED_EDGE('',*,*,#13941,.F.);
#19247=ORIENTED_EDGE('',*,*,#13945,.F.);
#19248=ORIENTED_EDGE('',*,*,#13943,.F.);
#19249=ORIENTED_EDGE('',*,*,#13946,.F.);
#19250=ORIENTED_EDGE('',*,*,#13791,.F.);
#19251=ORIENTED_EDGE('',*,*,#13947,.F.);
#19252=ORIENTED_EDGE('',*,*,#13948,.T.);
#19253=ORIENTED_EDGE('',*,*,#12660,.T.);
#19254=ORIENTED_EDGE('',*,*,#13949,.T.);
#19255=ORIENTED_EDGE('',*,*,#13580,.T.);
#19256=ORIENTED_EDGE('',*,*,#12676,.F.);
#19257=ORIENTED_EDGE('',*,*,#12678,.T.);
#19258=ORIENTED_EDGE('',*,*,#12669,.F.);
#19259=ORIENTED_EDGE('',*,*,#12673,.T.);
#19260=ORIENTED_EDGE('',*,*,#13930,.T.);
#19261=ORIENTED_EDGE('',*,*,#13583,.T.);
#19262=ORIENTED_EDGE('',*,*,#12689,.F.);
#19263=ORIENTED_EDGE('',*,*,#12691,.T.);
#19264=ORIENTED_EDGE('',*,*,#12682,.F.);
#19265=ORIENTED_EDGE('',*,*,#12686,.T.);
#19266=ORIENTED_EDGE('',*,*,#13928,.T.);
#19267=ORIENTED_EDGE('',*,*,#13586,.T.);
#19268=ORIENTED_EDGE('',*,*,#12702,.F.);
#19269=ORIENTED_EDGE('',*,*,#12704,.T.);
#19270=ORIENTED_EDGE('',*,*,#12695,.F.);
#19271=ORIENTED_EDGE('',*,*,#12699,.T.);
#19272=ORIENTED_EDGE('',*,*,#13926,.T.);
#19273=ORIENTED_EDGE('',*,*,#13589,.T.);
#19274=ORIENTED_EDGE('',*,*,#12715,.F.);
#19275=ORIENTED_EDGE('',*,*,#12717,.T.);
#19276=ORIENTED_EDGE('',*,*,#12708,.F.);
#19277=ORIENTED_EDGE('',*,*,#12712,.T.);
#19278=ORIENTED_EDGE('',*,*,#13924,.T.);
#19279=ORIENTED_EDGE('',*,*,#13592,.T.);
#19280=ORIENTED_EDGE('',*,*,#12728,.F.);
#19281=ORIENTED_EDGE('',*,*,#12730,.T.);
#19282=ORIENTED_EDGE('',*,*,#12721,.F.);
#19283=ORIENTED_EDGE('',*,*,#12725,.T.);
#19284=ORIENTED_EDGE('',*,*,#13922,.T.);
#19285=ORIENTED_EDGE('',*,*,#13595,.T.);
#19286=ORIENTED_EDGE('',*,*,#12741,.F.);
#19287=ORIENTED_EDGE('',*,*,#12743,.T.);
#19288=ORIENTED_EDGE('',*,*,#12734,.F.);
#19289=ORIENTED_EDGE('',*,*,#12738,.T.);
#19290=ORIENTED_EDGE('',*,*,#13920,.T.);
#19291=ORIENTED_EDGE('',*,*,#13598,.T.);
#19292=ORIENTED_EDGE('',*,*,#12754,.F.);
#19293=ORIENTED_EDGE('',*,*,#12756,.T.);
#19294=ORIENTED_EDGE('',*,*,#12747,.F.);
#19295=ORIENTED_EDGE('',*,*,#12751,.T.);
#19296=ORIENTED_EDGE('',*,*,#13918,.T.);
#19297=ORIENTED_EDGE('',*,*,#13601,.T.);
#19298=ORIENTED_EDGE('',*,*,#12767,.F.);
#19299=ORIENTED_EDGE('',*,*,#12769,.T.);
#19300=ORIENTED_EDGE('',*,*,#12760,.F.);
#19301=ORIENTED_EDGE('',*,*,#12764,.T.);
#19302=ORIENTED_EDGE('',*,*,#13916,.T.);
#19303=ORIENTED_EDGE('',*,*,#13604,.T.);
#19304=ORIENTED_EDGE('',*,*,#12780,.F.);
#19305=ORIENTED_EDGE('',*,*,#12782,.T.);
#19306=ORIENTED_EDGE('',*,*,#12773,.F.);
#19307=ORIENTED_EDGE('',*,*,#12777,.T.);
#19308=ORIENTED_EDGE('',*,*,#13914,.T.);
#19309=ORIENTED_EDGE('',*,*,#13607,.T.);
#19310=ORIENTED_EDGE('',*,*,#12793,.F.);
#19311=ORIENTED_EDGE('',*,*,#12795,.T.);
#19312=ORIENTED_EDGE('',*,*,#12786,.F.);
#19313=ORIENTED_EDGE('',*,*,#12790,.T.);
#19314=ORIENTED_EDGE('',*,*,#13912,.T.);
#19315=ORIENTED_EDGE('',*,*,#13610,.T.);
#19316=ORIENTED_EDGE('',*,*,#12806,.F.);
#19317=ORIENTED_EDGE('',*,*,#12808,.T.);
#19318=ORIENTED_EDGE('',*,*,#12799,.F.);
#19319=ORIENTED_EDGE('',*,*,#12803,.T.);
#19320=ORIENTED_EDGE('',*,*,#13910,.T.);
#19321=ORIENTED_EDGE('',*,*,#13613,.T.);
#19322=ORIENTED_EDGE('',*,*,#12819,.F.);
#19323=ORIENTED_EDGE('',*,*,#12821,.T.);
#19324=ORIENTED_EDGE('',*,*,#12812,.F.);
#19325=ORIENTED_EDGE('',*,*,#12816,.T.);
#19326=ORIENTED_EDGE('',*,*,#13908,.T.);
#19327=ORIENTED_EDGE('',*,*,#13616,.T.);
#19328=ORIENTED_EDGE('',*,*,#12832,.F.);
#19329=ORIENTED_EDGE('',*,*,#12834,.T.);
#19330=ORIENTED_EDGE('',*,*,#12825,.F.);
#19331=ORIENTED_EDGE('',*,*,#12829,.T.);
#19332=ORIENTED_EDGE('',*,*,#13906,.T.);
#19333=ORIENTED_EDGE('',*,*,#13619,.T.);
#19334=ORIENTED_EDGE('',*,*,#12845,.F.);
#19335=ORIENTED_EDGE('',*,*,#12847,.T.);
#19336=ORIENTED_EDGE('',*,*,#12838,.F.);
#19337=ORIENTED_EDGE('',*,*,#12842,.T.);
#19338=ORIENTED_EDGE('',*,*,#13904,.T.);
#19339=ORIENTED_EDGE('',*,*,#13622,.T.);
#19340=ORIENTED_EDGE('',*,*,#12858,.F.);
#19341=ORIENTED_EDGE('',*,*,#12860,.T.);
#19342=ORIENTED_EDGE('',*,*,#12851,.F.);
#19343=ORIENTED_EDGE('',*,*,#12855,.T.);
#19344=ORIENTED_EDGE('',*,*,#13902,.T.);
#19345=ORIENTED_EDGE('',*,*,#13625,.T.);
#19346=ORIENTED_EDGE('',*,*,#12871,.F.);
#19347=ORIENTED_EDGE('',*,*,#12873,.T.);
#19348=ORIENTED_EDGE('',*,*,#12864,.F.);
#19349=ORIENTED_EDGE('',*,*,#12868,.T.);
#19350=ORIENTED_EDGE('',*,*,#13900,.T.);
#19351=ORIENTED_EDGE('',*,*,#13628,.T.);
#19352=ORIENTED_EDGE('',*,*,#12884,.F.);
#19353=ORIENTED_EDGE('',*,*,#12886,.T.);
#19354=ORIENTED_EDGE('',*,*,#12877,.F.);
#19355=ORIENTED_EDGE('',*,*,#12881,.T.);
#19356=ORIENTED_EDGE('',*,*,#13898,.T.);
#19357=ORIENTED_EDGE('',*,*,#13631,.T.);
#19358=ORIENTED_EDGE('',*,*,#12897,.F.);
#19359=ORIENTED_EDGE('',*,*,#12899,.T.);
#19360=ORIENTED_EDGE('',*,*,#12890,.F.);
#19361=ORIENTED_EDGE('',*,*,#12894,.T.);
#19362=ORIENTED_EDGE('',*,*,#13896,.T.);
#19363=ORIENTED_EDGE('',*,*,#13634,.T.);
#19364=ORIENTED_EDGE('',*,*,#12910,.F.);
#19365=ORIENTED_EDGE('',*,*,#12912,.T.);
#19366=ORIENTED_EDGE('',*,*,#12903,.F.);
#19367=ORIENTED_EDGE('',*,*,#12907,.T.);
#19368=ORIENTED_EDGE('',*,*,#13894,.T.);
#19369=ORIENTED_EDGE('',*,*,#13637,.T.);
#19370=ORIENTED_EDGE('',*,*,#12923,.F.);
#19371=ORIENTED_EDGE('',*,*,#12925,.T.);
#19372=ORIENTED_EDGE('',*,*,#12916,.F.);
#19373=ORIENTED_EDGE('',*,*,#12920,.T.);
#19374=ORIENTED_EDGE('',*,*,#13892,.T.);
#19375=ORIENTED_EDGE('',*,*,#13640,.T.);
#19376=ORIENTED_EDGE('',*,*,#12936,.F.);
#19377=ORIENTED_EDGE('',*,*,#12938,.T.);
#19378=ORIENTED_EDGE('',*,*,#12929,.F.);
#19379=ORIENTED_EDGE('',*,*,#12933,.T.);
#19380=ORIENTED_EDGE('',*,*,#13890,.T.);
#19381=ORIENTED_EDGE('',*,*,#13643,.T.);
#19382=ORIENTED_EDGE('',*,*,#12949,.F.);
#19383=ORIENTED_EDGE('',*,*,#12951,.T.);
#19384=ORIENTED_EDGE('',*,*,#12942,.F.);
#19385=ORIENTED_EDGE('',*,*,#12946,.T.);
#19386=ORIENTED_EDGE('',*,*,#13888,.T.);
#19387=ORIENTED_EDGE('',*,*,#13646,.T.);
#19388=ORIENTED_EDGE('',*,*,#12962,.F.);
#19389=ORIENTED_EDGE('',*,*,#12964,.T.);
#19390=ORIENTED_EDGE('',*,*,#12955,.F.);
#19391=ORIENTED_EDGE('',*,*,#12959,.T.);
#19392=ORIENTED_EDGE('',*,*,#13886,.T.);
#19393=ORIENTED_EDGE('',*,*,#13649,.T.);
#19394=ORIENTED_EDGE('',*,*,#12975,.F.);
#19395=ORIENTED_EDGE('',*,*,#12977,.T.);
#19396=ORIENTED_EDGE('',*,*,#12968,.F.);
#19397=ORIENTED_EDGE('',*,*,#12972,.T.);
#19398=ORIENTED_EDGE('',*,*,#13884,.T.);
#19399=ORIENTED_EDGE('',*,*,#13652,.T.);
#19400=ORIENTED_EDGE('',*,*,#12988,.F.);
#19401=ORIENTED_EDGE('',*,*,#12990,.T.);
#19402=ORIENTED_EDGE('',*,*,#12981,.F.);
#19403=ORIENTED_EDGE('',*,*,#12985,.T.);
#19404=ORIENTED_EDGE('',*,*,#13882,.T.);
#19405=ORIENTED_EDGE('',*,*,#13655,.T.);
#19406=ORIENTED_EDGE('',*,*,#13001,.F.);
#19407=ORIENTED_EDGE('',*,*,#13003,.T.);
#19408=ORIENTED_EDGE('',*,*,#12994,.F.);
#19409=ORIENTED_EDGE('',*,*,#12998,.T.);
#19410=ORIENTED_EDGE('',*,*,#13880,.T.);
#19411=ORIENTED_EDGE('',*,*,#13658,.T.);
#19412=ORIENTED_EDGE('',*,*,#13014,.F.);
#19413=ORIENTED_EDGE('',*,*,#13016,.T.);
#19414=ORIENTED_EDGE('',*,*,#13007,.F.);
#19415=ORIENTED_EDGE('',*,*,#13011,.T.);
#19416=ORIENTED_EDGE('',*,*,#13878,.T.);
#19417=ORIENTED_EDGE('',*,*,#13661,.T.);
#19418=ORIENTED_EDGE('',*,*,#13027,.F.);
#19419=ORIENTED_EDGE('',*,*,#13029,.T.);
#19420=ORIENTED_EDGE('',*,*,#13020,.F.);
#19421=ORIENTED_EDGE('',*,*,#13024,.T.);
#19422=ORIENTED_EDGE('',*,*,#13876,.T.);
#19423=ORIENTED_EDGE('',*,*,#13664,.T.);
#19424=ORIENTED_EDGE('',*,*,#13040,.F.);
#19425=ORIENTED_EDGE('',*,*,#13042,.T.);
#19426=ORIENTED_EDGE('',*,*,#13033,.F.);
#19427=ORIENTED_EDGE('',*,*,#13037,.T.);
#19428=ORIENTED_EDGE('',*,*,#13874,.T.);
#19429=ORIENTED_EDGE('',*,*,#13667,.T.);
#19430=ORIENTED_EDGE('',*,*,#13053,.F.);
#19431=ORIENTED_EDGE('',*,*,#13055,.T.);
#19432=ORIENTED_EDGE('',*,*,#13046,.F.);
#19433=ORIENTED_EDGE('',*,*,#13050,.T.);
#19434=ORIENTED_EDGE('',*,*,#13872,.T.);
#19435=ORIENTED_EDGE('',*,*,#13670,.T.);
#19436=ORIENTED_EDGE('',*,*,#13066,.F.);
#19437=ORIENTED_EDGE('',*,*,#13068,.T.);
#19438=ORIENTED_EDGE('',*,*,#13059,.F.);
#19439=ORIENTED_EDGE('',*,*,#13063,.T.);
#19440=ORIENTED_EDGE('',*,*,#13870,.T.);
#19441=ORIENTED_EDGE('',*,*,#13673,.T.);
#19442=ORIENTED_EDGE('',*,*,#13079,.F.);
#19443=ORIENTED_EDGE('',*,*,#13081,.T.);
#19444=ORIENTED_EDGE('',*,*,#13072,.F.);
#19445=ORIENTED_EDGE('',*,*,#13076,.T.);
#19446=ORIENTED_EDGE('',*,*,#13868,.T.);
#19447=ORIENTED_EDGE('',*,*,#13676,.T.);
#19448=ORIENTED_EDGE('',*,*,#13092,.F.);
#19449=ORIENTED_EDGE('',*,*,#13094,.T.);
#19450=ORIENTED_EDGE('',*,*,#13085,.F.);
#19451=ORIENTED_EDGE('',*,*,#13089,.T.);
#19452=ORIENTED_EDGE('',*,*,#13866,.T.);
#19453=ORIENTED_EDGE('',*,*,#13679,.T.);
#19454=ORIENTED_EDGE('',*,*,#13105,.F.);
#19455=ORIENTED_EDGE('',*,*,#13107,.T.);
#19456=ORIENTED_EDGE('',*,*,#13098,.F.);
#19457=ORIENTED_EDGE('',*,*,#13102,.T.);
#19458=ORIENTED_EDGE('',*,*,#13864,.T.);
#19459=ORIENTED_EDGE('',*,*,#13682,.T.);
#19460=ORIENTED_EDGE('',*,*,#13118,.F.);
#19461=ORIENTED_EDGE('',*,*,#13120,.T.);
#19462=ORIENTED_EDGE('',*,*,#13111,.F.);
#19463=ORIENTED_EDGE('',*,*,#13115,.T.);
#19464=ORIENTED_EDGE('',*,*,#13862,.T.);
#19465=ORIENTED_EDGE('',*,*,#13685,.T.);
#19466=ORIENTED_EDGE('',*,*,#13131,.F.);
#19467=ORIENTED_EDGE('',*,*,#13133,.T.);
#19468=ORIENTED_EDGE('',*,*,#13124,.F.);
#19469=ORIENTED_EDGE('',*,*,#13128,.T.);
#19470=ORIENTED_EDGE('',*,*,#13860,.T.);
#19471=ORIENTED_EDGE('',*,*,#13688,.T.);
#19472=ORIENTED_EDGE('',*,*,#13144,.F.);
#19473=ORIENTED_EDGE('',*,*,#13146,.T.);
#19474=ORIENTED_EDGE('',*,*,#13137,.F.);
#19475=ORIENTED_EDGE('',*,*,#13141,.T.);
#19476=ORIENTED_EDGE('',*,*,#13858,.T.);
#19477=ORIENTED_EDGE('',*,*,#13691,.T.);
#19478=ORIENTED_EDGE('',*,*,#13157,.F.);
#19479=ORIENTED_EDGE('',*,*,#13159,.T.);
#19480=ORIENTED_EDGE('',*,*,#13150,.F.);
#19481=ORIENTED_EDGE('',*,*,#13154,.T.);
#19482=ORIENTED_EDGE('',*,*,#13856,.T.);
#19483=ORIENTED_EDGE('',*,*,#13694,.T.);
#19484=ORIENTED_EDGE('',*,*,#13170,.F.);
#19485=ORIENTED_EDGE('',*,*,#13172,.T.);
#19486=ORIENTED_EDGE('',*,*,#13163,.F.);
#19487=ORIENTED_EDGE('',*,*,#13167,.T.);
#19488=ORIENTED_EDGE('',*,*,#13854,.T.);
#19489=ORIENTED_EDGE('',*,*,#13697,.T.);
#19490=ORIENTED_EDGE('',*,*,#13183,.F.);
#19491=ORIENTED_EDGE('',*,*,#13185,.T.);
#19492=ORIENTED_EDGE('',*,*,#13176,.F.);
#19493=ORIENTED_EDGE('',*,*,#13180,.T.);
#19494=ORIENTED_EDGE('',*,*,#13852,.T.);
#19495=ORIENTED_EDGE('',*,*,#13700,.T.);
#19496=ORIENTED_EDGE('',*,*,#13196,.F.);
#19497=ORIENTED_EDGE('',*,*,#13198,.T.);
#19498=ORIENTED_EDGE('',*,*,#13189,.F.);
#19499=ORIENTED_EDGE('',*,*,#13193,.T.);
#19500=ORIENTED_EDGE('',*,*,#13850,.T.);
#19501=ORIENTED_EDGE('',*,*,#13703,.T.);
#19502=ORIENTED_EDGE('',*,*,#13209,.F.);
#19503=ORIENTED_EDGE('',*,*,#13211,.T.);
#19504=ORIENTED_EDGE('',*,*,#13202,.F.);
#19505=ORIENTED_EDGE('',*,*,#13206,.T.);
#19506=ORIENTED_EDGE('',*,*,#13848,.T.);
#19507=ORIENTED_EDGE('',*,*,#13706,.T.);
#19508=ORIENTED_EDGE('',*,*,#13222,.F.);
#19509=ORIENTED_EDGE('',*,*,#13224,.T.);
#19510=ORIENTED_EDGE('',*,*,#13215,.F.);
#19511=ORIENTED_EDGE('',*,*,#13219,.T.);
#19512=ORIENTED_EDGE('',*,*,#13846,.T.);
#19513=ORIENTED_EDGE('',*,*,#13709,.T.);
#19514=ORIENTED_EDGE('',*,*,#13235,.F.);
#19515=ORIENTED_EDGE('',*,*,#13237,.T.);
#19516=ORIENTED_EDGE('',*,*,#13228,.F.);
#19517=ORIENTED_EDGE('',*,*,#13232,.T.);
#19518=ORIENTED_EDGE('',*,*,#13844,.T.);
#19519=ORIENTED_EDGE('',*,*,#13712,.T.);
#19520=ORIENTED_EDGE('',*,*,#13248,.F.);
#19521=ORIENTED_EDGE('',*,*,#13250,.T.);
#19522=ORIENTED_EDGE('',*,*,#13241,.F.);
#19523=ORIENTED_EDGE('',*,*,#13245,.T.);
#19524=ORIENTED_EDGE('',*,*,#13842,.T.);
#19525=ORIENTED_EDGE('',*,*,#13715,.T.);
#19526=ORIENTED_EDGE('',*,*,#13261,.F.);
#19527=ORIENTED_EDGE('',*,*,#13263,.T.);
#19528=ORIENTED_EDGE('',*,*,#13254,.F.);
#19529=ORIENTED_EDGE('',*,*,#13258,.T.);
#19530=ORIENTED_EDGE('',*,*,#13840,.T.);
#19531=ORIENTED_EDGE('',*,*,#13718,.T.);
#19532=ORIENTED_EDGE('',*,*,#13274,.F.);
#19533=ORIENTED_EDGE('',*,*,#13276,.T.);
#19534=ORIENTED_EDGE('',*,*,#13267,.F.);
#19535=ORIENTED_EDGE('',*,*,#13271,.T.);
#19536=ORIENTED_EDGE('',*,*,#13838,.T.);
#19537=ORIENTED_EDGE('',*,*,#13721,.T.);
#19538=ORIENTED_EDGE('',*,*,#13287,.F.);
#19539=ORIENTED_EDGE('',*,*,#13289,.T.);
#19540=ORIENTED_EDGE('',*,*,#13280,.F.);
#19541=ORIENTED_EDGE('',*,*,#13284,.T.);
#19542=ORIENTED_EDGE('',*,*,#13836,.T.);
#19543=ORIENTED_EDGE('',*,*,#13724,.T.);
#19544=ORIENTED_EDGE('',*,*,#13300,.F.);
#19545=ORIENTED_EDGE('',*,*,#13302,.T.);
#19546=ORIENTED_EDGE('',*,*,#13293,.F.);
#19547=ORIENTED_EDGE('',*,*,#13297,.T.);
#19548=ORIENTED_EDGE('',*,*,#13834,.T.);
#19549=ORIENTED_EDGE('',*,*,#13727,.T.);
#19550=ORIENTED_EDGE('',*,*,#13313,.F.);
#19551=ORIENTED_EDGE('',*,*,#13315,.T.);
#19552=ORIENTED_EDGE('',*,*,#13306,.F.);
#19553=ORIENTED_EDGE('',*,*,#13310,.T.);
#19554=ORIENTED_EDGE('',*,*,#13832,.T.);
#19555=ORIENTED_EDGE('',*,*,#13730,.T.);
#19556=ORIENTED_EDGE('',*,*,#13326,.F.);
#19557=ORIENTED_EDGE('',*,*,#13328,.T.);
#19558=ORIENTED_EDGE('',*,*,#13319,.F.);
#19559=ORIENTED_EDGE('',*,*,#13323,.T.);
#19560=ORIENTED_EDGE('',*,*,#13830,.T.);
#19561=ORIENTED_EDGE('',*,*,#13733,.T.);
#19562=ORIENTED_EDGE('',*,*,#13339,.F.);
#19563=ORIENTED_EDGE('',*,*,#13341,.T.);
#19564=ORIENTED_EDGE('',*,*,#13332,.F.);
#19565=ORIENTED_EDGE('',*,*,#13336,.T.);
#19566=ORIENTED_EDGE('',*,*,#13828,.T.);
#19567=ORIENTED_EDGE('',*,*,#13736,.T.);
#19568=ORIENTED_EDGE('',*,*,#13352,.F.);
#19569=ORIENTED_EDGE('',*,*,#13354,.T.);
#19570=ORIENTED_EDGE('',*,*,#13345,.F.);
#19571=ORIENTED_EDGE('',*,*,#13349,.T.);
#19572=ORIENTED_EDGE('',*,*,#13826,.T.);
#19573=ORIENTED_EDGE('',*,*,#13739,.T.);
#19574=ORIENTED_EDGE('',*,*,#13365,.F.);
#19575=ORIENTED_EDGE('',*,*,#13367,.T.);
#19576=ORIENTED_EDGE('',*,*,#13358,.F.);
#19577=ORIENTED_EDGE('',*,*,#13362,.T.);
#19578=ORIENTED_EDGE('',*,*,#13824,.T.);
#19579=ORIENTED_EDGE('',*,*,#13742,.T.);
#19580=ORIENTED_EDGE('',*,*,#13378,.F.);
#19581=ORIENTED_EDGE('',*,*,#13380,.T.);
#19582=ORIENTED_EDGE('',*,*,#13371,.F.);
#19583=ORIENTED_EDGE('',*,*,#13375,.T.);
#19584=ORIENTED_EDGE('',*,*,#13822,.T.);
#19585=ORIENTED_EDGE('',*,*,#13745,.T.);
#19586=ORIENTED_EDGE('',*,*,#13391,.F.);
#19587=ORIENTED_EDGE('',*,*,#13393,.T.);
#19588=ORIENTED_EDGE('',*,*,#13384,.F.);
#19589=ORIENTED_EDGE('',*,*,#13388,.T.);
#19590=ORIENTED_EDGE('',*,*,#13820,.T.);
#19591=ORIENTED_EDGE('',*,*,#13748,.T.);
#19592=ORIENTED_EDGE('',*,*,#13404,.F.);
#19593=ORIENTED_EDGE('',*,*,#13406,.T.);
#19594=ORIENTED_EDGE('',*,*,#13397,.F.);
#19595=ORIENTED_EDGE('',*,*,#13401,.T.);
#19596=ORIENTED_EDGE('',*,*,#13818,.T.);
#19597=ORIENTED_EDGE('',*,*,#13751,.T.);
#19598=ORIENTED_EDGE('',*,*,#13417,.F.);
#19599=ORIENTED_EDGE('',*,*,#13419,.T.);
#19600=ORIENTED_EDGE('',*,*,#13410,.F.);
#19601=ORIENTED_EDGE('',*,*,#13414,.T.);
#19602=ORIENTED_EDGE('',*,*,#13816,.T.);
#19603=ORIENTED_EDGE('',*,*,#13754,.T.);
#19604=ORIENTED_EDGE('',*,*,#13430,.F.);
#19605=ORIENTED_EDGE('',*,*,#13432,.T.);
#19606=ORIENTED_EDGE('',*,*,#13423,.F.);
#19607=ORIENTED_EDGE('',*,*,#13427,.T.);
#19608=ORIENTED_EDGE('',*,*,#13814,.T.);
#19609=ORIENTED_EDGE('',*,*,#13757,.T.);
#19610=ORIENTED_EDGE('',*,*,#13443,.F.);
#19611=ORIENTED_EDGE('',*,*,#13445,.T.);
#19612=ORIENTED_EDGE('',*,*,#13436,.F.);
#19613=ORIENTED_EDGE('',*,*,#13440,.T.);
#19614=ORIENTED_EDGE('',*,*,#13812,.T.);
#19615=ORIENTED_EDGE('',*,*,#13760,.T.);
#19616=ORIENTED_EDGE('',*,*,#13456,.F.);
#19617=ORIENTED_EDGE('',*,*,#13458,.T.);
#19618=ORIENTED_EDGE('',*,*,#13449,.F.);
#19619=ORIENTED_EDGE('',*,*,#13453,.T.);
#19620=ORIENTED_EDGE('',*,*,#13810,.T.);
#19621=ORIENTED_EDGE('',*,*,#13763,.T.);
#19622=ORIENTED_EDGE('',*,*,#13469,.F.);
#19623=ORIENTED_EDGE('',*,*,#13471,.T.);
#19624=ORIENTED_EDGE('',*,*,#13462,.F.);
#19625=ORIENTED_EDGE('',*,*,#13466,.T.);
#19626=ORIENTED_EDGE('',*,*,#13808,.T.);
#19627=ORIENTED_EDGE('',*,*,#13766,.T.);
#19628=ORIENTED_EDGE('',*,*,#13482,.F.);
#19629=ORIENTED_EDGE('',*,*,#13484,.T.);
#19630=ORIENTED_EDGE('',*,*,#13475,.F.);
#19631=ORIENTED_EDGE('',*,*,#13479,.T.);
#19632=ORIENTED_EDGE('',*,*,#13806,.T.);
#19633=ORIENTED_EDGE('',*,*,#13769,.T.);
#19634=ORIENTED_EDGE('',*,*,#13495,.F.);
#19635=ORIENTED_EDGE('',*,*,#13497,.T.);
#19636=ORIENTED_EDGE('',*,*,#13488,.F.);
#19637=ORIENTED_EDGE('',*,*,#13492,.T.);
#19638=ORIENTED_EDGE('',*,*,#13804,.T.);
#19639=ORIENTED_EDGE('',*,*,#13772,.T.);
#19640=ORIENTED_EDGE('',*,*,#13508,.F.);
#19641=ORIENTED_EDGE('',*,*,#13510,.T.);
#19642=ORIENTED_EDGE('',*,*,#13501,.F.);
#19643=ORIENTED_EDGE('',*,*,#13505,.T.);
#19644=ORIENTED_EDGE('',*,*,#13802,.T.);
#19645=ORIENTED_EDGE('',*,*,#13775,.T.);
#19646=ORIENTED_EDGE('',*,*,#13521,.F.);
#19647=ORIENTED_EDGE('',*,*,#13523,.T.);
#19648=ORIENTED_EDGE('',*,*,#13514,.F.);
#19649=ORIENTED_EDGE('',*,*,#13518,.T.);
#19650=ORIENTED_EDGE('',*,*,#13800,.T.);
#19651=ORIENTED_EDGE('',*,*,#13778,.T.);
#19652=ORIENTED_EDGE('',*,*,#13534,.F.);
#19653=ORIENTED_EDGE('',*,*,#13536,.T.);
#19654=ORIENTED_EDGE('',*,*,#13527,.F.);
#19655=ORIENTED_EDGE('',*,*,#13531,.T.);
#19656=ORIENTED_EDGE('',*,*,#13798,.T.);
#19657=ORIENTED_EDGE('',*,*,#13781,.T.);
#19658=ORIENTED_EDGE('',*,*,#13547,.F.);
#19659=ORIENTED_EDGE('',*,*,#13549,.T.);
#19660=ORIENTED_EDGE('',*,*,#13540,.F.);
#19661=ORIENTED_EDGE('',*,*,#13544,.T.);
#19662=ORIENTED_EDGE('',*,*,#13796,.T.);
#19663=ORIENTED_EDGE('',*,*,#13784,.T.);
#19664=ORIENTED_EDGE('',*,*,#13560,.F.);
#19665=ORIENTED_EDGE('',*,*,#13562,.T.);
#19666=ORIENTED_EDGE('',*,*,#13553,.F.);
#19667=ORIENTED_EDGE('',*,*,#13557,.T.);
#19668=ORIENTED_EDGE('',*,*,#13794,.T.);
#19669=ORIENTED_EDGE('',*,*,#13787,.T.);
#19670=ORIENTED_EDGE('',*,*,#13573,.F.);
#19671=ORIENTED_EDGE('',*,*,#13575,.T.);
#19672=ORIENTED_EDGE('',*,*,#13566,.F.);
#19673=ORIENTED_EDGE('',*,*,#13570,.T.);
#19674=ORIENTED_EDGE('',*,*,#13792,.T.);
#19675=ORIENTED_EDGE('',*,*,#13946,.T.);
#19676=ORIENTED_EDGE('',*,*,#13942,.F.);
#19677=ORIENTED_EDGE('',*,*,#13944,.T.);
#19678=ORIENTED_EDGE('',*,*,#13936,.F.);
#19679=ORIENTED_EDGE('',*,*,#13939,.T.);
#19680=ORIENTED_EDGE('',*,*,#13931,.T.);
#19681=ORIENTED_EDGE('',*,*,#13577,.T.);
#19682=ORIENTED_EDGE('',*,*,#12663,.F.);
#19683=ORIENTED_EDGE('',*,*,#12665,.T.);
#19684=ORIENTED_EDGE('',*,*,#12656,.F.);
#19685=ORIENTED_EDGE('',*,*,#12659,.T.);
#19686=ORIENTED_EDGE('',*,*,#13950,.T.);
#19687=ORIENTED_EDGE('',*,*,#13581,.T.);
#19688=ORIENTED_EDGE('',*,*,#13949,.F.);
#19689=ORIENTED_EDGE('',*,*,#13948,.F.);
#19690=ORIENTED_EDGE('',*,*,#13951,.T.);
#19691=ORIENTED_EDGE('',*,*,#12644,.T.);
#19692=ORIENTED_EDGE('',*,*,#13952,.T.);
#19693=ORIENTED_EDGE('',*,*,#13953,.T.);
#19694=ORIENTED_EDGE('',*,*,#13952,.F.);
#19695=ORIENTED_EDGE('',*,*,#12648,.T.);
#19696=ORIENTED_EDGE('',*,*,#12645,.T.);
#19697=ORIENTED_EDGE('',*,*,#13951,.F.);
#19698=ORIENTED_EDGE('',*,*,#12636,.T.);
#19699=ORIENTED_EDGE('',*,*,#12639,.T.);
#19700=ORIENTED_EDGE('',*,*,#12640,.T.);
#19701=ORIENTED_EDGE('',*,*,#12641,.T.);
#19702=ORIENTED_EDGE('',*,*,#12649,.T.);
#19703=ORIENTED_EDGE('',*,*,#12653,.T.);
#19704=ORIENTED_EDGE('',*,*,#12650,.T.);
#19705=ORIENTED_EDGE('',*,*,#13953,.F.);
#19706=ORIENTED_EDGE('',*,*,#12658,.T.);
#19707=ORIENTED_EDGE('',*,*,#12654,.F.);
#19708=ORIENTED_EDGE('',*,*,#12666,.T.);
#19709=ORIENTED_EDGE('',*,*,#12661,.F.);
#19710=ORIENTED_EDGE('',*,*,#13579,.T.);
#19711=ORIENTED_EDGE('',*,*,#13933,.F.);
#19712=ORIENTED_EDGE('',*,*,#13938,.T.);
#19713=ORIENTED_EDGE('',*,*,#13934,.F.);
#19714=ORIENTED_EDGE('',*,*,#13945,.T.);
#19715=ORIENTED_EDGE('',*,*,#13940,.F.);
#19716=ORIENTED_EDGE('',*,*,#13947,.T.);
#19717=ORIENTED_EDGE('',*,*,#13790,.F.);
#19718=ORIENTED_EDGE('',*,*,#13568,.T.);
#19719=ORIENTED_EDGE('',*,*,#13564,.F.);
#19720=ORIENTED_EDGE('',*,*,#13576,.T.);
#19721=ORIENTED_EDGE('',*,*,#13571,.F.);
#19722=ORIENTED_EDGE('',*,*,#13789,.T.);
#19723=ORIENTED_EDGE('',*,*,#13793,.F.);
#19724=ORIENTED_EDGE('',*,*,#13555,.T.);
#19725=ORIENTED_EDGE('',*,*,#13551,.F.);
#19726=ORIENTED_EDGE('',*,*,#13563,.T.);
#19727=ORIENTED_EDGE('',*,*,#13558,.F.);
#19728=ORIENTED_EDGE('',*,*,#13786,.T.);
#19729=ORIENTED_EDGE('',*,*,#13795,.F.);
#19730=ORIENTED_EDGE('',*,*,#13542,.T.);
#19731=ORIENTED_EDGE('',*,*,#13538,.F.);
#19732=ORIENTED_EDGE('',*,*,#13550,.T.);
#19733=ORIENTED_EDGE('',*,*,#13545,.F.);
#19734=ORIENTED_EDGE('',*,*,#13783,.T.);
#19735=ORIENTED_EDGE('',*,*,#13797,.F.);
#19736=ORIENTED_EDGE('',*,*,#13529,.T.);
#19737=ORIENTED_EDGE('',*,*,#13525,.F.);
#19738=ORIENTED_EDGE('',*,*,#13537,.T.);
#19739=ORIENTED_EDGE('',*,*,#13532,.F.);
#19740=ORIENTED_EDGE('',*,*,#13780,.T.);
#19741=ORIENTED_EDGE('',*,*,#13799,.F.);
#19742=ORIENTED_EDGE('',*,*,#13516,.T.);
#19743=ORIENTED_EDGE('',*,*,#13512,.F.);
#19744=ORIENTED_EDGE('',*,*,#13524,.T.);
#19745=ORIENTED_EDGE('',*,*,#13519,.F.);
#19746=ORIENTED_EDGE('',*,*,#13777,.T.);
#19747=ORIENTED_EDGE('',*,*,#13801,.F.);
#19748=ORIENTED_EDGE('',*,*,#13503,.T.);
#19749=ORIENTED_EDGE('',*,*,#13499,.F.);
#19750=ORIENTED_EDGE('',*,*,#13511,.T.);
#19751=ORIENTED_EDGE('',*,*,#13506,.F.);
#19752=ORIENTED_EDGE('',*,*,#13774,.T.);
#19753=ORIENTED_EDGE('',*,*,#13803,.F.);
#19754=ORIENTED_EDGE('',*,*,#13490,.T.);
#19755=ORIENTED_EDGE('',*,*,#13486,.F.);
#19756=ORIENTED_EDGE('',*,*,#13498,.T.);
#19757=ORIENTED_EDGE('',*,*,#13493,.F.);
#19758=ORIENTED_EDGE('',*,*,#13771,.T.);
#19759=ORIENTED_EDGE('',*,*,#13805,.F.);
#19760=ORIENTED_EDGE('',*,*,#13477,.T.);
#19761=ORIENTED_EDGE('',*,*,#13473,.F.);
#19762=ORIENTED_EDGE('',*,*,#13485,.T.);
#19763=ORIENTED_EDGE('',*,*,#13480,.F.);
#19764=ORIENTED_EDGE('',*,*,#13768,.T.);
#19765=ORIENTED_EDGE('',*,*,#13807,.F.);
#19766=ORIENTED_EDGE('',*,*,#13464,.T.);
#19767=ORIENTED_EDGE('',*,*,#13460,.F.);
#19768=ORIENTED_EDGE('',*,*,#13472,.T.);
#19769=ORIENTED_EDGE('',*,*,#13467,.F.);
#19770=ORIENTED_EDGE('',*,*,#13765,.T.);
#19771=ORIENTED_EDGE('',*,*,#13809,.F.);
#19772=ORIENTED_EDGE('',*,*,#13451,.T.);
#19773=ORIENTED_EDGE('',*,*,#13447,.F.);
#19774=ORIENTED_EDGE('',*,*,#13459,.T.);
#19775=ORIENTED_EDGE('',*,*,#13454,.F.);
#19776=ORIENTED_EDGE('',*,*,#13762,.T.);
#19777=ORIENTED_EDGE('',*,*,#13811,.F.);
#19778=ORIENTED_EDGE('',*,*,#13438,.T.);
#19779=ORIENTED_EDGE('',*,*,#13434,.F.);
#19780=ORIENTED_EDGE('',*,*,#13446,.T.);
#19781=ORIENTED_EDGE('',*,*,#13441,.F.);
#19782=ORIENTED_EDGE('',*,*,#13759,.T.);
#19783=ORIENTED_EDGE('',*,*,#13813,.F.);
#19784=ORIENTED_EDGE('',*,*,#13425,.T.);
#19785=ORIENTED_EDGE('',*,*,#13421,.F.);
#19786=ORIENTED_EDGE('',*,*,#13433,.T.);
#19787=ORIENTED_EDGE('',*,*,#13428,.F.);
#19788=ORIENTED_EDGE('',*,*,#13756,.T.);
#19789=ORIENTED_EDGE('',*,*,#13815,.F.);
#19790=ORIENTED_EDGE('',*,*,#13412,.T.);
#19791=ORIENTED_EDGE('',*,*,#13408,.F.);
#19792=ORIENTED_EDGE('',*,*,#13420,.T.);
#19793=ORIENTED_EDGE('',*,*,#13415,.F.);
#19794=ORIENTED_EDGE('',*,*,#13753,.T.);
#19795=ORIENTED_EDGE('',*,*,#13817,.F.);
#19796=ORIENTED_EDGE('',*,*,#13399,.T.);
#19797=ORIENTED_EDGE('',*,*,#13395,.F.);
#19798=ORIENTED_EDGE('',*,*,#13407,.T.);
#19799=ORIENTED_EDGE('',*,*,#13402,.F.);
#19800=ORIENTED_EDGE('',*,*,#13750,.T.);
#19801=ORIENTED_EDGE('',*,*,#13819,.F.);
#19802=ORIENTED_EDGE('',*,*,#13386,.T.);
#19803=ORIENTED_EDGE('',*,*,#13382,.F.);
#19804=ORIENTED_EDGE('',*,*,#13394,.T.);
#19805=ORIENTED_EDGE('',*,*,#13389,.F.);
#19806=ORIENTED_EDGE('',*,*,#13747,.T.);
#19807=ORIENTED_EDGE('',*,*,#13821,.F.);
#19808=ORIENTED_EDGE('',*,*,#13373,.T.);
#19809=ORIENTED_EDGE('',*,*,#13369,.F.);
#19810=ORIENTED_EDGE('',*,*,#13381,.T.);
#19811=ORIENTED_EDGE('',*,*,#13376,.F.);
#19812=ORIENTED_EDGE('',*,*,#13744,.T.);
#19813=ORIENTED_EDGE('',*,*,#13823,.F.);
#19814=ORIENTED_EDGE('',*,*,#13360,.T.);
#19815=ORIENTED_EDGE('',*,*,#13356,.F.);
#19816=ORIENTED_EDGE('',*,*,#13368,.T.);
#19817=ORIENTED_EDGE('',*,*,#13363,.F.);
#19818=ORIENTED_EDGE('',*,*,#13741,.T.);
#19819=ORIENTED_EDGE('',*,*,#13825,.F.);
#19820=ORIENTED_EDGE('',*,*,#13347,.T.);
#19821=ORIENTED_EDGE('',*,*,#13343,.F.);
#19822=ORIENTED_EDGE('',*,*,#13355,.T.);
#19823=ORIENTED_EDGE('',*,*,#13350,.F.);
#19824=ORIENTED_EDGE('',*,*,#13738,.T.);
#19825=ORIENTED_EDGE('',*,*,#13827,.F.);
#19826=ORIENTED_EDGE('',*,*,#13334,.T.);
#19827=ORIENTED_EDGE('',*,*,#13330,.F.);
#19828=ORIENTED_EDGE('',*,*,#13342,.T.);
#19829=ORIENTED_EDGE('',*,*,#13337,.F.);
#19830=ORIENTED_EDGE('',*,*,#13735,.T.);
#19831=ORIENTED_EDGE('',*,*,#13829,.F.);
#19832=ORIENTED_EDGE('',*,*,#13321,.T.);
#19833=ORIENTED_EDGE('',*,*,#13317,.F.);
#19834=ORIENTED_EDGE('',*,*,#13329,.T.);
#19835=ORIENTED_EDGE('',*,*,#13324,.F.);
#19836=ORIENTED_EDGE('',*,*,#13732,.T.);
#19837=ORIENTED_EDGE('',*,*,#13831,.F.);
#19838=ORIENTED_EDGE('',*,*,#13308,.T.);
#19839=ORIENTED_EDGE('',*,*,#13304,.F.);
#19840=ORIENTED_EDGE('',*,*,#13316,.T.);
#19841=ORIENTED_EDGE('',*,*,#13311,.F.);
#19842=ORIENTED_EDGE('',*,*,#13729,.T.);
#19843=ORIENTED_EDGE('',*,*,#13833,.F.);
#19844=ORIENTED_EDGE('',*,*,#13295,.T.);
#19845=ORIENTED_EDGE('',*,*,#13291,.F.);
#19846=ORIENTED_EDGE('',*,*,#13303,.T.);
#19847=ORIENTED_EDGE('',*,*,#13298,.F.);
#19848=ORIENTED_EDGE('',*,*,#13726,.T.);
#19849=ORIENTED_EDGE('',*,*,#13835,.F.);
#19850=ORIENTED_EDGE('',*,*,#13282,.T.);
#19851=ORIENTED_EDGE('',*,*,#13278,.F.);
#19852=ORIENTED_EDGE('',*,*,#13290,.T.);
#19853=ORIENTED_EDGE('',*,*,#13285,.F.);
#19854=ORIENTED_EDGE('',*,*,#13723,.T.);
#19855=ORIENTED_EDGE('',*,*,#13837,.F.);
#19856=ORIENTED_EDGE('',*,*,#13269,.T.);
#19857=ORIENTED_EDGE('',*,*,#13265,.F.);
#19858=ORIENTED_EDGE('',*,*,#13277,.T.);
#19859=ORIENTED_EDGE('',*,*,#13272,.F.);
#19860=ORIENTED_EDGE('',*,*,#13720,.T.);
#19861=ORIENTED_EDGE('',*,*,#13839,.F.);
#19862=ORIENTED_EDGE('',*,*,#13256,.T.);
#19863=ORIENTED_EDGE('',*,*,#13252,.F.);
#19864=ORIENTED_EDGE('',*,*,#13264,.T.);
#19865=ORIENTED_EDGE('',*,*,#13259,.F.);
#19866=ORIENTED_EDGE('',*,*,#13717,.T.);
#19867=ORIENTED_EDGE('',*,*,#13841,.F.);
#19868=ORIENTED_EDGE('',*,*,#13243,.T.);
#19869=ORIENTED_EDGE('',*,*,#13239,.F.);
#19870=ORIENTED_EDGE('',*,*,#13251,.T.);
#19871=ORIENTED_EDGE('',*,*,#13246,.F.);
#19872=ORIENTED_EDGE('',*,*,#13714,.T.);
#19873=ORIENTED_EDGE('',*,*,#13843,.F.);
#19874=ORIENTED_EDGE('',*,*,#13230,.T.);
#19875=ORIENTED_EDGE('',*,*,#13226,.F.);
#19876=ORIENTED_EDGE('',*,*,#13238,.T.);
#19877=ORIENTED_EDGE('',*,*,#13233,.F.);
#19878=ORIENTED_EDGE('',*,*,#13711,.T.);
#19879=ORIENTED_EDGE('',*,*,#13845,.F.);
#19880=ORIENTED_EDGE('',*,*,#13217,.T.);
#19881=ORIENTED_EDGE('',*,*,#13213,.F.);
#19882=ORIENTED_EDGE('',*,*,#13225,.T.);
#19883=ORIENTED_EDGE('',*,*,#13220,.F.);
#19884=ORIENTED_EDGE('',*,*,#13708,.T.);
#19885=ORIENTED_EDGE('',*,*,#13847,.F.);
#19886=ORIENTED_EDGE('',*,*,#13204,.T.);
#19887=ORIENTED_EDGE('',*,*,#13200,.F.);
#19888=ORIENTED_EDGE('',*,*,#13212,.T.);
#19889=ORIENTED_EDGE('',*,*,#13207,.F.);
#19890=ORIENTED_EDGE('',*,*,#13705,.T.);
#19891=ORIENTED_EDGE('',*,*,#13849,.F.);
#19892=ORIENTED_EDGE('',*,*,#13191,.T.);
#19893=ORIENTED_EDGE('',*,*,#13187,.F.);
#19894=ORIENTED_EDGE('',*,*,#13199,.T.);
#19895=ORIENTED_EDGE('',*,*,#13194,.F.);
#19896=ORIENTED_EDGE('',*,*,#13702,.T.);
#19897=ORIENTED_EDGE('',*,*,#13851,.F.);
#19898=ORIENTED_EDGE('',*,*,#13178,.T.);
#19899=ORIENTED_EDGE('',*,*,#13174,.F.);
#19900=ORIENTED_EDGE('',*,*,#13186,.T.);
#19901=ORIENTED_EDGE('',*,*,#13181,.F.);
#19902=ORIENTED_EDGE('',*,*,#13699,.T.);
#19903=ORIENTED_EDGE('',*,*,#13853,.F.);
#19904=ORIENTED_EDGE('',*,*,#13165,.T.);
#19905=ORIENTED_EDGE('',*,*,#13161,.F.);
#19906=ORIENTED_EDGE('',*,*,#13173,.T.);
#19907=ORIENTED_EDGE('',*,*,#13168,.F.);
#19908=ORIENTED_EDGE('',*,*,#13696,.T.);
#19909=ORIENTED_EDGE('',*,*,#13855,.F.);
#19910=ORIENTED_EDGE('',*,*,#13152,.T.);
#19911=ORIENTED_EDGE('',*,*,#13148,.F.);
#19912=ORIENTED_EDGE('',*,*,#13160,.T.);
#19913=ORIENTED_EDGE('',*,*,#13155,.F.);
#19914=ORIENTED_EDGE('',*,*,#13693,.T.);
#19915=ORIENTED_EDGE('',*,*,#13857,.F.);
#19916=ORIENTED_EDGE('',*,*,#13139,.T.);
#19917=ORIENTED_EDGE('',*,*,#13135,.F.);
#19918=ORIENTED_EDGE('',*,*,#13147,.T.);
#19919=ORIENTED_EDGE('',*,*,#13142,.F.);
#19920=ORIENTED_EDGE('',*,*,#13690,.T.);
#19921=ORIENTED_EDGE('',*,*,#13859,.F.);
#19922=ORIENTED_EDGE('',*,*,#13126,.T.);
#19923=ORIENTED_EDGE('',*,*,#13122,.F.);
#19924=ORIENTED_EDGE('',*,*,#13134,.T.);
#19925=ORIENTED_EDGE('',*,*,#13129,.F.);
#19926=ORIENTED_EDGE('',*,*,#13687,.T.);
#19927=ORIENTED_EDGE('',*,*,#13861,.F.);
#19928=ORIENTED_EDGE('',*,*,#13113,.T.);
#19929=ORIENTED_EDGE('',*,*,#13109,.F.);
#19930=ORIENTED_EDGE('',*,*,#13121,.T.);
#19931=ORIENTED_EDGE('',*,*,#13116,.F.);
#19932=ORIENTED_EDGE('',*,*,#13684,.T.);
#19933=ORIENTED_EDGE('',*,*,#13863,.F.);
#19934=ORIENTED_EDGE('',*,*,#13100,.T.);
#19935=ORIENTED_EDGE('',*,*,#13096,.F.);
#19936=ORIENTED_EDGE('',*,*,#13108,.T.);
#19937=ORIENTED_EDGE('',*,*,#13103,.F.);
#19938=ORIENTED_EDGE('',*,*,#13681,.T.);
#19939=ORIENTED_EDGE('',*,*,#13865,.F.);
#19940=ORIENTED_EDGE('',*,*,#13087,.T.);
#19941=ORIENTED_EDGE('',*,*,#13083,.F.);
#19942=ORIENTED_EDGE('',*,*,#13095,.T.);
#19943=ORIENTED_EDGE('',*,*,#13090,.F.);
#19944=ORIENTED_EDGE('',*,*,#13678,.T.);
#19945=ORIENTED_EDGE('',*,*,#13867,.F.);
#19946=ORIENTED_EDGE('',*,*,#13074,.T.);
#19947=ORIENTED_EDGE('',*,*,#13070,.F.);
#19948=ORIENTED_EDGE('',*,*,#13082,.T.);
#19949=ORIENTED_EDGE('',*,*,#13077,.F.);
#19950=ORIENTED_EDGE('',*,*,#13675,.T.);
#19951=ORIENTED_EDGE('',*,*,#13869,.F.);
#19952=ORIENTED_EDGE('',*,*,#13061,.T.);
#19953=ORIENTED_EDGE('',*,*,#13057,.F.);
#19954=ORIENTED_EDGE('',*,*,#13069,.T.);
#19955=ORIENTED_EDGE('',*,*,#13064,.F.);
#19956=ORIENTED_EDGE('',*,*,#13672,.T.);
#19957=ORIENTED_EDGE('',*,*,#13871,.F.);
#19958=ORIENTED_EDGE('',*,*,#13048,.T.);
#19959=ORIENTED_EDGE('',*,*,#13044,.F.);
#19960=ORIENTED_EDGE('',*,*,#13056,.T.);
#19961=ORIENTED_EDGE('',*,*,#13051,.F.);
#19962=ORIENTED_EDGE('',*,*,#13669,.T.);
#19963=ORIENTED_EDGE('',*,*,#13873,.F.);
#19964=ORIENTED_EDGE('',*,*,#13035,.T.);
#19965=ORIENTED_EDGE('',*,*,#13031,.F.);
#19966=ORIENTED_EDGE('',*,*,#13043,.T.);
#19967=ORIENTED_EDGE('',*,*,#13038,.F.);
#19968=ORIENTED_EDGE('',*,*,#13666,.T.);
#19969=ORIENTED_EDGE('',*,*,#13875,.F.);
#19970=ORIENTED_EDGE('',*,*,#13022,.T.);
#19971=ORIENTED_EDGE('',*,*,#13018,.F.);
#19972=ORIENTED_EDGE('',*,*,#13030,.T.);
#19973=ORIENTED_EDGE('',*,*,#13025,.F.);
#19974=ORIENTED_EDGE('',*,*,#13663,.T.);
#19975=ORIENTED_EDGE('',*,*,#13877,.F.);
#19976=ORIENTED_EDGE('',*,*,#13009,.T.);
#19977=ORIENTED_EDGE('',*,*,#13005,.F.);
#19978=ORIENTED_EDGE('',*,*,#13017,.T.);
#19979=ORIENTED_EDGE('',*,*,#13012,.F.);
#19980=ORIENTED_EDGE('',*,*,#13660,.T.);
#19981=ORIENTED_EDGE('',*,*,#13879,.F.);
#19982=ORIENTED_EDGE('',*,*,#12996,.T.);
#19983=ORIENTED_EDGE('',*,*,#12992,.F.);
#19984=ORIENTED_EDGE('',*,*,#13004,.T.);
#19985=ORIENTED_EDGE('',*,*,#12999,.F.);
#19986=ORIENTED_EDGE('',*,*,#13657,.T.);
#19987=ORIENTED_EDGE('',*,*,#13881,.F.);
#19988=ORIENTED_EDGE('',*,*,#12983,.T.);
#19989=ORIENTED_EDGE('',*,*,#12979,.F.);
#19990=ORIENTED_EDGE('',*,*,#12991,.T.);
#19991=ORIENTED_EDGE('',*,*,#12986,.F.);
#19992=ORIENTED_EDGE('',*,*,#13654,.T.);
#19993=ORIENTED_EDGE('',*,*,#13883,.F.);
#19994=ORIENTED_EDGE('',*,*,#12970,.T.);
#19995=ORIENTED_EDGE('',*,*,#12966,.F.);
#19996=ORIENTED_EDGE('',*,*,#12978,.T.);
#19997=ORIENTED_EDGE('',*,*,#12973,.F.);
#19998=ORIENTED_EDGE('',*,*,#13651,.T.);
#19999=ORIENTED_EDGE('',*,*,#13885,.F.);
#20000=ORIENTED_EDGE('',*,*,#12957,.T.);
#20001=ORIENTED_EDGE('',*,*,#12953,.F.);
#20002=ORIENTED_EDGE('',*,*,#12965,.T.);
#20003=ORIENTED_EDGE('',*,*,#12960,.F.);
#20004=ORIENTED_EDGE('',*,*,#13648,.T.);
#20005=ORIENTED_EDGE('',*,*,#13887,.F.);
#20006=ORIENTED_EDGE('',*,*,#12944,.T.);
#20007=ORIENTED_EDGE('',*,*,#12940,.F.);
#20008=ORIENTED_EDGE('',*,*,#12952,.T.);
#20009=ORIENTED_EDGE('',*,*,#12947,.F.);
#20010=ORIENTED_EDGE('',*,*,#13645,.T.);
#20011=ORIENTED_EDGE('',*,*,#13889,.F.);
#20012=ORIENTED_EDGE('',*,*,#12931,.T.);
#20013=ORIENTED_EDGE('',*,*,#12927,.F.);
#20014=ORIENTED_EDGE('',*,*,#12939,.T.);
#20015=ORIENTED_EDGE('',*,*,#12934,.F.);
#20016=ORIENTED_EDGE('',*,*,#13642,.T.);
#20017=ORIENTED_EDGE('',*,*,#13891,.F.);
#20018=ORIENTED_EDGE('',*,*,#12918,.T.);
#20019=ORIENTED_EDGE('',*,*,#12914,.F.);
#20020=ORIENTED_EDGE('',*,*,#12926,.T.);
#20021=ORIENTED_EDGE('',*,*,#12921,.F.);
#20022=ORIENTED_EDGE('',*,*,#13639,.T.);
#20023=ORIENTED_EDGE('',*,*,#13893,.F.);
#20024=ORIENTED_EDGE('',*,*,#12905,.T.);
#20025=ORIENTED_EDGE('',*,*,#12901,.F.);
#20026=ORIENTED_EDGE('',*,*,#12913,.T.);
#20027=ORIENTED_EDGE('',*,*,#12908,.F.);
#20028=ORIENTED_EDGE('',*,*,#13636,.T.);
#20029=ORIENTED_EDGE('',*,*,#13895,.F.);
#20030=ORIENTED_EDGE('',*,*,#12892,.T.);
#20031=ORIENTED_EDGE('',*,*,#12888,.F.);
#20032=ORIENTED_EDGE('',*,*,#12900,.T.);
#20033=ORIENTED_EDGE('',*,*,#12895,.F.);
#20034=ORIENTED_EDGE('',*,*,#13633,.T.);
#20035=ORIENTED_EDGE('',*,*,#13897,.F.);
#20036=ORIENTED_EDGE('',*,*,#12879,.T.);
#20037=ORIENTED_EDGE('',*,*,#12875,.F.);
#20038=ORIENTED_EDGE('',*,*,#12887,.T.);
#20039=ORIENTED_EDGE('',*,*,#12882,.F.);
#20040=ORIENTED_EDGE('',*,*,#13630,.T.);
#20041=ORIENTED_EDGE('',*,*,#13899,.F.);
#20042=ORIENTED_EDGE('',*,*,#12866,.T.);
#20043=ORIENTED_EDGE('',*,*,#12862,.F.);
#20044=ORIENTED_EDGE('',*,*,#12874,.T.);
#20045=ORIENTED_EDGE('',*,*,#12869,.F.);
#20046=ORIENTED_EDGE('',*,*,#13627,.T.);
#20047=ORIENTED_EDGE('',*,*,#13901,.F.);
#20048=ORIENTED_EDGE('',*,*,#12853,.T.);
#20049=ORIENTED_EDGE('',*,*,#12849,.F.);
#20050=ORIENTED_EDGE('',*,*,#12861,.T.);
#20051=ORIENTED_EDGE('',*,*,#12856,.F.);
#20052=ORIENTED_EDGE('',*,*,#13624,.T.);
#20053=ORIENTED_EDGE('',*,*,#13903,.F.);
#20054=ORIENTED_EDGE('',*,*,#12840,.T.);
#20055=ORIENTED_EDGE('',*,*,#12836,.F.);
#20056=ORIENTED_EDGE('',*,*,#12848,.T.);
#20057=ORIENTED_EDGE('',*,*,#12843,.F.);
#20058=ORIENTED_EDGE('',*,*,#13621,.T.);
#20059=ORIENTED_EDGE('',*,*,#13905,.F.);
#20060=ORIENTED_EDGE('',*,*,#12827,.T.);
#20061=ORIENTED_EDGE('',*,*,#12823,.F.);
#20062=ORIENTED_EDGE('',*,*,#12835,.T.);
#20063=ORIENTED_EDGE('',*,*,#12830,.F.);
#20064=ORIENTED_EDGE('',*,*,#13618,.T.);
#20065=ORIENTED_EDGE('',*,*,#13907,.F.);
#20066=ORIENTED_EDGE('',*,*,#12814,.T.);
#20067=ORIENTED_EDGE('',*,*,#12810,.F.);
#20068=ORIENTED_EDGE('',*,*,#12822,.T.);
#20069=ORIENTED_EDGE('',*,*,#12817,.F.);
#20070=ORIENTED_EDGE('',*,*,#13615,.T.);
#20071=ORIENTED_EDGE('',*,*,#13909,.F.);
#20072=ORIENTED_EDGE('',*,*,#12801,.T.);
#20073=ORIENTED_EDGE('',*,*,#12797,.F.);
#20074=ORIENTED_EDGE('',*,*,#12809,.T.);
#20075=ORIENTED_EDGE('',*,*,#12804,.F.);
#20076=ORIENTED_EDGE('',*,*,#13612,.T.);
#20077=ORIENTED_EDGE('',*,*,#13911,.F.);
#20078=ORIENTED_EDGE('',*,*,#12788,.T.);
#20079=ORIENTED_EDGE('',*,*,#12784,.F.);
#20080=ORIENTED_EDGE('',*,*,#12796,.T.);
#20081=ORIENTED_EDGE('',*,*,#12791,.F.);
#20082=ORIENTED_EDGE('',*,*,#13609,.T.);
#20083=ORIENTED_EDGE('',*,*,#13913,.F.);
#20084=ORIENTED_EDGE('',*,*,#12775,.T.);
#20085=ORIENTED_EDGE('',*,*,#12771,.F.);
#20086=ORIENTED_EDGE('',*,*,#12783,.T.);
#20087=ORIENTED_EDGE('',*,*,#12778,.F.);
#20088=ORIENTED_EDGE('',*,*,#13606,.T.);
#20089=ORIENTED_EDGE('',*,*,#13915,.F.);
#20090=ORIENTED_EDGE('',*,*,#12762,.T.);
#20091=ORIENTED_EDGE('',*,*,#12758,.F.);
#20092=ORIENTED_EDGE('',*,*,#12770,.T.);
#20093=ORIENTED_EDGE('',*,*,#12765,.F.);
#20094=ORIENTED_EDGE('',*,*,#13603,.T.);
#20095=ORIENTED_EDGE('',*,*,#13917,.F.);
#20096=ORIENTED_EDGE('',*,*,#12749,.T.);
#20097=ORIENTED_EDGE('',*,*,#12745,.F.);
#20098=ORIENTED_EDGE('',*,*,#12757,.T.);
#20099=ORIENTED_EDGE('',*,*,#12752,.F.);
#20100=ORIENTED_EDGE('',*,*,#13600,.T.);
#20101=ORIENTED_EDGE('',*,*,#13919,.F.);
#20102=ORIENTED_EDGE('',*,*,#12736,.T.);
#20103=ORIENTED_EDGE('',*,*,#12732,.F.);
#20104=ORIENTED_EDGE('',*,*,#12744,.T.);
#20105=ORIENTED_EDGE('',*,*,#12739,.F.);
#20106=ORIENTED_EDGE('',*,*,#13597,.T.);
#20107=ORIENTED_EDGE('',*,*,#13921,.F.);
#20108=ORIENTED_EDGE('',*,*,#12723,.T.);
#20109=ORIENTED_EDGE('',*,*,#12719,.F.);
#20110=ORIENTED_EDGE('',*,*,#12731,.T.);
#20111=ORIENTED_EDGE('',*,*,#12726,.F.);
#20112=ORIENTED_EDGE('',*,*,#13594,.T.);
#20113=ORIENTED_EDGE('',*,*,#13923,.F.);
#20114=ORIENTED_EDGE('',*,*,#12710,.T.);
#20115=ORIENTED_EDGE('',*,*,#12706,.F.);
#20116=ORIENTED_EDGE('',*,*,#12718,.T.);
#20117=ORIENTED_EDGE('',*,*,#12713,.F.);
#20118=ORIENTED_EDGE('',*,*,#13591,.T.);
#20119=ORIENTED_EDGE('',*,*,#13925,.F.);
#20120=ORIENTED_EDGE('',*,*,#12697,.T.);
#20121=ORIENTED_EDGE('',*,*,#12693,.F.);
#20122=ORIENTED_EDGE('',*,*,#12705,.T.);
#20123=ORIENTED_EDGE('',*,*,#12700,.F.);
#20124=ORIENTED_EDGE('',*,*,#13588,.T.);
#20125=ORIENTED_EDGE('',*,*,#13927,.F.);
#20126=ORIENTED_EDGE('',*,*,#12684,.T.);
#20127=ORIENTED_EDGE('',*,*,#12680,.F.);
#20128=ORIENTED_EDGE('',*,*,#12692,.T.);
#20129=ORIENTED_EDGE('',*,*,#12687,.F.);
#20130=ORIENTED_EDGE('',*,*,#13585,.T.);
#20131=ORIENTED_EDGE('',*,*,#13929,.F.);
#20132=ORIENTED_EDGE('',*,*,#12671,.T.);
#20133=ORIENTED_EDGE('',*,*,#12667,.F.);
#20134=ORIENTED_EDGE('',*,*,#12679,.T.);
#20135=ORIENTED_EDGE('',*,*,#12674,.F.);
#20136=ORIENTED_EDGE('',*,*,#13582,.T.);
#20137=ORIENTED_EDGE('',*,*,#13950,.F.);
#23382=CYLINDRICAL_SURFACE('',#25865,2.);
#23383=CYLINDRICAL_SURFACE('',#25868,2.);
#23384=CYLINDRICAL_SURFACE('',#25871,2.);
#23385=CYLINDRICAL_SURFACE('',#25874,2.);
#23386=CYLINDRICAL_SURFACE('',#25877,74.4999999996252);
#23387=CYLINDRICAL_SURFACE('',#25880,74.4999999996252);
#23388=CYLINDRICAL_SURFACE('',#25883,74.4999999996252);
#23389=CYLINDRICAL_SURFACE('',#25886,74.4999999996252);
#23390=CYLINDRICAL_SURFACE('',#25889,74.4999999996252);
#23391=CYLINDRICAL_SURFACE('',#25892,74.4999999996252);
#23392=CYLINDRICAL_SURFACE('',#25895,74.4999999996252);
#23393=CYLINDRICAL_SURFACE('',#25898,74.4999999996252);
#23394=CYLINDRICAL_SURFACE('',#25901,74.4999999996252);
#23395=CYLINDRICAL_SURFACE('',#25904,74.4999999996252);
#23396=CYLINDRICAL_SURFACE('',#25907,74.4999999996252);
#23397=CYLINDRICAL_SURFACE('',#25910,74.4999999996252);
#23398=CYLINDRICAL_SURFACE('',#25913,74.4999999996252);
#23399=CYLINDRICAL_SURFACE('',#25916,74.4999999996252);
#23400=CYLINDRICAL_SURFACE('',#25919,74.4999999996252);
#23401=CYLINDRICAL_SURFACE('',#25922,74.4999999996252);
#23402=CYLINDRICAL_SURFACE('',#25925,74.4999999996252);
#23403=CYLINDRICAL_SURFACE('',#25928,74.4999999996252);
#23404=CYLINDRICAL_SURFACE('',#25931,74.4999999996252);
#23405=CYLINDRICAL_SURFACE('',#25934,74.4999999996252);
#23406=CYLINDRICAL_SURFACE('',#25937,74.4999999996252);
#23407=CYLINDRICAL_SURFACE('',#25940,74.4999999996252);
#23408=CYLINDRICAL_SURFACE('',#25943,74.4999999996252);
#23409=CYLINDRICAL_SURFACE('',#25946,74.4999999996252);
#23410=CYLINDRICAL_SURFACE('',#25949,74.4999999996252);
#23411=CYLINDRICAL_SURFACE('',#25952,74.4999999996252);
#23412=CYLINDRICAL_SURFACE('',#25955,74.4999999996252);
#23413=CYLINDRICAL_SURFACE('',#25958,74.4999999996252);
#23414=CYLINDRICAL_SURFACE('',#25961,74.4999999996252);
#23415=CYLINDRICAL_SURFACE('',#25964,74.4999999996252);
#23416=CYLINDRICAL_SURFACE('',#25967,74.4999999996252);
#23417=CYLINDRICAL_SURFACE('',#25970,74.4999999996252);
#23418=CYLINDRICAL_SURFACE('',#25973,74.4999999996252);
#23419=CYLINDRICAL_SURFACE('',#25976,74.4999999996252);
#23420=CYLINDRICAL_SURFACE('',#25979,74.4999999996252);
#23421=CYLINDRICAL_SURFACE('',#25982,74.4999999996252);
#23422=CYLINDRICAL_SURFACE('',#25985,74.4999999996252);
#23423=CYLINDRICAL_SURFACE('',#25988,74.4999999996252);
#23424=CYLINDRICAL_SURFACE('',#25991,74.4999999996252);
#23425=CYLINDRICAL_SURFACE('',#25994,74.4999999996252);
#23426=CYLINDRICAL_SURFACE('',#25997,74.4999999996252);
#23427=CYLINDRICAL_SURFACE('',#26000,74.4999999996252);
#23428=CYLINDRICAL_SURFACE('',#26003,74.4999999996252);
#23429=CYLINDRICAL_SURFACE('',#26006,74.4999999996252);
#23430=CYLINDRICAL_SURFACE('',#26009,74.4999999996252);
#23431=CYLINDRICAL_SURFACE('',#26012,74.4999999996252);
#23432=CYLINDRICAL_SURFACE('',#26015,74.4999999996252);
#23433=CYLINDRICAL_SURFACE('',#26018,74.4999999996252);
#23434=CYLINDRICAL_SURFACE('',#26021,74.4999999996252);
#23435=CYLINDRICAL_SURFACE('',#26024,74.4999999996252);
#23436=CYLINDRICAL_SURFACE('',#26027,74.4999999996252);
#23437=CYLINDRICAL_SURFACE('',#26030,74.4999999996252);
#23438=CYLINDRICAL_SURFACE('',#26033,74.4999999996252);
#23439=CYLINDRICAL_SURFACE('',#26036,74.4999999996252);
#23440=CYLINDRICAL_SURFACE('',#26039,74.4999999996252);
#23441=CYLINDRICAL_SURFACE('',#26042,74.4999999996252);
#23442=CYLINDRICAL_SURFACE('',#26045,74.4999999996252);
#23443=CYLINDRICAL_SURFACE('',#26048,74.4999999996252);
#23444=CYLINDRICAL_SURFACE('',#26051,74.4999999996252);
#23445=CYLINDRICAL_SURFACE('',#26054,74.4999999996252);
#23446=CYLINDRICAL_SURFACE('',#26057,74.4999999996252);
#23447=CYLINDRICAL_SURFACE('',#26060,74.4999999996252);
#23448=CYLINDRICAL_SURFACE('',#26063,74.4999999996252);
#23449=CYLINDRICAL_SURFACE('',#26066,74.4999999996252);
#23450=CYLINDRICAL_SURFACE('',#26069,74.4999999996252);
#23451=CYLINDRICAL_SURFACE('',#26072,74.4999999996252);
#23452=CYLINDRICAL_SURFACE('',#26075,74.4999999996252);
#23453=CYLINDRICAL_SURFACE('',#26078,74.4999999996252);
#23454=CYLINDRICAL_SURFACE('',#26081,74.4999999996252);
#23455=CYLINDRICAL_SURFACE('',#26084,74.4999999996252);
#23456=CYLINDRICAL_SURFACE('',#26087,74.4999999996252);
#23457=CYLINDRICAL_SURFACE('',#26090,70.);
#23458=CYLINDRICAL_SURFACE('',#26093,70.);
#23459=CYLINDRICAL_SURFACE('',#26096,70.);
#23460=CYLINDRICAL_SURFACE('',#26099,70.);
#23461=CYLINDRICAL_SURFACE('',#26102,70.);
#23462=CYLINDRICAL_SURFACE('',#26105,70.);
#23463=CYLINDRICAL_SURFACE('',#26108,70.);
#23464=CYLINDRICAL_SURFACE('',#26111,70.);
#23465=CYLINDRICAL_SURFACE('',#26114,70.);
#23466=CYLINDRICAL_SURFACE('',#26117,70.);
#23467=CYLINDRICAL_SURFACE('',#26120,70.);
#23468=CYLINDRICAL_SURFACE('',#26123,70.);
#23469=CYLINDRICAL_SURFACE('',#26126,70.);
#23470=CYLINDRICAL_SURFACE('',#26129,70.);
#23471=CYLINDRICAL_SURFACE('',#26132,70.);
#23472=CYLINDRICAL_SURFACE('',#26135,70.);
#23473=CYLINDRICAL_SURFACE('',#26138,70.);
#23474=CYLINDRICAL_SURFACE('',#26141,70.);
#23475=CYLINDRICAL_SURFACE('',#26144,70.);
#23476=CYLINDRICAL_SURFACE('',#26147,70.);
#23477=CYLINDRICAL_SURFACE('',#26150,70.);
#23478=CYLINDRICAL_SURFACE('',#26153,70.);
#23479=CYLINDRICAL_SURFACE('',#26156,70.);
#23480=CYLINDRICAL_SURFACE('',#26159,70.);
#23481=CYLINDRICAL_SURFACE('',#26162,70.);
#23482=CYLINDRICAL_SURFACE('',#26165,70.);
#23483=CYLINDRICAL_SURFACE('',#26168,70.);
#23484=CYLINDRICAL_SURFACE('',#26171,70.);
#23485=CYLINDRICAL_SURFACE('',#26174,70.);
#23486=CYLINDRICAL_SURFACE('',#26177,70.);
#23487=CYLINDRICAL_SURFACE('',#26180,70.);
#23488=CYLINDRICAL_SURFACE('',#26183,70.);
#23489=CYLINDRICAL_SURFACE('',#26186,70.);
#23490=CYLINDRICAL_SURFACE('',#26189,70.);
#23491=CYLINDRICAL_SURFACE('',#26192,70.);
#23492=CYLINDRICAL_SURFACE('',#26195,70.);
#23493=CYLINDRICAL_SURFACE('',#26198,70.);
#23494=CYLINDRICAL_SURFACE('',#26201,70.);
#23495=CYLINDRICAL_SURFACE('',#26204,70.);
#23496=CYLINDRICAL_SURFACE('',#26207,70.);
#23497=CYLINDRICAL_SURFACE('',#26210,70.);
#23498=CYLINDRICAL_SURFACE('',#26213,70.);
#23499=CYLINDRICAL_SURFACE('',#26216,70.);
#23500=CYLINDRICAL_SURFACE('',#26219,70.);
#23501=CYLINDRICAL_SURFACE('',#26222,70.);
#23502=CYLINDRICAL_SURFACE('',#26225,70.);
#23503=CYLINDRICAL_SURFACE('',#26228,70.);
#23504=CYLINDRICAL_SURFACE('',#26231,70.);
#23505=CYLINDRICAL_SURFACE('',#26234,70.);
#23506=CYLINDRICAL_SURFACE('',#26237,70.);
#23507=CYLINDRICAL_SURFACE('',#26240,70.);
#23508=CYLINDRICAL_SURFACE('',#26243,70.);
#23509=CYLINDRICAL_SURFACE('',#26246,70.);
#23510=CYLINDRICAL_SURFACE('',#26249,70.);
#23511=CYLINDRICAL_SURFACE('',#26252,70.);
#23512=CYLINDRICAL_SURFACE('',#26255,70.);
#23513=CYLINDRICAL_SURFACE('',#26258,70.);
#23514=CYLINDRICAL_SURFACE('',#26261,70.);
#23515=CYLINDRICAL_SURFACE('',#26264,70.);
#23516=CYLINDRICAL_SURFACE('',#26267,70.);
#23517=CYLINDRICAL_SURFACE('',#26270,70.);
#23518=CYLINDRICAL_SURFACE('',#26273,70.);
#23519=CYLINDRICAL_SURFACE('',#26276,70.);
#23520=CYLINDRICAL_SURFACE('',#26279,70.);
#23521=CYLINDRICAL_SURFACE('',#26282,70.);
#23522=CYLINDRICAL_SURFACE('',#26285,70.);
#23523=CYLINDRICAL_SURFACE('',#26288,70.);
#23524=CYLINDRICAL_SURFACE('',#26291,70.);
#23525=CYLINDRICAL_SURFACE('',#26294,70.);
#23526=CYLINDRICAL_SURFACE('',#26297,70.);
#23527=CYLINDRICAL_SURFACE('',#26300,70.);
#23528=CYLINDRICAL_SURFACE('',#26303,74.4999999996252);
#23529=CYLINDRICAL_SURFACE('',#26309,70.);
#23530=CYLINDRICAL_SURFACE('',#26311,90.);
#24170=ADVANCED_FACE('',(#2064),#23382,.F.);
#24171=ADVANCED_FACE('',(#2065),#1526,.F.);
#24172=ADVANCED_FACE('',(#2066),#23383,.F.);
#24173=ADVANCED_FACE('',(#2067),#1527,.F.);
#24174=ADVANCED_FACE('',(#2068),#23384,.F.);
#24175=ADVANCED_FACE('',(#2069),#1528,.F.);
#24176=ADVANCED_FACE('',(#2070),#23385,.F.);
#24177=ADVANCED_FACE('',(#2071),#1529,.F.);
#24178=ADVANCED_FACE('',(#2072),#1334,.T.);
#24179=ADVANCED_FACE('',(#2073),#883,.F.);
#24180=ADVANCED_FACE('',(#2074),#1335,.T.);
#24181=ADVANCED_FACE('',(#2075),#23386,.F.);
#24182=ADVANCED_FACE('',(#2076),#1336,.T.);
#24183=ADVANCED_FACE('',(#2077),#884,.F.);
#24184=ADVANCED_FACE('',(#2078),#1337,.T.);
#24185=ADVANCED_FACE('',(#2079),#23387,.F.);
#24186=ADVANCED_FACE('',(#2080),#1338,.T.);
#24187=ADVANCED_FACE('',(#2081),#885,.F.);
#24188=ADVANCED_FACE('',(#2082),#1339,.T.);
#24189=ADVANCED_FACE('',(#2083),#23388,.F.);
#24190=ADVANCED_FACE('',(#2084),#1340,.T.);
#24191=ADVANCED_FACE('',(#2085),#886,.F.);
#24192=ADVANCED_FACE('',(#2086),#1341,.T.);
#24193=ADVANCED_FACE('',(#2087),#23389,.F.);
#24194=ADVANCED_FACE('',(#2088),#1342,.T.);
#24195=ADVANCED_FACE('',(#2089),#887,.F.);
#24196=ADVANCED_FACE('',(#2090),#1343,.T.);
#24197=ADVANCED_FACE('',(#2091),#23390,.F.);
#24198=ADVANCED_FACE('',(#2092),#1344,.T.);
#24199=ADVANCED_FACE('',(#2093),#888,.F.);
#24200=ADVANCED_FACE('',(#2094),#1345,.T.);
#24201=ADVANCED_FACE('',(#2095),#23391,.F.);
#24202=ADVANCED_FACE('',(#2096),#1346,.T.);
#24203=ADVANCED_FACE('',(#2097),#889,.F.);
#24204=ADVANCED_FACE('',(#2098),#1347,.T.);
#24205=ADVANCED_FACE('',(#2099),#23392,.F.);
#24206=ADVANCED_FACE('',(#2100),#1348,.T.);
#24207=ADVANCED_FACE('',(#2101),#890,.F.);
#24208=ADVANCED_FACE('',(#2102),#1349,.T.);
#24209=ADVANCED_FACE('',(#2103),#23393,.F.);
#24210=ADVANCED_FACE('',(#2104),#1350,.T.);
#24211=ADVANCED_FACE('',(#2105),#891,.F.);
#24212=ADVANCED_FACE('',(#2106),#1351,.T.);
#24213=ADVANCED_FACE('',(#2107),#23394,.F.);
#24214=ADVANCED_FACE('',(#2108),#1352,.T.);
#24215=ADVANCED_FACE('',(#2109),#892,.F.);
#24216=ADVANCED_FACE('',(#2110),#1353,.T.);
#24217=ADVANCED_FACE('',(#2111),#23395,.F.);
#24218=ADVANCED_FACE('',(#2112),#1354,.T.);
#24219=ADVANCED_FACE('',(#2113),#893,.F.);
#24220=ADVANCED_FACE('',(#2114),#1355,.T.);
#24221=ADVANCED_FACE('',(#2115),#23396,.F.);
#24222=ADVANCED_FACE('',(#2116),#1356,.T.);
#24223=ADVANCED_FACE('',(#2117),#894,.F.);
#24224=ADVANCED_FACE('',(#2118),#1357,.T.);
#24225=ADVANCED_FACE('',(#2119),#23397,.F.);
#24226=ADVANCED_FACE('',(#2120),#1358,.T.);
#24227=ADVANCED_FACE('',(#2121),#895,.F.);
#24228=ADVANCED_FACE('',(#2122),#1359,.T.);
#24229=ADVANCED_FACE('',(#2123),#23398,.F.);
#24230=ADVANCED_FACE('',(#2124),#1360,.T.);
#24231=ADVANCED_FACE('',(#2125),#896,.F.);
#24232=ADVANCED_FACE('',(#2126),#1361,.T.);
#24233=ADVANCED_FACE('',(#2127),#23399,.F.);
#24234=ADVANCED_FACE('',(#2128),#1362,.T.);
#24235=ADVANCED_FACE('',(#2129),#897,.F.);
#24236=ADVANCED_FACE('',(#2130),#1363,.T.);
#24237=ADVANCED_FACE('',(#2131),#23400,.F.);
#24238=ADVANCED_FACE('',(#2132),#1364,.T.);
#24239=ADVANCED_FACE('',(#2133),#898,.F.);
#24240=ADVANCED_FACE('',(#2134),#1365,.T.);
#24241=ADVANCED_FACE('',(#2135),#23401,.F.);
#24242=ADVANCED_FACE('',(#2136),#1366,.T.);
#24243=ADVANCED_FACE('',(#2137),#899,.F.);
#24244=ADVANCED_FACE('',(#2138),#1367,.T.);
#24245=ADVANCED_FACE('',(#2139),#23402,.F.);
#24246=ADVANCED_FACE('',(#2140),#1368,.T.);
#24247=ADVANCED_FACE('',(#2141),#900,.F.);
#24248=ADVANCED_FACE('',(#2142),#1369,.T.);
#24249=ADVANCED_FACE('',(#2143),#23403,.F.);
#24250=ADVANCED_FACE('',(#2144),#1370,.T.);
#24251=ADVANCED_FACE('',(#2145),#901,.F.);
#24252=ADVANCED_FACE('',(#2146),#1371,.T.);
#24253=ADVANCED_FACE('',(#2147),#23404,.F.);
#24254=ADVANCED_FACE('',(#2148),#1372,.T.);
#24255=ADVANCED_FACE('',(#2149),#902,.F.);
#24256=ADVANCED_FACE('',(#2150),#1373,.T.);
#24257=ADVANCED_FACE('',(#2151),#23405,.F.);
#24258=ADVANCED_FACE('',(#2152),#1374,.T.);
#24259=ADVANCED_FACE('',(#2153),#903,.F.);
#24260=ADVANCED_FACE('',(#2154),#1375,.T.);
#24261=ADVANCED_FACE('',(#2155),#23406,.F.);
#24262=ADVANCED_FACE('',(#2156),#1376,.T.);
#24263=ADVANCED_FACE('',(#2157),#904,.F.);
#24264=ADVANCED_FACE('',(#2158),#1377,.T.);
#24265=ADVANCED_FACE('',(#2159),#23407,.F.);
#24266=ADVANCED_FACE('',(#2160),#1378,.T.);
#24267=ADVANCED_FACE('',(#2161),#905,.F.);
#24268=ADVANCED_FACE('',(#2162),#1379,.T.);
#24269=ADVANCED_FACE('',(#2163),#23408,.F.);
#24270=ADVANCED_FACE('',(#2164),#1380,.T.);
#24271=ADVANCED_FACE('',(#2165),#906,.F.);
#24272=ADVANCED_FACE('',(#2166),#1381,.T.);
#24273=ADVANCED_FACE('',(#2167),#23409,.F.);
#24274=ADVANCED_FACE('',(#2168),#1382,.T.);
#24275=ADVANCED_FACE('',(#2169),#907,.F.);
#24276=ADVANCED_FACE('',(#2170),#1383,.T.);
#24277=ADVANCED_FACE('',(#2171),#23410,.F.);
#24278=ADVANCED_FACE('',(#2172),#1384,.T.);
#24279=ADVANCED_FACE('',(#2173),#908,.F.);
#24280=ADVANCED_FACE('',(#2174),#1385,.T.);
#24281=ADVANCED_FACE('',(#2175),#23411,.F.);
#24282=ADVANCED_FACE('',(#2176),#1386,.T.);
#24283=ADVANCED_FACE('',(#2177),#909,.F.);
#24284=ADVANCED_FACE('',(#2178),#1387,.T.);
#24285=ADVANCED_FACE('',(#2179),#23412,.F.);
#24286=ADVANCED_FACE('',(#2180),#1388,.T.);
#24287=ADVANCED_FACE('',(#2181),#910,.F.);
#24288=ADVANCED_FACE('',(#2182),#1389,.T.);
#24289=ADVANCED_FACE('',(#2183),#23413,.F.);
#24290=ADVANCED_FACE('',(#2184),#1390,.T.);
#24291=ADVANCED_FACE('',(#2185),#911,.F.);
#24292=ADVANCED_FACE('',(#2186),#1391,.T.);
#24293=ADVANCED_FACE('',(#2187),#23414,.F.);
#24294=ADVANCED_FACE('',(#2188),#1392,.T.);
#24295=ADVANCED_FACE('',(#2189),#912,.F.);
#24296=ADVANCED_FACE('',(#2190),#1393,.T.);
#24297=ADVANCED_FACE('',(#2191),#23415,.F.);
#24298=ADVANCED_FACE('',(#2192),#1394,.T.);
#24299=ADVANCED_FACE('',(#2193),#913,.F.);
#24300=ADVANCED_FACE('',(#2194),#1395,.T.);
#24301=ADVANCED_FACE('',(#2195),#23416,.F.);
#24302=ADVANCED_FACE('',(#2196),#1396,.T.);
#24303=ADVANCED_FACE('',(#2197),#914,.F.);
#24304=ADVANCED_FACE('',(#2198),#1397,.T.);
#24305=ADVANCED_FACE('',(#2199),#23417,.F.);
#24306=ADVANCED_FACE('',(#2200),#1398,.T.);
#24307=ADVANCED_FACE('',(#2201),#915,.F.);
#24308=ADVANCED_FACE('',(#2202),#1399,.T.);
#24309=ADVANCED_FACE('',(#2203),#23418,.F.);
#24310=ADVANCED_FACE('',(#2204),#1400,.T.);
#24311=ADVANCED_FACE('',(#2205),#916,.F.);
#24312=ADVANCED_FACE('',(#2206),#1401,.T.);
#24313=ADVANCED_FACE('',(#2207),#23419,.F.);
#24314=ADVANCED_FACE('',(#2208),#1402,.T.);
#24315=ADVANCED_FACE('',(#2209),#917,.F.);
#24316=ADVANCED_FACE('',(#2210),#1403,.T.);
#24317=ADVANCED_FACE('',(#2211),#23420,.F.);
#24318=ADVANCED_FACE('',(#2212),#1404,.T.);
#24319=ADVANCED_FACE('',(#2213),#918,.F.);
#24320=ADVANCED_FACE('',(#2214),#1405,.T.);
#24321=ADVANCED_FACE('',(#2215),#23421,.F.);
#24322=ADVANCED_FACE('',(#2216),#1406,.T.);
#24323=ADVANCED_FACE('',(#2217),#919,.F.);
#24324=ADVANCED_FACE('',(#2218),#1407,.T.);
#24325=ADVANCED_FACE('',(#2219),#23422,.F.);
#24326=ADVANCED_FACE('',(#2220),#1408,.T.);
#24327=ADVANCED_FACE('',(#2221),#920,.F.);
#24328=ADVANCED_FACE('',(#2222),#1409,.T.);
#24329=ADVANCED_FACE('',(#2223),#23423,.F.);
#24330=ADVANCED_FACE('',(#2224),#1410,.T.);
#24331=ADVANCED_FACE('',(#2225),#921,.F.);
#24332=ADVANCED_FACE('',(#2226),#1411,.T.);
#24333=ADVANCED_FACE('',(#2227),#23424,.F.);
#24334=ADVANCED_FACE('',(#2228),#1412,.T.);
#24335=ADVANCED_FACE('',(#2229),#922,.F.);
#24336=ADVANCED_FACE('',(#2230),#1413,.T.);
#24337=ADVANCED_FACE('',(#2231),#23425,.F.);
#24338=ADVANCED_FACE('',(#2232),#1414,.T.);
#24339=ADVANCED_FACE('',(#2233),#923,.F.);
#24340=ADVANCED_FACE('',(#2234),#1415,.T.);
#24341=ADVANCED_FACE('',(#2235),#23426,.F.);
#24342=ADVANCED_FACE('',(#2236),#1416,.T.);
#24343=ADVANCED_FACE('',(#2237),#924,.F.);
#24344=ADVANCED_FACE('',(#2238),#1417,.T.);
#24345=ADVANCED_FACE('',(#2239),#23427,.F.);
#24346=ADVANCED_FACE('',(#2240),#1418,.T.);
#24347=ADVANCED_FACE('',(#2241),#925,.F.);
#24348=ADVANCED_FACE('',(#2242),#1419,.T.);
#24349=ADVANCED_FACE('',(#2243),#23428,.F.);
#24350=ADVANCED_FACE('',(#2244),#1420,.T.);
#24351=ADVANCED_FACE('',(#2245),#926,.F.);
#24352=ADVANCED_FACE('',(#2246),#1421,.T.);
#24353=ADVANCED_FACE('',(#2247),#23429,.F.);
#24354=ADVANCED_FACE('',(#2248),#1422,.T.);
#24355=ADVANCED_FACE('',(#2249),#927,.F.);
#24356=ADVANCED_FACE('',(#2250),#1423,.T.);
#24357=ADVANCED_FACE('',(#2251),#23430,.F.);
#24358=ADVANCED_FACE('',(#2252),#1424,.T.);
#24359=ADVANCED_FACE('',(#2253),#928,.F.);
#24360=ADVANCED_FACE('',(#2254),#1425,.T.);
#24361=ADVANCED_FACE('',(#2255),#23431,.F.);
#24362=ADVANCED_FACE('',(#2256),#1426,.T.);
#24363=ADVANCED_FACE('',(#2257),#929,.F.);
#24364=ADVANCED_FACE('',(#2258),#1427,.T.);
#24365=ADVANCED_FACE('',(#2259),#23432,.F.);
#24366=ADVANCED_FACE('',(#2260),#1428,.T.);
#24367=ADVANCED_FACE('',(#2261),#930,.F.);
#24368=ADVANCED_FACE('',(#2262),#1429,.T.);
#24369=ADVANCED_FACE('',(#2263),#23433,.F.);
#24370=ADVANCED_FACE('',(#2264),#1430,.T.);
#24371=ADVANCED_FACE('',(#2265),#931,.F.);
#24372=ADVANCED_FACE('',(#2266),#1431,.T.);
#24373=ADVANCED_FACE('',(#2267),#23434,.F.);
#24374=ADVANCED_FACE('',(#2268),#1432,.T.);
#24375=ADVANCED_FACE('',(#2269),#932,.F.);
#24376=ADVANCED_FACE('',(#2270),#1433,.T.);
#24377=ADVANCED_FACE('',(#2271),#23435,.F.);
#24378=ADVANCED_FACE('',(#2272),#1434,.T.);
#24379=ADVANCED_FACE('',(#2273),#933,.F.);
#24380=ADVANCED_FACE('',(#2274),#1435,.T.);
#24381=ADVANCED_FACE('',(#2275),#23436,.F.);
#24382=ADVANCED_FACE('',(#2276),#1436,.T.);
#24383=ADVANCED_FACE('',(#2277),#934,.F.);
#24384=ADVANCED_FACE('',(#2278),#1437,.T.);
#24385=ADVANCED_FACE('',(#2279),#23437,.F.);
#24386=ADVANCED_FACE('',(#2280),#1438,.T.);
#24387=ADVANCED_FACE('',(#2281),#935,.F.);
#24388=ADVANCED_FACE('',(#2282),#1439,.T.);
#24389=ADVANCED_FACE('',(#2283),#23438,.F.);
#24390=ADVANCED_FACE('',(#2284),#1440,.T.);
#24391=ADVANCED_FACE('',(#2285),#936,.F.);
#24392=ADVANCED_FACE('',(#2286),#1441,.T.);
#24393=ADVANCED_FACE('',(#2287),#23439,.F.);
#24394=ADVANCED_FACE('',(#2288),#1442,.T.);
#24395=ADVANCED_FACE('',(#2289),#937,.F.);
#24396=ADVANCED_FACE('',(#2290),#1443,.T.);
#24397=ADVANCED_FACE('',(#2291),#23440,.F.);
#24398=ADVANCED_FACE('',(#2292),#1444,.T.);
#24399=ADVANCED_FACE('',(#2293),#938,.F.);
#24400=ADVANCED_FACE('',(#2294),#1445,.T.);
#24401=ADVANCED_FACE('',(#2295),#23441,.F.);
#24402=ADVANCED_FACE('',(#2296),#1446,.T.);
#24403=ADVANCED_FACE('',(#2297),#939,.F.);
#24404=ADVANCED_FACE('',(#2298),#1447,.T.);
#24405=ADVANCED_FACE('',(#2299),#23442,.F.);
#24406=ADVANCED_FACE('',(#2300),#1448,.T.);
#24407=ADVANCED_FACE('',(#2301),#940,.F.);
#24408=ADVANCED_FACE('',(#2302),#1449,.T.);
#24409=ADVANCED_FACE('',(#2303),#23443,.F.);
#24410=ADVANCED_FACE('',(#2304),#1450,.T.);
#24411=ADVANCED_FACE('',(#2305),#941,.F.);
#24412=ADVANCED_FACE('',(#2306),#1451,.T.);
#24413=ADVANCED_FACE('',(#2307),#23444,.F.);
#24414=ADVANCED_FACE('',(#2308),#1452,.T.);
#24415=ADVANCED_FACE('',(#2309),#942,.F.);
#24416=ADVANCED_FACE('',(#2310),#1453,.T.);
#24417=ADVANCED_FACE('',(#2311),#23445,.F.);
#24418=ADVANCED_FACE('',(#2312),#1454,.T.);
#24419=ADVANCED_FACE('',(#2313),#943,.F.);
#24420=ADVANCED_FACE('',(#2314),#1455,.T.);
#24421=ADVANCED_FACE('',(#2315),#23446,.F.);
#24422=ADVANCED_FACE('',(#2316),#1456,.T.);
#24423=ADVANCED_FACE('',(#2317),#944,.F.);
#24424=ADVANCED_FACE('',(#2318),#1457,.T.);
#24425=ADVANCED_FACE('',(#2319),#23447,.F.);
#24426=ADVANCED_FACE('',(#2320),#1458,.T.);
#24427=ADVANCED_FACE('',(#2321),#945,.F.);
#24428=ADVANCED_FACE('',(#2322),#1459,.T.);
#24429=ADVANCED_FACE('',(#2323),#23448,.F.);
#24430=ADVANCED_FACE('',(#2324),#1460,.T.);
#24431=ADVANCED_FACE('',(#2325),#946,.F.);
#24432=ADVANCED_FACE('',(#2326),#1461,.T.);
#24433=ADVANCED_FACE('',(#2327),#23449,.F.);
#24434=ADVANCED_FACE('',(#2328),#1462,.T.);
#24435=ADVANCED_FACE('',(#2329),#947,.F.);
#24436=ADVANCED_FACE('',(#2330),#1463,.T.);
#24437=ADVANCED_FACE('',(#2331),#23450,.F.);
#24438=ADVANCED_FACE('',(#2332),#1464,.T.);
#24439=ADVANCED_FACE('',(#2333),#948,.F.);
#24440=ADVANCED_FACE('',(#2334),#1465,.T.);
#24441=ADVANCED_FACE('',(#2335),#23451,.F.);
#24442=ADVANCED_FACE('',(#2336),#1466,.T.);
#24443=ADVANCED_FACE('',(#2337),#949,.F.);
#24444=ADVANCED_FACE('',(#2338),#1467,.T.);
#24445=ADVANCED_FACE('',(#2339),#23452,.F.);
#24446=ADVANCED_FACE('',(#2340),#1468,.T.);
#24447=ADVANCED_FACE('',(#2341),#950,.F.);
#24448=ADVANCED_FACE('',(#2342),#1469,.T.);
#24449=ADVANCED_FACE('',(#2343),#23453,.F.);
#24450=ADVANCED_FACE('',(#2344),#1470,.T.);
#24451=ADVANCED_FACE('',(#2345),#951,.F.);
#24452=ADVANCED_FACE('',(#2346),#1471,.T.);
#24453=ADVANCED_FACE('',(#2347),#23454,.F.);
#24454=ADVANCED_FACE('',(#2348),#1472,.T.);
#24455=ADVANCED_FACE('',(#2349),#952,.F.);
#24456=ADVANCED_FACE('',(#2350),#1473,.T.);
#24457=ADVANCED_FACE('',(#2351),#23455,.F.);
#24458=ADVANCED_FACE('',(#2352),#1474,.T.);
#24459=ADVANCED_FACE('',(#2353),#953,.F.);
#24460=ADVANCED_FACE('',(#2354),#1475,.T.);
#24461=ADVANCED_FACE('',(#2355),#23456,.F.);
#24462=ADVANCED_FACE('',(#2356),#954,.F.);
#24463=ADVANCED_FACE('',(#2357),#955,.F.);
#24464=ADVANCED_FACE('',(#2358),#956,.F.);
#24465=ADVANCED_FACE('',(#2359),#957,.F.);
#24466=ADVANCED_FACE('',(#2360),#958,.F.);
#24467=ADVANCED_FACE('',(#2361),#959,.F.);
#24468=ADVANCED_FACE('',(#2362),#960,.F.);
#24469=ADVANCED_FACE('',(#2363),#961,.F.);
#24470=ADVANCED_FACE('',(#2364),#962,.F.);
#24471=ADVANCED_FACE('',(#2365),#963,.F.);
#24472=ADVANCED_FACE('',(#2366),#964,.F.);
#24473=ADVANCED_FACE('',(#2367),#965,.F.);
#24474=ADVANCED_FACE('',(#2368),#966,.F.);
#24475=ADVANCED_FACE('',(#2369),#967,.F.);
#24476=ADVANCED_FACE('',(#2370),#968,.F.);
#24477=ADVANCED_FACE('',(#2371),#969,.F.);
#24478=ADVANCED_FACE('',(#2372),#970,.F.);
#24479=ADVANCED_FACE('',(#2373),#971,.F.);
#24480=ADVANCED_FACE('',(#2374),#972,.F.);
#24481=ADVANCED_FACE('',(#2375),#973,.F.);
#24482=ADVANCED_FACE('',(#2376),#974,.F.);
#24483=ADVANCED_FACE('',(#2377),#975,.F.);
#24484=ADVANCED_FACE('',(#2378),#976,.F.);
#24485=ADVANCED_FACE('',(#2379),#977,.F.);
#24486=ADVANCED_FACE('',(#2380),#978,.F.);
#24487=ADVANCED_FACE('',(#2381),#979,.F.);
#24488=ADVANCED_FACE('',(#2382),#980,.F.);
#24489=ADVANCED_FACE('',(#2383),#981,.F.);
#24490=ADVANCED_FACE('',(#2384),#982,.F.);
#24491=ADVANCED_FACE('',(#2385),#983,.F.);
#24492=ADVANCED_FACE('',(#2386),#984,.F.);
#24493=ADVANCED_FACE('',(#2387),#985,.F.);
#24494=ADVANCED_FACE('',(#2388),#986,.F.);
#24495=ADVANCED_FACE('',(#2389),#987,.F.);
#24496=ADVANCED_FACE('',(#2390),#988,.F.);
#24497=ADVANCED_FACE('',(#2391),#989,.F.);
#24498=ADVANCED_FACE('',(#2392),#990,.F.);
#24499=ADVANCED_FACE('',(#2393),#991,.F.);
#24500=ADVANCED_FACE('',(#2394),#992,.F.);
#24501=ADVANCED_FACE('',(#2395),#993,.F.);
#24502=ADVANCED_FACE('',(#2396),#994,.F.);
#24503=ADVANCED_FACE('',(#2397),#995,.F.);
#24504=ADVANCED_FACE('',(#2398),#996,.F.);
#24505=ADVANCED_FACE('',(#2399),#997,.F.);
#24506=ADVANCED_FACE('',(#2400),#998,.F.);
#24507=ADVANCED_FACE('',(#2401),#999,.F.);
#24508=ADVANCED_FACE('',(#2402),#1000,.F.);
#24509=ADVANCED_FACE('',(#2403),#1001,.F.);
#24510=ADVANCED_FACE('',(#2404),#1002,.F.);
#24511=ADVANCED_FACE('',(#2405),#1003,.F.);
#24512=ADVANCED_FACE('',(#2406),#1004,.F.);
#24513=ADVANCED_FACE('',(#2407),#1005,.F.);
#24514=ADVANCED_FACE('',(#2408),#1006,.F.);
#24515=ADVANCED_FACE('',(#2409),#1007,.F.);
#24516=ADVANCED_FACE('',(#2410),#1008,.F.);
#24517=ADVANCED_FACE('',(#2411),#1009,.F.);
#24518=ADVANCED_FACE('',(#2412),#1010,.F.);
#24519=ADVANCED_FACE('',(#2413),#1011,.F.);
#24520=ADVANCED_FACE('',(#2414),#1012,.F.);
#24521=ADVANCED_FACE('',(#2415),#1013,.F.);
#24522=ADVANCED_FACE('',(#2416),#1014,.F.);
#24523=ADVANCED_FACE('',(#2417),#1015,.F.);
#24524=ADVANCED_FACE('',(#2418),#1016,.F.);
#24525=ADVANCED_FACE('',(#2419),#1017,.F.);
#24526=ADVANCED_FACE('',(#2420),#1018,.F.);
#24527=ADVANCED_FACE('',(#2421),#1019,.F.);
#24528=ADVANCED_FACE('',(#2422),#1020,.F.);
#24529=ADVANCED_FACE('',(#2423),#1021,.F.);
#24530=ADVANCED_FACE('',(#2424),#1022,.F.);
#24531=ADVANCED_FACE('',(#2425),#1023,.F.);
#24532=ADVANCED_FACE('',(#2426),#1024,.F.);
#24533=ADVANCED_FACE('',(#2427),#23457,.F.);
#24534=ADVANCED_FACE('',(#2428),#23458,.F.);
#24535=ADVANCED_FACE('',(#2429),#23459,.F.);
#24536=ADVANCED_FACE('',(#2430),#23460,.F.);
#24537=ADVANCED_FACE('',(#2431),#23461,.F.);
#24538=ADVANCED_FACE('',(#2432),#23462,.F.);
#24539=ADVANCED_FACE('',(#2433),#23463,.F.);
#24540=ADVANCED_FACE('',(#2434),#23464,.F.);
#24541=ADVANCED_FACE('',(#2435),#23465,.F.);
#24542=ADVANCED_FACE('',(#2436),#23466,.F.);
#24543=ADVANCED_FACE('',(#2437),#23467,.F.);
#24544=ADVANCED_FACE('',(#2438),#23468,.F.);
#24545=ADVANCED_FACE('',(#2439),#23469,.F.);
#24546=ADVANCED_FACE('',(#2440),#23470,.F.);
#24547=ADVANCED_FACE('',(#2441),#23471,.F.);
#24548=ADVANCED_FACE('',(#2442),#23472,.F.);
#24549=ADVANCED_FACE('',(#2443),#23473,.F.);
#24550=ADVANCED_FACE('',(#2444),#23474,.F.);
#24551=ADVANCED_FACE('',(#2445),#23475,.F.);
#24552=ADVANCED_FACE('',(#2446),#23476,.F.);
#24553=ADVANCED_FACE('',(#2447),#23477,.F.);
#24554=ADVANCED_FACE('',(#2448),#23478,.F.);
#24555=ADVANCED_FACE('',(#2449),#23479,.F.);
#24556=ADVANCED_FACE('',(#2450),#23480,.F.);
#24557=ADVANCED_FACE('',(#2451),#23481,.F.);
#24558=ADVANCED_FACE('',(#2452),#23482,.F.);
#24559=ADVANCED_FACE('',(#2453),#23483,.F.);
#24560=ADVANCED_FACE('',(#2454),#23484,.F.);
#24561=ADVANCED_FACE('',(#2455),#23485,.F.);
#24562=ADVANCED_FACE('',(#2456),#23486,.F.);
#24563=ADVANCED_FACE('',(#2457),#23487,.F.);
#24564=ADVANCED_FACE('',(#2458),#23488,.F.);
#24565=ADVANCED_FACE('',(#2459),#23489,.F.);
#24566=ADVANCED_FACE('',(#2460),#23490,.F.);
#24567=ADVANCED_FACE('',(#2461),#23491,.F.);
#24568=ADVANCED_FACE('',(#2462),#23492,.F.);
#24569=ADVANCED_FACE('',(#2463),#23493,.F.);
#24570=ADVANCED_FACE('',(#2464),#23494,.F.);
#24571=ADVANCED_FACE('',(#2465),#23495,.F.);
#24572=ADVANCED_FACE('',(#2466),#23496,.F.);
#24573=ADVANCED_FACE('',(#2467),#23497,.F.);
#24574=ADVANCED_FACE('',(#2468),#23498,.F.);
#24575=ADVANCED_FACE('',(#2469),#23499,.F.);
#24576=ADVANCED_FACE('',(#2470),#23500,.F.);
#24577=ADVANCED_FACE('',(#2471),#23501,.F.);
#24578=ADVANCED_FACE('',(#2472),#23502,.F.);
#24579=ADVANCED_FACE('',(#2473),#23503,.F.);
#24580=ADVANCED_FACE('',(#2474),#23504,.F.);
#24581=ADVANCED_FACE('',(#2475),#23505,.F.);
#24582=ADVANCED_FACE('',(#2476),#23506,.F.);
#24583=ADVANCED_FACE('',(#2477),#23507,.F.);
#24584=ADVANCED_FACE('',(#2478),#23508,.F.);
#24585=ADVANCED_FACE('',(#2479),#23509,.F.);
#24586=ADVANCED_FACE('',(#2480),#23510,.F.);
#24587=ADVANCED_FACE('',(#2481),#23511,.F.);
#24588=ADVANCED_FACE('',(#2482),#23512,.F.);
#24589=ADVANCED_FACE('',(#2483),#23513,.F.);
#24590=ADVANCED_FACE('',(#2484),#23514,.F.);
#24591=ADVANCED_FACE('',(#2485),#23515,.F.);
#24592=ADVANCED_FACE('',(#2486),#23516,.F.);
#24593=ADVANCED_FACE('',(#2487),#23517,.F.);
#24594=ADVANCED_FACE('',(#2488),#23518,.F.);
#24595=ADVANCED_FACE('',(#2489),#23519,.F.);
#24596=ADVANCED_FACE('',(#2490),#23520,.F.);
#24597=ADVANCED_FACE('',(#2491),#23521,.F.);
#24598=ADVANCED_FACE('',(#2492),#23522,.F.);
#24599=ADVANCED_FACE('',(#2493),#23523,.F.);
#24600=ADVANCED_FACE('',(#2494),#23524,.F.);
#24601=ADVANCED_FACE('',(#2495),#23525,.F.);
#24602=ADVANCED_FACE('',(#2496),#23526,.F.);
#24603=ADVANCED_FACE('',(#2497),#23527,.F.);
#24604=ADVANCED_FACE('',(#2498),#1476,.T.);
#24605=ADVANCED_FACE('',(#2499),#1025,.F.);
#24606=ADVANCED_FACE('',(#2500),#1477,.T.);
#24607=ADVANCED_FACE('',(#2501),#23528,.F.);
#24608=ADVANCED_FACE('',(#2502),#1026,.F.);
#24609=ADVANCED_FACE('',(#2503,#1276),#1530,.T.);
#24610=ADVANCED_FACE('',(#2504),#23529,.F.);
#24611=ADVANCED_FACE('',(#2505,#1277,#1278,#1279),#23530,.T.);
#24612=ADVANCED_FACE('',(#2506,#1280),#1531,.F.);
#25154=CLOSED_SHELL('',(#24170,#24171,#24172,#24173,#24174,#24175,#24176,
#24177,#24178,#24179,#24180,#24181,#24182,#24183,#24184,#24185,#24186,#24187,
#24188,#24189,#24190,#24191,#24192,#24193,#24194,#24195,#24196,#24197,#24198,
#24199,#24200,#24201,#24202,#24203,#24204,#24205,#24206,#24207,#24208,#24209,
#24210,#24211,#24212,#24213,#24214,#24215,#24216,#24217,#24218,#24219,#24220,
#24221,#24222,#24223,#24224,#24225,#24226,#24227,#24228,#24229,#24230,#24231,
#24232,#24233,#24234,#24235,#24236,#24237,#24238,#24239,#24240,#24241,#24242,
#24243,#24244,#24245,#24246,#24247,#24248,#24249,#24250,#24251,#24252,#24253,
#24254,#24255,#24256,#24257,#24258,#24259,#24260,#24261,#24262,#24263,#24264,
#24265,#24266,#24267,#24268,#24269,#24270,#24271,#24272,#24273,#24274,#24275,
#24276,#24277,#24278,#24279,#24280,#24281,#24282,#24283,#24284,#24285,#24286,
#24287,#24288,#24289,#24290,#24291,#24292,#24293,#24294,#24295,#24296,#24297,
#24298,#24299,#24300,#24301,#24302,#24303,#24304,#24305,#24306,#24307,#24308,
#24309,#24310,#24311,#24312,#24313,#24314,#24315,#24316,#24317,#24318,#24319,
#24320,#24321,#24322,#24323,#24324,#24325,#24326,#24327,#24328,#24329,#24330,
#24331,#24332,#24333,#24334,#24335,#24336,#24337,#24338,#24339,#24340,#24341,
#24342,#24343,#24344,#24345,#24346,#24347,#24348,#24349,#24350,#24351,#24352,
#24353,#24354,#24355,#24356,#24357,#24358,#24359,#24360,#24361,#24362,#24363,
#24364,#24365,#24366,#24367,#24368,#24369,#24370,#24371,#24372,#24373,#24374,
#24375,#24376,#24377,#24378,#24379,#24380,#24381,#24382,#24383,#24384,#24385,
#24386,#24387,#24388,#24389,#24390,#24391,#24392,#24393,#24394,#24395,#24396,
#24397,#24398,#24399,#24400,#24401,#24402,#24403,#24404,#24405,#24406,#24407,
#24408,#24409,#24410,#24411,#24412,#24413,#24414,#24415,#24416,#24417,#24418,
#24419,#24420,#24421,#24422,#24423,#24424,#24425,#24426,#24427,#24428,#24429,
#24430,#24431,#24432,#24433,#24434,#24435,#24436,#24437,#24438,#24439,#24440,
#24441,#24442,#24443,#24444,#24445,#24446,#24447,#24448,#24449,#24450,#24451,
#24452,#24453,#24454,#24455,#24456,#24457,#24458,#24459,#24460,#24461,#24462,
#24463,#24464,#24465,#24466,#24467,#24468,#24469,#24470,#24471,#24472,#24473,
#24474,#24475,#24476,#24477,#24478,#24479,#24480,#24481,#24482,#24483,#24484,
#24485,#24486,#24487,#24488,#24489,#24490,#24491,#24492,#24493,#24494,#24495,
#24496,#24497,#24498,#24499,#24500,#24501,#24502,#24503,#24504,#24505,#24506,
#24507,#24508,#24509,#24510,#24511,#24512,#24513,#24514,#24515,#24516,#24517,
#24518,#24519,#24520,#24521,#24522,#24523,#24524,#24525,#24526,#24527,#24528,
#24529,#24530,#24531,#24532,#24533,#24534,#24535,#24536,#24537,#24538,#24539,
#24540,#24541,#24542,#24543,#24544,#24545,#24546,#24547,#24548,#24549,#24550,
#24551,#24552,#24553,#24554,#24555,#24556,#24557,#24558,#24559,#24560,#24561,
#24562,#24563,#24564,#24565,#24566,#24567,#24568,#24569,#24570,#24571,#24572,
#24573,#24574,#24575,#24576,#24577,#24578,#24579,#24580,#24581,#24582,#24583,
#24584,#24585,#24586,#24587,#24588,#24589,#24590,#24591,#24592,#24593,#24594,
#24595,#24596,#24597,#24598,#24599,#24600,#24601,#24602,#24603,#24604,#24605,
#24606,#24607,#24608,#24609,#24610,#24611,#24612));
#25864=AXIS2_PLACEMENT_3D('',#52395,#28593,#28594);
#25865=AXIS2_PLACEMENT_3D('',#52396,#28595,#28596);
#25866=AXIS2_PLACEMENT_3D('',#52419,#28598,#28599);
#25867=AXIS2_PLACEMENT_3D('',#52439,#28600,#28601);
#25868=AXIS2_PLACEMENT_3D('',#52440,#28602,#28603);
#25869=AXIS2_PLACEMENT_3D('',#52482,#28605,#28606);
#25870=AXIS2_PLACEMENT_3D('',#52483,#28607,#28608);
#25871=AXIS2_PLACEMENT_3D('',#52484,#28609,#28610);
#25872=AXIS2_PLACEMENT_3D('',#52518,#28612,#28613);
#25873=AXIS2_PLACEMENT_3D('',#52529,#28614,#28615);
#25874=AXIS2_PLACEMENT_3D('',#52530,#28616,#28617);
#25875=AXIS2_PLACEMENT_3D('',#52564,#28619,#28620);
#25876=AXIS2_PLACEMENT_3D('',#52575,#28621,#28622);
#25877=AXIS2_PLACEMENT_3D('',#53469,#28624,#28625);
#25878=AXIS2_PLACEMENT_3D('',#53470,#28626,#28627);
#25879=AXIS2_PLACEMENT_3D('',#53471,#28628,#28629);
#25880=AXIS2_PLACEMENT_3D('',#54365,#28631,#28632);
#25881=AXIS2_PLACEMENT_3D('',#54366,#28633,#28634);
#25882=AXIS2_PLACEMENT_3D('',#54367,#28635,#28636);
#25883=AXIS2_PLACEMENT_3D('',#55261,#28638,#28639);
#25884=AXIS2_PLACEMENT_3D('',#55262,#28640,#28641);
#25885=AXIS2_PLACEMENT_3D('',#55263,#28642,#28643);
#25886=AXIS2_PLACEMENT_3D('',#56157,#28645,#28646);
#25887=AXIS2_PLACEMENT_3D('',#56158,#28647,#28648);
#25888=AXIS2_PLACEMENT_3D('',#56159,#28649,#28650);
#25889=AXIS2_PLACEMENT_3D('',#57053,#28652,#28653);
#25890=AXIS2_PLACEMENT_3D('',#57054,#28654,#28655);
#25891=AXIS2_PLACEMENT_3D('',#57055,#28656,#28657);
#25892=AXIS2_PLACEMENT_3D('',#57949,#28659,#28660);
#25893=AXIS2_PLACEMENT_3D('',#57950,#28661,#28662);
#25894=AXIS2_PLACEMENT_3D('',#57951,#28663,#28664);
#25895=AXIS2_PLACEMENT_3D('',#58845,#28666,#28667);
#25896=AXIS2_PLACEMENT_3D('',#58846,#28668,#28669);
#25897=AXIS2_PLACEMENT_3D('',#58847,#28670,#28671);
#25898=AXIS2_PLACEMENT_3D('',#59741,#28673,#28674);
#25899=AXIS2_PLACEMENT_3D('',#59742,#28675,#28676);
#25900=AXIS2_PLACEMENT_3D('',#59743,#28677,#28678);
#25901=AXIS2_PLACEMENT_3D('',#60637,#28680,#28681);
#25902=AXIS2_PLACEMENT_3D('',#60638,#28682,#28683);
#25903=AXIS2_PLACEMENT_3D('',#60639,#28684,#28685);
#25904=AXIS2_PLACEMENT_3D('',#61533,#28687,#28688);
#25905=AXIS2_PLACEMENT_3D('',#61534,#28689,#28690);
#25906=AXIS2_PLACEMENT_3D('',#61535,#28691,#28692);
#25907=AXIS2_PLACEMENT_3D('',#62429,#28694,#28695);
#25908=AXIS2_PLACEMENT_3D('',#62430,#28696,#28697);
#25909=AXIS2_PLACEMENT_3D('',#62431,#28698,#28699);
#25910=AXIS2_PLACEMENT_3D('',#63325,#28701,#28702);
#25911=AXIS2_PLACEMENT_3D('',#63326,#28703,#28704);
#25912=AXIS2_PLACEMENT_3D('',#63327,#28705,#28706);
#25913=AXIS2_PLACEMENT_3D('',#64221,#28708,#28709);
#25914=AXIS2_PLACEMENT_3D('',#64222,#28710,#28711);
#25915=AXIS2_PLACEMENT_3D('',#64223,#28712,#28713);
#25916=AXIS2_PLACEMENT_3D('',#65117,#28715,#28716);
#25917=AXIS2_PLACEMENT_3D('',#65118,#28717,#28718);
#25918=AXIS2_PLACEMENT_3D('',#65119,#28719,#28720);
#25919=AXIS2_PLACEMENT_3D('',#66013,#28722,#28723);
#25920=AXIS2_PLACEMENT_3D('',#66014,#28724,#28725);
#25921=AXIS2_PLACEMENT_3D('',#66015,#28726,#28727);
#25922=AXIS2_PLACEMENT_3D('',#66909,#28729,#28730);
#25923=AXIS2_PLACEMENT_3D('',#66910,#28731,#28732);
#25924=AXIS2_PLACEMENT_3D('',#66911,#28733,#28734);
#25925=AXIS2_PLACEMENT_3D('',#67805,#28736,#28737);
#25926=AXIS2_PLACEMENT_3D('',#67806,#28738,#28739);
#25927=AXIS2_PLACEMENT_3D('',#67807,#28740,#28741);
#25928=AXIS2_PLACEMENT_3D('',#68701,#28743,#28744);
#25929=AXIS2_PLACEMENT_3D('',#68702,#28745,#28746);
#25930=AXIS2_PLACEMENT_3D('',#68703,#28747,#28748);
#25931=AXIS2_PLACEMENT_3D('',#69597,#28750,#28751);
#25932=AXIS2_PLACEMENT_3D('',#69598,#28752,#28753);
#25933=AXIS2_PLACEMENT_3D('',#69599,#28754,#28755);
#25934=AXIS2_PLACEMENT_3D('',#70493,#28757,#28758);
#25935=AXIS2_PLACEMENT_3D('',#70494,#28759,#28760);
#25936=AXIS2_PLACEMENT_3D('',#70495,#28761,#28762);
#25937=AXIS2_PLACEMENT_3D('',#71389,#28764,#28765);
#25938=AXIS2_PLACEMENT_3D('',#71390,#28766,#28767);
#25939=AXIS2_PLACEMENT_3D('',#71391,#28768,#28769);
#25940=AXIS2_PLACEMENT_3D('',#72285,#28771,#28772);
#25941=AXIS2_PLACEMENT_3D('',#72286,#28773,#28774);
#25942=AXIS2_PLACEMENT_3D('',#72287,#28775,#28776);
#25943=AXIS2_PLACEMENT_3D('',#73181,#28778,#28779);
#25944=AXIS2_PLACEMENT_3D('',#73182,#28780,#28781);
#25945=AXIS2_PLACEMENT_3D('',#73183,#28782,#28783);
#25946=AXIS2_PLACEMENT_3D('',#74077,#28785,#28786);
#25947=AXIS2_PLACEMENT_3D('',#74078,#28787,#28788);
#25948=AXIS2_PLACEMENT_3D('',#74079,#28789,#28790);
#25949=AXIS2_PLACEMENT_3D('',#74973,#28792,#28793);
#25950=AXIS2_PLACEMENT_3D('',#74974,#28794,#28795);
#25951=AXIS2_PLACEMENT_3D('',#74975,#28796,#28797);
#25952=AXIS2_PLACEMENT_3D('',#75869,#28799,#28800);
#25953=AXIS2_PLACEMENT_3D('',#75870,#28801,#28802);
#25954=AXIS2_PLACEMENT_3D('',#75871,#28803,#28804);
#25955=AXIS2_PLACEMENT_3D('',#76765,#28806,#28807);
#25956=AXIS2_PLACEMENT_3D('',#76766,#28808,#28809);
#25957=AXIS2_PLACEMENT_3D('',#76767,#28810,#28811);
#25958=AXIS2_PLACEMENT_3D('',#77661,#28813,#28814);
#25959=AXIS2_PLACEMENT_3D('',#77662,#28815,#28816);
#25960=AXIS2_PLACEMENT_3D('',#77663,#28817,#28818);
#25961=AXIS2_PLACEMENT_3D('',#78557,#28820,#28821);
#25962=AXIS2_PLACEMENT_3D('',#78558,#28822,#28823);
#25963=AXIS2_PLACEMENT_3D('',#78559,#28824,#28825);
#25964=AXIS2_PLACEMENT_3D('',#79453,#28827,#28828);
#25965=AXIS2_PLACEMENT_3D('',#79454,#28829,#28830);
#25966=AXIS2_PLACEMENT_3D('',#79455,#28831,#28832);
#25967=AXIS2_PLACEMENT_3D('',#80349,#28834,#28835);
#25968=AXIS2_PLACEMENT_3D('',#80350,#28836,#28837);
#25969=AXIS2_PLACEMENT_3D('',#80351,#28838,#28839);
#25970=AXIS2_PLACEMENT_3D('',#81245,#28841,#28842);
#25971=AXIS2_PLACEMENT_3D('',#81246,#28843,#28844);
#25972=AXIS2_PLACEMENT_3D('',#81247,#28845,#28846);
#25973=AXIS2_PLACEMENT_3D('',#82141,#28848,#28849);
#25974=AXIS2_PLACEMENT_3D('',#82142,#28850,#28851);
#25975=AXIS2_PLACEMENT_3D('',#82143,#28852,#28853);
#25976=AXIS2_PLACEMENT_3D('',#83037,#28855,#28856);
#25977=AXIS2_PLACEMENT_3D('',#83038,#28857,#28858);
#25978=AXIS2_PLACEMENT_3D('',#83039,#28859,#28860);
#25979=AXIS2_PLACEMENT_3D('',#83933,#28862,#28863);
#25980=AXIS2_PLACEMENT_3D('',#83934,#28864,#28865);
#25981=AXIS2_PLACEMENT_3D('',#83935,#28866,#28867);
#25982=AXIS2_PLACEMENT_3D('',#84829,#28869,#28870);
#25983=AXIS2_PLACEMENT_3D('',#84830,#28871,#28872);
#25984=AXIS2_PLACEMENT_3D('',#84831,#28873,#28874);
#25985=AXIS2_PLACEMENT_3D('',#85725,#28876,#28877);
#25986=AXIS2_PLACEMENT_3D('',#85726,#28878,#28879);
#25987=AXIS2_PLACEMENT_3D('',#85727,#28880,#28881);
#25988=AXIS2_PLACEMENT_3D('',#86621,#28883,#28884);
#25989=AXIS2_PLACEMENT_3D('',#86622,#28885,#28886);
#25990=AXIS2_PLACEMENT_3D('',#86623,#28887,#28888);
#25991=AXIS2_PLACEMENT_3D('',#87517,#28890,#28891);
#25992=AXIS2_PLACEMENT_3D('',#87518,#28892,#28893);
#25993=AXIS2_PLACEMENT_3D('',#87519,#28894,#28895);
#25994=AXIS2_PLACEMENT_3D('',#88413,#28897,#28898);
#25995=AXIS2_PLACEMENT_3D('',#88414,#28899,#28900);
#25996=AXIS2_PLACEMENT_3D('',#88415,#28901,#28902);
#25997=AXIS2_PLACEMENT_3D('',#89309,#28904,#28905);
#25998=AXIS2_PLACEMENT_3D('',#89310,#28906,#28907);
#25999=AXIS2_PLACEMENT_3D('',#89311,#28908,#28909);
#26000=AXIS2_PLACEMENT_3D('',#90205,#28911,#28912);
#26001=AXIS2_PLACEMENT_3D('',#90206,#28913,#28914);
#26002=AXIS2_PLACEMENT_3D('',#90207,#28915,#28916);
#26003=AXIS2_PLACEMENT_3D('',#91101,#28918,#28919);
#26004=AXIS2_PLACEMENT_3D('',#91102,#28920,#28921);
#26005=AXIS2_PLACEMENT_3D('',#91103,#28922,#28923);
#26006=AXIS2_PLACEMENT_3D('',#91997,#28925,#28926);
#26007=AXIS2_PLACEMENT_3D('',#91998,#28927,#28928);
#26008=AXIS2_PLACEMENT_3D('',#91999,#28929,#28930);
#26009=AXIS2_PLACEMENT_3D('',#92893,#28932,#28933);
#26010=AXIS2_PLACEMENT_3D('',#92894,#28934,#28935);
#26011=AXIS2_PLACEMENT_3D('',#92895,#28936,#28937);
#26012=AXIS2_PLACEMENT_3D('',#93789,#28939,#28940);
#26013=AXIS2_PLACEMENT_3D('',#93790,#28941,#28942);
#26014=AXIS2_PLACEMENT_3D('',#93791,#28943,#28944);
#26015=AXIS2_PLACEMENT_3D('',#94685,#28946,#28947);
#26016=AXIS2_PLACEMENT_3D('',#94686,#28948,#28949);
#26017=AXIS2_PLACEMENT_3D('',#94687,#28950,#28951);
#26018=AXIS2_PLACEMENT_3D('',#95581,#28953,#28954);
#26019=AXIS2_PLACEMENT_3D('',#95582,#28955,#28956);
#26020=AXIS2_PLACEMENT_3D('',#95583,#28957,#28958);
#26021=AXIS2_PLACEMENT_3D('',#96477,#28960,#28961);
#26022=AXIS2_PLACEMENT_3D('',#96478,#28962,#28963);
#26023=AXIS2_PLACEMENT_3D('',#96479,#28964,#28965);
#26024=AXIS2_PLACEMENT_3D('',#97373,#28967,#28968);
#26025=AXIS2_PLACEMENT_3D('',#97374,#28969,#28970);
#26026=AXIS2_PLACEMENT_3D('',#97375,#28971,#28972);
#26027=AXIS2_PLACEMENT_3D('',#98269,#28974,#28975);
#26028=AXIS2_PLACEMENT_3D('',#98270,#28976,#28977);
#26029=AXIS2_PLACEMENT_3D('',#98271,#28978,#28979);
#26030=AXIS2_PLACEMENT_3D('',#99165,#28981,#28982);
#26031=AXIS2_PLACEMENT_3D('',#99166,#28983,#28984);
#26032=AXIS2_PLACEMENT_3D('',#99167,#28985,#28986);
#26033=AXIS2_PLACEMENT_3D('',#100061,#28988,#28989);
#26034=AXIS2_PLACEMENT_3D('',#100062,#28990,#28991);
#26035=AXIS2_PLACEMENT_3D('',#100063,#28992,#28993);
#26036=AXIS2_PLACEMENT_3D('',#100957,#28995,#28996);
#26037=AXIS2_PLACEMENT_3D('',#100958,#28997,#28998);
#26038=AXIS2_PLACEMENT_3D('',#100959,#28999,#29000);
#26039=AXIS2_PLACEMENT_3D('',#101853,#29002,#29003);
#26040=AXIS2_PLACEMENT_3D('',#101854,#29004,#29005);
#26041=AXIS2_PLACEMENT_3D('',#101855,#29006,#29007);
#26042=AXIS2_PLACEMENT_3D('',#102749,#29009,#29010);
#26043=AXIS2_PLACEMENT_3D('',#102750,#29011,#29012);
#26044=AXIS2_PLACEMENT_3D('',#102751,#29013,#29014);
#26045=AXIS2_PLACEMENT_3D('',#103645,#29016,#29017);
#26046=AXIS2_PLACEMENT_3D('',#103646,#29018,#29019);
#26047=AXIS2_PLACEMENT_3D('',#103647,#29020,#29021);
#26048=AXIS2_PLACEMENT_3D('',#104541,#29023,#29024);
#26049=AXIS2_PLACEMENT_3D('',#104542,#29025,#29026);
#26050=AXIS2_PLACEMENT_3D('',#104543,#29027,#29028);
#26051=AXIS2_PLACEMENT_3D('',#105437,#29030,#29031);
#26052=AXIS2_PLACEMENT_3D('',#105438,#29032,#29033);
#26053=AXIS2_PLACEMENT_3D('',#105439,#29034,#29035);
#26054=AXIS2_PLACEMENT_3D('',#106333,#29037,#29038);
#26055=AXIS2_PLACEMENT_3D('',#106334,#29039,#29040);
#26056=AXIS2_PLACEMENT_3D('',#106335,#29041,#29042);
#26057=AXIS2_PLACEMENT_3D('',#107229,#29044,#29045);
#26058=AXIS2_PLACEMENT_3D('',#107230,#29046,#29047);
#26059=AXIS2_PLACEMENT_3D('',#107231,#29048,#29049);
#26060=AXIS2_PLACEMENT_3D('',#108125,#29051,#29052);
#26061=AXIS2_PLACEMENT_3D('',#108126,#29053,#29054);
#26062=AXIS2_PLACEMENT_3D('',#108127,#29055,#29056);
#26063=AXIS2_PLACEMENT_3D('',#109021,#29058,#29059);
#26064=AXIS2_PLACEMENT_3D('',#109022,#29060,#29061);
#26065=AXIS2_PLACEMENT_3D('',#109023,#29062,#29063);
#26066=AXIS2_PLACEMENT_3D('',#109917,#29065,#29066);
#26067=AXIS2_PLACEMENT_3D('',#109918,#29067,#29068);
#26068=AXIS2_PLACEMENT_3D('',#109919,#29069,#29070);
#26069=AXIS2_PLACEMENT_3D('',#110813,#29072,#29073);
#26070=AXIS2_PLACEMENT_3D('',#110814,#29074,#29075);
#26071=AXIS2_PLACEMENT_3D('',#110815,#29076,#29077);
#26072=AXIS2_PLACEMENT_3D('',#111709,#29079,#29080);
#26073=AXIS2_PLACEMENT_3D('',#111710,#29081,#29082);
#26074=AXIS2_PLACEMENT_3D('',#111711,#29083,#29084);
#26075=AXIS2_PLACEMENT_3D('',#112605,#29086,#29087);
#26076=AXIS2_PLACEMENT_3D('',#112606,#29088,#29089);
#26077=AXIS2_PLACEMENT_3D('',#112607,#29090,#29091);
#26078=AXIS2_PLACEMENT_3D('',#113501,#29093,#29094);
#26079=AXIS2_PLACEMENT_3D('',#113502,#29095,#29096);
#26080=AXIS2_PLACEMENT_3D('',#113503,#29097,#29098);
#26081=AXIS2_PLACEMENT_3D('',#114397,#29100,#29101);
#26082=AXIS2_PLACEMENT_3D('',#114398,#29102,#29103);
#26083=AXIS2_PLACEMENT_3D('',#114399,#29104,#29105);
#26084=AXIS2_PLACEMENT_3D('',#115293,#29107,#29108);
#26085=AXIS2_PLACEMENT_3D('',#115294,#29109,#29110);
#26086=AXIS2_PLACEMENT_3D('',#115295,#29111,#29112);
#26087=AXIS2_PLACEMENT_3D('',#116189,#29114,#29115);
#26088=AXIS2_PLACEMENT_3D('',#116190,#29116,#29117);
#26089=AXIS2_PLACEMENT_3D('',#116191,#29118,#29119);
#26090=AXIS2_PLACEMENT_3D('',#173063,#29191,#29192);
#26091=AXIS2_PLACEMENT_3D('',#173065,#29193,#29194);
#26092=AXIS2_PLACEMENT_3D('',#173068,#29196,#29197);
#26093=AXIS2_PLACEMENT_3D('',#173069,#29198,#29199);
#26094=AXIS2_PLACEMENT_3D('',#173070,#29200,#29201);
#26095=AXIS2_PLACEMENT_3D('',#173071,#29202,#29203);
#26096=AXIS2_PLACEMENT_3D('',#173072,#29204,#29205);
#26097=AXIS2_PLACEMENT_3D('',#173073,#29206,#29207);
#26098=AXIS2_PLACEMENT_3D('',#173074,#29208,#29209);
#26099=AXIS2_PLACEMENT_3D('',#173075,#29210,#29211);
#26100=AXIS2_PLACEMENT_3D('',#173076,#29212,#29213);
#26101=AXIS2_PLACEMENT_3D('',#173077,#29214,#29215);
#26102=AXIS2_PLACEMENT_3D('',#173078,#29216,#29217);
#26103=AXIS2_PLACEMENT_3D('',#173079,#29218,#29219);
#26104=AXIS2_PLACEMENT_3D('',#173080,#29220,#29221);
#26105=AXIS2_PLACEMENT_3D('',#173081,#29222,#29223);
#26106=AXIS2_PLACEMENT_3D('',#173082,#29224,#29225);
#26107=AXIS2_PLACEMENT_3D('',#173083,#29226,#29227);
#26108=AXIS2_PLACEMENT_3D('',#173084,#29228,#29229);
#26109=AXIS2_PLACEMENT_3D('',#173085,#29230,#29231);
#26110=AXIS2_PLACEMENT_3D('',#173086,#29232,#29233);
#26111=AXIS2_PLACEMENT_3D('',#173087,#29234,#29235);
#26112=AXIS2_PLACEMENT_3D('',#173088,#29236,#29237);
#26113=AXIS2_PLACEMENT_3D('',#173089,#29238,#29239);
#26114=AXIS2_PLACEMENT_3D('',#173090,#29240,#29241);
#26115=AXIS2_PLACEMENT_3D('',#173091,#29242,#29243);
#26116=AXIS2_PLACEMENT_3D('',#173092,#29244,#29245);
#26117=AXIS2_PLACEMENT_3D('',#173093,#29246,#29247);
#26118=AXIS2_PLACEMENT_3D('',#173094,#29248,#29249);
#26119=AXIS2_PLACEMENT_3D('',#173095,#29250,#29251);
#26120=AXIS2_PLACEMENT_3D('',#173096,#29252,#29253);
#26121=AXIS2_PLACEMENT_3D('',#173097,#29254,#29255);
#26122=AXIS2_PLACEMENT_3D('',#173098,#29256,#29257);
#26123=AXIS2_PLACEMENT_3D('',#173099,#29258,#29259);
#26124=AXIS2_PLACEMENT_3D('',#173100,#29260,#29261);
#26125=AXIS2_PLACEMENT_3D('',#173101,#29262,#29263);
#26126=AXIS2_PLACEMENT_3D('',#173102,#29264,#29265);
#26127=AXIS2_PLACEMENT_3D('',#173103,#29266,#29267);
#26128=AXIS2_PLACEMENT_3D('',#173104,#29268,#29269);
#26129=AXIS2_PLACEMENT_3D('',#173105,#29270,#29271);
#26130=AXIS2_PLACEMENT_3D('',#173106,#29272,#29273);
#26131=AXIS2_PLACEMENT_3D('',#173107,#29274,#29275);
#26132=AXIS2_PLACEMENT_3D('',#173108,#29276,#29277);
#26133=AXIS2_PLACEMENT_3D('',#173109,#29278,#29279);
#26134=AXIS2_PLACEMENT_3D('',#173110,#29280,#29281);
#26135=AXIS2_PLACEMENT_3D('',#173111,#29282,#29283);
#26136=AXIS2_PLACEMENT_3D('',#173112,#29284,#29285);
#26137=AXIS2_PLACEMENT_3D('',#173113,#29286,#29287);
#26138=AXIS2_PLACEMENT_3D('',#173114,#29288,#29289);
#26139=AXIS2_PLACEMENT_3D('',#173115,#29290,#29291);
#26140=AXIS2_PLACEMENT_3D('',#173116,#29292,#29293);
#26141=AXIS2_PLACEMENT_3D('',#173117,#29294,#29295);
#26142=AXIS2_PLACEMENT_3D('',#173118,#29296,#29297);
#26143=AXIS2_PLACEMENT_3D('',#173119,#29298,#29299);
#26144=AXIS2_PLACEMENT_3D('',#173120,#29300,#29301);
#26145=AXIS2_PLACEMENT_3D('',#173121,#29302,#29303);
#26146=AXIS2_PLACEMENT_3D('',#173122,#29304,#29305);
#26147=AXIS2_PLACEMENT_3D('',#173123,#29306,#29307);
#26148=AXIS2_PLACEMENT_3D('',#173124,#29308,#29309);
#26149=AXIS2_PLACEMENT_3D('',#173125,#29310,#29311);
#26150=AXIS2_PLACEMENT_3D('',#173126,#29312,#29313);
#26151=AXIS2_PLACEMENT_3D('',#173127,#29314,#29315);
#26152=AXIS2_PLACEMENT_3D('',#173128,#29316,#29317);
#26153=AXIS2_PLACEMENT_3D('',#173129,#29318,#29319);
#26154=AXIS2_PLACEMENT_3D('',#173130,#29320,#29321);
#26155=AXIS2_PLACEMENT_3D('',#173131,#29322,#29323);
#26156=AXIS2_PLACEMENT_3D('',#173132,#29324,#29325);
#26157=AXIS2_PLACEMENT_3D('',#173133,#29326,#29327);
#26158=AXIS2_PLACEMENT_3D('',#173134,#29328,#29329);
#26159=AXIS2_PLACEMENT_3D('',#173135,#29330,#29331);
#26160=AXIS2_PLACEMENT_3D('',#173136,#29332,#29333);
#26161=AXIS2_PLACEMENT_3D('',#173137,#29334,#29335);
#26162=AXIS2_PLACEMENT_3D('',#173138,#29336,#29337);
#26163=AXIS2_PLACEMENT_3D('',#173139,#29338,#29339);
#26164=AXIS2_PLACEMENT_3D('',#173140,#29340,#29341);
#26165=AXIS2_PLACEMENT_3D('',#173141,#29342,#29343);
#26166=AXIS2_PLACEMENT_3D('',#173142,#29344,#29345);
#26167=AXIS2_PLACEMENT_3D('',#173143,#29346,#29347);
#26168=AXIS2_PLACEMENT_3D('',#173144,#29348,#29349);
#26169=AXIS2_PLACEMENT_3D('',#173145,#29350,#29351);
#26170=AXIS2_PLACEMENT_3D('',#173146,#29352,#29353);
#26171=AXIS2_PLACEMENT_3D('',#173147,#29354,#29355);
#26172=AXIS2_PLACEMENT_3D('',#173148,#29356,#29357);
#26173=AXIS2_PLACEMENT_3D('',#173149,#29358,#29359);
#26174=AXIS2_PLACEMENT_3D('',#173150,#29360,#29361);
#26175=AXIS2_PLACEMENT_3D('',#173151,#29362,#29363);
#26176=AXIS2_PLACEMENT_3D('',#173152,#29364,#29365);
#26177=AXIS2_PLACEMENT_3D('',#173153,#29366,#29367);
#26178=AXIS2_PLACEMENT_3D('',#173154,#29368,#29369);
#26179=AXIS2_PLACEMENT_3D('',#173155,#29370,#29371);
#26180=AXIS2_PLACEMENT_3D('',#173156,#29372,#29373);
#26181=AXIS2_PLACEMENT_3D('',#173157,#29374,#29375);
#26182=AXIS2_PLACEMENT_3D('',#173158,#29376,#29377);
#26183=AXIS2_PLACEMENT_3D('',#173159,#29378,#29379);
#26184=AXIS2_PLACEMENT_3D('',#173160,#29380,#29381);
#26185=AXIS2_PLACEMENT_3D('',#173161,#29382,#29383);
#26186=AXIS2_PLACEMENT_3D('',#173162,#29384,#29385);
#26187=AXIS2_PLACEMENT_3D('',#173163,#29386,#29387);
#26188=AXIS2_PLACEMENT_3D('',#173164,#29388,#29389);
#26189=AXIS2_PLACEMENT_3D('',#173165,#29390,#29391);
#26190=AXIS2_PLACEMENT_3D('',#173166,#29392,#29393);
#26191=AXIS2_PLACEMENT_3D('',#173167,#29394,#29395);
#26192=AXIS2_PLACEMENT_3D('',#173168,#29396,#29397);
#26193=AXIS2_PLACEMENT_3D('',#173169,#29398,#29399);
#26194=AXIS2_PLACEMENT_3D('',#173170,#29400,#29401);
#26195=AXIS2_PLACEMENT_3D('',#173171,#29402,#29403);
#26196=AXIS2_PLACEMENT_3D('',#173172,#29404,#29405);
#26197=AXIS2_PLACEMENT_3D('',#173173,#29406,#29407);
#26198=AXIS2_PLACEMENT_3D('',#173174,#29408,#29409);
#26199=AXIS2_PLACEMENT_3D('',#173175,#29410,#29411);
#26200=AXIS2_PLACEMENT_3D('',#173176,#29412,#29413);
#26201=AXIS2_PLACEMENT_3D('',#173177,#29414,#29415);
#26202=AXIS2_PLACEMENT_3D('',#173178,#29416,#29417);
#26203=AXIS2_PLACEMENT_3D('',#173179,#29418,#29419);
#26204=AXIS2_PLACEMENT_3D('',#173180,#29420,#29421);
#26205=AXIS2_PLACEMENT_3D('',#173181,#29422,#29423);
#26206=AXIS2_PLACEMENT_3D('',#173182,#29424,#29425);
#26207=AXIS2_PLACEMENT_3D('',#173183,#29426,#29427);
#26208=AXIS2_PLACEMENT_3D('',#173184,#29428,#29429);
#26209=AXIS2_PLACEMENT_3D('',#173185,#29430,#29431);
#26210=AXIS2_PLACEMENT_3D('',#173186,#29432,#29433);
#26211=AXIS2_PLACEMENT_3D('',#173187,#29434,#29435);
#26212=AXIS2_PLACEMENT_3D('',#173188,#29436,#29437);
#26213=AXIS2_PLACEMENT_3D('',#173189,#29438,#29439);
#26214=AXIS2_PLACEMENT_3D('',#173190,#29440,#29441);
#26215=AXIS2_PLACEMENT_3D('',#173191,#29442,#29443);
#26216=AXIS2_PLACEMENT_3D('',#173192,#29444,#29445);
#26217=AXIS2_PLACEMENT_3D('',#173193,#29446,#29447);
#26218=AXIS2_PLACEMENT_3D('',#173194,#29448,#29449);
#26219=AXIS2_PLACEMENT_3D('',#173195,#29450,#29451);
#26220=AXIS2_PLACEMENT_3D('',#173196,#29452,#29453);
#26221=AXIS2_PLACEMENT_3D('',#173197,#29454,#29455);
#26222=AXIS2_PLACEMENT_3D('',#173198,#29456,#29457);
#26223=AXIS2_PLACEMENT_3D('',#173199,#29458,#29459);
#26224=AXIS2_PLACEMENT_3D('',#173200,#29460,#29461);
#26225=AXIS2_PLACEMENT_3D('',#173201,#29462,#29463);
#26226=AXIS2_PLACEMENT_3D('',#173202,#29464,#29465);
#26227=AXIS2_PLACEMENT_3D('',#173203,#29466,#29467);
#26228=AXIS2_PLACEMENT_3D('',#173204,#29468,#29469);
#26229=AXIS2_PLACEMENT_3D('',#173205,#29470,#29471);
#26230=AXIS2_PLACEMENT_3D('',#173206,#29472,#29473);
#26231=AXIS2_PLACEMENT_3D('',#173207,#29474,#29475);
#26232=AXIS2_PLACEMENT_3D('',#173208,#29476,#29477);
#26233=AXIS2_PLACEMENT_3D('',#173209,#29478,#29479);
#26234=AXIS2_PLACEMENT_3D('',#173210,#29480,#29481);
#26235=AXIS2_PLACEMENT_3D('',#173211,#29482,#29483);
#26236=AXIS2_PLACEMENT_3D('',#173212,#29484,#29485);
#26237=AXIS2_PLACEMENT_3D('',#173213,#29486,#29487);
#26238=AXIS2_PLACEMENT_3D('',#173214,#29488,#29489);
#26239=AXIS2_PLACEMENT_3D('',#173215,#29490,#29491);
#26240=AXIS2_PLACEMENT_3D('',#173216,#29492,#29493);
#26241=AXIS2_PLACEMENT_3D('',#173217,#29494,#29495);
#26242=AXIS2_PLACEMENT_3D('',#173218,#29496,#29497);
#26243=AXIS2_PLACEMENT_3D('',#173219,#29498,#29499);
#26244=AXIS2_PLACEMENT_3D('',#173220,#29500,#29501);
#26245=AXIS2_PLACEMENT_3D('',#173221,#29502,#29503);
#26246=AXIS2_PLACEMENT_3D('',#173222,#29504,#29505);
#26247=AXIS2_PLACEMENT_3D('',#173223,#29506,#29507);
#26248=AXIS2_PLACEMENT_3D('',#173224,#29508,#29509);
#26249=AXIS2_PLACEMENT_3D('',#173225,#29510,#29511);
#26250=AXIS2_PLACEMENT_3D('',#173226,#29512,#29513);
#26251=AXIS2_PLACEMENT_3D('',#173227,#29514,#29515);
#26252=AXIS2_PLACEMENT_3D('',#173228,#29516,#29517);
#26253=AXIS2_PLACEMENT_3D('',#173229,#29518,#29519);
#26254=AXIS2_PLACEMENT_3D('',#173230,#29520,#29521);
#26255=AXIS2_PLACEMENT_3D('',#173231,#29522,#29523);
#26256=AXIS2_PLACEMENT_3D('',#173232,#29524,#29525);
#26257=AXIS2_PLACEMENT_3D('',#173233,#29526,#29527);
#26258=AXIS2_PLACEMENT_3D('',#173234,#29528,#29529);
#26259=AXIS2_PLACEMENT_3D('',#173235,#29530,#29531);
#26260=AXIS2_PLACEMENT_3D('',#173236,#29532,#29533);
#26261=AXIS2_PLACEMENT_3D('',#173237,#29534,#29535);
#26262=AXIS2_PLACEMENT_3D('',#173238,#29536,#29537);
#26263=AXIS2_PLACEMENT_3D('',#173239,#29538,#29539);
#26264=AXIS2_PLACEMENT_3D('',#173240,#29540,#29541);
#26265=AXIS2_PLACEMENT_3D('',#173241,#29542,#29543);
#26266=AXIS2_PLACEMENT_3D('',#173242,#29544,#29545);
#26267=AXIS2_PLACEMENT_3D('',#173243,#29546,#29547);
#26268=AXIS2_PLACEMENT_3D('',#173244,#29548,#29549);
#26269=AXIS2_PLACEMENT_3D('',#173245,#29550,#29551);
#26270=AXIS2_PLACEMENT_3D('',#173246,#29552,#29553);
#26271=AXIS2_PLACEMENT_3D('',#173247,#29554,#29555);
#26272=AXIS2_PLACEMENT_3D('',#173248,#29556,#29557);
#26273=AXIS2_PLACEMENT_3D('',#173249,#29558,#29559);
#26274=AXIS2_PLACEMENT_3D('',#173250,#29560,#29561);
#26275=AXIS2_PLACEMENT_3D('',#173251,#29562,#29563);
#26276=AXIS2_PLACEMENT_3D('',#173252,#29564,#29565);
#26277=AXIS2_PLACEMENT_3D('',#173253,#29566,#29567);
#26278=AXIS2_PLACEMENT_3D('',#173254,#29568,#29569);
#26279=AXIS2_PLACEMENT_3D('',#173255,#29570,#29571);
#26280=AXIS2_PLACEMENT_3D('',#173256,#29572,#29573);
#26281=AXIS2_PLACEMENT_3D('',#173257,#29574,#29575);
#26282=AXIS2_PLACEMENT_3D('',#173258,#29576,#29577);
#26283=AXIS2_PLACEMENT_3D('',#173259,#29578,#29579);
#26284=AXIS2_PLACEMENT_3D('',#173260,#29580,#29581);
#26285=AXIS2_PLACEMENT_3D('',#173261,#29582,#29583);
#26286=AXIS2_PLACEMENT_3D('',#173262,#29584,#29585);
#26287=AXIS2_PLACEMENT_3D('',#173263,#29586,#29587);
#26288=AXIS2_PLACEMENT_3D('',#173264,#29588,#29589);
#26289=AXIS2_PLACEMENT_3D('',#173265,#29590,#29591);
#26290=AXIS2_PLACEMENT_3D('',#173266,#29592,#29593);
#26291=AXIS2_PLACEMENT_3D('',#173267,#29594,#29595);
#26292=AXIS2_PLACEMENT_3D('',#173268,#29596,#29597);
#26293=AXIS2_PLACEMENT_3D('',#173269,#29598,#29599);
#26294=AXIS2_PLACEMENT_3D('',#173270,#29600,#29601);
#26295=AXIS2_PLACEMENT_3D('',#173271,#29602,#29603);
#26296=AXIS2_PLACEMENT_3D('',#173272,#29604,#29605);
#26297=AXIS2_PLACEMENT_3D('',#173273,#29606,#29607);
#26298=AXIS2_PLACEMENT_3D('',#173274,#29608,#29609);
#26299=AXIS2_PLACEMENT_3D('',#173275,#29610,#29611);
#26300=AXIS2_PLACEMENT_3D('',#173276,#29612,#29613);
#26301=AXIS2_PLACEMENT_3D('',#173278,#29614,#29615);
#26302=AXIS2_PLACEMENT_3D('',#173281,#29617,#29618);
#26303=AXIS2_PLACEMENT_3D('',#174172,#29619,#29620);
#26304=AXIS2_PLACEMENT_3D('',#174173,#29621,#29622);
#26305=AXIS2_PLACEMENT_3D('',#174174,#29623,#29624);
#26306=AXIS2_PLACEMENT_3D('',#174973,#29625,#29626);
#26307=AXIS2_PLACEMENT_3D('',#174975,#29627,#29628);
#26308=AXIS2_PLACEMENT_3D('',#174976,#29629,#29630);
#26309=AXIS2_PLACEMENT_3D('',#174977,#29631,#29632);
#26310=AXIS2_PLACEMENT_3D('',#174978,#29633,#29634);
#26311=AXIS2_PLACEMENT_3D('',#174979,#29635,#29636);
#26312=AXIS2_PLACEMENT_3D('',#174983,#29639,#29640);
#26313=AXIS2_PLACEMENT_3D('',#174984,#29641,#29642);
#28593=DIRECTION('axis',(0.,0.,1.));
#28594=DIRECTION('refdir',(1.,0.,0.));
#28595=DIRECTION('center_axis',(0.,1.,0.));
#28596=DIRECTION('ref_axis',(0.,0.,-1.));
#28597=DIRECTION('',(0.,1.,0.));
#28598=DIRECTION('center_axis',(0.,1.,0.));
#28599=DIRECTION('ref_axis',(0.,0.,-1.));
#28600=DIRECTION('center_axis',(0.,1.,0.));
#28601=DIRECTION('ref_axis',(0.,0.,-1.));
#28602=DIRECTION('center_axis',(0.,-1.,0.));
#28603=DIRECTION('ref_axis',(0.,0.,1.));
#28604=DIRECTION('',(0.,-1.,0.));
#28605=DIRECTION('center_axis',(0.,-1.,0.));
#28606=DIRECTION('ref_axis',(0.,0.,1.));
#28607=DIRECTION('center_axis',(0.,-1.,0.));
#28608=DIRECTION('ref_axis',(0.,0.,1.));
#28609=DIRECTION('center_axis',(1.,0.,0.));
#28610=DIRECTION('ref_axis',(0.,-1.,0.));
#28611=DIRECTION('',(1.,0.,0.));
#28612=DIRECTION('center_axis',(1.,0.,0.));
#28613=DIRECTION('ref_axis',(0.,-1.,0.));
#28614=DIRECTION('center_axis',(1.,0.,0.));
#28615=DIRECTION('ref_axis',(0.,-1.,0.));
#28616=DIRECTION('center_axis',(-1.,0.,0.));
#28617=DIRECTION('ref_axis',(0.,1.,0.));
#28618=DIRECTION('',(-1.,0.,0.));
#28619=DIRECTION('center_axis',(-1.,0.,0.));
#28620=DIRECTION('ref_axis',(0.,1.,0.));
#28621=DIRECTION('center_axis',(-1.,0.,0.));
#28622=DIRECTION('ref_axis',(0.,1.,0.));
#28623=DIRECTION('',(0.,0.,-1.));
#28624=DIRECTION('center_axis',(0.,0.,1.));
#28625=DIRECTION('ref_axis',(0.998647288695349,-0.0519960842893784,0.));
#28626=DIRECTION('center_axis',(0.,0.,-1.));
#28627=DIRECTION('ref_axis',(0.998647288695349,-0.0519960842893784,0.));
#28628=DIRECTION('center_axis',(0.,0.,1.));
#28629=DIRECTION('ref_axis',(0.998647288695349,-0.0519960842893784,0.));
#28630=DIRECTION('',(0.,0.,-1.));
#28631=DIRECTION('center_axis',(0.,0.,1.));
#28632=DIRECTION('ref_axis',(0.990315376915793,-0.138836069679788,0.));
#28633=DIRECTION('center_axis',(0.,0.,-1.));
#28634=DIRECTION('ref_axis',(0.990315376915793,-0.138836069679788,0.));
#28635=DIRECTION('center_axis',(0.,0.,1.));
#28636=DIRECTION('ref_axis',(0.990315376915793,-0.138836069679788,0.));
#28637=DIRECTION('',(0.,0.,-1.));
#28638=DIRECTION('center_axis',(0.,0.,1.));
#28639=DIRECTION('ref_axis',(0.974446567149134,-0.224619428748424,0.));
#28640=DIRECTION('center_axis',(0.,0.,-1.));
#28641=DIRECTION('ref_axis',(0.974446567149134,-0.224619428748424,0.));
#28642=DIRECTION('center_axis',(0.,0.,1.));
#28643=DIRECTION('ref_axis',(0.974446567149134,-0.224619428748424,0.));
#28644=DIRECTION('',(0.,0.,-1.));
#28645=DIRECTION('center_axis',(0.,0.,1.));
#28646=DIRECTION('ref_axis',(0.951161630619545,-0.308693298335366,0.));
#28647=DIRECTION('center_axis',(0.,0.,-1.));
#28648=DIRECTION('ref_axis',(0.951161630619545,-0.308693298335366,0.));
#28649=DIRECTION('center_axis',(0.,0.,1.));
#28650=DIRECTION('ref_axis',(0.951161630619545,-0.308693298335366,0.));
#28651=DIRECTION('',(0.,0.,-1.));
#28652=DIRECTION('center_axis',(0.,0.,1.));
#28653=DIRECTION('ref_axis',(0.920637779753847,-0.390417825527865,0.));
#28654=DIRECTION('center_axis',(0.,0.,-1.));
#28655=DIRECTION('ref_axis',(0.920637779753847,-0.390417825527865,0.));
#28656=DIRECTION('center_axis',(0.,0.,1.));
#28657=DIRECTION('ref_axis',(0.920637779753847,-0.390417825527865,0.));
#28658=DIRECTION('',(0.,0.,-1.));
#28659=DIRECTION('center_axis',(0.,0.,1.));
#28660=DIRECTION('ref_axis',(0.883107319487932,-0.469171037327369,0.));
#28661=DIRECTION('center_axis',(0.,0.,-1.));
#28662=DIRECTION('ref_axis',(0.883107319487932,-0.469171037327369,0.));
#28663=DIRECTION('center_axis',(0.,0.,1.));
#28664=DIRECTION('ref_axis',(0.883107319487932,-0.469171037327369,0.));
#28665=DIRECTION('',(0.,0.,-1.));
#28666=DIRECTION('center_axis',(0.,0.,1.));
#28667=DIRECTION('ref_axis',(0.838855879285935,-0.544353574239594,0.));
#28668=DIRECTION('center_axis',(0.,0.,-1.));
#28669=DIRECTION('ref_axis',(0.838855879285935,-0.544353574239594,0.));
#28670=DIRECTION('center_axis',(0.,0.,1.));
#28671=DIRECTION('ref_axis',(0.838855879285935,-0.544353574239594,0.));
#28672=DIRECTION('',(0.,0.,-1.));
#28673=DIRECTION('center_axis',(0.,0.,1.));
#28674=DIRECTION('ref_axis',(0.788220239327544,-0.61539325176218,0.));
#28675=DIRECTION('center_axis',(0.,0.,-1.));
#28676=DIRECTION('ref_axis',(0.788220239327544,-0.61539325176218,0.));
#28677=DIRECTION('center_axis',(0.,0.,1.));
#28678=DIRECTION('ref_axis',(0.788220239327544,-0.61539325176218,0.));
#28679=DIRECTION('',(0.,0.,-1.));
#28680=DIRECTION('center_axis',(0.,0.,1.));
#28681=DIRECTION('ref_axis',(0.731585767407476,-0.681749415054251,0.));
#28682=DIRECTION('center_axis',(0.,0.,-1.));
#28683=DIRECTION('ref_axis',(0.731585767407476,-0.681749415054251,0.));
#28684=DIRECTION('center_axis',(0.,0.,1.));
#28685=DIRECTION('ref_axis',(0.731585767407476,-0.681749415054251,0.));
#28686=DIRECTION('',(0.,0.,-1.));
#28687=DIRECTION('center_axis',(0.,0.,1.));
#28688=DIRECTION('ref_axis',(0.669383486053874,-0.742917053646208,0.));
#28689=DIRECTION('center_axis',(0.,0.,-1.));
#28690=DIRECTION('ref_axis',(0.669383486053874,-0.742917053646208,0.));
#28691=DIRECTION('center_axis',(0.,0.,1.));
#28692=DIRECTION('ref_axis',(0.669383486053874,-0.742917053646208,0.));
#28693=DIRECTION('',(0.,0.,-1.));
#28694=DIRECTION('center_axis',(0.,0.,1.));
#28695=DIRECTION('ref_axis',(0.602086792186603,-0.798430644874335,0.));
#28696=DIRECTION('center_axis',(0.,0.,-1.));
#28697=DIRECTION('ref_axis',(0.602086792186603,-0.798430644874335,0.));
#28698=DIRECTION('center_axis',(0.,0.,1.));
#28699=DIRECTION('ref_axis',(0.602086792186603,-0.798430644874335,0.));
#28700=DIRECTION('',(0.,0.,-1.));
#28701=DIRECTION('center_axis',(0.,0.,1.));
#28702=DIRECTION('ref_axis',(0.530207854280846,-0.847867696789364,0.));
#28703=DIRECTION('center_axis',(0.,0.,-1.));
#28704=DIRECTION('ref_axis',(0.530207854280846,-0.847867696789364,0.));
#28705=DIRECTION('center_axis',(0.,0.,1.));
#28706=DIRECTION('ref_axis',(0.530207854280846,-0.847867696789364,0.));
#28707=DIRECTION('',(0.,0.,-1.));
#28708=DIRECTION('center_axis',(0.,0.,1.));
#28709=DIRECTION('ref_axis',(0.454293714455755,-0.890851963575314,0.));
#28710=DIRECTION('center_axis',(0.,0.,-1.));
#28711=DIRECTION('ref_axis',(0.454293714455755,-0.890851963575314,0.));
#28712=DIRECTION('center_axis',(0.,0.,1.));
#28713=DIRECTION('ref_axis',(0.454293714455755,-0.890851963575314,0.));
#28714=DIRECTION('',(0.,0.,-1.));
#28715=DIRECTION('center_axis',(0.,0.,1.));
#28716=DIRECTION('ref_axis',(0.374922125153613,-0.927056309007332,0.));
#28717=DIRECTION('center_axis',(0.,0.,-1.));
#28718=DIRECTION('ref_axis',(0.374922125153613,-0.927056309007332,0.));
#28719=DIRECTION('center_axis',(0.,0.,1.));
#28720=DIRECTION('ref_axis',(0.374922125153613,-0.927056309007332,0.));
#28721=DIRECTION('',(0.,0.,-1.));
#28722=DIRECTION('center_axis',(0.,0.,1.));
#28723=DIRECTION('ref_axis',(0.292697152094883,-0.956205196155901,0.));
#28724=DIRECTION('center_axis',(0.,0.,-1.));
#28725=DIRECTION('ref_axis',(0.292697152094883,-0.956205196155901,0.));
#28726=DIRECTION('center_axis',(0.,0.,1.));
#28727=DIRECTION('ref_axis',(0.292697152094883,-0.956205196155901,0.));
#28728=DIRECTION('',(0.,0.,-1.));
#28729=DIRECTION('center_axis',(0.,0.,1.));
#28730=DIRECTION('ref_axis',(0.208244576973338,-0.97807678438924,0.));
#28731=DIRECTION('center_axis',(0.,0.,-1.));
#28732=DIRECTION('ref_axis',(0.208244576973338,-0.97807678438924,0.));
#28733=DIRECTION('center_axis',(0.,0.,1.));
#28734=DIRECTION('ref_axis',(0.208244576973338,-0.97807678438924,0.));
#28735=DIRECTION('',(0.,0.,-1.));
#28736=DIRECTION('center_axis',(0.,0.,1.));
#28737=DIRECTION('ref_axis',(0.122207134879512,-0.992504617714467,0.));
#28738=DIRECTION('center_axis',(0.,0.,-1.));
#28739=DIRECTION('ref_axis',(0.122207134879512,-0.992504617714467,0.));
#28740=DIRECTION('center_axis',(0.,0.,1.));
#28741=DIRECTION('ref_axis',(0.122207134879512,-0.992504617714467,0.));
#28742=DIRECTION('',(0.,0.,-1.));
#28743=DIRECTION('center_axis',(0.,0.,1.));
#28744=DIRECTION('ref_axis',(0.0352396226985678,-0.999378891608214,0.));
#28745=DIRECTION('center_axis',(0.,0.,-1.));
#28746=DIRECTION('ref_axis',(0.0352396226985678,-0.999378891608214,0.));
#28747=DIRECTION('center_axis',(0.,0.,1.));
#28748=DIRECTION('ref_axis',(0.0352396226985678,-0.999378891608214,0.));
#28749=DIRECTION('',(0.,0.,-1.));
#28750=DIRECTION('center_axis',(0.,0.,1.));
#28751=DIRECTION('ref_axis',(-0.0519960842893783,-0.998647288695349,0.));
#28752=DIRECTION('center_axis',(0.,0.,-1.));
#28753=DIRECTION('ref_axis',(-0.0519960842893783,-0.998647288695349,0.));
#28754=DIRECTION('center_axis',(0.,0.,1.));
#28755=DIRECTION('ref_axis',(-0.0519960842893783,-0.998647288695349,0.));
#28756=DIRECTION('',(0.,0.,-1.));
#28757=DIRECTION('center_axis',(0.,0.,1.));
#28758=DIRECTION('ref_axis',(-0.138836069679788,-0.990315376915793,0.));
#28759=DIRECTION('center_axis',(0.,0.,-1.));
#28760=DIRECTION('ref_axis',(-0.138836069679788,-0.990315376915793,0.));
#28761=DIRECTION('center_axis',(0.,0.,1.));
#28762=DIRECTION('ref_axis',(-0.138836069679788,-0.990315376915793,0.));
#28763=DIRECTION('',(0.,0.,-1.));
#28764=DIRECTION('center_axis',(0.,0.,1.));
#28765=DIRECTION('ref_axis',(-0.224619428748424,-0.974446567149134,0.));
#28766=DIRECTION('center_axis',(0.,0.,-1.));
#28767=DIRECTION('ref_axis',(-0.224619428748424,-0.974446567149134,0.));
#28768=DIRECTION('center_axis',(0.,0.,1.));
#28769=DIRECTION('ref_axis',(-0.224619428748424,-0.974446567149134,0.));
#28770=DIRECTION('',(0.,0.,-1.));
#28771=DIRECTION('center_axis',(0.,0.,1.));
#28772=DIRECTION('ref_axis',(-0.308693298335366,-0.951161630619545,0.));
#28773=DIRECTION('center_axis',(0.,0.,-1.));
#28774=DIRECTION('ref_axis',(-0.308693298335366,-0.951161630619545,0.));
#28775=DIRECTION('center_axis',(0.,0.,1.));
#28776=DIRECTION('ref_axis',(-0.308693298335366,-0.951161630619545,0.));
#28777=DIRECTION('',(0.,0.,-1.));
#28778=DIRECTION('center_axis',(0.,0.,1.));
#28779=DIRECTION('ref_axis',(-0.390417825527865,-0.920637779753847,0.));
#28780=DIRECTION('center_axis',(0.,0.,-1.));
#28781=DIRECTION('ref_axis',(-0.390417825527865,-0.920637779753847,0.));
#28782=DIRECTION('center_axis',(0.,0.,1.));
#28783=DIRECTION('ref_axis',(-0.390417825527865,-0.920637779753847,0.));
#28784=DIRECTION('',(0.,0.,-1.));
#28785=DIRECTION('center_axis',(0.,0.,1.));
#28786=DIRECTION('ref_axis',(-0.469171037327369,-0.883107319487932,0.));
#28787=DIRECTION('center_axis',(0.,0.,-1.));
#28788=DIRECTION('ref_axis',(-0.469171037327369,-0.883107319487932,0.));
#28789=DIRECTION('center_axis',(0.,0.,1.));
#28790=DIRECTION('ref_axis',(-0.469171037327369,-0.883107319487932,0.));
#28791=DIRECTION('',(0.,0.,-1.));
#28792=DIRECTION('center_axis',(0.,0.,1.));
#28793=DIRECTION('ref_axis',(-0.544353574239594,-0.838855879285935,0.));
#28794=DIRECTION('center_axis',(0.,0.,-1.));
#28795=DIRECTION('ref_axis',(-0.544353574239594,-0.838855879285935,0.));
#28796=DIRECTION('center_axis',(0.,0.,1.));
#28797=DIRECTION('ref_axis',(-0.544353574239594,-0.838855879285935,0.));
#28798=DIRECTION('',(0.,0.,-1.));
#28799=DIRECTION('center_axis',(0.,0.,1.));
#28800=DIRECTION('ref_axis',(-0.61539325176218,-0.788220239327544,0.));
#28801=DIRECTION('center_axis',(0.,0.,-1.));
#28802=DIRECTION('ref_axis',(-0.61539325176218,-0.788220239327544,0.));
#28803=DIRECTION('center_axis',(0.,0.,1.));
#28804=DIRECTION('ref_axis',(-0.61539325176218,-0.788220239327544,0.));
#28805=DIRECTION('',(0.,0.,-1.));
#28806=DIRECTION('center_axis',(0.,0.,1.));
#28807=DIRECTION('ref_axis',(-0.681749415054251,-0.731585767407477,0.));
#28808=DIRECTION('center_axis',(0.,0.,-1.));
#28809=DIRECTION('ref_axis',(-0.681749415054251,-0.731585767407477,0.));
#28810=DIRECTION('center_axis',(0.,0.,1.));
#28811=DIRECTION('ref_axis',(-0.681749415054251,-0.731585767407477,0.));
#28812=DIRECTION('',(0.,0.,-1.));
#28813=DIRECTION('center_axis',(0.,0.,1.));
#28814=DIRECTION('ref_axis',(-0.742917053646208,-0.669383486053874,0.));
#28815=DIRECTION('center_axis',(0.,0.,-1.));
#28816=DIRECTION('ref_axis',(-0.742917053646208,-0.669383486053874,0.));
#28817=DIRECTION('center_axis',(0.,0.,1.));
#28818=DIRECTION('ref_axis',(-0.742917053646208,-0.669383486053874,0.));
#28819=DIRECTION('',(0.,0.,-1.));
#28820=DIRECTION('center_axis',(0.,0.,1.));
#28821=DIRECTION('ref_axis',(-0.798430644874335,-0.602086792186602,0.));
#28822=DIRECTION('center_axis',(0.,0.,-1.));
#28823=DIRECTION('ref_axis',(-0.798430644874335,-0.602086792186602,0.));
#28824=DIRECTION('center_axis',(0.,0.,1.));
#28825=DIRECTION('ref_axis',(-0.798430644874335,-0.602086792186602,0.));
#28826=DIRECTION('',(0.,0.,-1.));
#28827=DIRECTION('center_axis',(0.,0.,1.));
#28828=DIRECTION('ref_axis',(-0.847867696789364,-0.530207854280845,0.));
#28829=DIRECTION('center_axis',(0.,0.,-1.));
#28830=DIRECTION('ref_axis',(-0.847867696789364,-0.530207854280845,0.));
#28831=DIRECTION('center_axis',(0.,0.,1.));
#28832=DIRECTION('ref_axis',(-0.847867696789364,-0.530207854280845,0.));
#28833=DIRECTION('',(0.,0.,-1.));
#28834=DIRECTION('center_axis',(0.,0.,1.));
#28835=DIRECTION('ref_axis',(-0.890851963575314,-0.454293714455756,0.));
#28836=DIRECTION('center_axis',(0.,0.,-1.));
#28837=DIRECTION('ref_axis',(-0.890851963575314,-0.454293714455756,0.));
#28838=DIRECTION('center_axis',(0.,0.,1.));
#28839=DIRECTION('ref_axis',(-0.890851963575314,-0.454293714455756,0.));
#28840=DIRECTION('',(0.,0.,-1.));
#28841=DIRECTION('center_axis',(0.,0.,1.));
#28842=DIRECTION('ref_axis',(-0.927056309007332,-0.374922125153613,0.));
#28843=DIRECTION('center_axis',(0.,0.,-1.));
#28844=DIRECTION('ref_axis',(-0.927056309007332,-0.374922125153613,0.));
#28845=DIRECTION('center_axis',(0.,0.,1.));
#28846=DIRECTION('ref_axis',(-0.927056309007332,-0.374922125153613,0.));
#28847=DIRECTION('',(0.,0.,-1.));
#28848=DIRECTION('center_axis',(0.,0.,1.));
#28849=DIRECTION('ref_axis',(-0.956205196155901,-0.292697152094883,0.));
#28850=DIRECTION('center_axis',(0.,0.,-1.));
#28851=DIRECTION('ref_axis',(-0.956205196155901,-0.292697152094883,0.));
#28852=DIRECTION('center_axis',(0.,0.,1.));
#28853=DIRECTION('ref_axis',(-0.956205196155901,-0.292697152094883,0.));
#28854=DIRECTION('',(0.,0.,-1.));
#28855=DIRECTION('center_axis',(0.,0.,1.));
#28856=DIRECTION('ref_axis',(-0.97807678438924,-0.208244576973338,0.));
#28857=DIRECTION('center_axis',(0.,0.,-1.));
#28858=DIRECTION('ref_axis',(-0.97807678438924,-0.208244576973338,0.));
#28859=DIRECTION('center_axis',(0.,0.,1.));
#28860=DIRECTION('ref_axis',(-0.97807678438924,-0.208244576973338,0.));
#28861=DIRECTION('',(0.,0.,-1.));
#28862=DIRECTION('center_axis',(0.,0.,1.));
#28863=DIRECTION('ref_axis',(-0.992504617714467,-0.122207134879512,0.));
#28864=DIRECTION('center_axis',(0.,0.,-1.));
#28865=DIRECTION('ref_axis',(-0.992504617714467,-0.122207134879512,0.));
#28866=DIRECTION('center_axis',(0.,0.,1.));
#28867=DIRECTION('ref_axis',(-0.992504617714467,-0.122207134879512,0.));
#28868=DIRECTION('',(0.,0.,-1.));
#28869=DIRECTION('center_axis',(0.,0.,1.));
#28870=DIRECTION('ref_axis',(-0.999378891608214,-0.0352396226985679,0.));
#28871=DIRECTION('center_axis',(0.,0.,-1.));
#28872=DIRECTION('ref_axis',(-0.999378891608214,-0.0352396226985679,0.));
#28873=DIRECTION('center_axis',(0.,0.,1.));
#28874=DIRECTION('ref_axis',(-0.999378891608214,-0.0352396226985679,0.));
#28875=DIRECTION('',(0.,0.,-1.));
#28876=DIRECTION('center_axis',(0.,0.,1.));
#28877=DIRECTION('ref_axis',(-0.998647288695349,0.0519960842893783,0.));
#28878=DIRECTION('center_axis',(0.,0.,-1.));
#28879=DIRECTION('ref_axis',(-0.998647288695349,0.0519960842893783,0.));
#28880=DIRECTION('center_axis',(0.,0.,1.));
#28881=DIRECTION('ref_axis',(-0.998647288695349,0.0519960842893783,0.));
#28882=DIRECTION('',(0.,0.,-1.));
#28883=DIRECTION('center_axis',(0.,0.,1.));
#28884=DIRECTION('ref_axis',(-0.990315376915793,0.138836069679789,0.));
#28885=DIRECTION('center_axis',(0.,0.,-1.));
#28886=DIRECTION('ref_axis',(-0.990315376915793,0.138836069679789,0.));
#28887=DIRECTION('center_axis',(0.,0.,1.));
#28888=DIRECTION('ref_axis',(-0.990315376915793,0.138836069679789,0.));
#28889=DIRECTION('',(0.,0.,-1.));
#28890=DIRECTION('center_axis',(0.,0.,1.));
#28891=DIRECTION('ref_axis',(-0.974446567149134,0.224619428748424,0.));
#28892=DIRECTION('center_axis',(0.,0.,-1.));
#28893=DIRECTION('ref_axis',(-0.974446567149134,0.224619428748424,0.));
#28894=DIRECTION('center_axis',(0.,0.,1.));
#28895=DIRECTION('ref_axis',(-0.974446567149134,0.224619428748424,0.));
#28896=DIRECTION('',(0.,0.,-1.));
#28897=DIRECTION('center_axis',(0.,0.,1.));
#28898=DIRECTION('ref_axis',(-0.951161630619546,0.308693298335365,0.));
#28899=DIRECTION('center_axis',(0.,0.,-1.));
#28900=DIRECTION('ref_axis',(-0.951161630619546,0.308693298335365,0.));
#28901=DIRECTION('center_axis',(0.,0.,1.));
#28902=DIRECTION('ref_axis',(-0.951161630619546,0.308693298335365,0.));
#28903=DIRECTION('',(0.,0.,-1.));
#28904=DIRECTION('center_axis',(0.,0.,1.));
#28905=DIRECTION('ref_axis',(-0.920637779753848,0.390417825527865,0.));
#28906=DIRECTION('center_axis',(0.,0.,-1.));
#28907=DIRECTION('ref_axis',(-0.920637779753848,0.390417825527865,0.));
#28908=DIRECTION('center_axis',(0.,0.,1.));
#28909=DIRECTION('ref_axis',(-0.920637779753848,0.390417825527865,0.));
#28910=DIRECTION('',(0.,0.,-1.));
#28911=DIRECTION('center_axis',(0.,0.,1.));
#28912=DIRECTION('ref_axis',(-0.883107319487933,0.469171037327368,0.));
#28913=DIRECTION('center_axis',(0.,0.,-1.));
#28914=DIRECTION('ref_axis',(-0.883107319487933,0.469171037327368,0.));
#28915=DIRECTION('center_axis',(0.,0.,1.));
#28916=DIRECTION('ref_axis',(-0.883107319487933,0.469171037327368,0.));
#28917=DIRECTION('',(0.,0.,-1.));
#28918=DIRECTION('center_axis',(0.,0.,1.));
#28919=DIRECTION('ref_axis',(-0.838855879285935,0.544353574239593,0.));
#28920=DIRECTION('center_axis',(0.,0.,-1.));
#28921=DIRECTION('ref_axis',(-0.838855879285935,0.544353574239593,0.));
#28922=DIRECTION('center_axis',(0.,0.,1.));
#28923=DIRECTION('ref_axis',(-0.838855879285935,0.544353574239593,0.));
#28924=DIRECTION('',(0.,0.,-1.));
#28925=DIRECTION('center_axis',(0.,0.,1.));
#28926=DIRECTION('ref_axis',(-0.788220239327544,0.61539325176218,0.));
#28927=DIRECTION('center_axis',(0.,0.,-1.));
#28928=DIRECTION('ref_axis',(-0.788220239327544,0.61539325176218,0.));
#28929=DIRECTION('center_axis',(0.,0.,1.));
#28930=DIRECTION('ref_axis',(-0.788220239327544,0.61539325176218,0.));
#28931=DIRECTION('',(0.,0.,-1.));
#28932=DIRECTION('center_axis',(0.,0.,1.));
#28933=DIRECTION('ref_axis',(-0.731585767407477,0.681749415054251,0.));
#28934=DIRECTION('center_axis',(0.,0.,-1.));
#28935=DIRECTION('ref_axis',(-0.731585767407477,0.681749415054251,0.));
#28936=DIRECTION('center_axis',(0.,0.,1.));
#28937=DIRECTION('ref_axis',(-0.731585767407477,0.681749415054251,0.));
#28938=DIRECTION('',(0.,0.,-1.));
#28939=DIRECTION('center_axis',(0.,0.,1.));
#28940=DIRECTION('ref_axis',(-0.669383486053874,0.742917053646208,0.));
#28941=DIRECTION('center_axis',(0.,0.,-1.));
#28942=DIRECTION('ref_axis',(-0.669383486053874,0.742917053646208,0.));
#28943=DIRECTION('center_axis',(0.,0.,1.));
#28944=DIRECTION('ref_axis',(-0.669383486053874,0.742917053646208,0.));
#28945=DIRECTION('',(0.,0.,-1.));
#28946=DIRECTION('center_axis',(0.,0.,1.));
#28947=DIRECTION('ref_axis',(-0.602086792186602,0.798430644874335,0.));
#28948=DIRECTION('center_axis',(0.,0.,-1.));
#28949=DIRECTION('ref_axis',(-0.602086792186602,0.798430644874335,0.));
#28950=DIRECTION('center_axis',(0.,0.,1.));
#28951=DIRECTION('ref_axis',(-0.602086792186602,0.798430644874335,0.));
#28952=DIRECTION('',(0.,0.,-1.));
#28953=DIRECTION('center_axis',(0.,0.,1.));
#28954=DIRECTION('ref_axis',(-0.530207854280846,0.847867696789364,0.));
#28955=DIRECTION('center_axis',(0.,0.,-1.));
#28956=DIRECTION('ref_axis',(-0.530207854280846,0.847867696789364,0.));
#28957=DIRECTION('center_axis',(0.,0.,1.));
#28958=DIRECTION('ref_axis',(-0.530207854280846,0.847867696789364,0.));
#28959=DIRECTION('',(0.,0.,-1.));
#28960=DIRECTION('center_axis',(0.,0.,1.));
#28961=DIRECTION('ref_axis',(-0.454293714455756,0.890851963575314,0.));
#28962=DIRECTION('center_axis',(0.,0.,-1.));
#28963=DIRECTION('ref_axis',(-0.454293714455756,0.890851963575314,0.));
#28964=DIRECTION('center_axis',(0.,0.,1.));
#28965=DIRECTION('ref_axis',(-0.454293714455756,0.890851963575314,0.));
#28966=DIRECTION('',(0.,0.,-1.));
#28967=DIRECTION('center_axis',(0.,0.,1.));
#28968=DIRECTION('ref_axis',(-0.374922125153613,0.927056309007332,0.));
#28969=DIRECTION('center_axis',(0.,0.,-1.));
#28970=DIRECTION('ref_axis',(-0.374922125153613,0.927056309007332,0.));
#28971=DIRECTION('center_axis',(0.,0.,1.));
#28972=DIRECTION('ref_axis',(-0.374922125153613,0.927056309007332,0.));
#28973=DIRECTION('',(0.,0.,-1.));
#28974=DIRECTION('center_axis',(0.,0.,1.));
#28975=DIRECTION('ref_axis',(-0.292697152094883,0.956205196155901,0.));
#28976=DIRECTION('center_axis',(0.,0.,-1.));
#28977=DIRECTION('ref_axis',(-0.292697152094883,0.956205196155901,0.));
#28978=DIRECTION('center_axis',(0.,0.,1.));
#28979=DIRECTION('ref_axis',(-0.292697152094883,0.956205196155901,0.));
#28980=DIRECTION('',(0.,0.,-1.));
#28981=DIRECTION('center_axis',(0.,0.,1.));
#28982=DIRECTION('ref_axis',(-0.208244576973338,0.97807678438924,0.));
#28983=DIRECTION('center_axis',(0.,0.,-1.));
#28984=DIRECTION('ref_axis',(-0.208244576973338,0.97807678438924,0.));
#28985=DIRECTION('center_axis',(0.,0.,1.));
#28986=DIRECTION('ref_axis',(-0.208244576973338,0.97807678438924,0.));
#28987=DIRECTION('',(0.,0.,-1.));
#28988=DIRECTION('center_axis',(0.,0.,1.));
#28989=DIRECTION('ref_axis',(-0.122207134879512,0.992504617714467,0.));
#28990=DIRECTION('center_axis',(0.,0.,-1.));
#28991=DIRECTION('ref_axis',(-0.122207134879512,0.992504617714467,0.));
#28992=DIRECTION('center_axis',(0.,0.,1.));
#28993=DIRECTION('ref_axis',(-0.122207134879512,0.992504617714467,0.));
#28994=DIRECTION('',(0.,0.,-1.));
#28995=DIRECTION('center_axis',(0.,0.,1.));
#28996=DIRECTION('ref_axis',(-0.035239622698568,0.999378891608214,0.));
#28997=DIRECTION('center_axis',(0.,0.,-1.));
#28998=DIRECTION('ref_axis',(-0.035239622698568,0.999378891608214,0.));
#28999=DIRECTION('center_axis',(0.,0.,1.));
#29000=DIRECTION('ref_axis',(-0.035239622698568,0.999378891608214,0.));
#29001=DIRECTION('',(0.,0.,-1.));
#29002=DIRECTION('center_axis',(0.,0.,1.));
#29003=DIRECTION('ref_axis',(0.0519960842893784,0.998647288695349,0.));
#29004=DIRECTION('center_axis',(0.,0.,-1.));
#29005=DIRECTION('ref_axis',(0.0519960842893784,0.998647288695349,0.));
#29006=DIRECTION('center_axis',(0.,0.,1.));
#29007=DIRECTION('ref_axis',(0.0519960842893784,0.998647288695349,0.));
#29008=DIRECTION('',(0.,0.,-1.));
#29009=DIRECTION('center_axis',(0.,0.,1.));
#29010=DIRECTION('ref_axis',(0.138836069679788,0.990315376915793,0.));
#29011=DIRECTION('center_axis',(0.,0.,-1.));
#29012=DIRECTION('ref_axis',(0.138836069679788,0.990315376915793,0.));
#29013=DIRECTION('center_axis',(0.,0.,1.));
#29014=DIRECTION('ref_axis',(0.138836069679788,0.990315376915793,0.));
#29015=DIRECTION('',(0.,0.,-1.));
#29016=DIRECTION('center_axis',(0.,0.,1.));
#29017=DIRECTION('ref_axis',(0.224619428748424,0.974446567149134,0.));
#29018=DIRECTION('center_axis',(0.,0.,-1.));
#29019=DIRECTION('ref_axis',(0.224619428748424,0.974446567149134,0.));
#29020=DIRECTION('center_axis',(0.,0.,1.));
#29021=DIRECTION('ref_axis',(0.224619428748424,0.974446567149134,0.));
#29022=DIRECTION('',(0.,0.,-1.));
#29023=DIRECTION('center_axis',(0.,0.,1.));
#29024=DIRECTION('ref_axis',(0.308693298335365,0.951161630619546,0.));
#29025=DIRECTION('center_axis',(0.,0.,-1.));
#29026=DIRECTION('ref_axis',(0.308693298335365,0.951161630619546,0.));
#29027=DIRECTION('center_axis',(0.,0.,1.));
#29028=DIRECTION('ref_axis',(0.308693298335365,0.951161630619546,0.));
#29029=DIRECTION('',(0.,0.,-1.));
#29030=DIRECTION('center_axis',(0.,0.,1.));
#29031=DIRECTION('ref_axis',(0.390417825527865,0.920637779753848,0.));
#29032=DIRECTION('center_axis',(0.,0.,-1.));
#29033=DIRECTION('ref_axis',(0.390417825527865,0.920637779753848,0.));
#29034=DIRECTION('center_axis',(0.,0.,1.));
#29035=DIRECTION('ref_axis',(0.390417825527865,0.920637779753848,0.));
#29036=DIRECTION('',(0.,0.,-1.));
#29037=DIRECTION('center_axis',(0.,0.,1.));
#29038=DIRECTION('ref_axis',(0.469171037327368,0.883107319487932,0.));
#29039=DIRECTION('center_axis',(0.,0.,-1.));
#29040=DIRECTION('ref_axis',(0.469171037327368,0.883107319487932,0.));
#29041=DIRECTION('center_axis',(0.,0.,1.));
#29042=DIRECTION('ref_axis',(0.469171037327368,0.883107319487932,0.));
#29043=DIRECTION('',(0.,0.,-1.));
#29044=DIRECTION('center_axis',(0.,0.,1.));
#29045=DIRECTION('ref_axis',(0.544353574239593,0.838855879285935,0.));
#29046=DIRECTION('center_axis',(0.,0.,-1.));
#29047=DIRECTION('ref_axis',(0.544353574239593,0.838855879285935,0.));
#29048=DIRECTION('center_axis',(0.,0.,1.));
#29049=DIRECTION('ref_axis',(0.544353574239593,0.838855879285935,0.));
#29050=DIRECTION('',(0.,0.,-1.));
#29051=DIRECTION('center_axis',(0.,0.,1.));
#29052=DIRECTION('ref_axis',(0.61539325176218,0.788220239327544,0.));
#29053=DIRECTION('center_axis',(0.,0.,-1.));
#29054=DIRECTION('ref_axis',(0.61539325176218,0.788220239327544,0.));
#29055=DIRECTION('center_axis',(0.,0.,1.));
#29056=DIRECTION('ref_axis',(0.61539325176218,0.788220239327544,0.));
#29057=DIRECTION('',(0.,0.,-1.));
#29058=DIRECTION('center_axis',(0.,0.,1.));
#29059=DIRECTION('ref_axis',(0.681749415054251,0.731585767407477,0.));
#29060=DIRECTION('center_axis',(0.,0.,-1.));
#29061=DIRECTION('ref_axis',(0.681749415054251,0.731585767407477,0.));
#29062=DIRECTION('center_axis',(0.,0.,1.));
#29063=DIRECTION('ref_axis',(0.681749415054251,0.731585767407477,0.));
#29064=DIRECTION('',(0.,0.,-1.));
#29065=DIRECTION('center_axis',(0.,0.,1.));
#29066=DIRECTION('ref_axis',(0.742917053646208,0.669383486053874,0.));
#29067=DIRECTION('center_axis',(0.,0.,-1.));
#29068=DIRECTION('ref_axis',(0.742917053646208,0.669383486053874,0.));
#29069=DIRECTION('center_axis',(0.,0.,1.));
#29070=DIRECTION('ref_axis',(0.742917053646208,0.669383486053874,0.));
#29071=DIRECTION('',(0.,0.,-1.));
#29072=DIRECTION('center_axis',(0.,0.,1.));
#29073=DIRECTION('ref_axis',(0.798430644874335,0.602086792186603,0.));
#29074=DIRECTION('center_axis',(0.,0.,-1.));
#29075=DIRECTION('ref_axis',(0.798430644874335,0.602086792186603,0.));
#29076=DIRECTION('center_axis',(0.,0.,1.));
#29077=DIRECTION('ref_axis',(0.798430644874335,0.602086792186603,0.));
#29078=DIRECTION('',(0.,0.,-1.));
#29079=DIRECTION('center_axis',(0.,0.,1.));
#29080=DIRECTION('ref_axis',(0.847867696789364,0.530207854280846,0.));
#29081=DIRECTION('center_axis',(0.,0.,-1.));
#29082=DIRECTION('ref_axis',(0.847867696789364,0.530207854280846,0.));
#29083=DIRECTION('center_axis',(0.,0.,1.));
#29084=DIRECTION('ref_axis',(0.847867696789364,0.530207854280846,0.));
#29085=DIRECTION('',(0.,0.,-1.));
#29086=DIRECTION('center_axis',(0.,0.,1.));
#29087=DIRECTION('ref_axis',(0.890851963575314,0.454293714455756,0.));
#29088=DIRECTION('center_axis',(0.,0.,-1.));
#29089=DIRECTION('ref_axis',(0.890851963575314,0.454293714455756,0.));
#29090=DIRECTION('center_axis',(0.,0.,1.));
#29091=DIRECTION('ref_axis',(0.890851963575314,0.454293714455756,0.));
#29092=DIRECTION('',(0.,0.,-1.));
#29093=DIRECTION('center_axis',(0.,0.,1.));
#29094=DIRECTION('ref_axis',(0.927056309007332,0.374922125153613,0.));
#29095=DIRECTION('center_axis',(0.,0.,-1.));
#29096=DIRECTION('ref_axis',(0.927056309007332,0.374922125153613,0.));
#29097=DIRECTION('center_axis',(0.,0.,1.));
#29098=DIRECTION('ref_axis',(0.927056309007332,0.374922125153613,0.));
#29099=DIRECTION('',(0.,0.,-1.));
#29100=DIRECTION('center_axis',(0.,0.,1.));
#29101=DIRECTION('ref_axis',(0.956205196155901,0.292697152094883,0.));
#29102=DIRECTION('center_axis',(0.,0.,-1.));
#29103=DIRECTION('ref_axis',(0.956205196155901,0.292697152094883,0.));
#29104=DIRECTION('center_axis',(0.,0.,1.));
#29105=DIRECTION('ref_axis',(0.956205196155901,0.292697152094883,0.));
#29106=DIRECTION('',(0.,0.,-1.));
#29107=DIRECTION('center_axis',(0.,0.,1.));
#29108=DIRECTION('ref_axis',(0.97807678438924,0.208244576973338,0.));
#29109=DIRECTION('center_axis',(0.,0.,-1.));
#29110=DIRECTION('ref_axis',(0.97807678438924,0.208244576973338,0.));
#29111=DIRECTION('center_axis',(0.,0.,1.));
#29112=DIRECTION('ref_axis',(0.97807678438924,0.208244576973338,0.));
#29113=DIRECTION('',(0.,0.,-1.));
#29114=DIRECTION('center_axis',(0.,0.,1.));
#29115=DIRECTION('ref_axis',(0.992504617714467,0.122207134879512,0.));
#29116=DIRECTION('center_axis',(0.,0.,-1.));
#29117=DIRECTION('ref_axis',(0.992504617714467,0.122207134879512,0.));
#29118=DIRECTION('center_axis',(0.,0.,1.));
#29119=DIRECTION('ref_axis',(0.992504617714467,0.122207134879512,0.));
#29120=DIRECTION('',(0.,0.,1.));
#29121=DIRECTION('',(0.,0.,1.));
#29122=DIRECTION('',(0.,0.,1.));
#29123=DIRECTION('',(0.,0.,1.));
#29124=DIRECTION('',(0.,0.,1.));
#29125=DIRECTION('',(0.,0.,1.));
#29126=DIRECTION('',(0.,0.,1.));
#29127=DIRECTION('',(0.,0.,1.));
#29128=DIRECTION('',(0.,0.,1.));
#29129=DIRECTION('',(0.,0.,1.));
#29130=DIRECTION('',(0.,0.,1.));
#29131=DIRECTION('',(0.,0.,1.));
#29132=DIRECTION('',(0.,0.,1.));
#29133=DIRECTION('',(0.,0.,1.));
#29134=DIRECTION('',(0.,0.,1.));
#29135=DIRECTION('',(0.,0.,1.));
#29136=DIRECTION('',(0.,0.,1.));
#29137=DIRECTION('',(0.,0.,1.));
#29138=DIRECTION('',(0.,0.,1.));
#29139=DIRECTION('',(0.,0.,1.));
#29140=DIRECTION('',(0.,0.,1.));
#29141=DIRECTION('',(0.,0.,1.));
#29142=DIRECTION('',(0.,0.,1.));
#29143=DIRECTION('',(0.,0.,1.));
#29144=DIRECTION('',(0.,0.,1.));
#29145=DIRECTION('',(0.,0.,1.));
#29146=DIRECTION('',(0.,0.,1.));
#29147=DIRECTION('',(0.,0.,1.));
#29148=DIRECTION('',(0.,0.,1.));
#29149=DIRECTION('',(0.,0.,1.));
#29150=DIRECTION('',(0.,0.,1.));
#29151=DIRECTION('',(0.,0.,1.));
#29152=DIRECTION('',(0.,0.,1.));
#29153=DIRECTION('',(0.,0.,1.));
#29154=DIRECTION('',(0.,0.,1.));
#29155=DIRECTION('',(0.,0.,1.));
#29156=DIRECTION('',(0.,0.,1.));
#29157=DIRECTION('',(0.,0.,1.));
#29158=DIRECTION('',(0.,0.,1.));
#29159=DIRECTION('',(0.,0.,1.));
#29160=DIRECTION('',(0.,0.,1.));
#29161=DIRECTION('',(0.,0.,1.));
#29162=DIRECTION('',(0.,0.,1.));
#29163=DIRECTION('',(0.,0.,1.));
#29164=DIRECTION('',(0.,0.,1.));
#29165=DIRECTION('',(0.,0.,1.));
#29166=DIRECTION('',(0.,0.,1.));
#29167=DIRECTION('',(0.,0.,1.));
#29168=DIRECTION('',(0.,0.,1.));
#29169=DIRECTION('',(0.,0.,1.));
#29170=DIRECTION('',(0.,0.,1.));
#29171=DIRECTION('',(0.,0.,1.));
#29172=DIRECTION('',(0.,0.,1.));
#29173=DIRECTION('',(0.,0.,1.));
#29174=DIRECTION('',(0.,0.,1.));
#29175=DIRECTION('',(0.,0.,1.));
#29176=DIRECTION('',(0.,0.,1.));
#29177=DIRECTION('',(0.,0.,1.));
#29178=DIRECTION('',(0.,0.,1.));
#29179=DIRECTION('',(0.,0.,1.));
#29180=DIRECTION('',(0.,0.,1.));
#29181=DIRECTION('',(0.,0.,1.));
#29182=DIRECTION('',(0.,0.,1.));
#29183=DIRECTION('',(0.,0.,1.));
#29184=DIRECTION('',(0.,0.,1.));
#29185=DIRECTION('',(0.,0.,1.));
#29186=DIRECTION('',(0.,0.,1.));
#29187=DIRECTION('',(0.,0.,1.));
#29188=DIRECTION('',(0.,0.,1.));
#29189=DIRECTION('',(0.,0.,1.));
#29190=DIRECTION('',(0.,0.,1.));
#29191=DIRECTION('center_axis',(0.,0.,1.));
#29192=DIRECTION('ref_axis',(1.,0.,0.));
#29193=DIRECTION('center_axis',(0.,0.,-1.));
#29194=DIRECTION('ref_axis',(1.,0.,0.));
#29195=DIRECTION('',(0.,0.,1.));
#29196=DIRECTION('center_axis',(0.,0.,-1.));
#29197=DIRECTION('ref_axis',(1.,0.,0.));
#29198=DIRECTION('center_axis',(0.,0.,1.));
#29199=DIRECTION('ref_axis',(1.,0.,0.));
#29200=DIRECTION('center_axis',(0.,0.,-1.));
#29201=DIRECTION('ref_axis',(1.,0.,0.));
#29202=DIRECTION('center_axis',(0.,0.,-1.));
#29203=DIRECTION('ref_axis',(1.,0.,0.));
#29204=DIRECTION('center_axis',(0.,0.,1.));
#29205=DIRECTION('ref_axis',(1.,0.,0.));
#29206=DIRECTION('center_axis',(0.,0.,-1.));
#29207=DIRECTION('ref_axis',(1.,0.,0.));
#29208=DIRECTION('center_axis',(0.,0.,-1.));
#29209=DIRECTION('ref_axis',(1.,0.,0.));
#29210=DIRECTION('center_axis',(0.,0.,1.));
#29211=DIRECTION('ref_axis',(1.,0.,0.));
#29212=DIRECTION('center_axis',(0.,0.,-1.));
#29213=DIRECTION('ref_axis',(1.,0.,0.));
#29214=DIRECTION('center_axis',(0.,0.,-1.));
#29215=DIRECTION('ref_axis',(1.,0.,0.));
#29216=DIRECTION('center_axis',(0.,0.,1.));
#29217=DIRECTION('ref_axis',(1.,0.,0.));
#29218=DIRECTION('center_axis',(0.,0.,-1.));
#29219=DIRECTION('ref_axis',(1.,0.,0.));
#29220=DIRECTION('center_axis',(0.,0.,-1.));
#29221=DIRECTION('ref_axis',(1.,0.,0.));
#29222=DIRECTION('center_axis',(0.,0.,1.));
#29223=DIRECTION('ref_axis',(1.,0.,0.));
#29224=DIRECTION('center_axis',(0.,0.,-1.));
#29225=DIRECTION('ref_axis',(1.,0.,0.));
#29226=DIRECTION('center_axis',(0.,0.,-1.));
#29227=DIRECTION('ref_axis',(1.,0.,0.));
#29228=DIRECTION('center_axis',(0.,0.,1.));
#29229=DIRECTION('ref_axis',(1.,0.,0.));
#29230=DIRECTION('center_axis',(0.,0.,-1.));
#29231=DIRECTION('ref_axis',(1.,0.,0.));
#29232=DIRECTION('center_axis',(0.,0.,-1.));
#29233=DIRECTION('ref_axis',(1.,0.,0.));
#29234=DIRECTION('center_axis',(0.,0.,1.));
#29235=DIRECTION('ref_axis',(1.,0.,0.));
#29236=DIRECTION('center_axis',(0.,0.,-1.));
#29237=DIRECTION('ref_axis',(1.,0.,0.));
#29238=DIRECTION('center_axis',(0.,0.,-1.));
#29239=DIRECTION('ref_axis',(1.,0.,0.));
#29240=DIRECTION('center_axis',(0.,0.,1.));
#29241=DIRECTION('ref_axis',(1.,0.,0.));
#29242=DIRECTION('center_axis',(0.,0.,-1.));
#29243=DIRECTION('ref_axis',(1.,0.,0.));
#29244=DIRECTION('center_axis',(0.,0.,-1.));
#29245=DIRECTION('ref_axis',(1.,0.,0.));
#29246=DIRECTION('center_axis',(0.,0.,1.));
#29247=DIRECTION('ref_axis',(1.,0.,0.));
#29248=DIRECTION('center_axis',(0.,0.,-1.));
#29249=DIRECTION('ref_axis',(1.,0.,0.));
#29250=DIRECTION('center_axis',(0.,0.,-1.));
#29251=DIRECTION('ref_axis',(1.,0.,0.));
#29252=DIRECTION('center_axis',(0.,0.,1.));
#29253=DIRECTION('ref_axis',(1.,0.,0.));
#29254=DIRECTION('center_axis',(0.,0.,-1.));
#29255=DIRECTION('ref_axis',(1.,0.,0.));
#29256=DIRECTION('center_axis',(0.,0.,-1.));
#29257=DIRECTION('ref_axis',(1.,0.,0.));
#29258=DIRECTION('center_axis',(0.,0.,1.));
#29259=DIRECTION('ref_axis',(1.,0.,0.));
#29260=DIRECTION('center_axis',(0.,0.,-1.));
#29261=DIRECTION('ref_axis',(1.,0.,0.));
#29262=DIRECTION('center_axis',(0.,0.,-1.));
#29263=DIRECTION('ref_axis',(1.,0.,0.));
#29264=DIRECTION('center_axis',(0.,0.,1.));
#29265=DIRECTION('ref_axis',(1.,0.,0.));
#29266=DIRECTION('center_axis',(0.,0.,-1.));
#29267=DIRECTION('ref_axis',(1.,0.,0.));
#29268=DIRECTION('center_axis',(0.,0.,-1.));
#29269=DIRECTION('ref_axis',(1.,0.,0.));
#29270=DIRECTION('center_axis',(0.,0.,1.));
#29271=DIRECTION('ref_axis',(1.,0.,0.));
#29272=DIRECTION('center_axis',(0.,0.,-1.));
#29273=DIRECTION('ref_axis',(1.,0.,0.));
#29274=DIRECTION('center_axis',(0.,0.,-1.));
#29275=DIRECTION('ref_axis',(1.,0.,0.));
#29276=DIRECTION('center_axis',(0.,0.,1.));
#29277=DIRECTION('ref_axis',(1.,0.,0.));
#29278=DIRECTION('center_axis',(0.,0.,-1.));
#29279=DIRECTION('ref_axis',(1.,0.,0.));
#29280=DIRECTION('center_axis',(0.,0.,-1.));
#29281=DIRECTION('ref_axis',(1.,0.,0.));
#29282=DIRECTION('center_axis',(0.,0.,1.));
#29283=DIRECTION('ref_axis',(1.,0.,0.));
#29284=DIRECTION('center_axis',(0.,0.,-1.));
#29285=DIRECTION('ref_axis',(1.,0.,0.));
#29286=DIRECTION('center_axis',(0.,0.,-1.));
#29287=DIRECTION('ref_axis',(1.,0.,0.));
#29288=DIRECTION('center_axis',(0.,0.,1.));
#29289=DIRECTION('ref_axis',(1.,0.,0.));
#29290=DIRECTION('center_axis',(0.,0.,-1.));
#29291=DIRECTION('ref_axis',(1.,0.,0.));
#29292=DIRECTION('center_axis',(0.,0.,-1.));
#29293=DIRECTION('ref_axis',(1.,0.,0.));
#29294=DIRECTION('center_axis',(0.,0.,1.));
#29295=DIRECTION('ref_axis',(1.,0.,0.));
#29296=DIRECTION('center_axis',(0.,0.,-1.));
#29297=DIRECTION('ref_axis',(1.,0.,0.));
#29298=DIRECTION('center_axis',(0.,0.,-1.));
#29299=DIRECTION('ref_axis',(1.,0.,0.));
#29300=DIRECTION('center_axis',(0.,0.,1.));
#29301=DIRECTION('ref_axis',(1.,0.,0.));
#29302=DIRECTION('center_axis',(0.,0.,-1.));
#29303=DIRECTION('ref_axis',(1.,0.,0.));
#29304=DIRECTION('center_axis',(0.,0.,-1.));
#29305=DIRECTION('ref_axis',(1.,0.,0.));
#29306=DIRECTION('center_axis',(0.,0.,1.));
#29307=DIRECTION('ref_axis',(1.,0.,0.));
#29308=DIRECTION('center_axis',(0.,0.,-1.));
#29309=DIRECTION('ref_axis',(1.,0.,0.));
#29310=DIRECTION('center_axis',(0.,0.,-1.));
#29311=DIRECTION('ref_axis',(1.,0.,0.));
#29312=DIRECTION('center_axis',(0.,0.,1.));
#29313=DIRECTION('ref_axis',(1.,0.,0.));
#29314=DIRECTION('center_axis',(0.,0.,-1.));
#29315=DIRECTION('ref_axis',(1.,0.,0.));
#29316=DIRECTION('center_axis',(0.,0.,-1.));
#29317=DIRECTION('ref_axis',(1.,0.,0.));
#29318=DIRECTION('center_axis',(0.,0.,1.));
#29319=DIRECTION('ref_axis',(1.,0.,0.));
#29320=DIRECTION('center_axis',(0.,0.,-1.));
#29321=DIRECTION('ref_axis',(1.,0.,0.));
#29322=DIRECTION('center_axis',(0.,0.,-1.));
#29323=DIRECTION('ref_axis',(1.,0.,0.));
#29324=DIRECTION('center_axis',(0.,0.,1.));
#29325=DIRECTION('ref_axis',(1.,0.,0.));
#29326=DIRECTION('center_axis',(0.,0.,-1.));
#29327=DIRECTION('ref_axis',(1.,0.,0.));
#29328=DIRECTION('center_axis',(0.,0.,-1.));
#29329=DIRECTION('ref_axis',(1.,0.,0.));
#29330=DIRECTION('center_axis',(0.,0.,1.));
#29331=DIRECTION('ref_axis',(1.,0.,0.));
#29332=DIRECTION('center_axis',(0.,0.,-1.));
#29333=DIRECTION('ref_axis',(1.,0.,0.));
#29334=DIRECTION('center_axis',(0.,0.,-1.));
#29335=DIRECTION('ref_axis',(1.,0.,0.));
#29336=DIRECTION('center_axis',(0.,0.,1.));
#29337=DIRECTION('ref_axis',(1.,0.,0.));
#29338=DIRECTION('center_axis',(0.,0.,-1.));
#29339=DIRECTION('ref_axis',(1.,0.,0.));
#29340=DIRECTION('center_axis',(0.,0.,-1.));
#29341=DIRECTION('ref_axis',(1.,0.,0.));
#29342=DIRECTION('center_axis',(0.,0.,1.));
#29343=DIRECTION('ref_axis',(1.,0.,0.));
#29344=DIRECTION('center_axis',(0.,0.,-1.));
#29345=DIRECTION('ref_axis',(1.,0.,0.));
#29346=DIRECTION('center_axis',(0.,0.,-1.));
#29347=DIRECTION('ref_axis',(1.,0.,0.));
#29348=DIRECTION('center_axis',(0.,0.,1.));
#29349=DIRECTION('ref_axis',(1.,0.,0.));
#29350=DIRECTION('center_axis',(0.,0.,-1.));
#29351=DIRECTION('ref_axis',(1.,0.,0.));
#29352=DIRECTION('center_axis',(0.,0.,-1.));
#29353=DIRECTION('ref_axis',(1.,0.,0.));
#29354=DIRECTION('center_axis',(0.,0.,1.));
#29355=DIRECTION('ref_axis',(1.,0.,0.));
#29356=DIRECTION('center_axis',(0.,0.,-1.));
#29357=DIRECTION('ref_axis',(1.,0.,0.));
#29358=DIRECTION('center_axis',(0.,0.,-1.));
#29359=DIRECTION('ref_axis',(1.,0.,0.));
#29360=DIRECTION('center_axis',(0.,0.,1.));
#29361=DIRECTION('ref_axis',(1.,0.,0.));
#29362=DIRECTION('center_axis',(0.,0.,-1.));
#29363=DIRECTION('ref_axis',(1.,0.,0.));
#29364=DIRECTION('center_axis',(0.,0.,-1.));
#29365=DIRECTION('ref_axis',(1.,0.,0.));
#29366=DIRECTION('center_axis',(0.,0.,1.));
#29367=DIRECTION('ref_axis',(1.,0.,0.));
#29368=DIRECTION('center_axis',(0.,0.,-1.));
#29369=DIRECTION('ref_axis',(1.,0.,0.));
#29370=DIRECTION('center_axis',(0.,0.,-1.));
#29371=DIRECTION('ref_axis',(1.,0.,0.));
#29372=DIRECTION('center_axis',(0.,0.,1.));
#29373=DIRECTION('ref_axis',(1.,0.,0.));
#29374=DIRECTION('center_axis',(0.,0.,-1.));
#29375=DIRECTION('ref_axis',(1.,0.,0.));
#29376=DIRECTION('center_axis',(0.,0.,-1.));
#29377=DIRECTION('ref_axis',(1.,0.,0.));
#29378=DIRECTION('center_axis',(0.,0.,1.));
#29379=DIRECTION('ref_axis',(1.,0.,0.));
#29380=DIRECTION('center_axis',(0.,0.,-1.));
#29381=DIRECTION('ref_axis',(1.,0.,0.));
#29382=DIRECTION('center_axis',(0.,0.,-1.));
#29383=DIRECTION('ref_axis',(1.,0.,0.));
#29384=DIRECTION('center_axis',(0.,0.,1.));
#29385=DIRECTION('ref_axis',(1.,0.,0.));
#29386=DIRECTION('center_axis',(0.,0.,-1.));
#29387=DIRECTION('ref_axis',(1.,0.,0.));
#29388=DIRECTION('center_axis',(0.,0.,-1.));
#29389=DIRECTION('ref_axis',(1.,0.,0.));
#29390=DIRECTION('center_axis',(0.,0.,1.));
#29391=DIRECTION('ref_axis',(1.,0.,0.));
#29392=DIRECTION('center_axis',(0.,0.,-1.));
#29393=DIRECTION('ref_axis',(1.,0.,0.));
#29394=DIRECTION('center_axis',(0.,0.,-1.));
#29395=DIRECTION('ref_axis',(1.,0.,0.));
#29396=DIRECTION('center_axis',(0.,0.,1.));
#29397=DIRECTION('ref_axis',(1.,0.,0.));
#29398=DIRECTION('center_axis',(0.,0.,-1.));
#29399=DIRECTION('ref_axis',(1.,0.,0.));
#29400=DIRECTION('center_axis',(0.,0.,-1.));
#29401=DIRECTION('ref_axis',(1.,0.,0.));
#29402=DIRECTION('center_axis',(0.,0.,1.));
#29403=DIRECTION('ref_axis',(-1.,-1.22464679914735E-16,0.));
#29404=DIRECTION('center_axis',(0.,0.,-1.));
#29405=DIRECTION('ref_axis',(1.,0.,0.));
#29406=DIRECTION('center_axis',(0.,0.,-1.));
#29407=DIRECTION('ref_axis',(1.,0.,0.));
#29408=DIRECTION('center_axis',(0.,0.,1.));
#29409=DIRECTION('ref_axis',(1.,0.,0.));
#29410=DIRECTION('center_axis',(0.,0.,-1.));
#29411=DIRECTION('ref_axis',(1.,0.,0.));
#29412=DIRECTION('center_axis',(0.,0.,-1.));
#29413=DIRECTION('ref_axis',(1.,0.,0.));
#29414=DIRECTION('center_axis',(0.,0.,1.));
#29415=DIRECTION('ref_axis',(1.,0.,0.));
#29416=DIRECTION('center_axis',(0.,0.,-1.));
#29417=DIRECTION('ref_axis',(1.,0.,0.));
#29418=DIRECTION('center_axis',(0.,0.,-1.));
#29419=DIRECTION('ref_axis',(1.,0.,0.));
#29420=DIRECTION('center_axis',(0.,0.,1.));
#29421=DIRECTION('ref_axis',(1.,0.,0.));
#29422=DIRECTION('center_axis',(0.,0.,-1.));
#29423=DIRECTION('ref_axis',(1.,0.,0.));
#29424=DIRECTION('center_axis',(0.,0.,-1.));
#29425=DIRECTION('ref_axis',(1.,0.,0.));
#29426=DIRECTION('center_axis',(0.,0.,1.));
#29427=DIRECTION('ref_axis',(1.,0.,0.));
#29428=DIRECTION('center_axis',(0.,0.,-1.));
#29429=DIRECTION('ref_axis',(1.,0.,0.));
#29430=DIRECTION('center_axis',(0.,0.,-1.));
#29431=DIRECTION('ref_axis',(1.,0.,0.));
#29432=DIRECTION('center_axis',(0.,0.,1.));
#29433=DIRECTION('ref_axis',(1.,0.,0.));
#29434=DIRECTION('center_axis',(0.,0.,-1.));
#29435=DIRECTION('ref_axis',(1.,0.,0.));
#29436=DIRECTION('center_axis',(0.,0.,-1.));
#29437=DIRECTION('ref_axis',(1.,0.,0.));
#29438=DIRECTION('center_axis',(0.,0.,1.));
#29439=DIRECTION('ref_axis',(1.,0.,0.));
#29440=DIRECTION('center_axis',(0.,0.,-1.));
#29441=DIRECTION('ref_axis',(1.,0.,0.));
#29442=DIRECTION('center_axis',(0.,0.,-1.));
#29443=DIRECTION('ref_axis',(1.,0.,0.));
#29444=DIRECTION('center_axis',(0.,0.,1.));
#29445=DIRECTION('ref_axis',(1.,0.,0.));
#29446=DIRECTION('center_axis',(0.,0.,-1.));
#29447=DIRECTION('ref_axis',(1.,0.,0.));
#29448=DIRECTION('center_axis',(0.,0.,-1.));
#29449=DIRECTION('ref_axis',(1.,0.,0.));
#29450=DIRECTION('center_axis',(0.,0.,1.));
#29451=DIRECTION('ref_axis',(1.,0.,0.));
#29452=DIRECTION('center_axis',(0.,0.,-1.));
#29453=DIRECTION('ref_axis',(1.,0.,0.));
#29454=DIRECTION('center_axis',(0.,0.,-1.));
#29455=DIRECTION('ref_axis',(1.,0.,0.));
#29456=DIRECTION('center_axis',(0.,0.,1.));
#29457=DIRECTION('ref_axis',(1.,0.,0.));
#29458=DIRECTION('center_axis',(0.,0.,-1.));
#29459=DIRECTION('ref_axis',(1.,0.,0.));
#29460=DIRECTION('center_axis',(0.,0.,-1.));
#29461=DIRECTION('ref_axis',(1.,0.,0.));
#29462=DIRECTION('center_axis',(0.,0.,1.));
#29463=DIRECTION('ref_axis',(1.,0.,0.));
#29464=DIRECTION('center_axis',(0.,0.,-1.));
#29465=DIRECTION('ref_axis',(1.,0.,0.));
#29466=DIRECTION('center_axis',(0.,0.,-1.));
#29467=DIRECTION('ref_axis',(1.,0.,0.));
#29468=DIRECTION('center_axis',(0.,0.,1.));
#29469=DIRECTION('ref_axis',(1.,0.,0.));
#29470=DIRECTION('center_axis',(0.,0.,-1.));
#29471=DIRECTION('ref_axis',(1.,0.,0.));
#29472=DIRECTION('center_axis',(0.,0.,-1.));
#29473=DIRECTION('ref_axis',(1.,0.,0.));
#29474=DIRECTION('center_axis',(0.,0.,1.));
#29475=DIRECTION('ref_axis',(1.,0.,0.));
#29476=DIRECTION('center_axis',(0.,0.,-1.));
#29477=DIRECTION('ref_axis',(1.,0.,0.));
#29478=DIRECTION('center_axis',(0.,0.,-1.));
#29479=DIRECTION('ref_axis',(1.,0.,0.));
#29480=DIRECTION('center_axis',(0.,0.,1.));
#29481=DIRECTION('ref_axis',(1.,0.,0.));
#29482=DIRECTION('center_axis',(0.,0.,-1.));
#29483=DIRECTION('ref_axis',(1.,0.,0.));
#29484=DIRECTION('center_axis',(0.,0.,-1.));
#29485=DIRECTION('ref_axis',(1.,0.,0.));
#29486=DIRECTION('center_axis',(0.,0.,1.));
#29487=DIRECTION('ref_axis',(1.,0.,0.));
#29488=DIRECTION('center_axis',(0.,0.,-1.));
#29489=DIRECTION('ref_axis',(1.,0.,0.));
#29490=DIRECTION('center_axis',(0.,0.,-1.));
#29491=DIRECTION('ref_axis',(1.,0.,0.));
#29492=DIRECTION('center_axis',(0.,0.,1.));
#29493=DIRECTION('ref_axis',(1.,0.,0.));
#29494=DIRECTION('center_axis',(0.,0.,-1.));
#29495=DIRECTION('ref_axis',(1.,0.,0.));
#29496=DIRECTION('center_axis',(0.,0.,-1.));
#29497=DIRECTION('ref_axis',(1.,0.,0.));
#29498=DIRECTION('center_axis',(0.,0.,1.));
#29499=DIRECTION('ref_axis',(1.,0.,0.));
#29500=DIRECTION('center_axis',(0.,0.,-1.));
#29501=DIRECTION('ref_axis',(1.,0.,0.));
#29502=DIRECTION('center_axis',(0.,0.,-1.));
#29503=DIRECTION('ref_axis',(1.,0.,0.));
#29504=DIRECTION('center_axis',(0.,0.,1.));
#29505=DIRECTION('ref_axis',(1.,0.,0.));
#29506=DIRECTION('center_axis',(0.,0.,-1.));
#29507=DIRECTION('ref_axis',(1.,0.,0.));
#29508=DIRECTION('center_axis',(0.,0.,-1.));
#29509=DIRECTION('ref_axis',(1.,0.,0.));
#29510=DIRECTION('center_axis',(0.,0.,1.));
#29511=DIRECTION('ref_axis',(1.,0.,0.));
#29512=DIRECTION('center_axis',(0.,0.,-1.));
#29513=DIRECTION('ref_axis',(1.,0.,0.));
#29514=DIRECTION('center_axis',(0.,0.,-1.));
#29515=DIRECTION('ref_axis',(1.,0.,0.));
#29516=DIRECTION('center_axis',(0.,0.,1.));
#29517=DIRECTION('ref_axis',(1.,0.,0.));
#29518=DIRECTION('center_axis',(0.,0.,-1.));
#29519=DIRECTION('ref_axis',(1.,0.,0.));
#29520=DIRECTION('center_axis',(0.,0.,-1.));
#29521=DIRECTION('ref_axis',(1.,0.,0.));
#29522=DIRECTION('center_axis',(0.,0.,1.));
#29523=DIRECTION('ref_axis',(1.,0.,0.));
#29524=DIRECTION('center_axis',(0.,0.,-1.));
#29525=DIRECTION('ref_axis',(1.,0.,0.));
#29526=DIRECTION('center_axis',(0.,0.,-1.));
#29527=DIRECTION('ref_axis',(1.,0.,0.));
#29528=DIRECTION('center_axis',(0.,0.,1.));
#29529=DIRECTION('ref_axis',(1.,0.,0.));
#29530=DIRECTION('center_axis',(0.,0.,-1.));
#29531=DIRECTION('ref_axis',(1.,0.,0.));
#29532=DIRECTION('center_axis',(0.,0.,-1.));
#29533=DIRECTION('ref_axis',(1.,0.,0.));
#29534=DIRECTION('center_axis',(0.,0.,1.));
#29535=DIRECTION('ref_axis',(1.,0.,0.));
#29536=DIRECTION('center_axis',(0.,0.,-1.));
#29537=DIRECTION('ref_axis',(1.,0.,0.));
#29538=DIRECTION('center_axis',(0.,0.,-1.));
#29539=DIRECTION('ref_axis',(1.,0.,0.));
#29540=DIRECTION('center_axis',(0.,0.,1.));
#29541=DIRECTION('ref_axis',(1.,0.,0.));
#29542=DIRECTION('center_axis',(0.,0.,-1.));
#29543=DIRECTION('ref_axis',(1.,0.,0.));
#29544=DIRECTION('center_axis',(0.,0.,-1.));
#29545=DIRECTION('ref_axis',(1.,0.,0.));
#29546=DIRECTION('center_axis',(0.,0.,1.));
#29547=DIRECTION('ref_axis',(1.,0.,0.));
#29548=DIRECTION('center_axis',(0.,0.,-1.));
#29549=DIRECTION('ref_axis',(1.,0.,0.));
#29550=DIRECTION('center_axis',(0.,0.,-1.));
#29551=DIRECTION('ref_axis',(1.,0.,0.));
#29552=DIRECTION('center_axis',(0.,0.,1.));
#29553=DIRECTION('ref_axis',(1.,0.,0.));
#29554=DIRECTION('center_axis',(0.,0.,-1.));
#29555=DIRECTION('ref_axis',(1.,0.,0.));
#29556=DIRECTION('center_axis',(0.,0.,-1.));
#29557=DIRECTION('ref_axis',(1.,0.,0.));
#29558=DIRECTION('center_axis',(0.,0.,1.));
#29559=DIRECTION('ref_axis',(1.,0.,0.));
#29560=DIRECTION('center_axis',(0.,0.,-1.));
#29561=DIRECTION('ref_axis',(1.,0.,0.));
#29562=DIRECTION('center_axis',(0.,0.,-1.));
#29563=DIRECTION('ref_axis',(1.,0.,0.));
#29564=DIRECTION('center_axis',(0.,0.,1.));
#29565=DIRECTION('ref_axis',(1.,0.,0.));
#29566=DIRECTION('center_axis',(0.,0.,-1.));
#29567=DIRECTION('ref_axis',(1.,0.,0.));
#29568=DIRECTION('center_axis',(0.,0.,-1.));
#29569=DIRECTION('ref_axis',(1.,0.,0.));
#29570=DIRECTION('center_axis',(0.,0.,1.));
#29571=DIRECTION('ref_axis',(1.,0.,0.));
#29572=DIRECTION('center_axis',(0.,0.,-1.));
#29573=DIRECTION('ref_axis',(1.,0.,0.));
#29574=DIRECTION('center_axis',(0.,0.,-1.));
#29575=DIRECTION('ref_axis',(1.,0.,0.));
#29576=DIRECTION('center_axis',(0.,0.,1.));
#29577=DIRECTION('ref_axis',(1.,0.,0.));
#29578=DIRECTION('center_axis',(0.,0.,-1.));
#29579=DIRECTION('ref_axis',(1.,0.,0.));
#29580=DIRECTION('center_axis',(0.,0.,-1.));
#29581=DIRECTION('ref_axis',(1.,0.,0.));
#29582=DIRECTION('center_axis',(0.,0.,1.));
#29583=DIRECTION('ref_axis',(1.,0.,0.));
#29584=DIRECTION('center_axis',(0.,0.,-1.));
#29585=DIRECTION('ref_axis',(1.,0.,0.));
#29586=DIRECTION('center_axis',(0.,0.,-1.));
#29587=DIRECTION('ref_axis',(1.,0.,0.));
#29588=DIRECTION('center_axis',(0.,0.,1.));
#29589=DIRECTION('ref_axis',(1.,0.,0.));
#29590=DIRECTION('center_axis',(0.,0.,-1.));
#29591=DIRECTION('ref_axis',(1.,0.,0.));
#29592=DIRECTION('center_axis',(0.,0.,-1.));
#29593=DIRECTION('ref_axis',(1.,0.,0.));
#29594=DIRECTION('center_axis',(0.,0.,1.));
#29595=DIRECTION('ref_axis',(1.,0.,0.));
#29596=DIRECTION('center_axis',(0.,0.,-1.));
#29597=DIRECTION('ref_axis',(1.,0.,0.));
#29598=DIRECTION('center_axis',(0.,0.,-1.));
#29599=DIRECTION('ref_axis',(1.,0.,0.));
#29600=DIRECTION('center_axis',(0.,0.,1.));
#29601=DIRECTION('ref_axis',(1.,0.,0.));
#29602=DIRECTION('center_axis',(0.,0.,-1.));
#29603=DIRECTION('ref_axis',(1.,0.,0.));
#29604=DIRECTION('center_axis',(0.,0.,-1.));
#29605=DIRECTION('ref_axis',(1.,0.,0.));
#29606=DIRECTION('center_axis',(0.,0.,1.));
#29607=DIRECTION('ref_axis',(1.,0.,0.));
#29608=DIRECTION('center_axis',(0.,0.,-1.));
#29609=DIRECTION('ref_axis',(1.,0.,0.));
#29610=DIRECTION('center_axis',(0.,0.,-1.));
#29611=DIRECTION('ref_axis',(1.,0.,0.));
#29612=DIRECTION('center_axis',(0.,0.,1.));
#29613=DIRECTION('ref_axis',(1.,0.,0.));
#29614=DIRECTION('center_axis',(0.,0.,-1.));
#29615=DIRECTION('ref_axis',(1.,0.,0.));
#29616=DIRECTION('',(0.,0.,-1.));
#29617=DIRECTION('center_axis',(0.,0.,-1.));
#29618=DIRECTION('ref_axis',(1.,0.,0.));
#29619=DIRECTION('center_axis',(0.,0.,1.));
#29620=DIRECTION('ref_axis',(0.999378891608214,0.035239622698568,0.));
#29621=DIRECTION('center_axis',(0.,0.,-1.));
#29622=DIRECTION('ref_axis',(0.999378891608214,0.035239622698568,0.));
#29623=DIRECTION('center_axis',(0.,0.,1.));
#29624=DIRECTION('ref_axis',(0.999378891608214,0.035239622698568,0.));
#29625=DIRECTION('center_axis',(0.,0.,1.));
#29626=DIRECTION('ref_axis',(1.,0.,0.));
#29627=DIRECTION('center_axis',(0.,0.,1.));
#29628=DIRECTION('ref_axis',(1.,0.,0.));
#29629=DIRECTION('center_axis',(0.,0.,-1.));
#29630=DIRECTION('ref_axis',(1.,0.,0.));
#29631=DIRECTION('center_axis',(0.,0.,1.));
#29632=DIRECTION('ref_axis',(1.,0.,0.));
#29633=DIRECTION('center_axis',(0.,0.,-1.));
#29634=DIRECTION('ref_axis',(1.,0.,0.));
#29635=DIRECTION('center_axis',(0.,0.,1.));
#29636=DIRECTION('ref_axis',(1.,0.,0.));
#29637=DIRECTION('',(0.,0.,-1.));
#29638=DIRECTION('',(0.,0.,-1.));
#29639=DIRECTION('center_axis',(0.,0.,1.));
#29640=DIRECTION('ref_axis',(1.,0.,0.));
#29641=DIRECTION('center_axis',(0.,0.,1.));
#29642=DIRECTION('ref_axis',(1.,0.,0.));
#52395=CARTESIAN_POINT('',(0.,0.,0.));
#52396=CARTESIAN_POINT('Origin',(0.,-86.,6.));
#52397=CARTESIAN_POINT('',(0.,-90.,8.));
#52398=CARTESIAN_POINT('',(0.,-90.,4.));
#52399=CARTESIAN_POINT('Ctrl Pts',(-2.08166817117217E-16,-90.,8.));
#52400=CARTESIAN_POINT('Ctrl Pts',(0.251133328053566,-90.,8.));
#52401=CARTESIAN_POINT('Ctrl Pts',(0.519000232590761,-89.9988407998655,
7.94980925763969));
#52402=CARTESIAN_POINT('Ctrl Pts',(1.01175644254643,-89.9946501491172,7.74569936791146));
#52403=CARTESIAN_POINT('Ctrl Pts',(1.23664644642618,-89.9916787455059,7.59178067832001));
#52404=CARTESIAN_POINT('Ctrl Pts',(1.59178067978086,-89.9860976603374,7.23664644496533));
#52405=CARTESIAN_POINT('Ctrl Pts',(1.74569936855887,-89.9831259365723,7.01175644187864));
#52406=CARTESIAN_POINT('Ctrl Pts',(1.94980925677131,-89.9789345539658,6.51900023379203));
#52407=CARTESIAN_POINT('Ctrl Pts',(2.,-89.9777750336159,6.25113333011964));
#52408=CARTESIAN_POINT('Ctrl Pts',(2.,-89.9777750336159,5.74886666988036));
#52409=CARTESIAN_POINT('Ctrl Pts',(1.94980925677131,-89.9789345539658,5.48099976620797));
#52410=CARTESIAN_POINT('Ctrl Pts',(1.74569936855887,-89.9831259365723,4.98824355812136));
#52411=CARTESIAN_POINT('Ctrl Pts',(1.59178067978086,-89.9860976603374,4.76335355503467));
#52412=CARTESIAN_POINT('Ctrl Pts',(1.23664644642618,-89.9916787455059,4.40821932167999));
#52413=CARTESIAN_POINT('Ctrl Pts',(1.01175644254643,-89.9946501491172,4.25430063208854));
#52414=CARTESIAN_POINT('Ctrl Pts',(0.519000232590762,-89.9988407998655,
4.05019074236031));
#52415=CARTESIAN_POINT('Ctrl Pts',(0.251133328053567,-90.,4.));
#52416=CARTESIAN_POINT('Ctrl Pts',(5.55111512312578E-16,-90.,4.));
#52417=CARTESIAN_POINT('',(2.44929359829471E-16,-82.,8.));
#52418=CARTESIAN_POINT('',(2.44929359829471E-16,-86.,8.));
#52419=CARTESIAN_POINT('Origin',(0.,-82.,6.));
#52420=CARTESIAN_POINT('Ctrl Pts',(4.85722573273506E-16,-90.,4.));
#52421=CARTESIAN_POINT('Ctrl Pts',(-0.251133328053566,-90.,4.));
#52422=CARTESIAN_POINT('Ctrl Pts',(-0.519000232590761,-89.9988407998655,
4.05019074236031));
#52423=CARTESIAN_POINT('Ctrl Pts',(-1.01175644254643,-89.9946501491172,
4.25430063208854));
#52424=CARTESIAN_POINT('Ctrl Pts',(-1.23664644642618,-89.9916787455059,
4.40821932167999));
#52425=CARTESIAN_POINT('Ctrl Pts',(-1.59178067978086,-89.9860976603374,
4.76335355503467));
#52426=CARTESIAN_POINT('Ctrl Pts',(-1.74569936855887,-89.9831259365723,
4.98824355812136));
#52427=CARTESIAN_POINT('Ctrl Pts',(-1.94980925677131,-89.9789345539658,
5.48099976620797));
#52428=CARTESIAN_POINT('Ctrl Pts',(-2.,-89.9777750336159,5.74886666988036));
#52429=CARTESIAN_POINT('Ctrl Pts',(-2.,-89.9777750336159,6.));
#52430=CARTESIAN_POINT('Ctrl Pts',(-2.,-89.9777750336159,6.25113333011964));
#52431=CARTESIAN_POINT('Ctrl Pts',(-1.94980925677131,-89.9789345539658,
6.51900023379203));
#52432=CARTESIAN_POINT('Ctrl Pts',(-1.74569936855887,-89.9831259365723,
7.01175644187864));
#52433=CARTESIAN_POINT('Ctrl Pts',(-1.59178067978086,-89.9860976603374,
7.23664644496533));
#52434=CARTESIAN_POINT('Ctrl Pts',(-1.23664644642618,-89.9916787455059,
7.59178067832001));
#52435=CARTESIAN_POINT('Ctrl Pts',(-1.01175644254643,-89.9946501491172,
7.74569936791146));
#52436=CARTESIAN_POINT('Ctrl Pts',(-0.519000232590761,-89.9988407998655,
7.94980925763969));
#52437=CARTESIAN_POINT('Ctrl Pts',(-0.251133328053566,-90.,8.));
#52438=CARTESIAN_POINT('Ctrl Pts',(-2.08166817117217E-16,-90.,8.));
#52439=CARTESIAN_POINT('Origin',(0.,-82.,6.));
#52440=CARTESIAN_POINT('Origin',(0.,86.,6.));
#52441=CARTESIAN_POINT('',(0.,90.,8.));
#52442=CARTESIAN_POINT('',(0.,90.,4.));
#52443=CARTESIAN_POINT('Ctrl Pts',(0.,90.,8.));
#52444=CARTESIAN_POINT('Ctrl Pts',(-0.251133328053566,90.,8.));
#52445=CARTESIAN_POINT('Ctrl Pts',(-0.519000232590761,89.9988407998655,
7.94980925763969));
#52446=CARTESIAN_POINT('Ctrl Pts',(-1.01175644254643,89.9946501491172,7.74569936791146));
#52447=CARTESIAN_POINT('Ctrl Pts',(-1.23664644642618,89.9916787455059,7.59178067832001));
#52448=CARTESIAN_POINT('Ctrl Pts',(-1.59178067978086,89.9860976603374,7.23664644496533));
#52449=CARTESIAN_POINT('Ctrl Pts',(-1.74569936855886,89.9831259365723,7.01175644187864));
#52450=CARTESIAN_POINT('Ctrl Pts',(-1.94980925677131,89.9789345539658,6.51900023379203));
#52451=CARTESIAN_POINT('Ctrl Pts',(-2.,89.9777750336159,6.25113333011964));
#52452=CARTESIAN_POINT('Ctrl Pts',(-2.,89.9777750336159,5.74886666988036));
#52453=CARTESIAN_POINT('Ctrl Pts',(-1.94980925677131,89.9789345539658,5.48099976620797));
#52454=CARTESIAN_POINT('Ctrl Pts',(-1.74569936855887,89.9831259365723,4.98824355812136));
#52455=CARTESIAN_POINT('Ctrl Pts',(-1.59178067978086,89.9860976603374,4.76335355503467));
#52456=CARTESIAN_POINT('Ctrl Pts',(-1.23664644642618,89.9916787455059,4.40821932167999));
#52457=CARTESIAN_POINT('Ctrl Pts',(-1.01175644254643,89.9946501491172,4.25430063208854));
#52458=CARTESIAN_POINT('Ctrl Pts',(-0.519000232590762,89.9988407998655,
4.05019074236031));
#52459=CARTESIAN_POINT('Ctrl Pts',(-0.251133328053566,90.,4.));
#52460=CARTESIAN_POINT('Ctrl Pts',(-2.08166817117217E-16,90.,4.));
#52461=CARTESIAN_POINT('Ctrl Pts',(-4.85722573273506E-16,90.,4.));
#52462=CARTESIAN_POINT('Ctrl Pts',(0.251133328053566,90.,4.));
#52463=CARTESIAN_POINT('Ctrl Pts',(0.519000232590762,89.9988407998655,4.05019074236031));
#52464=CARTESIAN_POINT('Ctrl Pts',(1.01175644254643,89.9946501491172,4.25430063208854));
#52465=CARTESIAN_POINT('Ctrl Pts',(1.23664644642618,89.9916787455059,4.40821932167999));
#52466=CARTESIAN_POINT('Ctrl Pts',(1.59178067978086,89.9860976603374,4.76335355503467));
#52467=CARTESIAN_POINT('Ctrl Pts',(1.74569936855886,89.9831259365723,4.98824355812136));
#52468=CARTESIAN_POINT('Ctrl Pts',(1.94980925677131,89.9789345539658,5.48099976620797));
#52469=CARTESIAN_POINT('Ctrl Pts',(2.,89.9777750336159,5.74886666988036));
#52470=CARTESIAN_POINT('Ctrl Pts',(2.,89.9777750336159,6.));
#52471=CARTESIAN_POINT('Ctrl Pts',(2.,89.9777750336159,6.25113333011964));
#52472=CARTESIAN_POINT('Ctrl Pts',(1.94980925677131,89.9789345539658,6.51900023379203));
#52473=CARTESIAN_POINT('Ctrl Pts',(1.74569936855887,89.9831259365723,7.01175644187864));
#52474=CARTESIAN_POINT('Ctrl Pts',(1.59178067978086,89.9860976603374,7.23664644496533));
#52475=CARTESIAN_POINT('Ctrl Pts',(1.23664644642618,89.9916787455059,7.59178067832001));
#52476=CARTESIAN_POINT('Ctrl Pts',(1.01175644254643,89.9946501491172,7.74569936791146));
#52477=CARTESIAN_POINT('Ctrl Pts',(0.519000232590761,89.9988407998655,7.94980925763969));
#52478=CARTESIAN_POINT('Ctrl Pts',(0.251133328053566,90.,8.));
#52479=CARTESIAN_POINT('Ctrl Pts',(-6.93889390390723E-17,90.,8.));
#52480=CARTESIAN_POINT('',(2.44929359829471E-16,82.,4.));
#52481=CARTESIAN_POINT('',(2.44929359829471E-16,86.,4.));
#52482=CARTESIAN_POINT('Origin',(0.,82.,6.));
#52483=CARTESIAN_POINT('Origin',(0.,82.,6.));
#52484=CARTESIAN_POINT('Origin',(-86.,0.,6.));
#52485=CARTESIAN_POINT('',(-90.,0.,8.));
#52486=CARTESIAN_POINT('',(-90.,0.,4.));
#52487=CARTESIAN_POINT('Ctrl Pts',(-90.,2.77555756156289E-16,8.));
#52488=CARTESIAN_POINT('Ctrl Pts',(-90.,-0.251133328053566,8.));
#52489=CARTESIAN_POINT('Ctrl Pts',(-89.9988407998655,-0.519000232590761,
7.94980925763969));
#52490=CARTESIAN_POINT('Ctrl Pts',(-89.9946501491172,-1.01175644254643,
7.74569936791146));
#52491=CARTESIAN_POINT('Ctrl Pts',(-89.9916787455059,-1.23664644642618,
7.59178067832001));
#52492=CARTESIAN_POINT('Ctrl Pts',(-89.9860976603374,-1.59178067978086,
7.23664644496533));
#52493=CARTESIAN_POINT('Ctrl Pts',(-89.9831259365723,-1.74569936855887,
7.01175644187864));
#52494=CARTESIAN_POINT('Ctrl Pts',(-89.9789345539658,-1.94980925677131,
6.51900023379203));
#52495=CARTESIAN_POINT('Ctrl Pts',(-89.9777750336159,-2.,6.25113333011964));
#52496=CARTESIAN_POINT('Ctrl Pts',(-89.9777750336159,-2.,5.74886666988036));
#52497=CARTESIAN_POINT('Ctrl Pts',(-89.9789345539658,-1.94980925677131,
5.48099976620797));
#52498=CARTESIAN_POINT('Ctrl Pts',(-89.9831259365723,-1.74569936855887,
4.98824355812136));
#52499=CARTESIAN_POINT('Ctrl Pts',(-89.9860976603374,-1.59178067978086,
4.76335355503467));
#52500=CARTESIAN_POINT('Ctrl Pts',(-89.9916787455059,-1.23664644642618,
4.40821932167999));
#52501=CARTESIAN_POINT('Ctrl Pts',(-89.9946501491172,-1.01175644254643,
4.25430063208854));
#52502=CARTESIAN_POINT('Ctrl Pts',(-89.9988407998655,-0.519000232590762,
4.05019074236031));
#52503=CARTESIAN_POINT('Ctrl Pts',(-90.,-0.251133328053567,4.));
#52504=CARTESIAN_POINT('Ctrl Pts',(-90.,-4.85722573273506E-16,4.));
#52505=CARTESIAN_POINT('',(-89.9777750336159,2.,6.));
#52506=CARTESIAN_POINT('Ctrl Pts',(-89.9777750336159,2.,6.));
#52507=CARTESIAN_POINT('Ctrl Pts',(-89.9777750336159,2.,6.25113333011964));
#52508=CARTESIAN_POINT('Ctrl Pts',(-89.9789345539658,1.94980925677131,6.51900023379203));
#52509=CARTESIAN_POINT('Ctrl Pts',(-89.9831259365723,1.74569936855887,7.01175644187864));
#52510=CARTESIAN_POINT('Ctrl Pts',(-89.9860976603374,1.59178067978086,7.23664644496533));
#52511=CARTESIAN_POINT('Ctrl Pts',(-89.9916787455059,1.23664644642618,7.59178067832001));
#52512=CARTESIAN_POINT('Ctrl Pts',(-89.9946501491172,1.01175644254643,7.74569936791146));
#52513=CARTESIAN_POINT('Ctrl Pts',(-89.9988407998655,0.519000232590762,
7.94980925763969));
#52514=CARTESIAN_POINT('Ctrl Pts',(-90.,0.251133328053567,8.));
#52515=CARTESIAN_POINT('Ctrl Pts',(-90.,2.77555756156289E-16,8.));
#52516=CARTESIAN_POINT('',(-82.,2.,6.));
#52517=CARTESIAN_POINT('',(-86.,2.,6.));
#52518=CARTESIAN_POINT('Origin',(-82.,0.,6.));
#52519=CARTESIAN_POINT('Ctrl Pts',(-90.,-4.16333634234434E-16,4.));
#52520=CARTESIAN_POINT('Ctrl Pts',(-90.,0.251133328053565,4.));
#52521=CARTESIAN_POINT('Ctrl Pts',(-89.9988407998655,0.519000232590761,
4.05019074236031));
#52522=CARTESIAN_POINT('Ctrl Pts',(-89.9946501491172,1.01175644254643,4.25430063208854));
#52523=CARTESIAN_POINT('Ctrl Pts',(-89.9916787455059,1.23664644642618,4.40821932167999));
#52524=CARTESIAN_POINT('Ctrl Pts',(-89.9860976603374,1.59178067978086,4.76335355503466));
#52525=CARTESIAN_POINT('Ctrl Pts',(-89.9831259365723,1.74569936855886,4.98824355812136));
#52526=CARTESIAN_POINT('Ctrl Pts',(-89.9789345539658,1.94980925677131,5.48099976620797));
#52527=CARTESIAN_POINT('Ctrl Pts',(-89.9777750336159,2.,5.74886666988035));
#52528=CARTESIAN_POINT('Ctrl Pts',(-89.9777750336159,2.,6.));
#52529=CARTESIAN_POINT('Origin',(-82.,0.,6.));
#52530=CARTESIAN_POINT('Origin',(86.,0.,6.));
#52531=CARTESIAN_POINT('',(90.,0.,8.));
#52532=CARTESIAN_POINT('',(90.,0.,4.));
#52533=CARTESIAN_POINT('Ctrl Pts',(90.,-2.77555756156289E-16,8.));
#52534=CARTESIAN_POINT('Ctrl Pts',(90.,0.251133328053566,8.));
#52535=CARTESIAN_POINT('Ctrl Pts',(89.9988407998655,0.519000232590761,7.94980925763969));
#52536=CARTESIAN_POINT('Ctrl Pts',(89.9946501491172,1.01175644254643,7.74569936791146));
#52537=CARTESIAN_POINT('Ctrl Pts',(89.9916787455059,1.23664644642618,7.59178067832001));
#52538=CARTESIAN_POINT('Ctrl Pts',(89.9860976603374,1.59178067978086,7.23664644496533));
#52539=CARTESIAN_POINT('Ctrl Pts',(89.9831259365723,1.74569936855887,7.01175644187864));
#52540=CARTESIAN_POINT('Ctrl Pts',(89.9789345539658,1.94980925677131,6.51900023379203));
#52541=CARTESIAN_POINT('Ctrl Pts',(89.9777750336159,2.,6.25113333011964));
#52542=CARTESIAN_POINT('Ctrl Pts',(89.9777750336159,2.,5.74886666988036));
#52543=CARTESIAN_POINT('Ctrl Pts',(89.9789345539658,1.94980925677131,5.48099976620797));
#52544=CARTESIAN_POINT('Ctrl Pts',(89.9831259365723,1.74569936855887,4.98824355812136));
#52545=CARTESIAN_POINT('Ctrl Pts',(89.9860976603374,1.59178067978086,4.76335355503467));
#52546=CARTESIAN_POINT('Ctrl Pts',(89.9916787455059,1.23664644642618,4.40821932167999));
#52547=CARTESIAN_POINT('Ctrl Pts',(89.9946501491172,1.01175644254643,4.25430063208854));
#52548=CARTESIAN_POINT('Ctrl Pts',(89.9988407998655,0.519000232590762,4.05019074236031));
#52549=CARTESIAN_POINT('Ctrl Pts',(90.,0.251133328053567,4.));
#52550=CARTESIAN_POINT('Ctrl Pts',(90.,4.85722573273506E-16,4.));
#52551=CARTESIAN_POINT('',(89.9777750336159,-2.,6.));
#52552=CARTESIAN_POINT('Ctrl Pts',(89.9777750336159,-2.,6.));
#52553=CARTESIAN_POINT('Ctrl Pts',(89.9777750336159,-2.,6.25113333011964));
#52554=CARTESIAN_POINT('Ctrl Pts',(89.9789345539658,-1.94980925677131,6.51900023379203));
#52555=CARTESIAN_POINT('Ctrl Pts',(89.9831259365723,-1.74569936855887,7.01175644187864));
#52556=CARTESIAN_POINT('Ctrl Pts',(89.9860976603374,-1.59178067978086,7.23664644496533));
#52557=CARTESIAN_POINT('Ctrl Pts',(89.9916787455059,-1.23664644642618,7.59178067832001));
#52558=CARTESIAN_POINT('Ctrl Pts',(89.9946501491172,-1.01175644254643,7.74569936791146));
#52559=CARTESIAN_POINT('Ctrl Pts',(89.9988407998655,-0.519000232590762,
7.94980925763969));
#52560=CARTESIAN_POINT('Ctrl Pts',(90.,-0.251133328053567,8.));
#52561=CARTESIAN_POINT('Ctrl Pts',(90.,-2.77555756156289E-16,8.));
#52562=CARTESIAN_POINT('',(82.,-2.,6.));
#52563=CARTESIAN_POINT('',(86.,-2.,6.));
#52564=CARTESIAN_POINT('Origin',(82.,0.,6.));
#52565=CARTESIAN_POINT('Ctrl Pts',(90.,4.16333634234434E-16,4.));
#52566=CARTESIAN_POINT('Ctrl Pts',(90.,-0.251133328053565,4.));
#52567=CARTESIAN_POINT('Ctrl Pts',(89.9988407998655,-0.519000232590761,
4.05019074236031));
#52568=CARTESIAN_POINT('Ctrl Pts',(89.9946501491172,-1.01175644254643,4.25430063208854));
#52569=CARTESIAN_POINT('Ctrl Pts',(89.9916787455059,-1.23664644642618,4.40821932167999));
#52570=CARTESIAN_POINT('Ctrl Pts',(89.9860976603374,-1.59178067978086,4.76335355503466));
#52571=CARTESIAN_POINT('Ctrl Pts',(89.9831259365723,-1.74569936855886,4.98824355812136));
#52572=CARTESIAN_POINT('Ctrl Pts',(89.9789345539658,-1.94980925677131,5.48099976620797));
#52573=CARTESIAN_POINT('Ctrl Pts',(89.9777750336159,-2.,5.74886666988035));
#52574=CARTESIAN_POINT('Ctrl Pts',(89.9777750336159,-2.,6.));
#52575=CARTESIAN_POINT('Origin',(82.,0.,6.));
#52576=CARTESIAN_POINT('Ctrl Pts',(74.4153560389001,-3.55032190142516,-5.55111512312578E-16));
#52577=CARTESIAN_POINT('Ctrl Pts',(74.4153560389001,-3.55032190142516,4.));
#52578=CARTESIAN_POINT('Ctrl Pts',(74.4153560389001,-3.55032190142516,8.));
#52579=CARTESIAN_POINT('Ctrl Pts',(74.4153560389001,-3.55032190142516,12.));
#52580=CARTESIAN_POINT('Ctrl Pts',(74.4101195539797,-3.66007952356781,-5.55111512312578E-16));
#52581=CARTESIAN_POINT('Ctrl Pts',(74.4101195539797,-3.66007952356781,4.));
#52582=CARTESIAN_POINT('Ctrl Pts',(74.4101195539797,-3.66007952356781,8.00000000000001));
#52583=CARTESIAN_POINT('Ctrl Pts',(74.4101195539797,-3.66007952356781,12.));
#52584=CARTESIAN_POINT('Ctrl Pts',(74.3352361483148,-3.84840282419241,-5.55111512312578E-16));
#52585=CARTESIAN_POINT('Ctrl Pts',(74.3352361483148,-3.84840282419241,4.));
#52586=CARTESIAN_POINT('Ctrl Pts',(74.3352361483148,-3.84840282419241,7.99999999999999));
#52587=CARTESIAN_POINT('Ctrl Pts',(74.3352361483148,-3.84840282419241,12.));
#52588=CARTESIAN_POINT('Ctrl Pts',(74.1732860426646,-3.96302207561158,-5.55111512312578E-16));
#52589=CARTESIAN_POINT('Ctrl Pts',(74.1732860426646,-3.96302207561158,4.));
#52590=CARTESIAN_POINT('Ctrl Pts',(74.1732860426646,-3.96302207561158,8.00000000000001));
#52591=CARTESIAN_POINT('Ctrl Pts',(74.1732860426646,-3.96302207561158,12.));
#52592=CARTESIAN_POINT('Ctrl Pts',(74.0964320765796,-3.99277406492185,-5.55111512312578E-16));
#52593=CARTESIAN_POINT('Ctrl Pts',(74.0964320765796,-3.99277406492185,4.));
#52594=CARTESIAN_POINT('Ctrl Pts',(74.0964320765796,-3.99277406492185,8.));
#52595=CARTESIAN_POINT('Ctrl Pts',(74.0964320765796,-3.99277406492185,12.));
#52596=CARTESIAN_POINT('',(74.4153560389001,-3.55032190142516,0.));
#52597=CARTESIAN_POINT('',(74.0964320765796,-3.99277406492185,0.));
#52598=CARTESIAN_POINT('Ctrl Pts',(74.4153560389001,-3.55032190142516,4.16333634234434E-16));
#52599=CARTESIAN_POINT('Ctrl Pts',(74.4101195539797,-3.66007952356781,4.16333634234433E-16));
#52600=CARTESIAN_POINT('Ctrl Pts',(74.3673290364569,-3.76769283821044,4.16333634234434E-16));
#52601=CARTESIAN_POINT('Ctrl Pts',(74.2961085760817,-3.85123952454109,4.16333634234434E-16));
#52602=CARTESIAN_POINT('Ctrl Pts',(74.2426932308004,-3.91389953928908,4.16333634234434E-16));
#52603=CARTESIAN_POINT('Ctrl Pts',(74.1732860426646,-3.96302207561158,4.16333634234433E-16));
#52604=CARTESIAN_POINT('Ctrl Pts',(74.0964320765796,-3.99277406492185,4.16333634234434E-16));
#52605=CARTESIAN_POINT('',(74.0964320765796,-3.99277406492185,12.));
#52606=CARTESIAN_POINT('Ctrl Pts',(74.0964320765796,-3.99277406492185,-5.55111512312578E-16));
#52607=CARTESIAN_POINT('Ctrl Pts',(74.0964320765796,-3.99277406492185,4.));
#52608=CARTESIAN_POINT('Ctrl Pts',(74.0964320765796,-3.99277406492185,8.));
#52609=CARTESIAN_POINT('Ctrl Pts',(74.0964320765796,-3.99277406492185,12.));
#52610=CARTESIAN_POINT('',(74.4153560389001,-3.55032190142516,12.));
#52611=CARTESIAN_POINT('Ctrl Pts',(74.0964320765796,-3.99277406492185,12.));
#52612=CARTESIAN_POINT('Ctrl Pts',(74.1732860426646,-3.96302207561158,12.));
#52613=CARTESIAN_POINT('Ctrl Pts',(74.2426932308004,-3.91389953928908,12.));
#52614=CARTESIAN_POINT('Ctrl Pts',(74.2961085760817,-3.85123952454109,12.));
#52615=CARTESIAN_POINT('Ctrl Pts',(74.3673290364569,-3.76769283821044,12.));
#52616=CARTESIAN_POINT('Ctrl Pts',(74.4101195539797,-3.66007952356781,12.));
#52617=CARTESIAN_POINT('Ctrl Pts',(74.4153560389001,-3.55032190142516,12.));
#52618=CARTESIAN_POINT('Ctrl Pts',(74.4153560389001,-3.55032190142516,12.));
#52619=CARTESIAN_POINT('Ctrl Pts',(74.4153560389001,-3.55032190142516,8.));
#52620=CARTESIAN_POINT('Ctrl Pts',(74.4153560389001,-3.55032190142516,4.));
#52621=CARTESIAN_POINT('Ctrl Pts',(74.4153560389001,-3.55032190142516,-5.55111512312578E-16));
#52622=CARTESIAN_POINT('Ctrl Pts',(69.8028570375097,-5.24987136994593,0.));
#52623=CARTESIAN_POINT('Ctrl Pts',(69.8028570375097,-5.24987136994593,12.));
#52624=CARTESIAN_POINT('Ctrl Pts',(69.8066748687772,-5.24915955997427,0.));
#52625=CARTESIAN_POINT('Ctrl Pts',(69.8066748687772,-5.24915955997427,12.));
#52626=CARTESIAN_POINT('Ctrl Pts',(69.8143154684204,-5.24773285666377,0.));
#52627=CARTESIAN_POINT('Ctrl Pts',(69.8143154684204,-5.24773285666377,12.));
#52628=CARTESIAN_POINT('Ctrl Pts',(69.8257911792159,-5.24558355159751,0.));
#52629=CARTESIAN_POINT('Ctrl Pts',(69.8257911792159,-5.24558355159751,12.));
#52630=CARTESIAN_POINT('Ctrl Pts',(69.841121750752,-5.2426993105457,0.));
#52631=CARTESIAN_POINT('Ctrl Pts',(69.841121750752,-5.2426993105457,12.));
#52632=CARTESIAN_POINT('Ctrl Pts',(69.8603343302743,-5.23906316634803,0.));
#52633=CARTESIAN_POINT('Ctrl Pts',(69.8603343302743,-5.23906316634803,12.));
#52634=CARTESIAN_POINT('Ctrl Pts',(69.8795962381599,-5.2353961627962,0.));
#52635=CARTESIAN_POINT('Ctrl Pts',(69.8795962381599,-5.2353961627962,12.));
#52636=CARTESIAN_POINT('Ctrl Pts',(69.8989073936688,-5.23169827290556,0.));
#52637=CARTESIAN_POINT('Ctrl Pts',(69.8989073936688,-5.23169827290556,12.));
#52638=CARTESIAN_POINT('Ctrl Pts',(69.9182676502048,-5.22796945602794,0.));
#52639=CARTESIAN_POINT('Ctrl Pts',(69.9182676502048,-5.22796945602794,12.));
#52640=CARTESIAN_POINT('Ctrl Pts',(69.9376767969095,-5.22420965879982,0.));
#52641=CARTESIAN_POINT('Ctrl Pts',(69.9376767969095,-5.22420965879982,12.));
#52642=CARTESIAN_POINT('Ctrl Pts',(69.9571345870076,-5.22041882075721,0.));
#52643=CARTESIAN_POINT('Ctrl Pts',(69.9571345870076,-5.22041882075721,12.));
#52644=CARTESIAN_POINT('Ctrl Pts',(69.9766407595385,-5.21659687881139,0.));
#52645=CARTESIAN_POINT('Ctrl Pts',(69.9766407595385,-5.21659687881139,12.));
#52646=CARTESIAN_POINT('Ctrl Pts',(69.9961950629965,-5.2127437720326,0.));
#52647=CARTESIAN_POINT('Ctrl Pts',(69.9961950629965,-5.2127437720326,12.));
#52648=CARTESIAN_POINT('Ctrl Pts',(70.0157972802182,-5.20885944672837,0.));
#52649=CARTESIAN_POINT('Ctrl Pts',(70.0157972802182,-5.20885944672837,12.));
#52650=CARTESIAN_POINT('Ctrl Pts',(70.0354472203546,-5.20494385478026,0.));
#52651=CARTESIAN_POINT('Ctrl Pts',(70.0354472203546,-5.20494385478026,12.));
#52652=CARTESIAN_POINT('Ctrl Pts',(70.0551447071082,-5.20099695122656,0.));
#52653=CARTESIAN_POINT('Ctrl Pts',(70.0551447071082,-5.20099695122656,12.));
#52654=CARTESIAN_POINT('Ctrl Pts',(70.0748895689729,-5.19701869225529,0.));
#52655=CARTESIAN_POINT('Ctrl Pts',(70.0748895689729,-5.19701869225529,12.));
#52656=CARTESIAN_POINT('Ctrl Pts',(70.0946816270997,-5.1930090327158,0.));
#52657=CARTESIAN_POINT('Ctrl Pts',(70.0946816270997,-5.1930090327158,12.));
#52658=CARTESIAN_POINT('Ctrl Pts',(70.1145206891885,-5.18896792486566,0.));
#52659=CARTESIAN_POINT('Ctrl Pts',(70.1145206891885,-5.18896792486566,12.));
#52660=CARTESIAN_POINT('Ctrl Pts',(70.1344065558145,-5.18489531966265,0.));
#52661=CARTESIAN_POINT('Ctrl Pts',(70.1344065558145,-5.18489531966265,12.));
#52662=CARTESIAN_POINT('Ctrl Pts',(70.1543390243892,-5.18079116757667,0.));
#52663=CARTESIAN_POINT('Ctrl Pts',(70.1543390243892,-5.18079116757667,12.));
#52664=CARTESIAN_POINT('Ctrl Pts',(70.1743178937077,-5.17665541952383,0.));
#52665=CARTESIAN_POINT('Ctrl Pts',(70.1743178937077,-5.17665541952383,12.));
#52666=CARTESIAN_POINT('Ctrl Pts',(70.1943429691167,-5.17248802793389,0.));
#52667=CARTESIAN_POINT('Ctrl Pts',(70.1943429691167,-5.17248802793389,12.));
#52668=CARTESIAN_POINT('Ctrl Pts',(70.2144140622953,-5.16828894670109,0.));
#52669=CARTESIAN_POINT('Ctrl Pts',(70.2144140622953,-5.16828894670109,12.));
#52670=CARTESIAN_POINT('Ctrl Pts',(70.2345309887833,-5.16405813066976,0.));
#52671=CARTESIAN_POINT('Ctrl Pts',(70.2345309887833,-5.16405813066976,12.));
#52672=CARTESIAN_POINT('Ctrl Pts',(70.2546935662722,-5.15979553528204,0.));
#52673=CARTESIAN_POINT('Ctrl Pts',(70.2546935662722,-5.15979553528204,12.));
#52674=CARTESIAN_POINT('Ctrl Pts',(70.2749016125105,-5.1555011161486,0.));
#52675=CARTESIAN_POINT('Ctrl Pts',(70.2749016125105,-5.1555011161486,12.));
#52676=CARTESIAN_POINT('Ctrl Pts',(70.2951549435512,-5.15117482869254,0.));
#52677=CARTESIAN_POINT('Ctrl Pts',(70.2951549435512,-5.15117482869254,12.));
#52678=CARTESIAN_POINT('Ctrl Pts',(70.3154533746736,-5.1468166283308,0.));
#52679=CARTESIAN_POINT('Ctrl Pts',(70.3154533746736,-5.1468166283308,12.));
#52680=CARTESIAN_POINT('Ctrl Pts',(70.3357967211796,-5.1424264706348,0.));
#52681=CARTESIAN_POINT('Ctrl Pts',(70.3357967211796,-5.1424264706348,12.));
#52682=CARTESIAN_POINT('Ctrl Pts',(70.3561847991714,-5.13800431148904,0.));
#52683=CARTESIAN_POINT('Ctrl Pts',(70.3561847991714,-5.13800431148904,12.));
#52684=CARTESIAN_POINT('Ctrl Pts',(70.3766174264757,-5.13355010728568,0.));
#52685=CARTESIAN_POINT('Ctrl Pts',(70.3766174264757,-5.13355010728568,12.));
#52686=CARTESIAN_POINT('Ctrl Pts',(70.3970944229851,-5.12906381499456,0.));
#52687=CARTESIAN_POINT('Ctrl Pts',(70.3970944229851,-5.12906381499456,12.));
#52688=CARTESIAN_POINT('Ctrl Pts',(70.417615610161,-5.12454539205329,0.));
#52689=CARTESIAN_POINT('Ctrl Pts',(70.417615610161,-5.12454539205329,12.));
#52690=CARTESIAN_POINT('Ctrl Pts',(70.4381808107245,-5.11999479630212,0.));
#52691=CARTESIAN_POINT('Ctrl Pts',(70.4381808107245,-5.11999479630212,12.));
#52692=CARTESIAN_POINT('Ctrl Pts',(70.458789848296,-5.11541198590933,0.));
#52693=CARTESIAN_POINT('Ctrl Pts',(70.458789848296,-5.11541198590933,12.));
#52694=CARTESIAN_POINT('Ctrl Pts',(70.4794425469825,-5.11079691929213,0.));
#52695=CARTESIAN_POINT('Ctrl Pts',(70.4794425469825,-5.11079691929213,12.));
#52696=CARTESIAN_POINT('Ctrl Pts',(70.500138731399,-5.10614955511664,0.));
#52697=CARTESIAN_POINT('Ctrl Pts',(70.500138731399,-5.10614955511664,12.));
#52698=CARTESIAN_POINT('Ctrl Pts',(70.5208782268497,-5.10146985232941,0.));
#52699=CARTESIAN_POINT('Ctrl Pts',(70.5208782268497,-5.10146985232941,12.));
#52700=CARTESIAN_POINT('Ctrl Pts',(70.5416608594526,-5.09675777018183,0.));
#52701=CARTESIAN_POINT('Ctrl Pts',(70.5416608594526,-5.09675777018183,12.));
#52702=CARTESIAN_POINT('Ctrl Pts',(70.5624864562824,-5.09201326826135,0.));
#52703=CARTESIAN_POINT('Ctrl Pts',(70.5624864562824,-5.09201326826135,12.));
#52704=CARTESIAN_POINT('Ctrl Pts',(70.5833548455014,-5.08723630652273,0.));
#52705=CARTESIAN_POINT('Ctrl Pts',(70.5833548455014,-5.08723630652273,12.));
#52706=CARTESIAN_POINT('Ctrl Pts',(70.6042658562923,-5.08242684526687,0.));
#52707=CARTESIAN_POINT('Ctrl Pts',(70.6042658562923,-5.08242684526687,12.));
#52708=CARTESIAN_POINT('Ctrl Pts',(70.6252193187878,-5.07758484512303,0.));
#52709=CARTESIAN_POINT('Ctrl Pts',(70.6252193187878,-5.07758484512303,12.));
#52710=CARTESIAN_POINT('Ctrl Pts',(70.6462150640015,-5.07271026703355,0.));
#52711=CARTESIAN_POINT('Ctrl Pts',(70.6462150640015,-5.07271026703355,12.));
#52712=CARTESIAN_POINT('Ctrl Pts',(70.6672529237455,-5.06780307224072,0.));
#52713=CARTESIAN_POINT('Ctrl Pts',(70.6672529237455,-5.06780307224072,12.));
#52714=CARTESIAN_POINT('Ctrl Pts',(70.6883327305784,-5.0628632222782,0.));
#52715=CARTESIAN_POINT('Ctrl Pts',(70.6883327305784,-5.0628632222782,12.));
#52716=CARTESIAN_POINT('Ctrl Pts',(70.7094543178438,-5.05789067897058,0.));
#52717=CARTESIAN_POINT('Ctrl Pts',(70.7094543178438,-5.05789067897058,12.));
#52718=CARTESIAN_POINT('Ctrl Pts',(70.7306175196863,-5.05288540443483,0.));
#52719=CARTESIAN_POINT('Ctrl Pts',(70.7306175196863,-5.05288540443483,12.));
#52720=CARTESIAN_POINT('Ctrl Pts',(70.7518221710706,-5.04784736108346,0.));
#52721=CARTESIAN_POINT('Ctrl Pts',(70.7518221710706,-5.04784736108346,12.));
#52722=CARTESIAN_POINT('Ctrl Pts',(70.7730681077983,-5.0427765116335,0.));
#52723=CARTESIAN_POINT('Ctrl Pts',(70.7730681077983,-5.0427765116335,12.));
#52724=CARTESIAN_POINT('Ctrl Pts',(70.7943551665059,-5.03767281910479,0.));
#52725=CARTESIAN_POINT('Ctrl Pts',(70.7943551665059,-5.03767281910479,12.));
#52726=CARTESIAN_POINT('Ctrl Pts',(70.8156831846488,-5.03253624680941,0.));
#52727=CARTESIAN_POINT('Ctrl Pts',(70.8156831846488,-5.03253624680941,12.));
#52728=CARTESIAN_POINT('Ctrl Pts',(70.8370520004843,-5.02736675834693,0.));
#52729=CARTESIAN_POINT('Ctrl Pts',(70.8370520004843,-5.02736675834693,12.));
#52730=CARTESIAN_POINT('Ctrl Pts',(70.8584614530519,-5.02216431760061,0.));
#52731=CARTESIAN_POINT('Ctrl Pts',(70.8584614530519,-5.02216431760061,12.));
#52732=CARTESIAN_POINT('Ctrl Pts',(70.8799113821452,-5.0169288887379,0.));
#52733=CARTESIAN_POINT('Ctrl Pts',(70.8799113821452,-5.0169288887379,12.));
#52734=CARTESIAN_POINT('Ctrl Pts',(70.9014016283124,-5.01166043620568,0.));
#52735=CARTESIAN_POINT('Ctrl Pts',(70.9014016283124,-5.01166043620568,12.));
#52736=CARTESIAN_POINT('Ctrl Pts',(70.9229320328589,-5.00635892472514,0.));
#52737=CARTESIAN_POINT('Ctrl Pts',(70.9229320328589,-5.00635892472514,12.));
#52738=CARTESIAN_POINT('Ctrl Pts',(70.9445024378439,-5.0010243192904,0.));
#52739=CARTESIAN_POINT('Ctrl Pts',(70.9445024378439,-5.0010243192904,12.));
#52740=CARTESIAN_POINT('Ctrl Pts',(70.9661126860773,-4.99565658516913,0.));
#52741=CARTESIAN_POINT('Ctrl Pts',(70.9661126860773,-4.99565658516913,12.));
#52742=CARTESIAN_POINT('Ctrl Pts',(70.9877626211113,-4.99025568790665,0.));
#52743=CARTESIAN_POINT('Ctrl Pts',(70.9877626211113,-4.99025568790665,12.));
#52744=CARTESIAN_POINT('Ctrl Pts',(71.0094520872377,-4.98482159331864,0.));
#52745=CARTESIAN_POINT('Ctrl Pts',(71.0094520872377,-4.98482159331864,12.));
#52746=CARTESIAN_POINT('Ctrl Pts',(71.0311809294821,-4.97935426748585,0.));
#52747=CARTESIAN_POINT('Ctrl Pts',(71.0311809294821,-4.97935426748585,12.));
#52748=CARTESIAN_POINT('Ctrl Pts',(71.0529489935961,-4.97385367675159,0.));
#52749=CARTESIAN_POINT('Ctrl Pts',(71.0529489935961,-4.97385367675159,12.));
#52750=CARTESIAN_POINT('Ctrl Pts',(71.0747561260436,-4.96831978772191,0.));
#52751=CARTESIAN_POINT('Ctrl Pts',(71.0747561260436,-4.96831978772191,12.));
#52752=CARTESIAN_POINT('Ctrl Pts',(71.0966021739907,-4.96275256726766,0.));
#52753=CARTESIAN_POINT('Ctrl Pts',(71.0966021739907,-4.96275256726766,12.));
#52754=CARTESIAN_POINT('Ctrl Pts',(71.1184869853056,-4.95715198251685,0.));
#52755=CARTESIAN_POINT('Ctrl Pts',(71.1184869853056,-4.95715198251685,12.));
#52756=CARTESIAN_POINT('Ctrl Pts',(71.1404104085552,-4.95151800085102,0.));
#52757=CARTESIAN_POINT('Ctrl Pts',(71.1404104085552,-4.95151800085102,12.));
#52758=CARTESIAN_POINT('Ctrl Pts',(71.1623722930001,-4.94585058990341,0.));
#52759=CARTESIAN_POINT('Ctrl Pts',(71.1623722930001,-4.94585058990341,12.));
#52760=CARTESIAN_POINT('Ctrl Pts',(71.1843724885847,-4.94014971756115,0.));
#52761=CARTESIAN_POINT('Ctrl Pts',(71.1843724885847,-4.94014971756115,12.));
#52762=CARTESIAN_POINT('Ctrl Pts',(71.2064108459286,-4.93441535196618,0.));
#52763=CARTESIAN_POINT('Ctrl Pts',(71.2064108459286,-4.93441535196618,12.));
#52764=CARTESIAN_POINT('Ctrl Pts',(71.2284872163273,-4.92864746150733,0.));
#52765=CARTESIAN_POINT('Ctrl Pts',(71.2284872163273,-4.92864746150733,12.));
#52766=CARTESIAN_POINT('Ctrl Pts',(71.250601451747,-4.92284601481722,0.));
#52767=CARTESIAN_POINT('Ctrl Pts',(71.250601451747,-4.92284601481722,12.));
#52768=CARTESIAN_POINT('Ctrl Pts',(71.2727534048192,-4.91701098077036,0.));
#52769=CARTESIAN_POINT('Ctrl Pts',(71.2727534048192,-4.91701098077036,12.));
#52770=CARTESIAN_POINT('Ctrl Pts',(71.294942928829,-4.91114232848603,0.));
#52771=CARTESIAN_POINT('Ctrl Pts',(71.294942928829,-4.91114232848603,12.));
#52772=CARTESIAN_POINT('Ctrl Pts',(71.3171698777084,-4.90524002732779,0.));
#52773=CARTESIAN_POINT('Ctrl Pts',(71.3171698777084,-4.90524002732779,12.));
#52774=CARTESIAN_POINT('Ctrl Pts',(71.3394341060359,-4.89930404689575,0.));
#52775=CARTESIAN_POINT('Ctrl Pts',(71.3394341060359,-4.89930404689575,12.));
#52776=CARTESIAN_POINT('Ctrl Pts',(71.3617354690325,-4.89333435702414,0.));
#52777=CARTESIAN_POINT('Ctrl Pts',(71.3617354690325,-4.89333435702414,12.));
#52778=CARTESIAN_POINT('Ctrl Pts',(71.3840738225562,-4.88733092777975,0.));
#52779=CARTESIAN_POINT('Ctrl Pts',(71.3840738225562,-4.88733092777975,12.));
#52780=CARTESIAN_POINT('Ctrl Pts',(71.4064490230899,-4.88129372946552,0.));
#52781=CARTESIAN_POINT('Ctrl Pts',(71.4064490230899,-4.88129372946552,12.));
#52782=CARTESIAN_POINT('Ctrl Pts',(71.4288609277374,-4.87522273261908,0.));
#52783=CARTESIAN_POINT('Ctrl Pts',(71.4288609277374,-4.87522273261908,12.));
#52784=CARTESIAN_POINT('Ctrl Pts',(71.4513093942255,-4.8691179080055,0.));
#52785=CARTESIAN_POINT('Ctrl Pts',(71.4513093942255,-4.8691179080055,12.));
#52786=CARTESIAN_POINT('Ctrl Pts',(71.4737942808982,-4.86297922661503,0.));
#52787=CARTESIAN_POINT('Ctrl Pts',(71.4737942808982,-4.86297922661503,12.));
#52788=CARTESIAN_POINT('Ctrl Pts',(71.4963154467113,-4.85680665966181,0.));
#52789=CARTESIAN_POINT('Ctrl Pts',(71.4963154467113,-4.85680665966181,12.));
#52790=CARTESIAN_POINT('Ctrl Pts',(71.5188727512197,-4.8506001785878,0.));
#52791=CARTESIAN_POINT('Ctrl Pts',(71.5188727512197,-4.8506001785878,12.));
#52792=CARTESIAN_POINT('Ctrl Pts',(71.5414660545739,-4.84435975506049,0.));
#52793=CARTESIAN_POINT('Ctrl Pts',(71.5414660545739,-4.84435975506049,12.));
#52794=CARTESIAN_POINT('Ctrl Pts',(71.564095217521,-4.83808536096584,0.));
#52795=CARTESIAN_POINT('Ctrl Pts',(71.564095217521,-4.83808536096584,12.));
#52796=CARTESIAN_POINT('Ctrl Pts',(71.5867601014,-4.83177696840638,0.));
#52797=CARTESIAN_POINT('Ctrl Pts',(71.5867601014,-4.83177696840638,12.));
#52798=CARTESIAN_POINT('Ctrl Pts',(71.6094605681366,-4.82543454970027,0.));
#52799=CARTESIAN_POINT('Ctrl Pts',(71.6094605681366,-4.82543454970027,12.));
#52800=CARTESIAN_POINT('Ctrl Pts',(71.6321964802326,-4.81905807738557,0.));
#52801=CARTESIAN_POINT('Ctrl Pts',(71.6321964802326,-4.81905807738557,12.));
#52802=CARTESIAN_POINT('Ctrl Pts',(71.6549677007613,-4.81264752421732,0.));
#52803=CARTESIAN_POINT('Ctrl Pts',(71.6549677007613,-4.81264752421732,12.));
#52804=CARTESIAN_POINT('Ctrl Pts',(71.6777740933705,-4.80620286316089,0.));
#52805=CARTESIAN_POINT('Ctrl Pts',(71.6777740933705,-4.80620286316089,12.));
#52806=CARTESIAN_POINT('Ctrl Pts',(71.7006155222766,-4.79972406739014,0.));
#52807=CARTESIAN_POINT('Ctrl Pts',(71.7006155222766,-4.79972406739014,12.));
#52808=CARTESIAN_POINT('Ctrl Pts',(71.7234918522604,-4.79321111028672,0.));
#52809=CARTESIAN_POINT('Ctrl Pts',(71.7234918522604,-4.79321111028672,12.));
#52810=CARTESIAN_POINT('Ctrl Pts',(71.7464029486552,-4.78666396544451,0.));
#52811=CARTESIAN_POINT('Ctrl Pts',(71.7464029486552,-4.78666396544451,12.));
#52812=CARTESIAN_POINT('Ctrl Pts',(71.7693486773449,-4.78008260666643,0.));
#52813=CARTESIAN_POINT('Ctrl Pts',(71.7693486773449,-4.78008260666643,12.));
#52814=CARTESIAN_POINT('Ctrl Pts',(71.7923289047636,-4.77346700795788,0.));
#52815=CARTESIAN_POINT('Ctrl Pts',(71.7923289047636,-4.77346700795788,12.));
#52816=CARTESIAN_POINT('Ctrl Pts',(71.8153434978924,-4.76681714352504,0.));
#52817=CARTESIAN_POINT('Ctrl Pts',(71.8153434978924,-4.76681714352504,12.));
#52818=CARTESIAN_POINT('Ctrl Pts',(71.8383923242533,-4.76013298777423,0.));
#52819=CARTESIAN_POINT('Ctrl Pts',(71.8383923242533,-4.76013298777423,12.));
#52820=CARTESIAN_POINT('Ctrl Pts',(71.8614752519008,-4.75341451531671,0.));
#52821=CARTESIAN_POINT('Ctrl Pts',(71.8614752519008,-4.75341451531671,12.));
#52822=CARTESIAN_POINT('Ctrl Pts',(71.8845921494186,-4.74666170096546,0.));
#52823=CARTESIAN_POINT('Ctrl Pts',(71.8845921494186,-4.74666170096546,12.));
#52824=CARTESIAN_POINT('Ctrl Pts',(71.9077428859207,-4.73987451972861,0.));
#52825=CARTESIAN_POINT('Ctrl Pts',(71.9077428859207,-4.73987451972861,12.));
#52826=CARTESIAN_POINT('Ctrl Pts',(71.9309273310469,-4.73305294680784,0.));
#52827=CARTESIAN_POINT('Ctrl Pts',(71.9309273310469,-4.73305294680784,12.));
#52828=CARTESIAN_POINT('Ctrl Pts',(71.9541453549582,-4.72619695759779,0.));
#52829=CARTESIAN_POINT('Ctrl Pts',(71.9541453549582,-4.72619695759779,12.));
#52830=CARTESIAN_POINT('Ctrl Pts',(71.9773968283267,-4.71930652769081,0.));
#52831=CARTESIAN_POINT('Ctrl Pts',(71.9773968283267,-4.71930652769081,12.));
#52832=CARTESIAN_POINT('Ctrl Pts',(72.0006816223335,-4.71238163287411,0.));
#52833=CARTESIAN_POINT('Ctrl Pts',(72.0006816223335,-4.71238163287411,12.));
#52834=CARTESIAN_POINT('Ctrl Pts',(72.0239996086694,-4.70542224912312,0.));
#52835=CARTESIAN_POINT('Ctrl Pts',(72.0239996086694,-4.70542224912312,12.));
#52836=CARTESIAN_POINT('Ctrl Pts',(72.047350659532,-4.69842835259997,0.));
#52837=CARTESIAN_POINT('Ctrl Pts',(72.047350659532,-4.69842835259997,12.));
#52838=CARTESIAN_POINT('Ctrl Pts',(72.070734647621,-4.6913999196528,0.));
#52839=CARTESIAN_POINT('Ctrl Pts',(72.070734647621,-4.6913999196528,12.));
#52840=CARTESIAN_POINT('Ctrl Pts',(72.0941514461283,-4.68433692682061,0.));
#52841=CARTESIAN_POINT('Ctrl Pts',(72.0941514461283,-4.68433692682061,12.));
#52842=CARTESIAN_POINT('Ctrl Pts',(72.1176009287349,-4.67723935083087,0.));
#52843=CARTESIAN_POINT('Ctrl Pts',(72.1176009287349,-4.67723935083087,12.));
#52844=CARTESIAN_POINT('Ctrl Pts',(72.1410829696129,-4.67010716859281,0.));
#52845=CARTESIAN_POINT('Ctrl Pts',(72.1410829696129,-4.67010716859281,12.));
#52846=CARTESIAN_POINT('Ctrl Pts',(72.1645974434218,-4.6629403571957,0.));
#52847=CARTESIAN_POINT('Ctrl Pts',(72.1645974434218,-4.6629403571957,12.));
#52848=CARTESIAN_POINT('Ctrl Pts',(72.1881442253052,-4.65573889390825,0.));
#52849=CARTESIAN_POINT('Ctrl Pts',(72.1881442253052,-4.65573889390825,12.));
#52850=CARTESIAN_POINT('Ctrl Pts',(72.2117231908816,-4.64850275618325,0.));
#52851=CARTESIAN_POINT('Ctrl Pts',(72.2117231908816,-4.64850275618325,12.));
#52852=CARTESIAN_POINT('Ctrl Pts',(72.2353342162408,-4.64123192165628,0.));
#52853=CARTESIAN_POINT('Ctrl Pts',(72.2353342162408,-4.64123192165628,12.));
#52854=CARTESIAN_POINT('Ctrl Pts',(72.2589771779447,-4.63392636813842,0.));
#52855=CARTESIAN_POINT('Ctrl Pts',(72.2589771779447,-4.63392636813842,12.));
#52856=CARTESIAN_POINT('Ctrl Pts',(72.2826519530254,-4.62658607361465,0.));
#52857=CARTESIAN_POINT('Ctrl Pts',(72.2826519530254,-4.62658607361465,12.));
#52858=CARTESIAN_POINT('Ctrl Pts',(72.306358418981,-4.61921101624295,0.));
#52859=CARTESIAN_POINT('Ctrl Pts',(72.306358418981,-4.61921101624295,12.));
#52860=CARTESIAN_POINT('Ctrl Pts',(72.330096453767,-4.61180117435869,0.));
#52861=CARTESIAN_POINT('Ctrl Pts',(72.330096453767,-4.61180117435869,12.));
#52862=CARTESIAN_POINT('Ctrl Pts',(72.3538659357932,-4.60435652647463,0.));
#52863=CARTESIAN_POINT('Ctrl Pts',(72.3538659357932,-4.60435652647463,12.));
#52864=CARTESIAN_POINT('Ctrl Pts',(72.3776667439244,-4.5968770512734,0.));
#52865=CARTESIAN_POINT('Ctrl Pts',(72.3776667439244,-4.5968770512734,12.));
#52866=CARTESIAN_POINT('Ctrl Pts',(72.4014987574789,-4.58936272760551,0.));
#52867=CARTESIAN_POINT('Ctrl Pts',(72.4014987574789,-4.58936272760551,12.));
#52868=CARTESIAN_POINT('Ctrl Pts',(72.4253618562249,-4.58181353448851,0.));
#52869=CARTESIAN_POINT('Ctrl Pts',(72.4253618562249,-4.58181353448851,12.));
#52870=CARTESIAN_POINT('Ctrl Pts',(72.449255920373,-4.57422945111094,0.));
#52871=CARTESIAN_POINT('Ctrl Pts',(72.449255920373,-4.57422945111094,12.));
#52872=CARTESIAN_POINT('Ctrl Pts',(72.473180830571,-4.56661045683367,0.));
#52873=CARTESIAN_POINT('Ctrl Pts',(72.473180830571,-4.56661045683367,12.));
#52874=CARTESIAN_POINT('Ctrl Pts',(72.4971364679055,-4.55895653118214,0.));
#52875=CARTESIAN_POINT('Ctrl Pts',(72.4971364679055,-4.55895653118214,12.));
#52876=CARTESIAN_POINT('Ctrl Pts',(72.5211227138997,-4.55126765384403,0.));
#52877=CARTESIAN_POINT('Ctrl Pts',(72.5211227138997,-4.55126765384403,12.));
#52878=CARTESIAN_POINT('Ctrl Pts',(72.5451394505106,-4.54354380466825,0.));
#52879=CARTESIAN_POINT('Ctrl Pts',(72.5451394505106,-4.54354380466825,12.));
#52880=CARTESIAN_POINT('Ctrl Pts',(72.5691865601225,-4.53578496366802,0.));
#52881=CARTESIAN_POINT('Ctrl Pts',(72.5691865601225,-4.53578496366802,12.));
#52882=CARTESIAN_POINT('Ctrl Pts',(72.5932639255406,-4.5279911110239,0.));
#52883=CARTESIAN_POINT('Ctrl Pts',(72.5932639255406,-4.5279911110239,12.));
#52884=CARTESIAN_POINT('Ctrl Pts',(72.6173714299935,-4.52016222707632,0.));
#52885=CARTESIAN_POINT('Ctrl Pts',(72.6173714299935,-4.52016222707632,12.));
#52886=CARTESIAN_POINT('Ctrl Pts',(72.6415089571314,-4.5122982923226,0.));
#52887=CARTESIAN_POINT('Ctrl Pts',(72.6415089571314,-4.5122982923226,12.));
#52888=CARTESIAN_POINT('Ctrl Pts',(72.6656763910241,-4.50439928741605,0.));
#52889=CARTESIAN_POINT('Ctrl Pts',(72.6656763910241,-4.50439928741605,12.));
#52890=CARTESIAN_POINT('Ctrl Pts',(72.689873616155,-4.49646519316822,0.));
#52891=CARTESIAN_POINT('Ctrl Pts',(72.689873616155,-4.49646519316822,12.));
#52892=CARTESIAN_POINT('Ctrl Pts',(72.7141005174153,-4.48849599055354,0.));
#52893=CARTESIAN_POINT('Ctrl Pts',(72.7141005174153,-4.48849599055354,12.));
#52894=CARTESIAN_POINT('Ctrl Pts',(72.7383569801042,-4.48049166070223,0.));
#52895=CARTESIAN_POINT('Ctrl Pts',(72.7383569801042,-4.48049166070223,12.));
#52896=CARTESIAN_POINT('Ctrl Pts',(72.7626428899287,-4.47245218489623,0.));
#52897=CARTESIAN_POINT('Ctrl Pts',(72.7626428899287,-4.47245218489623,12.));
#52898=CARTESIAN_POINT('Ctrl Pts',(72.7869581329994,-4.46437754456796,0.));
#52899=CARTESIAN_POINT('Ctrl Pts',(72.7869581329994,-4.46437754456796,12.));
#52900=CARTESIAN_POINT('Ctrl Pts',(72.8113025958258,-4.45626772130138,0.));
#52901=CARTESIAN_POINT('Ctrl Pts',(72.8113025958258,-4.45626772130138,12.));
#52902=CARTESIAN_POINT('Ctrl Pts',(72.8356761653064,-4.44812269683724,0.));
#52903=CARTESIAN_POINT('Ctrl Pts',(72.8356761653064,-4.44812269683724,12.));
#52904=CARTESIAN_POINT('Ctrl Pts',(72.8600787287316,-4.43994245306805,0.));
#52905=CARTESIAN_POINT('Ctrl Pts',(72.8600787287316,-4.43994245306805,12.));
#52906=CARTESIAN_POINT('Ctrl Pts',(72.8845101737856,-4.43172697203342,0.));
#52907=CARTESIAN_POINT('Ctrl Pts',(72.8845101737856,-4.43172697203342,12.));
#52908=CARTESIAN_POINT('Ctrl Pts',(72.9089703885463,-4.42347623591942,0.));
#52909=CARTESIAN_POINT('Ctrl Pts',(72.9089703885463,-4.42347623591942,12.));
#52910=CARTESIAN_POINT('Ctrl Pts',(72.9334592614828,-4.41519022705927,0.));
#52911=CARTESIAN_POINT('Ctrl Pts',(72.9334592614828,-4.41519022705927,12.));
#52912=CARTESIAN_POINT('Ctrl Pts',(72.9579766814495,-4.40686892793965,0.));
#52913=CARTESIAN_POINT('Ctrl Pts',(72.9579766814495,-4.40686892793965,12.));
#52914=CARTESIAN_POINT('Ctrl Pts',(72.9825225376839,-4.39851232119731,0.));
#52915=CARTESIAN_POINT('Ctrl Pts',(72.9825225376839,-4.39851232119731,12.));
#52916=CARTESIAN_POINT('Ctrl Pts',(73.0070967198033,-4.39012038961145,0.));
#52917=CARTESIAN_POINT('Ctrl Pts',(73.0070967198033,-4.39012038961145,12.));
#52918=CARTESIAN_POINT('Ctrl Pts',(73.031699117799,-4.38169311610153,0.));
#52919=CARTESIAN_POINT('Ctrl Pts',(73.031699117799,-4.38169311610153,12.));
#52920=CARTESIAN_POINT('Ctrl Pts',(73.0563296220301,-4.37323048372607,0.));
#52921=CARTESIAN_POINT('Ctrl Pts',(73.0563296220301,-4.37323048372607,12.));
#52922=CARTESIAN_POINT('Ctrl Pts',(73.0809881232111,-4.36473247568638,0.));
#52923=CARTESIAN_POINT('Ctrl Pts',(73.0809881232111,-4.36473247568638,12.));
#52924=CARTESIAN_POINT('Ctrl Pts',(73.1056745124099,-4.35619907532716,0.));
#52925=CARTESIAN_POINT('Ctrl Pts',(73.1056745124099,-4.35619907532716,12.));
#52926=CARTESIAN_POINT('Ctrl Pts',(73.1303886810602,-4.34763026613155,0.));
#52927=CARTESIAN_POINT('Ctrl Pts',(73.1303886810602,-4.34763026613155,12.));
#52928=CARTESIAN_POINT('Ctrl Pts',(73.1551305209692,-4.3390260317214,0.));
#52929=CARTESIAN_POINT('Ctrl Pts',(73.1551305209692,-4.3390260317214,12.));
#52930=CARTESIAN_POINT('Ctrl Pts',(73.1798999243234,-4.33038635585878,0.));
#52931=CARTESIAN_POINT('Ctrl Pts',(73.1798999243234,-4.33038635585878,12.));
#52932=CARTESIAN_POINT('Ctrl Pts',(73.204696783693,-4.32171122245219,0.));
#52933=CARTESIAN_POINT('Ctrl Pts',(73.204696783693,-4.32171122245219,12.));
#52934=CARTESIAN_POINT('Ctrl Pts',(73.2295209920319,-4.31300061556103,0.));
#52935=CARTESIAN_POINT('Ctrl Pts',(73.2295209920319,-4.31300061556103,12.));
#52936=CARTESIAN_POINT('Ctrl Pts',(73.2543724426562,-4.30425451938234,0.));
#52937=CARTESIAN_POINT('Ctrl Pts',(73.2543724426562,-4.30425451938234,12.));
#52938=CARTESIAN_POINT('Ctrl Pts',(73.2792510292243,-4.29547291824289,0.));
#52939=CARTESIAN_POINT('Ctrl Pts',(73.2792510292243,-4.29547291824289,12.));
#52940=CARTESIAN_POINT('Ctrl Pts',(73.3041566457134,-4.28665579659302,0.));
#52941=CARTESIAN_POINT('Ctrl Pts',(73.3041566457134,-4.28665579659302,12.));
#52942=CARTESIAN_POINT('Ctrl Pts',(73.3290891863959,-4.27780313900392,0.));
#52943=CARTESIAN_POINT('Ctrl Pts',(73.3290891863959,-4.27780313900392,12.));
#52944=CARTESIAN_POINT('Ctrl Pts',(73.354048545808,-4.26891493016703,0.));
#52945=CARTESIAN_POINT('Ctrl Pts',(73.354048545808,-4.26891493016703,12.));
#52946=CARTESIAN_POINT('Ctrl Pts',(73.3790346187953,-4.25999115489905,0.));
#52947=CARTESIAN_POINT('Ctrl Pts',(73.3790346187953,-4.25999115489905,12.));
#52948=CARTESIAN_POINT('Ctrl Pts',(73.4040473005603,-4.25103179814892,0.));
#52949=CARTESIAN_POINT('Ctrl Pts',(73.4040473005603,-4.25103179814892,12.));
#52950=CARTESIAN_POINT('Ctrl Pts',(73.4290864867103,-4.24203684500941,0.));
#52951=CARTESIAN_POINT('Ctrl Pts',(73.4290864867103,-4.24203684500941,12.));
#52952=CARTESIAN_POINT('Ctrl Pts',(73.4541520732943,-4.23300628072758,0.));
#52953=CARTESIAN_POINT('Ctrl Pts',(73.4541520732943,-4.23300628072758,12.));
#52954=CARTESIAN_POINT('Ctrl Pts',(73.4792439568624,-4.22394009072753,0.));
#52955=CARTESIAN_POINT('Ctrl Pts',(73.4792439568624,-4.22394009072753,12.));
#52956=CARTESIAN_POINT('Ctrl Pts',(73.5043620344107,-4.21483826059437,0.));
#52957=CARTESIAN_POINT('Ctrl Pts',(73.5043620344107,-4.21483826059437,12.));
#52958=CARTESIAN_POINT('Ctrl Pts',(73.5295062032621,-4.20570077603727,0.));
#52959=CARTESIAN_POINT('Ctrl Pts',(73.5295062032621,-4.20570077603727,12.));
#52960=CARTESIAN_POINT('Ctrl Pts',(73.554676360957,-4.19652762286127,0.));
#52961=CARTESIAN_POINT('Ctrl Pts',(73.554676360957,-4.19652762286127,12.));
#52962=CARTESIAN_POINT('Ctrl Pts',(73.5798724051519,-4.18731878694238,0.));
#52963=CARTESIAN_POINT('Ctrl Pts',(73.5798724051519,-4.18731878694238,12.));
#52964=CARTESIAN_POINT('Ctrl Pts',(73.6050942334773,-4.17807425419817,0.));
#52965=CARTESIAN_POINT('Ctrl Pts',(73.6050942334773,-4.17807425419817,12.));
#52966=CARTESIAN_POINT('Ctrl Pts',(73.6303417435262,-4.16879401058787,0.));
#52967=CARTESIAN_POINT('Ctrl Pts',(73.6303417435262,-4.16879401058787,12.));
#52968=CARTESIAN_POINT('Ctrl Pts',(73.6556148331504,-4.15947804217791,0.));
#52969=CARTESIAN_POINT('Ctrl Pts',(73.6556148331504,-4.15947804217791,12.));
#52970=CARTESIAN_POINT('Ctrl Pts',(73.6809134006909,-4.15012633519728,0.));
#52971=CARTESIAN_POINT('Ctrl Pts',(73.6809134006909,-4.15012633519728,12.));
#52972=CARTESIAN_POINT('Ctrl Pts',(73.7062373452344,-4.14073887610155,0.));
#52973=CARTESIAN_POINT('Ctrl Pts',(73.7062373452344,-4.14073887610155,12.));
#52974=CARTESIAN_POINT('Ctrl Pts',(73.7315865668508,-4.13131565163575,0.));
#52975=CARTESIAN_POINT('Ctrl Pts',(73.7315865668508,-4.13131565163575,12.));
#52976=CARTESIAN_POINT('Ctrl Pts',(73.7569609668501,-4.12185664890551,0.));
#52977=CARTESIAN_POINT('Ctrl Pts',(73.7569609668501,-4.12185664890551,12.));
#52978=CARTESIAN_POINT('Ctrl Pts',(73.7823604472126,-4.1123618552278,0.));
#52979=CARTESIAN_POINT('Ctrl Pts',(73.7823604472126,-4.1123618552278,12.));
#52980=CARTESIAN_POINT('Ctrl Pts',(73.8077849100314,-4.10283125798724,0.));
#52981=CARTESIAN_POINT('Ctrl Pts',(73.8077849100314,-4.10283125798724,12.));
#52982=CARTESIAN_POINT('Ctrl Pts',(73.8332342568978,-4.09326484448232,0.));
#52983=CARTESIAN_POINT('Ctrl Pts',(73.8332342568978,-4.09326484448232,12.));
#52984=CARTESIAN_POINT('Ctrl Pts',(73.8587083884208,-4.0836626018068,0.));
#52985=CARTESIAN_POINT('Ctrl Pts',(73.8587083884208,-4.0836626018068,12.));
#52986=CARTESIAN_POINT('Ctrl Pts',(73.884207203405,-4.07402451665253,0.));
#52987=CARTESIAN_POINT('Ctrl Pts',(73.884207203405,-4.07402451665253,12.));
#52988=CARTESIAN_POINT('Ctrl Pts',(73.9097305995173,-4.06435057547335,0.));
#52989=CARTESIAN_POINT('Ctrl Pts',(73.9097305995173,-4.06435057547335,12.));
#52990=CARTESIAN_POINT('Ctrl Pts',(73.9352784747665,-4.05464076484762,0.));
#52991=CARTESIAN_POINT('Ctrl Pts',(73.9352784747665,-4.05464076484762,12.));
#52992=CARTESIAN_POINT('Ctrl Pts',(73.9608507287943,-4.04489507179964,0.));
#52993=CARTESIAN_POINT('Ctrl Pts',(73.9608507287943,-4.04489507179964,12.));
#52994=CARTESIAN_POINT('Ctrl Pts',(73.9864472641025,-4.0351134841066,0.));
#52995=CARTESIAN_POINT('Ctrl Pts',(73.9864472641025,-4.0351134841066,12.));
#52996=CARTESIAN_POINT('Ctrl Pts',(74.0120679876396,-4.02529599070085,0.));
#52997=CARTESIAN_POINT('Ctrl Pts',(74.0120679876396,-4.02529599070085,12.));
#52998=CARTESIAN_POINT('Ctrl Pts',(74.0377128111754,-4.01544258176693,0.));
#52999=CARTESIAN_POINT('Ctrl Pts',(74.0377128111754,-4.01544258176693,12.));
#53000=CARTESIAN_POINT('Ctrl Pts',(74.0633816477912,-4.0055532478546,0.));
#53001=CARTESIAN_POINT('Ctrl Pts',(74.0633816477912,-4.0055532478546,12.));
#53002=CARTESIAN_POINT('Ctrl Pts',(74.0890744091088,-3.99562797918271,0.));
#53003=CARTESIAN_POINT('Ctrl Pts',(74.0890744091088,-3.99562797918271,12.));
#53004=CARTESIAN_POINT('Ctrl Pts',(74.1147910020869,-3.98566676483639,0.));
#53005=CARTESIAN_POINT('Ctrl Pts',(74.1147910020869,-3.98566676483639,12.));
#53006=CARTESIAN_POINT('Ctrl Pts',(74.1405313263198,-3.97566959209546,0.));
#53007=CARTESIAN_POINT('Ctrl Pts',(74.1405313263198,-3.97566959209546,12.));
#53008=CARTESIAN_POINT('Ctrl Pts',(74.1662952702689,-3.96563644549423,0.));
#53009=CARTESIAN_POINT('Ctrl Pts',(74.1662952702689,-3.96563644549423,12.));
#53010=CARTESIAN_POINT('Ctrl Pts',(74.1920827166861,-3.9555673082116,0.));
#53011=CARTESIAN_POINT('Ctrl Pts',(74.1920827166861,-3.9555673082116,12.));
#53012=CARTESIAN_POINT('Ctrl Pts',(74.217893549314,-3.94546216377499,0.));
#53013=CARTESIAN_POINT('Ctrl Pts',(74.217893549314,-3.94546216377499,12.));
#53014=CARTESIAN_POINT('Ctrl Pts',(74.2437276593763,-3.9353209977423,0.));
#53015=CARTESIAN_POINT('Ctrl Pts',(74.2437276593763,-3.9353209977423,12.));
#53016=CARTESIAN_POINT('Ctrl Pts',(74.2695849516134,-3.92514379920729,0.));
#53017=CARTESIAN_POINT('Ctrl Pts',(74.2695849516134,-3.92514379920729,12.));
#53018=CARTESIAN_POINT('Ctrl Pts',(74.2954653518346,-3.91493056284964,0.));
#53019=CARTESIAN_POINT('Ctrl Pts',(74.2954653518346,-3.91493056284964,12.));
#53020=CARTESIAN_POINT('Ctrl Pts',(74.3213688089495,-3.9046812890452,0.));
#53021=CARTESIAN_POINT('Ctrl Pts',(74.3213688089495,-3.9046812890452,12.));
#53022=CARTESIAN_POINT('Ctrl Pts',(74.3472952898,-3.89439598145194,0.));
#53023=CARTESIAN_POINT('Ctrl Pts',(74.3472952898,-3.89439598145194,12.));
#53024=CARTESIAN_POINT('Ctrl Pts',(74.3680548786039,-3.8861389124787,0.));
#53025=CARTESIAN_POINT('Ctrl Pts',(74.3680548786039,-3.8861389124787,12.));
#53026=CARTESIAN_POINT('Ctrl Pts',(74.3836349188809,-3.87992989995678,0.));
#53027=CARTESIAN_POINT('Ctrl Pts',(74.3836349188809,-3.87992989995678,12.));
#53028=CARTESIAN_POINT('Ctrl Pts',(74.3940262116251,-3.87578335377301,0.));
#53029=CARTESIAN_POINT('Ctrl Pts',(74.3940262116251,-3.87578335377301,12.));
#53030=CARTESIAN_POINT('Ctrl Pts',(74.3992230078037,-3.87370827955545,0.));
#53031=CARTESIAN_POINT('Ctrl Pts',(74.3992230078037,-3.87370827955545,12.));
#53032=CARTESIAN_POINT('',(69.8028570375097,-5.24987136994593,0.));
#53033=CARTESIAN_POINT('Ctrl Pts',(69.8028570375097,-5.24987136994593,0.));
#53034=CARTESIAN_POINT('Ctrl Pts',(69.8066748687772,-5.24915955997427,0.));
#53035=CARTESIAN_POINT('Ctrl Pts',(69.8143154684204,-5.24773285666377,0.));
#53036=CARTESIAN_POINT('Ctrl Pts',(69.8257911792159,-5.24558355159751,0.));
#53037=CARTESIAN_POINT('Ctrl Pts',(69.841121750752,-5.2426993105457,0.));
#53038=CARTESIAN_POINT('Ctrl Pts',(69.8603343302743,-5.23906316634803,0.));
#53039=CARTESIAN_POINT('Ctrl Pts',(69.8795962381599,-5.2353961627962,0.));
#53040=CARTESIAN_POINT('Ctrl Pts',(69.8989073936688,-5.23169827290556,0.));
#53041=CARTESIAN_POINT('Ctrl Pts',(69.9182676502048,-5.22796945602794,0.));
#53042=CARTESIAN_POINT('Ctrl Pts',(69.9376767969095,-5.22420965879982,0.));
#53043=CARTESIAN_POINT('Ctrl Pts',(69.9571345870076,-5.22041882075721,0.));
#53044=CARTESIAN_POINT('Ctrl Pts',(69.9766407595385,-5.21659687881139,0.));
#53045=CARTESIAN_POINT('Ctrl Pts',(69.9961950629965,-5.2127437720326,0.));
#53046=CARTESIAN_POINT('Ctrl Pts',(70.0157972802182,-5.20885944672837,0.));
#53047=CARTESIAN_POINT('Ctrl Pts',(70.0354472203546,-5.20494385478026,0.));
#53048=CARTESIAN_POINT('Ctrl Pts',(70.0551447071082,-5.20099695122656,0.));
#53049=CARTESIAN_POINT('Ctrl Pts',(70.0748895689729,-5.19701869225529,0.));
#53050=CARTESIAN_POINT('Ctrl Pts',(70.0946816270997,-5.1930090327158,0.));
#53051=CARTESIAN_POINT('Ctrl Pts',(70.1145206891885,-5.18896792486566,0.));
#53052=CARTESIAN_POINT('Ctrl Pts',(70.1344065558145,-5.18489531966265,0.));
#53053=CARTESIAN_POINT('Ctrl Pts',(70.1543390243892,-5.18079116757667,0.));
#53054=CARTESIAN_POINT('Ctrl Pts',(70.1743178937077,-5.17665541952383,0.));
#53055=CARTESIAN_POINT('Ctrl Pts',(70.1943429691167,-5.17248802793389,0.));
#53056=CARTESIAN_POINT('Ctrl Pts',(70.2144140622953,-5.16828894670109,0.));
#53057=CARTESIAN_POINT('Ctrl Pts',(70.2345309887833,-5.16405813066976,0.));
#53058=CARTESIAN_POINT('Ctrl Pts',(70.2546935662722,-5.15979553528204,0.));
#53059=CARTESIAN_POINT('Ctrl Pts',(70.2749016125105,-5.1555011161486,0.));
#53060=CARTESIAN_POINT('Ctrl Pts',(70.2951549435512,-5.15117482869254,0.));
#53061=CARTESIAN_POINT('Ctrl Pts',(70.3154533746736,-5.1468166283308,0.));
#53062=CARTESIAN_POINT('Ctrl Pts',(70.3357967211796,-5.1424264706348,0.));
#53063=CARTESIAN_POINT('Ctrl Pts',(70.3561847991714,-5.13800431148904,0.));
#53064=CARTESIAN_POINT('Ctrl Pts',(70.3766174264757,-5.13355010728568,0.));
#53065=CARTESIAN_POINT('Ctrl Pts',(70.3970944229851,-5.12906381499456,0.));
#53066=CARTESIAN_POINT('Ctrl Pts',(70.417615610161,-5.12454539205329,0.));
#53067=CARTESIAN_POINT('Ctrl Pts',(70.4381808107245,-5.11999479630212,0.));
#53068=CARTESIAN_POINT('Ctrl Pts',(70.458789848296,-5.11541198590933,0.));
#53069=CARTESIAN_POINT('Ctrl Pts',(70.4794425469825,-5.11079691929213,0.));
#53070=CARTESIAN_POINT('Ctrl Pts',(70.500138731399,-5.10614955511664,0.));
#53071=CARTESIAN_POINT('Ctrl Pts',(70.5208782268497,-5.10146985232941,0.));
#53072=CARTESIAN_POINT('Ctrl Pts',(70.5416608594526,-5.09675777018183,0.));
#53073=CARTESIAN_POINT('Ctrl Pts',(70.5624864562824,-5.09201326826135,0.));
#53074=CARTESIAN_POINT('Ctrl Pts',(70.5833548455014,-5.08723630652273,0.));
#53075=CARTESIAN_POINT('Ctrl Pts',(70.6042658562923,-5.08242684526687,0.));
#53076=CARTESIAN_POINT('Ctrl Pts',(70.6252193187878,-5.07758484512303,0.));
#53077=CARTESIAN_POINT('Ctrl Pts',(70.6462150640015,-5.07271026703355,0.));
#53078=CARTESIAN_POINT('Ctrl Pts',(70.6672529237455,-5.06780307224072,0.));
#53079=CARTESIAN_POINT('Ctrl Pts',(70.6883327305784,-5.0628632222782,0.));
#53080=CARTESIAN_POINT('Ctrl Pts',(70.7094543178438,-5.05789067897058,0.));
#53081=CARTESIAN_POINT('Ctrl Pts',(70.7306175196863,-5.05288540443483,0.));
#53082=CARTESIAN_POINT('Ctrl Pts',(70.7518221710706,-5.04784736108346,0.));
#53083=CARTESIAN_POINT('Ctrl Pts',(70.7730681077983,-5.0427765116335,0.));
#53084=CARTESIAN_POINT('Ctrl Pts',(70.7943551665059,-5.03767281910479,0.));
#53085=CARTESIAN_POINT('Ctrl Pts',(70.8156831846488,-5.03253624680941,0.));
#53086=CARTESIAN_POINT('Ctrl Pts',(70.8370520004843,-5.02736675834693,0.));
#53087=CARTESIAN_POINT('Ctrl Pts',(70.8584614530519,-5.02216431760061,0.));
#53088=CARTESIAN_POINT('Ctrl Pts',(70.8799113821452,-5.0169288887379,0.));
#53089=CARTESIAN_POINT('Ctrl Pts',(70.9014016283124,-5.01166043620568,0.));
#53090=CARTESIAN_POINT('Ctrl Pts',(70.9229320328589,-5.00635892472514,0.));
#53091=CARTESIAN_POINT('Ctrl Pts',(70.9445024378439,-5.0010243192904,0.));
#53092=CARTESIAN_POINT('Ctrl Pts',(70.9661126860773,-4.99565658516913,0.));
#53093=CARTESIAN_POINT('Ctrl Pts',(70.9877626211113,-4.99025568790665,0.));
#53094=CARTESIAN_POINT('Ctrl Pts',(71.0094520872377,-4.98482159331864,0.));
#53095=CARTESIAN_POINT('Ctrl Pts',(71.0311809294821,-4.97935426748585,0.));
#53096=CARTESIAN_POINT('Ctrl Pts',(71.0529489935961,-4.97385367675159,0.));
#53097=CARTESIAN_POINT('Ctrl Pts',(71.0747561260436,-4.96831978772191,0.));
#53098=CARTESIAN_POINT('Ctrl Pts',(71.0966021739907,-4.96275256726766,0.));
#53099=CARTESIAN_POINT('Ctrl Pts',(71.1184869853056,-4.95715198251685,0.));
#53100=CARTESIAN_POINT('Ctrl Pts',(71.1404104085552,-4.95151800085102,0.));
#53101=CARTESIAN_POINT('Ctrl Pts',(71.1623722930001,-4.94585058990341,0.));
#53102=CARTESIAN_POINT('Ctrl Pts',(71.1843724885847,-4.94014971756115,0.));
#53103=CARTESIAN_POINT('Ctrl Pts',(71.2064108459286,-4.93441535196618,0.));
#53104=CARTESIAN_POINT('Ctrl Pts',(71.2284872163273,-4.92864746150733,0.));
#53105=CARTESIAN_POINT('Ctrl Pts',(71.250601451747,-4.92284601481722,0.));
#53106=CARTESIAN_POINT('Ctrl Pts',(71.2727534048192,-4.91701098077036,0.));
#53107=CARTESIAN_POINT('Ctrl Pts',(71.294942928829,-4.91114232848603,0.));
#53108=CARTESIAN_POINT('Ctrl Pts',(71.3171698777084,-4.90524002732779,0.));
#53109=CARTESIAN_POINT('Ctrl Pts',(71.3394341060359,-4.89930404689575,0.));
#53110=CARTESIAN_POINT('Ctrl Pts',(71.3617354690325,-4.89333435702414,0.));
#53111=CARTESIAN_POINT('Ctrl Pts',(71.3840738225562,-4.88733092777975,0.));
#53112=CARTESIAN_POINT('Ctrl Pts',(71.4064490230899,-4.88129372946552,0.));
#53113=CARTESIAN_POINT('Ctrl Pts',(71.4288609277374,-4.87522273261908,0.));
#53114=CARTESIAN_POINT('Ctrl Pts',(71.4513093942255,-4.8691179080055,0.));
#53115=CARTESIAN_POINT('Ctrl Pts',(71.4737942808982,-4.86297922661503,0.));
#53116=CARTESIAN_POINT('Ctrl Pts',(71.4963154467113,-4.85680665966181,0.));
#53117=CARTESIAN_POINT('Ctrl Pts',(71.5188727512197,-4.8506001785878,0.));
#53118=CARTESIAN_POINT('Ctrl Pts',(71.5414660545739,-4.84435975506049,0.));
#53119=CARTESIAN_POINT('Ctrl Pts',(71.564095217521,-4.83808536096584,0.));
#53120=CARTESIAN_POINT('Ctrl Pts',(71.5867601014,-4.83177696840638,0.));
#53121=CARTESIAN_POINT('Ctrl Pts',(71.6094605681366,-4.82543454970027,0.));
#53122=CARTESIAN_POINT('Ctrl Pts',(71.6321964802326,-4.81905807738557,0.));
#53123=CARTESIAN_POINT('Ctrl Pts',(71.6549677007613,-4.81264752421732,0.));
#53124=CARTESIAN_POINT('Ctrl Pts',(71.6777740933705,-4.80620286316089,0.));
#53125=CARTESIAN_POINT('Ctrl Pts',(71.7006155222766,-4.79972406739014,0.));
#53126=CARTESIAN_POINT('Ctrl Pts',(71.7234918522604,-4.79321111028672,0.));
#53127=CARTESIAN_POINT('Ctrl Pts',(71.7464029486552,-4.78666396544451,0.));
#53128=CARTESIAN_POINT('Ctrl Pts',(71.7693486773449,-4.78008260666643,0.));
#53129=CARTESIAN_POINT('Ctrl Pts',(71.7923289047636,-4.77346700795788,0.));
#53130=CARTESIAN_POINT('Ctrl Pts',(71.8153434978924,-4.76681714352504,0.));
#53131=CARTESIAN_POINT('Ctrl Pts',(71.8383923242533,-4.76013298777423,0.));
#53132=CARTESIAN_POINT('Ctrl Pts',(71.8614752519008,-4.75341451531671,0.));
#53133=CARTESIAN_POINT('Ctrl Pts',(71.8845921494186,-4.74666170096546,0.));
#53134=CARTESIAN_POINT('Ctrl Pts',(71.9077428859207,-4.73987451972861,0.));
#53135=CARTESIAN_POINT('Ctrl Pts',(71.9309273310469,-4.73305294680784,0.));
#53136=CARTESIAN_POINT('Ctrl Pts',(71.9541453549582,-4.72619695759779,0.));
#53137=CARTESIAN_POINT('Ctrl Pts',(71.9773968283267,-4.71930652769081,0.));
#53138=CARTESIAN_POINT('Ctrl Pts',(72.0006816223335,-4.71238163287411,0.));
#53139=CARTESIAN_POINT('Ctrl Pts',(72.0239996086694,-4.70542224912312,0.));
#53140=CARTESIAN_POINT('Ctrl Pts',(72.047350659532,-4.69842835259997,0.));
#53141=CARTESIAN_POINT('Ctrl Pts',(72.070734647621,-4.6913999196528,0.));
#53142=CARTESIAN_POINT('Ctrl Pts',(72.0941514461283,-4.68433692682061,0.));
#53143=CARTESIAN_POINT('Ctrl Pts',(72.1176009287349,-4.67723935083087,0.));
#53144=CARTESIAN_POINT('Ctrl Pts',(72.1410829696129,-4.67010716859281,0.));
#53145=CARTESIAN_POINT('Ctrl Pts',(72.1645974434218,-4.6629403571957,0.));
#53146=CARTESIAN_POINT('Ctrl Pts',(72.1881442253052,-4.65573889390825,0.));
#53147=CARTESIAN_POINT('Ctrl Pts',(72.2117231908816,-4.64850275618325,0.));
#53148=CARTESIAN_POINT('Ctrl Pts',(72.2353342162408,-4.64123192165628,0.));
#53149=CARTESIAN_POINT('Ctrl Pts',(72.2589771779447,-4.63392636813842,0.));
#53150=CARTESIAN_POINT('Ctrl Pts',(72.2826519530254,-4.62658607361465,0.));
#53151=CARTESIAN_POINT('Ctrl Pts',(72.306358418981,-4.61921101624295,0.));
#53152=CARTESIAN_POINT('Ctrl Pts',(72.330096453767,-4.61180117435869,0.));
#53153=CARTESIAN_POINT('Ctrl Pts',(72.3538659357932,-4.60435652647463,0.));
#53154=CARTESIAN_POINT('Ctrl Pts',(72.3776667439244,-4.5968770512734,0.));
#53155=CARTESIAN_POINT('Ctrl Pts',(72.4014987574789,-4.58936272760551,0.));
#53156=CARTESIAN_POINT('Ctrl Pts',(72.4253618562249,-4.58181353448851,0.));
#53157=CARTESIAN_POINT('Ctrl Pts',(72.449255920373,-4.57422945111094,0.));
#53158=CARTESIAN_POINT('Ctrl Pts',(72.473180830571,-4.56661045683367,0.));
#53159=CARTESIAN_POINT('Ctrl Pts',(72.4971364679055,-4.55895653118214,0.));
#53160=CARTESIAN_POINT('Ctrl Pts',(72.5211227138997,-4.55126765384403,0.));
#53161=CARTESIAN_POINT('Ctrl Pts',(72.5451394505106,-4.54354380466825,0.));
#53162=CARTESIAN_POINT('Ctrl Pts',(72.5691865601225,-4.53578496366802,0.));
#53163=CARTESIAN_POINT('Ctrl Pts',(72.5932639255406,-4.5279911110239,0.));
#53164=CARTESIAN_POINT('Ctrl Pts',(72.6173714299935,-4.52016222707632,0.));
#53165=CARTESIAN_POINT('Ctrl Pts',(72.6415089571314,-4.5122982923226,0.));
#53166=CARTESIAN_POINT('Ctrl Pts',(72.6656763910241,-4.50439928741605,0.));
#53167=CARTESIAN_POINT('Ctrl Pts',(72.689873616155,-4.49646519316822,0.));
#53168=CARTESIAN_POINT('Ctrl Pts',(72.7141005174153,-4.48849599055354,0.));
#53169=CARTESIAN_POINT('Ctrl Pts',(72.7383569801042,-4.48049166070223,0.));
#53170=CARTESIAN_POINT('Ctrl Pts',(72.7626428899287,-4.47245218489623,0.));
#53171=CARTESIAN_POINT('Ctrl Pts',(72.7869581329994,-4.46437754456796,0.));
#53172=CARTESIAN_POINT('Ctrl Pts',(72.8113025958258,-4.45626772130138,0.));
#53173=CARTESIAN_POINT('Ctrl Pts',(72.8356761653064,-4.44812269683724,0.));
#53174=CARTESIAN_POINT('Ctrl Pts',(72.8600787287316,-4.43994245306805,0.));
#53175=CARTESIAN_POINT('Ctrl Pts',(72.8845101737856,-4.43172697203342,0.));
#53176=CARTESIAN_POINT('Ctrl Pts',(72.9089703885463,-4.42347623591942,0.));
#53177=CARTESIAN_POINT('Ctrl Pts',(72.9334592614828,-4.41519022705927,0.));
#53178=CARTESIAN_POINT('Ctrl Pts',(72.9579766814495,-4.40686892793965,0.));
#53179=CARTESIAN_POINT('Ctrl Pts',(72.9825225376839,-4.39851232119731,0.));
#53180=CARTESIAN_POINT('Ctrl Pts',(73.0070967198033,-4.39012038961145,0.));
#53181=CARTESIAN_POINT('Ctrl Pts',(73.031699117799,-4.38169311610153,0.));
#53182=CARTESIAN_POINT('Ctrl Pts',(73.0563296220301,-4.37323048372607,0.));
#53183=CARTESIAN_POINT('Ctrl Pts',(73.0809881232111,-4.36473247568638,0.));
#53184=CARTESIAN_POINT('Ctrl Pts',(73.1056745124099,-4.35619907532716,0.));
#53185=CARTESIAN_POINT('Ctrl Pts',(73.1303886810602,-4.34763026613155,0.));
#53186=CARTESIAN_POINT('Ctrl Pts',(73.1551305209692,-4.3390260317214,0.));
#53187=CARTESIAN_POINT('Ctrl Pts',(73.1798999243234,-4.33038635585878,0.));
#53188=CARTESIAN_POINT('Ctrl Pts',(73.204696783693,-4.32171122245219,0.));
#53189=CARTESIAN_POINT('Ctrl Pts',(73.2295209920319,-4.31300061556103,0.));
#53190=CARTESIAN_POINT('Ctrl Pts',(73.2543724426562,-4.30425451938234,0.));
#53191=CARTESIAN_POINT('Ctrl Pts',(73.2792510292243,-4.29547291824289,0.));
#53192=CARTESIAN_POINT('Ctrl Pts',(73.3041566457134,-4.28665579659302,0.));
#53193=CARTESIAN_POINT('Ctrl Pts',(73.3290891863959,-4.27780313900392,0.));
#53194=CARTESIAN_POINT('Ctrl Pts',(73.354048545808,-4.26891493016703,0.));
#53195=CARTESIAN_POINT('Ctrl Pts',(73.3790346187953,-4.25999115489905,0.));
#53196=CARTESIAN_POINT('Ctrl Pts',(73.4040473005603,-4.25103179814892,0.));
#53197=CARTESIAN_POINT('Ctrl Pts',(73.4290864867103,-4.24203684500941,0.));
#53198=CARTESIAN_POINT('Ctrl Pts',(73.4541520732943,-4.23300628072758,0.));
#53199=CARTESIAN_POINT('Ctrl Pts',(73.4792439568624,-4.22394009072753,0.));
#53200=CARTESIAN_POINT('Ctrl Pts',(73.5043620344107,-4.21483826059437,0.));
#53201=CARTESIAN_POINT('Ctrl Pts',(73.5295062032621,-4.20570077603727,0.));
#53202=CARTESIAN_POINT('Ctrl Pts',(73.554676360957,-4.19652762286127,0.));
#53203=CARTESIAN_POINT('Ctrl Pts',(73.5798724051519,-4.18731878694238,0.));
#53204=CARTESIAN_POINT('Ctrl Pts',(73.6050942334773,-4.17807425419817,0.));
#53205=CARTESIAN_POINT('Ctrl Pts',(73.6303417435262,-4.16879401058787,0.));
#53206=CARTESIAN_POINT('Ctrl Pts',(73.6556148331504,-4.15947804217791,0.));
#53207=CARTESIAN_POINT('Ctrl Pts',(73.6809134006909,-4.15012633519728,0.));
#53208=CARTESIAN_POINT('Ctrl Pts',(73.7062373452344,-4.14073887610155,0.));
#53209=CARTESIAN_POINT('Ctrl Pts',(73.7315865668508,-4.13131565163575,0.));
#53210=CARTESIAN_POINT('Ctrl Pts',(73.7569609668501,-4.12185664890551,0.));
#53211=CARTESIAN_POINT('Ctrl Pts',(73.7823604472126,-4.1123618552278,0.));
#53212=CARTESIAN_POINT('Ctrl Pts',(73.8077849100314,-4.10283125798724,0.));
#53213=CARTESIAN_POINT('Ctrl Pts',(73.8332342568978,-4.09326484448232,0.));
#53214=CARTESIAN_POINT('Ctrl Pts',(73.8587083884208,-4.0836626018068,0.));
#53215=CARTESIAN_POINT('Ctrl Pts',(73.884207203405,-4.07402451665253,0.));
#53216=CARTESIAN_POINT('Ctrl Pts',(73.9097305995173,-4.06435057547335,0.));
#53217=CARTESIAN_POINT('Ctrl Pts',(73.9352784747665,-4.05464076484762,0.));
#53218=CARTESIAN_POINT('Ctrl Pts',(73.9608507287943,-4.04489507179964,0.));
#53219=CARTESIAN_POINT('Ctrl Pts',(73.9864472641025,-4.0351134841066,0.));
#53220=CARTESIAN_POINT('Ctrl Pts',(74.0120679876396,-4.02529599070085,0.));
#53221=CARTESIAN_POINT('Ctrl Pts',(74.0377128111754,-4.01544258176693,0.));
#53222=CARTESIAN_POINT('Ctrl Pts',(74.0597159781918,-4.00696550627607,0.));
#53223=CARTESIAN_POINT('Ctrl Pts',(74.0765982943431,-4.00044689712493,0.));
#53224=CARTESIAN_POINT('Ctrl Pts',(74.0883491449661,-3.9959026674777,0.));
#53225=CARTESIAN_POINT('Ctrl Pts',(74.0949615399273,-3.99334334446576,0.));
#53226=CARTESIAN_POINT('Ctrl Pts',(74.0964320765796,-3.99277406492185,0.));
#53227=CARTESIAN_POINT('',(69.8028570375097,-5.24987136994593,12.));
#53228=CARTESIAN_POINT('',(69.8028570375097,-5.24987136994593,0.));
#53229=CARTESIAN_POINT('Ctrl Pts',(74.0964320765796,-3.99277406492185,12.));
#53230=CARTESIAN_POINT('Ctrl Pts',(74.0949615399273,-3.99334334446576,12.));
#53231=CARTESIAN_POINT('Ctrl Pts',(74.0883491449661,-3.9959026674777,12.));
#53232=CARTESIAN_POINT('Ctrl Pts',(74.0765982943431,-4.00044689712493,12.));
#53233=CARTESIAN_POINT('Ctrl Pts',(74.0597159781918,-4.00696550627607,12.));
#53234=CARTESIAN_POINT('Ctrl Pts',(74.0377128111754,-4.01544258176693,12.));
#53235=CARTESIAN_POINT('Ctrl Pts',(74.0120679876396,-4.02529599070085,12.));
#53236=CARTESIAN_POINT('Ctrl Pts',(73.9864472641025,-4.0351134841066,12.));
#53237=CARTESIAN_POINT('Ctrl Pts',(73.9608507287943,-4.04489507179964,12.));
#53238=CARTESIAN_POINT('Ctrl Pts',(73.9352784747665,-4.05464076484762,12.));
#53239=CARTESIAN_POINT('Ctrl Pts',(73.9097305995173,-4.06435057547335,12.));
#53240=CARTESIAN_POINT('Ctrl Pts',(73.884207203405,-4.07402451665253,12.));
#53241=CARTESIAN_POINT('Ctrl Pts',(73.8587083884208,-4.0836626018068,12.));
#53242=CARTESIAN_POINT('Ctrl Pts',(73.8332342568978,-4.09326484448232,12.));
#53243=CARTESIAN_POINT('Ctrl Pts',(73.8077849100314,-4.10283125798724,12.));
#53244=CARTESIAN_POINT('Ctrl Pts',(73.7823604472126,-4.1123618552278,12.));
#53245=CARTESIAN_POINT('Ctrl Pts',(73.7569609668501,-4.12185664890551,12.));
#53246=CARTESIAN_POINT('Ctrl Pts',(73.7315865668508,-4.13131565163575,12.));
#53247=CARTESIAN_POINT('Ctrl Pts',(73.7062373452344,-4.14073887610155,12.));
#53248=CARTESIAN_POINT('Ctrl Pts',(73.6809134006909,-4.15012633519728,12.));
#53249=CARTESIAN_POINT('Ctrl Pts',(73.6556148331504,-4.15947804217791,12.));
#53250=CARTESIAN_POINT('Ctrl Pts',(73.6303417435262,-4.16879401058787,12.));
#53251=CARTESIAN_POINT('Ctrl Pts',(73.6050942334773,-4.17807425419817,12.));
#53252=CARTESIAN_POINT('Ctrl Pts',(73.5798724051519,-4.18731878694238,12.));
#53253=CARTESIAN_POINT('Ctrl Pts',(73.554676360957,-4.19652762286127,12.));
#53254=CARTESIAN_POINT('Ctrl Pts',(73.5295062032621,-4.20570077603727,12.));
#53255=CARTESIAN_POINT('Ctrl Pts',(73.5043620344107,-4.21483826059437,12.));
#53256=CARTESIAN_POINT('Ctrl Pts',(73.4792439568624,-4.22394009072753,12.));
#53257=CARTESIAN_POINT('Ctrl Pts',(73.4541520732943,-4.23300628072758,12.));
#53258=CARTESIAN_POINT('Ctrl Pts',(73.4290864867103,-4.24203684500941,12.));
#53259=CARTESIAN_POINT('Ctrl Pts',(73.4040473005603,-4.25103179814892,12.));
#53260=CARTESIAN_POINT('Ctrl Pts',(73.3790346187953,-4.25999115489905,12.));
#53261=CARTESIAN_POINT('Ctrl Pts',(73.354048545808,-4.26891493016703,12.));
#53262=CARTESIAN_POINT('Ctrl Pts',(73.3290891863959,-4.27780313900392,12.));
#53263=CARTESIAN_POINT('Ctrl Pts',(73.3041566457134,-4.28665579659302,12.));
#53264=CARTESIAN_POINT('Ctrl Pts',(73.2792510292243,-4.29547291824289,12.));
#53265=CARTESIAN_POINT('Ctrl Pts',(73.2543724426562,-4.30425451938234,12.));
#53266=CARTESIAN_POINT('Ctrl Pts',(73.2295209920319,-4.31300061556103,12.));
#53267=CARTESIAN_POINT('Ctrl Pts',(73.204696783693,-4.32171122245219,12.));
#53268=CARTESIAN_POINT('Ctrl Pts',(73.1798999243234,-4.33038635585878,12.));
#53269=CARTESIAN_POINT('Ctrl Pts',(73.1551305209692,-4.3390260317214,12.));
#53270=CARTESIAN_POINT('Ctrl Pts',(73.1303886810602,-4.34763026613155,12.));
#53271=CARTESIAN_POINT('Ctrl Pts',(73.1056745124099,-4.35619907532716,12.));
#53272=CARTESIAN_POINT('Ctrl Pts',(73.0809881232111,-4.36473247568638,12.));
#53273=CARTESIAN_POINT('Ctrl Pts',(73.0563296220301,-4.37323048372607,12.));
#53274=CARTESIAN_POINT('Ctrl Pts',(73.031699117799,-4.38169311610153,12.));
#53275=CARTESIAN_POINT('Ctrl Pts',(73.0070967198033,-4.39012038961145,12.));
#53276=CARTESIAN_POINT('Ctrl Pts',(72.9825225376839,-4.39851232119731,12.));
#53277=CARTESIAN_POINT('Ctrl Pts',(72.9579766814495,-4.40686892793965,12.));
#53278=CARTESIAN_POINT('Ctrl Pts',(72.9334592614828,-4.41519022705927,12.));
#53279=CARTESIAN_POINT('Ctrl Pts',(72.9089703885463,-4.42347623591942,12.));
#53280=CARTESIAN_POINT('Ctrl Pts',(72.8845101737856,-4.43172697203342,12.));
#53281=CARTESIAN_POINT('Ctrl Pts',(72.8600787287316,-4.43994245306805,12.));
#53282=CARTESIAN_POINT('Ctrl Pts',(72.8356761653064,-4.44812269683724,12.));
#53283=CARTESIAN_POINT('Ctrl Pts',(72.8113025958258,-4.45626772130138,12.));
#53284=CARTESIAN_POINT('Ctrl Pts',(72.7869581329994,-4.46437754456796,12.));
#53285=CARTESIAN_POINT('Ctrl Pts',(72.7626428899287,-4.47245218489623,12.));
#53286=CARTESIAN_POINT('Ctrl Pts',(72.7383569801042,-4.48049166070223,12.));
#53287=CARTESIAN_POINT('Ctrl Pts',(72.7141005174153,-4.48849599055354,12.));
#53288=CARTESIAN_POINT('Ctrl Pts',(72.689873616155,-4.49646519316822,12.));
#53289=CARTESIAN_POINT('Ctrl Pts',(72.6656763910241,-4.50439928741605,12.));
#53290=CARTESIAN_POINT('Ctrl Pts',(72.6415089571314,-4.5122982923226,12.));
#53291=CARTESIAN_POINT('Ctrl Pts',(72.6173714299935,-4.52016222707632,12.));
#53292=CARTESIAN_POINT('Ctrl Pts',(72.5932639255406,-4.5279911110239,12.));
#53293=CARTESIAN_POINT('Ctrl Pts',(72.5691865601225,-4.53578496366802,12.));
#53294=CARTESIAN_POINT('Ctrl Pts',(72.5451394505106,-4.54354380466825,12.));
#53295=CARTESIAN_POINT('Ctrl Pts',(72.5211227138997,-4.55126765384403,12.));
#53296=CARTESIAN_POINT('Ctrl Pts',(72.4971364679055,-4.55895653118214,12.));
#53297=CARTESIAN_POINT('Ctrl Pts',(72.473180830571,-4.56661045683367,12.));
#53298=CARTESIAN_POINT('Ctrl Pts',(72.449255920373,-4.57422945111094,12.));
#53299=CARTESIAN_POINT('Ctrl Pts',(72.4253618562249,-4.58181353448851,12.));
#53300=CARTESIAN_POINT('Ctrl Pts',(72.4014987574789,-4.58936272760551,12.));
#53301=CARTESIAN_POINT('Ctrl Pts',(72.3776667439244,-4.5968770512734,12.));
#53302=CARTESIAN_POINT('Ctrl Pts',(72.3538659357932,-4.60435652647463,12.));
#53303=CARTESIAN_POINT('Ctrl Pts',(72.330096453767,-4.61180117435869,12.));
#53304=CARTESIAN_POINT('Ctrl Pts',(72.306358418981,-4.61921101624295,12.));
#53305=CARTESIAN_POINT('Ctrl Pts',(72.2826519530254,-4.62658607361465,12.));
#53306=CARTESIAN_POINT('Ctrl Pts',(72.2589771779447,-4.63392636813842,12.));
#53307=CARTESIAN_POINT('Ctrl Pts',(72.2353342162408,-4.64123192165628,12.));
#53308=CARTESIAN_POINT('Ctrl Pts',(72.2117231908816,-4.64850275618325,12.));
#53309=CARTESIAN_POINT('Ctrl Pts',(72.1881442253052,-4.65573889390825,12.));
#53310=CARTESIAN_POINT('Ctrl Pts',(72.1645974434218,-4.6629403571957,12.));
#53311=CARTESIAN_POINT('Ctrl Pts',(72.1410829696129,-4.67010716859281,12.));
#53312=CARTESIAN_POINT('Ctrl Pts',(72.1176009287349,-4.67723935083087,12.));
#53313=CARTESIAN_POINT('Ctrl Pts',(72.0941514461283,-4.68433692682061,12.));
#53314=CARTESIAN_POINT('Ctrl Pts',(72.070734647621,-4.6913999196528,12.));
#53315=CARTESIAN_POINT('Ctrl Pts',(72.047350659532,-4.69842835259997,12.));
#53316=CARTESIAN_POINT('Ctrl Pts',(72.0239996086694,-4.70542224912312,12.));
#53317=CARTESIAN_POINT('Ctrl Pts',(72.0006816223335,-4.71238163287411,12.));
#53318=CARTESIAN_POINT('Ctrl Pts',(71.9773968283267,-4.71930652769081,12.));
#53319=CARTESIAN_POINT('Ctrl Pts',(71.9541453549582,-4.72619695759779,12.));
#53320=CARTESIAN_POINT('Ctrl Pts',(71.9309273310469,-4.73305294680784,12.));
#53321=CARTESIAN_POINT('Ctrl Pts',(71.9077428859207,-4.73987451972861,12.));
#53322=CARTESIAN_POINT('Ctrl Pts',(71.8845921494186,-4.74666170096546,12.));
#53323=CARTESIAN_POINT('Ctrl Pts',(71.8614752519008,-4.75341451531671,12.));
#53324=CARTESIAN_POINT('Ctrl Pts',(71.8383923242533,-4.76013298777423,12.));
#53325=CARTESIAN_POINT('Ctrl Pts',(71.8153434978924,-4.76681714352504,12.));
#53326=CARTESIAN_POINT('Ctrl Pts',(71.7923289047636,-4.77346700795788,12.));
#53327=CARTESIAN_POINT('Ctrl Pts',(71.7693486773449,-4.78008260666643,12.));
#53328=CARTESIAN_POINT('Ctrl Pts',(71.7464029486552,-4.78666396544451,12.));
#53329=CARTESIAN_POINT('Ctrl Pts',(71.7234918522604,-4.79321111028672,12.));
#53330=CARTESIAN_POINT('Ctrl Pts',(71.7006155222766,-4.79972406739014,12.));
#53331=CARTESIAN_POINT('Ctrl Pts',(71.6777740933705,-4.80620286316089,12.));
#53332=CARTESIAN_POINT('Ctrl Pts',(71.6549677007613,-4.81264752421732,12.));
#53333=CARTESIAN_POINT('Ctrl Pts',(71.6321964802326,-4.81905807738557,12.));
#53334=CARTESIAN_POINT('Ctrl Pts',(71.6094605681366,-4.82543454970027,12.));
#53335=CARTESIAN_POINT('Ctrl Pts',(71.5867601014,-4.83177696840638,12.));
#53336=CARTESIAN_POINT('Ctrl Pts',(71.564095217521,-4.83808536096584,12.));
#53337=CARTESIAN_POINT('Ctrl Pts',(71.5414660545739,-4.84435975506049,12.));
#53338=CARTESIAN_POINT('Ctrl Pts',(71.5188727512197,-4.8506001785878,12.));
#53339=CARTESIAN_POINT('Ctrl Pts',(71.4963154467113,-4.85680665966181,12.));
#53340=CARTESIAN_POINT('Ctrl Pts',(71.4737942808982,-4.86297922661503,12.));
#53341=CARTESIAN_POINT('Ctrl Pts',(71.4513093942255,-4.8691179080055,12.));
#53342=CARTESIAN_POINT('Ctrl Pts',(71.4288609277374,-4.87522273261908,12.));
#53343=CARTESIAN_POINT('Ctrl Pts',(71.4064490230899,-4.88129372946552,12.));
#53344=CARTESIAN_POINT('Ctrl Pts',(71.3840738225562,-4.88733092777975,12.));
#53345=CARTESIAN_POINT('Ctrl Pts',(71.3617354690325,-4.89333435702414,12.));
#53346=CARTESIAN_POINT('Ctrl Pts',(71.3394341060359,-4.89930404689575,12.));
#53347=CARTESIAN_POINT('Ctrl Pts',(71.3171698777084,-4.90524002732779,12.));
#53348=CARTESIAN_POINT('Ctrl Pts',(71.294942928829,-4.91114232848603,12.));
#53349=CARTESIAN_POINT('Ctrl Pts',(71.2727534048192,-4.91701098077036,12.));
#53350=CARTESIAN_POINT('Ctrl Pts',(71.250601451747,-4.92284601481722,12.));
#53351=CARTESIAN_POINT('Ctrl Pts',(71.2284872163273,-4.92864746150733,12.));
#53352=CARTESIAN_POINT('Ctrl Pts',(71.2064108459286,-4.93441535196618,12.));
#53353=CARTESIAN_POINT('Ctrl Pts',(71.1843724885847,-4.94014971756115,12.));
#53354=CARTESIAN_POINT('Ctrl Pts',(71.1623722930001,-4.94585058990341,12.));
#53355=CARTESIAN_POINT('Ctrl Pts',(71.1404104085552,-4.95151800085102,12.));
#53356=CARTESIAN_POINT('Ctrl Pts',(71.1184869853056,-4.95715198251685,12.));
#53357=CARTESIAN_POINT('Ctrl Pts',(71.0966021739907,-4.96275256726766,12.));
#53358=CARTESIAN_POINT('Ctrl Pts',(71.0747561260436,-4.96831978772191,12.));
#53359=CARTESIAN_POINT('Ctrl Pts',(71.0529489935961,-4.97385367675159,12.));
#53360=CARTESIAN_POINT('Ctrl Pts',(71.0311809294821,-4.97935426748585,12.));
#53361=CARTESIAN_POINT('Ctrl Pts',(71.0094520872377,-4.98482159331864,12.));
#53362=CARTESIAN_POINT('Ctrl Pts',(70.9877626211113,-4.99025568790665,12.));
#53363=CARTESIAN_POINT('Ctrl Pts',(70.9661126860773,-4.99565658516913,12.));
#53364=CARTESIAN_POINT('Ctrl Pts',(70.9445024378439,-5.0010243192904,12.));
#53365=CARTESIAN_POINT('Ctrl Pts',(70.9229320328589,-5.00635892472514,12.));
#53366=CARTESIAN_POINT('Ctrl Pts',(70.9014016283124,-5.01166043620568,12.));
#53367=CARTESIAN_POINT('Ctrl Pts',(70.8799113821452,-5.0169288887379,12.));
#53368=CARTESIAN_POINT('Ctrl Pts',(70.8584614530519,-5.02216431760061,12.));
#53369=CARTESIAN_POINT('Ctrl Pts',(70.8370520004843,-5.02736675834693,12.));
#53370=CARTESIAN_POINT('Ctrl Pts',(70.8156831846488,-5.03253624680941,12.));
#53371=CARTESIAN_POINT('Ctrl Pts',(70.7943551665059,-5.03767281910479,12.));
#53372=CARTESIAN_POINT('Ctrl Pts',(70.7730681077983,-5.0427765116335,12.));
#53373=CARTESIAN_POINT('Ctrl Pts',(70.7518221710706,-5.04784736108346,12.));
#53374=CARTESIAN_POINT('Ctrl Pts',(70.7306175196863,-5.05288540443483,12.));
#53375=CARTESIAN_POINT('Ctrl Pts',(70.7094543178438,-5.05789067897058,12.));
#53376=CARTESIAN_POINT('Ctrl Pts',(70.6883327305784,-5.0628632222782,12.));
#53377=CARTESIAN_POINT('Ctrl Pts',(70.6672529237455,-5.06780307224072,12.));
#53378=CARTESIAN_POINT('Ctrl Pts',(70.6462150640015,-5.07271026703355,12.));
#53379=CARTESIAN_POINT('Ctrl Pts',(70.6252193187878,-5.07758484512303,12.));
#53380=CARTESIAN_POINT('Ctrl Pts',(70.6042658562923,-5.08242684526687,12.));
#53381=CARTESIAN_POINT('Ctrl Pts',(70.5833548455014,-5.08723630652273,12.));
#53382=CARTESIAN_POINT('Ctrl Pts',(70.5624864562824,-5.09201326826135,12.));
#53383=CARTESIAN_POINT('Ctrl Pts',(70.5416608594526,-5.09675777018183,12.));
#53384=CARTESIAN_POINT('Ctrl Pts',(70.5208782268497,-5.10146985232941,12.));
#53385=CARTESIAN_POINT('Ctrl Pts',(70.500138731399,-5.10614955511664,12.));
#53386=CARTESIAN_POINT('Ctrl Pts',(70.4794425469825,-5.11079691929213,12.));
#53387=CARTESIAN_POINT('Ctrl Pts',(70.458789848296,-5.11541198590933,12.));
#53388=CARTESIAN_POINT('Ctrl Pts',(70.4381808107245,-5.11999479630212,12.));
#53389=CARTESIAN_POINT('Ctrl Pts',(70.417615610161,-5.12454539205329,12.));
#53390=CARTESIAN_POINT('Ctrl Pts',(70.3970944229851,-5.12906381499456,12.));
#53391=CARTESIAN_POINT('Ctrl Pts',(70.3766174264757,-5.13355010728568,12.));
#53392=CARTESIAN_POINT('Ctrl Pts',(70.3561847991714,-5.13800431148904,12.));
#53393=CARTESIAN_POINT('Ctrl Pts',(70.3357967211796,-5.1424264706348,12.));
#53394=CARTESIAN_POINT('Ctrl Pts',(70.3154533746736,-5.1468166283308,12.));
#53395=CARTESIAN_POINT('Ctrl Pts',(70.2951549435512,-5.15117482869254,12.));
#53396=CARTESIAN_POINT('Ctrl Pts',(70.2749016125105,-5.1555011161486,12.));
#53397=CARTESIAN_POINT('Ctrl Pts',(70.2546935662722,-5.15979553528204,12.));
#53398=CARTESIAN_POINT('Ctrl Pts',(70.2345309887833,-5.16405813066976,12.));
#53399=CARTESIAN_POINT('Ctrl Pts',(70.2144140622953,-5.16828894670109,12.));
#53400=CARTESIAN_POINT('Ctrl Pts',(70.1943429691167,-5.17248802793389,12.));
#53401=CARTESIAN_POINT('Ctrl Pts',(70.1743178937077,-5.17665541952383,12.));
#53402=CARTESIAN_POINT('Ctrl Pts',(70.1543390243892,-5.18079116757667,12.));
#53403=CARTESIAN_POINT('Ctrl Pts',(70.1344065558145,-5.18489531966265,12.));
#53404=CARTESIAN_POINT('Ctrl Pts',(70.1145206891885,-5.18896792486566,12.));
#53405=CARTESIAN_POINT('Ctrl Pts',(70.0946816270997,-5.1930090327158,12.));
#53406=CARTESIAN_POINT('Ctrl Pts',(70.0748895689729,-5.19701869225529,12.));
#53407=CARTESIAN_POINT('Ctrl Pts',(70.0551447071082,-5.20099695122656,12.));
#53408=CARTESIAN_POINT('Ctrl Pts',(70.0354472203546,-5.20494385478026,12.));
#53409=CARTESIAN_POINT('Ctrl Pts',(70.0157972802182,-5.20885944672837,12.));
#53410=CARTESIAN_POINT('Ctrl Pts',(69.9961950629965,-5.2127437720326,12.));
#53411=CARTESIAN_POINT('Ctrl Pts',(69.9766407595385,-5.21659687881139,12.));
#53412=CARTESIAN_POINT('Ctrl Pts',(69.9571345870076,-5.22041882075721,12.));
#53413=CARTESIAN_POINT('Ctrl Pts',(69.9376767969095,-5.22420965879982,12.));
#53414=CARTESIAN_POINT('Ctrl Pts',(69.9182676502048,-5.22796945602794,12.));
#53415=CARTESIAN_POINT('Ctrl Pts',(69.8989073936688,-5.23169827290556,12.));
#53416=CARTESIAN_POINT('Ctrl Pts',(69.8795962381599,-5.2353961627962,12.));
#53417=CARTESIAN_POINT('Ctrl Pts',(69.8603343302743,-5.23906316634803,12.));
#53418=CARTESIAN_POINT('Ctrl Pts',(69.841121750752,-5.2426993105457,12.));
#53419=CARTESIAN_POINT('Ctrl Pts',(69.8257911792159,-5.24558355159751,12.));
#53420=CARTESIAN_POINT('Ctrl Pts',(69.8143154684204,-5.24773285666377,12.));
#53421=CARTESIAN_POINT('Ctrl Pts',(69.8066748687772,-5.24915955997427,12.));
#53422=CARTESIAN_POINT('Ctrl Pts',(69.8028570375097,-5.24987136994593,12.));
#53423=CARTESIAN_POINT('Ctrl Pts',(74.1624659714955,-2.48034921844903,0.));
#53424=CARTESIAN_POINT('Ctrl Pts',(74.1624659714955,-2.48034921844903,4.));
#53425=CARTESIAN_POINT('Ctrl Pts',(74.1624659714955,-2.48034921844902,8.));
#53426=CARTESIAN_POINT('Ctrl Pts',(74.1624659714955,-2.48034921844902,12.));
#53427=CARTESIAN_POINT('Ctrl Pts',(74.2610905805699,-2.52879860312842,0.));
#53428=CARTESIAN_POINT('Ctrl Pts',(74.2610905805699,-2.52879860312842,4.));
#53429=CARTESIAN_POINT('Ctrl Pts',(74.2610905805699,-2.52879860312839,8.));
#53430=CARTESIAN_POINT('Ctrl Pts',(74.2610905805699,-2.52879860312839,12.));
#53431=CARTESIAN_POINT('Ctrl Pts',(74.4041075779822,-2.67239300265256,0.));
#53432=CARTESIAN_POINT('Ctrl Pts',(74.4041075779822,-2.67239300265256,4.));
#53433=CARTESIAN_POINT('Ctrl Pts',(74.4041075779824,-2.67239300265254,8.));
#53434=CARTESIAN_POINT('Ctrl Pts',(74.4041075779824,-2.67239300265254,12.));
#53435=CARTESIAN_POINT('Ctrl Pts',(74.4448761712984,-2.86656650944691,0.));
#53436=CARTESIAN_POINT('Ctrl Pts',(74.4448761712984,-2.86656650944691,4.));
#53437=CARTESIAN_POINT('Ctrl Pts',(74.4448761712985,-2.86656650944694,8.00000000000001));
#53438=CARTESIAN_POINT('Ctrl Pts',(74.4448761712985,-2.86656650944694,12.));
#53439=CARTESIAN_POINT('Ctrl Pts',(74.4416140848743,-2.94891377268036,0.));
#53440=CARTESIAN_POINT('Ctrl Pts',(74.4416140848743,-2.94891377268036,4.));
#53441=CARTESIAN_POINT('Ctrl Pts',(74.4416140848744,-2.94891377268042,8.));
#53442=CARTESIAN_POINT('Ctrl Pts',(74.4416140848744,-2.94891377268042,12.));
#53443=CARTESIAN_POINT('',(74.1624659714955,-2.48034921844903,0.));
#53444=CARTESIAN_POINT('',(74.4416140848739,-2.94891377268035,0.));
#53445=CARTESIAN_POINT('Ctrl Pts',(74.1624659714955,-2.48034921844903,0.));
#53446=CARTESIAN_POINT('Ctrl Pts',(74.2610905805699,-2.52879860312842,0.));
#53447=CARTESIAN_POINT('Ctrl Pts',(74.3428145790912,-2.61085254571364,0.));
#53448=CARTESIAN_POINT('Ctrl Pts',(74.391151343622,-2.70942211516261,0.));
#53449=CARTESIAN_POINT('Ctrl Pts',(74.42740391702,-2.78334929224933,0.));
#53450=CARTESIAN_POINT('Ctrl Pts',(74.4448761712984,-2.86656650944691,0.));
#53451=CARTESIAN_POINT('Ctrl Pts',(74.4416140848743,-2.94891377268036,0.));
#53452=CARTESIAN_POINT('',(74.4416140848739,-2.9489137726804,12.));
#53453=CARTESIAN_POINT('Ctrl Pts',(74.4416140848743,-2.94891377268036,0.));
#53454=CARTESIAN_POINT('Ctrl Pts',(74.4416140848743,-2.94891377268036,4.));
#53455=CARTESIAN_POINT('Ctrl Pts',(74.4416140848744,-2.94891377268042,8.));
#53456=CARTESIAN_POINT('Ctrl Pts',(74.4416140848744,-2.94891377268042,12.));
#53457=CARTESIAN_POINT('',(74.1624659714955,-2.48034921844902,12.));
#53458=CARTESIAN_POINT('Ctrl Pts',(74.4416140848744,-2.94891377268042,12.));
#53459=CARTESIAN_POINT('Ctrl Pts',(74.4448761712985,-2.86656650944694,12.));
#53460=CARTESIAN_POINT('Ctrl Pts',(74.4274039170202,-2.78334929224934,12.));
#53461=CARTESIAN_POINT('Ctrl Pts',(74.3911513436221,-2.7094221151626,12.));
#53462=CARTESIAN_POINT('Ctrl Pts',(74.3428145790913,-2.61085254571361,12.));
#53463=CARTESIAN_POINT('Ctrl Pts',(74.2610905805699,-2.52879860312839,12.));
#53464=CARTESIAN_POINT('Ctrl Pts',(74.1624659714955,-2.48034921844902,12.));
#53465=CARTESIAN_POINT('Ctrl Pts',(74.1624659714955,-2.48034921844902,12.));
#53466=CARTESIAN_POINT('Ctrl Pts',(74.1624659714955,-2.48034921844902,8.));
#53467=CARTESIAN_POINT('Ctrl Pts',(74.1624659714955,-2.48034921844903,4.));
#53468=CARTESIAN_POINT('Ctrl Pts',(74.1624659714955,-2.48034921844903,0.));
#53469=CARTESIAN_POINT('Origin',(3.74491326291036E-10,-1.62512913209676E-11,
0.));
#53470=CARTESIAN_POINT('Origin',(3.74491326291036E-10,-1.62512913209676E-11,
12.));
#53471=CARTESIAN_POINT('Origin',(3.74491326291036E-10,-1.62512913209676E-11,
0.));
#53472=CARTESIAN_POINT('Ctrl Pts',(73.8227522002498,-10.0225374821205,0.));
#53473=CARTESIAN_POINT('Ctrl Pts',(73.8227522002498,-10.0225374821205,4.));
#53474=CARTESIAN_POINT('Ctrl Pts',(73.8227522002498,-10.0225374821205,8.));
#53475=CARTESIAN_POINT('Ctrl Pts',(73.8227522002498,-10.0225374821205,12.));
#53476=CARTESIAN_POINT('Ctrl Pts',(73.8079696346554,-10.1314210536415,0.));
#53477=CARTESIAN_POINT('Ctrl Pts',(73.8079696346554,-10.1314210536415,4.));
#53478=CARTESIAN_POINT('Ctrl Pts',(73.8079696346554,-10.1314210536415,8.00000000000001));
#53479=CARTESIAN_POINT('Ctrl Pts',(73.8079696346554,-10.1314210536415,12.));
#53480=CARTESIAN_POINT('Ctrl Pts',(73.7169567649191,-10.3125002643518,0.));
#53481=CARTESIAN_POINT('Ctrl Pts',(73.7169567649191,-10.3125002643518,4.));
#53482=CARTESIAN_POINT('Ctrl Pts',(73.7169567649191,-10.3125002643518,7.99999999999999));
#53483=CARTESIAN_POINT('Ctrl Pts',(73.7169567649191,-10.3125002643518,12.));
#53484=CARTESIAN_POINT('Ctrl Pts',(73.5456341632196,-10.4125694172277,0.));
#53485=CARTESIAN_POINT('Ctrl Pts',(73.5456341632196,-10.4125694172277,4.));
#53486=CARTESIAN_POINT('Ctrl Pts',(73.5456341632196,-10.4125694172277,8.00000000000001));
#53487=CARTESIAN_POINT('Ctrl Pts',(73.5456341632196,-10.4125694172277,12.));
#53488=CARTESIAN_POINT('Ctrl Pts',(73.4664795929519,-10.435509926739,0.));
#53489=CARTESIAN_POINT('Ctrl Pts',(73.4664795929519,-10.435509926739,4.));
#53490=CARTESIAN_POINT('Ctrl Pts',(73.4664795929519,-10.435509926739,8.));
#53491=CARTESIAN_POINT('Ctrl Pts',(73.4664795929519,-10.435509926739,12.));
#53492=CARTESIAN_POINT('',(73.8227522002498,-10.0225374821205,0.));
#53493=CARTESIAN_POINT('',(73.4664795929519,-10.4355099267391,0.));
#53494=CARTESIAN_POINT('Ctrl Pts',(73.8227522002498,-10.0225374821205,0.));
#53495=CARTESIAN_POINT('Ctrl Pts',(73.8079696346554,-10.1314210536415,0.));
#53496=CARTESIAN_POINT('Ctrl Pts',(73.7559622805204,-10.2348948883331,0.));
#53497=CARTESIAN_POINT('Ctrl Pts',(73.6777313404382,-10.311916459242,0.));
#53498=CARTESIAN_POINT('Ctrl Pts',(73.6190581353765,-10.3696826374238,0.));
#53499=CARTESIAN_POINT('Ctrl Pts',(73.5456341632196,-10.4125694172277,0.));
#53500=CARTESIAN_POINT('Ctrl Pts',(73.4664795929519,-10.435509926739,0.));
#53501=CARTESIAN_POINT('',(73.4664795929519,-10.4355099267391,12.));
#53502=CARTESIAN_POINT('Ctrl Pts',(73.4664795929519,-10.435509926739,0.));
#53503=CARTESIAN_POINT('Ctrl Pts',(73.4664795929519,-10.435509926739,4.));
#53504=CARTESIAN_POINT('Ctrl Pts',(73.4664795929519,-10.435509926739,8.));
#53505=CARTESIAN_POINT('Ctrl Pts',(73.4664795929519,-10.435509926739,12.));
#53506=CARTESIAN_POINT('',(73.8227522002498,-10.0225374821205,12.));
#53507=CARTESIAN_POINT('Ctrl Pts',(73.4664795929519,-10.435509926739,12.));
#53508=CARTESIAN_POINT('Ctrl Pts',(73.5456341632196,-10.4125694172277,12.));
#53509=CARTESIAN_POINT('Ctrl Pts',(73.6190581353765,-10.3696826374237,12.));
#53510=CARTESIAN_POINT('Ctrl Pts',(73.6777313404382,-10.311916459242,12.));
#53511=CARTESIAN_POINT('Ctrl Pts',(73.7559622805204,-10.2348948883331,12.));
#53512=CARTESIAN_POINT('Ctrl Pts',(73.8079696346554,-10.1314210536415,12.));
#53513=CARTESIAN_POINT('Ctrl Pts',(73.8227522002498,-10.0225374821205,12.));
#53514=CARTESIAN_POINT('Ctrl Pts',(73.8227522002498,-10.0225374821205,12.));
#53515=CARTESIAN_POINT('Ctrl Pts',(73.8227522002498,-10.0225374821205,8.));
#53516=CARTESIAN_POINT('Ctrl Pts',(73.8227522002498,-10.0225374821205,4.));
#53517=CARTESIAN_POINT('Ctrl Pts',(73.8227522002498,-10.0225374821205,0.));
#53518=CARTESIAN_POINT('Ctrl Pts',(69.079679653846,-11.3136138754165,0.));
#53519=CARTESIAN_POINT('Ctrl Pts',(69.079679653846,-11.3136138754165,12.));
#53520=CARTESIAN_POINT('Ctrl Pts',(69.0835449954396,-11.3132375200165,0.));
#53521=CARTESIAN_POINT('Ctrl Pts',(69.0835449954396,-11.3132375200165,12.));
#53522=CARTESIAN_POINT('Ctrl Pts',(69.0912808656811,-11.3124821678798,0.));
#53523=CARTESIAN_POINT('Ctrl Pts',(69.0912808656811,-11.3124821678798,12.));
#53524=CARTESIAN_POINT('Ctrl Pts',(69.1029002322118,-11.3113412156661,0.));
#53525=CARTESIAN_POINT('Ctrl Pts',(69.1029002322118,-11.3113412156661,12.));
#53526=CARTESIAN_POINT('Ctrl Pts',(69.118423844466,-11.3098040973713,0.));
#53527=CARTESIAN_POINT('Ctrl Pts',(69.118423844466,-11.3098040973713,12.));
#53528=CARTESIAN_POINT('Ctrl Pts',(69.1378802251711,-11.3078562764384,0.));
#53529=CARTESIAN_POINT('Ctrl Pts',(69.1378802251711,-11.3078562764384,12.));
#53530=CARTESIAN_POINT('Ctrl Pts',(69.1573884361,-11.3058820128307,0.));
#53531=CARTESIAN_POINT('Ctrl Pts',(69.1573884361,-11.3058820128307,12.));
#53532=CARTESIAN_POINT('Ctrl Pts',(69.1769483991721,-11.3038812726292,0.));
#53533=CARTESIAN_POINT('Ctrl Pts',(69.1769483991721,-11.3038812726292,12.));
#53534=CARTESIAN_POINT('Ctrl Pts',(69.1965599718914,-11.3018540025638,0.));
#53535=CARTESIAN_POINT('Ctrl Pts',(69.1965599718914,-11.3018540025638,12.));
#53536=CARTESIAN_POINT('Ctrl Pts',(69.2162229488531,-11.2998001310964,0.));
#53537=CARTESIAN_POINT('Ctrl Pts',(69.2162229488531,-11.2998001310964,12.));
#53538=CARTESIAN_POINT('Ctrl Pts',(69.2359370894907,-11.2977195764852,0.));
#53539=CARTESIAN_POINT('Ctrl Pts',(69.2359370894907,-11.2977195764852,12.));
#53540=CARTESIAN_POINT('Ctrl Pts',(69.255702139335,-11.2956122531375,0.));
#53541=CARTESIAN_POINT('Ctrl Pts',(69.255702139335,-11.2956122531375,12.));
#53542=CARTESIAN_POINT('Ctrl Pts',(69.275517853148,-11.2934780784351,0.));
#53543=CARTESIAN_POINT('Ctrl Pts',(69.275517853148,-11.2934780784351,12.));
#53544=CARTESIAN_POINT('Ctrl Pts',(69.295384019272,-11.2913169799628,0.));
#53545=CARTESIAN_POINT('Ctrl Pts',(69.295384019272,-11.2913169799628,12.));
#53546=CARTESIAN_POINT('Ctrl Pts',(69.3153004517783,-11.2891288931517,0.));
#53547=CARTESIAN_POINT('Ctrl Pts',(69.3153004517783,-11.2891288931517,12.));
#53548=CARTESIAN_POINT('Ctrl Pts',(69.3352669789587,-11.2869137578459,0.));
#53549=CARTESIAN_POINT('Ctrl Pts',(69.3352669789587,-11.2869137578459,12.));
#53550=CARTESIAN_POINT('Ctrl Pts',(69.3552834337784,-11.2846715154524,0.));
#53551=CARTESIAN_POINT('Ctrl Pts',(69.3552834337784,-11.2846715154524,12.));
#53552=CARTESIAN_POINT('Ctrl Pts',(69.3753496420039,-11.2824021054045,0.));
#53553=CARTESIAN_POINT('Ctrl Pts',(69.3753496420039,-11.2824021054045,12.));
#53554=CARTESIAN_POINT('Ctrl Pts',(69.3954654162281,-11.2801054633816,0.));
#53555=CARTESIAN_POINT('Ctrl Pts',(69.3954654162281,-11.2801054633816,12.));
#53556=CARTESIAN_POINT('Ctrl Pts',(69.4156305620593,-11.2777815231469,0.));
#53557=CARTESIAN_POINT('Ctrl Pts',(69.4156305620593,-11.2777815231469,12.));
#53558=CARTESIAN_POINT('Ctrl Pts',(69.4358448819967,-11.2754302177021,0.));
#53559=CARTESIAN_POINT('Ctrl Pts',(69.4358448819967,-11.2754302177021,12.));
#53560=CARTESIAN_POINT('Ctrl Pts',(69.456108179879,-11.2730514806139,0.));
#53561=CARTESIAN_POINT('Ctrl Pts',(69.456108179879,-11.2730514806139,12.));
#53562=CARTESIAN_POINT('Ctrl Pts',(69.4764202659397,-11.270645247528,0.));
#53563=CARTESIAN_POINT('Ctrl Pts',(69.4764202659397,-11.270645247528,12.));
#53564=CARTESIAN_POINT('Ctrl Pts',(69.4967809565929,-11.2682114561008,0.));
#53565=CARTESIAN_POINT('Ctrl Pts',(69.4967809565929,-11.2682114561008,12.));
#53566=CARTESIAN_POINT('Ctrl Pts',(69.5171900720158,-11.2657500452716,0.));
#53567=CARTESIAN_POINT('Ctrl Pts',(69.5171900720158,-11.2657500452716,12.));
#53568=CARTESIAN_POINT('Ctrl Pts',(69.5376474344771,-11.263260954763,0.));
#53569=CARTESIAN_POINT('Ctrl Pts',(69.5376474344771,-11.263260954763,12.));
#53570=CARTESIAN_POINT('Ctrl Pts',(69.5581528662877,-11.2607441244703,0.));
#53571=CARTESIAN_POINT('Ctrl Pts',(69.5581528662877,-11.2607441244703,12.));
#53572=CARTESIAN_POINT('Ctrl Pts',(69.5787061880857,-11.2581994939541,0.));
#53573=CARTESIAN_POINT('Ctrl Pts',(69.5787061880857,-11.2581994939541,12.));
#53574=CARTESIAN_POINT('Ctrl Pts',(69.599307219739,-11.2556270027016,0.));
#53575=CARTESIAN_POINT('Ctrl Pts',(69.599307219739,-11.2556270027016,12.));
#53576=CARTESIAN_POINT('Ctrl Pts',(69.6199557811245,-11.2530265903557,0.));
#53577=CARTESIAN_POINT('Ctrl Pts',(69.6199557811245,-11.2530265903557,12.));
#53578=CARTESIAN_POINT('Ctrl Pts',(69.6406516928891,-11.2503981969412,0.));
#53579=CARTESIAN_POINT('Ctrl Pts',(69.6406516928891,-11.2503981969412,12.));
#53580=CARTESIAN_POINT('Ctrl Pts',(69.6613947773534,-11.2477417631386,0.));
#53581=CARTESIAN_POINT('Ctrl Pts',(69.6613947773534,-11.2477417631386,12.));
#53582=CARTESIAN_POINT('Ctrl Pts',(69.6821848588457,-11.2450572303841,0.));
#53583=CARTESIAN_POINT('Ctrl Pts',(69.6821848588457,-11.2450572303841,12.));
#53584=CARTESIAN_POINT('Ctrl Pts',(69.7030217632164,-11.2423445407166,0.));
#53585=CARTESIAN_POINT('Ctrl Pts',(69.7030217632164,-11.2423445407166,12.));
#53586=CARTESIAN_POINT('Ctrl Pts',(69.7239053175356,-11.239603636686,0.));
#53587=CARTESIAN_POINT('Ctrl Pts',(69.7239053175356,-11.239603636686,12.));
#53588=CARTESIAN_POINT('Ctrl Pts',(69.7448353497408,-11.2368344612472,0.));
#53589=CARTESIAN_POINT('Ctrl Pts',(69.7448353497408,-11.2368344612472,12.));
#53590=CARTESIAN_POINT('Ctrl Pts',(69.7658116882324,-11.2340369576456,0.));
#53591=CARTESIAN_POINT('Ctrl Pts',(69.7658116882324,-11.2340369576456,12.));
#53592=CARTESIAN_POINT('Ctrl Pts',(69.7868341618954,-11.2312110694187,0.));
#53593=CARTESIAN_POINT('Ctrl Pts',(69.7868341618954,-11.2312110694187,12.));
#53594=CARTESIAN_POINT('Ctrl Pts',(69.8079026002768,-11.2283567404437,0.));
#53595=CARTESIAN_POINT('Ctrl Pts',(69.8079026002768,-11.2283567404437,12.));
#53596=CARTESIAN_POINT('Ctrl Pts',(69.8290168337076,-11.225473914972,0.));
#53597=CARTESIAN_POINT('Ctrl Pts',(69.8290168337076,-11.225473914972,12.));
#53598=CARTESIAN_POINT('Ctrl Pts',(69.8501766934428,-11.2225625376736,0.));
#53599=CARTESIAN_POINT('Ctrl Pts',(69.8501766934428,-11.2225625376736,12.));
#53600=CARTESIAN_POINT('Ctrl Pts',(69.871382011789,-11.219622553679,0.));
#53601=CARTESIAN_POINT('Ctrl Pts',(69.871382011789,-11.219622553679,12.));
#53602=CARTESIAN_POINT('Ctrl Pts',(69.8926326220385,-11.2166539085523,0.));
#53603=CARTESIAN_POINT('Ctrl Pts',(69.8926326220385,-11.2166539085523,12.));
#53604=CARTESIAN_POINT('Ctrl Pts',(69.9139283584022,-11.2136565482678,0.));
#53605=CARTESIAN_POINT('Ctrl Pts',(69.9139283584022,-11.2136565482678,12.));
#53606=CARTESIAN_POINT('Ctrl Pts',(69.9352690559405,-11.2106304191882,0.));
#53607=CARTESIAN_POINT('Ctrl Pts',(69.9352690559405,-11.2106304191882,12.));
#53608=CARTESIAN_POINT('Ctrl Pts',(69.9566545504837,-11.2075754680449,0.));
#53609=CARTESIAN_POINT('Ctrl Pts',(69.9566545504837,-11.2075754680449,12.));
#53610=CARTESIAN_POINT('Ctrl Pts',(69.97808467858,-11.2044916419244,0.));
#53611=CARTESIAN_POINT('Ctrl Pts',(69.97808467858,-11.2044916419244,12.));
#53612=CARTESIAN_POINT('Ctrl Pts',(69.9995592775343,-11.2013788882714,0.));
#53613=CARTESIAN_POINT('Ctrl Pts',(69.9995592775343,-11.2013788882714,12.));
#53614=CARTESIAN_POINT('Ctrl Pts',(70.0210781854243,-11.1982371548919,0.));
#53615=CARTESIAN_POINT('Ctrl Pts',(70.0210781854243,-11.1982371548919,12.));
#53616=CARTESIAN_POINT('Ctrl Pts',(70.0426412411185,-11.1950663899576,0.));
#53617=CARTESIAN_POINT('Ctrl Pts',(70.0426412411185,-11.1950663899576,12.));
#53618=CARTESIAN_POINT('Ctrl Pts',(70.0642482842928,-11.1918665420166,0.));
#53619=CARTESIAN_POINT('Ctrl Pts',(70.0642482842928,-11.1918665420166,12.));
#53620=CARTESIAN_POINT('Ctrl Pts',(70.0858991554283,-11.1886375599914,0.));
#53621=CARTESIAN_POINT('Ctrl Pts',(70.0858991554283,-11.1886375599914,12.));
#53622=CARTESIAN_POINT('Ctrl Pts',(70.1075936957968,-11.185379393167,0.));
#53623=CARTESIAN_POINT('Ctrl Pts',(70.1075936957968,-11.185379393167,12.));
#53624=CARTESIAN_POINT('Ctrl Pts',(70.1293317474432,-11.1820919911846,0.));
#53625=CARTESIAN_POINT('Ctrl Pts',(70.1293317474432,-11.1820919911846,12.));
#53626=CARTESIAN_POINT('Ctrl Pts',(70.1511131531674,-11.1787753040363,0.));
#53627=CARTESIAN_POINT('Ctrl Pts',(70.1511131531674,-11.1787753040363,12.));
#53628=CARTESIAN_POINT('Ctrl Pts',(70.1729377564956,-11.1754292820631,0.));
#53629=CARTESIAN_POINT('Ctrl Pts',(70.1729377564956,-11.1754292820631,12.));
#53630=CARTESIAN_POINT('Ctrl Pts',(70.1948054016817,-11.1720538759499,0.));
#53631=CARTESIAN_POINT('Ctrl Pts',(70.1948054016817,-11.1720538759499,12.));
#53632=CARTESIAN_POINT('Ctrl Pts',(70.2167159337095,-11.168649036721,0.));
#53633=CARTESIAN_POINT('Ctrl Pts',(70.2167159337095,-11.168649036721,12.));
#53634=CARTESIAN_POINT('Ctrl Pts',(70.2386691982902,-11.1652147157383,0.));
#53635=CARTESIAN_POINT('Ctrl Pts',(70.2386691982902,-11.1652147157383,12.));
#53636=CARTESIAN_POINT('Ctrl Pts',(70.2606650418589,-11.1617508647017,0.));
#53637=CARTESIAN_POINT('Ctrl Pts',(70.2606650418589,-11.1617508647017,12.));
#53638=CARTESIAN_POINT('Ctrl Pts',(70.2827033115662,-11.1582574356522,0.));
#53639=CARTESIAN_POINT('Ctrl Pts',(70.2827033115662,-11.1582574356522,12.));
#53640=CARTESIAN_POINT('Ctrl Pts',(70.3047838552758,-11.1547343809647,0.));
#53641=CARTESIAN_POINT('Ctrl Pts',(70.3047838552758,-11.1547343809647,12.));
#53642=CARTESIAN_POINT('Ctrl Pts',(70.3269065215591,-11.1511816533422,0.));
#53643=CARTESIAN_POINT('Ctrl Pts',(70.3269065215591,-11.1511816533422,12.));
#53644=CARTESIAN_POINT('Ctrl Pts',(70.3490711596882,-11.1475992058124,0.));
#53645=CARTESIAN_POINT('Ctrl Pts',(70.3490711596882,-11.1475992058124,12.));
#53646=CARTESIAN_POINT('Ctrl Pts',(70.3712776196216,-11.1439869917269,0.));
#53647=CARTESIAN_POINT('Ctrl Pts',(70.3712776196216,-11.1439869917269,12.));
#53648=CARTESIAN_POINT('Ctrl Pts',(70.3935257519945,-11.1403449647622,0.));
#53649=CARTESIAN_POINT('Ctrl Pts',(70.3935257519945,-11.1403449647622,12.));
#53650=CARTESIAN_POINT('Ctrl Pts',(70.415815408119,-11.1366730789122,0.));
#53651=CARTESIAN_POINT('Ctrl Pts',(70.415815408119,-11.1366730789122,12.));
#53652=CARTESIAN_POINT('Ctrl Pts',(70.438146439981,-11.1329712884845,0.));
#53653=CARTESIAN_POINT('Ctrl Pts',(70.438146439981,-11.1329712884845,12.));
#53654=CARTESIAN_POINT('Ctrl Pts',(70.4605187002356,-11.1292395480975,0.));
#53655=CARTESIAN_POINT('Ctrl Pts',(70.4605187002356,-11.1292395480975,12.));
#53656=CARTESIAN_POINT('Ctrl Pts',(70.4829320421973,-11.1254778126824,0.));
#53657=CARTESIAN_POINT('Ctrl Pts',(70.4829320421973,-11.1254778126824,12.));
#53658=CARTESIAN_POINT('Ctrl Pts',(70.5053863198306,-11.121686037483,0.));
#53659=CARTESIAN_POINT('Ctrl Pts',(70.5053863198306,-11.121686037483,12.));
#53660=CARTESIAN_POINT('Ctrl Pts',(70.5278813877519,-11.117864178048,0.));
#53661=CARTESIAN_POINT('Ctrl Pts',(70.5278813877519,-11.117864178048,12.));
#53662=CARTESIAN_POINT('Ctrl Pts',(70.5504171012247,-11.1140121902274,0.));
#53663=CARTESIAN_POINT('Ctrl Pts',(70.5504171012247,-11.1140121902274,12.));
#53664=CARTESIAN_POINT('Ctrl Pts',(70.5729933161538,-11.11013003017,0.));
#53665=CARTESIAN_POINT('Ctrl Pts',(70.5729933161538,-11.11013003017,12.));
#53666=CARTESIAN_POINT('Ctrl Pts',(70.5956098890744,-11.1062176543257,0.));
#53667=CARTESIAN_POINT('Ctrl Pts',(70.5956098890744,-11.1062176543257,12.));
#53668=CARTESIAN_POINT('Ctrl Pts',(70.6182666771441,-11.1022750194439,0.));
#53669=CARTESIAN_POINT('Ctrl Pts',(70.6182666771441,-11.1022750194439,12.));
#53670=CARTESIAN_POINT('Ctrl Pts',(70.6409635381446,-11.0983020825662,0.));
#53671=CARTESIAN_POINT('Ctrl Pts',(70.6409635381446,-11.0983020825662,12.));
#53672=CARTESIAN_POINT('Ctrl Pts',(70.6637003304768,-11.0942988010231,0.));
#53673=CARTESIAN_POINT('Ctrl Pts',(70.6637003304768,-11.0942988010231,12.));
#53674=CARTESIAN_POINT('Ctrl Pts',(70.686476913156,-11.0902651324325,0.));
#53675=CARTESIAN_POINT('Ctrl Pts',(70.686476913156,-11.0902651324325,12.));
#53676=CARTESIAN_POINT('Ctrl Pts',(70.7092931457996,-11.0862010347022,0.));
#53677=CARTESIAN_POINT('Ctrl Pts',(70.7092931457996,-11.0862010347022,12.));
#53678=CARTESIAN_POINT('Ctrl Pts',(70.7321488886229,-11.0821064660276,0.));
#53679=CARTESIAN_POINT('Ctrl Pts',(70.7321488886229,-11.0821064660276,12.));
#53680=CARTESIAN_POINT('Ctrl Pts',(70.7550440024422,-11.0779813848851,0.));
#53681=CARTESIAN_POINT('Ctrl Pts',(70.7550440024422,-11.0779813848851,12.));
#53682=CARTESIAN_POINT('Ctrl Pts',(70.7779783486689,-11.0738257500292,0.));
#53683=CARTESIAN_POINT('Ctrl Pts',(70.7779783486689,-11.0738257500292,12.));
#53684=CARTESIAN_POINT('Ctrl Pts',(70.8009517893042,-11.0696395204908,0.));
#53685=CARTESIAN_POINT('Ctrl Pts',(70.8009517893042,-11.0696395204908,12.));
#53686=CARTESIAN_POINT('Ctrl Pts',(70.8239641869266,-11.0654226555798,0.));
#53687=CARTESIAN_POINT('Ctrl Pts',(70.8239641869266,-11.0654226555798,12.));
#53688=CARTESIAN_POINT('Ctrl Pts',(70.847015404688,-11.061175114883,0.));
#53689=CARTESIAN_POINT('Ctrl Pts',(70.847015404688,-11.061175114883,12.));
#53690=CARTESIAN_POINT('Ctrl Pts',(70.8701053063158,-11.0568968582566,0.));
#53691=CARTESIAN_POINT('Ctrl Pts',(70.8701053063158,-11.0568968582566,12.));
#53692=CARTESIAN_POINT('Ctrl Pts',(70.8932337561078,-11.0525878458242,0.));
#53693=CARTESIAN_POINT('Ctrl Pts',(70.8932337561078,-11.0525878458242,12.));
#53694=CARTESIAN_POINT('Ctrl Pts',(70.9164006189283,-11.0482480379752,0.));
#53695=CARTESIAN_POINT('Ctrl Pts',(70.9164006189283,-11.0482480379752,12.));
#53696=CARTESIAN_POINT('Ctrl Pts',(70.9396057601953,-11.0438773953686,0.));
#53697=CARTESIAN_POINT('Ctrl Pts',(70.9396057601953,-11.0438773953686,12.));
#53698=CARTESIAN_POINT('Ctrl Pts',(70.9628490458779,-11.039475878929,0.));
#53699=CARTESIAN_POINT('Ctrl Pts',(70.9628490458779,-11.039475878929,12.));
#53700=CARTESIAN_POINT('Ctrl Pts',(70.9861303424989,-11.0350434498408,0.));
#53701=CARTESIAN_POINT('Ctrl Pts',(70.9861303424989,-11.0350434498408,12.));
#53702=CARTESIAN_POINT('Ctrl Pts',(71.0094495171295,-11.0305800695457,0.));
#53703=CARTESIAN_POINT('Ctrl Pts',(71.0094495171295,-11.0305800695457,12.));
#53704=CARTESIAN_POINT('Ctrl Pts',(71.0328064373849,-11.0260856997414,0.));
#53705=CARTESIAN_POINT('Ctrl Pts',(71.0328064373849,-11.0260856997414,12.));
#53706=CARTESIAN_POINT('Ctrl Pts',(71.0562009714125,-11.0215603023854,0.));
#53707=CARTESIAN_POINT('Ctrl Pts',(71.0562009714125,-11.0215603023854,12.));
#53708=CARTESIAN_POINT('Ctrl Pts',(71.0796329878896,-11.0170038396913,0.));
#53709=CARTESIAN_POINT('Ctrl Pts',(71.0796329878896,-11.0170038396913,12.));
#53710=CARTESIAN_POINT('Ctrl Pts',(71.1031023560243,-11.0124162741223,0.));
#53711=CARTESIAN_POINT('Ctrl Pts',(71.1031023560243,-11.0124162741223,12.));
#53712=CARTESIAN_POINT('Ctrl Pts',(71.1266089455517,-11.0077975683895,0.));
#53713=CARTESIAN_POINT('Ctrl Pts',(71.1266089455517,-11.0077975683895,12.));
#53714=CARTESIAN_POINT('Ctrl Pts',(71.1501526267288,-11.0031476854503,0.));
#53715=CARTESIAN_POINT('Ctrl Pts',(71.1501526267288,-11.0031476854503,12.));
#53716=CARTESIAN_POINT('Ctrl Pts',(71.1737332703248,-10.9984665885127,0.));
#53717=CARTESIAN_POINT('Ctrl Pts',(71.1737332703248,-10.9984665885127,12.));
#53718=CARTESIAN_POINT('Ctrl Pts',(71.1973507476188,-10.993754241032,0.));
#53719=CARTESIAN_POINT('Ctrl Pts',(71.1973507476188,-10.993754241032,12.));
#53720=CARTESIAN_POINT('Ctrl Pts',(71.221004930401,-10.9890106067038,0.));
#53721=CARTESIAN_POINT('Ctrl Pts',(71.221004930401,-10.9890106067038,12.));
#53722=CARTESIAN_POINT('Ctrl Pts',(71.2446956909685,-10.9842356494627,0.));
#53723=CARTESIAN_POINT('Ctrl Pts',(71.2446956909685,-10.9842356494627,12.));
#53724=CARTESIAN_POINT('Ctrl Pts',(71.2684229021209,-10.9794293334806,0.));
#53725=CARTESIAN_POINT('Ctrl Pts',(71.2684229021209,-10.9794293334806,12.));
#53726=CARTESIAN_POINT('Ctrl Pts',(71.2921864371499,-10.9745916231711,0.));
#53727=CARTESIAN_POINT('Ctrl Pts',(71.2921864371499,-10.9745916231711,12.));
#53728=CARTESIAN_POINT('Ctrl Pts',(71.3159861698368,-10.9697224831862,0.));
#53729=CARTESIAN_POINT('Ctrl Pts',(71.3159861698368,-10.9697224831862,12.));
#53730=CARTESIAN_POINT('Ctrl Pts',(71.3398219744547,-10.96482187841,0.));
#53731=CARTESIAN_POINT('Ctrl Pts',(71.3398219744547,-10.96482187841,12.));
#53732=CARTESIAN_POINT('Ctrl Pts',(71.3636937257651,-10.9598897739565,0.));
#53733=CARTESIAN_POINT('Ctrl Pts',(71.3636937257651,-10.9598897739565,12.));
#53734=CARTESIAN_POINT('Ctrl Pts',(71.3876012990135,-10.954926135169,0.));
#53735=CARTESIAN_POINT('Ctrl Pts',(71.3876012990135,-10.954926135169,12.));
#53736=CARTESIAN_POINT('Ctrl Pts',(71.411544569919,-10.9499309276235,0.));
#53737=CARTESIAN_POINT('Ctrl Pts',(71.411544569919,-10.9499309276235,12.));
#53738=CARTESIAN_POINT('Ctrl Pts',(71.4355234146718,-10.9449041171269,0.));
#53739=CARTESIAN_POINT('Ctrl Pts',(71.4355234146718,-10.9449041171269,12.));
#53740=CARTESIAN_POINT('Ctrl Pts',(71.4595377099352,-10.9398456697095,0.));
#53741=CARTESIAN_POINT('Ctrl Pts',(71.4595377099352,-10.9398456697095,12.));
#53742=CARTESIAN_POINT('Ctrl Pts',(71.4835873328425,-10.9347555516236,0.));
#53743=CARTESIAN_POINT('Ctrl Pts',(71.4835873328425,-10.9347555516236,12.));
#53744=CARTESIAN_POINT('Ctrl Pts',(71.5076721609936,-10.9296337293425,0.));
#53745=CARTESIAN_POINT('Ctrl Pts',(71.5076721609936,-10.9296337293425,12.));
#53746=CARTESIAN_POINT('Ctrl Pts',(71.5317920724453,-10.9244801695642,0.));
#53747=CARTESIAN_POINT('Ctrl Pts',(71.5317920724453,-10.9244801695642,12.));
#53748=CARTESIAN_POINT('Ctrl Pts',(71.5559469457082,-10.9192948392099,0.));
#53749=CARTESIAN_POINT('Ctrl Pts',(71.5559469457082,-10.9192948392099,12.));
#53750=CARTESIAN_POINT('Ctrl Pts',(71.5801366597479,-10.9140777054169,0.));
#53751=CARTESIAN_POINT('Ctrl Pts',(71.5801366597479,-10.9140777054169,12.));
#53752=CARTESIAN_POINT('Ctrl Pts',(71.604361093983,-10.9088287355364,0.));
#53753=CARTESIAN_POINT('Ctrl Pts',(71.604361093983,-10.9088287355364,12.));
#53754=CARTESIAN_POINT('Ctrl Pts',(71.6286201282815,-10.9035478971329,0.));
#53755=CARTESIAN_POINT('Ctrl Pts',(71.6286201282815,-10.9035478971329,12.));
#53756=CARTESIAN_POINT('Ctrl Pts',(71.6529136429515,-10.8982351579872,0.));
#53757=CARTESIAN_POINT('Ctrl Pts',(71.6529136429515,-10.8982351579872,12.));
#53758=CARTESIAN_POINT('Ctrl Pts',(71.6772415187382,-10.8928904860967,0.));
#53759=CARTESIAN_POINT('Ctrl Pts',(71.6772415187382,-10.8928904860967,12.));
#53760=CARTESIAN_POINT('Ctrl Pts',(71.7016036368254,-10.8875138496674,0.));
#53761=CARTESIAN_POINT('Ctrl Pts',(71.7016036368254,-10.8875138496674,12.));
#53762=CARTESIAN_POINT('Ctrl Pts',(71.7259998788337,-10.8821052171122,0.));
#53763=CARTESIAN_POINT('Ctrl Pts',(71.7259998788337,-10.8821052171122,12.));
#53764=CARTESIAN_POINT('Ctrl Pts',(71.7504301268177,-10.8766645570496,0.));
#53765=CARTESIAN_POINT('Ctrl Pts',(71.7504301268177,-10.8766645570496,12.));
#53766=CARTESIAN_POINT('Ctrl Pts',(71.7748942632578,-10.8711918383071,0.));
#53767=CARTESIAN_POINT('Ctrl Pts',(71.7748942632578,-10.8711918383071,12.));
#53768=CARTESIAN_POINT('Ctrl Pts',(71.7993921710546,-10.8656870299218,0.));
#53769=CARTESIAN_POINT('Ctrl Pts',(71.7993921710546,-10.8656870299218,12.));
#53770=CARTESIAN_POINT('Ctrl Pts',(71.8239237335318,-10.860150101133,0.));
#53771=CARTESIAN_POINT('Ctrl Pts',(71.8239237335318,-10.860150101133,12.));
#53772=CARTESIAN_POINT('Ctrl Pts',(71.8484888344335,-10.8545810213799,0.));
#53773=CARTESIAN_POINT('Ctrl Pts',(71.8484888344335,-10.8545810213799,12.));
#53774=CARTESIAN_POINT('Ctrl Pts',(71.8730873579226,-10.8489797602998,0.));
#53775=CARTESIAN_POINT('Ctrl Pts',(71.8730873579226,-10.8489797602998,12.));
#53776=CARTESIAN_POINT('Ctrl Pts',(71.8977191885726,-10.8433462877312,0.));
#53777=CARTESIAN_POINT('Ctrl Pts',(71.8977191885726,-10.8433462877312,12.));
#53778=CARTESIAN_POINT('Ctrl Pts',(71.9223842113622,-10.8376805737158,0.));
#53779=CARTESIAN_POINT('Ctrl Pts',(71.9223842113622,-10.8376805737158,12.));
#53780=CARTESIAN_POINT('Ctrl Pts',(71.9470823116777,-10.8319825884917,0.));
#53781=CARTESIAN_POINT('Ctrl Pts',(71.9470823116777,-10.8319825884917,12.));
#53782=CARTESIAN_POINT('Ctrl Pts',(71.971813375312,-10.8262523024897,0.));
#53783=CARTESIAN_POINT('Ctrl Pts',(71.971813375312,-10.8262523024897,12.));
#53784=CARTESIAN_POINT('Ctrl Pts',(71.996577288462,-10.8204896863328,0.));
#53785=CARTESIAN_POINT('Ctrl Pts',(71.996577288462,-10.8204896863328,12.));
#53786=CARTESIAN_POINT('Ctrl Pts',(72.0213739377231,-10.8146947108376,0.));
#53787=CARTESIAN_POINT('Ctrl Pts',(72.0213739377231,-10.8146947108376,12.));
#53788=CARTESIAN_POINT('Ctrl Pts',(72.0462032100828,-10.8088673470187,0.));
#53789=CARTESIAN_POINT('Ctrl Pts',(72.0462032100828,-10.8088673470187,12.));
#53790=CARTESIAN_POINT('Ctrl Pts',(72.0710649929214,-10.8030075660811,0.));
#53791=CARTESIAN_POINT('Ctrl Pts',(72.0710649929214,-10.8030075660811,12.));
#53792=CARTESIAN_POINT('Ctrl Pts',(72.095959174012,-10.7971153394168,0.));
#53793=CARTESIAN_POINT('Ctrl Pts',(72.095959174012,-10.7971153394168,12.));
#53794=CARTESIAN_POINT('Ctrl Pts',(72.1208856415171,-10.7911906386027,0.));
#53795=CARTESIAN_POINT('Ctrl Pts',(72.1208856415171,-10.7911906386027,12.));
#53796=CARTESIAN_POINT('Ctrl Pts',(72.145844283983,-10.7852334354015,0.));
#53797=CARTESIAN_POINT('Ctrl Pts',(72.145844283983,-10.7852334354015,12.));
#53798=CARTESIAN_POINT('Ctrl Pts',(72.17083499033,-10.779243701766,0.));
#53799=CARTESIAN_POINT('Ctrl Pts',(72.17083499033,-10.779243701766,12.));
#53800=CARTESIAN_POINT('Ctrl Pts',(72.1958576498556,-10.7732214098343,0.));
#53801=CARTESIAN_POINT('Ctrl Pts',(72.1958576498556,-10.7732214098343,12.));
#53802=CARTESIAN_POINT('Ctrl Pts',(72.2209121522367,-10.7671665319254,0.));
#53803=CARTESIAN_POINT('Ctrl Pts',(72.2209121522367,-10.7671665319254,12.));
#53804=CARTESIAN_POINT('Ctrl Pts',(72.2459983875298,-10.7610790405385,0.));
#53805=CARTESIAN_POINT('Ctrl Pts',(72.2459983875298,-10.7610790405385,12.));
#53806=CARTESIAN_POINT('Ctrl Pts',(72.2711162461679,-10.7549589083535,0.));
#53807=CARTESIAN_POINT('Ctrl Pts',(72.2711162461679,-10.7549589083535,12.));
#53808=CARTESIAN_POINT('Ctrl Pts',(72.296265618955,-10.7488061082368,0.));
#53809=CARTESIAN_POINT('Ctrl Pts',(72.296265618955,-10.7488061082368,12.));
#53810=CARTESIAN_POINT('Ctrl Pts',(72.3214463970634,-10.7426206132375,0.));
#53811=CARTESIAN_POINT('Ctrl Pts',(72.3214463970634,-10.7426206132375,12.));
#53812=CARTESIAN_POINT('Ctrl Pts',(72.3466584720311,-10.73640239658,0.));
#53813=CARTESIAN_POINT('Ctrl Pts',(72.3466584720311,-10.73640239658,12.));
#53814=CARTESIAN_POINT('Ctrl Pts',(72.3719017357568,-10.7301514316607,0.));
#53815=CARTESIAN_POINT('Ctrl Pts',(72.3719017357568,-10.7301514316607,12.));
#53816=CARTESIAN_POINT('Ctrl Pts',(72.3971760804935,-10.7238676920469,0.));
#53817=CARTESIAN_POINT('Ctrl Pts',(72.3971760804935,-10.7238676920469,12.));
#53818=CARTESIAN_POINT('Ctrl Pts',(72.4224813988355,-10.7175511514789,0.));
#53819=CARTESIAN_POINT('Ctrl Pts',(72.4224813988355,-10.7175511514789,12.));
#53820=CARTESIAN_POINT('Ctrl Pts',(72.4478175837168,-10.7112017838707,0.));
#53821=CARTESIAN_POINT('Ctrl Pts',(72.4478175837168,-10.7112017838707,12.));
#53822=CARTESIAN_POINT('Ctrl Pts',(72.4731845284238,-10.7048195633062,0.));
#53823=CARTESIAN_POINT('Ctrl Pts',(72.4731845284238,-10.7048195633062,12.));
#53824=CARTESIAN_POINT('Ctrl Pts',(72.4985821266031,-10.6984044640399,0.));
#53825=CARTESIAN_POINT('Ctrl Pts',(72.4985821266031,-10.6984044640399,12.));
#53826=CARTESIAN_POINT('Ctrl Pts',(72.5240102722662,-10.691956460499,0.));
#53827=CARTESIAN_POINT('Ctrl Pts',(72.5240102722662,-10.691956460499,12.));
#53828=CARTESIAN_POINT('Ctrl Pts',(72.5494688597951,-10.6854755272903,0.));
#53829=CARTESIAN_POINT('Ctrl Pts',(72.5494688597951,-10.6854755272903,12.));
#53830=CARTESIAN_POINT('Ctrl Pts',(72.57495778394,-10.6789616392041,0.));
#53831=CARTESIAN_POINT('Ctrl Pts',(72.57495778394,-10.6789616392041,12.));
#53832=CARTESIAN_POINT('Ctrl Pts',(72.6004769398004,-10.6724147711994,0.));
#53833=CARTESIAN_POINT('Ctrl Pts',(72.6004769398004,-10.6724147711994,12.));
#53834=CARTESIAN_POINT('Ctrl Pts',(72.6260262228055,-10.6658348983944,0.));
#53835=CARTESIAN_POINT('Ctrl Pts',(72.6260262228055,-10.6658348983944,12.));
#53836=CARTESIAN_POINT('Ctrl Pts',(72.6516055286908,-10.659221996058,0.));
#53837=CARTESIAN_POINT('Ctrl Pts',(72.6516055286908,-10.659221996058,12.));
#53838=CARTESIAN_POINT('Ctrl Pts',(72.6772147534762,-10.6525760396055,0.));
#53839=CARTESIAN_POINT('Ctrl Pts',(72.6772147534762,-10.6525760396055,12.));
#53840=CARTESIAN_POINT('Ctrl Pts',(72.7028537934332,-10.6458970045948,0.));
#53841=CARTESIAN_POINT('Ctrl Pts',(72.7028537934332,-10.6458970045948,12.));
#53842=CARTESIAN_POINT('Ctrl Pts',(72.7285225451309,-10.6391848667354,0.));
#53843=CARTESIAN_POINT('Ctrl Pts',(72.7285225451309,-10.6391848667354,12.));
#53844=CARTESIAN_POINT('Ctrl Pts',(72.7542209054823,-10.6324396018999,0.));
#53845=CARTESIAN_POINT('Ctrl Pts',(72.7542209054823,-10.6324396018999,12.));
#53846=CARTESIAN_POINT('Ctrl Pts',(72.7799487717914,-10.6256611861395,0.));
#53847=CARTESIAN_POINT('Ctrl Pts',(72.7799487717914,-10.6256611861395,12.));
#53848=CARTESIAN_POINT('Ctrl Pts',(72.8057060417882,-10.6188495956973,0.));
#53849=CARTESIAN_POINT('Ctrl Pts',(72.8057060417882,-10.6188495956973,12.));
#53850=CARTESIAN_POINT('Ctrl Pts',(72.8314926136872,-10.6120048070366,0.));
#53851=CARTESIAN_POINT('Ctrl Pts',(72.8314926136872,-10.6120048070366,12.));
#53852=CARTESIAN_POINT('Ctrl Pts',(72.8573083861328,-10.6051267968202,0.));
#53853=CARTESIAN_POINT('Ctrl Pts',(72.8573083861328,-10.6051267968202,12.));
#53854=CARTESIAN_POINT('Ctrl Pts',(72.8831532580839,-10.5982155418625,0.));
#53855=CARTESIAN_POINT('Ctrl Pts',(72.8831532580839,-10.5982155418625,12.));
#53856=CARTESIAN_POINT('Ctrl Pts',(72.9090271287081,-10.5912710190928,0.));
#53857=CARTESIAN_POINT('Ctrl Pts',(72.9090271287081,-10.5912710190928,12.));
#53858=CARTESIAN_POINT('Ctrl Pts',(72.9349298972823,-10.5842932055209,0.));
#53859=CARTESIAN_POINT('Ctrl Pts',(72.9349298972823,-10.5842932055209,12.));
#53860=CARTESIAN_POINT('Ctrl Pts',(72.9608614630539,-10.5772820781959,0.));
#53861=CARTESIAN_POINT('Ctrl Pts',(72.9608614630539,-10.5772820781959,12.));
#53862=CARTESIAN_POINT('Ctrl Pts',(72.9868217252293,-10.5702376142052,0.));
#53863=CARTESIAN_POINT('Ctrl Pts',(72.9868217252293,-10.5702376142052,12.));
#53864=CARTESIAN_POINT('Ctrl Pts',(73.0128105832635,-10.5631597907653,0.));
#53865=CARTESIAN_POINT('Ctrl Pts',(73.0128105832635,-10.5631597907653,12.));
#53866=CARTESIAN_POINT('Ctrl Pts',(73.0388279370845,-10.5560485852975,0.));
#53867=CARTESIAN_POINT('Ctrl Pts',(73.0388279370845,-10.5560485852975,12.));
#53868=CARTESIAN_POINT('Ctrl Pts',(73.0648736873435,-10.5489039755138,0.));
#53869=CARTESIAN_POINT('Ctrl Pts',(73.0648736873435,-10.5489039755138,12.));
#53870=CARTESIAN_POINT('Ctrl Pts',(73.090947735646,-10.5417259395001,0.));
#53871=CARTESIAN_POINT('Ctrl Pts',(73.090947735646,-10.5417259395001,12.));
#53872=CARTESIAN_POINT('Ctrl Pts',(73.1170499848012,-10.5345144558097,0.));
#53873=CARTESIAN_POINT('Ctrl Pts',(73.1170499848012,-10.5345144558097,12.));
#53874=CARTESIAN_POINT('Ctrl Pts',(73.1431803382677,-10.5272695032649,0.));
#53875=CARTESIAN_POINT('Ctrl Pts',(73.1431803382677,-10.5272695032649,12.));
#53876=CARTESIAN_POINT('Ctrl Pts',(73.169338699611,-10.5199910607652,0.));
#53877=CARTESIAN_POINT('Ctrl Pts',(73.169338699611,-10.5199910607652,12.));
#53878=CARTESIAN_POINT('Ctrl Pts',(73.1955249719037,-10.5126791070804,0.));
#53879=CARTESIAN_POINT('Ctrl Pts',(73.1955249719037,-10.5126791070804,12.));
#53880=CARTESIAN_POINT('Ctrl Pts',(73.2217390572578,-10.505333620691,0.));
#53881=CARTESIAN_POINT('Ctrl Pts',(73.2217390572578,-10.505333620691,12.));
#53882=CARTESIAN_POINT('Ctrl Pts',(73.247980856023,-10.4979545795197,0.));
#53883=CARTESIAN_POINT('Ctrl Pts',(73.247980856023,-10.4979545795197,12.));
#53884=CARTESIAN_POINT('Ctrl Pts',(73.2742502674361,-10.4905419611529,0.));
#53885=CARTESIAN_POINT('Ctrl Pts',(73.2742502674361,-10.4905419611529,12.));
#53886=CARTESIAN_POINT('Ctrl Pts',(73.3005471910639,-10.4830957433311,0.));
#53887=CARTESIAN_POINT('Ctrl Pts',(73.3005471910639,-10.4830957433311,12.));
#53888=CARTESIAN_POINT('Ctrl Pts',(73.3268715280609,-10.475615904381,0.));
#53889=CARTESIAN_POINT('Ctrl Pts',(73.3268715280609,-10.475615904381,12.));
#53890=CARTESIAN_POINT('Ctrl Pts',(73.353223182365,-10.4681024236288,0.));
#53891=CARTESIAN_POINT('Ctrl Pts',(73.353223182365,-10.4681024236288,12.));
#53892=CARTESIAN_POINT('Ctrl Pts',(73.3796020622437,-10.460555281939,0.));
#53893=CARTESIAN_POINT('Ctrl Pts',(73.3796020622437,-10.460555281939,12.));
#53894=CARTESIAN_POINT('Ctrl Pts',(73.4060080806577,-10.4529744618438,0.));
#53895=CARTESIAN_POINT('Ctrl Pts',(73.4060080806577,-10.4529744618438,12.));
#53896=CARTESIAN_POINT('Ctrl Pts',(73.432441151843,-10.4453599463534,0.));
#53897=CARTESIAN_POINT('Ctrl Pts',(73.432441151843,-10.4453599463534,12.));
#53898=CARTESIAN_POINT('Ctrl Pts',(73.45890118861,-10.4377117180212,0.));
#53899=CARTESIAN_POINT('Ctrl Pts',(73.45890118861,-10.4377117180212,12.));
#53900=CARTESIAN_POINT('Ctrl Pts',(73.4853880992228,-10.4300297578648,0.));
#53901=CARTESIAN_POINT('Ctrl Pts',(73.4853880992228,-10.4300297578648,12.));
#53902=CARTESIAN_POINT('Ctrl Pts',(73.5119017847664,-10.4223140444615,0.));
#53903=CARTESIAN_POINT('Ctrl Pts',(73.5119017847664,-10.4223140444615,12.));
#53904=CARTESIAN_POINT('Ctrl Pts',(73.5384421354746,-10.4145645526832,0.));
#53905=CARTESIAN_POINT('Ctrl Pts',(73.5384421354746,-10.4145645526832,12.));
#53906=CARTESIAN_POINT('Ctrl Pts',(73.5650090360114,-10.4067812555539,0.));
#53907=CARTESIAN_POINT('Ctrl Pts',(73.5650090360114,-10.4067812555539,12.));
#53908=CARTESIAN_POINT('Ctrl Pts',(73.5916023719976,-10.3989641265313,0.));
#53909=CARTESIAN_POINT('Ctrl Pts',(73.5916023719976,-10.3989641265313,12.));
#53910=CARTESIAN_POINT('Ctrl Pts',(73.6182220363295,-10.3911131417478,0.));
#53911=CARTESIAN_POINT('Ctrl Pts',(73.6182220363295,-10.3911131417478,12.));
#53912=CARTESIAN_POINT('Ctrl Pts',(73.6448679350605,-10.3832282820361,0.));
#53913=CARTESIAN_POINT('Ctrl Pts',(73.6448679350605,-10.3832282820361,12.));
#53914=CARTESIAN_POINT('Ctrl Pts',(73.6715399947459,-10.3753095356302,0.));
#53915=CARTESIAN_POINT('Ctrl Pts',(73.6715399947459,-10.3753095356302,12.));
#53916=CARTESIAN_POINT('Ctrl Pts',(73.6982381644571,-10.3673568984515,0.));
#53917=CARTESIAN_POINT('Ctrl Pts',(73.6982381644571,-10.3673568984515,12.));
#53918=CARTESIAN_POINT('Ctrl Pts',(73.7249624108433,-10.3593703712542,0.));
#53919=CARTESIAN_POINT('Ctrl Pts',(73.7249624108433,-10.3593703712542,12.));
#53920=CARTESIAN_POINT('Ctrl Pts',(73.7463626541235,-10.3529540403026,0.));
#53921=CARTESIAN_POINT('Ctrl Pts',(73.7463626541235,-10.3529540403026,12.));
#53922=CARTESIAN_POINT('Ctrl Pts',(73.7624245587416,-10.3481265449303,0.));
#53923=CARTESIAN_POINT('Ctrl Pts',(73.7624245587416,-10.3481265449303,12.));
#53924=CARTESIAN_POINT('Ctrl Pts',(73.7731377047922,-10.3449014384439,0.));
#53925=CARTESIAN_POINT('Ctrl Pts',(73.7731377047922,-10.3449014384439,12.));
#53926=CARTESIAN_POINT('Ctrl Pts',(73.778495580227,-10.343287191141,0.));
#53927=CARTESIAN_POINT('Ctrl Pts',(73.778495580227,-10.343287191141,12.));
#53928=CARTESIAN_POINT('',(69.079679653846,-11.3136138754165,0.));
#53929=CARTESIAN_POINT('Ctrl Pts',(69.079679653846,-11.3136138754165,0.));
#53930=CARTESIAN_POINT('Ctrl Pts',(69.0835449954396,-11.3132375200165,0.));
#53931=CARTESIAN_POINT('Ctrl Pts',(69.0912808656811,-11.3124821678798,0.));
#53932=CARTESIAN_POINT('Ctrl Pts',(69.1029002322118,-11.3113412156661,0.));
#53933=CARTESIAN_POINT('Ctrl Pts',(69.118423844466,-11.3098040973713,0.));
#53934=CARTESIAN_POINT('Ctrl Pts',(69.1378802251711,-11.3078562764384,0.));
#53935=CARTESIAN_POINT('Ctrl Pts',(69.1573884361,-11.3058820128307,0.));
#53936=CARTESIAN_POINT('Ctrl Pts',(69.1769483991721,-11.3038812726292,0.));
#53937=CARTESIAN_POINT('Ctrl Pts',(69.1965599718914,-11.3018540025638,0.));
#53938=CARTESIAN_POINT('Ctrl Pts',(69.2162229488531,-11.2998001310964,0.));
#53939=CARTESIAN_POINT('Ctrl Pts',(69.2359370894907,-11.2977195764852,0.));
#53940=CARTESIAN_POINT('Ctrl Pts',(69.255702139335,-11.2956122531375,0.));
#53941=CARTESIAN_POINT('Ctrl Pts',(69.275517853148,-11.2934780784351,0.));
#53942=CARTESIAN_POINT('Ctrl Pts',(69.295384019272,-11.2913169799628,0.));
#53943=CARTESIAN_POINT('Ctrl Pts',(69.3153004517783,-11.2891288931517,0.));
#53944=CARTESIAN_POINT('Ctrl Pts',(69.3352669789587,-11.2869137578459,0.));
#53945=CARTESIAN_POINT('Ctrl Pts',(69.3552834337784,-11.2846715154524,0.));
#53946=CARTESIAN_POINT('Ctrl Pts',(69.3753496420039,-11.2824021054045,0.));
#53947=CARTESIAN_POINT('Ctrl Pts',(69.3954654162281,-11.2801054633816,0.));
#53948=CARTESIAN_POINT('Ctrl Pts',(69.4156305620593,-11.2777815231469,0.));
#53949=CARTESIAN_POINT('Ctrl Pts',(69.4358448819967,-11.2754302177021,0.));
#53950=CARTESIAN_POINT('Ctrl Pts',(69.456108179879,-11.2730514806139,0.));
#53951=CARTESIAN_POINT('Ctrl Pts',(69.4764202659397,-11.270645247528,0.));
#53952=CARTESIAN_POINT('Ctrl Pts',(69.4967809565929,-11.2682114561008,0.));
#53953=CARTESIAN_POINT('Ctrl Pts',(69.5171900720158,-11.2657500452716,0.));
#53954=CARTESIAN_POINT('Ctrl Pts',(69.5376474344771,-11.263260954763,0.));
#53955=CARTESIAN_POINT('Ctrl Pts',(69.5581528662877,-11.2607441244703,0.));
#53956=CARTESIAN_POINT('Ctrl Pts',(69.5787061880857,-11.2581994939541,0.));
#53957=CARTESIAN_POINT('Ctrl Pts',(69.599307219739,-11.2556270027016,0.));
#53958=CARTESIAN_POINT('Ctrl Pts',(69.6199557811245,-11.2530265903557,0.));
#53959=CARTESIAN_POINT('Ctrl Pts',(69.6406516928891,-11.2503981969412,0.));
#53960=CARTESIAN_POINT('Ctrl Pts',(69.6613947773534,-11.2477417631386,0.));
#53961=CARTESIAN_POINT('Ctrl Pts',(69.6821848588457,-11.2450572303841,0.));
#53962=CARTESIAN_POINT('Ctrl Pts',(69.7030217632164,-11.2423445407166,0.));
#53963=CARTESIAN_POINT('Ctrl Pts',(69.7239053175356,-11.239603636686,0.));
#53964=CARTESIAN_POINT('Ctrl Pts',(69.7448353497408,-11.2368344612472,0.));
#53965=CARTESIAN_POINT('Ctrl Pts',(69.7658116882324,-11.2340369576456,0.));
#53966=CARTESIAN_POINT('Ctrl Pts',(69.7868341618954,-11.2312110694187,0.));
#53967=CARTESIAN_POINT('Ctrl Pts',(69.8079026002768,-11.2283567404437,0.));
#53968=CARTESIAN_POINT('Ctrl Pts',(69.8290168337076,-11.225473914972,0.));
#53969=CARTESIAN_POINT('Ctrl Pts',(69.8501766934428,-11.2225625376736,0.));
#53970=CARTESIAN_POINT('Ctrl Pts',(69.871382011789,-11.219622553679,0.));
#53971=CARTESIAN_POINT('Ctrl Pts',(69.8926326220385,-11.2166539085523,0.));
#53972=CARTESIAN_POINT('Ctrl Pts',(69.9139283584022,-11.2136565482678,0.));
#53973=CARTESIAN_POINT('Ctrl Pts',(69.9352690559405,-11.2106304191882,0.));
#53974=CARTESIAN_POINT('Ctrl Pts',(69.9566545504837,-11.2075754680449,0.));
#53975=CARTESIAN_POINT('Ctrl Pts',(69.97808467858,-11.2044916419244,0.));
#53976=CARTESIAN_POINT('Ctrl Pts',(69.9995592775343,-11.2013788882714,0.));
#53977=CARTESIAN_POINT('Ctrl Pts',(70.0210781854243,-11.1982371548919,0.));
#53978=CARTESIAN_POINT('Ctrl Pts',(70.0426412411185,-11.1950663899576,0.));
#53979=CARTESIAN_POINT('Ctrl Pts',(70.0642482842928,-11.1918665420166,0.));
#53980=CARTESIAN_POINT('Ctrl Pts',(70.0858991554283,-11.1886375599914,0.));
#53981=CARTESIAN_POINT('Ctrl Pts',(70.1075936957968,-11.185379393167,0.));
#53982=CARTESIAN_POINT('Ctrl Pts',(70.1293317474432,-11.1820919911846,0.));
#53983=CARTESIAN_POINT('Ctrl Pts',(70.1511131531674,-11.1787753040363,0.));
#53984=CARTESIAN_POINT('Ctrl Pts',(70.1729377564956,-11.1754292820631,0.));
#53985=CARTESIAN_POINT('Ctrl Pts',(70.1948054016817,-11.1720538759499,0.));
#53986=CARTESIAN_POINT('Ctrl Pts',(70.2167159337095,-11.168649036721,0.));
#53987=CARTESIAN_POINT('Ctrl Pts',(70.2386691982902,-11.1652147157383,0.));
#53988=CARTESIAN_POINT('Ctrl Pts',(70.2606650418589,-11.1617508647017,0.));
#53989=CARTESIAN_POINT('Ctrl Pts',(70.2827033115662,-11.1582574356522,0.));
#53990=CARTESIAN_POINT('Ctrl Pts',(70.3047838552758,-11.1547343809647,0.));
#53991=CARTESIAN_POINT('Ctrl Pts',(70.3269065215591,-11.1511816533422,0.));
#53992=CARTESIAN_POINT('Ctrl Pts',(70.3490711596882,-11.1475992058124,0.));
#53993=CARTESIAN_POINT('Ctrl Pts',(70.3712776196216,-11.1439869917269,0.));
#53994=CARTESIAN_POINT('Ctrl Pts',(70.3935257519945,-11.1403449647622,0.));
#53995=CARTESIAN_POINT('Ctrl Pts',(70.415815408119,-11.1366730789122,0.));
#53996=CARTESIAN_POINT('Ctrl Pts',(70.438146439981,-11.1329712884845,0.));
#53997=CARTESIAN_POINT('Ctrl Pts',(70.4605187002356,-11.1292395480975,0.));
#53998=CARTESIAN_POINT('Ctrl Pts',(70.4829320421973,-11.1254778126824,0.));
#53999=CARTESIAN_POINT('Ctrl Pts',(70.5053863198306,-11.121686037483,0.));
#54000=CARTESIAN_POINT('Ctrl Pts',(70.5278813877519,-11.117864178048,0.));
#54001=CARTESIAN_POINT('Ctrl Pts',(70.5504171012247,-11.1140121902274,0.));
#54002=CARTESIAN_POINT('Ctrl Pts',(70.5729933161538,-11.11013003017,0.));
#54003=CARTESIAN_POINT('Ctrl Pts',(70.5956098890744,-11.1062176543257,0.));
#54004=CARTESIAN_POINT('Ctrl Pts',(70.6182666771441,-11.1022750194439,0.));
#54005=CARTESIAN_POINT('Ctrl Pts',(70.6409635381446,-11.0983020825662,0.));
#54006=CARTESIAN_POINT('Ctrl Pts',(70.6637003304768,-11.0942988010231,0.));
#54007=CARTESIAN_POINT('Ctrl Pts',(70.686476913156,-11.0902651324325,0.));
#54008=CARTESIAN_POINT('Ctrl Pts',(70.7092931457996,-11.0862010347022,0.));
#54009=CARTESIAN_POINT('Ctrl Pts',(70.7321488886229,-11.0821064660276,0.));
#54010=CARTESIAN_POINT('Ctrl Pts',(70.7550440024422,-11.0779813848851,0.));
#54011=CARTESIAN_POINT('Ctrl Pts',(70.7779783486689,-11.0738257500292,0.));
#54012=CARTESIAN_POINT('Ctrl Pts',(70.8009517893042,-11.0696395204908,0.));
#54013=CARTESIAN_POINT('Ctrl Pts',(70.8239641869266,-11.0654226555798,0.));
#54014=CARTESIAN_POINT('Ctrl Pts',(70.847015404688,-11.061175114883,0.));
#54015=CARTESIAN_POINT('Ctrl Pts',(70.8701053063158,-11.0568968582566,0.));
#54016=CARTESIAN_POINT('Ctrl Pts',(70.8932337561078,-11.0525878458242,0.));
#54017=CARTESIAN_POINT('Ctrl Pts',(70.9164006189283,-11.0482480379752,0.));
#54018=CARTESIAN_POINT('Ctrl Pts',(70.9396057601953,-11.0438773953686,0.));
#54019=CARTESIAN_POINT('Ctrl Pts',(70.9628490458779,-11.039475878929,0.));
#54020=CARTESIAN_POINT('Ctrl Pts',(70.9861303424989,-11.0350434498408,0.));
#54021=CARTESIAN_POINT('Ctrl Pts',(71.0094495171295,-11.0305800695457,0.));
#54022=CARTESIAN_POINT('Ctrl Pts',(71.0328064373849,-11.0260856997414,0.));
#54023=CARTESIAN_POINT('Ctrl Pts',(71.0562009714125,-11.0215603023854,0.));
#54024=CARTESIAN_POINT('Ctrl Pts',(71.0796329878896,-11.0170038396913,0.));
#54025=CARTESIAN_POINT('Ctrl Pts',(71.1031023560243,-11.0124162741223,0.));
#54026=CARTESIAN_POINT('Ctrl Pts',(71.1266089455517,-11.0077975683895,0.));
#54027=CARTESIAN_POINT('Ctrl Pts',(71.1501526267288,-11.0031476854503,0.));
#54028=CARTESIAN_POINT('Ctrl Pts',(71.1737332703248,-10.9984665885127,0.));
#54029=CARTESIAN_POINT('Ctrl Pts',(71.1973507476188,-10.993754241032,0.));
#54030=CARTESIAN_POINT('Ctrl Pts',(71.221004930401,-10.9890106067038,0.));
#54031=CARTESIAN_POINT('Ctrl Pts',(71.2446956909685,-10.9842356494627,0.));
#54032=CARTESIAN_POINT('Ctrl Pts',(71.2684229021209,-10.9794293334806,0.));
#54033=CARTESIAN_POINT('Ctrl Pts',(71.2921864371499,-10.9745916231711,0.));
#54034=CARTESIAN_POINT('Ctrl Pts',(71.3159861698368,-10.9697224831862,0.));
#54035=CARTESIAN_POINT('Ctrl Pts',(71.3398219744547,-10.96482187841,0.));
#54036=CARTESIAN_POINT('Ctrl Pts',(71.3636937257651,-10.9598897739565,0.));
#54037=CARTESIAN_POINT('Ctrl Pts',(71.3876012990135,-10.954926135169,0.));
#54038=CARTESIAN_POINT('Ctrl Pts',(71.411544569919,-10.9499309276235,0.));
#54039=CARTESIAN_POINT('Ctrl Pts',(71.4355234146718,-10.9449041171269,0.));
#54040=CARTESIAN_POINT('Ctrl Pts',(71.4595377099352,-10.9398456697095,0.));
#54041=CARTESIAN_POINT('Ctrl Pts',(71.4835873328425,-10.9347555516236,0.));
#54042=CARTESIAN_POINT('Ctrl Pts',(71.5076721609936,-10.9296337293425,0.));
#54043=CARTESIAN_POINT('Ctrl Pts',(71.5317920724453,-10.9244801695642,0.));
#54044=CARTESIAN_POINT('Ctrl Pts',(71.5559469457082,-10.9192948392099,0.));
#54045=CARTESIAN_POINT('Ctrl Pts',(71.5801366597479,-10.9140777054169,0.));
#54046=CARTESIAN_POINT('Ctrl Pts',(71.604361093983,-10.9088287355364,0.));
#54047=CARTESIAN_POINT('Ctrl Pts',(71.6286201282815,-10.9035478971329,0.));
#54048=CARTESIAN_POINT('Ctrl Pts',(71.6529136429515,-10.8982351579872,0.));
#54049=CARTESIAN_POINT('Ctrl Pts',(71.6772415187382,-10.8928904860967,0.));
#54050=CARTESIAN_POINT('Ctrl Pts',(71.7016036368254,-10.8875138496674,0.));
#54051=CARTESIAN_POINT('Ctrl Pts',(71.7259998788337,-10.8821052171122,0.));
#54052=CARTESIAN_POINT('Ctrl Pts',(71.7504301268177,-10.8766645570496,0.));
#54053=CARTESIAN_POINT('Ctrl Pts',(71.7748942632578,-10.8711918383071,0.));
#54054=CARTESIAN_POINT('Ctrl Pts',(71.7993921710546,-10.8656870299218,0.));
#54055=CARTESIAN_POINT('Ctrl Pts',(71.8239237335318,-10.860150101133,0.));
#54056=CARTESIAN_POINT('Ctrl Pts',(71.8484888344335,-10.8545810213799,0.));
#54057=CARTESIAN_POINT('Ctrl Pts',(71.8730873579226,-10.8489797602998,0.));
#54058=CARTESIAN_POINT('Ctrl Pts',(71.8977191885726,-10.8433462877312,0.));
#54059=CARTESIAN_POINT('Ctrl Pts',(71.9223842113622,-10.8376805737158,0.));
#54060=CARTESIAN_POINT('Ctrl Pts',(71.9470823116777,-10.8319825884917,0.));
#54061=CARTESIAN_POINT('Ctrl Pts',(71.971813375312,-10.8262523024897,0.));
#54062=CARTESIAN_POINT('Ctrl Pts',(71.996577288462,-10.8204896863328,0.));
#54063=CARTESIAN_POINT('Ctrl Pts',(72.0213739377231,-10.8146947108376,0.));
#54064=CARTESIAN_POINT('Ctrl Pts',(72.0462032100828,-10.8088673470187,0.));
#54065=CARTESIAN_POINT('Ctrl Pts',(72.0710649929214,-10.8030075660811,0.));
#54066=CARTESIAN_POINT('Ctrl Pts',(72.095959174012,-10.7971153394168,0.));
#54067=CARTESIAN_POINT('Ctrl Pts',(72.1208856415171,-10.7911906386027,0.));
#54068=CARTESIAN_POINT('Ctrl Pts',(72.145844283983,-10.7852334354015,0.));
#54069=CARTESIAN_POINT('Ctrl Pts',(72.17083499033,-10.779243701766,0.));
#54070=CARTESIAN_POINT('Ctrl Pts',(72.1958576498556,-10.7732214098343,0.));
#54071=CARTESIAN_POINT('Ctrl Pts',(72.2209121522367,-10.7671665319254,0.));
#54072=CARTESIAN_POINT('Ctrl Pts',(72.2459983875298,-10.7610790405385,0.));
#54073=CARTESIAN_POINT('Ctrl Pts',(72.2711162461679,-10.7549589083535,0.));
#54074=CARTESIAN_POINT('Ctrl Pts',(72.296265618955,-10.7488061082368,0.));
#54075=CARTESIAN_POINT('Ctrl Pts',(72.3214463970634,-10.7426206132375,0.));
#54076=CARTESIAN_POINT('Ctrl Pts',(72.3466584720311,-10.73640239658,0.));
#54077=CARTESIAN_POINT('Ctrl Pts',(72.3719017357568,-10.7301514316607,0.));
#54078=CARTESIAN_POINT('Ctrl Pts',(72.3971760804935,-10.7238676920469,0.));
#54079=CARTESIAN_POINT('Ctrl Pts',(72.4224813988355,-10.7175511514789,0.));
#54080=CARTESIAN_POINT('Ctrl Pts',(72.4478175837168,-10.7112017838707,0.));
#54081=CARTESIAN_POINT('Ctrl Pts',(72.4731845284238,-10.7048195633062,0.));
#54082=CARTESIAN_POINT('Ctrl Pts',(72.4985821266031,-10.6984044640399,0.));
#54083=CARTESIAN_POINT('Ctrl Pts',(72.5240102722662,-10.691956460499,0.));
#54084=CARTESIAN_POINT('Ctrl Pts',(72.5494688597951,-10.6854755272903,0.));
#54085=CARTESIAN_POINT('Ctrl Pts',(72.57495778394,-10.6789616392041,0.));
#54086=CARTESIAN_POINT('Ctrl Pts',(72.6004769398004,-10.6724147711994,0.));
#54087=CARTESIAN_POINT('Ctrl Pts',(72.6260262228055,-10.6658348983944,0.));
#54088=CARTESIAN_POINT('Ctrl Pts',(72.6516055286908,-10.659221996058,0.));
#54089=CARTESIAN_POINT('Ctrl Pts',(72.6772147534762,-10.6525760396055,0.));
#54090=CARTESIAN_POINT('Ctrl Pts',(72.7028537934332,-10.6458970045948,0.));
#54091=CARTESIAN_POINT('Ctrl Pts',(72.7285225451309,-10.6391848667354,0.));
#54092=CARTESIAN_POINT('Ctrl Pts',(72.7542209054823,-10.6324396018999,0.));
#54093=CARTESIAN_POINT('Ctrl Pts',(72.7799487717914,-10.6256611861395,0.));
#54094=CARTESIAN_POINT('Ctrl Pts',(72.8057060417882,-10.6188495956973,0.));
#54095=CARTESIAN_POINT('Ctrl Pts',(72.8314926136872,-10.6120048070366,0.));
#54096=CARTESIAN_POINT('Ctrl Pts',(72.8573083861328,-10.6051267968202,0.));
#54097=CARTESIAN_POINT('Ctrl Pts',(72.8831532580839,-10.5982155418625,0.));
#54098=CARTESIAN_POINT('Ctrl Pts',(72.9090271287081,-10.5912710190928,0.));
#54099=CARTESIAN_POINT('Ctrl Pts',(72.9349298972823,-10.5842932055209,0.));
#54100=CARTESIAN_POINT('Ctrl Pts',(72.9608614630539,-10.5772820781959,0.));
#54101=CARTESIAN_POINT('Ctrl Pts',(72.9868217252293,-10.5702376142052,0.));
#54102=CARTESIAN_POINT('Ctrl Pts',(73.0128105832635,-10.5631597907653,0.));
#54103=CARTESIAN_POINT('Ctrl Pts',(73.0388279370845,-10.5560485852975,0.));
#54104=CARTESIAN_POINT('Ctrl Pts',(73.0648736873435,-10.5489039755138,0.));
#54105=CARTESIAN_POINT('Ctrl Pts',(73.090947735646,-10.5417259395001,0.));
#54106=CARTESIAN_POINT('Ctrl Pts',(73.1170499848012,-10.5345144558097,0.));
#54107=CARTESIAN_POINT('Ctrl Pts',(73.1431803382677,-10.5272695032649,0.));
#54108=CARTESIAN_POINT('Ctrl Pts',(73.169338699611,-10.5199910607652,0.));
#54109=CARTESIAN_POINT('Ctrl Pts',(73.1955249719037,-10.5126791070804,0.));
#54110=CARTESIAN_POINT('Ctrl Pts',(73.2217390572578,-10.505333620691,0.));
#54111=CARTESIAN_POINT('Ctrl Pts',(73.247980856023,-10.4979545795197,0.));
#54112=CARTESIAN_POINT('Ctrl Pts',(73.2742502674361,-10.4905419611529,0.));
#54113=CARTESIAN_POINT('Ctrl Pts',(73.3005471910639,-10.4830957433311,0.));
#54114=CARTESIAN_POINT('Ctrl Pts',(73.3268715280609,-10.475615904381,0.));
#54115=CARTESIAN_POINT('Ctrl Pts',(73.353223182365,-10.4681024236288,0.));
#54116=CARTESIAN_POINT('Ctrl Pts',(73.3796020622437,-10.460555281939,0.));
#54117=CARTESIAN_POINT('Ctrl Pts',(73.4060080806577,-10.4529744618438,0.));
#54118=CARTESIAN_POINT('Ctrl Pts',(73.4286663447915,-10.4464473465486,0.));
#54119=CARTESIAN_POINT('Ctrl Pts',(73.4460525528551,-10.4414249334768,0.));
#54120=CARTESIAN_POINT('Ctrl Pts',(73.4581547436539,-10.4379221501093,0.));
#54121=CARTESIAN_POINT('Ctrl Pts',(73.464965036154,-10.4359488742883,0.));
#54122=CARTESIAN_POINT('Ctrl Pts',(73.4664795929518,-10.4355099267391,0.));
#54123=CARTESIAN_POINT('',(69.079679653846,-11.3136138754165,12.));
#54124=CARTESIAN_POINT('',(69.079679653846,-11.3136138754165,0.));
#54125=CARTESIAN_POINT('Ctrl Pts',(73.4664795929519,-10.4355099267391,12.));
#54126=CARTESIAN_POINT('Ctrl Pts',(73.464965036154,-10.4359488742883,12.));
#54127=CARTESIAN_POINT('Ctrl Pts',(73.458154743654,-10.4379221501093,12.));
#54128=CARTESIAN_POINT('Ctrl Pts',(73.4460525528551,-10.4414249334768,12.));
#54129=CARTESIAN_POINT('Ctrl Pts',(73.4286663447915,-10.4464473465486,12.));
#54130=CARTESIAN_POINT('Ctrl Pts',(73.4060080806577,-10.4529744618438,12.));
#54131=CARTESIAN_POINT('Ctrl Pts',(73.3796020622437,-10.460555281939,12.));
#54132=CARTESIAN_POINT('Ctrl Pts',(73.353223182365,-10.4681024236288,12.));
#54133=CARTESIAN_POINT('Ctrl Pts',(73.3268715280609,-10.475615904381,12.));
#54134=CARTESIAN_POINT('Ctrl Pts',(73.3005471910639,-10.4830957433311,12.));
#54135=CARTESIAN_POINT('Ctrl Pts',(73.2742502674361,-10.4905419611529,12.));
#54136=CARTESIAN_POINT('Ctrl Pts',(73.247980856023,-10.4979545795197,12.));
#54137=CARTESIAN_POINT('Ctrl Pts',(73.2217390572578,-10.505333620691,12.));
#54138=CARTESIAN_POINT('Ctrl Pts',(73.1955249719037,-10.5126791070804,12.));
#54139=CARTESIAN_POINT('Ctrl Pts',(73.169338699611,-10.5199910607652,12.));
#54140=CARTESIAN_POINT('Ctrl Pts',(73.1431803382677,-10.5272695032649,12.));
#54141=CARTESIAN_POINT('Ctrl Pts',(73.1170499848012,-10.5345144558097,12.));
#54142=CARTESIAN_POINT('Ctrl Pts',(73.090947735646,-10.5417259395001,12.));
#54143=CARTESIAN_POINT('Ctrl Pts',(73.0648736873435,-10.5489039755138,12.));
#54144=CARTESIAN_POINT('Ctrl Pts',(73.0388279370845,-10.5560485852975,12.));
#54145=CARTESIAN_POINT('Ctrl Pts',(73.0128105832635,-10.5631597907653,12.));
#54146=CARTESIAN_POINT('Ctrl Pts',(72.9868217252293,-10.5702376142052,12.));
#54147=CARTESIAN_POINT('Ctrl Pts',(72.9608614630539,-10.5772820781959,12.));
#54148=CARTESIAN_POINT('Ctrl Pts',(72.9349298972823,-10.5842932055209,12.));
#54149=CARTESIAN_POINT('Ctrl Pts',(72.9090271287081,-10.5912710190928,12.));
#54150=CARTESIAN_POINT('Ctrl Pts',(72.8831532580839,-10.5982155418625,12.));
#54151=CARTESIAN_POINT('Ctrl Pts',(72.8573083861328,-10.6051267968202,12.));
#54152=CARTESIAN_POINT('Ctrl Pts',(72.8314926136872,-10.6120048070366,12.));
#54153=CARTESIAN_POINT('Ctrl Pts',(72.8057060417882,-10.6188495956973,12.));
#54154=CARTESIAN_POINT('Ctrl Pts',(72.7799487717914,-10.6256611861395,12.));
#54155=CARTESIAN_POINT('Ctrl Pts',(72.7542209054823,-10.6324396018999,12.));
#54156=CARTESIAN_POINT('Ctrl Pts',(72.7285225451309,-10.6391848667354,12.));
#54157=CARTESIAN_POINT('Ctrl Pts',(72.7028537934332,-10.6458970045948,12.));
#54158=CARTESIAN_POINT('Ctrl Pts',(72.6772147534762,-10.6525760396055,12.));
#54159=CARTESIAN_POINT('Ctrl Pts',(72.6516055286908,-10.659221996058,12.));
#54160=CARTESIAN_POINT('Ctrl Pts',(72.6260262228055,-10.6658348983944,12.));
#54161=CARTESIAN_POINT('Ctrl Pts',(72.6004769398004,-10.6724147711994,12.));
#54162=CARTESIAN_POINT('Ctrl Pts',(72.57495778394,-10.6789616392041,12.));
#54163=CARTESIAN_POINT('Ctrl Pts',(72.5494688597951,-10.6854755272903,12.));
#54164=CARTESIAN_POINT('Ctrl Pts',(72.5240102722662,-10.691956460499,12.));
#54165=CARTESIAN_POINT('Ctrl Pts',(72.4985821266031,-10.6984044640399,12.));
#54166=CARTESIAN_POINT('Ctrl Pts',(72.4731845284238,-10.7048195633062,12.));
#54167=CARTESIAN_POINT('Ctrl Pts',(72.4478175837168,-10.7112017838707,12.));
#54168=CARTESIAN_POINT('Ctrl Pts',(72.4224813988355,-10.7175511514789,12.));
#54169=CARTESIAN_POINT('Ctrl Pts',(72.3971760804935,-10.7238676920469,12.));
#54170=CARTESIAN_POINT('Ctrl Pts',(72.3719017357568,-10.7301514316607,12.));
#54171=CARTESIAN_POINT('Ctrl Pts',(72.3466584720311,-10.73640239658,12.));
#54172=CARTESIAN_POINT('Ctrl Pts',(72.3214463970634,-10.7426206132375,12.));
#54173=CARTESIAN_POINT('Ctrl Pts',(72.296265618955,-10.7488061082368,12.));
#54174=CARTESIAN_POINT('Ctrl Pts',(72.2711162461679,-10.7549589083535,12.));
#54175=CARTESIAN_POINT('Ctrl Pts',(72.2459983875298,-10.7610790405385,12.));
#54176=CARTESIAN_POINT('Ctrl Pts',(72.2209121522367,-10.7671665319254,12.));
#54177=CARTESIAN_POINT('Ctrl Pts',(72.1958576498556,-10.7732214098343,12.));
#54178=CARTESIAN_POINT('Ctrl Pts',(72.17083499033,-10.779243701766,12.));
#54179=CARTESIAN_POINT('Ctrl Pts',(72.145844283983,-10.7852334354015,12.));
#54180=CARTESIAN_POINT('Ctrl Pts',(72.1208856415171,-10.7911906386027,12.));
#54181=CARTESIAN_POINT('Ctrl Pts',(72.095959174012,-10.7971153394168,12.));
#54182=CARTESIAN_POINT('Ctrl Pts',(72.0710649929214,-10.8030075660811,12.));
#54183=CARTESIAN_POINT('Ctrl Pts',(72.0462032100828,-10.8088673470187,12.));
#54184=CARTESIAN_POINT('Ctrl Pts',(72.0213739377231,-10.8146947108376,12.));
#54185=CARTESIAN_POINT('Ctrl Pts',(71.996577288462,-10.8204896863328,12.));
#54186=CARTESIAN_POINT('Ctrl Pts',(71.971813375312,-10.8262523024897,12.));
#54187=CARTESIAN_POINT('Ctrl Pts',(71.9470823116777,-10.8319825884917,12.));
#54188=CARTESIAN_POINT('Ctrl Pts',(71.9223842113622,-10.8376805737158,12.));
#54189=CARTESIAN_POINT('Ctrl Pts',(71.8977191885726,-10.8433462877312,12.));
#54190=CARTESIAN_POINT('Ctrl Pts',(71.8730873579226,-10.8489797602998,12.));
#54191=CARTESIAN_POINT('Ctrl Pts',(71.8484888344335,-10.8545810213799,12.));
#54192=CARTESIAN_POINT('Ctrl Pts',(71.8239237335318,-10.860150101133,12.));
#54193=CARTESIAN_POINT('Ctrl Pts',(71.7993921710546,-10.8656870299218,12.));
#54194=CARTESIAN_POINT('Ctrl Pts',(71.7748942632578,-10.8711918383071,12.));
#54195=CARTESIAN_POINT('Ctrl Pts',(71.7504301268177,-10.8766645570496,12.));
#54196=CARTESIAN_POINT('Ctrl Pts',(71.7259998788337,-10.8821052171122,12.));
#54197=CARTESIAN_POINT('Ctrl Pts',(71.7016036368254,-10.8875138496674,12.));
#54198=CARTESIAN_POINT('Ctrl Pts',(71.6772415187382,-10.8928904860967,12.));
#54199=CARTESIAN_POINT('Ctrl Pts',(71.6529136429515,-10.8982351579872,12.));
#54200=CARTESIAN_POINT('Ctrl Pts',(71.6286201282815,-10.9035478971329,12.));
#54201=CARTESIAN_POINT('Ctrl Pts',(71.604361093983,-10.9088287355364,12.));
#54202=CARTESIAN_POINT('Ctrl Pts',(71.5801366597479,-10.9140777054169,12.));
#54203=CARTESIAN_POINT('Ctrl Pts',(71.5559469457082,-10.9192948392099,12.));
#54204=CARTESIAN_POINT('Ctrl Pts',(71.5317920724453,-10.9244801695642,12.));
#54205=CARTESIAN_POINT('Ctrl Pts',(71.5076721609936,-10.9296337293425,12.));
#54206=CARTESIAN_POINT('Ctrl Pts',(71.4835873328425,-10.9347555516236,12.));
#54207=CARTESIAN_POINT('Ctrl Pts',(71.4595377099352,-10.9398456697095,12.));
#54208=CARTESIAN_POINT('Ctrl Pts',(71.4355234146718,-10.9449041171269,12.));
#54209=CARTESIAN_POINT('Ctrl Pts',(71.411544569919,-10.9499309276235,12.));
#54210=CARTESIAN_POINT('Ctrl Pts',(71.3876012990135,-10.954926135169,12.));
#54211=CARTESIAN_POINT('Ctrl Pts',(71.3636937257651,-10.9598897739565,12.));
#54212=CARTESIAN_POINT('Ctrl Pts',(71.3398219744547,-10.96482187841,12.));
#54213=CARTESIAN_POINT('Ctrl Pts',(71.3159861698368,-10.9697224831862,12.));
#54214=CARTESIAN_POINT('Ctrl Pts',(71.2921864371499,-10.9745916231711,12.));
#54215=CARTESIAN_POINT('Ctrl Pts',(71.2684229021209,-10.9794293334806,12.));
#54216=CARTESIAN_POINT('Ctrl Pts',(71.2446956909685,-10.9842356494627,12.));
#54217=CARTESIAN_POINT('Ctrl Pts',(71.221004930401,-10.9890106067038,12.));
#54218=CARTESIAN_POINT('Ctrl Pts',(71.1973507476188,-10.993754241032,12.));
#54219=CARTESIAN_POINT('Ctrl Pts',(71.1737332703248,-10.9984665885127,12.));
#54220=CARTESIAN_POINT('Ctrl Pts',(71.1501526267288,-11.0031476854503,12.));
#54221=CARTESIAN_POINT('Ctrl Pts',(71.1266089455517,-11.0077975683895,12.));
#54222=CARTESIAN_POINT('Ctrl Pts',(71.1031023560243,-11.0124162741223,12.));
#54223=CARTESIAN_POINT('Ctrl Pts',(71.0796329878896,-11.0170038396913,12.));
#54224=CARTESIAN_POINT('Ctrl Pts',(71.0562009714125,-11.0215603023854,12.));
#54225=CARTESIAN_POINT('Ctrl Pts',(71.0328064373849,-11.0260856997414,12.));
#54226=CARTESIAN_POINT('Ctrl Pts',(71.0094495171295,-11.0305800695457,12.));
#54227=CARTESIAN_POINT('Ctrl Pts',(70.9861303424989,-11.0350434498408,12.));
#54228=CARTESIAN_POINT('Ctrl Pts',(70.9628490458779,-11.039475878929,12.));
#54229=CARTESIAN_POINT('Ctrl Pts',(70.9396057601953,-11.0438773953686,12.));
#54230=CARTESIAN_POINT('Ctrl Pts',(70.9164006189283,-11.0482480379752,12.));
#54231=CARTESIAN_POINT('Ctrl Pts',(70.8932337561078,-11.0525878458242,12.));
#54232=CARTESIAN_POINT('Ctrl Pts',(70.8701053063158,-11.0568968582566,12.));
#54233=CARTESIAN_POINT('Ctrl Pts',(70.847015404688,-11.061175114883,12.));
#54234=CARTESIAN_POINT('Ctrl Pts',(70.8239641869266,-11.0654226555798,12.));
#54235=CARTESIAN_POINT('Ctrl Pts',(70.8009517893042,-11.0696395204908,12.));
#54236=CARTESIAN_POINT('Ctrl Pts',(70.7779783486689,-11.0738257500292,12.));
#54237=CARTESIAN_POINT('Ctrl Pts',(70.7550440024422,-11.0779813848851,12.));
#54238=CARTESIAN_POINT('Ctrl Pts',(70.7321488886229,-11.0821064660276,12.));
#54239=CARTESIAN_POINT('Ctrl Pts',(70.7092931457996,-11.0862010347022,12.));
#54240=CARTESIAN_POINT('Ctrl Pts',(70.686476913156,-11.0902651324325,12.));
#54241=CARTESIAN_POINT('Ctrl Pts',(70.6637003304768,-11.0942988010231,12.));
#54242=CARTESIAN_POINT('Ctrl Pts',(70.6409635381446,-11.0983020825662,12.));
#54243=CARTESIAN_POINT('Ctrl Pts',(70.6182666771441,-11.1022750194439,12.));
#54244=CARTESIAN_POINT('Ctrl Pts',(70.5956098890744,-11.1062176543257,12.));
#54245=CARTESIAN_POINT('Ctrl Pts',(70.5729933161538,-11.11013003017,12.));
#54246=CARTESIAN_POINT('Ctrl Pts',(70.5504171012247,-11.1140121902274,12.));
#54247=CARTESIAN_POINT('Ctrl Pts',(70.5278813877519,-11.117864178048,12.));
#54248=CARTESIAN_POINT('Ctrl Pts',(70.5053863198306,-11.121686037483,12.));
#54249=CARTESIAN_POINT('Ctrl Pts',(70.4829320421973,-11.1254778126824,12.));
#54250=CARTESIAN_POINT('Ctrl Pts',(70.4605187002356,-11.1292395480975,12.));
#54251=CARTESIAN_POINT('Ctrl Pts',(70.438146439981,-11.1329712884845,12.));
#54252=CARTESIAN_POINT('Ctrl Pts',(70.415815408119,-11.1366730789122,12.));
#54253=CARTESIAN_POINT('Ctrl Pts',(70.3935257519945,-11.1403449647622,12.));
#54254=CARTESIAN_POINT('Ctrl Pts',(70.3712776196216,-11.1439869917269,12.));
#54255=CARTESIAN_POINT('Ctrl Pts',(70.3490711596882,-11.1475992058124,12.));
#54256=CARTESIAN_POINT('Ctrl Pts',(70.3269065215591,-11.1511816533422,12.));
#54257=CARTESIAN_POINT('Ctrl Pts',(70.3047838552758,-11.1547343809647,12.));
#54258=CARTESIAN_POINT('Ctrl Pts',(70.2827033115662,-11.1582574356522,12.));
#54259=CARTESIAN_POINT('Ctrl Pts',(70.2606650418589,-11.1617508647017,12.));
#54260=CARTESIAN_POINT('Ctrl Pts',(70.2386691982902,-11.1652147157383,12.));
#54261=CARTESIAN_POINT('Ctrl Pts',(70.2167159337095,-11.168649036721,12.));
#54262=CARTESIAN_POINT('Ctrl Pts',(70.1948054016817,-11.1720538759499,12.));
#54263=CARTESIAN_POINT('Ctrl Pts',(70.1729377564956,-11.1754292820631,12.));
#54264=CARTESIAN_POINT('Ctrl Pts',(70.1511131531674,-11.1787753040363,12.));
#54265=CARTESIAN_POINT('Ctrl Pts',(70.1293317474432,-11.1820919911846,12.));
#54266=CARTESIAN_POINT('Ctrl Pts',(70.1075936957968,-11.185379393167,12.));
#54267=CARTESIAN_POINT('Ctrl Pts',(70.0858991554283,-11.1886375599914,12.));
#54268=CARTESIAN_POINT('Ctrl Pts',(70.0642482842928,-11.1918665420166,12.));
#54269=CARTESIAN_POINT('Ctrl Pts',(70.0426412411185,-11.1950663899576,12.));
#54270=CARTESIAN_POINT('Ctrl Pts',(70.0210781854243,-11.1982371548919,12.));
#54271=CARTESIAN_POINT('Ctrl Pts',(69.9995592775343,-11.2013788882714,12.));
#54272=CARTESIAN_POINT('Ctrl Pts',(69.97808467858,-11.2044916419244,12.));
#54273=CARTESIAN_POINT('Ctrl Pts',(69.9566545504837,-11.2075754680449,12.));
#54274=CARTESIAN_POINT('Ctrl Pts',(69.9352690559405,-11.2106304191882,12.));
#54275=CARTESIAN_POINT('Ctrl Pts',(69.9139283584022,-11.2136565482678,12.));
#54276=CARTESIAN_POINT('Ctrl Pts',(69.8926326220385,-11.2166539085523,12.));
#54277=CARTESIAN_POINT('Ctrl Pts',(69.871382011789,-11.219622553679,12.));
#54278=CARTESIAN_POINT('Ctrl Pts',(69.8501766934428,-11.2225625376736,12.));
#54279=CARTESIAN_POINT('Ctrl Pts',(69.8290168337076,-11.225473914972,12.));
#54280=CARTESIAN_POINT('Ctrl Pts',(69.8079026002768,-11.2283567404437,12.));
#54281=CARTESIAN_POINT('Ctrl Pts',(69.7868341618954,-11.2312110694187,12.));
#54282=CARTESIAN_POINT('Ctrl Pts',(69.7658116882324,-11.2340369576456,12.));
#54283=CARTESIAN_POINT('Ctrl Pts',(69.7448353497408,-11.2368344612472,12.));
#54284=CARTESIAN_POINT('Ctrl Pts',(69.7239053175356,-11.239603636686,12.));
#54285=CARTESIAN_POINT('Ctrl Pts',(69.7030217632164,-11.2423445407166,12.));
#54286=CARTESIAN_POINT('Ctrl Pts',(69.6821848588457,-11.2450572303841,12.));
#54287=CARTESIAN_POINT('Ctrl Pts',(69.6613947773534,-11.2477417631386,12.));
#54288=CARTESIAN_POINT('Ctrl Pts',(69.6406516928891,-11.2503981969412,12.));
#54289=CARTESIAN_POINT('Ctrl Pts',(69.6199557811245,-11.2530265903557,12.));
#54290=CARTESIAN_POINT('Ctrl Pts',(69.599307219739,-11.2556270027016,12.));
#54291=CARTESIAN_POINT('Ctrl Pts',(69.5787061880857,-11.2581994939541,12.));
#54292=CARTESIAN_POINT('Ctrl Pts',(69.5581528662877,-11.2607441244703,12.));
#54293=CARTESIAN_POINT('Ctrl Pts',(69.5376474344771,-11.263260954763,12.));
#54294=CARTESIAN_POINT('Ctrl Pts',(69.5171900720158,-11.2657500452716,12.));
#54295=CARTESIAN_POINT('Ctrl Pts',(69.4967809565929,-11.2682114561008,12.));
#54296=CARTESIAN_POINT('Ctrl Pts',(69.4764202659397,-11.270645247528,12.));
#54297=CARTESIAN_POINT('Ctrl Pts',(69.456108179879,-11.2730514806139,12.));
#54298=CARTESIAN_POINT('Ctrl Pts',(69.4358448819967,-11.2754302177021,12.));
#54299=CARTESIAN_POINT('Ctrl Pts',(69.4156305620593,-11.2777815231469,12.));
#54300=CARTESIAN_POINT('Ctrl Pts',(69.3954654162281,-11.2801054633816,12.));
#54301=CARTESIAN_POINT('Ctrl Pts',(69.3753496420039,-11.2824021054045,12.));
#54302=CARTESIAN_POINT('Ctrl Pts',(69.3552834337784,-11.2846715154524,12.));
#54303=CARTESIAN_POINT('Ctrl Pts',(69.3352669789587,-11.2869137578459,12.));
#54304=CARTESIAN_POINT('Ctrl Pts',(69.3153004517783,-11.2891288931517,12.));
#54305=CARTESIAN_POINT('Ctrl Pts',(69.295384019272,-11.2913169799628,12.));
#54306=CARTESIAN_POINT('Ctrl Pts',(69.275517853148,-11.2934780784351,12.));
#54307=CARTESIAN_POINT('Ctrl Pts',(69.255702139335,-11.2956122531375,12.));
#54308=CARTESIAN_POINT('Ctrl Pts',(69.2359370894907,-11.2977195764852,12.));
#54309=CARTESIAN_POINT('Ctrl Pts',(69.2162229488531,-11.2998001310964,12.));
#54310=CARTESIAN_POINT('Ctrl Pts',(69.1965599718914,-11.3018540025638,12.));
#54311=CARTESIAN_POINT('Ctrl Pts',(69.1769483991721,-11.3038812726292,12.));
#54312=CARTESIAN_POINT('Ctrl Pts',(69.1573884361,-11.3058820128307,12.));
#54313=CARTESIAN_POINT('Ctrl Pts',(69.1378802251711,-11.3078562764384,12.));
#54314=CARTESIAN_POINT('Ctrl Pts',(69.118423844466,-11.3098040973713,12.));
#54315=CARTESIAN_POINT('Ctrl Pts',(69.1029002322118,-11.3113412156661,12.));
#54316=CARTESIAN_POINT('Ctrl Pts',(69.0912808656811,-11.3124821678798,12.));
#54317=CARTESIAN_POINT('Ctrl Pts',(69.0835449954396,-11.3132375200165,12.));
#54318=CARTESIAN_POINT('Ctrl Pts',(69.079679653846,-11.3136138754165,12.));
#54319=CARTESIAN_POINT('Ctrl Pts',(73.664078719806,-8.93459554657863,0.));
#54320=CARTESIAN_POINT('Ctrl Pts',(73.664078719806,-8.93459554657863,4.));
#54321=CARTESIAN_POINT('Ctrl Pts',(73.664078719806,-8.93459554657865,8.));
#54322=CARTESIAN_POINT('Ctrl Pts',(73.664078719806,-8.93459554657865,12.));
#54323=CARTESIAN_POINT('Ctrl Pts',(73.7581053903597,-8.99145626777918,0.));
#54324=CARTESIAN_POINT('Ctrl Pts',(73.7581053903597,-8.99145626777918,4.));
#54325=CARTESIAN_POINT('Ctrl Pts',(73.7581053903597,-8.9914562677792,8.00000000000001));
#54326=CARTESIAN_POINT('Ctrl Pts',(73.7581053903597,-8.9914562677792,12.));
#54327=CARTESIAN_POINT('Ctrl Pts',(73.8880618019208,-9.14696952162308,0.));
#54328=CARTESIAN_POINT('Ctrl Pts',(73.8880618019208,-9.14696952162308,4.));
#54329=CARTESIAN_POINT('Ctrl Pts',(73.8880618019208,-9.1469695216231,7.99999999999999));
#54330=CARTESIAN_POINT('Ctrl Pts',(73.8880618019208,-9.1469695216231,12.));
#54331=CARTESIAN_POINT('Ctrl Pts',(73.9117532086772,-9.34395683490516,0.));
#54332=CARTESIAN_POINT('Ctrl Pts',(73.9117532086772,-9.34395683490516,4.));
#54333=CARTESIAN_POINT('Ctrl Pts',(73.9117532086772,-9.34395683490517,8.00000000000001));
#54334=CARTESIAN_POINT('Ctrl Pts',(73.9117532086772,-9.34395683490517,12.));
#54335=CARTESIAN_POINT('Ctrl Pts',(73.9013264985864,-9.4257064323754,0.));
#54336=CARTESIAN_POINT('Ctrl Pts',(73.9013264985864,-9.4257064323754,4.));
#54337=CARTESIAN_POINT('Ctrl Pts',(73.9013264985864,-9.4257064323754,8.));
#54338=CARTESIAN_POINT('Ctrl Pts',(73.9013264985864,-9.4257064323754,12.));
#54339=CARTESIAN_POINT('',(73.664078719806,-8.93459554657863,0.));
#54340=CARTESIAN_POINT('',(73.9013264985865,-9.4257064323754,0.));
#54341=CARTESIAN_POINT('Ctrl Pts',(73.664078719806,-8.93459554657863,6.97125684381022E-35));
#54342=CARTESIAN_POINT('Ctrl Pts',(73.7581053903597,-8.99145626777918,6.97125684381022E-35));
#54343=CARTESIAN_POINT('Ctrl Pts',(73.832366196966,-9.08032098426141,6.97125684381023E-35));
#54344=CARTESIAN_POINT('Ctrl Pts',(73.8719282264933,-9.18272825076427,6.97125684381023E-35));
#54345=CARTESIAN_POINT('Ctrl Pts',(73.9015997486387,-9.25953370064141,6.97125684381022E-35));
#54346=CARTESIAN_POINT('Ctrl Pts',(73.9117532086772,-9.34395683490516,6.97125684381022E-35));
#54347=CARTESIAN_POINT('Ctrl Pts',(73.9013264985864,-9.4257064323754,6.97125684381022E-35));
#54348=CARTESIAN_POINT('',(73.9013264985865,-9.4257064323754,12.));
#54349=CARTESIAN_POINT('Ctrl Pts',(73.9013264985864,-9.4257064323754,0.));
#54350=CARTESIAN_POINT('Ctrl Pts',(73.9013264985864,-9.4257064323754,4.));
#54351=CARTESIAN_POINT('Ctrl Pts',(73.9013264985864,-9.4257064323754,8.));
#54352=CARTESIAN_POINT('Ctrl Pts',(73.9013264985864,-9.4257064323754,12.));
#54353=CARTESIAN_POINT('',(73.664078719806,-8.93459554657865,12.));
#54354=CARTESIAN_POINT('Ctrl Pts',(73.9013264985864,-9.4257064323754,12.));
#54355=CARTESIAN_POINT('Ctrl Pts',(73.9117532086772,-9.34395683490517,12.));
#54356=CARTESIAN_POINT('Ctrl Pts',(73.9015997486387,-9.25953370064143,12.));
#54357=CARTESIAN_POINT('Ctrl Pts',(73.8719282264933,-9.18272825076428,12.));
#54358=CARTESIAN_POINT('Ctrl Pts',(73.832366196966,-9.08032098426143,12.));
#54359=CARTESIAN_POINT('Ctrl Pts',(73.7581053903597,-8.9914562677792,12.));
#54360=CARTESIAN_POINT('Ctrl Pts',(73.664078719806,-8.93459554657865,12.));
#54361=CARTESIAN_POINT('Ctrl Pts',(73.664078719806,-8.93459554657865,12.));
#54362=CARTESIAN_POINT('Ctrl Pts',(73.664078719806,-8.93459554657865,8.));
#54363=CARTESIAN_POINT('Ctrl Pts',(73.664078719806,-8.93459554657863,4.));
#54364=CARTESIAN_POINT('Ctrl Pts',(73.664078719806,-8.93459554657863,0.));
#54365=CARTESIAN_POINT('Origin',(3.71649880366789E-10,-4.88285199465431E-11,
0.));
#54366=CARTESIAN_POINT('Origin',(3.71649880366789E-10,-4.88285199465431E-11,
12.));
#54367=CARTESIAN_POINT('Origin',(3.71649880366789E-10,-4.88285199465431E-11,
0.));
#54368=CARTESIAN_POINT('Ctrl Pts',(72.6683126419592,-16.4184755008033,-5.55111512312578E-16));
#54369=CARTESIAN_POINT('Ctrl Pts',(72.6683126419592,-16.4184755008033,4.));
#54370=CARTESIAN_POINT('Ctrl Pts',(72.6683126419592,-16.4184755008033,8.));
#54371=CARTESIAN_POINT('Ctrl Pts',(72.6683126419592,-16.4184755008033,12.));
#54372=CARTESIAN_POINT('Ctrl Pts',(72.644096499941,-16.5256563519777,-5.55111512312578E-16));
#54373=CARTESIAN_POINT('Ctrl Pts',(72.644096499941,-16.5256563519777,4.));
#54374=CARTESIAN_POINT('Ctrl Pts',(72.644096499941,-16.5256563519777,8.00000000000001));
#54375=CARTESIAN_POINT('Ctrl Pts',(72.644096499941,-16.5256563519777,12.));
#54376=CARTESIAN_POINT('Ctrl Pts',(72.5376471652845,-16.6981133841325,-5.55111512312578E-16));
#54377=CARTESIAN_POINT('Ctrl Pts',(72.5376471652845,-16.6981133841325,4.));
#54378=CARTESIAN_POINT('Ctrl Pts',(72.5376471652845,-16.6981133841324,7.99999999999999));
#54379=CARTESIAN_POINT('Ctrl Pts',(72.5376471652845,-16.6981133841324,12.));
#54380=CARTESIAN_POINT('Ctrl Pts',(72.3582555997247,-16.7828708182973,-5.55111512312578E-16));
#54381=CARTESIAN_POINT('Ctrl Pts',(72.3582555997247,-16.7828708182973,4.));
#54382=CARTESIAN_POINT('Ctrl Pts',(72.3582555997247,-16.7828708182972,8.00000000000001));
#54383=CARTESIAN_POINT('Ctrl Pts',(72.3582555997247,-16.7828708182972,12.));
#54384=CARTESIAN_POINT('Ctrl Pts',(72.2774028393488,-16.7988252568804,-5.55111512312578E-16));
#54385=CARTESIAN_POINT('Ctrl Pts',(72.2774028393488,-16.7988252568804,4.));
#54386=CARTESIAN_POINT('Ctrl Pts',(72.2774028393488,-16.7988252568804,8.));
#54387=CARTESIAN_POINT('Ctrl Pts',(72.2774028393488,-16.7988252568804,12.));
#54388=CARTESIAN_POINT('',(72.6683126419592,-16.4184755008033,2.77555756156289E-16));
#54389=CARTESIAN_POINT('',(72.2774028393488,-16.7988252568806,0.));
#54390=CARTESIAN_POINT('Ctrl Pts',(72.6683126419592,-16.4184755008033,1.02909569064144E-17));
#54391=CARTESIAN_POINT('Ctrl Pts',(72.644096499941,-16.5256563519777,1.02909569064142E-17));
#54392=CARTESIAN_POINT('Ctrl Pts',(72.5832683087087,-16.6242032274947,1.02909569064147E-17));
#54393=CARTESIAN_POINT('Ctrl Pts',(72.4986222461611,-16.6941134995864,1.02909569064145E-17));
#54394=CARTESIAN_POINT('Ctrl Pts',(72.4351376992503,-16.7465462036552,1.02909569064144E-17));
#54395=CARTESIAN_POINT('Ctrl Pts',(72.3582555997247,-16.7828708182973,1.0290956906414E-17));
#54396=CARTESIAN_POINT('Ctrl Pts',(72.2774028393488,-16.7988252568804,1.02909569064144E-17));
#54397=CARTESIAN_POINT('',(72.2774028393489,-16.7988252568806,12.));
#54398=CARTESIAN_POINT('Ctrl Pts',(72.2774028393488,-16.7988252568804,-5.55111512312578E-16));
#54399=CARTESIAN_POINT('Ctrl Pts',(72.2774028393488,-16.7988252568804,4.));
#54400=CARTESIAN_POINT('Ctrl Pts',(72.2774028393488,-16.7988252568804,8.));
#54401=CARTESIAN_POINT('Ctrl Pts',(72.2774028393488,-16.7988252568804,12.));
#54402=CARTESIAN_POINT('',(72.6683126419592,-16.4184755008033,12.));
#54403=CARTESIAN_POINT('Ctrl Pts',(72.2774028393488,-16.7988252568804,12.));
#54404=CARTESIAN_POINT('Ctrl Pts',(72.3582555997247,-16.7828708182972,12.));
#54405=CARTESIAN_POINT('Ctrl Pts',(72.4351376992503,-16.7465462036552,12.));
#54406=CARTESIAN_POINT('Ctrl Pts',(72.4986222461611,-16.6941134995864,12.));
#54407=CARTESIAN_POINT('Ctrl Pts',(72.5832683087087,-16.6242032274947,12.));
#54408=CARTESIAN_POINT('Ctrl Pts',(72.644096499941,-16.5256563519777,12.));
#54409=CARTESIAN_POINT('Ctrl Pts',(72.6683126419592,-16.4184755008033,12.));
#54410=CARTESIAN_POINT('Ctrl Pts',(72.6683126419592,-16.4184755008033,12.));
#54411=CARTESIAN_POINT('Ctrl Pts',(72.6683126419592,-16.4184755008033,8.));
#54412=CARTESIAN_POINT('Ctrl Pts',(72.6683126419592,-16.4184755008033,4.));
#54413=CARTESIAN_POINT('Ctrl Pts',(72.6683126419592,-16.4184755008033,-5.55111512312578E-16));
#54414=CARTESIAN_POINT('Ctrl Pts',(67.8307641965655,-17.2912529479484,0.));
#54415=CARTESIAN_POINT('Ctrl Pts',(67.8307641965655,-17.2912529479484,12.));
#54416=CARTESIAN_POINT('Ctrl Pts',(67.8346476309018,-17.2912149114119,0.));
#54417=CARTESIAN_POINT('Ctrl Pts',(67.8346476309018,-17.2912149114119,12.));
#54418=CARTESIAN_POINT('Ctrl Pts',(67.842419897098,-17.2911366591348,0.));
#54419=CARTESIAN_POINT('Ctrl Pts',(67.842419897098,-17.2911366591348,12.));
#54420=CARTESIAN_POINT('Ctrl Pts',(67.8540944889687,-17.291012743109,0.));
#54421=CARTESIAN_POINT('Ctrl Pts',(67.8540944889687,-17.291012743109,12.));
#54422=CARTESIAN_POINT('Ctrl Pts',(67.8696929978782,-17.2908344459694,0.));
#54423=CARTESIAN_POINT('Ctrl Pts',(67.8696929978782,-17.2908344459694,12.));
#54424=CARTESIAN_POINT('Ctrl Pts',(67.8892451049608,-17.2905897723948,0.));
#54425=CARTESIAN_POINT('Ctrl Pts',(67.8892451049608,-17.2905897723948,12.));
#54426=CARTESIAN_POINT('Ctrl Pts',(67.9088511496686,-17.2903232740694,0.));
#54427=CARTESIAN_POINT('Ctrl Pts',(67.9088511496686,-17.2903232740694,12.));
#54428=CARTESIAN_POINT('Ctrl Pts',(67.9285110571741,-17.2900349103981,0.));
#54429=CARTESIAN_POINT('Ctrl Pts',(67.9285110571741,-17.2900349103981,12.));
#54430=CARTESIAN_POINT('Ctrl Pts',(67.9482246901667,-17.2897246158941,0.));
#54431=CARTESIAN_POINT('Ctrl Pts',(67.9482246901667,-17.2897246158941,12.));
#54432=CARTESIAN_POINT('Ctrl Pts',(67.9679918502579,-17.2893923013894,0.));
#54433=CARTESIAN_POINT('Ctrl Pts',(67.9679918502579,-17.2893923013894,12.));
#54434=CARTESIAN_POINT('Ctrl Pts',(67.987812304921,-17.2890378644866,0.));
#54435=CARTESIAN_POINT('Ctrl Pts',(67.987812304921,-17.2890378644866,12.));
#54436=CARTESIAN_POINT('Ctrl Pts',(68.007685808115,-17.28866119774,0.));
#54437=CARTESIAN_POINT('Ctrl Pts',(68.007685808115,-17.28866119774,12.));
#54438=CARTESIAN_POINT('Ctrl Pts',(68.0276121227356,-17.2882621974721,0.));
#54439=CARTESIAN_POINT('Ctrl Pts',(68.0276121227356,-17.2882621974721,12.));
#54440=CARTESIAN_POINT('Ctrl Pts',(68.0475910442424,-17.2878407730961,0.));
#54441=CARTESIAN_POINT('Ctrl Pts',(68.0475910442424,-17.2878407730961,12.));
#54442=CARTESIAN_POINT('Ctrl Pts',(68.0676223930412,-17.2873968440839,0.));
#54443=CARTESIAN_POINT('Ctrl Pts',(68.0676223930412,-17.2873968440839,12.));
#54444=CARTESIAN_POINT('Ctrl Pts',(68.0877060033205,-17.2869303355432,0.));
#54445=CARTESIAN_POINT('Ctrl Pts',(68.0877060033205,-17.2869303355432,12.));
#54446=CARTESIAN_POINT('Ctrl Pts',(68.1078417137877,-17.2864411745459,0.));
#54447=CARTESIAN_POINT('Ctrl Pts',(68.1078417137877,-17.2864411745459,12.));
#54448=CARTESIAN_POINT('Ctrl Pts',(68.1280293561511,-17.2859292855705,0.));
#54449=CARTESIAN_POINT('Ctrl Pts',(68.1280293561511,-17.2859292855705,12.));
#54450=CARTESIAN_POINT('Ctrl Pts',(68.1482687493226,-17.2853945882072,0.));
#54451=CARTESIAN_POINT('Ctrl Pts',(68.1482687493226,-17.2853945882072,12.));
#54452=CARTESIAN_POINT('Ctrl Pts',(68.1685597054232,-17.2848369995293,0.));
#54453=CARTESIAN_POINT('Ctrl Pts',(68.1685597054232,-17.2848369995293,12.));
#54454=CARTESIAN_POINT('Ctrl Pts',(68.1889020335427,-17.2842564355799,0.));
#54455=CARTESIAN_POINT('Ctrl Pts',(68.1889020335427,-17.2842564355799,12.));
#54456=CARTESIAN_POINT('Ctrl Pts',(68.2092955440567,-17.2836528130819,0.));
#54457=CARTESIAN_POINT('Ctrl Pts',(68.2092955440567,-17.2836528130819,12.));
#54458=CARTESIAN_POINT('Ctrl Pts',(68.2297400535294,-17.2830260513867,0.));
#54459=CARTESIAN_POINT('Ctrl Pts',(68.2297400535294,-17.2830260513867,12.));
#54460=CARTESIAN_POINT('Ctrl Pts',(68.2502353845071,-17.2823760723874,0.));
#54461=CARTESIAN_POINT('Ctrl Pts',(68.2502353845071,-17.2823760723874,12.));
#54462=CARTESIAN_POINT('Ctrl Pts',(68.2707813631731,-17.2817027995831,0.));
#54463=CARTESIAN_POINT('Ctrl Pts',(68.2707813631731,-17.2817027995831,12.));
#54464=CARTESIAN_POINT('Ctrl Pts',(68.2913778177261,-17.2810061574353,0.));
#54465=CARTESIAN_POINT('Ctrl Pts',(68.2913778177261,-17.2810061574353,12.));
#54466=CARTESIAN_POINT('Ctrl Pts',(68.3120245763914,-17.2802860705815,0.));
#54467=CARTESIAN_POINT('Ctrl Pts',(68.3120245763914,-17.2802860705815,12.));
#54468=CARTESIAN_POINT('Ctrl Pts',(68.3327214657575,-17.2795424631799,0.));
#54469=CARTESIAN_POINT('Ctrl Pts',(68.3327214657575,-17.2795424631799,12.));
#54470=CARTESIAN_POINT('Ctrl Pts',(68.3534683116515,-17.2787752592484,0.));
#54471=CARTESIAN_POINT('Ctrl Pts',(68.3534683116515,-17.2787752592484,12.));
#54472=CARTESIAN_POINT('Ctrl Pts',(68.3742649398964,-17.2779843829608,0.));
#54473=CARTESIAN_POINT('Ctrl Pts',(68.3742649398964,-17.2779843829608,12.));
#54474=CARTESIAN_POINT('Ctrl Pts',(68.3951111770487,-17.2771697589384,0.));
#54475=CARTESIAN_POINT('Ctrl Pts',(68.3951111770487,-17.2771697589384,12.));
#54476=CARTESIAN_POINT('Ctrl Pts',(68.4160068512753,-17.2763313126018,0.));
#54477=CARTESIAN_POINT('Ctrl Pts',(68.4160068512753,-17.2763313126018,12.));
#54478=CARTESIAN_POINT('Ctrl Pts',(68.436951792677,-17.2754689702992,0.));
#54479=CARTESIAN_POINT('Ctrl Pts',(68.436951792677,-17.2754689702992,12.));
#54480=CARTESIAN_POINT('Ctrl Pts',(68.4579458328185,-17.2745826591119,0.));
#54481=CARTESIAN_POINT('Ctrl Pts',(68.4579458328185,-17.2745826591119,12.));
#54482=CARTESIAN_POINT('Ctrl Pts',(68.4789888044351,-17.2736723067365,0.));
#54483=CARTESIAN_POINT('Ctrl Pts',(68.4789888044351,-17.2736723067365,12.));
#54484=CARTESIAN_POINT('Ctrl Pts',(68.5000805410911,-17.2727378413489,0.));
#54485=CARTESIAN_POINT('Ctrl Pts',(68.5000805410911,-17.2727378413489,12.));
#54486=CARTESIAN_POINT('Ctrl Pts',(68.521220876786,-17.2717791914544,0.));
#54487=CARTESIAN_POINT('Ctrl Pts',(68.521220876786,-17.2717791914544,12.));
#54488=CARTESIAN_POINT('Ctrl Pts',(68.5424096459772,-17.2707962858919,0.));
#54489=CARTESIAN_POINT('Ctrl Pts',(68.5424096459772,-17.2707962858919,12.));
#54490=CARTESIAN_POINT('Ctrl Pts',(68.5636466837517,-17.269789053896,0.));
#54491=CARTESIAN_POINT('Ctrl Pts',(68.5636466837517,-17.269789053896,12.));
#54492=CARTESIAN_POINT('Ctrl Pts',(68.5849318259449,-17.2687574251428,0.));
#54493=CARTESIAN_POINT('Ctrl Pts',(68.5849318259449,-17.2687574251428,12.));
#54494=CARTESIAN_POINT('Ctrl Pts',(68.6062649092764,-17.2677013298057,0.));
#54495=CARTESIAN_POINT('Ctrl Pts',(68.6062649092764,-17.2677013298057,12.));
#54496=CARTESIAN_POINT('Ctrl Pts',(68.6276457714729,-17.2666206986084,0.));
#54497=CARTESIAN_POINT('Ctrl Pts',(68.6276457714729,-17.2666206986084,12.));
#54498=CARTESIAN_POINT('Ctrl Pts',(68.6490742512057,-17.2655154627928,0.));
#54499=CARTESIAN_POINT('Ctrl Pts',(68.6490742512057,-17.2655154627928,12.));
#54500=CARTESIAN_POINT('Ctrl Pts',(68.6705501880249,-17.2643855540892,0.));
#54501=CARTESIAN_POINT('Ctrl Pts',(68.6705501880249,-17.2643855540892,12.));
#54502=CARTESIAN_POINT('Ctrl Pts',(68.6920734222938,-17.2632309046892,0.));
#54503=CARTESIAN_POINT('Ctrl Pts',(68.6920734222938,-17.2632309046892,12.));
#54504=CARTESIAN_POINT('Ctrl Pts',(68.7136437951097,-17.2620514472182,0.));
#54505=CARTESIAN_POINT('Ctrl Pts',(68.7136437951097,-17.2620514472182,12.));
#54506=CARTESIAN_POINT('Ctrl Pts',(68.7352611482547,-17.2608471147185,0.));
#54507=CARTESIAN_POINT('Ctrl Pts',(68.7352611482547,-17.2608471147185,12.));
#54508=CARTESIAN_POINT('Ctrl Pts',(68.7569253242333,-17.259617840655,0.));
#54509=CARTESIAN_POINT('Ctrl Pts',(68.7569253242333,-17.259617840655,12.));
#54510=CARTESIAN_POINT('Ctrl Pts',(68.7786361662882,-17.2583635589198,0.));
#54511=CARTESIAN_POINT('Ctrl Pts',(68.7786361662882,-17.2583635589198,12.));
#54512=CARTESIAN_POINT('Ctrl Pts',(68.8003935184184,-17.2570842038383,0.));
#54513=CARTESIAN_POINT('Ctrl Pts',(68.8003935184184,-17.2570842038383,12.));
#54514=CARTESIAN_POINT('Ctrl Pts',(68.8221972253941,-17.2557797101812,0.));
#54515=CARTESIAN_POINT('Ctrl Pts',(68.8221972253941,-17.2557797101812,12.));
#54516=CARTESIAN_POINT('Ctrl Pts',(68.844047132755,-17.2544500131624,0.));
#54517=CARTESIAN_POINT('Ctrl Pts',(68.844047132755,-17.2544500131624,12.));
#54518=CARTESIAN_POINT('Ctrl Pts',(68.8659430867972,-17.2530950484258,0.));
#54519=CARTESIAN_POINT('Ctrl Pts',(68.8659430867972,-17.2530950484258,12.));
#54520=CARTESIAN_POINT('Ctrl Pts',(68.8878849345557,-17.2517147520376,0.));
#54521=CARTESIAN_POINT('Ctrl Pts',(68.8878849345557,-17.2517147520376,12.));
#54522=CARTESIAN_POINT('Ctrl Pts',(68.909872523787,-17.2503090604792,0.));
#54523=CARTESIAN_POINT('Ctrl Pts',(68.909872523787,-17.2503090604792,12.));
#54524=CARTESIAN_POINT('Ctrl Pts',(68.9319057029409,-17.248877910643,0.));
#54525=CARTESIAN_POINT('Ctrl Pts',(68.9319057029409,-17.248877910643,12.));
#54526=CARTESIAN_POINT('Ctrl Pts',(68.9539843211619,-17.2474212398275,0.));
#54527=CARTESIAN_POINT('Ctrl Pts',(68.9539843211619,-17.2474212398275,12.));
#54528=CARTESIAN_POINT('Ctrl Pts',(68.9761082282922,-17.2459389857327,0.));
#54529=CARTESIAN_POINT('Ctrl Pts',(68.9761082282922,-17.2459389857327,12.));
#54530=CARTESIAN_POINT('Ctrl Pts',(68.9982772748694,-17.2444310864585,0.));
#54531=CARTESIAN_POINT('Ctrl Pts',(68.9982772748694,-17.2444310864585,12.));
#54532=CARTESIAN_POINT('Ctrl Pts',(69.0204913121225,-17.2428974805044,0.));
#54533=CARTESIAN_POINT('Ctrl Pts',(69.0204913121225,-17.2428974805044,12.));
#54534=CARTESIAN_POINT('Ctrl Pts',(69.0427501919636,-17.2413381067723,0.));
#54535=CARTESIAN_POINT('Ctrl Pts',(69.0427501919636,-17.2413381067723,12.));
#54536=CARTESIAN_POINT('Ctrl Pts',(69.065053766986,-17.2397529045589,0.));
#54537=CARTESIAN_POINT('Ctrl Pts',(69.065053766986,-17.2397529045589,12.));
#54538=CARTESIAN_POINT('Ctrl Pts',(69.0874018904599,-17.2381418135491,0.));
#54539=CARTESIAN_POINT('Ctrl Pts',(69.0874018904599,-17.2381418135491,12.));
#54540=CARTESIAN_POINT('Ctrl Pts',(69.1097944163245,-17.2365047738125,0.));
#54541=CARTESIAN_POINT('Ctrl Pts',(69.1097944163245,-17.2365047738125,12.));
#54542=CARTESIAN_POINT('Ctrl Pts',(69.1322311991752,-17.2348417258015,0.));
#54543=CARTESIAN_POINT('Ctrl Pts',(69.1322311991752,-17.2348417258015,12.));
#54544=CARTESIAN_POINT('Ctrl Pts',(69.1547120942527,-17.2331526103506,0.));
#54545=CARTESIAN_POINT('Ctrl Pts',(69.1547120942527,-17.2331526103506,12.));
#54546=CARTESIAN_POINT('Ctrl Pts',(69.1772369574447,-17.23143736867,0.));
#54547=CARTESIAN_POINT('Ctrl Pts',(69.1772369574447,-17.23143736867,12.));
#54548=CARTESIAN_POINT('Ctrl Pts',(69.1998056452828,-17.2296959423407,0.));
#54549=CARTESIAN_POINT('Ctrl Pts',(69.1998056452828,-17.2296959423407,12.));
#54550=CARTESIAN_POINT('Ctrl Pts',(69.222418014938,-17.227928273312,0.));
#54551=CARTESIAN_POINT('Ctrl Pts',(69.222418014938,-17.227928273312,12.));
#54552=CARTESIAN_POINT('Ctrl Pts',(69.2450739242109,-17.226134303902,0.));
#54553=CARTESIAN_POINT('Ctrl Pts',(69.2450739242109,-17.226134303902,12.));
#54554=CARTESIAN_POINT('Ctrl Pts',(69.2677732315224,-17.224313976797,0.));
#54555=CARTESIAN_POINT('Ctrl Pts',(69.2677732315224,-17.224313976797,12.));
#54556=CARTESIAN_POINT('Ctrl Pts',(69.2905157959166,-17.2224672350438,0.));
#54557=CARTESIAN_POINT('Ctrl Pts',(69.2905157959166,-17.2224672350438,12.));
#54558=CARTESIAN_POINT('Ctrl Pts',(69.3133014770555,-17.2205940220459,0.));
#54559=CARTESIAN_POINT('Ctrl Pts',(69.3133014770555,-17.2205940220459,12.));
#54560=CARTESIAN_POINT('Ctrl Pts',(69.3361301352141,-17.2186942815602,0.));
#54561=CARTESIAN_POINT('Ctrl Pts',(69.3361301352141,-17.2186942815602,12.));
#54562=CARTESIAN_POINT('Ctrl Pts',(69.3590016312692,-17.2167679576984,0.));
#54563=CARTESIAN_POINT('Ctrl Pts',(69.3590016312692,-17.2167679576984,12.));
#54564=CARTESIAN_POINT('Ctrl Pts',(69.3819158266916,-17.2148149949252,0.));
#54565=CARTESIAN_POINT('Ctrl Pts',(69.3819158266916,-17.2148149949252,12.));
#54566=CARTESIAN_POINT('Ctrl Pts',(69.404872583548,-17.2128353380502,0.));
#54567=CARTESIAN_POINT('Ctrl Pts',(69.404872583548,-17.2128353380502,12.));
#54568=CARTESIAN_POINT('Ctrl Pts',(69.4278717644973,-17.2108289322254,0.));
#54569=CARTESIAN_POINT('Ctrl Pts',(69.4278717644973,-17.2108289322254,12.));
#54570=CARTESIAN_POINT('Ctrl Pts',(69.450913232785,-17.2087957229423,0.));
#54571=CARTESIAN_POINT('Ctrl Pts',(69.450913232785,-17.2087957229423,12.));
#54572=CARTESIAN_POINT('Ctrl Pts',(69.4739968522313,-17.2067356560336,0.));
#54573=CARTESIAN_POINT('Ctrl Pts',(69.4739968522313,-17.2067356560336,12.));
#54574=CARTESIAN_POINT('Ctrl Pts',(69.4971224872269,-17.2046486776708,0.));
#54575=CARTESIAN_POINT('Ctrl Pts',(69.4971224872269,-17.2046486776708,12.));
#54576=CARTESIAN_POINT('Ctrl Pts',(69.5202900027367,-17.2025347343577,0.));
#54577=CARTESIAN_POINT('Ctrl Pts',(69.5202900027367,-17.2025347343577,12.));
#54578=CARTESIAN_POINT('Ctrl Pts',(69.5434992642944,-17.2003937729268,0.));
#54579=CARTESIAN_POINT('Ctrl Pts',(69.5434992642944,-17.2003937729268,12.));
#54580=CARTESIAN_POINT('Ctrl Pts',(69.5667501379969,-17.1982257405377,0.));
#54581=CARTESIAN_POINT('Ctrl Pts',(69.5667501379969,-17.1982257405377,12.));
#54582=CARTESIAN_POINT('Ctrl Pts',(69.5900424904921,-17.196030584678,0.));
#54583=CARTESIAN_POINT('Ctrl Pts',(69.5900424904921,-17.196030584678,12.));
#54584=CARTESIAN_POINT('Ctrl Pts',(69.6133761889749,-17.1938082531612,0.));
#54585=CARTESIAN_POINT('Ctrl Pts',(69.6133761889749,-17.1938082531612,12.));
#54586=CARTESIAN_POINT('Ctrl Pts',(69.6367511011898,-17.1915586941192,0.));
#54587=CARTESIAN_POINT('Ctrl Pts',(69.6367511011898,-17.1915586941192,12.));
#54588=CARTESIAN_POINT('Ctrl Pts',(69.6601670954269,-17.1892818560002,0.));
#54589=CARTESIAN_POINT('Ctrl Pts',(69.6601670954269,-17.1892818560002,12.));
#54590=CARTESIAN_POINT('Ctrl Pts',(69.6836240405164,-17.1869776875666,0.));
#54591=CARTESIAN_POINT('Ctrl Pts',(69.6836240405164,-17.1869776875666,12.));
#54592=CARTESIAN_POINT('Ctrl Pts',(69.7071218058178,-17.1846461378973,0.));
#54593=CARTESIAN_POINT('Ctrl Pts',(69.7071218058178,-17.1846461378973,12.));
#54594=CARTESIAN_POINT('Ctrl Pts',(69.7306602612155,-17.1822871563842,0.));
#54595=CARTESIAN_POINT('Ctrl Pts',(69.7306602612155,-17.1822871563842,12.));
#54596=CARTESIAN_POINT('Ctrl Pts',(69.7542392771234,-17.179900692726,0.));
#54597=CARTESIAN_POINT('Ctrl Pts',(69.7542392771234,-17.179900692726,12.));
#54598=CARTESIAN_POINT('Ctrl Pts',(69.777858724479,-17.1774866969256,0.));
#54599=CARTESIAN_POINT('Ctrl Pts',(69.777858724479,-17.1774866969256,12.));
#54600=CARTESIAN_POINT('Ctrl Pts',(69.8015184747398,-17.1750451192885,0.));
#54601=CARTESIAN_POINT('Ctrl Pts',(69.8015184747398,-17.1750451192885,12.));
#54602=CARTESIAN_POINT('Ctrl Pts',(69.8252183998702,-17.1725759104252,0.));
#54603=CARTESIAN_POINT('Ctrl Pts',(69.8252183998702,-17.1725759104252,12.));
#54604=CARTESIAN_POINT('Ctrl Pts',(69.8489583723407,-17.1700790212473,0.));
#54605=CARTESIAN_POINT('Ctrl Pts',(69.8489583723407,-17.1700790212473,12.));
#54606=CARTESIAN_POINT('Ctrl Pts',(69.8727382651286,-17.167554402962,0.));
#54607=CARTESIAN_POINT('Ctrl Pts',(69.8727382651286,-17.167554402962,12.));
#54608=CARTESIAN_POINT('Ctrl Pts',(69.8965579517147,-17.1650020070686,0.));
#54609=CARTESIAN_POINT('Ctrl Pts',(69.8965579517147,-17.1650020070686,12.));
#54610=CARTESIAN_POINT('Ctrl Pts',(69.9204173060781,-17.1624217853578,0.));
#54611=CARTESIAN_POINT('Ctrl Pts',(69.9204173060781,-17.1624217853578,12.));
#54612=CARTESIAN_POINT('Ctrl Pts',(69.9443162026865,-17.1598136899144,0.));
#54613=CARTESIAN_POINT('Ctrl Pts',(69.9443162026865,-17.1598136899144,12.));
#54614=CARTESIAN_POINT('Ctrl Pts',(69.9682545164939,-17.157177673114,0.));
#54615=CARTESIAN_POINT('Ctrl Pts',(69.9682545164939,-17.157177673114,12.));
#54616=CARTESIAN_POINT('Ctrl Pts',(69.9922321229424,-17.154513687616,0.));
#54617=CARTESIAN_POINT('Ctrl Pts',(69.9922321229424,-17.154513687616,12.));
#54618=CARTESIAN_POINT('Ctrl Pts',(70.0162488979584,-17.1518216863623,0.));
#54619=CARTESIAN_POINT('Ctrl Pts',(70.0162488979584,-17.1518216863623,12.));
#54620=CARTESIAN_POINT('Ctrl Pts',(70.0403047179483,-17.1491016225749,0.));
#54621=CARTESIAN_POINT('Ctrl Pts',(70.0403047179483,-17.1491016225749,12.));
#54622=CARTESIAN_POINT('Ctrl Pts',(70.0643994597873,-17.1463534497594,0.));
#54623=CARTESIAN_POINT('Ctrl Pts',(70.0643994597873,-17.1463534497594,12.));
#54624=CARTESIAN_POINT('Ctrl Pts',(70.0885330008179,-17.1435771217018,0.));
#54625=CARTESIAN_POINT('Ctrl Pts',(70.0885330008179,-17.1435771217018,12.));
#54626=CARTESIAN_POINT('Ctrl Pts',(70.1127052188522,-17.1407725924617,0.));
#54627=CARTESIAN_POINT('Ctrl Pts',(70.1127052188522,-17.1407725924617,12.));
#54628=CARTESIAN_POINT('Ctrl Pts',(70.1369159921687,-17.1379398163709,0.));
#54629=CARTESIAN_POINT('Ctrl Pts',(70.1369159921687,-17.1379398163709,12.));
#54630=CARTESIAN_POINT('Ctrl Pts',(70.1611651995083,-17.1350787480312,0.));
#54631=CARTESIAN_POINT('Ctrl Pts',(70.1611651995083,-17.1350787480312,12.));
#54632=CARTESIAN_POINT('Ctrl Pts',(70.1854527200631,-17.1321893423182,0.));
#54633=CARTESIAN_POINT('Ctrl Pts',(70.1854527200631,-17.1321893423182,12.));
#54634=CARTESIAN_POINT('Ctrl Pts',(70.2097784334747,-17.1292715543778,0.));
#54635=CARTESIAN_POINT('Ctrl Pts',(70.2097784334747,-17.1292715543778,12.));
#54636=CARTESIAN_POINT('Ctrl Pts',(70.2341422198363,-17.1263253396202,0.));
#54637=CARTESIAN_POINT('Ctrl Pts',(70.2341422198363,-17.1263253396202,12.));
#54638=CARTESIAN_POINT('Ctrl Pts',(70.2585439596901,-17.1233506537176,0.));
#54639=CARTESIAN_POINT('Ctrl Pts',(70.2585439596901,-17.1233506537176,12.));
#54640=CARTESIAN_POINT('Ctrl Pts',(70.2829835340238,-17.1203474526031,0.));
#54641=CARTESIAN_POINT('Ctrl Pts',(70.2829835340238,-17.1203474526031,12.));
#54642=CARTESIAN_POINT('Ctrl Pts',(70.3074608242608,-17.1173156924733,0.));
#54643=CARTESIAN_POINT('Ctrl Pts',(70.3074608242608,-17.1173156924733,12.));
#54644=CARTESIAN_POINT('Ctrl Pts',(70.3319757122568,-17.1142553297867,0.));
#54645=CARTESIAN_POINT('Ctrl Pts',(70.3319757122568,-17.1142553297867,12.));
#54646=CARTESIAN_POINT('Ctrl Pts',(70.3565280803022,-17.1111663212568,0.));
#54647=CARTESIAN_POINT('Ctrl Pts',(70.3565280803022,-17.1111663212568,12.));
#54648=CARTESIAN_POINT('Ctrl Pts',(70.3811178111201,-17.1080486238499,0.));
#54649=CARTESIAN_POINT('Ctrl Pts',(70.3811178111201,-17.1080486238499,12.));
#54650=CARTESIAN_POINT('Ctrl Pts',(70.4057447878624,-17.1049021947834,0.));
#54651=CARTESIAN_POINT('Ctrl Pts',(70.4057447878624,-17.1049021947834,12.));
#54652=CARTESIAN_POINT('Ctrl Pts',(70.430408894101,-17.1017269915292,0.));
#54653=CARTESIAN_POINT('Ctrl Pts',(70.430408894101,-17.1017269915292,12.));
#54654=CARTESIAN_POINT('Ctrl Pts',(70.4551100138238,-17.0985229718124,0.));
#54655=CARTESIAN_POINT('Ctrl Pts',(70.4551100138238,-17.0985229718124,12.));
#54656=CARTESIAN_POINT('Ctrl Pts',(70.4798480314381,-17.0952900936048,0.));
#54657=CARTESIAN_POINT('Ctrl Pts',(70.4798480314381,-17.0952900936048,12.));
#54658=CARTESIAN_POINT('Ctrl Pts',(70.5046228317677,-17.0920283151219,0.));
#54659=CARTESIAN_POINT('Ctrl Pts',(70.5046228317677,-17.0920283151219,12.));
#54660=CARTESIAN_POINT('Ctrl Pts',(70.5294343000513,-17.088737594822,0.));
#54661=CARTESIAN_POINT('Ctrl Pts',(70.5294343000513,-17.088737594822,12.));
#54662=CARTESIAN_POINT('Ctrl Pts',(70.5542823219331,-17.0854178914087,0.));
#54663=CARTESIAN_POINT('Ctrl Pts',(70.5542823219331,-17.0854178914087,12.));
#54664=CARTESIAN_POINT('Ctrl Pts',(70.5791667834582,-17.082069163831,0.));
#54665=CARTESIAN_POINT('Ctrl Pts',(70.5791667834582,-17.082069163831,12.));
#54666=CARTESIAN_POINT('Ctrl Pts',(70.6040875710749,-17.0786913712763,0.));
#54667=CARTESIAN_POINT('Ctrl Pts',(70.6040875710749,-17.0786913712763,12.));
#54668=CARTESIAN_POINT('Ctrl Pts',(70.6290445716337,-17.0752844731678,0.));
#54669=CARTESIAN_POINT('Ctrl Pts',(70.6290445716337,-17.0752844731678,12.));
#54670=CARTESIAN_POINT('Ctrl Pts',(70.6540376723841,-17.0718484291624,0.));
#54671=CARTESIAN_POINT('Ctrl Pts',(70.6540376723841,-17.0718484291624,12.));
#54672=CARTESIAN_POINT('Ctrl Pts',(70.6790667609679,-17.0683831991532,0.));
#54673=CARTESIAN_POINT('Ctrl Pts',(70.6790667609679,-17.0683831991532,12.));
#54674=CARTESIAN_POINT('Ctrl Pts',(70.7041317254125,-17.0648887432713,0.));
#54675=CARTESIAN_POINT('Ctrl Pts',(70.7041317254125,-17.0648887432713,12.));
#54676=CARTESIAN_POINT('Ctrl Pts',(70.7292324541341,-17.0613650218787,0.));
#54677=CARTESIAN_POINT('Ctrl Pts',(70.7292324541341,-17.0613650218787,12.));
#54678=CARTESIAN_POINT('Ctrl Pts',(70.7543688359374,-17.0578119955649,0.));
#54679=CARTESIAN_POINT('Ctrl Pts',(70.7543688359374,-17.0578119955649,12.));
#54680=CARTESIAN_POINT('Ctrl Pts',(70.7795407600127,-17.0542296251462,0.));
#54681=CARTESIAN_POINT('Ctrl Pts',(70.7795407600127,-17.0542296251462,12.));
#54682=CARTESIAN_POINT('Ctrl Pts',(70.8047481159306,-17.0506178716664,0.));
#54683=CARTESIAN_POINT('Ctrl Pts',(70.8047481159306,-17.0506178716664,12.));
#54684=CARTESIAN_POINT('Ctrl Pts',(70.8299907936346,-17.0469766964005,0.));
#54685=CARTESIAN_POINT('Ctrl Pts',(70.8299907936346,-17.0469766964005,12.));
#54686=CARTESIAN_POINT('Ctrl Pts',(70.8552686834435,-17.0433060608478,0.));
#54687=CARTESIAN_POINT('Ctrl Pts',(70.8552686834435,-17.0433060608478,12.));
#54688=CARTESIAN_POINT('Ctrl Pts',(70.8805816760507,-17.0396059267279,0.));
#54689=CARTESIAN_POINT('Ctrl Pts',(70.8805816760507,-17.0396059267279,12.));
#54690=CARTESIAN_POINT('Ctrl Pts',(70.9059296625214,-17.0358762559786,0.));
#54691=CARTESIAN_POINT('Ctrl Pts',(70.9059296625214,-17.0358762559786,12.));
#54692=CARTESIAN_POINT('Ctrl Pts',(70.9313125342872,-17.0321170107562,0.));
#54693=CARTESIAN_POINT('Ctrl Pts',(70.9313125342872,-17.0321170107562,12.));
#54694=CARTESIAN_POINT('Ctrl Pts',(70.9567301831355,-17.028328153439,0.));
#54695=CARTESIAN_POINT('Ctrl Pts',(70.9567301831355,-17.028328153439,12.));
#54696=CARTESIAN_POINT('Ctrl Pts',(70.9821825012134,-17.0245096466228,0.));
#54697=CARTESIAN_POINT('Ctrl Pts',(70.9821825012134,-17.0245096466228,12.));
#54698=CARTESIAN_POINT('Ctrl Pts',(71.0076693810303,-17.0206614531165,0.));
#54699=CARTESIAN_POINT('Ctrl Pts',(71.0076693810303,-17.0206614531165,12.));
#54700=CARTESIAN_POINT('Ctrl Pts',(71.0331907154575,-17.0167835359419,0.));
#54701=CARTESIAN_POINT('Ctrl Pts',(71.0331907154575,-17.0167835359419,12.));
#54702=CARTESIAN_POINT('Ctrl Pts',(71.0587463977266,-17.0128758583335,0.));
#54703=CARTESIAN_POINT('Ctrl Pts',(71.0587463977266,-17.0128758583335,12.));
#54704=CARTESIAN_POINT('Ctrl Pts',(71.0843363214216,-17.0089383837437,0.));
#54705=CARTESIAN_POINT('Ctrl Pts',(71.0843363214216,-17.0089383837437,12.));
#54706=CARTESIAN_POINT('Ctrl Pts',(71.1099603804779,-17.0049710758393,0.));
#54707=CARTESIAN_POINT('Ctrl Pts',(71.1099603804779,-17.0049710758393,12.));
#54708=CARTESIAN_POINT('Ctrl Pts',(71.1356184691799,-17.0009738984935,0.));
#54709=CARTESIAN_POINT('Ctrl Pts',(71.1356184691799,-17.0009738984935,12.));
#54710=CARTESIAN_POINT('Ctrl Pts',(71.1613104821565,-16.9969468157824,0.));
#54711=CARTESIAN_POINT('Ctrl Pts',(71.1613104821565,-16.9969468157824,12.));
#54712=CARTESIAN_POINT('Ctrl Pts',(71.1870363143742,-16.9928897919829,0.));
#54713=CARTESIAN_POINT('Ctrl Pts',(71.1870363143742,-16.9928897919829,12.));
#54714=CARTESIAN_POINT('Ctrl Pts',(71.2127958611248,-16.9888027915743,0.));
#54715=CARTESIAN_POINT('Ctrl Pts',(71.2127958611248,-16.9888027915743,12.));
#54716=CARTESIAN_POINT('Ctrl Pts',(71.2385890180233,-16.9846857792385,0.));
#54717=CARTESIAN_POINT('Ctrl Pts',(71.2385890180233,-16.9846857792385,12.));
#54718=CARTESIAN_POINT('Ctrl Pts',(71.2644156810209,-16.9805387198573,0.));
#54719=CARTESIAN_POINT('Ctrl Pts',(71.2644156810209,-16.9805387198573,12.));
#54720=CARTESIAN_POINT('Ctrl Pts',(71.2902757464127,-16.9763615785138,0.));
#54721=CARTESIAN_POINT('Ctrl Pts',(71.2902757464127,-16.9763615785138,12.));
#54722=CARTESIAN_POINT('Ctrl Pts',(71.3161691108425,-16.9721543204951,0.));
#54723=CARTESIAN_POINT('Ctrl Pts',(71.3161691108425,-16.9721543204951,12.));
#54724=CARTESIAN_POINT('Ctrl Pts',(71.3420956713072,-16.9679169112993,0.));
#54725=CARTESIAN_POINT('Ctrl Pts',(71.3420956713072,-16.9679169112993,12.));
#54726=CARTESIAN_POINT('Ctrl Pts',(71.3680553251548,-16.9636493166395,0.));
#54727=CARTESIAN_POINT('Ctrl Pts',(71.3680553251548,-16.9636493166395,12.));
#54728=CARTESIAN_POINT('Ctrl Pts',(71.3940479700663,-16.9593515024274,0.));
#54729=CARTESIAN_POINT('Ctrl Pts',(71.3940479700663,-16.9593515024274,12.));
#54730=CARTESIAN_POINT('Ctrl Pts',(71.4200735040374,-16.9550234347619,0.));
#54731=CARTESIAN_POINT('Ctrl Pts',(71.4200735040374,-16.9550234347619,12.));
#54732=CARTESIAN_POINT('Ctrl Pts',(71.4461318253561,-16.9506650799188,0.));
#54733=CARTESIAN_POINT('Ctrl Pts',(71.4461318253561,-16.9506650799188,12.));
#54734=CARTESIAN_POINT('Ctrl Pts',(71.4722228325805,-16.9462764043445,0.));
#54735=CARTESIAN_POINT('Ctrl Pts',(71.4722228325805,-16.9462764043445,12.));
#54736=CARTESIAN_POINT('Ctrl Pts',(71.498346424507,-16.9418573746492,0.));
#54737=CARTESIAN_POINT('Ctrl Pts',(71.498346424507,-16.9418573746492,12.));
#54738=CARTESIAN_POINT('Ctrl Pts',(71.5245025002154,-16.9374079576204,0.));
#54739=CARTESIAN_POINT('Ctrl Pts',(71.5245025002154,-16.9374079576204,12.));
#54740=CARTESIAN_POINT('Ctrl Pts',(71.5506909591139,-16.9329281202379,0.));
#54741=CARTESIAN_POINT('Ctrl Pts',(71.5506909591139,-16.9329281202379,12.));
#54742=CARTESIAN_POINT('Ctrl Pts',(71.5769117009844,-16.9284178296934,0.));
#54743=CARTESIAN_POINT('Ctrl Pts',(71.5769117009844,-16.9284178296934,12.));
#54744=CARTESIAN_POINT('Ctrl Pts',(71.6031646260169,-16.923877053407,0.));
#54745=CARTESIAN_POINT('Ctrl Pts',(71.6031646260169,-16.923877053407,12.));
#54746=CARTESIAN_POINT('Ctrl Pts',(71.6294496348644,-16.9193057590605,0.));
#54747=CARTESIAN_POINT('Ctrl Pts',(71.6294496348644,-16.9193057590605,12.));
#54748=CARTESIAN_POINT('Ctrl Pts',(71.6557666285908,-16.9147039145715,0.));
#54749=CARTESIAN_POINT('Ctrl Pts',(71.6557666285908,-16.9147039145715,12.));
#54750=CARTESIAN_POINT('Ctrl Pts',(71.6821155085605,-16.9100714880367,0.));
#54751=CARTESIAN_POINT('Ctrl Pts',(71.6821155085605,-16.9100714880367,12.));
#54752=CARTESIAN_POINT('Ctrl Pts',(71.7084961763355,-16.9054084476847,0.));
#54753=CARTESIAN_POINT('Ctrl Pts',(71.7084961763355,-16.9054084476847,12.));
#54754=CARTESIAN_POINT('Ctrl Pts',(71.7349085335796,-16.9007147618344,0.));
#54755=CARTESIAN_POINT('Ctrl Pts',(71.7349085335796,-16.9007147618344,12.));
#54756=CARTESIAN_POINT('Ctrl Pts',(71.761352481924,-16.8959903988411,0.));
#54757=CARTESIAN_POINT('Ctrl Pts',(71.761352481924,-16.8959903988411,12.));
#54758=CARTESIAN_POINT('Ctrl Pts',(71.7878279229556,-16.8912353270944,0.));
#54759=CARTESIAN_POINT('Ctrl Pts',(71.7878279229556,-16.8912353270944,12.));
#54760=CARTESIAN_POINT('Ctrl Pts',(71.8143347584977,-16.8864495151347,0.));
#54761=CARTESIAN_POINT('Ctrl Pts',(71.8143347584977,-16.8864495151347,12.));
#54762=CARTESIAN_POINT('Ctrl Pts',(71.8408728908269,-16.8816329317473,0.));
#54763=CARTESIAN_POINT('Ctrl Pts',(71.8408728908269,-16.8816329317473,12.));
#54764=CARTESIAN_POINT('Ctrl Pts',(71.8674422229151,-16.87678554607,0.));
#54765=CARTESIAN_POINT('Ctrl Pts',(71.8674422229151,-16.87678554607,12.));
#54766=CARTESIAN_POINT('Ctrl Pts',(71.8940426586521,-16.8719073276967,0.));
#54767=CARTESIAN_POINT('Ctrl Pts',(71.8940426586521,-16.8719073276967,12.));
#54768=CARTESIAN_POINT('Ctrl Pts',(71.920674103086,-16.8669982467915,0.));
#54769=CARTESIAN_POINT('Ctrl Pts',(71.920674103086,-16.8669982467915,12.));
#54770=CARTESIAN_POINT('Ctrl Pts',(71.9473364618889,-16.8620582738431,0.));
#54771=CARTESIAN_POINT('Ctrl Pts',(71.9473364618889,-16.8620582738431,12.));
#54772=CARTESIAN_POINT('Ctrl Pts',(71.9740296408319,-16.8570873794264,0.));
#54773=CARTESIAN_POINT('Ctrl Pts',(71.9740296408319,-16.8570873794264,12.));
#54774=CARTESIAN_POINT('Ctrl Pts',(72.0007535452071,-16.8520855339444,0.));
#54775=CARTESIAN_POINT('Ctrl Pts',(72.0007535452071,-16.8520855339444,12.));
#54776=CARTESIAN_POINT('Ctrl Pts',(72.0275080793742,-16.8470527074278,0.));
#54777=CARTESIAN_POINT('Ctrl Pts',(72.0275080793742,-16.8470527074278,12.));
#54778=CARTESIAN_POINT('Ctrl Pts',(72.0542931459865,-16.8419888691984,0.));
#54779=CARTESIAN_POINT('Ctrl Pts',(72.0542931459865,-16.8419888691984,12.));
#54780=CARTESIAN_POINT('Ctrl Pts',(72.0811086466177,-16.8368939881457,0.));
#54781=CARTESIAN_POINT('Ctrl Pts',(72.0811086466177,-16.8368939881457,12.));
#54782=CARTESIAN_POINT('Ctrl Pts',(72.1079544831569,-16.8317680333415,0.));
#54783=CARTESIAN_POINT('Ctrl Pts',(72.1079544831569,-16.8317680333415,12.));
#54784=CARTESIAN_POINT('Ctrl Pts',(72.1348305590233,-16.8266109745801,0.));
#54785=CARTESIAN_POINT('Ctrl Pts',(72.1348305590233,-16.8266109745801,12.));
#54786=CARTESIAN_POINT('Ctrl Pts',(72.1617367803226,-16.8214227828941,0.));
#54787=CARTESIAN_POINT('Ctrl Pts',(72.1617367803226,-16.8214227828941,12.));
#54788=CARTESIAN_POINT('Ctrl Pts',(72.1886730573389,-16.8162034312257,0.));
#54789=CARTESIAN_POINT('Ctrl Pts',(72.1886730573389,-16.8162034312257,12.));
#54790=CARTESIAN_POINT('Ctrl Pts',(72.2156393048868,-16.8109528945876,0.));
#54791=CARTESIAN_POINT('Ctrl Pts',(72.2156393048868,-16.8109528945876,12.));
#54792=CARTESIAN_POINT('Ctrl Pts',(72.242635439009,-16.8056711485797,0.));
#54793=CARTESIAN_POINT('Ctrl Pts',(72.242635439009,-16.8056711485797,12.));
#54794=CARTESIAN_POINT('Ctrl Pts',(72.2696613743687,-16.800358168223,0.));
#54795=CARTESIAN_POINT('Ctrl Pts',(72.2696613743687,-16.800358168223,12.));
#54796=CARTESIAN_POINT('Ctrl Pts',(72.2967170212331,-16.7950139266117,0.));
#54797=CARTESIAN_POINT('Ctrl Pts',(72.2967170212331,-16.7950139266117,12.));
#54798=CARTESIAN_POINT('Ctrl Pts',(72.323802282931,-16.7896383937839,0.));
#54799=CARTESIAN_POINT('Ctrl Pts',(72.323802282931,-16.7896383937839,12.));
#54800=CARTESIAN_POINT('Ctrl Pts',(72.3509170523038,-16.7842315351401,0.));
#54801=CARTESIAN_POINT('Ctrl Pts',(72.3509170523038,-16.7842315351401,12.));
#54802=CARTESIAN_POINT('Ctrl Pts',(72.3780612168057,-16.7787933137551,0.));
#54803=CARTESIAN_POINT('Ctrl Pts',(72.3780612168057,-16.7787933137551,12.));
#54804=CARTESIAN_POINT('Ctrl Pts',(72.4052346648058,-16.7733236932185,0.));
#54805=CARTESIAN_POINT('Ctrl Pts',(72.4052346648058,-16.7733236932185,12.));
#54806=CARTESIAN_POINT('Ctrl Pts',(72.4324372916884,-16.7678226404189,0.));
#54807=CARTESIAN_POINT('Ctrl Pts',(72.4324372916884,-16.7678226404189,12.));
#54808=CARTESIAN_POINT('Ctrl Pts',(72.4596690055347,-16.7622901280741,0.));
#54809=CARTESIAN_POINT('Ctrl Pts',(72.4596690055347,-16.7622901280741,12.));
#54810=CARTESIAN_POINT('Ctrl Pts',(72.4869297342051,-16.7567261380614,0.));
#54811=CARTESIAN_POINT('Ctrl Pts',(72.4869297342051,-16.7567261380614,12.));
#54812=CARTESIAN_POINT('Ctrl Pts',(72.5142194273203,-16.7511306618793,0.));
#54813=CARTESIAN_POINT('Ctrl Pts',(72.5142194273203,-16.7511306618793,12.));
#54814=CARTESIAN_POINT('Ctrl Pts',(72.5415380515905,-16.7455036973724,0.));
#54815=CARTESIAN_POINT('Ctrl Pts',(72.5415380515905,-16.7455036973724,12.));
#54816=CARTESIAN_POINT('Ctrl Pts',(72.563416080574,-16.7409769365953,0.));
#54817=CARTESIAN_POINT('Ctrl Pts',(72.563416080574,-16.7409769365953,12.));
#54818=CARTESIAN_POINT('Ctrl Pts',(72.5798376087406,-16.7375676985272,0.));
#54819=CARTESIAN_POINT('Ctrl Pts',(72.5798376087406,-16.7375676985272,12.));
#54820=CARTESIAN_POINT('Ctrl Pts',(72.5907910745874,-16.7352885767459,0.));
#54821=CARTESIAN_POINT('Ctrl Pts',(72.5907910745874,-16.7352885767459,12.));
#54822=CARTESIAN_POINT('Ctrl Pts',(72.5962692526112,-16.7341474417544,0.));
#54823=CARTESIAN_POINT('Ctrl Pts',(72.5962692526112,-16.7341474417544,12.));
#54824=CARTESIAN_POINT('',(67.8307641965655,-17.2912529479484,0.));
#54825=CARTESIAN_POINT('Ctrl Pts',(67.8307641965655,-17.2912529479484,0.));
#54826=CARTESIAN_POINT('Ctrl Pts',(67.8346476309018,-17.2912149114119,0.));
#54827=CARTESIAN_POINT('Ctrl Pts',(67.842419897098,-17.2911366591348,0.));
#54828=CARTESIAN_POINT('Ctrl Pts',(67.8540944889687,-17.291012743109,0.));
#54829=CARTESIAN_POINT('Ctrl Pts',(67.8696929978782,-17.2908344459694,0.));
#54830=CARTESIAN_POINT('Ctrl Pts',(67.8892451049608,-17.2905897723948,0.));
#54831=CARTESIAN_POINT('Ctrl Pts',(67.9088511496686,-17.2903232740694,0.));
#54832=CARTESIAN_POINT('Ctrl Pts',(67.9285110571741,-17.2900349103981,0.));
#54833=CARTESIAN_POINT('Ctrl Pts',(67.9482246901667,-17.2897246158941,0.));
#54834=CARTESIAN_POINT('Ctrl Pts',(67.9679918502579,-17.2893923013894,0.));
#54835=CARTESIAN_POINT('Ctrl Pts',(67.987812304921,-17.2890378644866,0.));
#54836=CARTESIAN_POINT('Ctrl Pts',(68.007685808115,-17.28866119774,0.));
#54837=CARTESIAN_POINT('Ctrl Pts',(68.0276121227356,-17.2882621974721,0.));
#54838=CARTESIAN_POINT('Ctrl Pts',(68.0475910442424,-17.2878407730961,0.));
#54839=CARTESIAN_POINT('Ctrl Pts',(68.0676223930412,-17.2873968440839,0.));
#54840=CARTESIAN_POINT('Ctrl Pts',(68.0877060033205,-17.2869303355432,0.));
#54841=CARTESIAN_POINT('Ctrl Pts',(68.1078417137877,-17.2864411745459,0.));
#54842=CARTESIAN_POINT('Ctrl Pts',(68.1280293561511,-17.2859292855705,0.));
#54843=CARTESIAN_POINT('Ctrl Pts',(68.1482687493226,-17.2853945882072,0.));
#54844=CARTESIAN_POINT('Ctrl Pts',(68.1685597054232,-17.2848369995293,0.));
#54845=CARTESIAN_POINT('Ctrl Pts',(68.1889020335427,-17.2842564355799,0.));
#54846=CARTESIAN_POINT('Ctrl Pts',(68.2092955440567,-17.2836528130819,0.));
#54847=CARTESIAN_POINT('Ctrl Pts',(68.2297400535294,-17.2830260513867,0.));
#54848=CARTESIAN_POINT('Ctrl Pts',(68.2502353845071,-17.2823760723874,0.));
#54849=CARTESIAN_POINT('Ctrl Pts',(68.2707813631731,-17.2817027995831,0.));
#54850=CARTESIAN_POINT('Ctrl Pts',(68.2913778177261,-17.2810061574353,0.));
#54851=CARTESIAN_POINT('Ctrl Pts',(68.3120245763914,-17.2802860705815,0.));
#54852=CARTESIAN_POINT('Ctrl Pts',(68.3327214657575,-17.2795424631799,0.));
#54853=CARTESIAN_POINT('Ctrl Pts',(68.3534683116515,-17.2787752592484,0.));
#54854=CARTESIAN_POINT('Ctrl Pts',(68.3742649398964,-17.2779843829608,0.));
#54855=CARTESIAN_POINT('Ctrl Pts',(68.3951111770487,-17.2771697589384,0.));
#54856=CARTESIAN_POINT('Ctrl Pts',(68.4160068512753,-17.2763313126018,0.));
#54857=CARTESIAN_POINT('Ctrl Pts',(68.436951792677,-17.2754689702992,0.));
#54858=CARTESIAN_POINT('Ctrl Pts',(68.4579458328185,-17.2745826591119,0.));
#54859=CARTESIAN_POINT('Ctrl Pts',(68.4789888044351,-17.2736723067365,0.));
#54860=CARTESIAN_POINT('Ctrl Pts',(68.5000805410911,-17.2727378413489,0.));
#54861=CARTESIAN_POINT('Ctrl Pts',(68.521220876786,-17.2717791914544,0.));
#54862=CARTESIAN_POINT('Ctrl Pts',(68.5424096459772,-17.2707962858919,0.));
#54863=CARTESIAN_POINT('Ctrl Pts',(68.5636466837517,-17.269789053896,0.));
#54864=CARTESIAN_POINT('Ctrl Pts',(68.5849318259449,-17.2687574251428,0.));
#54865=CARTESIAN_POINT('Ctrl Pts',(68.6062649092764,-17.2677013298057,0.));
#54866=CARTESIAN_POINT('Ctrl Pts',(68.6276457714729,-17.2666206986084,0.));
#54867=CARTESIAN_POINT('Ctrl Pts',(68.6490742512057,-17.2655154627928,0.));
#54868=CARTESIAN_POINT('Ctrl Pts',(68.6705501880249,-17.2643855540892,0.));
#54869=CARTESIAN_POINT('Ctrl Pts',(68.6920734222938,-17.2632309046892,0.));
#54870=CARTESIAN_POINT('Ctrl Pts',(68.7136437951097,-17.2620514472182,0.));
#54871=CARTESIAN_POINT('Ctrl Pts',(68.7352611482547,-17.2608471147185,0.));
#54872=CARTESIAN_POINT('Ctrl Pts',(68.7569253242333,-17.259617840655,0.));
#54873=CARTESIAN_POINT('Ctrl Pts',(68.7786361662882,-17.2583635589198,0.));
#54874=CARTESIAN_POINT('Ctrl Pts',(68.8003935184184,-17.2570842038383,0.));
#54875=CARTESIAN_POINT('Ctrl Pts',(68.8221972253941,-17.2557797101812,0.));
#54876=CARTESIAN_POINT('Ctrl Pts',(68.844047132755,-17.2544500131624,0.));
#54877=CARTESIAN_POINT('Ctrl Pts',(68.8659430867972,-17.2530950484258,0.));
#54878=CARTESIAN_POINT('Ctrl Pts',(68.8878849345557,-17.2517147520376,0.));
#54879=CARTESIAN_POINT('Ctrl Pts',(68.909872523787,-17.2503090604792,0.));
#54880=CARTESIAN_POINT('Ctrl Pts',(68.9319057029409,-17.248877910643,0.));
#54881=CARTESIAN_POINT('Ctrl Pts',(68.9539843211619,-17.2474212398275,0.));
#54882=CARTESIAN_POINT('Ctrl Pts',(68.9761082282922,-17.2459389857327,0.));
#54883=CARTESIAN_POINT('Ctrl Pts',(68.9982772748694,-17.2444310864585,0.));
#54884=CARTESIAN_POINT('Ctrl Pts',(69.0204913121225,-17.2428974805044,0.));
#54885=CARTESIAN_POINT('Ctrl Pts',(69.0427501919636,-17.2413381067723,0.));
#54886=CARTESIAN_POINT('Ctrl Pts',(69.065053766986,-17.2397529045589,0.));
#54887=CARTESIAN_POINT('Ctrl Pts',(69.0874018904599,-17.2381418135491,0.));
#54888=CARTESIAN_POINT('Ctrl Pts',(69.1097944163245,-17.2365047738125,0.));
#54889=CARTESIAN_POINT('Ctrl Pts',(69.1322311991752,-17.2348417258015,0.));
#54890=CARTESIAN_POINT('Ctrl Pts',(69.1547120942527,-17.2331526103506,0.));
#54891=CARTESIAN_POINT('Ctrl Pts',(69.1772369574447,-17.23143736867,0.));
#54892=CARTESIAN_POINT('Ctrl Pts',(69.1998056452828,-17.2296959423407,0.));
#54893=CARTESIAN_POINT('Ctrl Pts',(69.222418014938,-17.227928273312,0.));
#54894=CARTESIAN_POINT('Ctrl Pts',(69.2450739242109,-17.226134303902,0.));
#54895=CARTESIAN_POINT('Ctrl Pts',(69.2677732315224,-17.224313976797,0.));
#54896=CARTESIAN_POINT('Ctrl Pts',(69.2905157959166,-17.2224672350438,0.));
#54897=CARTESIAN_POINT('Ctrl Pts',(69.3133014770555,-17.2205940220459,0.));
#54898=CARTESIAN_POINT('Ctrl Pts',(69.3361301352141,-17.2186942815602,0.));
#54899=CARTESIAN_POINT('Ctrl Pts',(69.3590016312692,-17.2167679576984,0.));
#54900=CARTESIAN_POINT('Ctrl Pts',(69.3819158266916,-17.2148149949252,0.));
#54901=CARTESIAN_POINT('Ctrl Pts',(69.404872583548,-17.2128353380502,0.));
#54902=CARTESIAN_POINT('Ctrl Pts',(69.4278717644973,-17.2108289322254,0.));
#54903=CARTESIAN_POINT('Ctrl Pts',(69.450913232785,-17.2087957229423,0.));
#54904=CARTESIAN_POINT('Ctrl Pts',(69.4739968522313,-17.2067356560336,0.));
#54905=CARTESIAN_POINT('Ctrl Pts',(69.4971224872269,-17.2046486776708,0.));
#54906=CARTESIAN_POINT('Ctrl Pts',(69.5202900027367,-17.2025347343577,0.));
#54907=CARTESIAN_POINT('Ctrl Pts',(69.5434992642944,-17.2003937729268,0.));
#54908=CARTESIAN_POINT('Ctrl Pts',(69.5667501379969,-17.1982257405377,0.));
#54909=CARTESIAN_POINT('Ctrl Pts',(69.5900424904921,-17.196030584678,0.));
#54910=CARTESIAN_POINT('Ctrl Pts',(69.6133761889749,-17.1938082531612,0.));
#54911=CARTESIAN_POINT('Ctrl Pts',(69.6367511011898,-17.1915586941192,0.));
#54912=CARTESIAN_POINT('Ctrl Pts',(69.6601670954269,-17.1892818560002,0.));
#54913=CARTESIAN_POINT('Ctrl Pts',(69.6836240405164,-17.1869776875666,0.));
#54914=CARTESIAN_POINT('Ctrl Pts',(69.7071218058178,-17.1846461378973,0.));
#54915=CARTESIAN_POINT('Ctrl Pts',(69.7306602612155,-17.1822871563842,0.));
#54916=CARTESIAN_POINT('Ctrl Pts',(69.7542392771234,-17.179900692726,0.));
#54917=CARTESIAN_POINT('Ctrl Pts',(69.777858724479,-17.1774866969256,0.));
#54918=CARTESIAN_POINT('Ctrl Pts',(69.8015184747398,-17.1750451192885,0.));
#54919=CARTESIAN_POINT('Ctrl Pts',(69.8252183998702,-17.1725759104252,0.));
#54920=CARTESIAN_POINT('Ctrl Pts',(69.8489583723407,-17.1700790212473,0.));
#54921=CARTESIAN_POINT('Ctrl Pts',(69.8727382651286,-17.167554402962,0.));
#54922=CARTESIAN_POINT('Ctrl Pts',(69.8965579517147,-17.1650020070686,0.));
#54923=CARTESIAN_POINT('Ctrl Pts',(69.9204173060781,-17.1624217853578,0.));
#54924=CARTESIAN_POINT('Ctrl Pts',(69.9443162026865,-17.1598136899144,0.));
#54925=CARTESIAN_POINT('Ctrl Pts',(69.9682545164939,-17.157177673114,0.));
#54926=CARTESIAN_POINT('Ctrl Pts',(69.9922321229424,-17.154513687616,0.));
#54927=CARTESIAN_POINT('Ctrl Pts',(70.0162488979584,-17.1518216863623,0.));
#54928=CARTESIAN_POINT('Ctrl Pts',(70.0403047179483,-17.1491016225749,0.));
#54929=CARTESIAN_POINT('Ctrl Pts',(70.0643994597873,-17.1463534497594,0.));
#54930=CARTESIAN_POINT('Ctrl Pts',(70.0885330008179,-17.1435771217018,0.));
#54931=CARTESIAN_POINT('Ctrl Pts',(70.1127052188522,-17.1407725924617,0.));
#54932=CARTESIAN_POINT('Ctrl Pts',(70.1369159921687,-17.1379398163709,0.));
#54933=CARTESIAN_POINT('Ctrl Pts',(70.1611651995083,-17.1350787480312,0.));
#54934=CARTESIAN_POINT('Ctrl Pts',(70.1854527200631,-17.1321893423182,0.));
#54935=CARTESIAN_POINT('Ctrl Pts',(70.2097784334747,-17.1292715543778,0.));
#54936=CARTESIAN_POINT('Ctrl Pts',(70.2341422198363,-17.1263253396202,0.));
#54937=CARTESIAN_POINT('Ctrl Pts',(70.2585439596901,-17.1233506537176,0.));
#54938=CARTESIAN_POINT('Ctrl Pts',(70.2829835340238,-17.1203474526031,0.));
#54939=CARTESIAN_POINT('Ctrl Pts',(70.3074608242608,-17.1173156924733,0.));
#54940=CARTESIAN_POINT('Ctrl Pts',(70.3319757122568,-17.1142553297867,0.));
#54941=CARTESIAN_POINT('Ctrl Pts',(70.3565280803022,-17.1111663212568,0.));
#54942=CARTESIAN_POINT('Ctrl Pts',(70.3811178111201,-17.1080486238499,0.));
#54943=CARTESIAN_POINT('Ctrl Pts',(70.4057447878624,-17.1049021947834,0.));
#54944=CARTESIAN_POINT('Ctrl Pts',(70.430408894101,-17.1017269915292,0.));
#54945=CARTESIAN_POINT('Ctrl Pts',(70.4551100138238,-17.0985229718124,0.));
#54946=CARTESIAN_POINT('Ctrl Pts',(70.4798480314381,-17.0952900936048,0.));
#54947=CARTESIAN_POINT('Ctrl Pts',(70.5046228317677,-17.0920283151219,0.));
#54948=CARTESIAN_POINT('Ctrl Pts',(70.5294343000513,-17.088737594822,0.));
#54949=CARTESIAN_POINT('Ctrl Pts',(70.5542823219331,-17.0854178914087,0.));
#54950=CARTESIAN_POINT('Ctrl Pts',(70.5791667834582,-17.082069163831,0.));
#54951=CARTESIAN_POINT('Ctrl Pts',(70.6040875710749,-17.0786913712763,0.));
#54952=CARTESIAN_POINT('Ctrl Pts',(70.6290445716337,-17.0752844731678,0.));
#54953=CARTESIAN_POINT('Ctrl Pts',(70.6540376723841,-17.0718484291624,0.));
#54954=CARTESIAN_POINT('Ctrl Pts',(70.6790667609679,-17.0683831991532,0.));
#54955=CARTESIAN_POINT('Ctrl Pts',(70.7041317254125,-17.0648887432713,0.));
#54956=CARTESIAN_POINT('Ctrl Pts',(70.7292324541341,-17.0613650218787,0.));
#54957=CARTESIAN_POINT('Ctrl Pts',(70.7543688359374,-17.0578119955649,0.));
#54958=CARTESIAN_POINT('Ctrl Pts',(70.7795407600127,-17.0542296251462,0.));
#54959=CARTESIAN_POINT('Ctrl Pts',(70.8047481159306,-17.0506178716664,0.));
#54960=CARTESIAN_POINT('Ctrl Pts',(70.8299907936346,-17.0469766964005,0.));
#54961=CARTESIAN_POINT('Ctrl Pts',(70.8552686834435,-17.0433060608478,0.));
#54962=CARTESIAN_POINT('Ctrl Pts',(70.8805816760507,-17.0396059267279,0.));
#54963=CARTESIAN_POINT('Ctrl Pts',(70.9059296625214,-17.0358762559786,0.));
#54964=CARTESIAN_POINT('Ctrl Pts',(70.9313125342872,-17.0321170107562,0.));
#54965=CARTESIAN_POINT('Ctrl Pts',(70.9567301831355,-17.028328153439,0.));
#54966=CARTESIAN_POINT('Ctrl Pts',(70.9821825012134,-17.0245096466228,0.));
#54967=CARTESIAN_POINT('Ctrl Pts',(71.0076693810303,-17.0206614531165,0.));
#54968=CARTESIAN_POINT('Ctrl Pts',(71.0331907154575,-17.0167835359419,0.));
#54969=CARTESIAN_POINT('Ctrl Pts',(71.0587463977266,-17.0128758583335,0.));
#54970=CARTESIAN_POINT('Ctrl Pts',(71.0843363214216,-17.0089383837437,0.));
#54971=CARTESIAN_POINT('Ctrl Pts',(71.1099603804779,-17.0049710758393,0.));
#54972=CARTESIAN_POINT('Ctrl Pts',(71.1356184691799,-17.0009738984935,0.));
#54973=CARTESIAN_POINT('Ctrl Pts',(71.1613104821565,-16.9969468157824,0.));
#54974=CARTESIAN_POINT('Ctrl Pts',(71.1870363143742,-16.9928897919829,0.));
#54975=CARTESIAN_POINT('Ctrl Pts',(71.2127958611248,-16.9888027915743,0.));
#54976=CARTESIAN_POINT('Ctrl Pts',(71.2385890180233,-16.9846857792385,0.));
#54977=CARTESIAN_POINT('Ctrl Pts',(71.2644156810209,-16.9805387198573,0.));
#54978=CARTESIAN_POINT('Ctrl Pts',(71.2902757464127,-16.9763615785138,0.));
#54979=CARTESIAN_POINT('Ctrl Pts',(71.3161691108425,-16.9721543204951,0.));
#54980=CARTESIAN_POINT('Ctrl Pts',(71.3420956713072,-16.9679169112993,0.));
#54981=CARTESIAN_POINT('Ctrl Pts',(71.3680553251548,-16.9636493166395,0.));
#54982=CARTESIAN_POINT('Ctrl Pts',(71.3940479700663,-16.9593515024274,0.));
#54983=CARTESIAN_POINT('Ctrl Pts',(71.4200735040374,-16.9550234347619,0.));
#54984=CARTESIAN_POINT('Ctrl Pts',(71.4461318253561,-16.9506650799188,0.));
#54985=CARTESIAN_POINT('Ctrl Pts',(71.4722228325805,-16.9462764043445,0.));
#54986=CARTESIAN_POINT('Ctrl Pts',(71.498346424507,-16.9418573746492,0.));
#54987=CARTESIAN_POINT('Ctrl Pts',(71.5245025002154,-16.9374079576204,0.));
#54988=CARTESIAN_POINT('Ctrl Pts',(71.5506909591139,-16.9329281202379,0.));
#54989=CARTESIAN_POINT('Ctrl Pts',(71.5769117009844,-16.9284178296934,0.));
#54990=CARTESIAN_POINT('Ctrl Pts',(71.6031646260169,-16.923877053407,0.));
#54991=CARTESIAN_POINT('Ctrl Pts',(71.6294496348644,-16.9193057590605,0.));
#54992=CARTESIAN_POINT('Ctrl Pts',(71.6557666285908,-16.9147039145715,0.));
#54993=CARTESIAN_POINT('Ctrl Pts',(71.6821155085605,-16.9100714880367,0.));
#54994=CARTESIAN_POINT('Ctrl Pts',(71.7084961763355,-16.9054084476847,0.));
#54995=CARTESIAN_POINT('Ctrl Pts',(71.7349085335796,-16.9007147618344,0.));
#54996=CARTESIAN_POINT('Ctrl Pts',(71.761352481924,-16.8959903988411,0.));
#54997=CARTESIAN_POINT('Ctrl Pts',(71.7878279229556,-16.8912353270944,0.));
#54998=CARTESIAN_POINT('Ctrl Pts',(71.8143347584977,-16.8864495151347,0.));
#54999=CARTESIAN_POINT('Ctrl Pts',(71.8408728908269,-16.8816329317473,0.));
#55000=CARTESIAN_POINT('Ctrl Pts',(71.8674422229151,-16.87678554607,0.));
#55001=CARTESIAN_POINT('Ctrl Pts',(71.8940426586521,-16.8719073276967,0.));
#55002=CARTESIAN_POINT('Ctrl Pts',(71.920674103086,-16.8669982467915,0.));
#55003=CARTESIAN_POINT('Ctrl Pts',(71.9473364618889,-16.8620582738431,0.));
#55004=CARTESIAN_POINT('Ctrl Pts',(71.9740296408319,-16.8570873794264,0.));
#55005=CARTESIAN_POINT('Ctrl Pts',(72.0007535452071,-16.8520855339444,0.));
#55006=CARTESIAN_POINT('Ctrl Pts',(72.0275080793742,-16.8470527074278,0.));
#55007=CARTESIAN_POINT('Ctrl Pts',(72.0542931459865,-16.8419888691984,0.));
#55008=CARTESIAN_POINT('Ctrl Pts',(72.0811086466177,-16.8368939881457,0.));
#55009=CARTESIAN_POINT('Ctrl Pts',(72.1079544831569,-16.8317680333415,0.));
#55010=CARTESIAN_POINT('Ctrl Pts',(72.1348305590233,-16.8266109745801,0.));
#55011=CARTESIAN_POINT('Ctrl Pts',(72.1617367803226,-16.8214227828941,0.));
#55012=CARTESIAN_POINT('Ctrl Pts',(72.1886730573389,-16.8162034312257,0.));
#55013=CARTESIAN_POINT('Ctrl Pts',(72.2156393048868,-16.8109528945876,0.));
#55014=CARTESIAN_POINT('Ctrl Pts',(72.2387802230664,-16.8064254147766,0.));
#55015=CARTESIAN_POINT('Ctrl Pts',(72.2565380035009,-16.8029374213801,0.));
#55016=CARTESIAN_POINT('Ctrl Pts',(72.2688994294962,-16.8005027425888,0.));
#55017=CARTESIAN_POINT('Ctrl Pts',(72.2758557890971,-16.7991305317792,0.));
#55018=CARTESIAN_POINT('Ctrl Pts',(72.2774028393488,-16.7988252568806,0.));
#55019=CARTESIAN_POINT('',(67.8307641965655,-17.2912529479484,12.));
#55020=CARTESIAN_POINT('',(67.8307641965655,-17.2912529479484,0.));
#55021=CARTESIAN_POINT('Ctrl Pts',(72.2774028393489,-16.7988252568806,12.));
#55022=CARTESIAN_POINT('Ctrl Pts',(72.2758557890971,-16.7991305317792,12.));
#55023=CARTESIAN_POINT('Ctrl Pts',(72.2688994294962,-16.8005027425888,12.));
#55024=CARTESIAN_POINT('Ctrl Pts',(72.2565380035009,-16.8029374213801,12.));
#55025=CARTESIAN_POINT('Ctrl Pts',(72.2387802230664,-16.8064254147766,12.));
#55026=CARTESIAN_POINT('Ctrl Pts',(72.2156393048868,-16.8109528945876,12.));
#55027=CARTESIAN_POINT('Ctrl Pts',(72.1886730573389,-16.8162034312257,12.));
#55028=CARTESIAN_POINT('Ctrl Pts',(72.1617367803226,-16.8214227828941,12.));
#55029=CARTESIAN_POINT('Ctrl Pts',(72.1348305590233,-16.8266109745801,12.));
#55030=CARTESIAN_POINT('Ctrl Pts',(72.1079544831569,-16.8317680333415,12.));
#55031=CARTESIAN_POINT('Ctrl Pts',(72.0811086466177,-16.8368939881457,12.));
#55032=CARTESIAN_POINT('Ctrl Pts',(72.0542931459865,-16.8419888691984,12.));
#55033=CARTESIAN_POINT('Ctrl Pts',(72.0275080793742,-16.8470527074278,12.));
#55034=CARTESIAN_POINT('Ctrl Pts',(72.0007535452071,-16.8520855339444,12.));
#55035=CARTESIAN_POINT('Ctrl Pts',(71.9740296408319,-16.8570873794264,12.));
#55036=CARTESIAN_POINT('Ctrl Pts',(71.9473364618889,-16.8620582738431,12.));
#55037=CARTESIAN_POINT('Ctrl Pts',(71.920674103086,-16.8669982467915,12.));
#55038=CARTESIAN_POINT('Ctrl Pts',(71.8940426586521,-16.8719073276967,12.));
#55039=CARTESIAN_POINT('Ctrl Pts',(71.8674422229151,-16.87678554607,12.));
#55040=CARTESIAN_POINT('Ctrl Pts',(71.8408728908269,-16.8816329317473,12.));
#55041=CARTESIAN_POINT('Ctrl Pts',(71.8143347584977,-16.8864495151347,12.));
#55042=CARTESIAN_POINT('Ctrl Pts',(71.7878279229556,-16.8912353270944,12.));
#55043=CARTESIAN_POINT('Ctrl Pts',(71.761352481924,-16.8959903988411,12.));
#55044=CARTESIAN_POINT('Ctrl Pts',(71.7349085335796,-16.9007147618344,12.));
#55045=CARTESIAN_POINT('Ctrl Pts',(71.7084961763355,-16.9054084476847,12.));
#55046=CARTESIAN_POINT('Ctrl Pts',(71.6821155085605,-16.9100714880367,12.));
#55047=CARTESIAN_POINT('Ctrl Pts',(71.6557666285908,-16.9147039145715,12.));
#55048=CARTESIAN_POINT('Ctrl Pts',(71.6294496348644,-16.9193057590605,12.));
#55049=CARTESIAN_POINT('Ctrl Pts',(71.6031646260169,-16.923877053407,12.));
#55050=CARTESIAN_POINT('Ctrl Pts',(71.5769117009844,-16.9284178296934,12.));
#55051=CARTESIAN_POINT('Ctrl Pts',(71.5506909591139,-16.9329281202379,12.));
#55052=CARTESIAN_POINT('Ctrl Pts',(71.5245025002154,-16.9374079576204,12.));
#55053=CARTESIAN_POINT('Ctrl Pts',(71.498346424507,-16.9418573746492,12.));
#55054=CARTESIAN_POINT('Ctrl Pts',(71.4722228325805,-16.9462764043445,12.));
#55055=CARTESIAN_POINT('Ctrl Pts',(71.4461318253561,-16.9506650799188,12.));
#55056=CARTESIAN_POINT('Ctrl Pts',(71.4200735040374,-16.9550234347619,12.));
#55057=CARTESIAN_POINT('Ctrl Pts',(71.3940479700663,-16.9593515024274,12.));
#55058=CARTESIAN_POINT('Ctrl Pts',(71.3680553251548,-16.9636493166395,12.));
#55059=CARTESIAN_POINT('Ctrl Pts',(71.3420956713072,-16.9679169112993,12.));
#55060=CARTESIAN_POINT('Ctrl Pts',(71.3161691108425,-16.9721543204951,12.));
#55061=CARTESIAN_POINT('Ctrl Pts',(71.2902757464127,-16.9763615785138,12.));
#55062=CARTESIAN_POINT('Ctrl Pts',(71.2644156810209,-16.9805387198573,12.));
#55063=CARTESIAN_POINT('Ctrl Pts',(71.2385890180233,-16.9846857792385,12.));
#55064=CARTESIAN_POINT('Ctrl Pts',(71.2127958611248,-16.9888027915743,12.));
#55065=CARTESIAN_POINT('Ctrl Pts',(71.1870363143742,-16.9928897919829,12.));
#55066=CARTESIAN_POINT('Ctrl Pts',(71.1613104821565,-16.9969468157824,12.));
#55067=CARTESIAN_POINT('Ctrl Pts',(71.1356184691799,-17.0009738984935,12.));
#55068=CARTESIAN_POINT('Ctrl Pts',(71.1099603804779,-17.0049710758393,12.));
#55069=CARTESIAN_POINT('Ctrl Pts',(71.0843363214216,-17.0089383837437,12.));
#55070=CARTESIAN_POINT('Ctrl Pts',(71.0587463977266,-17.0128758583335,12.));
#55071=CARTESIAN_POINT('Ctrl Pts',(71.0331907154575,-17.0167835359419,12.));
#55072=CARTESIAN_POINT('Ctrl Pts',(71.0076693810303,-17.0206614531165,12.));
#55073=CARTESIAN_POINT('Ctrl Pts',(70.9821825012134,-17.0245096466228,12.));
#55074=CARTESIAN_POINT('Ctrl Pts',(70.9567301831355,-17.028328153439,12.));
#55075=CARTESIAN_POINT('Ctrl Pts',(70.9313125342872,-17.0321170107562,12.));
#55076=CARTESIAN_POINT('Ctrl Pts',(70.9059296625214,-17.0358762559786,12.));
#55077=CARTESIAN_POINT('Ctrl Pts',(70.8805816760507,-17.0396059267279,12.));
#55078=CARTESIAN_POINT('Ctrl Pts',(70.8552686834435,-17.0433060608478,12.));
#55079=CARTESIAN_POINT('Ctrl Pts',(70.8299907936346,-17.0469766964005,12.));
#55080=CARTESIAN_POINT('Ctrl Pts',(70.8047481159306,-17.0506178716664,12.));
#55081=CARTESIAN_POINT('Ctrl Pts',(70.7795407600127,-17.0542296251462,12.));
#55082=CARTESIAN_POINT('Ctrl Pts',(70.7543688359374,-17.0578119955649,12.));
#55083=CARTESIAN_POINT('Ctrl Pts',(70.7292324541341,-17.0613650218787,12.));
#55084=CARTESIAN_POINT('Ctrl Pts',(70.7041317254125,-17.0648887432713,12.));
#55085=CARTESIAN_POINT('Ctrl Pts',(70.6790667609679,-17.0683831991532,12.));
#55086=CARTESIAN_POINT('Ctrl Pts',(70.6540376723841,-17.0718484291624,12.));
#55087=CARTESIAN_POINT('Ctrl Pts',(70.6290445716337,-17.0752844731678,12.));
#55088=CARTESIAN_POINT('Ctrl Pts',(70.6040875710749,-17.0786913712763,12.));
#55089=CARTESIAN_POINT('Ctrl Pts',(70.5791667834582,-17.082069163831,12.));
#55090=CARTESIAN_POINT('Ctrl Pts',(70.5542823219331,-17.0854178914087,12.));
#55091=CARTESIAN_POINT('Ctrl Pts',(70.5294343000513,-17.088737594822,12.));
#55092=CARTESIAN_POINT('Ctrl Pts',(70.5046228317677,-17.0920283151219,12.));
#55093=CARTESIAN_POINT('Ctrl Pts',(70.4798480314381,-17.0952900936048,12.));
#55094=CARTESIAN_POINT('Ctrl Pts',(70.4551100138238,-17.0985229718124,12.));
#55095=CARTESIAN_POINT('Ctrl Pts',(70.430408894101,-17.1017269915292,12.));
#55096=CARTESIAN_POINT('Ctrl Pts',(70.4057447878624,-17.1049021947834,12.));
#55097=CARTESIAN_POINT('Ctrl Pts',(70.3811178111201,-17.1080486238499,12.));
#55098=CARTESIAN_POINT('Ctrl Pts',(70.3565280803022,-17.1111663212568,12.));
#55099=CARTESIAN_POINT('Ctrl Pts',(70.3319757122568,-17.1142553297867,12.));
#55100=CARTESIAN_POINT('Ctrl Pts',(70.3074608242608,-17.1173156924733,12.));
#55101=CARTESIAN_POINT('Ctrl Pts',(70.2829835340238,-17.1203474526031,12.));
#55102=CARTESIAN_POINT('Ctrl Pts',(70.2585439596901,-17.1233506537176,12.));
#55103=CARTESIAN_POINT('Ctrl Pts',(70.2341422198363,-17.1263253396202,12.));
#55104=CARTESIAN_POINT('Ctrl Pts',(70.2097784334747,-17.1292715543778,12.));
#55105=CARTESIAN_POINT('Ctrl Pts',(70.1854527200631,-17.1321893423182,12.));
#55106=CARTESIAN_POINT('Ctrl Pts',(70.1611651995083,-17.1350787480312,12.));
#55107=CARTESIAN_POINT('Ctrl Pts',(70.1369159921687,-17.1379398163709,12.));
#55108=CARTESIAN_POINT('Ctrl Pts',(70.1127052188522,-17.1407725924617,12.));
#55109=CARTESIAN_POINT('Ctrl Pts',(70.0885330008179,-17.1435771217018,12.));
#55110=CARTESIAN_POINT('Ctrl Pts',(70.0643994597873,-17.1463534497594,12.));
#55111=CARTESIAN_POINT('Ctrl Pts',(70.0403047179483,-17.1491016225749,12.));
#55112=CARTESIAN_POINT('Ctrl Pts',(70.0162488979584,-17.1518216863623,12.));
#55113=CARTESIAN_POINT('Ctrl Pts',(69.9922321229424,-17.154513687616,12.));
#55114=CARTESIAN_POINT('Ctrl Pts',(69.9682545164939,-17.157177673114,12.));
#55115=CARTESIAN_POINT('Ctrl Pts',(69.9443162026865,-17.1598136899144,12.));
#55116=CARTESIAN_POINT('Ctrl Pts',(69.9204173060781,-17.1624217853578,12.));
#55117=CARTESIAN_POINT('Ctrl Pts',(69.8965579517147,-17.1650020070686,12.));
#55118=CARTESIAN_POINT('Ctrl Pts',(69.8727382651286,-17.167554402962,12.));
#55119=CARTESIAN_POINT('Ctrl Pts',(69.8489583723407,-17.1700790212473,12.));
#55120=CARTESIAN_POINT('Ctrl Pts',(69.8252183998702,-17.1725759104252,12.));
#55121=CARTESIAN_POINT('Ctrl Pts',(69.8015184747398,-17.1750451192885,12.));
#55122=CARTESIAN_POINT('Ctrl Pts',(69.777858724479,-17.1774866969256,12.));
#55123=CARTESIAN_POINT('Ctrl Pts',(69.7542392771234,-17.179900692726,12.));
#55124=CARTESIAN_POINT('Ctrl Pts',(69.7306602612155,-17.1822871563842,12.));
#55125=CARTESIAN_POINT('Ctrl Pts',(69.7071218058178,-17.1846461378973,12.));
#55126=CARTESIAN_POINT('Ctrl Pts',(69.6836240405164,-17.1869776875666,12.));
#55127=CARTESIAN_POINT('Ctrl Pts',(69.6601670954269,-17.1892818560002,12.));
#55128=CARTESIAN_POINT('Ctrl Pts',(69.6367511011898,-17.1915586941192,12.));
#55129=CARTESIAN_POINT('Ctrl Pts',(69.6133761889749,-17.1938082531612,12.));
#55130=CARTESIAN_POINT('Ctrl Pts',(69.5900424904921,-17.196030584678,12.));
#55131=CARTESIAN_POINT('Ctrl Pts',(69.5667501379969,-17.1982257405377,12.));
#55132=CARTESIAN_POINT('Ctrl Pts',(69.5434992642944,-17.2003937729268,12.));
#55133=CARTESIAN_POINT('Ctrl Pts',(69.5202900027367,-17.2025347343577,12.));
#55134=CARTESIAN_POINT('Ctrl Pts',(69.4971224872269,-17.2046486776708,12.));
#55135=CARTESIAN_POINT('Ctrl Pts',(69.4739968522313,-17.2067356560336,12.));
#55136=CARTESIAN_POINT('Ctrl Pts',(69.450913232785,-17.2087957229423,12.));
#55137=CARTESIAN_POINT('Ctrl Pts',(69.4278717644973,-17.2108289322254,12.));
#55138=CARTESIAN_POINT('Ctrl Pts',(69.404872583548,-17.2128353380502,12.));
#55139=CARTESIAN_POINT('Ctrl Pts',(69.3819158266916,-17.2148149949252,12.));
#55140=CARTESIAN_POINT('Ctrl Pts',(69.3590016312692,-17.2167679576984,12.));
#55141=CARTESIAN_POINT('Ctrl Pts',(69.3361301352141,-17.2186942815602,12.));
#55142=CARTESIAN_POINT('Ctrl Pts',(69.3133014770555,-17.2205940220459,12.));
#55143=CARTESIAN_POINT('Ctrl Pts',(69.2905157959166,-17.2224672350438,12.));
#55144=CARTESIAN_POINT('Ctrl Pts',(69.2677732315224,-17.224313976797,12.));
#55145=CARTESIAN_POINT('Ctrl Pts',(69.2450739242109,-17.226134303902,12.));
#55146=CARTESIAN_POINT('Ctrl Pts',(69.222418014938,-17.227928273312,12.));
#55147=CARTESIAN_POINT('Ctrl Pts',(69.1998056452828,-17.2296959423407,12.));
#55148=CARTESIAN_POINT('Ctrl Pts',(69.1772369574447,-17.23143736867,12.));
#55149=CARTESIAN_POINT('Ctrl Pts',(69.1547120942527,-17.2331526103506,12.));
#55150=CARTESIAN_POINT('Ctrl Pts',(69.1322311991752,-17.2348417258015,12.));
#55151=CARTESIAN_POINT('Ctrl Pts',(69.1097944163245,-17.2365047738125,12.));
#55152=CARTESIAN_POINT('Ctrl Pts',(69.0874018904599,-17.2381418135491,12.));
#55153=CARTESIAN_POINT('Ctrl Pts',(69.065053766986,-17.2397529045589,12.));
#55154=CARTESIAN_POINT('Ctrl Pts',(69.0427501919636,-17.2413381067723,12.));
#55155=CARTESIAN_POINT('Ctrl Pts',(69.0204913121225,-17.2428974805044,12.));
#55156=CARTESIAN_POINT('Ctrl Pts',(68.9982772748694,-17.2444310864585,12.));
#55157=CARTESIAN_POINT('Ctrl Pts',(68.9761082282922,-17.2459389857327,12.));
#55158=CARTESIAN_POINT('Ctrl Pts',(68.9539843211619,-17.2474212398275,12.));
#55159=CARTESIAN_POINT('Ctrl Pts',(68.9319057029409,-17.248877910643,12.));
#55160=CARTESIAN_POINT('Ctrl Pts',(68.909872523787,-17.2503090604792,12.));
#55161=CARTESIAN_POINT('Ctrl Pts',(68.8878849345557,-17.2517147520376,12.));
#55162=CARTESIAN_POINT('Ctrl Pts',(68.8659430867972,-17.2530950484258,12.));
#55163=CARTESIAN_POINT('Ctrl Pts',(68.844047132755,-17.2544500131624,12.));
#55164=CARTESIAN_POINT('Ctrl Pts',(68.8221972253941,-17.2557797101812,12.));
#55165=CARTESIAN_POINT('Ctrl Pts',(68.8003935184184,-17.2570842038383,12.));
#55166=CARTESIAN_POINT('Ctrl Pts',(68.7786361662882,-17.2583635589198,12.));
#55167=CARTESIAN_POINT('Ctrl Pts',(68.7569253242333,-17.259617840655,12.));
#55168=CARTESIAN_POINT('Ctrl Pts',(68.7352611482547,-17.2608471147185,12.));
#55169=CARTESIAN_POINT('Ctrl Pts',(68.7136437951097,-17.2620514472182,12.));
#55170=CARTESIAN_POINT('Ctrl Pts',(68.6920734222938,-17.2632309046892,12.));
#55171=CARTESIAN_POINT('Ctrl Pts',(68.6705501880249,-17.2643855540892,12.));
#55172=CARTESIAN_POINT('Ctrl Pts',(68.6490742512057,-17.2655154627928,12.));
#55173=CARTESIAN_POINT('Ctrl Pts',(68.6276457714729,-17.2666206986084,12.));
#55174=CARTESIAN_POINT('Ctrl Pts',(68.6062649092764,-17.2677013298057,12.));
#55175=CARTESIAN_POINT('Ctrl Pts',(68.5849318259449,-17.2687574251428,12.));
#55176=CARTESIAN_POINT('Ctrl Pts',(68.5636466837517,-17.269789053896,12.));
#55177=CARTESIAN_POINT('Ctrl Pts',(68.5424096459772,-17.2707962858919,12.));
#55178=CARTESIAN_POINT('Ctrl Pts',(68.521220876786,-17.2717791914544,12.));
#55179=CARTESIAN_POINT('Ctrl Pts',(68.5000805410911,-17.2727378413489,12.));
#55180=CARTESIAN_POINT('Ctrl Pts',(68.4789888044351,-17.2736723067365,12.));
#55181=CARTESIAN_POINT('Ctrl Pts',(68.4579458328185,-17.2745826591119,12.));
#55182=CARTESIAN_POINT('Ctrl Pts',(68.436951792677,-17.2754689702992,12.));
#55183=CARTESIAN_POINT('Ctrl Pts',(68.4160068512753,-17.2763313126018,12.));
#55184=CARTESIAN_POINT('Ctrl Pts',(68.3951111770487,-17.2771697589384,12.));
#55185=CARTESIAN_POINT('Ctrl Pts',(68.3742649398964,-17.2779843829608,12.));
#55186=CARTESIAN_POINT('Ctrl Pts',(68.3534683116515,-17.2787752592484,12.));
#55187=CARTESIAN_POINT('Ctrl Pts',(68.3327214657575,-17.2795424631799,12.));
#55188=CARTESIAN_POINT('Ctrl Pts',(68.3120245763914,-17.2802860705815,12.));
#55189=CARTESIAN_POINT('Ctrl Pts',(68.2913778177261,-17.2810061574353,12.));
#55190=CARTESIAN_POINT('Ctrl Pts',(68.2707813631731,-17.2817027995831,12.));
#55191=CARTESIAN_POINT('Ctrl Pts',(68.2502353845071,-17.2823760723874,12.));
#55192=CARTESIAN_POINT('Ctrl Pts',(68.2297400535294,-17.2830260513867,12.));
#55193=CARTESIAN_POINT('Ctrl Pts',(68.2092955440567,-17.2836528130819,12.));
#55194=CARTESIAN_POINT('Ctrl Pts',(68.1889020335427,-17.2842564355799,12.));
#55195=CARTESIAN_POINT('Ctrl Pts',(68.1685597054232,-17.2848369995293,12.));
#55196=CARTESIAN_POINT('Ctrl Pts',(68.1482687493226,-17.2853945882072,12.));
#55197=CARTESIAN_POINT('Ctrl Pts',(68.1280293561511,-17.2859292855705,12.));
#55198=CARTESIAN_POINT('Ctrl Pts',(68.1078417137877,-17.2864411745459,12.));
#55199=CARTESIAN_POINT('Ctrl Pts',(68.0877060033205,-17.2869303355432,12.));
#55200=CARTESIAN_POINT('Ctrl Pts',(68.0676223930412,-17.2873968440839,12.));
#55201=CARTESIAN_POINT('Ctrl Pts',(68.0475910442424,-17.2878407730961,12.));
#55202=CARTESIAN_POINT('Ctrl Pts',(68.0276121227356,-17.2882621974721,12.));
#55203=CARTESIAN_POINT('Ctrl Pts',(68.007685808115,-17.28866119774,12.));
#55204=CARTESIAN_POINT('Ctrl Pts',(67.987812304921,-17.2890378644866,12.));
#55205=CARTESIAN_POINT('Ctrl Pts',(67.9679918502579,-17.2893923013894,12.));
#55206=CARTESIAN_POINT('Ctrl Pts',(67.9482246901667,-17.2897246158941,12.));
#55207=CARTESIAN_POINT('Ctrl Pts',(67.9285110571741,-17.2900349103981,12.));
#55208=CARTESIAN_POINT('Ctrl Pts',(67.9088511496686,-17.2903232740694,12.));
#55209=CARTESIAN_POINT('Ctrl Pts',(67.8892451049608,-17.2905897723948,12.));
#55210=CARTESIAN_POINT('Ctrl Pts',(67.8696929978782,-17.2908344459694,12.));
#55211=CARTESIAN_POINT('Ctrl Pts',(67.8540944889687,-17.291012743109,12.));
#55212=CARTESIAN_POINT('Ctrl Pts',(67.842419897098,-17.2911366591348,12.));
#55213=CARTESIAN_POINT('Ctrl Pts',(67.8346476309018,-17.2912149114119,12.));
#55214=CARTESIAN_POINT('Ctrl Pts',(67.8307641965655,-17.2912529479484,12.));
#55215=CARTESIAN_POINT('Ctrl Pts',(72.6050633494717,-15.3208442077424,-5.55111512312578E-16));
#55216=CARTESIAN_POINT('Ctrl Pts',(72.6050633494717,-15.3208442077424,4.));
#55217=CARTESIAN_POINT('Ctrl Pts',(72.6050633494717,-15.3208442077424,8.));
#55218=CARTESIAN_POINT('Ctrl Pts',(72.6050633494717,-15.3208442077424,12.));
#55219=CARTESIAN_POINT('Ctrl Pts',(72.6937764817671,-15.3856835210422,-5.55111512312578E-16));
#55220=CARTESIAN_POINT('Ctrl Pts',(72.6937764817671,-15.3856835210422,3.99999999999999));
#55221=CARTESIAN_POINT('Ctrl Pts',(72.6937764817672,-15.3856835210423,8.));
#55222=CARTESIAN_POINT('Ctrl Pts',(72.6937764817672,-15.3856835210423,12.));
#55223=CARTESIAN_POINT('Ctrl Pts',(72.8096834307711,-15.5519317750289,-5.55111512312578E-16));
#55224=CARTESIAN_POINT('Ctrl Pts',(72.8096834307711,-15.5519317750289,4.00000000000001));
#55225=CARTESIAN_POINT('Ctrl Pts',(72.8096834307711,-15.551931775029,8.));
#55226=CARTESIAN_POINT('Ctrl Pts',(72.8096834307711,-15.551931775029,12.));
#55227=CARTESIAN_POINT('Ctrl Pts',(72.8161171750016,-15.7502340068145,-5.55111512312578E-16));
#55228=CARTESIAN_POINT('Ctrl Pts',(72.8161171750016,-15.7502340068145,3.99999999999999));
#55229=CARTESIAN_POINT('Ctrl Pts',(72.8161171750016,-15.7502340068145,8.00000000000001));
#55230=CARTESIAN_POINT('Ctrl Pts',(72.8161171750016,-15.7502340068145,12.));
#55231=CARTESIAN_POINT('Ctrl Pts',(72.7986051948038,-15.8307637747231,-5.55111512312578E-16));
#55232=CARTESIAN_POINT('Ctrl Pts',(72.7986051948038,-15.8307637747231,4.));
#55233=CARTESIAN_POINT('Ctrl Pts',(72.7986051948038,-15.8307637747231,8.));
#55234=CARTESIAN_POINT('Ctrl Pts',(72.7986051948038,-15.8307637747231,12.));
#55235=CARTESIAN_POINT('',(72.6050633494717,-15.3208442077424,-2.77555756156289E-16));
#55236=CARTESIAN_POINT('',(72.7986051948038,-15.8307637747231,2.77555756156289E-16));
#55237=CARTESIAN_POINT('Ctrl Pts',(72.6050633494717,-15.3208442077424,-5.55111512312578E-16));
#55238=CARTESIAN_POINT('Ctrl Pts',(72.6937764817671,-15.3856835210422,-5.55111512312578E-16));
#55239=CARTESIAN_POINT('Ctrl Pts',(72.7600090240551,-15.4806825233204,-5.55111512312578E-16));
#55240=CARTESIAN_POINT('Ctrl Pts',(72.790495213764,-15.586148130594,-5.55111512312578E-16));
#55241=CARTESIAN_POINT('Ctrl Pts',(72.8133598560457,-15.6652473360493,-5.55111512312578E-16));
#55242=CARTESIAN_POINT('Ctrl Pts',(72.8161171750016,-15.7502340068145,-5.55111512312578E-16));
#55243=CARTESIAN_POINT('Ctrl Pts',(72.7986051948038,-15.8307637747231,-5.55111512312578E-16));
#55244=CARTESIAN_POINT('',(72.7986051948038,-15.8307637747231,12.));
#55245=CARTESIAN_POINT('Ctrl Pts',(72.7986051948038,-15.8307637747231,-5.55111512312578E-16));
#55246=CARTESIAN_POINT('Ctrl Pts',(72.7986051948038,-15.8307637747231,4.));
#55247=CARTESIAN_POINT('Ctrl Pts',(72.7986051948038,-15.8307637747231,8.));
#55248=CARTESIAN_POINT('Ctrl Pts',(72.7986051948038,-15.8307637747231,12.));
#55249=CARTESIAN_POINT('',(72.6050633494717,-15.3208442077424,12.));
#55250=CARTESIAN_POINT('Ctrl Pts',(72.7986051948038,-15.8307637747231,12.));
#55251=CARTESIAN_POINT('Ctrl Pts',(72.8161171750016,-15.7502340068145,12.));
#55252=CARTESIAN_POINT('Ctrl Pts',(72.8133598560457,-15.6652473360493,12.));
#55253=CARTESIAN_POINT('Ctrl Pts',(72.790495213764,-15.5861481305941,12.));
#55254=CARTESIAN_POINT('Ctrl Pts',(72.7600090240551,-15.4806825233204,12.));
#55255=CARTESIAN_POINT('Ctrl Pts',(72.6937764817672,-15.3856835210423,12.));
#55256=CARTESIAN_POINT('Ctrl Pts',(72.6050633494717,-15.3208442077424,12.));
#55257=CARTESIAN_POINT('Ctrl Pts',(72.6050633494717,-15.3208442077424,12.));
#55258=CARTESIAN_POINT('Ctrl Pts',(72.6050633494717,-15.3208442077424,8.));
#55259=CARTESIAN_POINT('Ctrl Pts',(72.6050633494717,-15.3208442077424,4.));
#55260=CARTESIAN_POINT('Ctrl Pts',(72.6050633494717,-15.3208442077424,-5.55111512312578E-16));
#55261=CARTESIAN_POINT('Origin',(3.65979954444617E-10,-8.10341340518591E-11,
0.));
#55262=CARTESIAN_POINT('Origin',(3.65979954444617E-10,-8.10341340518591E-11,
12.));
#55263=CARTESIAN_POINT('Origin',(3.65979954444617E-10,-8.10341340518591E-11,
0.));
#55264=CARTESIAN_POINT('Ctrl Pts',(70.9608233461364,-22.6894590071785,0.));
#55265=CARTESIAN_POINT('Ctrl Pts',(70.9608233461364,-22.6894590071785,4.));
#55266=CARTESIAN_POINT('Ctrl Pts',(70.9608233461364,-22.6894590071785,8.));
#55267=CARTESIAN_POINT('Ctrl Pts',(70.9608233461364,-22.6894590071785,12.));
#55268=CARTESIAN_POINT('Ctrl Pts',(70.9273579271571,-22.7941214270113,0.));
#55269=CARTESIAN_POINT('Ctrl Pts',(70.9273579271571,-22.7941214270113,4.));
#55270=CARTESIAN_POINT('Ctrl Pts',(70.9273579271571,-22.7941214270113,8.00000000000001));
#55271=CARTESIAN_POINT('Ctrl Pts',(70.9273579271571,-22.7941214270113,12.));
#55272=CARTESIAN_POINT('Ctrl Pts',(70.8062825417802,-22.9566438338674,0.));
#55273=CARTESIAN_POINT('Ctrl Pts',(70.8062825417802,-22.9566438338674,4.));
#55274=CARTESIAN_POINT('Ctrl Pts',(70.8062825417802,-22.9566438338674,7.99999999999999));
#55275=CARTESIAN_POINT('Ctrl Pts',(70.8062825417802,-22.9566438338674,12.));
#55276=CARTESIAN_POINT('Ctrl Pts',(70.6201870200063,-23.0254444386654,0.));
#55277=CARTESIAN_POINT('Ctrl Pts',(70.6201870200063,-23.0254444386654,4.));
#55278=CARTESIAN_POINT('Ctrl Pts',(70.6201870200063,-23.0254444386654,8.00000000000001));
#55279=CARTESIAN_POINT('Ctrl Pts',(70.6201870200063,-23.0254444386654,12.));
#55280=CARTESIAN_POINT('Ctrl Pts',(70.5382514078489,-23.0342913834092,0.));
#55281=CARTESIAN_POINT('Ctrl Pts',(70.5382514078489,-23.0342913834092,4.));
#55282=CARTESIAN_POINT('Ctrl Pts',(70.5382514078489,-23.0342913834092,8.));
#55283=CARTESIAN_POINT('Ctrl Pts',(70.5382514078489,-23.0342913834092,12.));
#55284=CARTESIAN_POINT('',(70.9608233461364,-22.6894590071785,0.));
#55285=CARTESIAN_POINT('',(70.5382514078489,-23.0342913834093,0.));
#55286=CARTESIAN_POINT('Ctrl Pts',(70.9608233461364,-22.6894590071785,0.));
#55287=CARTESIAN_POINT('Ctrl Pts',(70.9273579271571,-22.7941214270113,0.));
#55288=CARTESIAN_POINT('Ctrl Pts',(70.858171992656,-22.8869913737862,0.));
#55289=CARTESIAN_POINT('Ctrl Pts',(70.767754993209,-22.9492582831544,0.));
#55290=CARTESIAN_POINT('Ctrl Pts',(70.6999422436237,-22.9959584651805,0.));
#55291=CARTESIAN_POINT('Ctrl Pts',(70.6201870200063,-23.0254444386654,0.));
#55292=CARTESIAN_POINT('Ctrl Pts',(70.5382514078489,-23.0342913834092,0.));
#55293=CARTESIAN_POINT('',(70.5382514078489,-23.0342913834093,12.));
#55294=CARTESIAN_POINT('Ctrl Pts',(70.5382514078489,-23.0342913834092,0.));
#55295=CARTESIAN_POINT('Ctrl Pts',(70.5382514078489,-23.0342913834092,4.));
#55296=CARTESIAN_POINT('Ctrl Pts',(70.5382514078489,-23.0342913834092,8.));
#55297=CARTESIAN_POINT('Ctrl Pts',(70.5382514078489,-23.0342913834092,12.));
#55298=CARTESIAN_POINT('',(70.9608233461364,-22.6894590071785,12.));
#55299=CARTESIAN_POINT('Ctrl Pts',(70.5382514078489,-23.0342913834092,12.));
#55300=CARTESIAN_POINT('Ctrl Pts',(70.6201870200063,-23.0254444386654,12.));
#55301=CARTESIAN_POINT('Ctrl Pts',(70.6999422436237,-22.9959584651805,12.));
#55302=CARTESIAN_POINT('Ctrl Pts',(70.767754993209,-22.9492582831544,12.));
#55303=CARTESIAN_POINT('Ctrl Pts',(70.858171992656,-22.8869913737862,12.));
#55304=CARTESIAN_POINT('Ctrl Pts',(70.9273579271571,-22.7941214270113,12.));
#55305=CARTESIAN_POINT('Ctrl Pts',(70.9608233461364,-22.6894590071785,12.));
#55306=CARTESIAN_POINT('Ctrl Pts',(70.9608233461364,-22.6894590071785,12.));
#55307=CARTESIAN_POINT('Ctrl Pts',(70.9608233461364,-22.6894590071785,8.));
#55308=CARTESIAN_POINT('Ctrl Pts',(70.9608233461364,-22.6894590071785,4.));
#55309=CARTESIAN_POINT('Ctrl Pts',(70.9608233461364,-22.6894590071785,0.));
#55310=CARTESIAN_POINT('Ctrl Pts',(66.0656156664138,-23.1372951448024,0.));
#55311=CARTESIAN_POINT('Ctrl Pts',(66.0656156664138,-23.1372951448024,12.));
#55312=CARTESIAN_POINT('Ctrl Pts',(66.0694876382126,-23.1375957166104,0.));
#55313=CARTESIAN_POINT('Ctrl Pts',(66.0694876382126,-23.1375957166104,12.));
#55314=CARTESIAN_POINT('Ctrl Pts',(66.0772371487248,-23.13819515974,0.));
#55315=CARTESIAN_POINT('Ctrl Pts',(66.0772371487248,-23.13819515974,12.));
#55316=CARTESIAN_POINT('Ctrl Pts',(66.088878115242,-23.1390892229779,0.));
#55317=CARTESIAN_POINT('Ctrl Pts',(66.088878115242,-23.1390892229779,12.));
#55318=CARTESIAN_POINT('Ctrl Pts',(66.1044328067355,-23.1402711039425,0.));
#55319=CARTESIAN_POINT('Ctrl Pts',(66.1044328067355,-23.1402711039425,12.));
#55320=CARTESIAN_POINT('Ctrl Pts',(66.1239318368548,-23.1417314398398,0.));
#55321=CARTESIAN_POINT('Ctrl Pts',(66.1239318368548,-23.1417314398398,12.));
#55322=CARTESIAN_POINT('Ctrl Pts',(66.1434865015027,-23.1431747350098,0.));
#55323=CARTESIAN_POINT('Ctrl Pts',(66.1434865015027,-23.1431747350098,12.));
#55324=CARTESIAN_POINT('Ctrl Pts',(66.1630967296747,-23.1446009424903,0.));
#55325=CARTESIAN_POINT('Ctrl Pts',(66.1630967296747,-23.1446009424903,12.));
#55326=CARTESIAN_POINT('Ctrl Pts',(66.1827623902899,-23.1460099850763,0.));
#55327=CARTESIAN_POINT('Ctrl Pts',(66.1827623902899,-23.1460099850763,12.));
#55328=CARTESIAN_POINT('Ctrl Pts',(66.2024832934866,-23.1474017566484,0.));
#55329=CARTESIAN_POINT('Ctrl Pts',(66.2024832934866,-23.1474017566484,12.));
#55330=CARTESIAN_POINT('Ctrl Pts',(66.2222592165473,-23.1487761349328,0.));
#55331=CARTESIAN_POINT('Ctrl Pts',(66.2222592165473,-23.1487761349328,12.));
#55332=CARTESIAN_POINT('Ctrl Pts',(66.2420899237317,-23.1501329914488,0.));
#55333=CARTESIAN_POINT('Ctrl Pts',(66.2420899237317,-23.1501329914488,12.));
#55334=CARTESIAN_POINT('Ctrl Pts',(66.2619751878741,-23.1514722022483,0.));
#55335=CARTESIAN_POINT('Ctrl Pts',(66.2619751878741,-23.1514722022483,12.));
#55336=CARTESIAN_POINT('Ctrl Pts',(66.2819148131071,-23.1527936592625,0.));
#55337=CARTESIAN_POINT('Ctrl Pts',(66.2819148131071,-23.1527936592625,12.));
#55338=CARTESIAN_POINT('Ctrl Pts',(66.301908627539,-23.154097266617,0.));
#55339=CARTESIAN_POINT('Ctrl Pts',(66.301908627539,-23.154097266617,12.));
#55340=CARTESIAN_POINT('Ctrl Pts',(66.3219564725161,-23.1553829352531,0.));
#55341=CARTESIAN_POINT('Ctrl Pts',(66.3219564725161,-23.1553829352531,12.));
#55342=CARTESIAN_POINT('Ctrl Pts',(66.3420581937159,-23.1566505784626,0.));
#55343=CARTESIAN_POINT('Ctrl Pts',(66.3420581937159,-23.1566505784626,12.));
#55344=CARTESIAN_POINT('Ctrl Pts',(66.3622136300691,-23.1579001063438,0.));
#55345=CARTESIAN_POINT('Ctrl Pts',(66.3622136300691,-23.1579001063438,12.));
#55346=CARTESIAN_POINT('Ctrl Pts',(66.382422608185,-23.1591314230101,0.));
#55347=CARTESIAN_POINT('Ctrl Pts',(66.382422608185,-23.1591314230101,12.));
#55348=CARTESIAN_POINT('Ctrl Pts',(66.402684948127,-23.1603444294754,0.));
#55349=CARTESIAN_POINT('Ctrl Pts',(66.402684948127,-23.1603444294754,12.));
#55350=CARTESIAN_POINT('Ctrl Pts',(66.4230004670288,-23.1615390254636,0.));
#55351=CARTESIAN_POINT('Ctrl Pts',(66.4230004670288,-23.1615390254636,12.));
#55352=CARTESIAN_POINT('Ctrl Pts',(66.4433689832454,-23.1627151114875,0.));
#55353=CARTESIAN_POINT('Ctrl Pts',(66.4433689832454,-23.1627151114875,12.));
#55354=CARTESIAN_POINT('Ctrl Pts',(66.4637903210682,-23.163872591218,0.));
#55355=CARTESIAN_POINT('Ctrl Pts',(66.4637903210682,-23.163872591218,12.));
#55356=CARTESIAN_POINT('Ctrl Pts',(66.4842643105263,-23.1650113713792,0.));
#55357=CARTESIAN_POINT('Ctrl Pts',(66.4842643105263,-23.1650113713792,12.));
#55358=CARTESIAN_POINT('Ctrl Pts',(66.5047907851318,-23.1661313606123,0.));
#55359=CARTESIAN_POINT('Ctrl Pts',(66.5047907851318,-23.1661313606123,12.));
#55360=CARTESIAN_POINT('Ctrl Pts',(66.5253695803208,-23.1672324686928,0.));
#55361=CARTESIAN_POINT('Ctrl Pts',(66.5253695803208,-23.1672324686928,12.));
#55362=CARTESIAN_POINT('Ctrl Pts',(66.5460005315406,-23.1683146055736,0.));
#55363=CARTESIAN_POINT('Ctrl Pts',(66.5460005315406,-23.1683146055736,12.));
#55364=CARTESIAN_POINT('Ctrl Pts',(66.5666834726494,-23.169377680588,0.));
#55365=CARTESIAN_POINT('Ctrl Pts',(66.5666834726494,-23.169377680588,12.));
#55366=CARTESIAN_POINT('Ctrl Pts',(66.5874182367596,-23.1704216028626,0.));
#55367=CARTESIAN_POINT('Ctrl Pts',(66.5874182367596,-23.1704216028626,12.));
#55368=CARTESIAN_POINT('Ctrl Pts',(66.6082046569657,-23.1714462816794,0.));
#55369=CARTESIAN_POINT('Ctrl Pts',(66.6082046569657,-23.1714462816794,12.));
#55370=CARTESIAN_POINT('Ctrl Pts',(66.6290425670538,-23.1724516268299,0.));
#55371=CARTESIAN_POINT('Ctrl Pts',(66.6290425670538,-23.1724516268299,12.));
#55372=CARTESIAN_POINT('Ctrl Pts',(66.6499318023445,-23.1734375490421,0.));
#55373=CARTESIAN_POINT('Ctrl Pts',(66.6499318023445,-23.1734375490421,12.));
#55374=CARTESIAN_POINT('Ctrl Pts',(66.6708722000046,-23.174403960137,0.));
#55375=CARTESIAN_POINT('Ctrl Pts',(66.6708722000046,-23.174403960137,12.));
#55376=CARTESIAN_POINT('Ctrl Pts',(66.691863598595,-23.1753507727932,0.));
#55377=CARTESIAN_POINT('Ctrl Pts',(66.691863598595,-23.1753507727932,12.));
#55378=CARTESIAN_POINT('Ctrl Pts',(66.712905837789,-23.1762779004043,0.));
#55379=CARTESIAN_POINT('Ctrl Pts',(66.712905837789,-23.1762779004043,12.));
#55380=CARTESIAN_POINT('Ctrl Pts',(66.7339987580441,-23.1771852569137,0.));
#55381=CARTESIAN_POINT('Ctrl Pts',(66.7339987580441,-23.1771852569137,12.));
#55382=CARTESIAN_POINT('Ctrl Pts',(66.7551422002229,-23.1780727566309,0.));
#55383=CARTESIAN_POINT('Ctrl Pts',(66.7551422002229,-23.1780727566309,12.));
#55384=CARTESIAN_POINT('Ctrl Pts',(66.7763360056146,-23.1789403142376,0.));
#55385=CARTESIAN_POINT('Ctrl Pts',(66.7763360056146,-23.1789403142376,12.));
#55386=CARTESIAN_POINT('Ctrl Pts',(66.7975800161014,-23.1797878448645,0.));
#55387=CARTESIAN_POINT('Ctrl Pts',(66.7975800161014,-23.1797878448645,12.));
#55388=CARTESIAN_POINT('Ctrl Pts',(66.8188740742727,-23.1806152641475,0.));
#55389=CARTESIAN_POINT('Ctrl Pts',(66.8188740742727,-23.1806152641475,12.));
#55390=CARTESIAN_POINT('Ctrl Pts',(66.8402180235549,-23.1814224882948,0.));
#55391=CARTESIAN_POINT('Ctrl Pts',(66.8402180235549,-23.1814224882948,12.));
#55392=CARTESIAN_POINT('Ctrl Pts',(66.8616117083304,-23.1822094341508,0.));
#55393=CARTESIAN_POINT('Ctrl Pts',(66.8616117083304,-23.1822094341508,12.));
#55394=CARTESIAN_POINT('Ctrl Pts',(66.8830549738768,-23.1829760191583,0.));
#55395=CARTESIAN_POINT('Ctrl Pts',(66.8830549738768,-23.1829760191583,12.));
#55396=CARTESIAN_POINT('Ctrl Pts',(66.904547666305,-23.1837221613231,0.));
#55397=CARTESIAN_POINT('Ctrl Pts',(66.904547666305,-23.1837221613231,12.));
#55398=CARTESIAN_POINT('Ctrl Pts',(66.9260896324955,-23.1844477791816,0.));
#55399=CARTESIAN_POINT('Ctrl Pts',(66.9260896324955,-23.1844477791816,12.));
#55400=CARTESIAN_POINT('Ctrl Pts',(66.9476807200225,-23.1851527917666,0.));
#55401=CARTESIAN_POINT('Ctrl Pts',(66.9476807200225,-23.1851527917666,12.));
#55402=CARTESIAN_POINT('Ctrl Pts',(66.9693207771058,-23.1858371185852,0.));
#55403=CARTESIAN_POINT('Ctrl Pts',(66.9693207771058,-23.1858371185852,12.));
#55404=CARTESIAN_POINT('Ctrl Pts',(66.9910096526483,-23.1865006796291,0.));
#55405=CARTESIAN_POINT('Ctrl Pts',(66.9910096526483,-23.1865006796291,12.));
#55406=CARTESIAN_POINT('Ctrl Pts',(67.0127471962507,-23.1871433953796,0.));
#55407=CARTESIAN_POINT('Ctrl Pts',(67.0127471962507,-23.1871433953796,12.));
#55408=CARTESIAN_POINT('Ctrl Pts',(67.0345332582297,-23.1877651868155,0.));
#55409=CARTESIAN_POINT('Ctrl Pts',(67.0345332582297,-23.1877651868155,12.));
#55410=CARTESIAN_POINT('Ctrl Pts',(67.0563676896312,-23.1883659754268,0.));
#55411=CARTESIAN_POINT('Ctrl Pts',(67.0563676896312,-23.1883659754268,12.));
#55412=CARTESIAN_POINT('Ctrl Pts',(67.0782503422293,-23.1889456832116,0.));
#55413=CARTESIAN_POINT('Ctrl Pts',(67.0782503422293,-23.1889456832116,12.));
#55414=CARTESIAN_POINT('Ctrl Pts',(67.1001810685137,-23.1895042326626,0.));
#55415=CARTESIAN_POINT('Ctrl Pts',(67.1001810685137,-23.1895042326626,12.));
#55416=CARTESIAN_POINT('Ctrl Pts',(67.122159721674,-23.1900415467575,0.));
#55417=CARTESIAN_POINT('Ctrl Pts',(67.122159721674,-23.1900415467575,12.));
#55418=CARTESIAN_POINT('Ctrl Pts',(67.1441861555819,-23.1905575489506,0.));
#55419=CARTESIAN_POINT('Ctrl Pts',(67.1441861555819,-23.1905575489506,12.));
#55420=CARTESIAN_POINT('Ctrl Pts',(67.1662602247641,-23.1910521631658,0.));
#55421=CARTESIAN_POINT('Ctrl Pts',(67.1662602247641,-23.1910521631658,12.));
#55422=CARTESIAN_POINT('Ctrl Pts',(67.1883817844039,-23.1915253137924,0.));
#55423=CARTESIAN_POINT('Ctrl Pts',(67.1883817844039,-23.1915253137924,12.));
#55424=CARTESIAN_POINT('Ctrl Pts',(67.2105506903448,-23.1919769256804,0.));
#55425=CARTESIAN_POINT('Ctrl Pts',(67.2105506903448,-23.1919769256804,12.));
#55426=CARTESIAN_POINT('Ctrl Pts',(67.232766799088,-23.1924069241386,0.));
#55427=CARTESIAN_POINT('Ctrl Pts',(67.232766799088,-23.1924069241386,12.));
#55428=CARTESIAN_POINT('Ctrl Pts',(67.2550299677888,-23.1928152349344,0.));
#55429=CARTESIAN_POINT('Ctrl Pts',(67.2550299677888,-23.1928152349344,12.));
#55430=CARTESIAN_POINT('Ctrl Pts',(67.2773400542477,-23.1932017842954,0.));
#55431=CARTESIAN_POINT('Ctrl Pts',(67.2773400542477,-23.1932017842954,12.));
#55432=CARTESIAN_POINT('Ctrl Pts',(67.2996969169099,-23.193566498902,0.));
#55433=CARTESIAN_POINT('Ctrl Pts',(67.2996969169099,-23.193566498902,12.));
#55434=CARTESIAN_POINT('Ctrl Pts',(67.3221004148604,-23.1939093058802,0.));
#55435=CARTESIAN_POINT('Ctrl Pts',(67.3221004148604,-23.1939093058802,12.));
#55436=CARTESIAN_POINT('Ctrl Pts',(67.3445504078178,-23.1942301327979,0.));
#55437=CARTESIAN_POINT('Ctrl Pts',(67.3445504078178,-23.1942301327979,12.));
#55438=CARTESIAN_POINT('Ctrl Pts',(67.3670467561205,-23.1945289076608,0.));
#55439=CARTESIAN_POINT('Ctrl Pts',(67.3670467561205,-23.1945289076608,12.));
#55440=CARTESIAN_POINT('Ctrl Pts',(67.3895893207168,-23.1948055589123,0.));
#55441=CARTESIAN_POINT('Ctrl Pts',(67.3895893207168,-23.1948055589123,12.));
#55442=CARTESIAN_POINT('Ctrl Pts',(67.4121779631666,-23.195060015426,0.));
#55443=CARTESIAN_POINT('Ctrl Pts',(67.4121779631666,-23.195060015426,12.));
#55444=CARTESIAN_POINT('Ctrl Pts',(67.4348125456389,-23.1952922065009,0.));
#55445=CARTESIAN_POINT('Ctrl Pts',(67.4348125456389,-23.1952922065009,12.));
#55446=CARTESIAN_POINT('Ctrl Pts',(67.4574929309078,-23.1955020618591,0.));
#55447=CARTESIAN_POINT('Ctrl Pts',(67.4574929309078,-23.1955020618591,12.));
#55448=CARTESIAN_POINT('Ctrl Pts',(67.4802189823423,-23.1956895116446,0.));
#55449=CARTESIAN_POINT('Ctrl Pts',(67.4802189823423,-23.1956895116446,12.));
#55450=CARTESIAN_POINT('Ctrl Pts',(67.5029905638973,-23.1958544864225,0.));
#55451=CARTESIAN_POINT('Ctrl Pts',(67.5029905638973,-23.1958544864225,12.));
#55452=CARTESIAN_POINT('Ctrl Pts',(67.525807540117,-23.195996917171,0.));
#55453=CARTESIAN_POINT('Ctrl Pts',(67.525807540117,-23.195996917171,12.));
#55454=CARTESIAN_POINT('Ctrl Pts',(67.5486697761301,-23.1961167352777,0.));
#55455=CARTESIAN_POINT('Ctrl Pts',(67.5486697761301,-23.1961167352777,12.));
#55456=CARTESIAN_POINT('Ctrl Pts',(67.5715771376454,-23.1962138725358,0.));
#55457=CARTESIAN_POINT('Ctrl Pts',(67.5715771376454,-23.1962138725358,12.));
#55458=CARTESIAN_POINT('Ctrl Pts',(67.5945294909398,-23.1962882611444,0.));
#55459=CARTESIAN_POINT('Ctrl Pts',(67.5945294909398,-23.1962882611444,12.));
#55460=CARTESIAN_POINT('Ctrl Pts',(67.6175267028516,-23.1963398337056,0.));
#55461=CARTESIAN_POINT('Ctrl Pts',(67.6175267028516,-23.1963398337056,12.));
#55462=CARTESIAN_POINT('Ctrl Pts',(67.6405686407828,-23.1963685232176,0.));
#55463=CARTESIAN_POINT('Ctrl Pts',(67.6405686407828,-23.1963685232176,12.));
#55464=CARTESIAN_POINT('Ctrl Pts',(67.6636551726948,-23.196374263071,0.));
#55465=CARTESIAN_POINT('Ctrl Pts',(67.6636551726948,-23.196374263071,12.));
#55466=CARTESIAN_POINT('Ctrl Pts',(67.6867861671044,-23.1963569870457,0.));
#55467=CARTESIAN_POINT('Ctrl Pts',(67.6867861671044,-23.1963569870457,12.));
#55468=CARTESIAN_POINT('Ctrl Pts',(67.7099614930711,-23.1963166293116,0.));
#55469=CARTESIAN_POINT('Ctrl Pts',(67.7099614930711,-23.1963166293116,12.));
#55470=CARTESIAN_POINT('Ctrl Pts',(67.7331810201931,-23.1962531244261,0.));
#55471=CARTESIAN_POINT('Ctrl Pts',(67.7331810201931,-23.1962531244261,12.));
#55472=CARTESIAN_POINT('Ctrl Pts',(67.7564446186115,-23.1961664073274,0.));
#55473=CARTESIAN_POINT('Ctrl Pts',(67.7564446186115,-23.1961664073274,12.));
#55474=CARTESIAN_POINT('Ctrl Pts',(67.7797521590056,-23.1960564133308,0.));
#55475=CARTESIAN_POINT('Ctrl Pts',(67.7797521590056,-23.1960564133308,12.));
#55476=CARTESIAN_POINT('Ctrl Pts',(67.8031035125873,-23.1959230781265,0.));
#55477=CARTESIAN_POINT('Ctrl Pts',(67.8031035125873,-23.1959230781265,12.));
#55478=CARTESIAN_POINT('Ctrl Pts',(67.8264985510884,-23.1957663377798,0.));
#55479=CARTESIAN_POINT('Ctrl Pts',(67.8264985510884,-23.1957663377798,12.));
#55480=CARTESIAN_POINT('Ctrl Pts',(67.8499371467578,-23.1955861287276,0.));
#55481=CARTESIAN_POINT('Ctrl Pts',(67.8499371467578,-23.1955861287276,12.));
#55482=CARTESIAN_POINT('Ctrl Pts',(67.8734191723639,-23.1953823877727,0.));
#55483=CARTESIAN_POINT('Ctrl Pts',(67.8734191723639,-23.1953823877727,12.));
#55484=CARTESIAN_POINT('Ctrl Pts',(67.8969445011907,-23.19515505208,0.));
#55485=CARTESIAN_POINT('Ctrl Pts',(67.8969445011907,-23.19515505208,12.));
#55486=CARTESIAN_POINT('Ctrl Pts',(67.9205130070337,-23.1949040591748,0.));
#55487=CARTESIAN_POINT('Ctrl Pts',(67.9205130070337,-23.1949040591748,12.));
#55488=CARTESIAN_POINT('Ctrl Pts',(67.944124564187,-23.1946293469437,0.));
#55489=CARTESIAN_POINT('Ctrl Pts',(67.944124564187,-23.1946293469437,12.));
#55490=CARTESIAN_POINT('Ctrl Pts',(67.9677790474414,-23.1943308536307,0.));
#55491=CARTESIAN_POINT('Ctrl Pts',(67.9677790474414,-23.1943308536307,12.));
#55492=CARTESIAN_POINT('Ctrl Pts',(67.9914763320878,-23.194008517832,0.));
#55493=CARTESIAN_POINT('Ctrl Pts',(67.9914763320878,-23.194008517832,12.));
#55494=CARTESIAN_POINT('Ctrl Pts',(68.0152162939123,-23.193662278492,0.));
#55495=CARTESIAN_POINT('Ctrl Pts',(68.0152162939123,-23.193662278492,12.));
#55496=CARTESIAN_POINT('Ctrl Pts',(68.0389988091926,-23.1932920749021,0.));
#55497=CARTESIAN_POINT('Ctrl Pts',(68.0389988091926,-23.1932920749021,12.));
#55498=CARTESIAN_POINT('Ctrl Pts',(68.0628237546852,-23.1928978467018,0.));
#55499=CARTESIAN_POINT('Ctrl Pts',(68.0628237546852,-23.1928978467018,12.));
#55500=CARTESIAN_POINT('Ctrl Pts',(68.086691007624,-23.1924795338746,0.));
#55501=CARTESIAN_POINT('Ctrl Pts',(68.086691007624,-23.1924795338746,12.));
#55502=CARTESIAN_POINT('Ctrl Pts',(68.1106004457223,-23.1920370767424,0.));
#55503=CARTESIAN_POINT('Ctrl Pts',(68.1106004457223,-23.1920370767424,12.));
#55504=CARTESIAN_POINT('Ctrl Pts',(68.1345519471695,-23.1915704159624,0.));
#55505=CARTESIAN_POINT('Ctrl Pts',(68.1345519471695,-23.1915704159624,12.));
#55506=CARTESIAN_POINT('Ctrl Pts',(68.1585453906259,-23.1910794925252,0.));
#55507=CARTESIAN_POINT('Ctrl Pts',(68.1585453906259,-23.1910794925252,12.));
#55508=CARTESIAN_POINT('Ctrl Pts',(68.182580655213,-23.1905642477572,0.));
#55509=CARTESIAN_POINT('Ctrl Pts',(68.182580655213,-23.1905642477572,12.));
#55510=CARTESIAN_POINT('Ctrl Pts',(68.2066576205113,-23.1900246233165,0.));
#55511=CARTESIAN_POINT('Ctrl Pts',(68.2066576205113,-23.1900246233165,12.));
#55512=CARTESIAN_POINT('Ctrl Pts',(68.2307761665629,-23.189460561187,0.));
#55513=CARTESIAN_POINT('Ctrl Pts',(68.2307761665629,-23.189460561187,12.));
#55514=CARTESIAN_POINT('Ctrl Pts',(68.2549361738679,-23.1888720036757,0.));
#55515=CARTESIAN_POINT('Ctrl Pts',(68.2549361738679,-23.1888720036757,12.));
#55516=CARTESIAN_POINT('Ctrl Pts',(68.2791375233798,-23.1882588934108,0.));
#55517=CARTESIAN_POINT('Ctrl Pts',(68.2791375233798,-23.1882588934108,12.));
#55518=CARTESIAN_POINT('Ctrl Pts',(68.3033800964946,-23.1876211733439,0.));
#55519=CARTESIAN_POINT('Ctrl Pts',(68.3033800964946,-23.1876211733439,12.));
#55520=CARTESIAN_POINT('Ctrl Pts',(68.3276637750494,-23.1869587867464,0.));
#55521=CARTESIAN_POINT('Ctrl Pts',(68.3276637750494,-23.1869587867464,12.));
#55522=CARTESIAN_POINT('Ctrl Pts',(68.3519884413253,-23.1862716772034,0.));
#55523=CARTESIAN_POINT('Ctrl Pts',(68.3519884413253,-23.1862716772034,12.));
#55524=CARTESIAN_POINT('Ctrl Pts',(68.3763539780442,-23.1855597886117,0.));
#55525=CARTESIAN_POINT('Ctrl Pts',(68.3763539780442,-23.1855597886117,12.));
#55526=CARTESIAN_POINT('Ctrl Pts',(68.4007602683649,-23.1848230651776,0.));
#55527=CARTESIAN_POINT('Ctrl Pts',(68.4007602683649,-23.1848230651776,12.));
#55528=CARTESIAN_POINT('Ctrl Pts',(68.4252071958725,-23.1840614514191,0.));
#55529=CARTESIAN_POINT('Ctrl Pts',(68.4252071958725,-23.1840614514191,12.));
#55530=CARTESIAN_POINT('Ctrl Pts',(68.4496946445756,-23.1832748921629,0.));
#55531=CARTESIAN_POINT('Ctrl Pts',(68.4496946445756,-23.1832748921629,12.));
#55532=CARTESIAN_POINT('Ctrl Pts',(68.4742224989099,-23.1824633325385,0.));
#55533=CARTESIAN_POINT('Ctrl Pts',(68.4742224989099,-23.1824633325385,12.));
#55534=CARTESIAN_POINT('Ctrl Pts',(68.4987906437357,-23.1816267179752,0.));
#55535=CARTESIAN_POINT('Ctrl Pts',(68.4987906437357,-23.1816267179752,12.));
#55536=CARTESIAN_POINT('Ctrl Pts',(68.5233989643343,-23.1807649942011,0.));
#55537=CARTESIAN_POINT('Ctrl Pts',(68.5233989643343,-23.1807649942011,12.));
#55538=CARTESIAN_POINT('Ctrl Pts',(68.548047346398,-23.1798781072449,0.));
#55539=CARTESIAN_POINT('Ctrl Pts',(68.548047346398,-23.1798781072449,12.));
#55540=CARTESIAN_POINT('Ctrl Pts',(68.572735676027,-23.178966003434,0.));
#55541=CARTESIAN_POINT('Ctrl Pts',(68.572735676027,-23.178966003434,12.));
#55542=CARTESIAN_POINT('Ctrl Pts',(68.5974638397322,-23.1780286293873,0.));
#55543=CARTESIAN_POINT('Ctrl Pts',(68.5974638397322,-23.1780286293873,12.));
#55544=CARTESIAN_POINT('Ctrl Pts',(68.6222317244336,-23.1770659320137,0.));
#55545=CARTESIAN_POINT('Ctrl Pts',(68.6222317244336,-23.1770659320137,12.));
#55546=CARTESIAN_POINT('Ctrl Pts',(68.6470392174567,-23.1760778585094,0.));
#55547=CARTESIAN_POINT('Ctrl Pts',(68.6470392174567,-23.1760778585094,12.));
#55548=CARTESIAN_POINT('Ctrl Pts',(68.6718862065227,-23.1750643563606,0.));
#55549=CARTESIAN_POINT('Ctrl Pts',(68.6718862065227,-23.1750643563606,12.));
#55550=CARTESIAN_POINT('Ctrl Pts',(68.6967725797457,-23.1740253733423,0.));
#55551=CARTESIAN_POINT('Ctrl Pts',(68.6967725797457,-23.1740253733423,12.));
#55552=CARTESIAN_POINT('Ctrl Pts',(68.7216982256357,-23.1729608575116,0.));
#55553=CARTESIAN_POINT('Ctrl Pts',(68.7216982256357,-23.1729608575116,12.));
#55554=CARTESIAN_POINT('Ctrl Pts',(68.7466630330968,-23.1718707572047,0.));
#55555=CARTESIAN_POINT('Ctrl Pts',(68.7466630330968,-23.1718707572047,12.));
#55556=CARTESIAN_POINT('Ctrl Pts',(68.7716668914246,-23.1707550210359,0.));
#55557=CARTESIAN_POINT('Ctrl Pts',(68.7716668914246,-23.1707550210359,12.));
#55558=CARTESIAN_POINT('Ctrl Pts',(68.7967096902981,-23.1696135978993,0.));
#55559=CARTESIAN_POINT('Ctrl Pts',(68.7967096902981,-23.1696135978993,12.));
#55560=CARTESIAN_POINT('Ctrl Pts',(68.8217913197735,-23.1684464369681,0.));
#55561=CARTESIAN_POINT('Ctrl Pts',(68.8217913197735,-23.1684464369681,12.));
#55562=CARTESIAN_POINT('Ctrl Pts',(68.8469116702885,-23.1672534876885,0.));
#55563=CARTESIAN_POINT('Ctrl Pts',(68.8469116702885,-23.1672534876885,12.));
#55564=CARTESIAN_POINT('Ctrl Pts',(68.8720706326605,-23.1660346997763,0.));
#55565=CARTESIAN_POINT('Ctrl Pts',(68.8720706326605,-23.1660346997763,12.));
#55566=CARTESIAN_POINT('Ctrl Pts',(68.8972680980844,-23.1647900232152,0.));
#55567=CARTESIAN_POINT('Ctrl Pts',(68.8972680980844,-23.1647900232152,12.));
#55568=CARTESIAN_POINT('Ctrl Pts',(68.9225039581249,-23.1635194082582,0.));
#55569=CARTESIAN_POINT('Ctrl Pts',(68.9225039581249,-23.1635194082582,12.));
#55570=CARTESIAN_POINT('Ctrl Pts',(68.9477781047103,-23.1622228054291,0.));
#55571=CARTESIAN_POINT('Ctrl Pts',(68.9477781047103,-23.1622228054291,12.));
#55572=CARTESIAN_POINT('Ctrl Pts',(68.9730904301362,-23.1609001655154,0.));
#55573=CARTESIAN_POINT('Ctrl Pts',(68.9730904301362,-23.1609001655154,12.));
#55574=CARTESIAN_POINT('Ctrl Pts',(68.9984408270652,-23.1595514395655,0.));
#55575=CARTESIAN_POINT('Ctrl Pts',(68.9984408270652,-23.1595514395655,12.));
#55576=CARTESIAN_POINT('Ctrl Pts',(69.0238291885245,-23.1581765788869,0.));
#55577=CARTESIAN_POINT('Ctrl Pts',(69.0238291885245,-23.1581765788869,12.));
#55578=CARTESIAN_POINT('Ctrl Pts',(69.0492554078999,-23.1567755350472,0.));
#55579=CARTESIAN_POINT('Ctrl Pts',(69.0492554078999,-23.1567755350472,12.));
#55580=CARTESIAN_POINT('Ctrl Pts',(69.0747193789291,-23.1553482598768,0.));
#55581=CARTESIAN_POINT('Ctrl Pts',(69.0747193789291,-23.1553482598768,12.));
#55582=CARTESIAN_POINT('Ctrl Pts',(69.1002209957036,-23.153894705462,0.));
#55583=CARTESIAN_POINT('Ctrl Pts',(69.1002209957036,-23.153894705462,12.));
#55584=CARTESIAN_POINT('Ctrl Pts',(69.1257601526692,-23.1524148241413,0.));
#55585=CARTESIAN_POINT('Ctrl Pts',(69.1257601526692,-23.1524148241413,12.));
#55586=CARTESIAN_POINT('Ctrl Pts',(69.1513367446231,-23.1509085685033,0.));
#55587=CARTESIAN_POINT('Ctrl Pts',(69.1513367446231,-23.1509085685033,12.));
#55588=CARTESIAN_POINT('Ctrl Pts',(69.176950666708,-23.1493758913857,0.));
#55589=CARTESIAN_POINT('Ctrl Pts',(69.176950666708,-23.1493758913857,12.));
#55590=CARTESIAN_POINT('Ctrl Pts',(69.2026018144023,-23.1478167458788,0.));
#55591=CARTESIAN_POINT('Ctrl Pts',(69.2026018144023,-23.1478167458788,12.));
#55592=CARTESIAN_POINT('Ctrl Pts',(69.2282900835234,-23.1462310853205,0.));
#55593=CARTESIAN_POINT('Ctrl Pts',(69.2282900835234,-23.1462310853205,12.));
#55594=CARTESIAN_POINT('Ctrl Pts',(69.2540153702311,-23.1446188632931,0.));
#55595=CARTESIAN_POINT('Ctrl Pts',(69.2540153702311,-23.1446188632931,12.));
#55596=CARTESIAN_POINT('Ctrl Pts',(69.2797775710275,-23.1429800336221,0.));
#55597=CARTESIAN_POINT('Ctrl Pts',(69.2797775710275,-23.1429800336221,12.));
#55598=CARTESIAN_POINT('Ctrl Pts',(69.3055765827544,-23.1413145503763,0.));
#55599=CARTESIAN_POINT('Ctrl Pts',(69.3055765827544,-23.1413145503763,12.));
#55600=CARTESIAN_POINT('Ctrl Pts',(69.3314123025863,-23.1396223678725,0.));
#55601=CARTESIAN_POINT('Ctrl Pts',(69.3314123025863,-23.1396223678725,12.));
#55602=CARTESIAN_POINT('Ctrl Pts',(69.3572846280289,-23.1379034406718,0.));
#55603=CARTESIAN_POINT('Ctrl Pts',(69.3572846280289,-23.1379034406718,12.));
#55604=CARTESIAN_POINT('Ctrl Pts',(69.3831934569176,-23.1361577235708,0.));
#55605=CARTESIAN_POINT('Ctrl Pts',(69.3831934569176,-23.1361577235708,12.));
#55606=CARTESIAN_POINT('Ctrl Pts',(69.4091386874129,-23.1343851715989,0.));
#55607=CARTESIAN_POINT('Ctrl Pts',(69.4091386874129,-23.1343851715989,12.));
#55608=CARTESIAN_POINT('Ctrl Pts',(69.4351202179948,-23.1325857400145,0.));
#55609=CARTESIAN_POINT('Ctrl Pts',(69.4351202179948,-23.1325857400145,12.));
#55610=CARTESIAN_POINT('Ctrl Pts',(69.4611379474491,-23.1307593843063,0.));
#55611=CARTESIAN_POINT('Ctrl Pts',(69.4611379474491,-23.1307593843063,12.));
#55612=CARTESIAN_POINT('Ctrl Pts',(69.4871917748665,-23.1289060601927,0.));
#55613=CARTESIAN_POINT('Ctrl Pts',(69.4871917748665,-23.1289060601927,12.));
#55614=CARTESIAN_POINT('Ctrl Pts',(69.5132815996548,-23.1270257236207,0.));
#55615=CARTESIAN_POINT('Ctrl Pts',(69.5132815996548,-23.1270257236207,12.));
#55616=CARTESIAN_POINT('Ctrl Pts',(69.5394073215467,-23.1251183307678,0.));
#55617=CARTESIAN_POINT('Ctrl Pts',(69.5394073215467,-23.1251183307678,12.));
#55618=CARTESIAN_POINT('Ctrl Pts',(69.565568840605,-23.1231838380452,0.));
#55619=CARTESIAN_POINT('Ctrl Pts',(69.565568840605,-23.1231838380452,12.));
#55620=CARTESIAN_POINT('Ctrl Pts',(69.5917660572255,-23.1212222021049,0.));
#55621=CARTESIAN_POINT('Ctrl Pts',(69.5917660572255,-23.1212222021049,12.));
#55622=CARTESIAN_POINT('Ctrl Pts',(69.617998872135,-23.1192333798438,0.));
#55623=CARTESIAN_POINT('Ctrl Pts',(69.617998872135,-23.1192333798438,12.));
#55624=CARTESIAN_POINT('Ctrl Pts',(69.6442671863751,-23.1172173283856,0.));
#55625=CARTESIAN_POINT('Ctrl Pts',(69.6442671863751,-23.1172173283856,12.));
#55626=CARTESIAN_POINT('Ctrl Pts',(69.6705709012842,-23.1151740050679,0.));
#55627=CARTESIAN_POINT('Ctrl Pts',(69.6705709012842,-23.1151740050679,12.));
#55628=CARTESIAN_POINT('Ctrl Pts',(69.6969099184766,-23.1131033674301,0.));
#55629=CARTESIAN_POINT('Ctrl Pts',(69.6969099184766,-23.1131033674301,12.));
#55630=CARTESIAN_POINT('Ctrl Pts',(69.7232841398207,-23.111005373205,0.));
#55631=CARTESIAN_POINT('Ctrl Pts',(69.7232841398207,-23.111005373205,12.));
#55632=CARTESIAN_POINT('Ctrl Pts',(69.7496934674083,-23.1088799803094,0.));
#55633=CARTESIAN_POINT('Ctrl Pts',(69.7496934674083,-23.1088799803094,12.));
#55634=CARTESIAN_POINT('Ctrl Pts',(69.7761378035978,-23.1067271468615,0.));
#55635=CARTESIAN_POINT('Ctrl Pts',(69.7761378035978,-23.1067271468615,12.));
#55636=CARTESIAN_POINT('Ctrl Pts',(69.8026170510582,-23.1045468311994,0.));
#55637=CARTESIAN_POINT('Ctrl Pts',(69.8026170510582,-23.1045468311994,12.));
#55638=CARTESIAN_POINT('Ctrl Pts',(69.8291311128121,-23.1023389919052,0.));
#55639=CARTESIAN_POINT('Ctrl Pts',(69.8291311128121,-23.1023389919052,12.));
#55640=CARTESIAN_POINT('Ctrl Pts',(69.8556798922687,-23.100103587824,0.));
#55641=CARTESIAN_POINT('Ctrl Pts',(69.8556798922687,-23.100103587824,12.));
#55642=CARTESIAN_POINT('Ctrl Pts',(69.8822632932759,-23.0978405781018,0.));
#55643=CARTESIAN_POINT('Ctrl Pts',(69.8822632932759,-23.0978405781018,12.));
#55644=CARTESIAN_POINT('Ctrl Pts',(69.9088812200703,-23.0955499221556,0.));
#55645=CARTESIAN_POINT('Ctrl Pts',(69.9088812200703,-23.0955499221556,12.));
#55646=CARTESIAN_POINT('Ctrl Pts',(69.9355335771722,-23.0932315796066,0.));
#55647=CARTESIAN_POINT('Ctrl Pts',(69.9355335771722,-23.0932315796066,12.));
#55648=CARTESIAN_POINT('Ctrl Pts',(69.9622202692871,-23.0908855102251,0.));
#55649=CARTESIAN_POINT('Ctrl Pts',(69.9622202692871,-23.0908855102251,12.));
#55650=CARTESIAN_POINT('Ctrl Pts',(69.9889412012143,-23.0885116738799,0.));
#55651=CARTESIAN_POINT('Ctrl Pts',(69.9889412012143,-23.0885116738799,12.));
#55652=CARTESIAN_POINT('Ctrl Pts',(70.0156962777173,-23.0861100304731,0.));
#55653=CARTESIAN_POINT('Ctrl Pts',(70.0156962777173,-23.0861100304731,12.));
#55654=CARTESIAN_POINT('Ctrl Pts',(70.0424854035125,-23.0836805399378,0.));
#55655=CARTESIAN_POINT('Ctrl Pts',(70.0424854035125,-23.0836805399378,12.));
#55656=CARTESIAN_POINT('Ctrl Pts',(70.0693084835387,-23.081223162377,0.));
#55657=CARTESIAN_POINT('Ctrl Pts',(70.0693084835387,-23.081223162377,12.));
#55658=CARTESIAN_POINT('Ctrl Pts',(70.096165423165,-23.0787378581778,0.));
#55659=CARTESIAN_POINT('Ctrl Pts',(70.096165423165,-23.0787378581778,12.));
#55660=CARTESIAN_POINT('Ctrl Pts',(70.1230561284222,-23.076224588139,0.));
#55661=CARTESIAN_POINT('Ctrl Pts',(70.1230561284222,-23.076224588139,12.));
#55662=CARTESIAN_POINT('Ctrl Pts',(70.1499805062159,-23.0736833135934,0.));
#55663=CARTESIAN_POINT('Ctrl Pts',(70.1499805062159,-23.0736833135934,12.));
#55664=CARTESIAN_POINT('Ctrl Pts',(70.176938464556,-23.0711139965432,0.));
#55665=CARTESIAN_POINT('Ctrl Pts',(70.176938464556,-23.0711139965432,12.));
#55666=CARTESIAN_POINT('Ctrl Pts',(70.2039299120456,-23.0685165993682,0.));
#55667=CARTESIAN_POINT('Ctrl Pts',(70.2039299120456,-23.0685165993682,12.));
#55668=CARTESIAN_POINT('Ctrl Pts',(70.2309547573788,-23.0658910845425,0.));
#55669=CARTESIAN_POINT('Ctrl Pts',(70.2309547573788,-23.0658910845425,12.));
#55670=CARTESIAN_POINT('Ctrl Pts',(70.2580129087877,-23.0632374143276,0.));
#55671=CARTESIAN_POINT('Ctrl Pts',(70.2580129087877,-23.0632374143276,12.));
#55672=CARTESIAN_POINT('Ctrl Pts',(70.2851042736081,-23.0605555505326,0.));
#55673=CARTESIAN_POINT('Ctrl Pts',(70.2851042736081,-23.0605555505326,12.));
#55674=CARTESIAN_POINT('Ctrl Pts',(70.3122287575374,-23.0578454541116,0.));
#55675=CARTESIAN_POINT('Ctrl Pts',(70.3122287575374,-23.0578454541116,12.));
#55676=CARTESIAN_POINT('Ctrl Pts',(70.3393862652353,-23.0551070854942,0.));
#55677=CARTESIAN_POINT('Ctrl Pts',(70.3393862652353,-23.0551070854942,12.));
#55678=CARTESIAN_POINT('Ctrl Pts',(70.3665767016596,-23.0523404053188,0.));
#55679=CARTESIAN_POINT('Ctrl Pts',(70.3665767016596,-23.0523404053188,12.));
#55680=CARTESIAN_POINT('Ctrl Pts',(70.39379997323,-23.0495453750773,0.));
#55681=CARTESIAN_POINT('Ctrl Pts',(70.39379997323,-23.0495453750773,12.));
#55682=CARTESIAN_POINT('Ctrl Pts',(70.421055988934,-23.0467219577289,0.));
#55683=CARTESIAN_POINT('Ctrl Pts',(70.421055988934,-23.0467219577289,12.));
#55684=CARTESIAN_POINT('Ctrl Pts',(70.4483446617552,-23.0438701184996,0.));
#55685=CARTESIAN_POINT('Ctrl Pts',(70.4483446617552,-23.0438701184996,12.));
#55686=CARTESIAN_POINT('Ctrl Pts',(70.4756659090104,-23.0409898250727,0.));
#55687=CARTESIAN_POINT('Ctrl Pts',(70.4756659090104,-23.0409898250727,12.));
#55688=CARTESIAN_POINT('Ctrl Pts',(70.5030196491883,-23.0380810458237,0.));
#55689=CARTESIAN_POINT('Ctrl Pts',(70.5030196491883,-23.0380810458237,12.));
#55690=CARTESIAN_POINT('Ctrl Pts',(70.5304057994537,-23.035143748431,0.));
#55691=CARTESIAN_POINT('Ctrl Pts',(70.5304057994537,-23.035143748431,12.));
#55692=CARTESIAN_POINT('Ctrl Pts',(70.5578242727606,-23.0321778982705,0.));
#55693=CARTESIAN_POINT('Ctrl Pts',(70.5578242727606,-23.0321778982705,12.));
#55694=CARTESIAN_POINT('Ctrl Pts',(70.5852749754167,-23.0291834570688,0.));
#55695=CARTESIAN_POINT('Ctrl Pts',(70.5852749754167,-23.0291834570688,12.));
#55696=CARTESIAN_POINT('Ctrl Pts',(70.6127578036869,-23.0261603810187,0.));
#55697=CARTESIAN_POINT('Ctrl Pts',(70.6127578036869,-23.0261603810187,12.));
#55698=CARTESIAN_POINT('Ctrl Pts',(70.6402726486718,-23.0231086235263,0.));
#55699=CARTESIAN_POINT('Ctrl Pts',(70.6402726486718,-23.0231086235263,12.));
#55700=CARTESIAN_POINT('Ctrl Pts',(70.6678194023388,-23.0200281385906,0.));
#55701=CARTESIAN_POINT('Ctrl Pts',(70.6678194023388,-23.0200281385906,12.));
#55702=CARTESIAN_POINT('Ctrl Pts',(70.6953979633561,-23.0169188841084,0.));
#55703=CARTESIAN_POINT('Ctrl Pts',(70.6953979633561,-23.0169188841084,12.));
#55704=CARTESIAN_POINT('Ctrl Pts',(70.7230082425324,-23.0137808248899,0.));
#55705=CARTESIAN_POINT('Ctrl Pts',(70.7230082425324,-23.0137808248899,12.));
#55706=CARTESIAN_POINT('Ctrl Pts',(70.7506501695822,-23.0106139365941,0.));
#55707=CARTESIAN_POINT('Ctrl Pts',(70.7506501695822,-23.0106139365941,12.));
#55708=CARTESIAN_POINT('Ctrl Pts',(70.7783236950588,-23.0074182063611,0.));
#55709=CARTESIAN_POINT('Ctrl Pts',(70.7783236950588,-23.0074182063611,12.));
#55710=CARTESIAN_POINT('Ctrl Pts',(70.806028785987,-23.004193629142,0.));
#55711=CARTESIAN_POINT('Ctrl Pts',(70.806028785987,-23.004193629142,12.));
#55712=CARTESIAN_POINT('Ctrl Pts',(70.8282180956627,-23.0015908899222,0.));
#55713=CARTESIAN_POINT('Ctrl Pts',(70.8282180956627,-23.0015908899222,12.));
#55714=CARTESIAN_POINT('Ctrl Pts',(70.8448742696328,-22.9996258555187,0.));
#55715=CARTESIAN_POINT('Ctrl Pts',(70.8448742696328,-22.9996258555187,12.));
#55716=CARTESIAN_POINT('Ctrl Pts',(70.8559846927868,-22.9983100639354,0.));
#55717=CARTESIAN_POINT('Ctrl Pts',(70.8559846927868,-22.9983100639354,12.));
#55718=CARTESIAN_POINT('Ctrl Pts',(70.8615414811571,-22.9976507259817,0.));
#55719=CARTESIAN_POINT('Ctrl Pts',(70.8615414811571,-22.9976507259817,12.));
#55720=CARTESIAN_POINT('',(66.0656156664138,-23.1372951448024,0.));
#55721=CARTESIAN_POINT('Ctrl Pts',(66.0656156664138,-23.1372951448024,0.));
#55722=CARTESIAN_POINT('Ctrl Pts',(66.0694876382126,-23.1375957166104,0.));
#55723=CARTESIAN_POINT('Ctrl Pts',(66.0772371487248,-23.13819515974,0.));
#55724=CARTESIAN_POINT('Ctrl Pts',(66.088878115242,-23.1390892229779,0.));
#55725=CARTESIAN_POINT('Ctrl Pts',(66.1044328067355,-23.1402711039425,0.));
#55726=CARTESIAN_POINT('Ctrl Pts',(66.1239318368548,-23.1417314398398,0.));
#55727=CARTESIAN_POINT('Ctrl Pts',(66.1434865015027,-23.1431747350098,0.));
#55728=CARTESIAN_POINT('Ctrl Pts',(66.1630967296747,-23.1446009424903,0.));
#55729=CARTESIAN_POINT('Ctrl Pts',(66.1827623902899,-23.1460099850763,0.));
#55730=CARTESIAN_POINT('Ctrl Pts',(66.2024832934866,-23.1474017566484,0.));
#55731=CARTESIAN_POINT('Ctrl Pts',(66.2222592165473,-23.1487761349328,0.));
#55732=CARTESIAN_POINT('Ctrl Pts',(66.2420899237317,-23.1501329914488,0.));
#55733=CARTESIAN_POINT('Ctrl Pts',(66.2619751878741,-23.1514722022483,0.));
#55734=CARTESIAN_POINT('Ctrl Pts',(66.2819148131071,-23.1527936592625,0.));
#55735=CARTESIAN_POINT('Ctrl Pts',(66.301908627539,-23.154097266617,0.));
#55736=CARTESIAN_POINT('Ctrl Pts',(66.3219564725161,-23.1553829352531,0.));
#55737=CARTESIAN_POINT('Ctrl Pts',(66.3420581937159,-23.1566505784626,0.));
#55738=CARTESIAN_POINT('Ctrl Pts',(66.3622136300691,-23.1579001063438,0.));
#55739=CARTESIAN_POINT('Ctrl Pts',(66.382422608185,-23.1591314230101,0.));
#55740=CARTESIAN_POINT('Ctrl Pts',(66.402684948127,-23.1603444294754,0.));
#55741=CARTESIAN_POINT('Ctrl Pts',(66.4230004670288,-23.1615390254636,0.));
#55742=CARTESIAN_POINT('Ctrl Pts',(66.4433689832454,-23.1627151114875,0.));
#55743=CARTESIAN_POINT('Ctrl Pts',(66.4637903210682,-23.163872591218,0.));
#55744=CARTESIAN_POINT('Ctrl Pts',(66.4842643105263,-23.1650113713792,0.));
#55745=CARTESIAN_POINT('Ctrl Pts',(66.5047907851318,-23.1661313606123,0.));
#55746=CARTESIAN_POINT('Ctrl Pts',(66.5253695803208,-23.1672324686928,0.));
#55747=CARTESIAN_POINT('Ctrl Pts',(66.5460005315406,-23.1683146055736,0.));
#55748=CARTESIAN_POINT('Ctrl Pts',(66.5666834726494,-23.169377680588,0.));
#55749=CARTESIAN_POINT('Ctrl Pts',(66.5874182367596,-23.1704216028626,0.));
#55750=CARTESIAN_POINT('Ctrl Pts',(66.6082046569657,-23.1714462816794,0.));
#55751=CARTESIAN_POINT('Ctrl Pts',(66.6290425670538,-23.1724516268299,0.));
#55752=CARTESIAN_POINT('Ctrl Pts',(66.6499318023445,-23.1734375490421,0.));
#55753=CARTESIAN_POINT('Ctrl Pts',(66.6708722000046,-23.174403960137,0.));
#55754=CARTESIAN_POINT('Ctrl Pts',(66.691863598595,-23.1753507727932,0.));
#55755=CARTESIAN_POINT('Ctrl Pts',(66.712905837789,-23.1762779004043,0.));
#55756=CARTESIAN_POINT('Ctrl Pts',(66.7339987580441,-23.1771852569137,0.));
#55757=CARTESIAN_POINT('Ctrl Pts',(66.7551422002229,-23.1780727566309,0.));
#55758=CARTESIAN_POINT('Ctrl Pts',(66.7763360056146,-23.1789403142376,0.));
#55759=CARTESIAN_POINT('Ctrl Pts',(66.7975800161014,-23.1797878448645,0.));
#55760=CARTESIAN_POINT('Ctrl Pts',(66.8188740742727,-23.1806152641475,0.));
#55761=CARTESIAN_POINT('Ctrl Pts',(66.8402180235549,-23.1814224882948,0.));
#55762=CARTESIAN_POINT('Ctrl Pts',(66.8616117083304,-23.1822094341508,0.));
#55763=CARTESIAN_POINT('Ctrl Pts',(66.8830549738768,-23.1829760191583,0.));
#55764=CARTESIAN_POINT('Ctrl Pts',(66.904547666305,-23.1837221613231,0.));
#55765=CARTESIAN_POINT('Ctrl Pts',(66.9260896324955,-23.1844477791816,0.));
#55766=CARTESIAN_POINT('Ctrl Pts',(66.9476807200225,-23.1851527917666,0.));
#55767=CARTESIAN_POINT('Ctrl Pts',(66.9693207771058,-23.1858371185852,0.));
#55768=CARTESIAN_POINT('Ctrl Pts',(66.9910096526483,-23.1865006796291,0.));
#55769=CARTESIAN_POINT('Ctrl Pts',(67.0127471962507,-23.1871433953796,0.));
#55770=CARTESIAN_POINT('Ctrl Pts',(67.0345332582297,-23.1877651868155,0.));
#55771=CARTESIAN_POINT('Ctrl Pts',(67.0563676896312,-23.1883659754268,0.));
#55772=CARTESIAN_POINT('Ctrl Pts',(67.0782503422293,-23.1889456832116,0.));
#55773=CARTESIAN_POINT('Ctrl Pts',(67.1001810685137,-23.1895042326626,0.));
#55774=CARTESIAN_POINT('Ctrl Pts',(67.122159721674,-23.1900415467575,0.));
#55775=CARTESIAN_POINT('Ctrl Pts',(67.1441861555819,-23.1905575489506,0.));
#55776=CARTESIAN_POINT('Ctrl Pts',(67.1662602247641,-23.1910521631658,0.));
#55777=CARTESIAN_POINT('Ctrl Pts',(67.1883817844039,-23.1915253137924,0.));
#55778=CARTESIAN_POINT('Ctrl Pts',(67.2105506903448,-23.1919769256804,0.));
#55779=CARTESIAN_POINT('Ctrl Pts',(67.232766799088,-23.1924069241386,0.));
#55780=CARTESIAN_POINT('Ctrl Pts',(67.2550299677888,-23.1928152349344,0.));
#55781=CARTESIAN_POINT('Ctrl Pts',(67.2773400542477,-23.1932017842954,0.));
#55782=CARTESIAN_POINT('Ctrl Pts',(67.2996969169099,-23.193566498902,0.));
#55783=CARTESIAN_POINT('Ctrl Pts',(67.3221004148604,-23.1939093058802,0.));
#55784=CARTESIAN_POINT('Ctrl Pts',(67.3445504078178,-23.1942301327979,0.));
#55785=CARTESIAN_POINT('Ctrl Pts',(67.3670467561205,-23.1945289076608,0.));
#55786=CARTESIAN_POINT('Ctrl Pts',(67.3895893207168,-23.1948055589123,0.));
#55787=CARTESIAN_POINT('Ctrl Pts',(67.4121779631666,-23.195060015426,0.));
#55788=CARTESIAN_POINT('Ctrl Pts',(67.4348125456389,-23.1952922065009,0.));
#55789=CARTESIAN_POINT('Ctrl Pts',(67.4574929309078,-23.1955020618591,0.));
#55790=CARTESIAN_POINT('Ctrl Pts',(67.4802189823423,-23.1956895116446,0.));
#55791=CARTESIAN_POINT('Ctrl Pts',(67.5029905638973,-23.1958544864225,0.));
#55792=CARTESIAN_POINT('Ctrl Pts',(67.525807540117,-23.195996917171,0.));
#55793=CARTESIAN_POINT('Ctrl Pts',(67.5486697761301,-23.1961167352777,0.));
#55794=CARTESIAN_POINT('Ctrl Pts',(67.5715771376454,-23.1962138725358,0.));
#55795=CARTESIAN_POINT('Ctrl Pts',(67.5945294909398,-23.1962882611444,0.));
#55796=CARTESIAN_POINT('Ctrl Pts',(67.6175267028516,-23.1963398337056,0.));
#55797=CARTESIAN_POINT('Ctrl Pts',(67.6405686407828,-23.1963685232176,0.));
#55798=CARTESIAN_POINT('Ctrl Pts',(67.6636551726948,-23.196374263071,0.));
#55799=CARTESIAN_POINT('Ctrl Pts',(67.6867861671044,-23.1963569870457,0.));
#55800=CARTESIAN_POINT('Ctrl Pts',(67.7099614930711,-23.1963166293116,0.));
#55801=CARTESIAN_POINT('Ctrl Pts',(67.7331810201931,-23.1962531244261,0.));
#55802=CARTESIAN_POINT('Ctrl Pts',(67.7564446186115,-23.1961664073274,0.));
#55803=CARTESIAN_POINT('Ctrl Pts',(67.7797521590056,-23.1960564133308,0.));
#55804=CARTESIAN_POINT('Ctrl Pts',(67.8031035125873,-23.1959230781265,0.));
#55805=CARTESIAN_POINT('Ctrl Pts',(67.8264985510884,-23.1957663377798,0.));
#55806=CARTESIAN_POINT('Ctrl Pts',(67.8499371467578,-23.1955861287276,0.));
#55807=CARTESIAN_POINT('Ctrl Pts',(67.8734191723639,-23.1953823877727,0.));
#55808=CARTESIAN_POINT('Ctrl Pts',(67.8969445011907,-23.19515505208,0.));
#55809=CARTESIAN_POINT('Ctrl Pts',(67.9205130070337,-23.1949040591748,0.));
#55810=CARTESIAN_POINT('Ctrl Pts',(67.944124564187,-23.1946293469437,0.));
#55811=CARTESIAN_POINT('Ctrl Pts',(67.9677790474414,-23.1943308536307,0.));
#55812=CARTESIAN_POINT('Ctrl Pts',(67.9914763320878,-23.194008517832,0.));
#55813=CARTESIAN_POINT('Ctrl Pts',(68.0152162939123,-23.193662278492,0.));
#55814=CARTESIAN_POINT('Ctrl Pts',(68.0389988091926,-23.1932920749021,0.));
#55815=CARTESIAN_POINT('Ctrl Pts',(68.0628237546852,-23.1928978467018,0.));
#55816=CARTESIAN_POINT('Ctrl Pts',(68.086691007624,-23.1924795338746,0.));
#55817=CARTESIAN_POINT('Ctrl Pts',(68.1106004457223,-23.1920370767424,0.));
#55818=CARTESIAN_POINT('Ctrl Pts',(68.1345519471695,-23.1915704159624,0.));
#55819=CARTESIAN_POINT('Ctrl Pts',(68.1585453906259,-23.1910794925252,0.));
#55820=CARTESIAN_POINT('Ctrl Pts',(68.182580655213,-23.1905642477572,0.));
#55821=CARTESIAN_POINT('Ctrl Pts',(68.2066576205113,-23.1900246233165,0.));
#55822=CARTESIAN_POINT('Ctrl Pts',(68.2307761665629,-23.189460561187,0.));
#55823=CARTESIAN_POINT('Ctrl Pts',(68.2549361738679,-23.1888720036757,0.));
#55824=CARTESIAN_POINT('Ctrl Pts',(68.2791375233798,-23.1882588934108,0.));
#55825=CARTESIAN_POINT('Ctrl Pts',(68.3033800964946,-23.1876211733439,0.));
#55826=CARTESIAN_POINT('Ctrl Pts',(68.3276637750494,-23.1869587867464,0.));
#55827=CARTESIAN_POINT('Ctrl Pts',(68.3519884413253,-23.1862716772034,0.));
#55828=CARTESIAN_POINT('Ctrl Pts',(68.3763539780442,-23.1855597886117,0.));
#55829=CARTESIAN_POINT('Ctrl Pts',(68.4007602683649,-23.1848230651776,0.));
#55830=CARTESIAN_POINT('Ctrl Pts',(68.4252071958725,-23.1840614514191,0.));
#55831=CARTESIAN_POINT('Ctrl Pts',(68.4496946445756,-23.1832748921629,0.));
#55832=CARTESIAN_POINT('Ctrl Pts',(68.4742224989099,-23.1824633325385,0.));
#55833=CARTESIAN_POINT('Ctrl Pts',(68.4987906437357,-23.1816267179752,0.));
#55834=CARTESIAN_POINT('Ctrl Pts',(68.5233989643343,-23.1807649942011,0.));
#55835=CARTESIAN_POINT('Ctrl Pts',(68.548047346398,-23.1798781072449,0.));
#55836=CARTESIAN_POINT('Ctrl Pts',(68.572735676027,-23.178966003434,0.));
#55837=CARTESIAN_POINT('Ctrl Pts',(68.5974638397322,-23.1780286293873,0.));
#55838=CARTESIAN_POINT('Ctrl Pts',(68.6222317244336,-23.1770659320137,0.));
#55839=CARTESIAN_POINT('Ctrl Pts',(68.6470392174567,-23.1760778585094,0.));
#55840=CARTESIAN_POINT('Ctrl Pts',(68.6718862065227,-23.1750643563606,0.));
#55841=CARTESIAN_POINT('Ctrl Pts',(68.6967725797457,-23.1740253733423,0.));
#55842=CARTESIAN_POINT('Ctrl Pts',(68.7216982256357,-23.1729608575116,0.));
#55843=CARTESIAN_POINT('Ctrl Pts',(68.7466630330968,-23.1718707572047,0.));
#55844=CARTESIAN_POINT('Ctrl Pts',(68.7716668914246,-23.1707550210359,0.));
#55845=CARTESIAN_POINT('Ctrl Pts',(68.7967096902981,-23.1696135978993,0.));
#55846=CARTESIAN_POINT('Ctrl Pts',(68.8217913197735,-23.1684464369681,0.));
#55847=CARTESIAN_POINT('Ctrl Pts',(68.8469116702885,-23.1672534876885,0.));
#55848=CARTESIAN_POINT('Ctrl Pts',(68.8720706326605,-23.1660346997763,0.));
#55849=CARTESIAN_POINT('Ctrl Pts',(68.8972680980844,-23.1647900232152,0.));
#55850=CARTESIAN_POINT('Ctrl Pts',(68.9225039581249,-23.1635194082582,0.));
#55851=CARTESIAN_POINT('Ctrl Pts',(68.9477781047103,-23.1622228054291,0.));
#55852=CARTESIAN_POINT('Ctrl Pts',(68.9730904301362,-23.1609001655154,0.));
#55853=CARTESIAN_POINT('Ctrl Pts',(68.9984408270652,-23.1595514395655,0.));
#55854=CARTESIAN_POINT('Ctrl Pts',(69.0238291885245,-23.1581765788869,0.));
#55855=CARTESIAN_POINT('Ctrl Pts',(69.0492554078999,-23.1567755350472,0.));
#55856=CARTESIAN_POINT('Ctrl Pts',(69.0747193789291,-23.1553482598768,0.));
#55857=CARTESIAN_POINT('Ctrl Pts',(69.1002209957036,-23.153894705462,0.));
#55858=CARTESIAN_POINT('Ctrl Pts',(69.1257601526692,-23.1524148241413,0.));
#55859=CARTESIAN_POINT('Ctrl Pts',(69.1513367446231,-23.1509085685033,0.));
#55860=CARTESIAN_POINT('Ctrl Pts',(69.176950666708,-23.1493758913857,0.));
#55861=CARTESIAN_POINT('Ctrl Pts',(69.2026018144023,-23.1478167458788,0.));
#55862=CARTESIAN_POINT('Ctrl Pts',(69.2282900835234,-23.1462310853205,0.));
#55863=CARTESIAN_POINT('Ctrl Pts',(69.2540153702311,-23.1446188632931,0.));
#55864=CARTESIAN_POINT('Ctrl Pts',(69.2797775710275,-23.1429800336221,0.));
#55865=CARTESIAN_POINT('Ctrl Pts',(69.3055765827544,-23.1413145503763,0.));
#55866=CARTESIAN_POINT('Ctrl Pts',(69.3314123025863,-23.1396223678725,0.));
#55867=CARTESIAN_POINT('Ctrl Pts',(69.3572846280289,-23.1379034406718,0.));
#55868=CARTESIAN_POINT('Ctrl Pts',(69.3831934569176,-23.1361577235708,0.));
#55869=CARTESIAN_POINT('Ctrl Pts',(69.4091386874129,-23.1343851715989,0.));
#55870=CARTESIAN_POINT('Ctrl Pts',(69.4351202179948,-23.1325857400145,0.));
#55871=CARTESIAN_POINT('Ctrl Pts',(69.4611379474491,-23.1307593843063,0.));
#55872=CARTESIAN_POINT('Ctrl Pts',(69.4871917748665,-23.1289060601927,0.));
#55873=CARTESIAN_POINT('Ctrl Pts',(69.5132815996548,-23.1270257236207,0.));
#55874=CARTESIAN_POINT('Ctrl Pts',(69.5394073215467,-23.1251183307678,0.));
#55875=CARTESIAN_POINT('Ctrl Pts',(69.565568840605,-23.1231838380452,0.));
#55876=CARTESIAN_POINT('Ctrl Pts',(69.5917660572255,-23.1212222021049,0.));
#55877=CARTESIAN_POINT('Ctrl Pts',(69.617998872135,-23.1192333798438,0.));
#55878=CARTESIAN_POINT('Ctrl Pts',(69.6442671863751,-23.1172173283856,0.));
#55879=CARTESIAN_POINT('Ctrl Pts',(69.6705709012842,-23.1151740050679,0.));
#55880=CARTESIAN_POINT('Ctrl Pts',(69.6969099184766,-23.1131033674301,0.));
#55881=CARTESIAN_POINT('Ctrl Pts',(69.7232841398207,-23.111005373205,0.));
#55882=CARTESIAN_POINT('Ctrl Pts',(69.7496934674083,-23.1088799803094,0.));
#55883=CARTESIAN_POINT('Ctrl Pts',(69.7761378035978,-23.1067271468615,0.));
#55884=CARTESIAN_POINT('Ctrl Pts',(69.8026170510582,-23.1045468311994,0.));
#55885=CARTESIAN_POINT('Ctrl Pts',(69.8291311128121,-23.1023389919052,0.));
#55886=CARTESIAN_POINT('Ctrl Pts',(69.8556798922687,-23.100103587824,0.));
#55887=CARTESIAN_POINT('Ctrl Pts',(69.8822632932759,-23.0978405781018,0.));
#55888=CARTESIAN_POINT('Ctrl Pts',(69.9088812200703,-23.0955499221556,0.));
#55889=CARTESIAN_POINT('Ctrl Pts',(69.9355335771722,-23.0932315796066,0.));
#55890=CARTESIAN_POINT('Ctrl Pts',(69.9622202692871,-23.0908855102251,0.));
#55891=CARTESIAN_POINT('Ctrl Pts',(69.9889412012143,-23.0885116738799,0.));
#55892=CARTESIAN_POINT('Ctrl Pts',(70.0156962777173,-23.0861100304731,0.));
#55893=CARTESIAN_POINT('Ctrl Pts',(70.0424854035125,-23.0836805399378,0.));
#55894=CARTESIAN_POINT('Ctrl Pts',(70.0693084835387,-23.081223162377,0.));
#55895=CARTESIAN_POINT('Ctrl Pts',(70.096165423165,-23.0787378581778,0.));
#55896=CARTESIAN_POINT('Ctrl Pts',(70.1230561284222,-23.076224588139,0.));
#55897=CARTESIAN_POINT('Ctrl Pts',(70.1499805062159,-23.0736833135934,0.));
#55898=CARTESIAN_POINT('Ctrl Pts',(70.176938464556,-23.0711139965432,0.));
#55899=CARTESIAN_POINT('Ctrl Pts',(70.2039299120456,-23.0685165993682,0.));
#55900=CARTESIAN_POINT('Ctrl Pts',(70.2309547573788,-23.0658910845425,0.));
#55901=CARTESIAN_POINT('Ctrl Pts',(70.2580129087877,-23.0632374143276,0.));
#55902=CARTESIAN_POINT('Ctrl Pts',(70.2851042736081,-23.0605555505326,0.));
#55903=CARTESIAN_POINT('Ctrl Pts',(70.3122287575374,-23.0578454541116,0.));
#55904=CARTESIAN_POINT('Ctrl Pts',(70.3393862652353,-23.0551070854942,0.));
#55905=CARTESIAN_POINT('Ctrl Pts',(70.3665767016596,-23.0523404053188,0.));
#55906=CARTESIAN_POINT('Ctrl Pts',(70.39379997323,-23.0495453750773,0.));
#55907=CARTESIAN_POINT('Ctrl Pts',(70.421055988934,-23.0467219577289,0.));
#55908=CARTESIAN_POINT('Ctrl Pts',(70.4483446617552,-23.0438701184996,0.));
#55909=CARTESIAN_POINT('Ctrl Pts',(70.4756659090104,-23.0409898250727,0.));
#55910=CARTESIAN_POINT('Ctrl Pts',(70.4991133648756,-23.0384964376011,0.));
#55911=CARTESIAN_POINT('Ctrl Pts',(70.5171075702495,-23.0365694096159,0.));
#55912=CARTESIAN_POINT('Ctrl Pts',(70.5296341535253,-23.0352213647764,0.));
#55913=CARTESIAN_POINT('Ctrl Pts',(70.53668363813,-23.034460662331,0.));
#55914=CARTESIAN_POINT('Ctrl Pts',(70.5382514078489,-23.0342913834093,0.));
#55915=CARTESIAN_POINT('',(66.0656156664138,-23.1372951448024,12.));
#55916=CARTESIAN_POINT('',(66.0656156664138,-23.1372951448024,0.));
#55917=CARTESIAN_POINT('Ctrl Pts',(70.5382514078489,-23.0342913834094,12.));
#55918=CARTESIAN_POINT('Ctrl Pts',(70.53668363813,-23.034460662331,12.));
#55919=CARTESIAN_POINT('Ctrl Pts',(70.5296341535253,-23.0352213647764,12.));
#55920=CARTESIAN_POINT('Ctrl Pts',(70.5171075702495,-23.0365694096159,12.));
#55921=CARTESIAN_POINT('Ctrl Pts',(70.4991133648756,-23.0384964376011,12.));
#55922=CARTESIAN_POINT('Ctrl Pts',(70.4756659090104,-23.0409898250727,12.));
#55923=CARTESIAN_POINT('Ctrl Pts',(70.4483446617552,-23.0438701184996,12.));
#55924=CARTESIAN_POINT('Ctrl Pts',(70.421055988934,-23.0467219577289,12.));
#55925=CARTESIAN_POINT('Ctrl Pts',(70.39379997323,-23.0495453750773,12.));
#55926=CARTESIAN_POINT('Ctrl Pts',(70.3665767016596,-23.0523404053188,12.));
#55927=CARTESIAN_POINT('Ctrl Pts',(70.3393862652353,-23.0551070854942,12.));
#55928=CARTESIAN_POINT('Ctrl Pts',(70.3122287575374,-23.0578454541116,12.));
#55929=CARTESIAN_POINT('Ctrl Pts',(70.2851042736081,-23.0605555505326,12.));
#55930=CARTESIAN_POINT('Ctrl Pts',(70.2580129087877,-23.0632374143276,12.));
#55931=CARTESIAN_POINT('Ctrl Pts',(70.2309547573788,-23.0658910845425,12.));
#55932=CARTESIAN_POINT('Ctrl Pts',(70.2039299120456,-23.0685165993682,12.));
#55933=CARTESIAN_POINT('Ctrl Pts',(70.176938464556,-23.0711139965432,12.));
#55934=CARTESIAN_POINT('Ctrl Pts',(70.1499805062159,-23.0736833135934,12.));
#55935=CARTESIAN_POINT('Ctrl Pts',(70.1230561284222,-23.076224588139,12.));
#55936=CARTESIAN_POINT('Ctrl Pts',(70.096165423165,-23.0787378581778,12.));
#55937=CARTESIAN_POINT('Ctrl Pts',(70.0693084835387,-23.081223162377,12.));
#55938=CARTESIAN_POINT('Ctrl Pts',(70.0424854035125,-23.0836805399378,12.));
#55939=CARTESIAN_POINT('Ctrl Pts',(70.0156962777173,-23.0861100304731,12.));
#55940=CARTESIAN_POINT('Ctrl Pts',(69.9889412012143,-23.0885116738799,12.));
#55941=CARTESIAN_POINT('Ctrl Pts',(69.9622202692871,-23.0908855102251,12.));
#55942=CARTESIAN_POINT('Ctrl Pts',(69.9355335771722,-23.0932315796066,12.));
#55943=CARTESIAN_POINT('Ctrl Pts',(69.9088812200703,-23.0955499221556,12.));
#55944=CARTESIAN_POINT('Ctrl Pts',(69.8822632932759,-23.0978405781018,12.));
#55945=CARTESIAN_POINT('Ctrl Pts',(69.8556798922687,-23.100103587824,12.));
#55946=CARTESIAN_POINT('Ctrl Pts',(69.8291311128121,-23.1023389919052,12.));
#55947=CARTESIAN_POINT('Ctrl Pts',(69.8026170510582,-23.1045468311994,12.));
#55948=CARTESIAN_POINT('Ctrl Pts',(69.7761378035978,-23.1067271468615,12.));
#55949=CARTESIAN_POINT('Ctrl Pts',(69.7496934674083,-23.1088799803094,12.));
#55950=CARTESIAN_POINT('Ctrl Pts',(69.7232841398207,-23.111005373205,12.));
#55951=CARTESIAN_POINT('Ctrl Pts',(69.6969099184766,-23.1131033674301,12.));
#55952=CARTESIAN_POINT('Ctrl Pts',(69.6705709012842,-23.1151740050679,12.));
#55953=CARTESIAN_POINT('Ctrl Pts',(69.6442671863751,-23.1172173283856,12.));
#55954=CARTESIAN_POINT('Ctrl Pts',(69.617998872135,-23.1192333798438,12.));
#55955=CARTESIAN_POINT('Ctrl Pts',(69.5917660572255,-23.1212222021049,12.));
#55956=CARTESIAN_POINT('Ctrl Pts',(69.565568840605,-23.1231838380452,12.));
#55957=CARTESIAN_POINT('Ctrl Pts',(69.5394073215467,-23.1251183307678,12.));
#55958=CARTESIAN_POINT('Ctrl Pts',(69.5132815996548,-23.1270257236207,12.));
#55959=CARTESIAN_POINT('Ctrl Pts',(69.4871917748665,-23.1289060601927,12.));
#55960=CARTESIAN_POINT('Ctrl Pts',(69.4611379474491,-23.1307593843063,12.));
#55961=CARTESIAN_POINT('Ctrl Pts',(69.4351202179948,-23.1325857400145,12.));
#55962=CARTESIAN_POINT('Ctrl Pts',(69.4091386874129,-23.1343851715989,12.));
#55963=CARTESIAN_POINT('Ctrl Pts',(69.3831934569176,-23.1361577235708,12.));
#55964=CARTESIAN_POINT('Ctrl Pts',(69.3572846280289,-23.1379034406718,12.));
#55965=CARTESIAN_POINT('Ctrl Pts',(69.3314123025863,-23.1396223678725,12.));
#55966=CARTESIAN_POINT('Ctrl Pts',(69.3055765827544,-23.1413145503763,12.));
#55967=CARTESIAN_POINT('Ctrl Pts',(69.2797775710275,-23.1429800336221,12.));
#55968=CARTESIAN_POINT('Ctrl Pts',(69.2540153702311,-23.1446188632931,12.));
#55969=CARTESIAN_POINT('Ctrl Pts',(69.2282900835234,-23.1462310853205,12.));
#55970=CARTESIAN_POINT('Ctrl Pts',(69.2026018144023,-23.1478167458788,12.));
#55971=CARTESIAN_POINT('Ctrl Pts',(69.176950666708,-23.1493758913857,12.));
#55972=CARTESIAN_POINT('Ctrl Pts',(69.1513367446231,-23.1509085685033,12.));
#55973=CARTESIAN_POINT('Ctrl Pts',(69.1257601526692,-23.1524148241413,12.));
#55974=CARTESIAN_POINT('Ctrl Pts',(69.1002209957036,-23.153894705462,12.));
#55975=CARTESIAN_POINT('Ctrl Pts',(69.0747193789291,-23.1553482598768,12.));
#55976=CARTESIAN_POINT('Ctrl Pts',(69.0492554078999,-23.1567755350472,12.));
#55977=CARTESIAN_POINT('Ctrl Pts',(69.0238291885245,-23.1581765788869,12.));
#55978=CARTESIAN_POINT('Ctrl Pts',(68.9984408270652,-23.1595514395655,12.));
#55979=CARTESIAN_POINT('Ctrl Pts',(68.9730904301362,-23.1609001655154,12.));
#55980=CARTESIAN_POINT('Ctrl Pts',(68.9477781047103,-23.1622228054291,12.));
#55981=CARTESIAN_POINT('Ctrl Pts',(68.9225039581249,-23.1635194082582,12.));
#55982=CARTESIAN_POINT('Ctrl Pts',(68.8972680980844,-23.1647900232152,12.));
#55983=CARTESIAN_POINT('Ctrl Pts',(68.8720706326605,-23.1660346997763,12.));
#55984=CARTESIAN_POINT('Ctrl Pts',(68.8469116702885,-23.1672534876885,12.));
#55985=CARTESIAN_POINT('Ctrl Pts',(68.8217913197735,-23.1684464369681,12.));
#55986=CARTESIAN_POINT('Ctrl Pts',(68.7967096902981,-23.1696135978993,12.));
#55987=CARTESIAN_POINT('Ctrl Pts',(68.7716668914246,-23.1707550210359,12.));
#55988=CARTESIAN_POINT('Ctrl Pts',(68.7466630330968,-23.1718707572047,12.));
#55989=CARTESIAN_POINT('Ctrl Pts',(68.7216982256357,-23.1729608575116,12.));
#55990=CARTESIAN_POINT('Ctrl Pts',(68.6967725797457,-23.1740253733423,12.));
#55991=CARTESIAN_POINT('Ctrl Pts',(68.6718862065227,-23.1750643563606,12.));
#55992=CARTESIAN_POINT('Ctrl Pts',(68.6470392174567,-23.1760778585094,12.));
#55993=CARTESIAN_POINT('Ctrl Pts',(68.6222317244336,-23.1770659320137,12.));
#55994=CARTESIAN_POINT('Ctrl Pts',(68.5974638397322,-23.1780286293873,12.));
#55995=CARTESIAN_POINT('Ctrl Pts',(68.572735676027,-23.178966003434,12.));
#55996=CARTESIAN_POINT('Ctrl Pts',(68.548047346398,-23.1798781072449,12.));
#55997=CARTESIAN_POINT('Ctrl Pts',(68.5233989643343,-23.1807649942011,12.));
#55998=CARTESIAN_POINT('Ctrl Pts',(68.4987906437357,-23.1816267179752,12.));
#55999=CARTESIAN_POINT('Ctrl Pts',(68.4742224989099,-23.1824633325385,12.));
#56000=CARTESIAN_POINT('Ctrl Pts',(68.4496946445756,-23.1832748921629,12.));
#56001=CARTESIAN_POINT('Ctrl Pts',(68.4252071958725,-23.1840614514191,12.));
#56002=CARTESIAN_POINT('Ctrl Pts',(68.4007602683649,-23.1848230651776,12.));
#56003=CARTESIAN_POINT('Ctrl Pts',(68.3763539780442,-23.1855597886117,12.));
#56004=CARTESIAN_POINT('Ctrl Pts',(68.3519884413253,-23.1862716772034,12.));
#56005=CARTESIAN_POINT('Ctrl Pts',(68.3276637750494,-23.1869587867464,12.));
#56006=CARTESIAN_POINT('Ctrl Pts',(68.3033800964946,-23.1876211733439,12.));
#56007=CARTESIAN_POINT('Ctrl Pts',(68.2791375233798,-23.1882588934108,12.));
#56008=CARTESIAN_POINT('Ctrl Pts',(68.2549361738679,-23.1888720036757,12.));
#56009=CARTESIAN_POINT('Ctrl Pts',(68.2307761665629,-23.189460561187,12.));
#56010=CARTESIAN_POINT('Ctrl Pts',(68.2066576205113,-23.1900246233165,12.));
#56011=CARTESIAN_POINT('Ctrl Pts',(68.182580655213,-23.1905642477572,12.));
#56012=CARTESIAN_POINT('Ctrl Pts',(68.1585453906259,-23.1910794925252,12.));
#56013=CARTESIAN_POINT('Ctrl Pts',(68.1345519471695,-23.1915704159624,12.));
#56014=CARTESIAN_POINT('Ctrl Pts',(68.1106004457223,-23.1920370767424,12.));
#56015=CARTESIAN_POINT('Ctrl Pts',(68.086691007624,-23.1924795338746,12.));
#56016=CARTESIAN_POINT('Ctrl Pts',(68.0628237546852,-23.1928978467018,12.));
#56017=CARTESIAN_POINT('Ctrl Pts',(68.0389988091926,-23.1932920749021,12.));
#56018=CARTESIAN_POINT('Ctrl Pts',(68.0152162939123,-23.193662278492,12.));
#56019=CARTESIAN_POINT('Ctrl Pts',(67.9914763320878,-23.194008517832,12.));
#56020=CARTESIAN_POINT('Ctrl Pts',(67.9677790474414,-23.1943308536307,12.));
#56021=CARTESIAN_POINT('Ctrl Pts',(67.944124564187,-23.1946293469437,12.));
#56022=CARTESIAN_POINT('Ctrl Pts',(67.9205130070337,-23.1949040591748,12.));
#56023=CARTESIAN_POINT('Ctrl Pts',(67.8969445011907,-23.19515505208,12.));
#56024=CARTESIAN_POINT('Ctrl Pts',(67.8734191723639,-23.1953823877727,12.));
#56025=CARTESIAN_POINT('Ctrl Pts',(67.8499371467578,-23.1955861287276,12.));
#56026=CARTESIAN_POINT('Ctrl Pts',(67.8264985510884,-23.1957663377798,12.));
#56027=CARTESIAN_POINT('Ctrl Pts',(67.8031035125873,-23.1959230781265,12.));
#56028=CARTESIAN_POINT('Ctrl Pts',(67.7797521590056,-23.1960564133308,12.));
#56029=CARTESIAN_POINT('Ctrl Pts',(67.7564446186115,-23.1961664073274,12.));
#56030=CARTESIAN_POINT('Ctrl Pts',(67.7331810201931,-23.1962531244261,12.));
#56031=CARTESIAN_POINT('Ctrl Pts',(67.7099614930711,-23.1963166293116,12.));
#56032=CARTESIAN_POINT('Ctrl Pts',(67.6867861671044,-23.1963569870457,12.));
#56033=CARTESIAN_POINT('Ctrl Pts',(67.6636551726948,-23.196374263071,12.));
#56034=CARTESIAN_POINT('Ctrl Pts',(67.6405686407828,-23.1963685232176,12.));
#56035=CARTESIAN_POINT('Ctrl Pts',(67.6175267028516,-23.1963398337056,12.));
#56036=CARTESIAN_POINT('Ctrl Pts',(67.5945294909398,-23.1962882611444,12.));
#56037=CARTESIAN_POINT('Ctrl Pts',(67.5715771376454,-23.1962138725358,12.));
#56038=CARTESIAN_POINT('Ctrl Pts',(67.5486697761301,-23.1961167352777,12.));
#56039=CARTESIAN_POINT('Ctrl Pts',(67.525807540117,-23.195996917171,12.));
#56040=CARTESIAN_POINT('Ctrl Pts',(67.5029905638973,-23.1958544864225,12.));
#56041=CARTESIAN_POINT('Ctrl Pts',(67.4802189823423,-23.1956895116446,12.));
#56042=CARTESIAN_POINT('Ctrl Pts',(67.4574929309078,-23.1955020618591,12.));
#56043=CARTESIAN_POINT('Ctrl Pts',(67.4348125456389,-23.1952922065009,12.));
#56044=CARTESIAN_POINT('Ctrl Pts',(67.4121779631666,-23.195060015426,12.));
#56045=CARTESIAN_POINT('Ctrl Pts',(67.3895893207168,-23.1948055589123,12.));
#56046=CARTESIAN_POINT('Ctrl Pts',(67.3670467561205,-23.1945289076608,12.));
#56047=CARTESIAN_POINT('Ctrl Pts',(67.3445504078178,-23.1942301327979,12.));
#56048=CARTESIAN_POINT('Ctrl Pts',(67.3221004148604,-23.1939093058802,12.));
#56049=CARTESIAN_POINT('Ctrl Pts',(67.2996969169099,-23.193566498902,12.));
#56050=CARTESIAN_POINT('Ctrl Pts',(67.2773400542477,-23.1932017842954,12.));
#56051=CARTESIAN_POINT('Ctrl Pts',(67.2550299677888,-23.1928152349344,12.));
#56052=CARTESIAN_POINT('Ctrl Pts',(67.232766799088,-23.1924069241386,12.));
#56053=CARTESIAN_POINT('Ctrl Pts',(67.2105506903448,-23.1919769256804,12.));
#56054=CARTESIAN_POINT('Ctrl Pts',(67.1883817844039,-23.1915253137924,12.));
#56055=CARTESIAN_POINT('Ctrl Pts',(67.1662602247641,-23.1910521631658,12.));
#56056=CARTESIAN_POINT('Ctrl Pts',(67.1441861555819,-23.1905575489506,12.));
#56057=CARTESIAN_POINT('Ctrl Pts',(67.122159721674,-23.1900415467575,12.));
#56058=CARTESIAN_POINT('Ctrl Pts',(67.1001810685137,-23.1895042326626,12.));
#56059=CARTESIAN_POINT('Ctrl Pts',(67.0782503422293,-23.1889456832116,12.));
#56060=CARTESIAN_POINT('Ctrl Pts',(67.0563676896312,-23.1883659754268,12.));
#56061=CARTESIAN_POINT('Ctrl Pts',(67.0345332582297,-23.1877651868155,12.));
#56062=CARTESIAN_POINT('Ctrl Pts',(67.0127471962507,-23.1871433953796,12.));
#56063=CARTESIAN_POINT('Ctrl Pts',(66.9910096526483,-23.1865006796291,12.));
#56064=CARTESIAN_POINT('Ctrl Pts',(66.9693207771058,-23.1858371185852,12.));
#56065=CARTESIAN_POINT('Ctrl Pts',(66.9476807200225,-23.1851527917666,12.));
#56066=CARTESIAN_POINT('Ctrl Pts',(66.9260896324955,-23.1844477791816,12.));
#56067=CARTESIAN_POINT('Ctrl Pts',(66.904547666305,-23.1837221613231,12.));
#56068=CARTESIAN_POINT('Ctrl Pts',(66.8830549738768,-23.1829760191583,12.));
#56069=CARTESIAN_POINT('Ctrl Pts',(66.8616117083304,-23.1822094341508,12.));
#56070=CARTESIAN_POINT('Ctrl Pts',(66.8402180235549,-23.1814224882948,12.));
#56071=CARTESIAN_POINT('Ctrl Pts',(66.8188740742727,-23.1806152641475,12.));
#56072=CARTESIAN_POINT('Ctrl Pts',(66.7975800161014,-23.1797878448645,12.));
#56073=CARTESIAN_POINT('Ctrl Pts',(66.7763360056146,-23.1789403142376,12.));
#56074=CARTESIAN_POINT('Ctrl Pts',(66.7551422002229,-23.1780727566309,12.));
#56075=CARTESIAN_POINT('Ctrl Pts',(66.7339987580441,-23.1771852569137,12.));
#56076=CARTESIAN_POINT('Ctrl Pts',(66.712905837789,-23.1762779004043,12.));
#56077=CARTESIAN_POINT('Ctrl Pts',(66.691863598595,-23.1753507727932,12.));
#56078=CARTESIAN_POINT('Ctrl Pts',(66.6708722000046,-23.174403960137,12.));
#56079=CARTESIAN_POINT('Ctrl Pts',(66.6499318023445,-23.1734375490421,12.));
#56080=CARTESIAN_POINT('Ctrl Pts',(66.6290425670538,-23.1724516268299,12.));
#56081=CARTESIAN_POINT('Ctrl Pts',(66.6082046569657,-23.1714462816794,12.));
#56082=CARTESIAN_POINT('Ctrl Pts',(66.5874182367596,-23.1704216028626,12.));
#56083=CARTESIAN_POINT('Ctrl Pts',(66.5666834726494,-23.169377680588,12.));
#56084=CARTESIAN_POINT('Ctrl Pts',(66.5460005315406,-23.1683146055736,12.));
#56085=CARTESIAN_POINT('Ctrl Pts',(66.5253695803208,-23.1672324686928,12.));
#56086=CARTESIAN_POINT('Ctrl Pts',(66.5047907851318,-23.1661313606123,12.));
#56087=CARTESIAN_POINT('Ctrl Pts',(66.4842643105263,-23.1650113713792,12.));
#56088=CARTESIAN_POINT('Ctrl Pts',(66.4637903210682,-23.163872591218,12.));
#56089=CARTESIAN_POINT('Ctrl Pts',(66.4433689832454,-23.1627151114875,12.));
#56090=CARTESIAN_POINT('Ctrl Pts',(66.4230004670288,-23.1615390254636,12.));
#56091=CARTESIAN_POINT('Ctrl Pts',(66.402684948127,-23.1603444294754,12.));
#56092=CARTESIAN_POINT('Ctrl Pts',(66.382422608185,-23.1591314230101,12.));
#56093=CARTESIAN_POINT('Ctrl Pts',(66.3622136300691,-23.1579001063438,12.));
#56094=CARTESIAN_POINT('Ctrl Pts',(66.3420581937159,-23.1566505784626,12.));
#56095=CARTESIAN_POINT('Ctrl Pts',(66.3219564725161,-23.1553829352531,12.));
#56096=CARTESIAN_POINT('Ctrl Pts',(66.301908627539,-23.154097266617,12.));
#56097=CARTESIAN_POINT('Ctrl Pts',(66.2819148131071,-23.1527936592625,12.));
#56098=CARTESIAN_POINT('Ctrl Pts',(66.2619751878741,-23.1514722022483,12.));
#56099=CARTESIAN_POINT('Ctrl Pts',(66.2420899237317,-23.1501329914488,12.));
#56100=CARTESIAN_POINT('Ctrl Pts',(66.2222592165473,-23.1487761349328,12.));
#56101=CARTESIAN_POINT('Ctrl Pts',(66.2024832934866,-23.1474017566484,12.));
#56102=CARTESIAN_POINT('Ctrl Pts',(66.1827623902899,-23.1460099850763,12.));
#56103=CARTESIAN_POINT('Ctrl Pts',(66.1630967296747,-23.1446009424903,12.));
#56104=CARTESIAN_POINT('Ctrl Pts',(66.1434865015027,-23.1431747350098,12.));
#56105=CARTESIAN_POINT('Ctrl Pts',(66.1239318368548,-23.1417314398398,12.));
#56106=CARTESIAN_POINT('Ctrl Pts',(66.1044328067355,-23.1402711039425,12.));
#56107=CARTESIAN_POINT('Ctrl Pts',(66.088878115242,-23.1390892229779,12.));
#56108=CARTESIAN_POINT('Ctrl Pts',(66.0772371487248,-23.13819515974,12.));
#56109=CARTESIAN_POINT('Ctrl Pts',(66.0694876382126,-23.1375957166104,12.));
#56110=CARTESIAN_POINT('Ctrl Pts',(66.0656156664138,-23.1372951448024,12.));
#56111=CARTESIAN_POINT('Ctrl Pts',(70.9934796069117,-21.5904919935063,-5.55111512312578E-16));
#56112=CARTESIAN_POINT('Ctrl Pts',(70.9934796069117,-21.5904919935063,4.));
#56113=CARTESIAN_POINT('Ctrl Pts',(70.9934796069117,-21.5904919935063,8.));
#56114=CARTESIAN_POINT('Ctrl Pts',(70.9934796069117,-21.5904919935063,12.));
#56115=CARTESIAN_POINT('Ctrl Pts',(71.0762040404458,-21.6628164325802,-5.55111512312578E-16));
#56116=CARTESIAN_POINT('Ctrl Pts',(71.0762040404458,-21.6628164325802,4.));
#56117=CARTESIAN_POINT('Ctrl Pts',(71.0762040404458,-21.6628164325802,8.00000000000001));
#56118=CARTESIAN_POINT('Ctrl Pts',(71.0762040404458,-21.6628164325802,12.));
#56119=CARTESIAN_POINT('Ctrl Pts',(71.1771795679081,-21.8385342042357,-5.55111512312578E-16));
#56120=CARTESIAN_POINT('Ctrl Pts',(71.1771795679081,-21.8385342042357,4.));
#56121=CARTESIAN_POINT('Ctrl Pts',(71.1771795679082,-21.8385342042357,7.99999999999999));
#56122=CARTESIAN_POINT('Ctrl Pts',(71.1771795679082,-21.8385342042357,12.));
#56123=CARTESIAN_POINT('Ctrl Pts',(71.1663065220506,-22.0366423876808,-5.55111512312578E-16));
#56124=CARTESIAN_POINT('Ctrl Pts',(71.1663065220506,-22.0366423876808,4.));
#56125=CARTESIAN_POINT('Ctrl Pts',(71.1663065220506,-22.0366423876808,8.00000000000001));
#56126=CARTESIAN_POINT('Ctrl Pts',(71.1663065220506,-22.0366423876808,12.));
#56127=CARTESIAN_POINT('Ctrl Pts',(71.1418425484891,-22.1153394458689,-5.55111512312578E-16));
#56128=CARTESIAN_POINT('Ctrl Pts',(71.1418425484891,-22.1153394458689,4.));
#56129=CARTESIAN_POINT('Ctrl Pts',(71.1418425484892,-22.1153394458689,8.));
#56130=CARTESIAN_POINT('Ctrl Pts',(71.1418425484892,-22.1153394458689,12.));
#56131=CARTESIAN_POINT('',(70.9934796069117,-21.5904919935063,2.77555756156289E-16));
#56132=CARTESIAN_POINT('',(71.141842548489,-22.1153394458688,0.));
#56133=CARTESIAN_POINT('Ctrl Pts',(70.9934796069117,-21.5904919935063,-1.38777878078145E-16));
#56134=CARTESIAN_POINT('Ctrl Pts',(71.0762040404458,-21.6628164325802,-1.38777878078145E-16));
#56135=CARTESIAN_POINT('Ctrl Pts',(71.1339043418528,-21.7632265878119,-1.38777878078144E-16));
#56136=CARTESIAN_POINT('Ctrl Pts',(71.1550826601351,-21.8709478979137,-1.38777878078145E-16));
#56137=CARTESIAN_POINT('Ctrl Pts',(71.1709663988467,-21.95173888049,-1.38777878078145E-16));
#56138=CARTESIAN_POINT('Ctrl Pts',(71.1663065220506,-22.0366423876808,-1.38777878078145E-16));
#56139=CARTESIAN_POINT('Ctrl Pts',(71.1418425484891,-22.1153394458689,-1.38777878078145E-16));
#56140=CARTESIAN_POINT('',(71.141842548489,-22.1153394458688,12.));
#56141=CARTESIAN_POINT('Ctrl Pts',(71.1418425484891,-22.1153394458689,-5.55111512312578E-16));
#56142=CARTESIAN_POINT('Ctrl Pts',(71.1418425484891,-22.1153394458689,4.));
#56143=CARTESIAN_POINT('Ctrl Pts',(71.1418425484892,-22.1153394458689,8.));
#56144=CARTESIAN_POINT('Ctrl Pts',(71.1418425484892,-22.1153394458689,12.));
#56145=CARTESIAN_POINT('',(70.9934796069117,-21.5904919935063,12.));
#56146=CARTESIAN_POINT('Ctrl Pts',(71.1418425484892,-22.1153394458689,12.));
#56147=CARTESIAN_POINT('Ctrl Pts',(71.1663065220506,-22.0366423876808,12.));
#56148=CARTESIAN_POINT('Ctrl Pts',(71.1709663988467,-21.9517388804901,12.));
#56149=CARTESIAN_POINT('Ctrl Pts',(71.1550826601351,-21.8709478979137,12.));
#56150=CARTESIAN_POINT('Ctrl Pts',(71.1339043418529,-21.7632265878119,12.));
#56151=CARTESIAN_POINT('Ctrl Pts',(71.0762040404458,-21.6628164325802,12.));
#56152=CARTESIAN_POINT('Ctrl Pts',(70.9934796069117,-21.5904919935063,12.));
#56153=CARTESIAN_POINT('Ctrl Pts',(70.9934796069117,-21.5904919935063,12.));
#56154=CARTESIAN_POINT('Ctrl Pts',(70.9934796069117,-21.5904919935063,8.));
#56155=CARTESIAN_POINT('Ctrl Pts',(70.9934796069117,-21.5904919935063,4.));
#56156=CARTESIAN_POINT('Ctrl Pts',(70.9934796069117,-21.5904919935063,-5.55111512312578E-16));
#56157=CARTESIAN_POINT('Origin',(3.57524700084383E-10,-1.12623029467293E-10,
0.));
#56158=CARTESIAN_POINT('Origin',(3.57524700084383E-10,-1.12623029467293E-10,
12.));
#56159=CARTESIAN_POINT('Origin',(3.57524700084383E-10,-1.12623029467293E-10,
0.));
#56160=CARTESIAN_POINT('Ctrl Pts',(68.7132793373328,-28.7877620302391,0.));
#56161=CARTESIAN_POINT('Ctrl Pts',(68.7132793373328,-28.7877620302391,4.));
#56162=CARTESIAN_POINT('Ctrl Pts',(68.7132793373328,-28.7877620302391,8.));
#56163=CARTESIAN_POINT('Ctrl Pts',(68.7132793373328,-28.7877620302391,12.));
#56164=CARTESIAN_POINT('Ctrl Pts',(68.6708193334379,-28.8891094745186,0.));
#56165=CARTESIAN_POINT('Ctrl Pts',(68.6708193334379,-28.8891094745186,4.));
#56166=CARTESIAN_POINT('Ctrl Pts',(68.6708193334379,-28.8891094745186,8.));
#56167=CARTESIAN_POINT('Ctrl Pts',(68.6708193334379,-28.8891094745186,12.));
#56168=CARTESIAN_POINT('Ctrl Pts',(68.5360395709811,-29.0404604348957,0.));
#56169=CARTESIAN_POINT('Ctrl Pts',(68.5360395709811,-29.0404604348957,4.));
#56170=CARTESIAN_POINT('Ctrl Pts',(68.5360395709811,-29.0404604348957,7.99999999999999));
#56171=CARTESIAN_POINT('Ctrl Pts',(68.5360395709811,-29.0404604348957,12.));
#56172=CARTESIAN_POINT('Ctrl Pts',(68.3446561754307,-29.0927805237118,0.));
#56173=CARTESIAN_POINT('Ctrl Pts',(68.3446561754307,-29.0927805237118,4.));
#56174=CARTESIAN_POINT('Ctrl Pts',(68.3446561754307,-29.0927805237118,8.00000000000001));
#56175=CARTESIAN_POINT('Ctrl Pts',(68.3446561754307,-29.0927805237118,12.));
#56176=CARTESIAN_POINT('Ctrl Pts',(68.2622612909744,-29.0944526440248,0.));
#56177=CARTESIAN_POINT('Ctrl Pts',(68.2622612909744,-29.0944526440248,4.));
#56178=CARTESIAN_POINT('Ctrl Pts',(68.2622612909744,-29.0944526440248,8.));
#56179=CARTESIAN_POINT('Ctrl Pts',(68.2622612909744,-29.0944526440248,12.));
#56180=CARTESIAN_POINT('',(68.7132793373328,-28.7877620302391,0.));
#56181=CARTESIAN_POINT('',(68.2622612909744,-29.0944526440249,0.));
#56182=CARTESIAN_POINT('Ctrl Pts',(68.7132793373328,-28.7877620302391,0.));
#56183=CARTESIAN_POINT('Ctrl Pts',(68.6708193334379,-28.8891094745186,0.));
#56184=CARTESIAN_POINT('Ctrl Pts',(68.5938023263198,-28.9755957375912,0.));
#56185=CARTESIAN_POINT('Ctrl Pts',(68.4983025002323,-29.0297453895419,0.));
#56186=CARTESIAN_POINT('Ctrl Pts',(68.4266776306666,-29.0703576285049,0.));
#56187=CARTESIAN_POINT('Ctrl Pts',(68.3446561754307,-29.0927805237118,0.));
#56188=CARTESIAN_POINT('Ctrl Pts',(68.2622612909744,-29.0944526440248,0.));
#56189=CARTESIAN_POINT('',(68.2622612909744,-29.0944526440249,12.));
#56190=CARTESIAN_POINT('Ctrl Pts',(68.2622612909744,-29.0944526440248,0.));
#56191=CARTESIAN_POINT('Ctrl Pts',(68.2622612909744,-29.0944526440248,4.));
#56192=CARTESIAN_POINT('Ctrl Pts',(68.2622612909744,-29.0944526440248,8.));
#56193=CARTESIAN_POINT('Ctrl Pts',(68.2622612909744,-29.0944526440248,12.));
#56194=CARTESIAN_POINT('',(68.7132793373328,-28.7877620302391,12.));
#56195=CARTESIAN_POINT('Ctrl Pts',(68.2622612909744,-29.0944526440248,12.));
#56196=CARTESIAN_POINT('Ctrl Pts',(68.3446561754307,-29.0927805237118,12.));
#56197=CARTESIAN_POINT('Ctrl Pts',(68.4266776306666,-29.0703576285049,12.));
#56198=CARTESIAN_POINT('Ctrl Pts',(68.4983025002323,-29.0297453895419,12.));
#56199=CARTESIAN_POINT('Ctrl Pts',(68.5938023263198,-28.9755957375912,12.));
#56200=CARTESIAN_POINT('Ctrl Pts',(68.6708193334379,-28.8891094745186,12.));
#56201=CARTESIAN_POINT('Ctrl Pts',(68.7132793373328,-28.7877620302391,12.));
#56202=CARTESIAN_POINT('Ctrl Pts',(68.7132793373328,-28.7877620302391,12.));
#56203=CARTESIAN_POINT('Ctrl Pts',(68.7132793373328,-28.7877620302391,8.));
#56204=CARTESIAN_POINT('Ctrl Pts',(68.7132793373328,-28.7877620302391,4.));
#56205=CARTESIAN_POINT('Ctrl Pts',(68.7132793373328,-28.7877620302391,0.));
#56206=CARTESIAN_POINT('Ctrl Pts',(63.7976679095314,-28.8072485549237,0.));
#56207=CARTESIAN_POINT('Ctrl Pts',(63.7976679095314,-28.8072485549237,12.));
#56208=CARTESIAN_POINT('Ctrl Pts',(63.8014989507494,-28.8078854475432,0.));
#56209=CARTESIAN_POINT('Ctrl Pts',(63.8014989507494,-28.8078854475432,12.));
#56210=CARTESIAN_POINT('Ctrl Pts',(63.8091667271231,-28.8091580239553,0.));
#56211=CARTESIAN_POINT('Ctrl Pts',(63.8091667271231,-28.8091580239553,12.));
#56212=CARTESIAN_POINT('Ctrl Pts',(63.8206854735027,-28.8110632620958,0.));
#56213=CARTESIAN_POINT('Ctrl Pts',(63.8206854735027,-28.8110632620958,12.));
#56214=CARTESIAN_POINT('Ctrl Pts',(63.8360779669856,-28.8135963263369,0.));
#56215=CARTESIAN_POINT('Ctrl Pts',(63.8360779669856,-28.8135963263369,12.));
#56216=CARTESIAN_POINT('Ctrl Pts',(63.8553755207486,-28.8167505576681,0.));
#56217=CARTESIAN_POINT('Ctrl Pts',(63.8553755207486,-28.8167505576681,12.));
#56218=CARTESIAN_POINT('Ctrl Pts',(63.8747299825313,-28.8198926619858,0.));
#56219=CARTESIAN_POINT('Ctrl Pts',(63.8747299825313,-28.8198926619858,12.));
#56220=CARTESIAN_POINT('Ctrl Pts',(63.8941412856923,-28.823022586318,0.));
#56221=CARTESIAN_POINT('Ctrl Pts',(63.8941412856923,-28.823022586318,12.));
#56222=CARTESIAN_POINT('Ctrl Pts',(63.9136093063786,-28.8261402423291,0.));
#56223=CARTESIAN_POINT('Ctrl Pts',(63.9136093063786,-28.8261402423291,12.));
#56224=CARTESIAN_POINT('Ctrl Pts',(63.9331338646996,-28.829245507756,0.));
#56225=CARTESIAN_POINT('Ctrl Pts',(63.9331338646996,-28.829245507756,12.));
#56226=CARTESIAN_POINT('Ctrl Pts',(63.9527147494423,-28.8323382413789,0.));
#56227=CARTESIAN_POINT('Ctrl Pts',(63.9527147494423,-28.8323382413789,12.));
#56228=CARTESIAN_POINT('Ctrl Pts',(63.9723517369614,-28.8354182946601,0.));
#56229=CARTESIAN_POINT('Ctrl Pts',(63.9723517369614,-28.8354182946601,12.));
#56230=CARTESIAN_POINT('Ctrl Pts',(63.9920446117582,-28.8384855243243,0.));
#56231=CARTESIAN_POINT('Ctrl Pts',(63.9920446117582,-28.8384855243243,12.));
#56232=CARTESIAN_POINT('Ctrl Pts',(64.0117931881298,-28.8415398056428,0.));
#56233=CARTESIAN_POINT('Ctrl Pts',(64.0117931881298,-28.8415398056428,12.));
#56234=CARTESIAN_POINT('Ctrl Pts',(64.0315973031942,-28.844581028125,0.));
#56235=CARTESIAN_POINT('Ctrl Pts',(64.0315973031942,-28.844581028125,12.));
#56236=CARTESIAN_POINT('Ctrl Pts',(64.0514568066637,-28.8476090892232,0.));
#56237=CARTESIAN_POINT('Ctrl Pts',(64.0514568066637,-28.8476090892232,12.));
#56238=CARTESIAN_POINT('Ctrl Pts',(64.0713715523599,-28.8506238891093,0.));
#56239=CARTESIAN_POINT('Ctrl Pts',(64.0713715523599,-28.8506238891093,12.));
#56240=CARTESIAN_POINT('Ctrl Pts',(64.0913413876622,-28.8536253241854,0.));
#56241=CARTESIAN_POINT('Ctrl Pts',(64.0913413876622,-28.8536253241854,12.));
#56242=CARTESIAN_POINT('Ctrl Pts',(64.1113661481965,-28.8566132838179,0.));
#56243=CARTESIAN_POINT('Ctrl Pts',(64.1113661481965,-28.8566132838179,12.));
#56244=CARTESIAN_POINT('Ctrl Pts',(64.1314456633381,-28.8595876537148,0.));
#56245=CARTESIAN_POINT('Ctrl Pts',(64.1314456633381,-28.8595876537148,12.));
#56246=CARTESIAN_POINT('Ctrl Pts',(64.1515797596564,-28.8625483180438,0.));
#56247=CARTESIAN_POINT('Ctrl Pts',(64.1515797596564,-28.8625483180438,12.));
#56248=CARTESIAN_POINT('Ctrl Pts',(64.1717682648685,-28.8654951618649,0.));
#56249=CARTESIAN_POINT('Ctrl Pts',(64.1717682648685,-28.8654951618649,12.));
#56250=CARTESIAN_POINT('Ctrl Pts',(64.1920110123299,-28.8684280739014,0.));
#56251=CARTESIAN_POINT('Ctrl Pts',(64.1920110123299,-28.8684280739014,12.));
#56252=CARTESIAN_POINT('Ctrl Pts',(64.2123078408461,-28.8713469464185,0.));
#56253=CARTESIAN_POINT('Ctrl Pts',(64.2123078408461,-28.8713469464185,12.));
#56254=CARTESIAN_POINT('Ctrl Pts',(64.2326585925252,-28.8742516738947,0.));
#56255=CARTESIAN_POINT('Ctrl Pts',(64.2326585925252,-28.8742516738947,12.));
#56256=CARTESIAN_POINT('Ctrl Pts',(64.2530631112929,-28.877142152106,0.));
#56257=CARTESIAN_POINT('Ctrl Pts',(64.2530631112929,-28.877142152106,12.));
#56258=CARTESIAN_POINT('Ctrl Pts',(64.273521241071,-28.8800182770065,0.));
#56259=CARTESIAN_POINT('Ctrl Pts',(64.273521241071,-28.8800182770065,12.));
#56260=CARTESIAN_POINT('Ctrl Pts',(64.2940328242521,-28.882879943794,0.));
#56261=CARTESIAN_POINT('Ctrl Pts',(64.2940328242521,-28.882879943794,12.));
#56262=CARTESIAN_POINT('Ctrl Pts',(64.3145977025037,-28.8857270473959,0.));
#56263=CARTESIAN_POINT('Ctrl Pts',(64.3145977025037,-28.8857270473959,12.));
#56264=CARTESIAN_POINT('Ctrl Pts',(64.3352157174619,-28.8885594828926,0.));
#56265=CARTESIAN_POINT('Ctrl Pts',(64.3352157174619,-28.8885594828926,12.));
#56266=CARTESIAN_POINT('Ctrl Pts',(64.3558867114076,-28.8913771459323,0.));
#56267=CARTESIAN_POINT('Ctrl Pts',(64.3558867114076,-28.8913771459323,12.));
#56268=CARTESIAN_POINT('Ctrl Pts',(64.3766105280688,-28.89417993323,0.));
#56269=CARTESIAN_POINT('Ctrl Pts',(64.3766105280688,-28.89417993323,12.));
#56270=CARTESIAN_POINT('Ctrl Pts',(64.3973870129169,-28.8969677427504,0.));
#56271=CARTESIAN_POINT('Ctrl Pts',(64.3973870129169,-28.8969677427504,12.));
#56272=CARTESIAN_POINT('Ctrl Pts',(64.4182160127379,-28.899740473434,0.));
#56273=CARTESIAN_POINT('Ctrl Pts',(64.4182160127379,-28.899740473434,12.));
#56274=CARTESIAN_POINT('Ctrl Pts',(64.4390973753634,-28.9024980250307,0.));
#56275=CARTESIAN_POINT('Ctrl Pts',(64.4390973753634,-28.9024980250307,12.));
#56276=CARTESIAN_POINT('Ctrl Pts',(64.4600309493583,-28.9052402979062,0.));
#56277=CARTESIAN_POINT('Ctrl Pts',(64.4600309493583,-28.9052402979062,12.));
#56278=CARTESIAN_POINT('Ctrl Pts',(64.4810165836592,-28.9079671928264,0.));
#56279=CARTESIAN_POINT('Ctrl Pts',(64.4810165836592,-28.9079671928264,12.));
#56280=CARTESIAN_POINT('Ctrl Pts',(64.5020541275951,-28.910678610965,0.));
#56281=CARTESIAN_POINT('Ctrl Pts',(64.5020541275951,-28.910678610965,12.));
#56282=CARTESIAN_POINT('Ctrl Pts',(64.523143431047,-28.9133744539949,0.));
#56283=CARTESIAN_POINT('Ctrl Pts',(64.523143431047,-28.9133744539949,12.));
#56284=CARTESIAN_POINT('Ctrl Pts',(64.5442843445559,-28.9160546241538,0.));
#56285=CARTESIAN_POINT('Ctrl Pts',(64.5442843445559,-28.9160546241538,12.));
#56286=CARTESIAN_POINT('Ctrl Pts',(64.5654767194471,-28.9187190243224,0.));
#56287=CARTESIAN_POINT('Ctrl Pts',(64.5654767194471,-28.9187190243224,12.));
#56288=CARTESIAN_POINT('Ctrl Pts',(64.5867204079426,-28.9213675580985,0.));
#56289=CARTESIAN_POINT('Ctrl Pts',(64.5867204079426,-28.9213675580985,12.));
#56290=CARTESIAN_POINT('Ctrl Pts',(64.6080152631039,-28.9240001297542,0.));
#56291=CARTESIAN_POINT('Ctrl Pts',(64.6080152631039,-28.9240001297542,12.));
#56292=CARTESIAN_POINT('Ctrl Pts',(64.629361138774,-28.9266166441951,0.));
#56293=CARTESIAN_POINT('Ctrl Pts',(64.629361138774,-28.9266166441951,12.));
#56294=CARTESIAN_POINT('Ctrl Pts',(64.6507578895161,-28.9292170069222,0.));
#56295=CARTESIAN_POINT('Ctrl Pts',(64.6507578895161,-28.9292170069222,12.));
#56296=CARTESIAN_POINT('Ctrl Pts',(64.672205370541,-28.9318011239915,0.));
#56297=CARTESIAN_POINT('Ctrl Pts',(64.672205370541,-28.9318011239915,12.));
#56298=CARTESIAN_POINT('Ctrl Pts',(64.6937034376617,-28.9343689019882,0.));
#56299=CARTESIAN_POINT('Ctrl Pts',(64.6937034376617,-28.9343689019882,12.));
#56300=CARTESIAN_POINT('Ctrl Pts',(64.715251947329,-28.9369202480393,0.));
#56301=CARTESIAN_POINT('Ctrl Pts',(64.715251947329,-28.9369202480393,12.));
#56302=CARTESIAN_POINT('Ctrl Pts',(64.7368507566467,-28.9394550698204,0.));
#56303=CARTESIAN_POINT('Ctrl Pts',(64.7368507566467,-28.9394550698204,12.));
#56304=CARTESIAN_POINT('Ctrl Pts',(64.758499723388,-28.9419732755656,0.));
#56305=CARTESIAN_POINT('Ctrl Pts',(64.758499723388,-28.9419732755656,12.));
#56306=CARTESIAN_POINT('Ctrl Pts',(64.7801987060084,-28.944474774081,0.));
#56307=CARTESIAN_POINT('Ctrl Pts',(64.7801987060084,-28.944474774081,12.));
#56308=CARTESIAN_POINT('Ctrl Pts',(64.8019475636442,-28.9469594747432,0.));
#56309=CARTESIAN_POINT('Ctrl Pts',(64.8019475636442,-28.9469594747432,12.));
#56310=CARTESIAN_POINT('Ctrl Pts',(64.8237461561018,-28.9494272874832,0.));
#56311=CARTESIAN_POINT('Ctrl Pts',(64.8237461561018,-28.9494272874832,12.));
#56312=CARTESIAN_POINT('Ctrl Pts',(64.8455943438423,-28.9518781227765,0.));
#56313=CARTESIAN_POINT('Ctrl Pts',(64.8455943438423,-28.9518781227765,12.));
#56314=CARTESIAN_POINT('Ctrl Pts',(64.8674919879648,-28.9543118916328,0.));
#56315=CARTESIAN_POINT('Ctrl Pts',(64.8674919879648,-28.9543118916328,12.));
#56316=CARTESIAN_POINT('Ctrl Pts',(64.8894389501801,-28.9567285055867,0.));
#56317=CARTESIAN_POINT('Ctrl Pts',(64.8894389501801,-28.9567285055867,12.));
#56318=CARTESIAN_POINT('Ctrl Pts',(64.9114350928125,-28.9591278766934,0.));
#56319=CARTESIAN_POINT('Ctrl Pts',(64.9114350928125,-28.9591278766934,12.));
#56320=CARTESIAN_POINT('Ctrl Pts',(64.9334802788038,-28.961509917525,0.));
#56321=CARTESIAN_POINT('Ctrl Pts',(64.9334802788038,-28.961509917525,12.));
#56322=CARTESIAN_POINT('Ctrl Pts',(64.9555743717109,-28.9638745411677,0.));
#56323=CARTESIAN_POINT('Ctrl Pts',(64.9555743717109,-28.9638745411677,12.));
#56324=CARTESIAN_POINT('Ctrl Pts',(64.9777172357027,-28.9662216612217,0.));
#56325=CARTESIAN_POINT('Ctrl Pts',(64.9777172357027,-28.9662216612217,12.));
#56326=CARTESIAN_POINT('Ctrl Pts',(64.9999087355504,-28.9685511918019,0.));
#56327=CARTESIAN_POINT('Ctrl Pts',(64.9999087355504,-28.9685511918019,12.));
#56328=CARTESIAN_POINT('Ctrl Pts',(65.022148736628,-28.97086304753,0.));
#56329=CARTESIAN_POINT('Ctrl Pts',(65.022148736628,-28.97086304753,12.));
#56330=CARTESIAN_POINT('Ctrl Pts',(65.0444371049082,-28.9731571435283,0.));
#56331=CARTESIAN_POINT('Ctrl Pts',(65.0444371049082,-28.9731571435283,12.));
#56332=CARTESIAN_POINT('Ctrl Pts',(65.0667737069563,-28.9754333954135,0.));
#56333=CARTESIAN_POINT('Ctrl Pts',(65.0667737069563,-28.9754333954135,12.));
#56334=CARTESIAN_POINT('Ctrl Pts',(65.0891584099168,-28.9776917192933,0.));
#56335=CARTESIAN_POINT('Ctrl Pts',(65.0891584099168,-28.9776917192933,12.));
#56336=CARTESIAN_POINT('Ctrl Pts',(65.1115910815037,-28.9799320317641,0.));
#56337=CARTESIAN_POINT('Ctrl Pts',(65.1115910815037,-28.9799320317641,12.));
#56338=CARTESIAN_POINT('Ctrl Pts',(65.1340715900028,-28.9821542499043,0.));
#56339=CARTESIAN_POINT('Ctrl Pts',(65.1340715900028,-28.9821542499043,12.));
#56340=CARTESIAN_POINT('Ctrl Pts',(65.1565998042697,-28.9843582912693,0.));
#56341=CARTESIAN_POINT('Ctrl Pts',(65.1565998042697,-28.9843582912693,12.));
#56342=CARTESIAN_POINT('Ctrl Pts',(65.1791755937256,-28.9865440738884,0.));
#56343=CARTESIAN_POINT('Ctrl Pts',(65.1791755937256,-28.9865440738884,12.));
#56344=CARTESIAN_POINT('Ctrl Pts',(65.2017988283479,-28.9887115162634,0.));
#56345=CARTESIAN_POINT('Ctrl Pts',(65.2017988283479,-28.9887115162634,12.));
#56346=CARTESIAN_POINT('Ctrl Pts',(65.2244693786609,-28.9908605373663,0.));
#56347=CARTESIAN_POINT('Ctrl Pts',(65.2244693786609,-28.9908605373663,12.));
#56348=CARTESIAN_POINT('Ctrl Pts',(65.2471871157397,-28.9929910566325,0.));
#56349=CARTESIAN_POINT('Ctrl Pts',(65.2471871157397,-28.9929910566325,12.));
#56350=CARTESIAN_POINT('Ctrl Pts',(65.2699519112064,-28.9951029939557,0.));
#56351=CARTESIAN_POINT('Ctrl Pts',(65.2699519112064,-28.9951029939557,12.));
#56352=CARTESIAN_POINT('Ctrl Pts',(65.2927636372253,-28.9971962696845,0.));
#56353=CARTESIAN_POINT('Ctrl Pts',(65.2927636372253,-28.9971962696845,12.));
#56354=CARTESIAN_POINT('Ctrl Pts',(65.3156221664916,-28.9992708046212,0.));
#56355=CARTESIAN_POINT('Ctrl Pts',(65.3156221664916,-28.9992708046212,12.));
#56356=CARTESIAN_POINT('Ctrl Pts',(65.3385273722241,-29.0013265200185,0.));
#56357=CARTESIAN_POINT('Ctrl Pts',(65.3385273722241,-29.0013265200185,12.));
#56358=CARTESIAN_POINT('Ctrl Pts',(65.3614791281692,-29.003363337573,0.));
#56359=CARTESIAN_POINT('Ctrl Pts',(65.3614791281692,-29.003363337573,12.));
#56360=CARTESIAN_POINT('Ctrl Pts',(65.3844773085961,-29.0053811794207,0.));
#56361=CARTESIAN_POINT('Ctrl Pts',(65.3844773085961,-29.0053811794207,12.));
#56362=CARTESIAN_POINT('Ctrl Pts',(65.4075217882934,-29.0073799681342,0.));
#56363=CARTESIAN_POINT('Ctrl Pts',(65.4075217882934,-29.0073799681342,12.));
#56364=CARTESIAN_POINT('Ctrl Pts',(65.4306124425562,-29.0093596267216,0.));
#56365=CARTESIAN_POINT('Ctrl Pts',(65.4306124425562,-29.0093596267216,12.));
#56366=CARTESIAN_POINT('Ctrl Pts',(65.4537491471828,-29.0113200786239,0.));
#56367=CARTESIAN_POINT('Ctrl Pts',(65.4537491471828,-29.0113200786239,12.));
#56368=CARTESIAN_POINT('Ctrl Pts',(65.4769317784789,-29.013261247709,0.));
#56369=CARTESIAN_POINT('Ctrl Pts',(65.4769317784789,-29.013261247709,12.));
#56370=CARTESIAN_POINT('Ctrl Pts',(65.5001602132535,-29.0151830582675,0.));
#56371=CARTESIAN_POINT('Ctrl Pts',(65.5001602132535,-29.0151830582675,12.));
#56372=CARTESIAN_POINT('Ctrl Pts',(65.5234343288136,-29.0170854350095,0.));
#56373=CARTESIAN_POINT('Ctrl Pts',(65.5234343288136,-29.0170854350095,12.));
#56374=CARTESIAN_POINT('Ctrl Pts',(65.5467540029514,-29.0189683030642,0.));
#56375=CARTESIAN_POINT('Ctrl Pts',(65.5467540029514,-29.0189683030642,12.));
#56376=CARTESIAN_POINT('Ctrl Pts',(65.5701191139418,-29.0208315879764,0.));
#56377=CARTESIAN_POINT('Ctrl Pts',(65.5701191139418,-29.0208315879764,12.));
#56378=CARTESIAN_POINT('Ctrl Pts',(65.5935295405453,-29.0226752157003,0.));
#56379=CARTESIAN_POINT('Ctrl Pts',(65.5935295405453,-29.0226752157003,12.));
#56380=CARTESIAN_POINT('Ctrl Pts',(65.6169851620046,-29.0244991125959,0.));
#56381=CARTESIAN_POINT('Ctrl Pts',(65.6169851620046,-29.0244991125959,12.));
#56382=CARTESIAN_POINT('Ctrl Pts',(65.6404858580403,-29.0263032054267,0.));
#56383=CARTESIAN_POINT('Ctrl Pts',(65.6404858580403,-29.0263032054267,12.));
#56384=CARTESIAN_POINT('Ctrl Pts',(65.6640315088388,-29.0280874213596,0.));
#56385=CARTESIAN_POINT('Ctrl Pts',(65.6640315088388,-29.0280874213596,12.));
#56386=CARTESIAN_POINT('Ctrl Pts',(65.6876219950493,-29.0298516879612,0.));
#56387=CARTESIAN_POINT('Ctrl Pts',(65.6876219950493,-29.0298516879612,12.));
#56388=CARTESIAN_POINT('Ctrl Pts',(65.7112571977891,-29.0315959331919,0.));
#56389=CARTESIAN_POINT('Ctrl Pts',(65.7112571977891,-29.0315959331919,12.));
#56390=CARTESIAN_POINT('Ctrl Pts',(65.7349369986384,-29.0333200854028,0.));
#56391=CARTESIAN_POINT('Ctrl Pts',(65.7349369986384,-29.0333200854028,12.));
#56392=CARTESIAN_POINT('Ctrl Pts',(65.7586612796368,-29.035024073333,0.));
#56393=CARTESIAN_POINT('Ctrl Pts',(65.7586612796368,-29.035024073333,12.));
#56394=CARTESIAN_POINT('Ctrl Pts',(65.7824299232705,-29.0367078261103,0.));
#56395=CARTESIAN_POINT('Ctrl Pts',(65.7824299232705,-29.0367078261103,12.));
#56396=CARTESIAN_POINT('Ctrl Pts',(65.8062428124713,-29.0383712732469,0.));
#56397=CARTESIAN_POINT('Ctrl Pts',(65.8062428124713,-29.0383712732469,12.));
#56398=CARTESIAN_POINT('Ctrl Pts',(65.8300998306191,-29.0400143446338,0.));
#56399=CARTESIAN_POINT('Ctrl Pts',(65.8300998306191,-29.0400143446338,12.));
#56400=CARTESIAN_POINT('Ctrl Pts',(65.854000861539,-29.0416369705376,0.));
#56401=CARTESIAN_POINT('Ctrl Pts',(65.854000861539,-29.0416369705376,12.));
#56402=CARTESIAN_POINT('Ctrl Pts',(65.8779457894961,-29.0432390815978,0.));
#56403=CARTESIAN_POINT('Ctrl Pts',(65.8779457894961,-29.0432390815978,12.));
#56404=CARTESIAN_POINT('Ctrl Pts',(65.9019344991854,-29.0448206088289,0.));
#56405=CARTESIAN_POINT('Ctrl Pts',(65.9019344991854,-29.0448206088289,12.));
#56406=CARTESIAN_POINT('Ctrl Pts',(65.9259668757306,-29.0463814836158,0.));
#56407=CARTESIAN_POINT('Ctrl Pts',(65.9259668757306,-29.0463814836158,12.));
#56408=CARTESIAN_POINT('Ctrl Pts',(65.9500428046868,-29.0479216377081,0.));
#56409=CARTESIAN_POINT('Ctrl Pts',(65.9500428046868,-29.0479216377081,12.));
#56410=CARTESIAN_POINT('Ctrl Pts',(65.9741621720369,-29.0494410032173,0.));
#56411=CARTESIAN_POINT('Ctrl Pts',(65.9741621720369,-29.0494410032173,12.));
#56412=CARTESIAN_POINT('Ctrl Pts',(65.9983248641879,-29.0509395126143,0.));
#56413=CARTESIAN_POINT('Ctrl Pts',(65.9983248641879,-29.0509395126143,12.));
#56414=CARTESIAN_POINT('Ctrl Pts',(66.0225307679591,-29.0524170987307,0.));
#56415=CARTESIAN_POINT('Ctrl Pts',(66.0225307679591,-29.0524170987307,12.));
#56416=CARTESIAN_POINT('Ctrl Pts',(66.0467797705815,-29.0538736947552,0.));
#56417=CARTESIAN_POINT('Ctrl Pts',(66.0467797705815,-29.0538736947552,12.));
#56418=CARTESIAN_POINT('Ctrl Pts',(66.0710717597009,-29.0553092342279,0.));
#56419=CARTESIAN_POINT('Ctrl Pts',(66.0710717597009,-29.0553092342279,12.));
#56420=CARTESIAN_POINT('Ctrl Pts',(66.0954066233754,-29.0567236510374,0.));
#56421=CARTESIAN_POINT('Ctrl Pts',(66.0954066233754,-29.0567236510374,12.));
#56422=CARTESIAN_POINT('Ctrl Pts',(66.1197842500711,-29.058116879419,0.));
#56423=CARTESIAN_POINT('Ctrl Pts',(66.1197842500711,-29.058116879419,12.));
#56424=CARTESIAN_POINT('Ctrl Pts',(66.1442045286516,-29.0594888539556,0.));
#56425=CARTESIAN_POINT('Ctrl Pts',(66.1442045286516,-29.0594888539556,12.));
#56426=CARTESIAN_POINT('Ctrl Pts',(66.1686673483755,-29.0608395095746,0.));
#56427=CARTESIAN_POINT('Ctrl Pts',(66.1686673483755,-29.0608395095746,12.));
#56428=CARTESIAN_POINT('Ctrl Pts',(66.1931725989008,-29.062168781542,0.));
#56429=CARTESIAN_POINT('Ctrl Pts',(66.1931725989008,-29.062168781542,12.));
#56430=CARTESIAN_POINT('Ctrl Pts',(66.2177201702819,-29.0634766054599,0.));
#56431=CARTESIAN_POINT('Ctrl Pts',(66.2177201702819,-29.0634766054599,12.));
#56432=CARTESIAN_POINT('Ctrl Pts',(66.2423099529668,-29.0647629172645,0.));
#56433=CARTESIAN_POINT('Ctrl Pts',(66.2423099529668,-29.0647629172645,12.));
#56434=CARTESIAN_POINT('Ctrl Pts',(66.2669418377865,-29.0660276532272,0.));
#56435=CARTESIAN_POINT('Ctrl Pts',(66.2669418377865,-29.0660276532272,12.));
#56436=CARTESIAN_POINT('Ctrl Pts',(66.2916157159527,-29.0672707499527,0.));
#56437=CARTESIAN_POINT('Ctrl Pts',(66.2916157159527,-29.0672707499527,12.));
#56438=CARTESIAN_POINT('Ctrl Pts',(66.3163314790607,-29.0684921443718,0.));
#56439=CARTESIAN_POINT('Ctrl Pts',(66.3163314790607,-29.0684921443718,12.));
#56440=CARTESIAN_POINT('Ctrl Pts',(66.3410890190879,-29.0696917737398,0.));
#56441=CARTESIAN_POINT('Ctrl Pts',(66.3410890190879,-29.0696917737398,12.));
#56442=CARTESIAN_POINT('Ctrl Pts',(66.3658882283906,-29.0708695756336,0.));
#56443=CARTESIAN_POINT('Ctrl Pts',(66.3658882283906,-29.0708695756336,12.));
#56444=CARTESIAN_POINT('Ctrl Pts',(66.3907289996942,-29.0720254879535,0.));
#56445=CARTESIAN_POINT('Ctrl Pts',(66.3907289996942,-29.0720254879535,12.));
#56446=CARTESIAN_POINT('Ctrl Pts',(66.4156112260904,-29.0731594489219,0.));
#56447=CARTESIAN_POINT('Ctrl Pts',(66.4156112260904,-29.0731594489219,12.));
#56448=CARTESIAN_POINT('Ctrl Pts',(66.4405348010404,-29.0742713970763,0.));
#56449=CARTESIAN_POINT('Ctrl Pts',(66.4405348010404,-29.0742713970763,12.));
#56450=CARTESIAN_POINT('Ctrl Pts',(66.4654996183739,-29.075361271267,0.));
#56451=CARTESIAN_POINT('Ctrl Pts',(66.4654996183739,-29.075361271267,12.));
#56452=CARTESIAN_POINT('Ctrl Pts',(66.4905055722864,-29.0764290106553,0.));
#56453=CARTESIAN_POINT('Ctrl Pts',(66.4905055722864,-29.0764290106553,12.));
#56454=CARTESIAN_POINT('Ctrl Pts',(66.5155525573308,-29.0774745547146,0.));
#56455=CARTESIAN_POINT('Ctrl Pts',(66.5155525573308,-29.0774745547146,12.));
#56456=CARTESIAN_POINT('Ctrl Pts',(66.5406404684116,-29.0784978432294,0.));
#56457=CARTESIAN_POINT('Ctrl Pts',(66.5406404684116,-29.0784978432294,12.));
#56458=CARTESIAN_POINT('Ctrl Pts',(66.5657692007894,-29.0794988162892,0.));
#56459=CARTESIAN_POINT('Ctrl Pts',(66.5657692007894,-29.0794988162892,12.));
#56460=CARTESIAN_POINT('Ctrl Pts',(66.5909386500796,-29.0804774142852,0.));
#56461=CARTESIAN_POINT('Ctrl Pts',(66.5909386500796,-29.0804774142852,12.));
#56462=CARTESIAN_POINT('Ctrl Pts',(66.6161487122504,-29.0814335779086,0.));
#56463=CARTESIAN_POINT('Ctrl Pts',(66.6161487122504,-29.0814335779086,12.));
#56464=CARTESIAN_POINT('Ctrl Pts',(66.6413992836148,-29.0823672481508,0.));
#56465=CARTESIAN_POINT('Ctrl Pts',(66.6413992836148,-29.0823672481508,12.));
#56466=CARTESIAN_POINT('Ctrl Pts',(66.6666902608246,-29.0832783663049,0.));
#56467=CARTESIAN_POINT('Ctrl Pts',(66.6666902608246,-29.0832783663049,12.));
#56468=CARTESIAN_POINT('Ctrl Pts',(66.6920215408744,-29.0841668739585,0.));
#56469=CARTESIAN_POINT('Ctrl Pts',(66.6920215408744,-29.0841668739585,12.));
#56470=CARTESIAN_POINT('Ctrl Pts',(66.7173930211015,-29.0850327129914,0.));
#56471=CARTESIAN_POINT('Ctrl Pts',(66.7173930211015,-29.0850327129914,12.));
#56472=CARTESIAN_POINT('Ctrl Pts',(66.742804599184,-29.0858758255729,0.));
#56473=CARTESIAN_POINT('Ctrl Pts',(66.742804599184,-29.0858758255729,12.));
#56474=CARTESIAN_POINT('Ctrl Pts',(66.7682561731348,-29.086696154163,0.));
#56475=CARTESIAN_POINT('Ctrl Pts',(66.7682561731348,-29.086696154163,12.));
#56476=CARTESIAN_POINT('Ctrl Pts',(66.7937476412941,-29.0874936415138,0.));
#56477=CARTESIAN_POINT('Ctrl Pts',(66.7937476412941,-29.0874936415138,12.));
#56478=CARTESIAN_POINT('Ctrl Pts',(66.8192789023323,-29.0882682306636,0.));
#56479=CARTESIAN_POINT('Ctrl Pts',(66.8192789023323,-29.0882682306636,12.));
#56480=CARTESIAN_POINT('Ctrl Pts',(66.8448498552508,-29.0890198649327,0.));
#56481=CARTESIAN_POINT('Ctrl Pts',(66.8448498552508,-29.0890198649327,12.));
#56482=CARTESIAN_POINT('Ctrl Pts',(66.8704603993794,-29.0897484879208,0.));
#56483=CARTESIAN_POINT('Ctrl Pts',(66.8704603993794,-29.0897484879208,12.));
#56484=CARTESIAN_POINT('Ctrl Pts',(66.8961104343703,-29.0904540435064,0.));
#56485=CARTESIAN_POINT('Ctrl Pts',(66.8961104343703,-29.0904540435064,12.));
#56486=CARTESIAN_POINT('Ctrl Pts',(66.9217998601881,-29.0911364758484,0.));
#56487=CARTESIAN_POINT('Ctrl Pts',(66.9217998601881,-29.0911364758484,12.));
#56488=CARTESIAN_POINT('Ctrl Pts',(66.9475285771133,-29.0917957293825,0.));
#56489=CARTESIAN_POINT('Ctrl Pts',(66.9475285771133,-29.0917957293825,12.));
#56490=CARTESIAN_POINT('Ctrl Pts',(66.9732964857467,-29.092431748817,0.));
#56491=CARTESIAN_POINT('Ctrl Pts',(66.9732964857467,-29.092431748817,12.));
#56492=CARTESIAN_POINT('Ctrl Pts',(66.9991034870084,-29.0930444791329,0.));
#56493=CARTESIAN_POINT('Ctrl Pts',(66.9991034870084,-29.0930444791329,12.));
#56494=CARTESIAN_POINT('Ctrl Pts',(67.0249494821361,-29.0936338655828,0.));
#56495=CARTESIAN_POINT('Ctrl Pts',(67.0249494821361,-29.0936338655828,12.));
#56496=CARTESIAN_POINT('Ctrl Pts',(67.0508343726771,-29.0941998536958,0.));
#56497=CARTESIAN_POINT('Ctrl Pts',(67.0508343726771,-29.0941998536958,12.));
#56498=CARTESIAN_POINT('Ctrl Pts',(67.0767580604872,-29.0947423892725,0.));
#56499=CARTESIAN_POINT('Ctrl Pts',(67.0767580604872,-29.0947423892725,12.));
#56500=CARTESIAN_POINT('Ctrl Pts',(67.1027204477304,-29.0952614183778,0.));
#56501=CARTESIAN_POINT('Ctrl Pts',(67.1027204477304,-29.0952614183778,12.));
#56502=CARTESIAN_POINT('Ctrl Pts',(67.1287214368743,-29.0957568873358,0.));
#56503=CARTESIAN_POINT('Ctrl Pts',(67.1287214368743,-29.0957568873358,12.));
#56504=CARTESIAN_POINT('Ctrl Pts',(67.1547609306845,-29.0962287427275,0.));
#56505=CARTESIAN_POINT('Ctrl Pts',(67.1547609306845,-29.0962287427275,12.));
#56506=CARTESIAN_POINT('Ctrl Pts',(67.1808388322116,-29.0966769313893,0.));
#56507=CARTESIAN_POINT('Ctrl Pts',(67.1808388322116,-29.0966769313893,12.));
#56508=CARTESIAN_POINT('Ctrl Pts',(67.2069550447895,-29.0971014004135,0.));
#56509=CARTESIAN_POINT('Ctrl Pts',(67.2069550447895,-29.0971014004135,12.));
#56510=CARTESIAN_POINT('Ctrl Pts',(67.2331094720482,-29.0975020971474,0.));
#56511=CARTESIAN_POINT('Ctrl Pts',(67.2331094720482,-29.0975020971474,12.));
#56512=CARTESIAN_POINT('Ctrl Pts',(67.2593020179216,-29.0978789691965,0.));
#56513=CARTESIAN_POINT('Ctrl Pts',(67.2593020179216,-29.0978789691965,12.));
#56514=CARTESIAN_POINT('Ctrl Pts',(67.2855325866516,-29.0982319644277,0.));
#56515=CARTESIAN_POINT('Ctrl Pts',(67.2855325866516,-29.0982319644277,12.));
#56516=CARTESIAN_POINT('Ctrl Pts',(67.311801082791,-29.0985610309768,0.));
#56517=CARTESIAN_POINT('Ctrl Pts',(67.311801082791,-29.0985610309768,12.));
#56518=CARTESIAN_POINT('Ctrl Pts',(67.3381074112013,-29.0988661172526,0.));
#56519=CARTESIAN_POINT('Ctrl Pts',(67.3381074112013,-29.0988661172526,12.));
#56520=CARTESIAN_POINT('Ctrl Pts',(67.3644514770373,-29.0991471719172,0.));
#56521=CARTESIAN_POINT('Ctrl Pts',(67.3644514770373,-29.0991471719172,12.));
#56522=CARTESIAN_POINT('Ctrl Pts',(67.3908331857313,-29.0994041438715,0.));
#56523=CARTESIAN_POINT('Ctrl Pts',(67.3908331857313,-29.0994041438715,12.));
#56524=CARTESIAN_POINT('Ctrl Pts',(67.4172524429726,-29.0996369822418,0.));
#56525=CARTESIAN_POINT('Ctrl Pts',(67.4172524429726,-29.0996369822418,12.));
#56526=CARTESIAN_POINT('Ctrl Pts',(67.4437091546869,-29.0998456363687,0.));
#56527=CARTESIAN_POINT('Ctrl Pts',(67.4437091546869,-29.0998456363687,12.));
#56528=CARTESIAN_POINT('Ctrl Pts',(67.4702032270062,-29.1000300557961,0.));
#56529=CARTESIAN_POINT('Ctrl Pts',(67.4702032270062,-29.1000300557961,12.));
#56530=CARTESIAN_POINT('Ctrl Pts',(67.496734566311,-29.1001901902915,0.));
#56531=CARTESIAN_POINT('Ctrl Pts',(67.496734566311,-29.1001901902915,12.));
#56532=CARTESIAN_POINT('Ctrl Pts',(67.5233030792714,-29.1003259898686,0.));
#56533=CARTESIAN_POINT('Ctrl Pts',(67.5233030792714,-29.1003259898686,12.));
#56534=CARTESIAN_POINT('Ctrl Pts',(67.5499086728891,-29.1004374048149,0.));
#56535=CARTESIAN_POINT('Ctrl Pts',(67.5499086728891,-29.1004374048149,12.));
#56536=CARTESIAN_POINT('Ctrl Pts',(67.5765512545276,-29.1005243857137,0.));
#56537=CARTESIAN_POINT('Ctrl Pts',(67.5765512545276,-29.1005243857137,12.));
#56538=CARTESIAN_POINT('Ctrl Pts',(67.6032307319614,-29.1005868834863,0.));
#56539=CARTESIAN_POINT('Ctrl Pts',(67.6032307319614,-29.1005868834863,12.));
#56540=CARTESIAN_POINT('Ctrl Pts',(67.6299470133286,-29.1006248493577,0.));
#56541=CARTESIAN_POINT('Ctrl Pts',(67.6299470133286,-29.1006248493577,12.));
#56542=CARTESIAN_POINT('Ctrl Pts',(67.6567000070319,-29.1006382347812,0.));
#56543=CARTESIAN_POINT('Ctrl Pts',(67.6567000070319,-29.1006382347812,12.));
#56544=CARTESIAN_POINT('Ctrl Pts',(67.6834896216458,-29.1006269913747,0.));
#56545=CARTESIAN_POINT('Ctrl Pts',(67.6834896216458,-29.1006269913747,12.));
#56546=CARTESIAN_POINT('Ctrl Pts',(67.7103157658296,-29.1005910708625,0.));
#56547=CARTESIAN_POINT('Ctrl Pts',(67.7103157658296,-29.1005910708625,12.));
#56548=CARTESIAN_POINT('Ctrl Pts',(67.7371783482039,-29.1005304249989,0.));
#56549=CARTESIAN_POINT('Ctrl Pts',(67.7371783482039,-29.1005304249989,12.));
#56550=CARTESIAN_POINT('Ctrl Pts',(67.7640772773397,-29.1004450055647,0.));
#56551=CARTESIAN_POINT('Ctrl Pts',(67.7640772773397,-29.1004450055647,12.));
#56552=CARTESIAN_POINT('Ctrl Pts',(67.7910124620148,-29.10033476453,0.));
#56553=CARTESIAN_POINT('Ctrl Pts',(67.7910124620148,-29.10033476453,12.));
#56554=CARTESIAN_POINT('Ctrl Pts',(67.817983811411,-29.1001996541847,0.));
#56555=CARTESIAN_POINT('Ctrl Pts',(67.817983811411,-29.1001996541847,12.));
#56556=CARTESIAN_POINT('Ctrl Pts',(67.844991235333,-29.1000396272868,0.));
#56557=CARTESIAN_POINT('Ctrl Pts',(67.844991235333,-29.1000396272868,12.));
#56558=CARTESIAN_POINT('Ctrl Pts',(67.8720346444111,-29.0998546372027,0.));
#56559=CARTESIAN_POINT('Ctrl Pts',(67.8720346444111,-29.0998546372027,12.));
#56560=CARTESIAN_POINT('Ctrl Pts',(67.8991139503168,-29.0996446380617,0.));
#56561=CARTESIAN_POINT('Ctrl Pts',(67.8991139503168,-29.0996446380617,12.));
#56562=CARTESIAN_POINT('Ctrl Pts',(67.9262290652797,-29.0994095844208,0.));
#56563=CARTESIAN_POINT('Ctrl Pts',(67.9262290652797,-29.0994095844208,12.));
#56564=CARTESIAN_POINT('Ctrl Pts',(67.9533799016122,-29.0991494309395,0.));
#56565=CARTESIAN_POINT('Ctrl Pts',(67.9533799016122,-29.0991494309395,12.));
#56566=CARTESIAN_POINT('Ctrl Pts',(67.9805663711845,-29.0988641320243,0.));
#56567=CARTESIAN_POINT('Ctrl Pts',(67.9805663711845,-29.0988641320243,12.));
#56568=CARTESIAN_POINT('Ctrl Pts',(68.0077883850136,-29.0985536415537,0.));
#56569=CARTESIAN_POINT('Ctrl Pts',(68.0077883850136,-29.0985536415537,12.));
#56570=CARTESIAN_POINT('Ctrl Pts',(68.0350458525589,-29.0982179124113,0.));
#56571=CARTESIAN_POINT('Ctrl Pts',(68.0350458525589,-29.0982179124113,12.));
#56572=CARTESIAN_POINT('Ctrl Pts',(68.0623386822917,-29.0978568968678,0.));
#56573=CARTESIAN_POINT('Ctrl Pts',(68.0623386822917,-29.0978568968678,12.));
#56574=CARTESIAN_POINT('Ctrl Pts',(68.089666782962,-29.0974705474279,0.));
#56575=CARTESIAN_POINT('Ctrl Pts',(68.089666782962,-29.0974705474279,12.));
#56576=CARTESIAN_POINT('Ctrl Pts',(68.1170300647019,-29.0970588175741,0.));
#56577=CARTESIAN_POINT('Ctrl Pts',(68.1170300647019,-29.0970588175741,12.));
#56578=CARTESIAN_POINT('Ctrl Pts',(68.1444284400734,-29.0966216624741,0.));
#56579=CARTESIAN_POINT('Ctrl Pts',(68.1444284400734,-29.0966216624741,12.));
#56580=CARTESIAN_POINT('Ctrl Pts',(68.1718618254221,-29.0961590399024,0.));
#56581=CARTESIAN_POINT('Ctrl Pts',(68.1718618254221,-29.0961590399024,12.));
#56582=CARTESIAN_POINT('Ctrl Pts',(68.1993301411959,-29.0956709104588,0.));
#56583=CARTESIAN_POINT('Ctrl Pts',(68.1993301411959,-29.0956709104588,12.));
#56584=CARTESIAN_POINT('Ctrl Pts',(68.22683330895,-29.0951572355353,0.));
#56585=CARTESIAN_POINT('Ctrl Pts',(68.22683330895,-29.0951572355353,12.));
#56586=CARTESIAN_POINT('Ctrl Pts',(68.2543712489815,-29.0946179757133,0.));
#56587=CARTESIAN_POINT('Ctrl Pts',(68.2543712489815,-29.0946179757133,12.));
#56588=CARTESIAN_POINT('Ctrl Pts',(68.2819438775932,-29.0940530889142,0.));
#56589=CARTESIAN_POINT('Ctrl Pts',(68.2819438775932,-29.0940530889142,12.));
#56590=CARTESIAN_POINT('Ctrl Pts',(68.3095511047852,-29.0934625288442,0.));
#56591=CARTESIAN_POINT('Ctrl Pts',(68.3095511047852,-29.0934625288442,12.));
#56592=CARTESIAN_POINT('Ctrl Pts',(68.3371928310351,-29.0928462428219,0.));
#56593=CARTESIAN_POINT('Ctrl Pts',(68.3371928310351,-29.0928462428219,12.));
#56594=CARTESIAN_POINT('Ctrl Pts',(68.3648689519188,-29.0922041749393,0.));
#56595=CARTESIAN_POINT('Ctrl Pts',(68.3648689519188,-29.0922041749393,12.));
#56596=CARTESIAN_POINT('Ctrl Pts',(68.3925793638241,-29.091536269955,0.));
#56597=CARTESIAN_POINT('Ctrl Pts',(68.3925793638241,-29.091536269955,12.));
#56598=CARTESIAN_POINT('Ctrl Pts',(68.4203239694742,-29.0908424770941,0.));
#56599=CARTESIAN_POINT('Ctrl Pts',(68.4203239694742,-29.0908424770941,12.));
#56600=CARTESIAN_POINT('Ctrl Pts',(68.4481026830845,-29.0901227535274,0.));
#56601=CARTESIAN_POINT('Ctrl Pts',(68.4481026830845,-29.0901227535274,12.));
#56602=CARTESIAN_POINT('Ctrl Pts',(68.4759154367582,-29.0893770688808,0.));
#56603=CARTESIAN_POINT('Ctrl Pts',(68.4759154367582,-29.0893770688808,12.));
#56604=CARTESIAN_POINT('Ctrl Pts',(68.5037621823575,-29.0886054060334,0.));
#56605=CARTESIAN_POINT('Ctrl Pts',(68.5037621823575,-29.0886054060334,12.));
#56606=CARTESIAN_POINT('Ctrl Pts',(68.5316428874729,-29.0878077570819,0.));
#56607=CARTESIAN_POINT('Ctrl Pts',(68.5316428874729,-29.0878077570819,12.));
#56608=CARTESIAN_POINT('Ctrl Pts',(68.5539746037961,-29.0871488478365,0.));
#56609=CARTESIAN_POINT('Ctrl Pts',(68.5539746037961,-29.0871488478365,12.));
#56610=CARTESIAN_POINT('Ctrl Pts',(68.5707386600286,-29.0866429721959,0.));
#56611=CARTESIAN_POINT('Ctrl Pts',(68.5707386600286,-29.0866429721959,12.));
#56612=CARTESIAN_POINT('Ctrl Pts',(68.5819214834609,-29.086300524779,0.));
#56613=CARTESIAN_POINT('Ctrl Pts',(68.5819214834609,-29.086300524779,12.));
#56614=CARTESIAN_POINT('Ctrl Pts',(68.5875145916629,-29.086128001823,0.));
#56615=CARTESIAN_POINT('Ctrl Pts',(68.5875145916629,-29.086128001823,12.));
#56616=CARTESIAN_POINT('',(63.7976679095314,-28.8072485549237,0.));
#56617=CARTESIAN_POINT('Ctrl Pts',(63.7976679095314,-28.8072485549237,0.));
#56618=CARTESIAN_POINT('Ctrl Pts',(63.8014989507494,-28.8078854475432,0.));
#56619=CARTESIAN_POINT('Ctrl Pts',(63.8091667271231,-28.8091580239553,0.));
#56620=CARTESIAN_POINT('Ctrl Pts',(63.8206854735027,-28.8110632620958,0.));
#56621=CARTESIAN_POINT('Ctrl Pts',(63.8360779669856,-28.8135963263369,0.));
#56622=CARTESIAN_POINT('Ctrl Pts',(63.8553755207486,-28.8167505576681,0.));
#56623=CARTESIAN_POINT('Ctrl Pts',(63.8747299825313,-28.8198926619858,0.));
#56624=CARTESIAN_POINT('Ctrl Pts',(63.8941412856923,-28.823022586318,0.));
#56625=CARTESIAN_POINT('Ctrl Pts',(63.9136093063786,-28.8261402423291,0.));
#56626=CARTESIAN_POINT('Ctrl Pts',(63.9331338646996,-28.829245507756,0.));
#56627=CARTESIAN_POINT('Ctrl Pts',(63.9527147494423,-28.8323382413789,0.));
#56628=CARTESIAN_POINT('Ctrl Pts',(63.9723517369614,-28.8354182946601,0.));
#56629=CARTESIAN_POINT('Ctrl Pts',(63.9920446117582,-28.8384855243243,0.));
#56630=CARTESIAN_POINT('Ctrl Pts',(64.0117931881298,-28.8415398056428,0.));
#56631=CARTESIAN_POINT('Ctrl Pts',(64.0315973031942,-28.844581028125,0.));
#56632=CARTESIAN_POINT('Ctrl Pts',(64.0514568066637,-28.8476090892232,0.));
#56633=CARTESIAN_POINT('Ctrl Pts',(64.0713715523599,-28.8506238891093,0.));
#56634=CARTESIAN_POINT('Ctrl Pts',(64.0913413876622,-28.8536253241854,0.));
#56635=CARTESIAN_POINT('Ctrl Pts',(64.1113661481965,-28.8566132838179,0.));
#56636=CARTESIAN_POINT('Ctrl Pts',(64.1314456633381,-28.8595876537148,0.));
#56637=CARTESIAN_POINT('Ctrl Pts',(64.1515797596564,-28.8625483180438,0.));
#56638=CARTESIAN_POINT('Ctrl Pts',(64.1717682648685,-28.8654951618649,0.));
#56639=CARTESIAN_POINT('Ctrl Pts',(64.1920110123299,-28.8684280739014,0.));
#56640=CARTESIAN_POINT('Ctrl Pts',(64.2123078408461,-28.8713469464185,0.));
#56641=CARTESIAN_POINT('Ctrl Pts',(64.2326585925252,-28.8742516738947,0.));
#56642=CARTESIAN_POINT('Ctrl Pts',(64.2530631112929,-28.877142152106,0.));
#56643=CARTESIAN_POINT('Ctrl Pts',(64.273521241071,-28.8800182770065,0.));
#56644=CARTESIAN_POINT('Ctrl Pts',(64.2940328242521,-28.882879943794,0.));
#56645=CARTESIAN_POINT('Ctrl Pts',(64.3145977025037,-28.8857270473959,0.));
#56646=CARTESIAN_POINT('Ctrl Pts',(64.3352157174619,-28.8885594828926,0.));
#56647=CARTESIAN_POINT('Ctrl Pts',(64.3558867114076,-28.8913771459323,0.));
#56648=CARTESIAN_POINT('Ctrl Pts',(64.3766105280688,-28.89417993323,0.));
#56649=CARTESIAN_POINT('Ctrl Pts',(64.3973870129169,-28.8969677427504,0.));
#56650=CARTESIAN_POINT('Ctrl Pts',(64.4182160127379,-28.899740473434,0.));
#56651=CARTESIAN_POINT('Ctrl Pts',(64.4390973753634,-28.9024980250307,0.));
#56652=CARTESIAN_POINT('Ctrl Pts',(64.4600309493583,-28.9052402979062,0.));
#56653=CARTESIAN_POINT('Ctrl Pts',(64.4810165836592,-28.9079671928264,0.));
#56654=CARTESIAN_POINT('Ctrl Pts',(64.5020541275951,-28.910678610965,0.));
#56655=CARTESIAN_POINT('Ctrl Pts',(64.523143431047,-28.9133744539949,0.));
#56656=CARTESIAN_POINT('Ctrl Pts',(64.5442843445559,-28.9160546241538,0.));
#56657=CARTESIAN_POINT('Ctrl Pts',(64.5654767194471,-28.9187190243224,0.));
#56658=CARTESIAN_POINT('Ctrl Pts',(64.5867204079426,-28.9213675580985,0.));
#56659=CARTESIAN_POINT('Ctrl Pts',(64.6080152631039,-28.9240001297542,0.));
#56660=CARTESIAN_POINT('Ctrl Pts',(64.629361138774,-28.9266166441951,0.));
#56661=CARTESIAN_POINT('Ctrl Pts',(64.6507578895161,-28.9292170069222,0.));
#56662=CARTESIAN_POINT('Ctrl Pts',(64.672205370541,-28.9318011239915,0.));
#56663=CARTESIAN_POINT('Ctrl Pts',(64.6937034376617,-28.9343689019882,0.));
#56664=CARTESIAN_POINT('Ctrl Pts',(64.715251947329,-28.9369202480393,0.));
#56665=CARTESIAN_POINT('Ctrl Pts',(64.7368507566467,-28.9394550698204,0.));
#56666=CARTESIAN_POINT('Ctrl Pts',(64.758499723388,-28.9419732755656,0.));
#56667=CARTESIAN_POINT('Ctrl Pts',(64.7801987060084,-28.944474774081,0.));
#56668=CARTESIAN_POINT('Ctrl Pts',(64.8019475636442,-28.9469594747432,0.));
#56669=CARTESIAN_POINT('Ctrl Pts',(64.8237461561018,-28.9494272874832,0.));
#56670=CARTESIAN_POINT('Ctrl Pts',(64.8455943438423,-28.9518781227765,0.));
#56671=CARTESIAN_POINT('Ctrl Pts',(64.8674919879648,-28.9543118916328,0.));
#56672=CARTESIAN_POINT('Ctrl Pts',(64.8894389501801,-28.9567285055867,0.));
#56673=CARTESIAN_POINT('Ctrl Pts',(64.9114350928125,-28.9591278766934,0.));
#56674=CARTESIAN_POINT('Ctrl Pts',(64.9334802788038,-28.961509917525,0.));
#56675=CARTESIAN_POINT('Ctrl Pts',(64.9555743717109,-28.9638745411677,0.));
#56676=CARTESIAN_POINT('Ctrl Pts',(64.9777172357027,-28.9662216612217,0.));
#56677=CARTESIAN_POINT('Ctrl Pts',(64.9999087355504,-28.9685511918019,0.));
#56678=CARTESIAN_POINT('Ctrl Pts',(65.022148736628,-28.97086304753,0.));
#56679=CARTESIAN_POINT('Ctrl Pts',(65.0444371049082,-28.9731571435283,0.));
#56680=CARTESIAN_POINT('Ctrl Pts',(65.0667737069563,-28.9754333954135,0.));
#56681=CARTESIAN_POINT('Ctrl Pts',(65.0891584099168,-28.9776917192933,0.));
#56682=CARTESIAN_POINT('Ctrl Pts',(65.1115910815037,-28.9799320317641,0.));
#56683=CARTESIAN_POINT('Ctrl Pts',(65.1340715900028,-28.9821542499043,0.));
#56684=CARTESIAN_POINT('Ctrl Pts',(65.1565998042697,-28.9843582912693,0.));
#56685=CARTESIAN_POINT('Ctrl Pts',(65.1791755937256,-28.9865440738884,0.));
#56686=CARTESIAN_POINT('Ctrl Pts',(65.2017988283479,-28.9887115162634,0.));
#56687=CARTESIAN_POINT('Ctrl Pts',(65.2244693786609,-28.9908605373663,0.));
#56688=CARTESIAN_POINT('Ctrl Pts',(65.2471871157397,-28.9929910566325,0.));
#56689=CARTESIAN_POINT('Ctrl Pts',(65.2699519112064,-28.9951029939557,0.));
#56690=CARTESIAN_POINT('Ctrl Pts',(65.2927636372253,-28.9971962696845,0.));
#56691=CARTESIAN_POINT('Ctrl Pts',(65.3156221664916,-28.9992708046212,0.));
#56692=CARTESIAN_POINT('Ctrl Pts',(65.3385273722241,-29.0013265200185,0.));
#56693=CARTESIAN_POINT('Ctrl Pts',(65.3614791281692,-29.003363337573,0.));
#56694=CARTESIAN_POINT('Ctrl Pts',(65.3844773085961,-29.0053811794207,0.));
#56695=CARTESIAN_POINT('Ctrl Pts',(65.4075217882934,-29.0073799681342,0.));
#56696=CARTESIAN_POINT('Ctrl Pts',(65.4306124425562,-29.0093596267216,0.));
#56697=CARTESIAN_POINT('Ctrl Pts',(65.4537491471828,-29.0113200786239,0.));
#56698=CARTESIAN_POINT('Ctrl Pts',(65.4769317784789,-29.013261247709,0.));
#56699=CARTESIAN_POINT('Ctrl Pts',(65.5001602132535,-29.0151830582675,0.));
#56700=CARTESIAN_POINT('Ctrl Pts',(65.5234343288136,-29.0170854350095,0.));
#56701=CARTESIAN_POINT('Ctrl Pts',(65.5467540029514,-29.0189683030642,0.));
#56702=CARTESIAN_POINT('Ctrl Pts',(65.5701191139418,-29.0208315879764,0.));
#56703=CARTESIAN_POINT('Ctrl Pts',(65.5935295405453,-29.0226752157003,0.));
#56704=CARTESIAN_POINT('Ctrl Pts',(65.6169851620046,-29.0244991125959,0.));
#56705=CARTESIAN_POINT('Ctrl Pts',(65.6404858580403,-29.0263032054267,0.));
#56706=CARTESIAN_POINT('Ctrl Pts',(65.6640315088388,-29.0280874213596,0.));
#56707=CARTESIAN_POINT('Ctrl Pts',(65.6876219950493,-29.0298516879612,0.));
#56708=CARTESIAN_POINT('Ctrl Pts',(65.7112571977891,-29.0315959331919,0.));
#56709=CARTESIAN_POINT('Ctrl Pts',(65.7349369986384,-29.0333200854028,0.));
#56710=CARTESIAN_POINT('Ctrl Pts',(65.7586612796368,-29.035024073333,0.));
#56711=CARTESIAN_POINT('Ctrl Pts',(65.7824299232705,-29.0367078261103,0.));
#56712=CARTESIAN_POINT('Ctrl Pts',(65.8062428124713,-29.0383712732469,0.));
#56713=CARTESIAN_POINT('Ctrl Pts',(65.8300998306191,-29.0400143446338,0.));
#56714=CARTESIAN_POINT('Ctrl Pts',(65.854000861539,-29.0416369705376,0.));
#56715=CARTESIAN_POINT('Ctrl Pts',(65.8779457894961,-29.0432390815978,0.));
#56716=CARTESIAN_POINT('Ctrl Pts',(65.9019344991854,-29.0448206088289,0.));
#56717=CARTESIAN_POINT('Ctrl Pts',(65.9259668757306,-29.0463814836158,0.));
#56718=CARTESIAN_POINT('Ctrl Pts',(65.9500428046868,-29.0479216377081,0.));
#56719=CARTESIAN_POINT('Ctrl Pts',(65.9741621720369,-29.0494410032173,0.));
#56720=CARTESIAN_POINT('Ctrl Pts',(65.9983248641879,-29.0509395126143,0.));
#56721=CARTESIAN_POINT('Ctrl Pts',(66.0225307679591,-29.0524170987307,0.));
#56722=CARTESIAN_POINT('Ctrl Pts',(66.0467797705815,-29.0538736947552,0.));
#56723=CARTESIAN_POINT('Ctrl Pts',(66.0710717597009,-29.0553092342279,0.));
#56724=CARTESIAN_POINT('Ctrl Pts',(66.0954066233754,-29.0567236510374,0.));
#56725=CARTESIAN_POINT('Ctrl Pts',(66.1197842500711,-29.058116879419,0.));
#56726=CARTESIAN_POINT('Ctrl Pts',(66.1442045286516,-29.0594888539556,0.));
#56727=CARTESIAN_POINT('Ctrl Pts',(66.1686673483755,-29.0608395095746,0.));
#56728=CARTESIAN_POINT('Ctrl Pts',(66.1931725989008,-29.062168781542,0.));
#56729=CARTESIAN_POINT('Ctrl Pts',(66.2177201702819,-29.0634766054599,0.));
#56730=CARTESIAN_POINT('Ctrl Pts',(66.2423099529668,-29.0647629172645,0.));
#56731=CARTESIAN_POINT('Ctrl Pts',(66.2669418377865,-29.0660276532272,0.));
#56732=CARTESIAN_POINT('Ctrl Pts',(66.2916157159527,-29.0672707499527,0.));
#56733=CARTESIAN_POINT('Ctrl Pts',(66.3163314790607,-29.0684921443718,0.));
#56734=CARTESIAN_POINT('Ctrl Pts',(66.3410890190879,-29.0696917737398,0.));
#56735=CARTESIAN_POINT('Ctrl Pts',(66.3658882283906,-29.0708695756336,0.));
#56736=CARTESIAN_POINT('Ctrl Pts',(66.3907289996942,-29.0720254879535,0.));
#56737=CARTESIAN_POINT('Ctrl Pts',(66.4156112260904,-29.0731594489219,0.));
#56738=CARTESIAN_POINT('Ctrl Pts',(66.4405348010404,-29.0742713970763,0.));
#56739=CARTESIAN_POINT('Ctrl Pts',(66.4654996183739,-29.075361271267,0.));
#56740=CARTESIAN_POINT('Ctrl Pts',(66.4905055722864,-29.0764290106553,0.));
#56741=CARTESIAN_POINT('Ctrl Pts',(66.5155525573308,-29.0774745547146,0.));
#56742=CARTESIAN_POINT('Ctrl Pts',(66.5406404684116,-29.0784978432294,0.));
#56743=CARTESIAN_POINT('Ctrl Pts',(66.5657692007894,-29.0794988162892,0.));
#56744=CARTESIAN_POINT('Ctrl Pts',(66.5909386500796,-29.0804774142852,0.));
#56745=CARTESIAN_POINT('Ctrl Pts',(66.6161487122504,-29.0814335779086,0.));
#56746=CARTESIAN_POINT('Ctrl Pts',(66.6413992836148,-29.0823672481508,0.));
#56747=CARTESIAN_POINT('Ctrl Pts',(66.6666902608246,-29.0832783663049,0.));
#56748=CARTESIAN_POINT('Ctrl Pts',(66.6920215408744,-29.0841668739585,0.));
#56749=CARTESIAN_POINT('Ctrl Pts',(66.7173930211015,-29.0850327129914,0.));
#56750=CARTESIAN_POINT('Ctrl Pts',(66.742804599184,-29.0858758255729,0.));
#56751=CARTESIAN_POINT('Ctrl Pts',(66.7682561731348,-29.086696154163,0.));
#56752=CARTESIAN_POINT('Ctrl Pts',(66.7937476412941,-29.0874936415138,0.));
#56753=CARTESIAN_POINT('Ctrl Pts',(66.8192789023323,-29.0882682306636,0.));
#56754=CARTESIAN_POINT('Ctrl Pts',(66.8448498552508,-29.0890198649327,0.));
#56755=CARTESIAN_POINT('Ctrl Pts',(66.8704603993794,-29.0897484879208,0.));
#56756=CARTESIAN_POINT('Ctrl Pts',(66.8961104343703,-29.0904540435064,0.));
#56757=CARTESIAN_POINT('Ctrl Pts',(66.9217998601881,-29.0911364758484,0.));
#56758=CARTESIAN_POINT('Ctrl Pts',(66.9475285771133,-29.0917957293825,0.));
#56759=CARTESIAN_POINT('Ctrl Pts',(66.9732964857467,-29.092431748817,0.));
#56760=CARTESIAN_POINT('Ctrl Pts',(66.9991034870084,-29.0930444791329,0.));
#56761=CARTESIAN_POINT('Ctrl Pts',(67.0249494821361,-29.0936338655828,0.));
#56762=CARTESIAN_POINT('Ctrl Pts',(67.0508343726771,-29.0941998536958,0.));
#56763=CARTESIAN_POINT('Ctrl Pts',(67.0767580604872,-29.0947423892725,0.));
#56764=CARTESIAN_POINT('Ctrl Pts',(67.1027204477304,-29.0952614183778,0.));
#56765=CARTESIAN_POINT('Ctrl Pts',(67.1287214368743,-29.0957568873358,0.));
#56766=CARTESIAN_POINT('Ctrl Pts',(67.1547609306845,-29.0962287427275,0.));
#56767=CARTESIAN_POINT('Ctrl Pts',(67.1808388322116,-29.0966769313893,0.));
#56768=CARTESIAN_POINT('Ctrl Pts',(67.2069550447895,-29.0971014004135,0.));
#56769=CARTESIAN_POINT('Ctrl Pts',(67.2331094720482,-29.0975020971474,0.));
#56770=CARTESIAN_POINT('Ctrl Pts',(67.2593020179216,-29.0978789691965,0.));
#56771=CARTESIAN_POINT('Ctrl Pts',(67.2855325866516,-29.0982319644277,0.));
#56772=CARTESIAN_POINT('Ctrl Pts',(67.311801082791,-29.0985610309768,0.));
#56773=CARTESIAN_POINT('Ctrl Pts',(67.3381074112013,-29.0988661172526,0.));
#56774=CARTESIAN_POINT('Ctrl Pts',(67.3644514770373,-29.0991471719172,0.));
#56775=CARTESIAN_POINT('Ctrl Pts',(67.3908331857313,-29.0994041438715,0.));
#56776=CARTESIAN_POINT('Ctrl Pts',(67.4172524429726,-29.0996369822418,0.));
#56777=CARTESIAN_POINT('Ctrl Pts',(67.4437091546869,-29.0998456363687,0.));
#56778=CARTESIAN_POINT('Ctrl Pts',(67.4702032270062,-29.1000300557961,0.));
#56779=CARTESIAN_POINT('Ctrl Pts',(67.496734566311,-29.1001901902915,0.));
#56780=CARTESIAN_POINT('Ctrl Pts',(67.5233030792714,-29.1003259898686,0.));
#56781=CARTESIAN_POINT('Ctrl Pts',(67.5499086728891,-29.1004374048149,0.));
#56782=CARTESIAN_POINT('Ctrl Pts',(67.5765512545276,-29.1005243857137,0.));
#56783=CARTESIAN_POINT('Ctrl Pts',(67.6032307319614,-29.1005868834863,0.));
#56784=CARTESIAN_POINT('Ctrl Pts',(67.6299470133286,-29.1006248493577,0.));
#56785=CARTESIAN_POINT('Ctrl Pts',(67.6567000070319,-29.1006382347812,0.));
#56786=CARTESIAN_POINT('Ctrl Pts',(67.6834896216458,-29.1006269913747,0.));
#56787=CARTESIAN_POINT('Ctrl Pts',(67.7103157658296,-29.1005910708625,0.));
#56788=CARTESIAN_POINT('Ctrl Pts',(67.7371783482039,-29.1005304249989,0.));
#56789=CARTESIAN_POINT('Ctrl Pts',(67.7640772773397,-29.1004450055647,0.));
#56790=CARTESIAN_POINT('Ctrl Pts',(67.7910124620148,-29.10033476453,0.));
#56791=CARTESIAN_POINT('Ctrl Pts',(67.817983811411,-29.1001996541847,0.));
#56792=CARTESIAN_POINT('Ctrl Pts',(67.844991235333,-29.1000396272868,0.));
#56793=CARTESIAN_POINT('Ctrl Pts',(67.8720346444111,-29.0998546372027,0.));
#56794=CARTESIAN_POINT('Ctrl Pts',(67.8991139503168,-29.0996446380617,0.));
#56795=CARTESIAN_POINT('Ctrl Pts',(67.9262290652797,-29.0994095844208,0.));
#56796=CARTESIAN_POINT('Ctrl Pts',(67.9533799016122,-29.0991494309395,0.));
#56797=CARTESIAN_POINT('Ctrl Pts',(67.9805663711845,-29.0988641320243,0.));
#56798=CARTESIAN_POINT('Ctrl Pts',(68.0077883850136,-29.0985536415537,0.));
#56799=CARTESIAN_POINT('Ctrl Pts',(68.0350458525589,-29.0982179124113,0.));
#56800=CARTESIAN_POINT('Ctrl Pts',(68.0623386822917,-29.0978568968678,0.));
#56801=CARTESIAN_POINT('Ctrl Pts',(68.089666782962,-29.0974705474279,0.));
#56802=CARTESIAN_POINT('Ctrl Pts',(68.1170300647019,-29.0970588175741,0.));
#56803=CARTESIAN_POINT('Ctrl Pts',(68.1444284400734,-29.0966216624741,0.));
#56804=CARTESIAN_POINT('Ctrl Pts',(68.1718618254221,-29.0961590399024,0.));
#56805=CARTESIAN_POINT('Ctrl Pts',(68.1993301411959,-29.0956709104588,0.));
#56806=CARTESIAN_POINT('Ctrl Pts',(68.2229056854495,-29.0952305915108,0.));
#56807=CARTESIAN_POINT('Ctrl Pts',(68.2409993689947,-29.0948791947834,0.));
#56808=CARTESIAN_POINT('Ctrl Pts',(68.2535957746883,-29.0946280433311,0.));
#56809=CARTESIAN_POINT('Ctrl Pts',(68.2606847334624,-29.0944846386549,0.));
#56810=CARTESIAN_POINT('Ctrl Pts',(68.2622612909744,-29.0944526440249,0.));
#56811=CARTESIAN_POINT('',(63.7976679095314,-28.8072485549237,12.));
#56812=CARTESIAN_POINT('',(63.7976679095314,-28.8072485549237,0.));
#56813=CARTESIAN_POINT('Ctrl Pts',(68.2622612909744,-29.0944526440249,12.));
#56814=CARTESIAN_POINT('Ctrl Pts',(68.2606847334624,-29.0944846386549,12.));
#56815=CARTESIAN_POINT('Ctrl Pts',(68.2535957746883,-29.0946280433311,12.));
#56816=CARTESIAN_POINT('Ctrl Pts',(68.2409993689947,-29.0948791947834,12.));
#56817=CARTESIAN_POINT('Ctrl Pts',(68.2229056854495,-29.0952305915108,12.));
#56818=CARTESIAN_POINT('Ctrl Pts',(68.1993301411959,-29.0956709104588,12.));
#56819=CARTESIAN_POINT('Ctrl Pts',(68.1718618254221,-29.0961590399024,12.));
#56820=CARTESIAN_POINT('Ctrl Pts',(68.1444284400734,-29.0966216624741,12.));
#56821=CARTESIAN_POINT('Ctrl Pts',(68.1170300647019,-29.0970588175741,12.));
#56822=CARTESIAN_POINT('Ctrl Pts',(68.089666782962,-29.0974705474279,12.));
#56823=CARTESIAN_POINT('Ctrl Pts',(68.0623386822917,-29.0978568968678,12.));
#56824=CARTESIAN_POINT('Ctrl Pts',(68.0350458525589,-29.0982179124113,12.));
#56825=CARTESIAN_POINT('Ctrl Pts',(68.0077883850136,-29.0985536415537,12.));
#56826=CARTESIAN_POINT('Ctrl Pts',(67.9805663711845,-29.0988641320243,12.));
#56827=CARTESIAN_POINT('Ctrl Pts',(67.9533799016122,-29.0991494309395,12.));
#56828=CARTESIAN_POINT('Ctrl Pts',(67.9262290652797,-29.0994095844208,12.));
#56829=CARTESIAN_POINT('Ctrl Pts',(67.8991139503168,-29.0996446380617,12.));
#56830=CARTESIAN_POINT('Ctrl Pts',(67.8720346444111,-29.0998546372027,12.));
#56831=CARTESIAN_POINT('Ctrl Pts',(67.844991235333,-29.1000396272868,12.));
#56832=CARTESIAN_POINT('Ctrl Pts',(67.817983811411,-29.1001996541847,12.));
#56833=CARTESIAN_POINT('Ctrl Pts',(67.7910124620148,-29.10033476453,12.));
#56834=CARTESIAN_POINT('Ctrl Pts',(67.7640772773397,-29.1004450055647,12.));
#56835=CARTESIAN_POINT('Ctrl Pts',(67.7371783482039,-29.1005304249989,12.));
#56836=CARTESIAN_POINT('Ctrl Pts',(67.7103157658296,-29.1005910708625,12.));
#56837=CARTESIAN_POINT('Ctrl Pts',(67.6834896216458,-29.1006269913747,12.));
#56838=CARTESIAN_POINT('Ctrl Pts',(67.6567000070319,-29.1006382347812,12.));
#56839=CARTESIAN_POINT('Ctrl Pts',(67.6299470133286,-29.1006248493577,12.));
#56840=CARTESIAN_POINT('Ctrl Pts',(67.6032307319614,-29.1005868834863,12.));
#56841=CARTESIAN_POINT('Ctrl Pts',(67.5765512545276,-29.1005243857137,12.));
#56842=CARTESIAN_POINT('Ctrl Pts',(67.5499086728891,-29.1004374048149,12.));
#56843=CARTESIAN_POINT('Ctrl Pts',(67.5233030792714,-29.1003259898686,12.));
#56844=CARTESIAN_POINT('Ctrl Pts',(67.496734566311,-29.1001901902915,12.));
#56845=CARTESIAN_POINT('Ctrl Pts',(67.4702032270062,-29.1000300557961,12.));
#56846=CARTESIAN_POINT('Ctrl Pts',(67.4437091546869,-29.0998456363687,12.));
#56847=CARTESIAN_POINT('Ctrl Pts',(67.4172524429726,-29.0996369822418,12.));
#56848=CARTESIAN_POINT('Ctrl Pts',(67.3908331857313,-29.0994041438715,12.));
#56849=CARTESIAN_POINT('Ctrl Pts',(67.3644514770373,-29.0991471719172,12.));
#56850=CARTESIAN_POINT('Ctrl Pts',(67.3381074112013,-29.0988661172526,12.));
#56851=CARTESIAN_POINT('Ctrl Pts',(67.311801082791,-29.0985610309768,12.));
#56852=CARTESIAN_POINT('Ctrl Pts',(67.2855325866516,-29.0982319644277,12.));
#56853=CARTESIAN_POINT('Ctrl Pts',(67.2593020179216,-29.0978789691965,12.));
#56854=CARTESIAN_POINT('Ctrl Pts',(67.2331094720482,-29.0975020971474,12.));
#56855=CARTESIAN_POINT('Ctrl Pts',(67.2069550447895,-29.0971014004135,12.));
#56856=CARTESIAN_POINT('Ctrl Pts',(67.1808388322116,-29.0966769313893,12.));
#56857=CARTESIAN_POINT('Ctrl Pts',(67.1547609306845,-29.0962287427275,12.));
#56858=CARTESIAN_POINT('Ctrl Pts',(67.1287214368743,-29.0957568873358,12.));
#56859=CARTESIAN_POINT('Ctrl Pts',(67.1027204477304,-29.0952614183778,12.));
#56860=CARTESIAN_POINT('Ctrl Pts',(67.0767580604872,-29.0947423892725,12.));
#56861=CARTESIAN_POINT('Ctrl Pts',(67.0508343726771,-29.0941998536958,12.));
#56862=CARTESIAN_POINT('Ctrl Pts',(67.0249494821361,-29.0936338655828,12.));
#56863=CARTESIAN_POINT('Ctrl Pts',(66.9991034870084,-29.0930444791329,12.));
#56864=CARTESIAN_POINT('Ctrl Pts',(66.9732964857467,-29.092431748817,12.));
#56865=CARTESIAN_POINT('Ctrl Pts',(66.9475285771133,-29.0917957293825,12.));
#56866=CARTESIAN_POINT('Ctrl Pts',(66.9217998601881,-29.0911364758484,12.));
#56867=CARTESIAN_POINT('Ctrl Pts',(66.8961104343703,-29.0904540435064,12.));
#56868=CARTESIAN_POINT('Ctrl Pts',(66.8704603993794,-29.0897484879208,12.));
#56869=CARTESIAN_POINT('Ctrl Pts',(66.8448498552508,-29.0890198649327,12.));
#56870=CARTESIAN_POINT('Ctrl Pts',(66.8192789023323,-29.0882682306636,12.));
#56871=CARTESIAN_POINT('Ctrl Pts',(66.7937476412941,-29.0874936415138,12.));
#56872=CARTESIAN_POINT('Ctrl Pts',(66.7682561731348,-29.086696154163,12.));
#56873=CARTESIAN_POINT('Ctrl Pts',(66.742804599184,-29.0858758255729,12.));
#56874=CARTESIAN_POINT('Ctrl Pts',(66.7173930211015,-29.0850327129914,12.));
#56875=CARTESIAN_POINT('Ctrl Pts',(66.6920215408744,-29.0841668739585,12.));
#56876=CARTESIAN_POINT('Ctrl Pts',(66.6666902608246,-29.0832783663049,12.));
#56877=CARTESIAN_POINT('Ctrl Pts',(66.6413992836148,-29.0823672481508,12.));
#56878=CARTESIAN_POINT('Ctrl Pts',(66.6161487122504,-29.0814335779086,12.));
#56879=CARTESIAN_POINT('Ctrl Pts',(66.5909386500796,-29.0804774142852,12.));
#56880=CARTESIAN_POINT('Ctrl Pts',(66.5657692007894,-29.0794988162892,12.));
#56881=CARTESIAN_POINT('Ctrl Pts',(66.5406404684116,-29.0784978432294,12.));
#56882=CARTESIAN_POINT('Ctrl Pts',(66.5155525573308,-29.0774745547146,12.));
#56883=CARTESIAN_POINT('Ctrl Pts',(66.4905055722864,-29.0764290106553,12.));
#56884=CARTESIAN_POINT('Ctrl Pts',(66.4654996183739,-29.075361271267,12.));
#56885=CARTESIAN_POINT('Ctrl Pts',(66.4405348010404,-29.0742713970763,12.));
#56886=CARTESIAN_POINT('Ctrl Pts',(66.4156112260904,-29.0731594489219,12.));
#56887=CARTESIAN_POINT('Ctrl Pts',(66.3907289996942,-29.0720254879535,12.));
#56888=CARTESIAN_POINT('Ctrl Pts',(66.3658882283906,-29.0708695756336,12.));
#56889=CARTESIAN_POINT('Ctrl Pts',(66.3410890190879,-29.0696917737398,12.));
#56890=CARTESIAN_POINT('Ctrl Pts',(66.3163314790607,-29.0684921443718,12.));
#56891=CARTESIAN_POINT('Ctrl Pts',(66.2916157159527,-29.0672707499527,12.));
#56892=CARTESIAN_POINT('Ctrl Pts',(66.2669418377865,-29.0660276532272,12.));
#56893=CARTESIAN_POINT('Ctrl Pts',(66.2423099529668,-29.0647629172645,12.));
#56894=CARTESIAN_POINT('Ctrl Pts',(66.2177201702819,-29.0634766054599,12.));
#56895=CARTESIAN_POINT('Ctrl Pts',(66.1931725989008,-29.062168781542,12.));
#56896=CARTESIAN_POINT('Ctrl Pts',(66.1686673483755,-29.0608395095746,12.));
#56897=CARTESIAN_POINT('Ctrl Pts',(66.1442045286516,-29.0594888539556,12.));
#56898=CARTESIAN_POINT('Ctrl Pts',(66.1197842500711,-29.058116879419,12.));
#56899=CARTESIAN_POINT('Ctrl Pts',(66.0954066233754,-29.0567236510374,12.));
#56900=CARTESIAN_POINT('Ctrl Pts',(66.0710717597009,-29.0553092342279,12.));
#56901=CARTESIAN_POINT('Ctrl Pts',(66.0467797705815,-29.0538736947552,12.));
#56902=CARTESIAN_POINT('Ctrl Pts',(66.0225307679591,-29.0524170987307,12.));
#56903=CARTESIAN_POINT('Ctrl Pts',(65.9983248641879,-29.0509395126143,12.));
#56904=CARTESIAN_POINT('Ctrl Pts',(65.9741621720369,-29.0494410032173,12.));
#56905=CARTESIAN_POINT('Ctrl Pts',(65.9500428046868,-29.0479216377081,12.));
#56906=CARTESIAN_POINT('Ctrl Pts',(65.9259668757306,-29.0463814836158,12.));
#56907=CARTESIAN_POINT('Ctrl Pts',(65.9019344991854,-29.0448206088289,12.));
#56908=CARTESIAN_POINT('Ctrl Pts',(65.8779457894961,-29.0432390815978,12.));
#56909=CARTESIAN_POINT('Ctrl Pts',(65.854000861539,-29.0416369705376,12.));
#56910=CARTESIAN_POINT('Ctrl Pts',(65.8300998306191,-29.0400143446338,12.));
#56911=CARTESIAN_POINT('Ctrl Pts',(65.8062428124713,-29.0383712732469,12.));
#56912=CARTESIAN_POINT('Ctrl Pts',(65.7824299232705,-29.0367078261103,12.));
#56913=CARTESIAN_POINT('Ctrl Pts',(65.7586612796368,-29.035024073333,12.));
#56914=CARTESIAN_POINT('Ctrl Pts',(65.7349369986384,-29.0333200854028,12.));
#56915=CARTESIAN_POINT('Ctrl Pts',(65.7112571977891,-29.0315959331919,12.));
#56916=CARTESIAN_POINT('Ctrl Pts',(65.6876219950493,-29.0298516879612,12.));
#56917=CARTESIAN_POINT('Ctrl Pts',(65.6640315088388,-29.0280874213596,12.));
#56918=CARTESIAN_POINT('Ctrl Pts',(65.6404858580403,-29.0263032054267,12.));
#56919=CARTESIAN_POINT('Ctrl Pts',(65.6169851620046,-29.0244991125959,12.));
#56920=CARTESIAN_POINT('Ctrl Pts',(65.5935295405453,-29.0226752157003,12.));
#56921=CARTESIAN_POINT('Ctrl Pts',(65.5701191139418,-29.0208315879764,12.));
#56922=CARTESIAN_POINT('Ctrl Pts',(65.5467540029514,-29.0189683030642,12.));
#56923=CARTESIAN_POINT('Ctrl Pts',(65.5234343288136,-29.0170854350095,12.));
#56924=CARTESIAN_POINT('Ctrl Pts',(65.5001602132535,-29.0151830582675,12.));
#56925=CARTESIAN_POINT('Ctrl Pts',(65.4769317784789,-29.013261247709,12.));
#56926=CARTESIAN_POINT('Ctrl Pts',(65.4537491471828,-29.0113200786239,12.));
#56927=CARTESIAN_POINT('Ctrl Pts',(65.4306124425562,-29.0093596267216,12.));
#56928=CARTESIAN_POINT('Ctrl Pts',(65.4075217882934,-29.0073799681342,12.));
#56929=CARTESIAN_POINT('Ctrl Pts',(65.3844773085961,-29.0053811794207,12.));
#56930=CARTESIAN_POINT('Ctrl Pts',(65.3614791281692,-29.003363337573,12.));
#56931=CARTESIAN_POINT('Ctrl Pts',(65.3385273722241,-29.0013265200185,12.));
#56932=CARTESIAN_POINT('Ctrl Pts',(65.3156221664916,-28.9992708046212,12.));
#56933=CARTESIAN_POINT('Ctrl Pts',(65.2927636372253,-28.9971962696845,12.));
#56934=CARTESIAN_POINT('Ctrl Pts',(65.2699519112064,-28.9951029939557,12.));
#56935=CARTESIAN_POINT('Ctrl Pts',(65.2471871157397,-28.9929910566325,12.));
#56936=CARTESIAN_POINT('Ctrl Pts',(65.2244693786609,-28.9908605373663,12.));
#56937=CARTESIAN_POINT('Ctrl Pts',(65.2017988283479,-28.9887115162634,12.));
#56938=CARTESIAN_POINT('Ctrl Pts',(65.1791755937256,-28.9865440738884,12.));
#56939=CARTESIAN_POINT('Ctrl Pts',(65.1565998042697,-28.9843582912693,12.));
#56940=CARTESIAN_POINT('Ctrl Pts',(65.1340715900028,-28.9821542499043,12.));
#56941=CARTESIAN_POINT('Ctrl Pts',(65.1115910815037,-28.9799320317641,12.));
#56942=CARTESIAN_POINT('Ctrl Pts',(65.0891584099168,-28.9776917192933,12.));
#56943=CARTESIAN_POINT('Ctrl Pts',(65.0667737069563,-28.9754333954135,12.));
#56944=CARTESIAN_POINT('Ctrl Pts',(65.0444371049082,-28.9731571435283,12.));
#56945=CARTESIAN_POINT('Ctrl Pts',(65.022148736628,-28.97086304753,12.));
#56946=CARTESIAN_POINT('Ctrl Pts',(64.9999087355504,-28.9685511918019,12.));
#56947=CARTESIAN_POINT('Ctrl Pts',(64.9777172357027,-28.9662216612217,12.));
#56948=CARTESIAN_POINT('Ctrl Pts',(64.9555743717109,-28.9638745411677,12.));
#56949=CARTESIAN_POINT('Ctrl Pts',(64.9334802788038,-28.961509917525,12.));
#56950=CARTESIAN_POINT('Ctrl Pts',(64.9114350928125,-28.9591278766934,12.));
#56951=CARTESIAN_POINT('Ctrl Pts',(64.8894389501801,-28.9567285055867,12.));
#56952=CARTESIAN_POINT('Ctrl Pts',(64.8674919879648,-28.9543118916328,12.));
#56953=CARTESIAN_POINT('Ctrl Pts',(64.8455943438423,-28.9518781227765,12.));
#56954=CARTESIAN_POINT('Ctrl Pts',(64.8237461561018,-28.9494272874832,12.));
#56955=CARTESIAN_POINT('Ctrl Pts',(64.8019475636442,-28.9469594747432,12.));
#56956=CARTESIAN_POINT('Ctrl Pts',(64.7801987060084,-28.944474774081,12.));
#56957=CARTESIAN_POINT('Ctrl Pts',(64.758499723388,-28.9419732755656,12.));
#56958=CARTESIAN_POINT('Ctrl Pts',(64.7368507566467,-28.9394550698204,12.));
#56959=CARTESIAN_POINT('Ctrl Pts',(64.715251947329,-28.9369202480393,12.));
#56960=CARTESIAN_POINT('Ctrl Pts',(64.6937034376617,-28.9343689019882,12.));
#56961=CARTESIAN_POINT('Ctrl Pts',(64.672205370541,-28.9318011239915,12.));
#56962=CARTESIAN_POINT('Ctrl Pts',(64.6507578895161,-28.9292170069222,12.));
#56963=CARTESIAN_POINT('Ctrl Pts',(64.629361138774,-28.9266166441951,12.));
#56964=CARTESIAN_POINT('Ctrl Pts',(64.6080152631039,-28.9240001297542,12.));
#56965=CARTESIAN_POINT('Ctrl Pts',(64.5867204079426,-28.9213675580985,12.));
#56966=CARTESIAN_POINT('Ctrl Pts',(64.5654767194471,-28.9187190243224,12.));
#56967=CARTESIAN_POINT('Ctrl Pts',(64.5442843445559,-28.9160546241538,12.));
#56968=CARTESIAN_POINT('Ctrl Pts',(64.523143431047,-28.9133744539949,12.));
#56969=CARTESIAN_POINT('Ctrl Pts',(64.5020541275951,-28.910678610965,12.));
#56970=CARTESIAN_POINT('Ctrl Pts',(64.4810165836592,-28.9079671928264,12.));
#56971=CARTESIAN_POINT('Ctrl Pts',(64.4600309493583,-28.9052402979062,12.));
#56972=CARTESIAN_POINT('Ctrl Pts',(64.4390973753634,-28.9024980250307,12.));
#56973=CARTESIAN_POINT('Ctrl Pts',(64.4182160127379,-28.899740473434,12.));
#56974=CARTESIAN_POINT('Ctrl Pts',(64.3973870129169,-28.8969677427504,12.));
#56975=CARTESIAN_POINT('Ctrl Pts',(64.3766105280688,-28.89417993323,12.));
#56976=CARTESIAN_POINT('Ctrl Pts',(64.3558867114076,-28.8913771459323,12.));
#56977=CARTESIAN_POINT('Ctrl Pts',(64.3352157174619,-28.8885594828926,12.));
#56978=CARTESIAN_POINT('Ctrl Pts',(64.3145977025037,-28.8857270473959,12.));
#56979=CARTESIAN_POINT('Ctrl Pts',(64.2940328242521,-28.882879943794,12.));
#56980=CARTESIAN_POINT('Ctrl Pts',(64.273521241071,-28.8800182770065,12.));
#56981=CARTESIAN_POINT('Ctrl Pts',(64.2530631112929,-28.877142152106,12.));
#56982=CARTESIAN_POINT('Ctrl Pts',(64.2326585925252,-28.8742516738947,12.));
#56983=CARTESIAN_POINT('Ctrl Pts',(64.2123078408461,-28.8713469464185,12.));
#56984=CARTESIAN_POINT('Ctrl Pts',(64.1920110123299,-28.8684280739014,12.));
#56985=CARTESIAN_POINT('Ctrl Pts',(64.1717682648685,-28.8654951618649,12.));
#56986=CARTESIAN_POINT('Ctrl Pts',(64.1515797596564,-28.8625483180438,12.));
#56987=CARTESIAN_POINT('Ctrl Pts',(64.1314456633381,-28.8595876537148,12.));
#56988=CARTESIAN_POINT('Ctrl Pts',(64.1113661481965,-28.8566132838179,12.));
#56989=CARTESIAN_POINT('Ctrl Pts',(64.0913413876622,-28.8536253241854,12.));
#56990=CARTESIAN_POINT('Ctrl Pts',(64.0713715523599,-28.8506238891093,12.));
#56991=CARTESIAN_POINT('Ctrl Pts',(64.0514568066637,-28.8476090892232,12.));
#56992=CARTESIAN_POINT('Ctrl Pts',(64.0315973031942,-28.844581028125,12.));
#56993=CARTESIAN_POINT('Ctrl Pts',(64.0117931881298,-28.8415398056428,12.));
#56994=CARTESIAN_POINT('Ctrl Pts',(63.9920446117582,-28.8384855243243,12.));
#56995=CARTESIAN_POINT('Ctrl Pts',(63.9723517369614,-28.8354182946601,12.));
#56996=CARTESIAN_POINT('Ctrl Pts',(63.9527147494423,-28.8323382413789,12.));
#56997=CARTESIAN_POINT('Ctrl Pts',(63.9331338646996,-28.829245507756,12.));
#56998=CARTESIAN_POINT('Ctrl Pts',(63.9136093063786,-28.8261402423291,12.));
#56999=CARTESIAN_POINT('Ctrl Pts',(63.8941412856923,-28.823022586318,12.));
#57000=CARTESIAN_POINT('Ctrl Pts',(63.8747299825313,-28.8198926619858,12.));
#57001=CARTESIAN_POINT('Ctrl Pts',(63.8553755207486,-28.8167505576681,12.));
#57002=CARTESIAN_POINT('Ctrl Pts',(63.8360779669856,-28.8135963263369,12.));
#57003=CARTESIAN_POINT('Ctrl Pts',(63.8206854735027,-28.8110632620958,12.));
#57004=CARTESIAN_POINT('Ctrl Pts',(63.8091667271231,-28.8091580239553,12.));
#57005=CARTESIAN_POINT('Ctrl Pts',(63.8014989507494,-28.8078854475432,12.));
#57006=CARTESIAN_POINT('Ctrl Pts',(63.7976679095314,-28.8072485549237,12.));
#57007=CARTESIAN_POINT('Ctrl Pts',(68.8415926175082,-27.6958230985041,-5.55111512312578E-16));
#57008=CARTESIAN_POINT('Ctrl Pts',(68.8415926175082,-27.6958230985041,4.));
#57009=CARTESIAN_POINT('Ctrl Pts',(68.8415926175082,-27.6958230985041,8.));
#57010=CARTESIAN_POINT('Ctrl Pts',(68.8415926175082,-27.6958230985041,12.));
#57011=CARTESIAN_POINT('Ctrl Pts',(68.9176987693914,-27.7750822307,-5.55111512312578E-16));
#57012=CARTESIAN_POINT('Ctrl Pts',(68.9176987693914,-27.7750822307,4.));
#57013=CARTESIAN_POINT('Ctrl Pts',(68.9176987693914,-27.7750822307,8.));
#57014=CARTESIAN_POINT('Ctrl Pts',(68.9176987693914,-27.7750822307,12.));
#57015=CARTESIAN_POINT('Ctrl Pts',(69.0029745467582,-27.9589320265197,-5.55111512312578E-16));
#57016=CARTESIAN_POINT('Ctrl Pts',(69.0029745467582,-27.9589320265197,4.00000000000001));
#57017=CARTESIAN_POINT('Ctrl Pts',(69.0029745467582,-27.9589320265197,7.99999999999999));
#57018=CARTESIAN_POINT('Ctrl Pts',(69.0029745467582,-27.9589320265197,12.));
#57019=CARTESIAN_POINT('Ctrl Pts',(68.9748773050761,-28.1553386138883,-5.55111512312578E-16));
#57020=CARTESIAN_POINT('Ctrl Pts',(68.9748773050761,-28.1553386138883,4.));
#57021=CARTESIAN_POINT('Ctrl Pts',(68.9748773050761,-28.1553386138883,8.00000000000001));
#57022=CARTESIAN_POINT('Ctrl Pts',(68.9748773050761,-28.1553386138883,12.));
#57023=CARTESIAN_POINT('Ctrl Pts',(68.9436475237615,-28.2316040302245,-5.55111512312578E-16));
#57024=CARTESIAN_POINT('Ctrl Pts',(68.9436475237615,-28.2316040302245,4.));
#57025=CARTESIAN_POINT('Ctrl Pts',(68.9436475237615,-28.2316040302245,8.));
#57026=CARTESIAN_POINT('Ctrl Pts',(68.9436475237615,-28.2316040302245,12.));
#57027=CARTESIAN_POINT('',(68.8415926175082,-27.6958230985041,0.));
#57028=CARTESIAN_POINT('',(68.9436475237612,-28.2316040302243,0.));
#57029=CARTESIAN_POINT('Ctrl Pts',(68.8415926175082,-27.6958230985041,-5.55111512312578E-16));
#57030=CARTESIAN_POINT('Ctrl Pts',(68.9176987693914,-27.7750822307,-5.55111512312578E-16));
#57031=CARTESIAN_POINT('Ctrl Pts',(68.9664277850296,-27.8801392568827,-5.55111512312578E-16));
#57032=CARTESIAN_POINT('Ctrl Pts',(68.9781370393457,-27.9892964598977,-5.55111512312578E-16));
#57033=CARTESIAN_POINT('Ctrl Pts',(68.9869189800827,-28.0711643621589,-5.55111512312578E-16));
#57034=CARTESIAN_POINT('Ctrl Pts',(68.9748773050761,-28.1553386138883,-5.55111512312578E-16));
#57035=CARTESIAN_POINT('Ctrl Pts',(68.9436475237615,-28.2316040302245,-5.55111512312578E-16));
#57036=CARTESIAN_POINT('',(68.9436475237612,-28.2316040302243,12.));
#57037=CARTESIAN_POINT('Ctrl Pts',(68.9436475237615,-28.2316040302245,-5.55111512312578E-16));
#57038=CARTESIAN_POINT('Ctrl Pts',(68.9436475237615,-28.2316040302245,4.));
#57039=CARTESIAN_POINT('Ctrl Pts',(68.9436475237615,-28.2316040302245,8.));
#57040=CARTESIAN_POINT('Ctrl Pts',(68.9436475237615,-28.2316040302245,12.));
#57041=CARTESIAN_POINT('',(68.8415926175082,-27.6958230985041,12.));
#57042=CARTESIAN_POINT('Ctrl Pts',(68.9436475237615,-28.2316040302245,12.));
#57043=CARTESIAN_POINT('Ctrl Pts',(68.9748773050761,-28.1553386138883,12.));
#57044=CARTESIAN_POINT('Ctrl Pts',(68.9869189800827,-28.0711643621589,12.));
#57045=CARTESIAN_POINT('Ctrl Pts',(68.9781370393457,-27.9892964598977,12.));
#57046=CARTESIAN_POINT('Ctrl Pts',(68.9664277850296,-27.8801392568827,12.));
#57047=CARTESIAN_POINT('Ctrl Pts',(68.9176987693914,-27.7750822307,12.));
#57048=CARTESIAN_POINT('Ctrl Pts',(68.8415926175082,-27.6958230985041,12.));
#57049=CARTESIAN_POINT('Ctrl Pts',(68.8415926175082,-27.6958230985041,12.));
#57050=CARTESIAN_POINT('Ctrl Pts',(68.8415926175082,-27.6958230985041,8.));
#57051=CARTESIAN_POINT('Ctrl Pts',(68.8415926175082,-27.6958230985041,4.));
#57052=CARTESIAN_POINT('Ctrl Pts',(68.8415926175082,-27.6958230985041,-5.55111512312578E-16));
#57053=CARTESIAN_POINT('Origin',(3.4634846687719E-10,-1.43354795624835E-10,
0.));
#57054=CARTESIAN_POINT('Origin',(3.4634846687719E-10,-1.43354795624835E-10,
12.));
#57055=CARTESIAN_POINT('Origin',(3.4634846687719E-10,-1.43354795624835E-10,
0.));
#57056=CARTESIAN_POINT('Ctrl Pts',(65.9427857825597,-34.6669728017237,-5.55111512312578E-16));
#57057=CARTESIAN_POINT('Ctrl Pts',(65.9427857825597,-34.6669728017237,4.));
#57058=CARTESIAN_POINT('Ctrl Pts',(65.9427857825597,-34.6669728017237,8.));
#57059=CARTESIAN_POINT('Ctrl Pts',(65.9427857825597,-34.6669728017237,12.));
#57060=CARTESIAN_POINT('Ctrl Pts',(65.8916543400169,-34.7642339552035,-5.55111512312578E-16));
#57061=CARTESIAN_POINT('Ctrl Pts',(65.8916543400169,-34.7642339552035,4.));
#57062=CARTESIAN_POINT('Ctrl Pts',(65.8916543400169,-34.7642339552036,8.));
#57063=CARTESIAN_POINT('Ctrl Pts',(65.8916543400169,-34.7642339552036,12.));
#57064=CARTESIAN_POINT('Ctrl Pts',(65.7441961270804,-34.9032616822024,-5.55111512312578E-16));
#57065=CARTESIAN_POINT('Ctrl Pts',(65.7441961270804,-34.9032616822024,4.));
#57066=CARTESIAN_POINT('Ctrl Pts',(65.7441961270804,-34.9032616822024,8.));
#57067=CARTESIAN_POINT('Ctrl Pts',(65.7441961270804,-34.9032616822024,12.));
#57068=CARTESIAN_POINT('Ctrl Pts',(65.5489812297286,-34.9387029822717,-5.55111512312578E-16));
#57069=CARTESIAN_POINT('Ctrl Pts',(65.5489812297286,-34.9387029822717,4.));
#57070=CARTESIAN_POINT('Ctrl Pts',(65.5489812297286,-34.9387029822717,8.));
#57071=CARTESIAN_POINT('Ctrl Pts',(65.5489812297286,-34.9387029822717,12.));
#57072=CARTESIAN_POINT('Ctrl Pts',(65.4667541477954,-34.9331875523087,-5.55111512312578E-16));
#57073=CARTESIAN_POINT('Ctrl Pts',(65.4667541477954,-34.9331875523087,4.));
#57074=CARTESIAN_POINT('Ctrl Pts',(65.4667541477954,-34.9331875523087,8.));
#57075=CARTESIAN_POINT('Ctrl Pts',(65.4667541477954,-34.9331875523087,12.));
#57076=CARTESIAN_POINT('',(65.9427857825597,-34.6669728017237,0.));
#57077=CARTESIAN_POINT('',(65.4667541477955,-34.9331875523085,2.77555756156289E-16));
#57078=CARTESIAN_POINT('Ctrl Pts',(65.9427857825597,-34.6669728017237,-1.38777878078145E-16));
#57079=CARTESIAN_POINT('Ctrl Pts',(65.8916543400169,-34.7642339552035,-1.38777878078145E-16));
#57080=CARTESIAN_POINT('Ctrl Pts',(65.8073925040532,-34.8436783706315,-1.38777878078144E-16));
#57081=CARTESIAN_POINT('Ctrl Pts',(65.7075366486885,-34.8892986466538,-1.38777878078145E-16));
#57082=CARTESIAN_POINT('Ctrl Pts',(65.6326447571651,-34.9235138536706,-1.38777878078145E-16));
#57083=CARTESIAN_POINT('Ctrl Pts',(65.5489812297286,-34.9387029822717,-1.38777878078145E-16));
#57084=CARTESIAN_POINT('Ctrl Pts',(65.4667541477954,-34.9331875523087,-1.38777878078145E-16));
#57085=CARTESIAN_POINT('',(65.4667541477955,-34.9331875523085,12.));
#57086=CARTESIAN_POINT('Ctrl Pts',(65.4667541477954,-34.9331875523087,-5.55111512312578E-16));
#57087=CARTESIAN_POINT('Ctrl Pts',(65.4667541477954,-34.9331875523087,4.));
#57088=CARTESIAN_POINT('Ctrl Pts',(65.4667541477954,-34.9331875523087,8.));
#57089=CARTESIAN_POINT('Ctrl Pts',(65.4667541477954,-34.9331875523087,12.));
#57090=CARTESIAN_POINT('',(65.9427857825597,-34.6669728017237,12.));
#57091=CARTESIAN_POINT('Ctrl Pts',(65.4667541477954,-34.9331875523087,12.));
#57092=CARTESIAN_POINT('Ctrl Pts',(65.5489812297286,-34.9387029822717,12.));
#57093=CARTESIAN_POINT('Ctrl Pts',(65.6326447571651,-34.9235138536706,12.));
#57094=CARTESIAN_POINT('Ctrl Pts',(65.7075366486885,-34.8892986466538,12.));
#57095=CARTESIAN_POINT('Ctrl Pts',(65.8073925040532,-34.8436783706315,12.));
#57096=CARTESIAN_POINT('Ctrl Pts',(65.8916543400169,-34.7642339552036,12.));
#57097=CARTESIAN_POINT('Ctrl Pts',(65.9427857825597,-34.6669728017237,12.));
#57098=CARTESIAN_POINT('Ctrl Pts',(65.9427857825597,-34.6669728017237,12.));
#57099=CARTESIAN_POINT('Ctrl Pts',(65.9427857825597,-34.6669728017237,8.));
#57100=CARTESIAN_POINT('Ctrl Pts',(65.9427857825597,-34.6669728017237,4.));
#57101=CARTESIAN_POINT('Ctrl Pts',(65.9427857825597,-34.6669728017237,-5.55111512312578E-16));
#57102=CARTESIAN_POINT('Ctrl Pts',(61.0441813777723,-34.2579614092497,0.));
#57103=CARTESIAN_POINT('Ctrl Pts',(61.0441813777723,-34.2579614092497,12.));
#57104=CARTESIAN_POINT('Ctrl Pts',(61.0479423318725,-34.2589297755434,0.));
#57105=CARTESIAN_POINT('Ctrl Pts',(61.0479423318725,-34.2589297755434,12.));
#57106=CARTESIAN_POINT('Ctrl Pts',(61.0554700176998,-34.2608658001631,0.));
#57107=CARTESIAN_POINT('Ctrl Pts',(61.0554700176998,-34.2608658001631,12.));
#57108=CARTESIAN_POINT('Ctrl Pts',(61.0667788793266,-34.2637677131935,0.));
#57109=CARTESIAN_POINT('Ctrl Pts',(61.0667788793266,-34.2637677131935,12.));
#57110=CARTESIAN_POINT('Ctrl Pts',(61.0818920286293,-34.2676326825626,0.));
#57111=CARTESIAN_POINT('Ctrl Pts',(61.0818920286293,-34.2676326825626,12.));
#57112=CARTESIAN_POINT('Ctrl Pts',(61.1008412399997,-34.2724568037228,0.));
#57113=CARTESIAN_POINT('Ctrl Pts',(61.1008412399997,-34.2724568037228,12.));
#57114=CARTESIAN_POINT('Ctrl Pts',(61.1198481997764,-34.2772738038771,0.));
#57115=CARTESIAN_POINT('Ctrl Pts',(61.1198481997764,-34.2772738038771,12.));
#57116=CARTESIAN_POINT('Ctrl Pts',(61.1389128461885,-34.282083624447,0.));
#57117=CARTESIAN_POINT('Ctrl Pts',(61.1389128461885,-34.282083624447,12.));
#57118=CARTESIAN_POINT('Ctrl Pts',(61.1580350635532,-34.2868861666384,0.));
#57119=CARTESIAN_POINT('Ctrl Pts',(61.1580350635532,-34.2868861666384,12.));
#57120=CARTESIAN_POINT('Ctrl Pts',(61.1772146833205,-34.2916812929751,0.));
#57121=CARTESIAN_POINT('Ctrl Pts',(61.1772146833205,-34.2916812929751,12.));
#57122=CARTESIAN_POINT('Ctrl Pts',(61.1964515073891,-34.2964688443663,0.));
#57123=CARTESIAN_POINT('Ctrl Pts',(61.1964515073891,-34.2964688443663,12.));
#57124=CARTESIAN_POINT('Ctrl Pts',(61.2157453259107,-34.3012486533474,0.));
#57125=CARTESIAN_POINT('Ctrl Pts',(61.2157453259107,-34.3012486533474,12.));
#57126=CARTESIAN_POINT('Ctrl Pts',(61.2350959366939,-34.3060205584065,0.));
#57127=CARTESIAN_POINT('Ctrl Pts',(61.2350959366939,-34.3060205584065,12.));
#57128=CARTESIAN_POINT('Ctrl Pts',(61.2545031656133,-34.3107844191044,0.));
#57129=CARTESIAN_POINT('Ctrl Pts',(61.2545031656133,-34.3107844191044,12.));
#57130=CARTESIAN_POINT('Ctrl Pts',(61.2739668600365,-34.3155401111747,0.));
#57131=CARTESIAN_POINT('Ctrl Pts',(61.2739668600365,-34.3155401111747,12.));
#57132=CARTESIAN_POINT('Ctrl Pts',(61.2934868791854,-34.3202875193618,0.));
#57133=CARTESIAN_POINT('Ctrl Pts',(61.2934868791854,-34.3202875193618,12.));
#57134=CARTESIAN_POINT('Ctrl Pts',(61.3130630861386,-34.3250265314768,0.));
#57135=CARTESIAN_POINT('Ctrl Pts',(61.3130630861386,-34.3250265314768,12.));
#57136=CARTESIAN_POINT('Ctrl Pts',(61.3326953378851,-34.3297570310146,0.));
#57137=CARTESIAN_POINT('Ctrl Pts',(61.3326953378851,-34.3297570310146,12.));
#57138=CARTESIAN_POINT('Ctrl Pts',(61.3523834803188,-34.3344788934363,0.));
#57139=CARTESIAN_POINT('Ctrl Pts',(61.3523834803188,-34.3344788934363,12.));
#57140=CARTESIAN_POINT('Ctrl Pts',(61.3721273534256,-34.339191990014,0.));
#57141=CARTESIAN_POINT('Ctrl Pts',(61.3721273534256,-34.339191990014,12.));
#57142=CARTESIAN_POINT('Ctrl Pts',(61.3919267945302,-34.3438961902405,0.));
#57143=CARTESIAN_POINT('Ctrl Pts',(61.3919267945302,-34.3438961902405,12.));
#57144=CARTESIAN_POINT('Ctrl Pts',(61.4117816420228,-34.3485913645979,0.));
#57145=CARTESIAN_POINT('Ctrl Pts',(61.4117816420228,-34.3485913645979,12.));
#57146=CARTESIAN_POINT('Ctrl Pts',(61.4316917395918,-34.3532773877089,0.));
#57147=CARTESIAN_POINT('Ctrl Pts',(61.4316917395918,-34.3532773877089,12.));
#57148=CARTESIAN_POINT('Ctrl Pts',(61.4516569360454,-34.3579541381996,0.));
#57149=CARTESIAN_POINT('Ctrl Pts',(61.4516569360454,-34.3579541381996,12.));
#57150=CARTESIAN_POINT('Ctrl Pts',(61.4716770832896,-34.3626214971889,0.));
#57151=CARTESIAN_POINT('Ctrl Pts',(61.4716770832896,-34.3626214971889,12.));
#57152=CARTESIAN_POINT('Ctrl Pts',(61.4917520349278,-34.3672793472466,0.));
#57153=CARTESIAN_POINT('Ctrl Pts',(61.4917520349278,-34.3672793472466,12.));
#57154=CARTESIAN_POINT('Ctrl Pts',(61.5118816445437,-34.3719275711195,0.));
#57155=CARTESIAN_POINT('Ctrl Pts',(61.5118816445437,-34.3719275711195,12.));
#57156=CARTESIAN_POINT('Ctrl Pts',(61.5320657642638,-34.376566050668,0.));
#57157=CARTESIAN_POINT('Ctrl Pts',(61.5320657642638,-34.376566050668,12.));
#57158=CARTESIAN_POINT('Ctrl Pts',(61.5523042455158,-34.3811946674197,0.));
#57159=CARTESIAN_POINT('Ctrl Pts',(61.5523042455158,-34.3811946674197,12.));
#57160=CARTESIAN_POINT('Ctrl Pts',(61.5725969396829,-34.3858133030518,0.));
#57161=CARTESIAN_POINT('Ctrl Pts',(61.5725969396829,-34.3858133030518,12.));
#57162=CARTESIAN_POINT('Ctrl Pts',(61.5929436987409,-34.3904218398637,0.));
#57163=CARTESIAN_POINT('Ctrl Pts',(61.5929436987409,-34.3904218398637,12.));
#57164=CARTESIAN_POINT('Ctrl Pts',(61.6133443760142,-34.3950201613432,0.));
#57165=CARTESIAN_POINT('Ctrl Pts',(61.6133443760142,-34.3950201613432,12.));
#57166=CARTESIAN_POINT('Ctrl Pts',(61.6337988264556,-34.3996081523753,0.));
#57167=CARTESIAN_POINT('Ctrl Pts',(61.6337988264556,-34.3996081523753,12.));
#57168=CARTESIAN_POINT('Ctrl Pts',(61.6543069062416,-34.4041856989317,0.));
#57169=CARTESIAN_POINT('Ctrl Pts',(61.6543069062416,-34.4041856989317,12.));
#57170=CARTESIAN_POINT('Ctrl Pts',(61.6748684725205,-34.4087526878812,0.));
#57171=CARTESIAN_POINT('Ctrl Pts',(61.6748684725205,-34.4087526878812,12.));
#57172=CARTESIAN_POINT('Ctrl Pts',(61.695483383117,-34.4133090067704,0.));
#57173=CARTESIAN_POINT('Ctrl Pts',(61.695483383117,-34.4133090067704,12.));
#57174=CARTESIAN_POINT('Ctrl Pts',(61.7161514961914,-34.4178545435767,0.));
#57175=CARTESIAN_POINT('Ctrl Pts',(61.7161514961914,-34.4178545435767,12.));
#57176=CARTESIAN_POINT('Ctrl Pts',(61.7368726702596,-34.422389186718,0.));
#57177=CARTESIAN_POINT('Ctrl Pts',(61.7368726702596,-34.422389186718,12.));
#57178=CARTESIAN_POINT('Ctrl Pts',(61.7576467643432,-34.4269128251577,0.));
#57179=CARTESIAN_POINT('Ctrl Pts',(61.7576467643432,-34.4269128251577,12.));
#57180=CARTESIAN_POINT('Ctrl Pts',(61.7784736380727,-34.4314253484792,0.));
#57181=CARTESIAN_POINT('Ctrl Pts',(61.7784736380727,-34.4314253484792,12.));
#57182=CARTESIAN_POINT('Ctrl Pts',(61.7993531518036,-34.4359266469749,0.));
#57183=CARTESIAN_POINT('Ctrl Pts',(61.7993531518036,-34.4359266469749,12.));
#57184=CARTESIAN_POINT('Ctrl Pts',(61.8202851667222,-34.4404166117299,0.));
#57185=CARTESIAN_POINT('Ctrl Pts',(61.8202851667222,-34.4404166117299,12.));
#57186=CARTESIAN_POINT('Ctrl Pts',(61.8412695447926,-34.444895134574,0.));
#57187=CARTESIAN_POINT('Ctrl Pts',(61.8412695447926,-34.444895134574,12.));
#57188=CARTESIAN_POINT('Ctrl Pts',(61.8623061487018,-34.4493621080361,0.));
#57189=CARTESIAN_POINT('Ctrl Pts',(61.8623061487018,-34.4493621080361,12.));
#57190=CARTESIAN_POINT('Ctrl Pts',(61.8833948418025,-34.4538174253012,0.));
#57191=CARTESIAN_POINT('Ctrl Pts',(61.8833948418025,-34.4538174253012,12.));
#57192=CARTESIAN_POINT('Ctrl Pts',(61.9045354880444,-34.4582609801637,0.));
#57193=CARTESIAN_POINT('Ctrl Pts',(61.9045354880444,-34.4582609801637,12.));
#57194=CARTESIAN_POINT('Ctrl Pts',(61.9257279519308,-34.4626926669975,0.));
#57195=CARTESIAN_POINT('Ctrl Pts',(61.9257279519308,-34.4626926669975,12.));
#57196=CARTESIAN_POINT('Ctrl Pts',(61.9469720985531,-34.4671123807717,0.));
#57197=CARTESIAN_POINT('Ctrl Pts',(61.9469720985531,-34.4671123807717,12.));
#57198=CARTESIAN_POINT('Ctrl Pts',(61.9682677936053,-34.4715200170592,0.));
#57199=CARTESIAN_POINT('Ctrl Pts',(61.9682677936053,-34.4715200170592,12.));
#57200=CARTESIAN_POINT('Ctrl Pts',(61.9896149034001,-34.4759154720473,0.));
#57201=CARTESIAN_POINT('Ctrl Pts',(61.9896149034001,-34.4759154720473,12.));
#57202=CARTESIAN_POINT('Ctrl Pts',(62.0110132948794,-34.4802986425528,0.));
#57203=CARTESIAN_POINT('Ctrl Pts',(62.0110132948794,-34.4802986425528,12.));
#57204=CARTESIAN_POINT('Ctrl Pts',(62.0324628356141,-34.48466942602,0.));
#57205=CARTESIAN_POINT('Ctrl Pts',(62.0324628356141,-34.48466942602,12.));
#57206=CARTESIAN_POINT('Ctrl Pts',(62.0539633937939,-34.489027720504,0.));
#57207=CARTESIAN_POINT('Ctrl Pts',(62.0539633937939,-34.489027720504,12.));
#57208=CARTESIAN_POINT('Ctrl Pts',(62.0755148382135,-34.4933734246593,0.));
#57209=CARTESIAN_POINT('Ctrl Pts',(62.0755148382135,-34.4933734246593,12.));
#57210=CARTESIAN_POINT('Ctrl Pts',(62.0971170382567,-34.4977064377282,0.));
#57211=CARTESIAN_POINT('Ctrl Pts',(62.0971170382567,-34.4977064377282,12.));
#57212=CARTESIAN_POINT('Ctrl Pts',(62.1187698638707,-34.5020266595293,0.));
#57213=CARTESIAN_POINT('Ctrl Pts',(62.1187698638707,-34.5020266595293,12.));
#57214=CARTESIAN_POINT('Ctrl Pts',(62.1404731855687,-34.5063339904533,0.));
#57215=CARTESIAN_POINT('Ctrl Pts',(62.1404731855687,-34.5063339904533,12.));
#57216=CARTESIAN_POINT('Ctrl Pts',(62.1622268744337,-34.5106283314594,0.));
#57217=CARTESIAN_POINT('Ctrl Pts',(62.1622268744337,-34.5106283314594,12.));
#57218=CARTESIAN_POINT('Ctrl Pts',(62.184030802117,-34.514909584073,0.));
#57219=CARTESIAN_POINT('Ctrl Pts',(62.184030802117,-34.514909584073,12.));
#57220=CARTESIAN_POINT('Ctrl Pts',(62.2058848408346,-34.5191776503843,0.));
#57221=CARTESIAN_POINT('Ctrl Pts',(62.2058848408346,-34.5191776503843,12.));
#57222=CARTESIAN_POINT('Ctrl Pts',(62.2277888633576,-34.5234324330492,0.));
#57223=CARTESIAN_POINT('Ctrl Pts',(62.2277888633576,-34.5234324330492,12.));
#57224=CARTESIAN_POINT('Ctrl Pts',(62.2497427430136,-34.527673835281,0.));
#57225=CARTESIAN_POINT('Ctrl Pts',(62.2497427430136,-34.527673835281,12.));
#57226=CARTESIAN_POINT('Ctrl Pts',(62.2717463536828,-34.5319017608435,0.));
#57227=CARTESIAN_POINT('Ctrl Pts',(62.2717463536828,-34.5319017608435,12.));
#57228=CARTESIAN_POINT('Ctrl Pts',(62.2937995697927,-34.536116114045,0.));
#57229=CARTESIAN_POINT('Ctrl Pts',(62.2937995697927,-34.536116114045,12.));
#57230=CARTESIAN_POINT('Ctrl Pts',(62.3159022663052,-34.5403167997333,0.));
#57231=CARTESIAN_POINT('Ctrl Pts',(62.3159022663052,-34.5403167997333,12.));
#57232=CARTESIAN_POINT('Ctrl Pts',(62.3380543187067,-34.5445037232928,0.));
#57233=CARTESIAN_POINT('Ctrl Pts',(62.3380543187067,-34.5445037232928,12.));
#57234=CARTESIAN_POINT('Ctrl Pts',(62.3602556030114,-34.5486767906376,0.));
#57235=CARTESIAN_POINT('Ctrl Pts',(62.3602556030114,-34.5486767906376,12.));
#57236=CARTESIAN_POINT('Ctrl Pts',(62.3825059957593,-34.552835908207,0.));
#57237=CARTESIAN_POINT('Ctrl Pts',(62.3825059957593,-34.552835908207,12.));
#57238=CARTESIAN_POINT('Ctrl Pts',(62.4048053740129,-34.5569809829615,0.));
#57239=CARTESIAN_POINT('Ctrl Pts',(62.4048053740129,-34.5569809829615,12.));
#57240=CARTESIAN_POINT('Ctrl Pts',(62.4271536153473,-34.5611119223807,0.));
#57241=CARTESIAN_POINT('Ctrl Pts',(62.4271536153473,-34.5611119223807,12.));
#57242=CARTESIAN_POINT('Ctrl Pts',(62.4495505978415,-34.5652286344606,0.));
#57243=CARTESIAN_POINT('Ctrl Pts',(62.4495505978415,-34.5652286344606,12.));
#57244=CARTESIAN_POINT('Ctrl Pts',(62.4719962000829,-34.5693310277064,0.));
#57245=CARTESIAN_POINT('Ctrl Pts',(62.4719962000829,-34.5693310277064,12.));
#57246=CARTESIAN_POINT('Ctrl Pts',(62.494490301164,-34.5734190111279,0.));
#57247=CARTESIAN_POINT('Ctrl Pts',(62.494490301164,-34.5734190111279,12.));
#57248=CARTESIAN_POINT('Ctrl Pts',(62.5170327806774,-34.5774924942351,0.));
#57249=CARTESIAN_POINT('Ctrl Pts',(62.5170327806774,-34.5774924942351,12.));
#57250=CARTESIAN_POINT('Ctrl Pts',(62.5396235187053,-34.5815513870363,0.));
#57251=CARTESIAN_POINT('Ctrl Pts',(62.5396235187053,-34.5815513870363,12.));
#57252=CARTESIAN_POINT('Ctrl Pts',(62.5622623958125,-34.5855956000344,0.));
#57253=CARTESIAN_POINT('Ctrl Pts',(62.5622623958125,-34.5855956000344,12.));
#57254=CARTESIAN_POINT('Ctrl Pts',(62.5849492930501,-34.5896250442199,0.));
#57255=CARTESIAN_POINT('Ctrl Pts',(62.5849492930501,-34.5896250442199,12.));
#57256=CARTESIAN_POINT('Ctrl Pts',(62.6076840919521,-34.5936396310671,0.));
#57257=CARTESIAN_POINT('Ctrl Pts',(62.6076840919521,-34.5936396310671,12.));
#57258=CARTESIAN_POINT('Ctrl Pts',(62.6304666745319,-34.5976392725303,0.));
#57259=CARTESIAN_POINT('Ctrl Pts',(62.6304666745319,-34.5976392725303,12.));
#57260=CARTESIAN_POINT('Ctrl Pts',(62.6532969232695,-34.6016238810419,0.));
#57261=CARTESIAN_POINT('Ctrl Pts',(62.6532969232695,-34.6016238810419,12.));
#57262=CARTESIAN_POINT('Ctrl Pts',(62.6761747211081,-34.6055933695093,0.));
#57263=CARTESIAN_POINT('Ctrl Pts',(62.6761747211081,-34.6055933695093,12.));
#57264=CARTESIAN_POINT('Ctrl Pts',(62.6990999514597,-34.6095476513095,0.));
#57265=CARTESIAN_POINT('Ctrl Pts',(62.6990999514597,-34.6095476513095,12.));
#57266=CARTESIAN_POINT('Ctrl Pts',(62.7220724982005,-34.6134866402842,0.));
#57267=CARTESIAN_POINT('Ctrl Pts',(62.7220724982005,-34.6134866402842,12.));
#57268=CARTESIAN_POINT('Ctrl Pts',(62.7450922456662,-34.6174102507368,0.));
#57269=CARTESIAN_POINT('Ctrl Pts',(62.7450922456662,-34.6174102507368,12.));
#57270=CARTESIAN_POINT('Ctrl Pts',(62.7681590786398,-34.6213183974303,0.));
#57271=CARTESIAN_POINT('Ctrl Pts',(62.7681590786398,-34.6213183974303,12.));
#57272=CARTESIAN_POINT('Ctrl Pts',(62.7912728823482,-34.6252109955836,0.));
#57273=CARTESIAN_POINT('Ctrl Pts',(62.7912728823482,-34.6252109955836,12.));
#57274=CARTESIAN_POINT('Ctrl Pts',(62.8144335424671,-34.629087960866,0.));
#57275=CARTESIAN_POINT('Ctrl Pts',(62.8144335424671,-34.629087960866,12.));
#57276=CARTESIAN_POINT('Ctrl Pts',(62.8376409451167,-34.6329492093932,0.));
#57277=CARTESIAN_POINT('Ctrl Pts',(62.8376409451167,-34.6329492093932,12.));
#57278=CARTESIAN_POINT('Ctrl Pts',(62.8608949768583,-34.6367946577241,0.));
#57279=CARTESIAN_POINT('Ctrl Pts',(62.8608949768583,-34.6367946577241,12.));
#57280=CARTESIAN_POINT('Ctrl Pts',(62.8841955246819,-34.6406242228606,0.));
#57281=CARTESIAN_POINT('Ctrl Pts',(62.8841955246819,-34.6406242228606,12.));
#57282=CARTESIAN_POINT('Ctrl Pts',(62.9075424760042,-34.6444378222425,0.));
#57283=CARTESIAN_POINT('Ctrl Pts',(62.9075424760042,-34.6444378222425,12.));
#57284=CARTESIAN_POINT('Ctrl Pts',(62.9309357186733,-34.6482353737434,0.));
#57285=CARTESIAN_POINT('Ctrl Pts',(62.9309357186733,-34.6482353737434,12.));
#57286=CARTESIAN_POINT('Ctrl Pts',(62.9543751409647,-34.6520167956657,0.));
#57287=CARTESIAN_POINT('Ctrl Pts',(62.9543751409647,-34.6520167956657,12.));
#57288=CARTESIAN_POINT('Ctrl Pts',(62.9778606315777,-34.655782006739,0.));
#57289=CARTESIAN_POINT('Ctrl Pts',(62.9778606315777,-34.655782006739,12.));
#57290=CARTESIAN_POINT('Ctrl Pts',(63.0013920796225,-34.6595309261186,0.));
#57291=CARTESIAN_POINT('Ctrl Pts',(63.0013920796225,-34.6595309261186,12.));
#57292=CARTESIAN_POINT('Ctrl Pts',(63.0249693746198,-34.6632634733819,0.));
#57293=CARTESIAN_POINT('Ctrl Pts',(63.0249693746198,-34.6632634733819,12.));
#57294=CARTESIAN_POINT('Ctrl Pts',(63.0485924065039,-34.6669795685225,0.));
#57295=CARTESIAN_POINT('Ctrl Pts',(63.0485924065039,-34.6669795685225,12.));
#57296=CARTESIAN_POINT('Ctrl Pts',(63.0722610656194,-34.6706791319471,0.));
#57297=CARTESIAN_POINT('Ctrl Pts',(63.0722610656194,-34.6706791319471,12.));
#57298=CARTESIAN_POINT('Ctrl Pts',(63.0959752427169,-34.6743620844722,0.));
#57299=CARTESIAN_POINT('Ctrl Pts',(63.0959752427169,-34.6743620844722,12.));
#57300=CARTESIAN_POINT('Ctrl Pts',(63.119734828943,-34.6780283473252,0.));
#57301=CARTESIAN_POINT('Ctrl Pts',(63.119734828943,-34.6780283473252,12.));
#57302=CARTESIAN_POINT('Ctrl Pts',(63.1435397158385,-34.6816778421401,0.));
#57303=CARTESIAN_POINT('Ctrl Pts',(63.1435397158385,-34.6816778421401,12.));
#57304=CARTESIAN_POINT('Ctrl Pts',(63.1673897953425,-34.6853104909516,0.));
#57305=CARTESIAN_POINT('Ctrl Pts',(63.1673897953425,-34.6853104909516,12.));
#57306=CARTESIAN_POINT('Ctrl Pts',(63.1912849597885,-34.6889262161923,0.));
#57307=CARTESIAN_POINT('Ctrl Pts',(63.1912849597885,-34.6889262161923,12.));
#57308=CARTESIAN_POINT('Ctrl Pts',(63.2152251019014,-34.6925249406899,0.));
#57309=CARTESIAN_POINT('Ctrl Pts',(63.2152251019014,-34.6925249406899,12.));
#57310=CARTESIAN_POINT('Ctrl Pts',(63.2392101147853,-34.6961065876671,0.));
#57311=CARTESIAN_POINT('Ctrl Pts',(63.2392101147853,-34.6961065876671,12.));
#57312=CARTESIAN_POINT('Ctrl Pts',(63.2632398919234,-34.6996710807384,0.));
#57313=CARTESIAN_POINT('Ctrl Pts',(63.2632398919234,-34.6996710807384,12.));
#57314=CARTESIAN_POINT('Ctrl Pts',(63.2873143271812,-34.7032183439045,0.));
#57315=CARTESIAN_POINT('Ctrl Pts',(63.2873143271812,-34.7032183439045,12.));
#57316=CARTESIAN_POINT('Ctrl Pts',(63.311433314805,-34.7067483015492,0.));
#57317=CARTESIAN_POINT('Ctrl Pts',(63.311433314805,-34.7067483015492,12.));
#57318=CARTESIAN_POINT('Ctrl Pts',(63.3355967494169,-34.7102608784373,0.));
#57319=CARTESIAN_POINT('Ctrl Pts',(63.3355967494169,-34.7102608784373,12.));
#57320=CARTESIAN_POINT('Ctrl Pts',(63.3598045260049,-34.7137559997143,0.));
#57321=CARTESIAN_POINT('Ctrl Pts',(63.3598045260049,-34.7137559997143,12.));
#57322=CARTESIAN_POINT('Ctrl Pts',(63.3840565399206,-34.7172335909037,0.));
#57323=CARTESIAN_POINT('Ctrl Pts',(63.3840565399206,-34.7172335909037,12.));
#57324=CARTESIAN_POINT('Ctrl Pts',(63.4083526868837,-34.7206935779007,0.));
#57325=CARTESIAN_POINT('Ctrl Pts',(63.4083526868837,-34.7206935779007,12.));
#57326=CARTESIAN_POINT('Ctrl Pts',(63.4326928629796,-34.7241358869702,0.));
#57327=CARTESIAN_POINT('Ctrl Pts',(63.4326928629796,-34.7241358869702,12.));
#57328=CARTESIAN_POINT('Ctrl Pts',(63.4570769646568,-34.7275604447439,0.));
#57329=CARTESIAN_POINT('Ctrl Pts',(63.4570769646568,-34.7275604447439,12.));
#57330=CARTESIAN_POINT('Ctrl Pts',(63.481504888716,-34.7309671782212,0.));
#57331=CARTESIAN_POINT('Ctrl Pts',(63.481504888716,-34.7309671782212,12.));
#57332=CARTESIAN_POINT('Ctrl Pts',(63.5059765323082,-34.7343560147663,0.));
#57333=CARTESIAN_POINT('Ctrl Pts',(63.5059765323082,-34.7343560147663,12.));
#57334=CARTESIAN_POINT('Ctrl Pts',(63.5304917929378,-34.7377268821022,0.));
#57335=CARTESIAN_POINT('Ctrl Pts',(63.5304917929378,-34.7377268821022,12.));
#57336=CARTESIAN_POINT('Ctrl Pts',(63.5550505684621,-34.7410797083079,0.));
#57337=CARTESIAN_POINT('Ctrl Pts',(63.5550505684621,-34.7410797083079,12.));
#57338=CARTESIAN_POINT('Ctrl Pts',(63.5796527570874,-34.7444144218162,0.));
#57339=CARTESIAN_POINT('Ctrl Pts',(63.5796527570874,-34.7444144218162,12.));
#57340=CARTESIAN_POINT('Ctrl Pts',(63.6042982573598,-34.7477309514142,0.));
#57341=CARTESIAN_POINT('Ctrl Pts',(63.6042982573598,-34.7477309514142,12.));
#57342=CARTESIAN_POINT('Ctrl Pts',(63.628986968162,-34.7510292262415,0.));
#57343=CARTESIAN_POINT('Ctrl Pts',(63.628986968162,-34.7510292262415,12.));
#57344=CARTESIAN_POINT('Ctrl Pts',(63.6537187887174,-34.7543091757842,0.));
#57345=CARTESIAN_POINT('Ctrl Pts',(63.6537187887174,-34.7543091757842,12.));
#57346=CARTESIAN_POINT('Ctrl Pts',(63.6784936185893,-34.7575707298718,0.));
#57347=CARTESIAN_POINT('Ctrl Pts',(63.6784936185893,-34.7575707298718,12.));
#57348=CARTESIAN_POINT('Ctrl Pts',(63.7033113576782,-34.7608138186758,0.));
#57349=CARTESIAN_POINT('Ctrl Pts',(63.7033113576782,-34.7608138186758,12.));
#57350=CARTESIAN_POINT('Ctrl Pts',(63.7281719062135,-34.7640383727094,0.));
#57351=CARTESIAN_POINT('Ctrl Pts',(63.7281719062135,-34.7640383727094,12.));
#57352=CARTESIAN_POINT('Ctrl Pts',(63.7530751647478,-34.7672443228267,0.));
#57353=CARTESIAN_POINT('Ctrl Pts',(63.7530751647478,-34.7672443228267,12.));
#57354=CARTESIAN_POINT('Ctrl Pts',(63.7780210341618,-34.7704316002165,0.));
#57355=CARTESIAN_POINT('Ctrl Pts',(63.7780210341618,-34.7704316002165,12.));
#57356=CARTESIAN_POINT('Ctrl Pts',(63.8030094156635,-34.7736001363991,0.));
#57357=CARTESIAN_POINT('Ctrl Pts',(63.8030094156635,-34.7736001363991,12.));
#57358=CARTESIAN_POINT('Ctrl Pts',(63.8280402107858,-34.7767498632244,0.));
#57359=CARTESIAN_POINT('Ctrl Pts',(63.8280402107858,-34.7767498632244,12.));
#57360=CARTESIAN_POINT('Ctrl Pts',(63.8531133213794,-34.7798807128716,0.));
#57361=CARTESIAN_POINT('Ctrl Pts',(63.8531133213794,-34.7798807128716,12.));
#57362=CARTESIAN_POINT('Ctrl Pts',(63.8782286496059,-34.7829926178495,0.));
#57363=CARTESIAN_POINT('Ctrl Pts',(63.8782286496059,-34.7829926178495,12.));
#57364=CARTESIAN_POINT('Ctrl Pts',(63.9033860979428,-34.7860855109908,0.));
#57365=CARTESIAN_POINT('Ctrl Pts',(63.9033860979428,-34.7860855109908,12.));
#57366=CARTESIAN_POINT('Ctrl Pts',(63.9285855691838,-34.7891593254485,0.));
#57367=CARTESIAN_POINT('Ctrl Pts',(63.9285855691838,-34.7891593254485,12.));
#57368=CARTESIAN_POINT('Ctrl Pts',(63.9538269664365,-34.7922139946943,0.));
#57369=CARTESIAN_POINT('Ctrl Pts',(63.9538269664365,-34.7922139946943,12.));
#57370=CARTESIAN_POINT('Ctrl Pts',(63.9791101931169,-34.7952494525182,0.));
#57371=CARTESIAN_POINT('Ctrl Pts',(63.9791101931169,-34.7952494525182,12.));
#57372=CARTESIAN_POINT('Ctrl Pts',(64.0044351529413,-34.79826563303,0.));
#57373=CARTESIAN_POINT('Ctrl Pts',(64.0044351529413,-34.79826563303,12.));
#57374=CARTESIAN_POINT('Ctrl Pts',(64.0298017499304,-34.8012624706534,0.));
#57375=CARTESIAN_POINT('Ctrl Pts',(64.0298017499304,-34.8012624706534,12.));
#57376=CARTESIAN_POINT('Ctrl Pts',(64.05520988841,-34.8042399001215,0.));
#57377=CARTESIAN_POINT('Ctrl Pts',(64.05520988841,-34.8042399001215,12.));
#57378=CARTESIAN_POINT('Ctrl Pts',(64.0806594730084,-34.8071978564748,0.));
#57379=CARTESIAN_POINT('Ctrl Pts',(64.0806594730084,-34.8071978564748,12.));
#57380=CARTESIAN_POINT('Ctrl Pts',(64.1061504086512,-34.8101362750595,0.));
#57381=CARTESIAN_POINT('Ctrl Pts',(64.1061504086512,-34.8101362750595,12.));
#57382=CARTESIAN_POINT('Ctrl Pts',(64.1316826005502,-34.8130550915284,0.));
#57383=CARTESIAN_POINT('Ctrl Pts',(64.1316826005502,-34.8130550915284,12.));
#57384=CARTESIAN_POINT('Ctrl Pts',(64.1572559542084,-34.8159542418372,0.));
#57385=CARTESIAN_POINT('Ctrl Pts',(64.1572559542084,-34.8159542418372,12.));
#57386=CARTESIAN_POINT('Ctrl Pts',(64.1828703754237,-34.8188336622419,0.));
#57387=CARTESIAN_POINT('Ctrl Pts',(64.1828703754237,-34.8188336622419,12.));
#57388=CARTESIAN_POINT('Ctrl Pts',(64.2085257702885,-34.8216932892969,0.));
#57389=CARTESIAN_POINT('Ctrl Pts',(64.2085257702885,-34.8216932892969,12.));
#57390=CARTESIAN_POINT('Ctrl Pts',(64.2342220451878,-34.8245330598559,0.));
#57391=CARTESIAN_POINT('Ctrl Pts',(64.2342220451878,-34.8245330598559,12.));
#57392=CARTESIAN_POINT('Ctrl Pts',(64.259959106791,-34.8273529110742,0.));
#57393=CARTESIAN_POINT('Ctrl Pts',(64.259959106791,-34.8273529110742,12.));
#57394=CARTESIAN_POINT('Ctrl Pts',(64.2857368620513,-34.8301527804052,0.));
#57395=CARTESIAN_POINT('Ctrl Pts',(64.2857368620513,-34.8301527804052,12.));
#57396=CARTESIAN_POINT('Ctrl Pts',(64.3115552182056,-34.8329326055916,0.));
#57397=CARTESIAN_POINT('Ctrl Pts',(64.3115552182056,-34.8329326055916,12.));
#57398=CARTESIAN_POINT('Ctrl Pts',(64.3374140827708,-34.8356923246617,0.));
#57399=CARTESIAN_POINT('Ctrl Pts',(64.3374140827708,-34.8356923246617,12.));
#57400=CARTESIAN_POINT('Ctrl Pts',(64.3633133635384,-34.838431875925,0.));
#57401=CARTESIAN_POINT('Ctrl Pts',(64.3633133635384,-34.838431875925,12.));
#57402=CARTESIAN_POINT('Ctrl Pts',(64.3892529685614,-34.8411511979705,0.));
#57403=CARTESIAN_POINT('Ctrl Pts',(64.3892529685614,-34.8411511979705,12.));
#57404=CARTESIAN_POINT('Ctrl Pts',(64.4152328061526,-34.8438502296669,0.));
#57405=CARTESIAN_POINT('Ctrl Pts',(64.4152328061526,-34.8438502296669,12.));
#57406=CARTESIAN_POINT('Ctrl Pts',(64.4412527848979,-34.8465289101626,0.));
#57407=CARTESIAN_POINT('Ctrl Pts',(64.4412527848979,-34.8465289101626,12.));
#57408=CARTESIAN_POINT('Ctrl Pts',(64.4673128136631,-34.8491871788899,0.));
#57409=CARTESIAN_POINT('Ctrl Pts',(64.4673128136631,-34.8491871788899,12.));
#57410=CARTESIAN_POINT('Ctrl Pts',(64.4934128015983,-34.851824975568,0.));
#57411=CARTESIAN_POINT('Ctrl Pts',(64.4934128015983,-34.851824975568,12.));
#57412=CARTESIAN_POINT('Ctrl Pts',(64.5195526581398,-34.8544422402114,0.));
#57413=CARTESIAN_POINT('Ctrl Pts',(64.5195526581398,-34.8544422402114,12.));
#57414=CARTESIAN_POINT('Ctrl Pts',(64.5457322930074,-34.8570389131334,0.));
#57415=CARTESIAN_POINT('Ctrl Pts',(64.5457322930074,-34.8570389131334,12.));
#57416=CARTESIAN_POINT('Ctrl Pts',(64.5719516161913,-34.8596149349251,0.));
#57417=CARTESIAN_POINT('Ctrl Pts',(64.5719516161913,-34.8596149349251,12.));
#57418=CARTESIAN_POINT('Ctrl Pts',(64.5982105379374,-34.8621702464397,0.));
#57419=CARTESIAN_POINT('Ctrl Pts',(64.5982105379374,-34.8621702464397,12.));
#57420=CARTESIAN_POINT('Ctrl Pts',(64.6245089687276,-34.8647047887774,0.));
#57421=CARTESIAN_POINT('Ctrl Pts',(64.6245089687276,-34.8647047887774,12.));
#57422=CARTESIAN_POINT('Ctrl Pts',(64.6508468192609,-34.8672185032725,0.));
#57423=CARTESIAN_POINT('Ctrl Pts',(64.6508468192609,-34.8672185032725,12.));
#57424=CARTESIAN_POINT('Ctrl Pts',(64.6772240004241,-34.8697113314797,0.));
#57425=CARTESIAN_POINT('Ctrl Pts',(64.6772240004241,-34.8697113314797,12.));
#57426=CARTESIAN_POINT('Ctrl Pts',(64.7036404233319,-34.8721832151982,0.));
#57427=CARTESIAN_POINT('Ctrl Pts',(64.7036404233319,-34.8721832151982,12.));
#57428=CARTESIAN_POINT('Ctrl Pts',(64.7300959993662,-34.8746340964977,0.));
#57429=CARTESIAN_POINT('Ctrl Pts',(64.7300959993662,-34.8746340964977,12.));
#57430=CARTESIAN_POINT('Ctrl Pts',(64.7565906402153,-34.8770639177494,0.));
#57431=CARTESIAN_POINT('Ctrl Pts',(64.7565906402153,-34.8770639177494,12.));
#57432=CARTESIAN_POINT('Ctrl Pts',(64.7831242579023,-34.8794726216511,0.));
#57433=CARTESIAN_POINT('Ctrl Pts',(64.7831242579023,-34.8794726216511,12.));
#57434=CARTESIAN_POINT('Ctrl Pts',(64.8096967648299,-34.8818601512726,0.));
#57435=CARTESIAN_POINT('Ctrl Pts',(64.8096967648299,-34.8818601512726,12.));
#57436=CARTESIAN_POINT('Ctrl Pts',(64.8363080737369,-34.8842264500184,0.));
#57437=CARTESIAN_POINT('Ctrl Pts',(64.8363080737369,-34.8842264500184,12.));
#57438=CARTESIAN_POINT('Ctrl Pts',(64.8629580976057,-34.8865714615433,0.));
#57439=CARTESIAN_POINT('Ctrl Pts',(64.8629580976057,-34.8865714615433,12.));
#57440=CARTESIAN_POINT('Ctrl Pts',(64.8896467495754,-34.888895129681,0.));
#57441=CARTESIAN_POINT('Ctrl Pts',(64.8896467495754,-34.888895129681,12.));
#57442=CARTESIAN_POINT('Ctrl Pts',(64.9163739428606,-34.8911973983785,0.));
#57443=CARTESIAN_POINT('Ctrl Pts',(64.9163739428606,-34.8911973983785,12.));
#57444=CARTESIAN_POINT('Ctrl Pts',(64.943139590634,-34.8934782116097,0.));
#57445=CARTESIAN_POINT('Ctrl Pts',(64.943139590634,-34.8934782116097,12.));
#57446=CARTESIAN_POINT('Ctrl Pts',(64.9699436060178,-34.8957375133702,0.));
#57447=CARTESIAN_POINT('Ctrl Pts',(64.9699436060178,-34.8957375133702,12.));
#57448=CARTESIAN_POINT('Ctrl Pts',(64.9967859023225,-34.8979752478623,0.));
#57449=CARTESIAN_POINT('Ctrl Pts',(64.9967859023225,-34.8979752478623,12.));
#57450=CARTESIAN_POINT('Ctrl Pts',(65.0236663932338,-34.9001913596422,0.));
#57451=CARTESIAN_POINT('Ctrl Pts',(65.0236663932338,-34.9001913596422,12.));
#57452=CARTESIAN_POINT('Ctrl Pts',(65.0505849930172,-34.9023857937866,0.));
#57453=CARTESIAN_POINT('Ctrl Pts',(65.0505849930172,-34.9023857937866,12.));
#57454=CARTESIAN_POINT('Ctrl Pts',(65.0775416167073,-34.9045584960503,0.));
#57455=CARTESIAN_POINT('Ctrl Pts',(65.0775416167073,-34.9045584960503,12.));
#57456=CARTESIAN_POINT('Ctrl Pts',(65.1045361803097,-34.9067094130387,0.));
#57457=CARTESIAN_POINT('Ctrl Pts',(65.1045361803097,-34.9067094130387,12.));
#57458=CARTESIAN_POINT('Ctrl Pts',(65.1315686003485,-34.9088384918322,0.));
#57459=CARTESIAN_POINT('Ctrl Pts',(65.1315686003485,-34.9088384918322,12.));
#57460=CARTESIAN_POINT('Ctrl Pts',(65.1586387934216,-34.9109456796201,0.));
#57461=CARTESIAN_POINT('Ctrl Pts',(65.1586387934216,-34.9109456796201,12.));
#57462=CARTESIAN_POINT('Ctrl Pts',(65.1857466757082,-34.9130309233017,0.));
#57463=CARTESIAN_POINT('Ctrl Pts',(65.1857466757082,-34.9130309233017,12.));
#57464=CARTESIAN_POINT('Ctrl Pts',(65.2128921625837,-34.9150941691754,0.));
#57465=CARTESIAN_POINT('Ctrl Pts',(65.2128921625837,-34.9150941691754,12.));
#57466=CARTESIAN_POINT('Ctrl Pts',(65.2400751679586,-34.9171353624131,0.));
#57467=CARTESIAN_POINT('Ctrl Pts',(65.2400751679586,-34.9171353624131,12.));
#57468=CARTESIAN_POINT('Ctrl Pts',(65.2672956048121,-34.9191544474898,0.));
#57469=CARTESIAN_POINT('Ctrl Pts',(65.2672956048121,-34.9191544474898,12.));
#57470=CARTESIAN_POINT('Ctrl Pts',(65.2945533863812,-34.921151369138,0.));
#57471=CARTESIAN_POINT('Ctrl Pts',(65.2945533863812,-34.921151369138,12.));
#57472=CARTESIAN_POINT('Ctrl Pts',(65.3218484271941,-34.9231260731846,0.));
#57473=CARTESIAN_POINT('Ctrl Pts',(65.3218484271941,-34.9231260731846,12.));
#57474=CARTESIAN_POINT('Ctrl Pts',(65.3491806440529,-34.9250785073473,0.));
#57475=CARTESIAN_POINT('Ctrl Pts',(65.3491806440529,-34.9250785073473,12.));
#57476=CARTESIAN_POINT('Ctrl Pts',(65.3765499573019,-34.9270086222703,0.));
#57477=CARTESIAN_POINT('Ctrl Pts',(65.3765499573019,-34.9270086222703,12.));
#57478=CARTESIAN_POINT('Ctrl Pts',(65.4039562911254,-34.92891637177,0.));
#57479=CARTESIAN_POINT('Ctrl Pts',(65.4039562911254,-34.92891637177,12.));
#57480=CARTESIAN_POINT('Ctrl Pts',(65.4313995707423,-34.9308017105481,0.));
#57481=CARTESIAN_POINT('Ctrl Pts',(65.4313995707423,-34.9308017105481,12.));
#57482=CARTESIAN_POINT('Ctrl Pts',(65.4588797201884,-34.9326645923897,0.));
#57483=CARTESIAN_POINT('Ctrl Pts',(65.4588797201884,-34.9326645923897,12.));
#57484=CARTESIAN_POINT('Ctrl Pts',(65.4863966597523,-34.9345049680816,0.));
#57485=CARTESIAN_POINT('Ctrl Pts',(65.4863966597523,-34.9345049680816,12.));
#57486=CARTESIAN_POINT('Ctrl Pts',(65.5139503038116,-34.9363227836621,0.));
#57487=CARTESIAN_POINT('Ctrl Pts',(65.5139503038116,-34.9363227836621,12.));
#57488=CARTESIAN_POINT('Ctrl Pts',(65.5415405578138,-34.9381179779763,0.));
#57489=CARTESIAN_POINT('Ctrl Pts',(65.5415405578138,-34.9381179779763,12.));
#57490=CARTESIAN_POINT('Ctrl Pts',(65.5691673226051,-34.9398904862279,0.));
#57491=CARTESIAN_POINT('Ctrl Pts',(65.5691673226051,-34.9398904862279,12.));
#57492=CARTESIAN_POINT('Ctrl Pts',(65.5968304997821,-34.9416402443551,0.));
#57493=CARTESIAN_POINT('Ctrl Pts',(65.5968304997821,-34.9416402443551,12.));
#57494=CARTESIAN_POINT('Ctrl Pts',(65.6245299968635,-34.9433671932982,0.));
#57495=CARTESIAN_POINT('Ctrl Pts',(65.6245299968635,-34.9433671932982,12.));
#57496=CARTESIAN_POINT('Ctrl Pts',(65.6522657321239,-34.9450712829143,0.));
#57497=CARTESIAN_POINT('Ctrl Pts',(65.6522657321239,-34.9450712829143,12.));
#57498=CARTESIAN_POINT('Ctrl Pts',(65.6800376405722,-34.9467524770271,0.));
#57499=CARTESIAN_POINT('Ctrl Pts',(65.6800376405722,-34.9467524770271,12.));
#57500=CARTESIAN_POINT('Ctrl Pts',(65.707845675746,-34.9484107543857,0.));
#57501=CARTESIAN_POINT('Ctrl Pts',(65.707845675746,-34.9484107543857,12.));
#57502=CARTESIAN_POINT('Ctrl Pts',(65.7356898060478,-34.9500461042919,0.));
#57503=CARTESIAN_POINT('Ctrl Pts',(65.7356898060478,-34.9500461042919,12.));
#57504=CARTESIAN_POINT('Ctrl Pts',(65.757993971173,-34.9513360397181,0.));
#57505=CARTESIAN_POINT('Ctrl Pts',(65.757993971173,-34.9513360397181,12.));
#57506=CARTESIAN_POINT('Ctrl Pts',(65.7747383250775,-34.9522931728594,0.));
#57507=CARTESIAN_POINT('Ctrl Pts',(65.7747383250775,-34.9522931728594,12.));
#57508=CARTESIAN_POINT('Ctrl Pts',(65.7859084407494,-34.9529266758406,0.));
#57509=CARTESIAN_POINT('Ctrl Pts',(65.7859084407494,-34.9529266758406,12.));
#57510=CARTESIAN_POINT('Ctrl Pts',(65.7914953018524,-34.9532422808861,0.));
#57511=CARTESIAN_POINT('Ctrl Pts',(65.7914953018524,-34.9532422808861,12.));
#57512=CARTESIAN_POINT('',(61.0441813777723,-34.2579614092497,0.));
#57513=CARTESIAN_POINT('Ctrl Pts',(61.0441813777723,-34.2579614092497,0.));
#57514=CARTESIAN_POINT('Ctrl Pts',(61.0479423318725,-34.2589297755434,0.));
#57515=CARTESIAN_POINT('Ctrl Pts',(61.0554700176998,-34.2608658001631,0.));
#57516=CARTESIAN_POINT('Ctrl Pts',(61.0667788793266,-34.2637677131935,0.));
#57517=CARTESIAN_POINT('Ctrl Pts',(61.0818920286293,-34.2676326825626,0.));
#57518=CARTESIAN_POINT('Ctrl Pts',(61.1008412399997,-34.2724568037228,0.));
#57519=CARTESIAN_POINT('Ctrl Pts',(61.1198481997764,-34.2772738038771,0.));
#57520=CARTESIAN_POINT('Ctrl Pts',(61.1389128461885,-34.282083624447,0.));
#57521=CARTESIAN_POINT('Ctrl Pts',(61.1580350635532,-34.2868861666384,0.));
#57522=CARTESIAN_POINT('Ctrl Pts',(61.1772146833205,-34.2916812929751,0.));
#57523=CARTESIAN_POINT('Ctrl Pts',(61.1964515073891,-34.2964688443663,0.));
#57524=CARTESIAN_POINT('Ctrl Pts',(61.2157453259107,-34.3012486533474,0.));
#57525=CARTESIAN_POINT('Ctrl Pts',(61.2350959366939,-34.3060205584065,0.));
#57526=CARTESIAN_POINT('Ctrl Pts',(61.2545031656133,-34.3107844191044,0.));
#57527=CARTESIAN_POINT('Ctrl Pts',(61.2739668600365,-34.3155401111747,0.));
#57528=CARTESIAN_POINT('Ctrl Pts',(61.2934868791854,-34.3202875193618,0.));
#57529=CARTESIAN_POINT('Ctrl Pts',(61.3130630861386,-34.3250265314768,0.));
#57530=CARTESIAN_POINT('Ctrl Pts',(61.3326953378851,-34.3297570310146,0.));
#57531=CARTESIAN_POINT('Ctrl Pts',(61.3523834803188,-34.3344788934363,0.));
#57532=CARTESIAN_POINT('Ctrl Pts',(61.3721273534256,-34.339191990014,0.));
#57533=CARTESIAN_POINT('Ctrl Pts',(61.3919267945302,-34.3438961902405,0.));
#57534=CARTESIAN_POINT('Ctrl Pts',(61.4117816420228,-34.3485913645979,0.));
#57535=CARTESIAN_POINT('Ctrl Pts',(61.4316917395918,-34.3532773877089,0.));
#57536=CARTESIAN_POINT('Ctrl Pts',(61.4516569360454,-34.3579541381996,0.));
#57537=CARTESIAN_POINT('Ctrl Pts',(61.4716770832896,-34.3626214971889,0.));
#57538=CARTESIAN_POINT('Ctrl Pts',(61.4917520349278,-34.3672793472466,0.));
#57539=CARTESIAN_POINT('Ctrl Pts',(61.5118816445437,-34.3719275711195,0.));
#57540=CARTESIAN_POINT('Ctrl Pts',(61.5320657642638,-34.376566050668,0.));
#57541=CARTESIAN_POINT('Ctrl Pts',(61.5523042455158,-34.3811946674197,0.));
#57542=CARTESIAN_POINT('Ctrl Pts',(61.5725969396829,-34.3858133030518,0.));
#57543=CARTESIAN_POINT('Ctrl Pts',(61.5929436987409,-34.3904218398637,0.));
#57544=CARTESIAN_POINT('Ctrl Pts',(61.6133443760142,-34.3950201613432,0.));
#57545=CARTESIAN_POINT('Ctrl Pts',(61.6337988264556,-34.3996081523753,0.));
#57546=CARTESIAN_POINT('Ctrl Pts',(61.6543069062416,-34.4041856989317,0.));
#57547=CARTESIAN_POINT('Ctrl Pts',(61.6748684725205,-34.4087526878812,0.));
#57548=CARTESIAN_POINT('Ctrl Pts',(61.695483383117,-34.4133090067704,0.));
#57549=CARTESIAN_POINT('Ctrl Pts',(61.7161514961914,-34.4178545435767,0.));
#57550=CARTESIAN_POINT('Ctrl Pts',(61.7368726702596,-34.422389186718,0.));
#57551=CARTESIAN_POINT('Ctrl Pts',(61.7576467643432,-34.4269128251577,0.));
#57552=CARTESIAN_POINT('Ctrl Pts',(61.7784736380727,-34.4314253484792,0.));
#57553=CARTESIAN_POINT('Ctrl Pts',(61.7993531518036,-34.4359266469749,0.));
#57554=CARTESIAN_POINT('Ctrl Pts',(61.8202851667222,-34.4404166117299,0.));
#57555=CARTESIAN_POINT('Ctrl Pts',(61.8412695447926,-34.444895134574,0.));
#57556=CARTESIAN_POINT('Ctrl Pts',(61.8623061487018,-34.4493621080361,0.));
#57557=CARTESIAN_POINT('Ctrl Pts',(61.8833948418025,-34.4538174253012,0.));
#57558=CARTESIAN_POINT('Ctrl Pts',(61.9045354880444,-34.4582609801637,0.));
#57559=CARTESIAN_POINT('Ctrl Pts',(61.9257279519308,-34.4626926669975,0.));
#57560=CARTESIAN_POINT('Ctrl Pts',(61.9469720985531,-34.4671123807717,0.));
#57561=CARTESIAN_POINT('Ctrl Pts',(61.9682677936053,-34.4715200170592,0.));
#57562=CARTESIAN_POINT('Ctrl Pts',(61.9896149034001,-34.4759154720473,0.));
#57563=CARTESIAN_POINT('Ctrl Pts',(62.0110132948794,-34.4802986425528,0.));
#57564=CARTESIAN_POINT('Ctrl Pts',(62.0324628356141,-34.48466942602,0.));
#57565=CARTESIAN_POINT('Ctrl Pts',(62.0539633937939,-34.489027720504,0.));
#57566=CARTESIAN_POINT('Ctrl Pts',(62.0755148382135,-34.4933734246593,0.));
#57567=CARTESIAN_POINT('Ctrl Pts',(62.0971170382567,-34.4977064377282,0.));
#57568=CARTESIAN_POINT('Ctrl Pts',(62.1187698638707,-34.5020266595293,0.));
#57569=CARTESIAN_POINT('Ctrl Pts',(62.1404731855687,-34.5063339904533,0.));
#57570=CARTESIAN_POINT('Ctrl Pts',(62.1622268744337,-34.5106283314594,0.));
#57571=CARTESIAN_POINT('Ctrl Pts',(62.184030802117,-34.514909584073,0.));
#57572=CARTESIAN_POINT('Ctrl Pts',(62.2058848408346,-34.5191776503843,0.));
#57573=CARTESIAN_POINT('Ctrl Pts',(62.2277888633576,-34.5234324330492,0.));
#57574=CARTESIAN_POINT('Ctrl Pts',(62.2497427430136,-34.527673835281,0.));
#57575=CARTESIAN_POINT('Ctrl Pts',(62.2717463536828,-34.5319017608435,0.));
#57576=CARTESIAN_POINT('Ctrl Pts',(62.2937995697927,-34.536116114045,0.));
#57577=CARTESIAN_POINT('Ctrl Pts',(62.3159022663052,-34.5403167997333,0.));
#57578=CARTESIAN_POINT('Ctrl Pts',(62.3380543187067,-34.5445037232928,0.));
#57579=CARTESIAN_POINT('Ctrl Pts',(62.3602556030114,-34.5486767906376,0.));
#57580=CARTESIAN_POINT('Ctrl Pts',(62.3825059957593,-34.552835908207,0.));
#57581=CARTESIAN_POINT('Ctrl Pts',(62.4048053740129,-34.5569809829615,0.));
#57582=CARTESIAN_POINT('Ctrl Pts',(62.4271536153473,-34.5611119223807,0.));
#57583=CARTESIAN_POINT('Ctrl Pts',(62.4495505978415,-34.5652286344606,0.));
#57584=CARTESIAN_POINT('Ctrl Pts',(62.4719962000829,-34.5693310277064,0.));
#57585=CARTESIAN_POINT('Ctrl Pts',(62.494490301164,-34.5734190111279,0.));
#57586=CARTESIAN_POINT('Ctrl Pts',(62.5170327806774,-34.5774924942351,0.));
#57587=CARTESIAN_POINT('Ctrl Pts',(62.5396235187053,-34.5815513870363,0.));
#57588=CARTESIAN_POINT('Ctrl Pts',(62.5622623958125,-34.5855956000344,0.));
#57589=CARTESIAN_POINT('Ctrl Pts',(62.5849492930501,-34.5896250442199,0.));
#57590=CARTESIAN_POINT('Ctrl Pts',(62.6076840919521,-34.5936396310671,0.));
#57591=CARTESIAN_POINT('Ctrl Pts',(62.6304666745319,-34.5976392725303,0.));
#57592=CARTESIAN_POINT('Ctrl Pts',(62.6532969232695,-34.6016238810419,0.));
#57593=CARTESIAN_POINT('Ctrl Pts',(62.6761747211081,-34.6055933695093,0.));
#57594=CARTESIAN_POINT('Ctrl Pts',(62.6990999514597,-34.6095476513095,0.));
#57595=CARTESIAN_POINT('Ctrl Pts',(62.7220724982005,-34.6134866402842,0.));
#57596=CARTESIAN_POINT('Ctrl Pts',(62.7450922456662,-34.6174102507368,0.));
#57597=CARTESIAN_POINT('Ctrl Pts',(62.7681590786398,-34.6213183974303,0.));
#57598=CARTESIAN_POINT('Ctrl Pts',(62.7912728823482,-34.6252109955836,0.));
#57599=CARTESIAN_POINT('Ctrl Pts',(62.8144335424671,-34.629087960866,0.));
#57600=CARTESIAN_POINT('Ctrl Pts',(62.8376409451167,-34.6329492093932,0.));
#57601=CARTESIAN_POINT('Ctrl Pts',(62.8608949768583,-34.6367946577241,0.));
#57602=CARTESIAN_POINT('Ctrl Pts',(62.8841955246819,-34.6406242228606,0.));
#57603=CARTESIAN_POINT('Ctrl Pts',(62.9075424760042,-34.6444378222425,0.));
#57604=CARTESIAN_POINT('Ctrl Pts',(62.9309357186733,-34.6482353737434,0.));
#57605=CARTESIAN_POINT('Ctrl Pts',(62.9543751409647,-34.6520167956657,0.));
#57606=CARTESIAN_POINT('Ctrl Pts',(62.9778606315777,-34.655782006739,0.));
#57607=CARTESIAN_POINT('Ctrl Pts',(63.0013920796225,-34.6595309261186,0.));
#57608=CARTESIAN_POINT('Ctrl Pts',(63.0249693746198,-34.6632634733819,0.));
#57609=CARTESIAN_POINT('Ctrl Pts',(63.0485924065039,-34.6669795685225,0.));
#57610=CARTESIAN_POINT('Ctrl Pts',(63.0722610656194,-34.6706791319471,0.));
#57611=CARTESIAN_POINT('Ctrl Pts',(63.0959752427169,-34.6743620844722,0.));
#57612=CARTESIAN_POINT('Ctrl Pts',(63.119734828943,-34.6780283473252,0.));
#57613=CARTESIAN_POINT('Ctrl Pts',(63.1435397158385,-34.6816778421401,0.));
#57614=CARTESIAN_POINT('Ctrl Pts',(63.1673897953425,-34.6853104909516,0.));
#57615=CARTESIAN_POINT('Ctrl Pts',(63.1912849597885,-34.6889262161923,0.));
#57616=CARTESIAN_POINT('Ctrl Pts',(63.2152251019014,-34.6925249406899,0.));
#57617=CARTESIAN_POINT('Ctrl Pts',(63.2392101147853,-34.6961065876671,0.));
#57618=CARTESIAN_POINT('Ctrl Pts',(63.2632398919234,-34.6996710807384,0.));
#57619=CARTESIAN_POINT('Ctrl Pts',(63.2873143271812,-34.7032183439045,0.));
#57620=CARTESIAN_POINT('Ctrl Pts',(63.311433314805,-34.7067483015492,0.));
#57621=CARTESIAN_POINT('Ctrl Pts',(63.3355967494169,-34.7102608784373,0.));
#57622=CARTESIAN_POINT('Ctrl Pts',(63.3598045260049,-34.7137559997143,0.));
#57623=CARTESIAN_POINT('Ctrl Pts',(63.3840565399206,-34.7172335909037,0.));
#57624=CARTESIAN_POINT('Ctrl Pts',(63.4083526868837,-34.7206935779007,0.));
#57625=CARTESIAN_POINT('Ctrl Pts',(63.4326928629796,-34.7241358869702,0.));
#57626=CARTESIAN_POINT('Ctrl Pts',(63.4570769646568,-34.7275604447439,0.));
#57627=CARTESIAN_POINT('Ctrl Pts',(63.481504888716,-34.7309671782212,0.));
#57628=CARTESIAN_POINT('Ctrl Pts',(63.5059765323082,-34.7343560147663,0.));
#57629=CARTESIAN_POINT('Ctrl Pts',(63.5304917929378,-34.7377268821022,0.));
#57630=CARTESIAN_POINT('Ctrl Pts',(63.5550505684621,-34.7410797083079,0.));
#57631=CARTESIAN_POINT('Ctrl Pts',(63.5796527570874,-34.7444144218162,0.));
#57632=CARTESIAN_POINT('Ctrl Pts',(63.6042982573598,-34.7477309514142,0.));
#57633=CARTESIAN_POINT('Ctrl Pts',(63.628986968162,-34.7510292262415,0.));
#57634=CARTESIAN_POINT('Ctrl Pts',(63.6537187887174,-34.7543091757842,0.));
#57635=CARTESIAN_POINT('Ctrl Pts',(63.6784936185893,-34.7575707298718,0.));
#57636=CARTESIAN_POINT('Ctrl Pts',(63.7033113576782,-34.7608138186758,0.));
#57637=CARTESIAN_POINT('Ctrl Pts',(63.7281719062135,-34.7640383727094,0.));
#57638=CARTESIAN_POINT('Ctrl Pts',(63.7530751647478,-34.7672443228267,0.));
#57639=CARTESIAN_POINT('Ctrl Pts',(63.7780210341618,-34.7704316002165,0.));
#57640=CARTESIAN_POINT('Ctrl Pts',(63.8030094156635,-34.7736001363991,0.));
#57641=CARTESIAN_POINT('Ctrl Pts',(63.8280402107858,-34.7767498632244,0.));
#57642=CARTESIAN_POINT('Ctrl Pts',(63.8531133213794,-34.7798807128716,0.));
#57643=CARTESIAN_POINT('Ctrl Pts',(63.8782286496059,-34.7829926178495,0.));
#57644=CARTESIAN_POINT('Ctrl Pts',(63.9033860979428,-34.7860855109908,0.));
#57645=CARTESIAN_POINT('Ctrl Pts',(63.9285855691838,-34.7891593254485,0.));
#57646=CARTESIAN_POINT('Ctrl Pts',(63.9538269664365,-34.7922139946943,0.));
#57647=CARTESIAN_POINT('Ctrl Pts',(63.9791101931169,-34.7952494525182,0.));
#57648=CARTESIAN_POINT('Ctrl Pts',(64.0044351529413,-34.79826563303,0.));
#57649=CARTESIAN_POINT('Ctrl Pts',(64.0298017499304,-34.8012624706534,0.));
#57650=CARTESIAN_POINT('Ctrl Pts',(64.05520988841,-34.8042399001215,0.));
#57651=CARTESIAN_POINT('Ctrl Pts',(64.0806594730084,-34.8071978564748,0.));
#57652=CARTESIAN_POINT('Ctrl Pts',(64.1061504086512,-34.8101362750595,0.));
#57653=CARTESIAN_POINT('Ctrl Pts',(64.1316826005502,-34.8130550915284,0.));
#57654=CARTESIAN_POINT('Ctrl Pts',(64.1572559542084,-34.8159542418372,0.));
#57655=CARTESIAN_POINT('Ctrl Pts',(64.1828703754237,-34.8188336622419,0.));
#57656=CARTESIAN_POINT('Ctrl Pts',(64.2085257702885,-34.8216932892969,0.));
#57657=CARTESIAN_POINT('Ctrl Pts',(64.2342220451878,-34.8245330598559,0.));
#57658=CARTESIAN_POINT('Ctrl Pts',(64.259959106791,-34.8273529110742,0.));
#57659=CARTESIAN_POINT('Ctrl Pts',(64.2857368620513,-34.8301527804052,0.));
#57660=CARTESIAN_POINT('Ctrl Pts',(64.3115552182056,-34.8329326055916,0.));
#57661=CARTESIAN_POINT('Ctrl Pts',(64.3374140827708,-34.8356923246617,0.));
#57662=CARTESIAN_POINT('Ctrl Pts',(64.3633133635384,-34.838431875925,0.));
#57663=CARTESIAN_POINT('Ctrl Pts',(64.3892529685614,-34.8411511979705,0.));
#57664=CARTESIAN_POINT('Ctrl Pts',(64.4152328061526,-34.8438502296669,0.));
#57665=CARTESIAN_POINT('Ctrl Pts',(64.4412527848979,-34.8465289101626,0.));
#57666=CARTESIAN_POINT('Ctrl Pts',(64.4673128136631,-34.8491871788899,0.));
#57667=CARTESIAN_POINT('Ctrl Pts',(64.4934128015983,-34.851824975568,0.));
#57668=CARTESIAN_POINT('Ctrl Pts',(64.5195526581398,-34.8544422402114,0.));
#57669=CARTESIAN_POINT('Ctrl Pts',(64.5457322930074,-34.8570389131334,0.));
#57670=CARTESIAN_POINT('Ctrl Pts',(64.5719516161913,-34.8596149349251,0.));
#57671=CARTESIAN_POINT('Ctrl Pts',(64.5982105379374,-34.8621702464397,0.));
#57672=CARTESIAN_POINT('Ctrl Pts',(64.6245089687276,-34.8647047887774,0.));
#57673=CARTESIAN_POINT('Ctrl Pts',(64.6508468192609,-34.8672185032725,0.));
#57674=CARTESIAN_POINT('Ctrl Pts',(64.6772240004241,-34.8697113314797,0.));
#57675=CARTESIAN_POINT('Ctrl Pts',(64.7036404233319,-34.8721832151982,0.));
#57676=CARTESIAN_POINT('Ctrl Pts',(64.7300959993662,-34.8746340964977,0.));
#57677=CARTESIAN_POINT('Ctrl Pts',(64.7565906402153,-34.8770639177494,0.));
#57678=CARTESIAN_POINT('Ctrl Pts',(64.7831242579023,-34.8794726216511,0.));
#57679=CARTESIAN_POINT('Ctrl Pts',(64.8096967648299,-34.8818601512726,0.));
#57680=CARTESIAN_POINT('Ctrl Pts',(64.8363080737369,-34.8842264500184,0.));
#57681=CARTESIAN_POINT('Ctrl Pts',(64.8629580976057,-34.8865714615433,0.));
#57682=CARTESIAN_POINT('Ctrl Pts',(64.8896467495754,-34.888895129681,0.));
#57683=CARTESIAN_POINT('Ctrl Pts',(64.9163739428606,-34.8911973983785,0.));
#57684=CARTESIAN_POINT('Ctrl Pts',(64.943139590634,-34.8934782116097,0.));
#57685=CARTESIAN_POINT('Ctrl Pts',(64.9699436060178,-34.8957375133702,0.));
#57686=CARTESIAN_POINT('Ctrl Pts',(64.9967859023225,-34.8979752478623,0.));
#57687=CARTESIAN_POINT('Ctrl Pts',(65.0236663932338,-34.9001913596422,0.));
#57688=CARTESIAN_POINT('Ctrl Pts',(65.0505849930172,-34.9023857937866,0.));
#57689=CARTESIAN_POINT('Ctrl Pts',(65.0775416167073,-34.9045584960503,0.));
#57690=CARTESIAN_POINT('Ctrl Pts',(65.1045361803097,-34.9067094130387,0.));
#57691=CARTESIAN_POINT('Ctrl Pts',(65.1315686003485,-34.9088384918322,0.));
#57692=CARTESIAN_POINT('Ctrl Pts',(65.1586387934216,-34.9109456796201,0.));
#57693=CARTESIAN_POINT('Ctrl Pts',(65.1857466757082,-34.9130309233017,0.));
#57694=CARTESIAN_POINT('Ctrl Pts',(65.2128921625837,-34.9150941691754,0.));
#57695=CARTESIAN_POINT('Ctrl Pts',(65.2400751679586,-34.9171353624131,0.));
#57696=CARTESIAN_POINT('Ctrl Pts',(65.2672956048121,-34.9191544474898,0.));
#57697=CARTESIAN_POINT('Ctrl Pts',(65.2945533863812,-34.921151369138,0.));
#57698=CARTESIAN_POINT('Ctrl Pts',(65.3218484271941,-34.9231260731846,0.));
#57699=CARTESIAN_POINT('Ctrl Pts',(65.3491806440529,-34.9250785073473,0.));
#57700=CARTESIAN_POINT('Ctrl Pts',(65.3765499573019,-34.9270086222703,0.));
#57701=CARTESIAN_POINT('Ctrl Pts',(65.4039562911254,-34.92891637177,0.));
#57702=CARTESIAN_POINT('Ctrl Pts',(65.4274804996405,-34.9305324724386,0.));
#57703=CARTESIAN_POINT('Ctrl Pts',(65.4455359574999,-34.9317593813103,0.));
#57704=CARTESIAN_POINT('Ctrl Pts',(65.4581063193583,-34.9326070346592,0.));
#57705=CARTESIAN_POINT('Ctrl Pts',(65.4651808010451,-34.9330820191484,0.));
#57706=CARTESIAN_POINT('Ctrl Pts',(65.4667541477954,-34.9331875523085,0.));
#57707=CARTESIAN_POINT('',(61.0441813777723,-34.2579614092497,12.));
#57708=CARTESIAN_POINT('',(61.0441813777723,-34.2579614092497,0.));
#57709=CARTESIAN_POINT('Ctrl Pts',(65.4667541477954,-34.9331875523085,12.));
#57710=CARTESIAN_POINT('Ctrl Pts',(65.4651808010451,-34.9330820191484,12.));
#57711=CARTESIAN_POINT('Ctrl Pts',(65.4581063193583,-34.9326070346592,12.));
#57712=CARTESIAN_POINT('Ctrl Pts',(65.4455359574999,-34.9317593813103,12.));
#57713=CARTESIAN_POINT('Ctrl Pts',(65.4274804996405,-34.9305324724386,12.));
#57714=CARTESIAN_POINT('Ctrl Pts',(65.4039562911254,-34.92891637177,12.));
#57715=CARTESIAN_POINT('Ctrl Pts',(65.3765499573019,-34.9270086222703,12.));
#57716=CARTESIAN_POINT('Ctrl Pts',(65.3491806440529,-34.9250785073473,12.));
#57717=CARTESIAN_POINT('Ctrl Pts',(65.3218484271941,-34.9231260731846,12.));
#57718=CARTESIAN_POINT('Ctrl Pts',(65.2945533863812,-34.921151369138,12.));
#57719=CARTESIAN_POINT('Ctrl Pts',(65.2672956048121,-34.9191544474898,12.));
#57720=CARTESIAN_POINT('Ctrl Pts',(65.2400751679586,-34.9171353624131,12.));
#57721=CARTESIAN_POINT('Ctrl Pts',(65.2128921625837,-34.9150941691754,12.));
#57722=CARTESIAN_POINT('Ctrl Pts',(65.1857466757082,-34.9130309233017,12.));
#57723=CARTESIAN_POINT('Ctrl Pts',(65.1586387934216,-34.9109456796201,12.));
#57724=CARTESIAN_POINT('Ctrl Pts',(65.1315686003485,-34.9088384918322,12.));
#57725=CARTESIAN_POINT('Ctrl Pts',(65.1045361803097,-34.9067094130387,12.));
#57726=CARTESIAN_POINT('Ctrl Pts',(65.0775416167073,-34.9045584960503,12.));
#57727=CARTESIAN_POINT('Ctrl Pts',(65.0505849930172,-34.9023857937866,12.));
#57728=CARTESIAN_POINT('Ctrl Pts',(65.0236663932338,-34.9001913596422,12.));
#57729=CARTESIAN_POINT('Ctrl Pts',(64.9967859023225,-34.8979752478623,12.));
#57730=CARTESIAN_POINT('Ctrl Pts',(64.9699436060178,-34.8957375133702,12.));
#57731=CARTESIAN_POINT('Ctrl Pts',(64.943139590634,-34.8934782116097,12.));
#57732=CARTESIAN_POINT('Ctrl Pts',(64.9163739428606,-34.8911973983785,12.));
#57733=CARTESIAN_POINT('Ctrl Pts',(64.8896467495754,-34.888895129681,12.));
#57734=CARTESIAN_POINT('Ctrl Pts',(64.8629580976057,-34.8865714615433,12.));
#57735=CARTESIAN_POINT('Ctrl Pts',(64.8363080737369,-34.8842264500184,12.));
#57736=CARTESIAN_POINT('Ctrl Pts',(64.8096967648299,-34.8818601512726,12.));
#57737=CARTESIAN_POINT('Ctrl Pts',(64.7831242579023,-34.8794726216511,12.));
#57738=CARTESIAN_POINT('Ctrl Pts',(64.7565906402153,-34.8770639177494,12.));
#57739=CARTESIAN_POINT('Ctrl Pts',(64.7300959993662,-34.8746340964977,12.));
#57740=CARTESIAN_POINT('Ctrl Pts',(64.7036404233319,-34.8721832151982,12.));
#57741=CARTESIAN_POINT('Ctrl Pts',(64.6772240004241,-34.8697113314797,12.));
#57742=CARTESIAN_POINT('Ctrl Pts',(64.6508468192609,-34.8672185032725,12.));
#57743=CARTESIAN_POINT('Ctrl Pts',(64.6245089687276,-34.8647047887774,12.));
#57744=CARTESIAN_POINT('Ctrl Pts',(64.5982105379374,-34.8621702464397,12.));
#57745=CARTESIAN_POINT('Ctrl Pts',(64.5719516161913,-34.8596149349251,12.));
#57746=CARTESIAN_POINT('Ctrl Pts',(64.5457322930074,-34.8570389131334,12.));
#57747=CARTESIAN_POINT('Ctrl Pts',(64.5195526581398,-34.8544422402114,12.));
#57748=CARTESIAN_POINT('Ctrl Pts',(64.4934128015983,-34.851824975568,12.));
#57749=CARTESIAN_POINT('Ctrl Pts',(64.4673128136631,-34.8491871788899,12.));
#57750=CARTESIAN_POINT('Ctrl Pts',(64.4412527848979,-34.8465289101626,12.));
#57751=CARTESIAN_POINT('Ctrl Pts',(64.4152328061526,-34.8438502296669,12.));
#57752=CARTESIAN_POINT('Ctrl Pts',(64.3892529685614,-34.8411511979705,12.));
#57753=CARTESIAN_POINT('Ctrl Pts',(64.3633133635384,-34.838431875925,12.));
#57754=CARTESIAN_POINT('Ctrl Pts',(64.3374140827708,-34.8356923246617,12.));
#57755=CARTESIAN_POINT('Ctrl Pts',(64.3115552182056,-34.8329326055916,12.));
#57756=CARTESIAN_POINT('Ctrl Pts',(64.2857368620513,-34.8301527804052,12.));
#57757=CARTESIAN_POINT('Ctrl Pts',(64.259959106791,-34.8273529110742,12.));
#57758=CARTESIAN_POINT('Ctrl Pts',(64.2342220451878,-34.8245330598559,12.));
#57759=CARTESIAN_POINT('Ctrl Pts',(64.2085257702885,-34.8216932892969,12.));
#57760=CARTESIAN_POINT('Ctrl Pts',(64.1828703754237,-34.8188336622419,12.));
#57761=CARTESIAN_POINT('Ctrl Pts',(64.1572559542084,-34.8159542418372,12.));
#57762=CARTESIAN_POINT('Ctrl Pts',(64.1316826005502,-34.8130550915284,12.));
#57763=CARTESIAN_POINT('Ctrl Pts',(64.1061504086512,-34.8101362750595,12.));
#57764=CARTESIAN_POINT('Ctrl Pts',(64.0806594730084,-34.8071978564748,12.));
#57765=CARTESIAN_POINT('Ctrl Pts',(64.05520988841,-34.8042399001215,12.));
#57766=CARTESIAN_POINT('Ctrl Pts',(64.0298017499304,-34.8012624706534,12.));
#57767=CARTESIAN_POINT('Ctrl Pts',(64.0044351529413,-34.79826563303,12.));
#57768=CARTESIAN_POINT('Ctrl Pts',(63.9791101931169,-34.7952494525182,12.));
#57769=CARTESIAN_POINT('Ctrl Pts',(63.9538269664365,-34.7922139946943,12.));
#57770=CARTESIAN_POINT('Ctrl Pts',(63.9285855691838,-34.7891593254485,12.));
#57771=CARTESIAN_POINT('Ctrl Pts',(63.9033860979428,-34.7860855109908,12.));
#57772=CARTESIAN_POINT('Ctrl Pts',(63.8782286496059,-34.7829926178495,12.));
#57773=CARTESIAN_POINT('Ctrl Pts',(63.8531133213794,-34.7798807128716,12.));
#57774=CARTESIAN_POINT('Ctrl Pts',(63.8280402107858,-34.7767498632244,12.));
#57775=CARTESIAN_POINT('Ctrl Pts',(63.8030094156635,-34.7736001363991,12.));
#57776=CARTESIAN_POINT('Ctrl Pts',(63.7780210341618,-34.7704316002165,12.));
#57777=CARTESIAN_POINT('Ctrl Pts',(63.7530751647478,-34.7672443228267,12.));
#57778=CARTESIAN_POINT('Ctrl Pts',(63.7281719062135,-34.7640383727094,12.));
#57779=CARTESIAN_POINT('Ctrl Pts',(63.7033113576782,-34.7608138186758,12.));
#57780=CARTESIAN_POINT('Ctrl Pts',(63.6784936185893,-34.7575707298718,12.));
#57781=CARTESIAN_POINT('Ctrl Pts',(63.6537187887174,-34.7543091757842,12.));
#57782=CARTESIAN_POINT('Ctrl Pts',(63.628986968162,-34.7510292262415,12.));
#57783=CARTESIAN_POINT('Ctrl Pts',(63.6042982573598,-34.7477309514142,12.));
#57784=CARTESIAN_POINT('Ctrl Pts',(63.5796527570874,-34.7444144218162,12.));
#57785=CARTESIAN_POINT('Ctrl Pts',(63.5550505684621,-34.7410797083079,12.));
#57786=CARTESIAN_POINT('Ctrl Pts',(63.5304917929378,-34.7377268821022,12.));
#57787=CARTESIAN_POINT('Ctrl Pts',(63.5059765323082,-34.7343560147663,12.));
#57788=CARTESIAN_POINT('Ctrl Pts',(63.481504888716,-34.7309671782212,12.));
#57789=CARTESIAN_POINT('Ctrl Pts',(63.4570769646568,-34.7275604447439,12.));
#57790=CARTESIAN_POINT('Ctrl Pts',(63.4326928629796,-34.7241358869702,12.));
#57791=CARTESIAN_POINT('Ctrl Pts',(63.4083526868837,-34.7206935779007,12.));
#57792=CARTESIAN_POINT('Ctrl Pts',(63.3840565399206,-34.7172335909037,12.));
#57793=CARTESIAN_POINT('Ctrl Pts',(63.3598045260049,-34.7137559997143,12.));
#57794=CARTESIAN_POINT('Ctrl Pts',(63.3355967494169,-34.7102608784373,12.));
#57795=CARTESIAN_POINT('Ctrl Pts',(63.311433314805,-34.7067483015492,12.));
#57796=CARTESIAN_POINT('Ctrl Pts',(63.2873143271812,-34.7032183439045,12.));
#57797=CARTESIAN_POINT('Ctrl Pts',(63.2632398919234,-34.6996710807384,12.));
#57798=CARTESIAN_POINT('Ctrl Pts',(63.2392101147853,-34.6961065876671,12.));
#57799=CARTESIAN_POINT('Ctrl Pts',(63.2152251019014,-34.6925249406899,12.));
#57800=CARTESIAN_POINT('Ctrl Pts',(63.1912849597885,-34.6889262161923,12.));
#57801=CARTESIAN_POINT('Ctrl Pts',(63.1673897953425,-34.6853104909516,12.));
#57802=CARTESIAN_POINT('Ctrl Pts',(63.1435397158385,-34.6816778421401,12.));
#57803=CARTESIAN_POINT('Ctrl Pts',(63.119734828943,-34.6780283473252,12.));
#57804=CARTESIAN_POINT('Ctrl Pts',(63.0959752427169,-34.6743620844722,12.));
#57805=CARTESIAN_POINT('Ctrl Pts',(63.0722610656194,-34.6706791319471,12.));
#57806=CARTESIAN_POINT('Ctrl Pts',(63.0485924065039,-34.6669795685225,12.));
#57807=CARTESIAN_POINT('Ctrl Pts',(63.0249693746198,-34.6632634733819,12.));
#57808=CARTESIAN_POINT('Ctrl Pts',(63.0013920796225,-34.6595309261186,12.));
#57809=CARTESIAN_POINT('Ctrl Pts',(62.9778606315777,-34.655782006739,12.));
#57810=CARTESIAN_POINT('Ctrl Pts',(62.9543751409647,-34.6520167956657,12.));
#57811=CARTESIAN_POINT('Ctrl Pts',(62.9309357186733,-34.6482353737434,12.));
#57812=CARTESIAN_POINT('Ctrl Pts',(62.9075424760042,-34.6444378222425,12.));
#57813=CARTESIAN_POINT('Ctrl Pts',(62.8841955246819,-34.6406242228606,12.));
#57814=CARTESIAN_POINT('Ctrl Pts',(62.8608949768583,-34.6367946577241,12.));
#57815=CARTESIAN_POINT('Ctrl Pts',(62.8376409451167,-34.6329492093932,12.));
#57816=CARTESIAN_POINT('Ctrl Pts',(62.8144335424671,-34.629087960866,12.));
#57817=CARTESIAN_POINT('Ctrl Pts',(62.7912728823482,-34.6252109955836,12.));
#57818=CARTESIAN_POINT('Ctrl Pts',(62.7681590786398,-34.6213183974303,12.));
#57819=CARTESIAN_POINT('Ctrl Pts',(62.7450922456662,-34.6174102507368,12.));
#57820=CARTESIAN_POINT('Ctrl Pts',(62.7220724982005,-34.6134866402842,12.));
#57821=CARTESIAN_POINT('Ctrl Pts',(62.6990999514597,-34.6095476513095,12.));
#57822=CARTESIAN_POINT('Ctrl Pts',(62.6761747211081,-34.6055933695093,12.));
#57823=CARTESIAN_POINT('Ctrl Pts',(62.6532969232695,-34.6016238810419,12.));
#57824=CARTESIAN_POINT('Ctrl Pts',(62.6304666745319,-34.5976392725303,12.));
#57825=CARTESIAN_POINT('Ctrl Pts',(62.6076840919521,-34.5936396310671,12.));
#57826=CARTESIAN_POINT('Ctrl Pts',(62.5849492930501,-34.5896250442199,12.));
#57827=CARTESIAN_POINT('Ctrl Pts',(62.5622623958125,-34.5855956000344,12.));
#57828=CARTESIAN_POINT('Ctrl Pts',(62.5396235187053,-34.5815513870363,12.));
#57829=CARTESIAN_POINT('Ctrl Pts',(62.5170327806774,-34.5774924942351,12.));
#57830=CARTESIAN_POINT('Ctrl Pts',(62.494490301164,-34.5734190111279,12.));
#57831=CARTESIAN_POINT('Ctrl Pts',(62.4719962000829,-34.5693310277064,12.));
#57832=CARTESIAN_POINT('Ctrl Pts',(62.4495505978415,-34.5652286344606,12.));
#57833=CARTESIAN_POINT('Ctrl Pts',(62.4271536153473,-34.5611119223807,12.));
#57834=CARTESIAN_POINT('Ctrl Pts',(62.4048053740129,-34.5569809829615,12.));
#57835=CARTESIAN_POINT('Ctrl Pts',(62.3825059957593,-34.552835908207,12.));
#57836=CARTESIAN_POINT('Ctrl Pts',(62.3602556030114,-34.5486767906376,12.));
#57837=CARTESIAN_POINT('Ctrl Pts',(62.3380543187067,-34.5445037232928,12.));
#57838=CARTESIAN_POINT('Ctrl Pts',(62.3159022663052,-34.5403167997333,12.));
#57839=CARTESIAN_POINT('Ctrl Pts',(62.2937995697927,-34.536116114045,12.));
#57840=CARTESIAN_POINT('Ctrl Pts',(62.2717463536828,-34.5319017608435,12.));
#57841=CARTESIAN_POINT('Ctrl Pts',(62.2497427430136,-34.527673835281,12.));
#57842=CARTESIAN_POINT('Ctrl Pts',(62.2277888633576,-34.5234324330492,12.));
#57843=CARTESIAN_POINT('Ctrl Pts',(62.2058848408346,-34.5191776503843,12.));
#57844=CARTESIAN_POINT('Ctrl Pts',(62.184030802117,-34.514909584073,12.));
#57845=CARTESIAN_POINT('Ctrl Pts',(62.1622268744337,-34.5106283314594,12.));
#57846=CARTESIAN_POINT('Ctrl Pts',(62.1404731855687,-34.5063339904533,12.));
#57847=CARTESIAN_POINT('Ctrl Pts',(62.1187698638707,-34.5020266595293,12.));
#57848=CARTESIAN_POINT('Ctrl Pts',(62.0971170382567,-34.4977064377282,12.));
#57849=CARTESIAN_POINT('Ctrl Pts',(62.0755148382135,-34.4933734246593,12.));
#57850=CARTESIAN_POINT('Ctrl Pts',(62.0539633937939,-34.489027720504,12.));
#57851=CARTESIAN_POINT('Ctrl Pts',(62.0324628356141,-34.48466942602,12.));
#57852=CARTESIAN_POINT('Ctrl Pts',(62.0110132948794,-34.4802986425528,12.));
#57853=CARTESIAN_POINT('Ctrl Pts',(61.9896149034001,-34.4759154720473,12.));
#57854=CARTESIAN_POINT('Ctrl Pts',(61.9682677936053,-34.4715200170592,12.));
#57855=CARTESIAN_POINT('Ctrl Pts',(61.9469720985531,-34.4671123807717,12.));
#57856=CARTESIAN_POINT('Ctrl Pts',(61.9257279519308,-34.4626926669975,12.));
#57857=CARTESIAN_POINT('Ctrl Pts',(61.9045354880444,-34.4582609801637,12.));
#57858=CARTESIAN_POINT('Ctrl Pts',(61.8833948418025,-34.4538174253012,12.));
#57859=CARTESIAN_POINT('Ctrl Pts',(61.8623061487018,-34.4493621080361,12.));
#57860=CARTESIAN_POINT('Ctrl Pts',(61.8412695447926,-34.444895134574,12.));
#57861=CARTESIAN_POINT('Ctrl Pts',(61.8202851667222,-34.4404166117299,12.));
#57862=CARTESIAN_POINT('Ctrl Pts',(61.7993531518036,-34.4359266469749,12.));
#57863=CARTESIAN_POINT('Ctrl Pts',(61.7784736380727,-34.4314253484792,12.));
#57864=CARTESIAN_POINT('Ctrl Pts',(61.7576467643432,-34.4269128251577,12.));
#57865=CARTESIAN_POINT('Ctrl Pts',(61.7368726702596,-34.422389186718,12.));
#57866=CARTESIAN_POINT('Ctrl Pts',(61.7161514961914,-34.4178545435767,12.));
#57867=CARTESIAN_POINT('Ctrl Pts',(61.695483383117,-34.4133090067704,12.));
#57868=CARTESIAN_POINT('Ctrl Pts',(61.6748684725205,-34.4087526878812,12.));
#57869=CARTESIAN_POINT('Ctrl Pts',(61.6543069062416,-34.4041856989317,12.));
#57870=CARTESIAN_POINT('Ctrl Pts',(61.6337988264556,-34.3996081523753,12.));
#57871=CARTESIAN_POINT('Ctrl Pts',(61.6133443760142,-34.3950201613432,12.));
#57872=CARTESIAN_POINT('Ctrl Pts',(61.5929436987409,-34.3904218398637,12.));
#57873=CARTESIAN_POINT('Ctrl Pts',(61.5725969396829,-34.3858133030518,12.));
#57874=CARTESIAN_POINT('Ctrl Pts',(61.5523042455158,-34.3811946674197,12.));
#57875=CARTESIAN_POINT('Ctrl Pts',(61.5320657642638,-34.376566050668,12.));
#57876=CARTESIAN_POINT('Ctrl Pts',(61.5118816445437,-34.3719275711195,12.));
#57877=CARTESIAN_POINT('Ctrl Pts',(61.4917520349278,-34.3672793472466,12.));
#57878=CARTESIAN_POINT('Ctrl Pts',(61.4716770832896,-34.3626214971889,12.));
#57879=CARTESIAN_POINT('Ctrl Pts',(61.4516569360454,-34.3579541381996,12.));
#57880=CARTESIAN_POINT('Ctrl Pts',(61.4316917395918,-34.3532773877089,12.));
#57881=CARTESIAN_POINT('Ctrl Pts',(61.4117816420228,-34.3485913645979,12.));
#57882=CARTESIAN_POINT('Ctrl Pts',(61.3919267945302,-34.3438961902405,12.));
#57883=CARTESIAN_POINT('Ctrl Pts',(61.3721273534256,-34.339191990014,12.));
#57884=CARTESIAN_POINT('Ctrl Pts',(61.3523834803188,-34.3344788934363,12.));
#57885=CARTESIAN_POINT('Ctrl Pts',(61.3326953378851,-34.3297570310146,12.));
#57886=CARTESIAN_POINT('Ctrl Pts',(61.3130630861386,-34.3250265314768,12.));
#57887=CARTESIAN_POINT('Ctrl Pts',(61.2934868791854,-34.3202875193618,12.));
#57888=CARTESIAN_POINT('Ctrl Pts',(61.2739668600365,-34.3155401111747,12.));
#57889=CARTESIAN_POINT('Ctrl Pts',(61.2545031656133,-34.3107844191044,12.));
#57890=CARTESIAN_POINT('Ctrl Pts',(61.2350959366939,-34.3060205584065,12.));
#57891=CARTESIAN_POINT('Ctrl Pts',(61.2157453259107,-34.3012486533474,12.));
#57892=CARTESIAN_POINT('Ctrl Pts',(61.1964515073891,-34.2964688443663,12.));
#57893=CARTESIAN_POINT('Ctrl Pts',(61.1772146833205,-34.2916812929751,12.));
#57894=CARTESIAN_POINT('Ctrl Pts',(61.1580350635532,-34.2868861666384,12.));
#57895=CARTESIAN_POINT('Ctrl Pts',(61.1389128461885,-34.282083624447,12.));
#57896=CARTESIAN_POINT('Ctrl Pts',(61.1198481997764,-34.2772738038771,12.));
#57897=CARTESIAN_POINT('Ctrl Pts',(61.1008412399997,-34.2724568037228,12.));
#57898=CARTESIAN_POINT('Ctrl Pts',(61.0818920286293,-34.2676326825626,12.));
#57899=CARTESIAN_POINT('Ctrl Pts',(61.0667788793266,-34.2637677131935,12.));
#57900=CARTESIAN_POINT('Ctrl Pts',(61.0554700176998,-34.2608658001631,12.));
#57901=CARTESIAN_POINT('Ctrl Pts',(61.0479423318725,-34.2589297755434,12.));
#57902=CARTESIAN_POINT('Ctrl Pts',(61.0441813777723,-34.2579614092497,12.));
#57903=CARTESIAN_POINT('Ctrl Pts',(66.1657795405962,-33.590372266528,-5.55111512312578E-16));
#57904=CARTESIAN_POINT('Ctrl Pts',(66.1657795405962,-33.590372266528,4.));
#57905=CARTESIAN_POINT('Ctrl Pts',(66.1657795405962,-33.590372266528,8.));
#57906=CARTESIAN_POINT('Ctrl Pts',(66.1657795405962,-33.590372266528,12.));
#57907=CARTESIAN_POINT('Ctrl Pts',(66.2346881970582,-33.6759628819919,-5.55111512312578E-16));
#57908=CARTESIAN_POINT('Ctrl Pts',(66.2346881970582,-33.6759628819919,4.));
#57909=CARTESIAN_POINT('Ctrl Pts',(66.2346881970582,-33.675962881992,8.));
#57910=CARTESIAN_POINT('Ctrl Pts',(66.2346881970582,-33.675962881992,12.));
#57911=CARTESIAN_POINT('Ctrl Pts',(66.3036153738448,-33.8665453669335,-5.55111512312578E-16));
#57912=CARTESIAN_POINT('Ctrl Pts',(66.3036153738448,-33.8665453669335,4.));
#57913=CARTESIAN_POINT('Ctrl Pts',(66.3036153738447,-33.8665453669334,8.));
#57914=CARTESIAN_POINT('Ctrl Pts',(66.3036153738447,-33.8665453669334,12.));
#57915=CARTESIAN_POINT('Ctrl Pts',(66.2585076236406,-34.0597557125863,-5.55111512312578E-16));
#57916=CARTESIAN_POINT('Ctrl Pts',(66.2585076236406,-34.0597557125863,4.));
#57917=CARTESIAN_POINT('Ctrl Pts',(66.2585076236405,-34.0597557125862,8.));
#57918=CARTESIAN_POINT('Ctrl Pts',(66.2585076236405,-34.0597557125862,12.));
#57919=CARTESIAN_POINT('Ctrl Pts',(66.2207497120656,-34.1330090612018,-5.55111512312578E-16));
#57920=CARTESIAN_POINT('Ctrl Pts',(66.2207497120656,-34.1330090612018,4.));
#57921=CARTESIAN_POINT('Ctrl Pts',(66.2207497120656,-34.1330090612017,8.));
#57922=CARTESIAN_POINT('Ctrl Pts',(66.2207497120656,-34.1330090612017,12.));
#57923=CARTESIAN_POINT('',(66.1657795405962,-33.590372266528,-2.77555756156289E-16));
#57924=CARTESIAN_POINT('',(66.2207497120649,-34.1330090612014,2.77555756156289E-16));
#57925=CARTESIAN_POINT('Ctrl Pts',(66.1657795405962,-33.590372266528,-5.44214888274584E-16));
#57926=CARTESIAN_POINT('Ctrl Pts',(66.2346881970582,-33.6759628819919,-5.44214888274584E-16));
#57927=CARTESIAN_POINT('Ctrl Pts',(66.274075155222,-33.7848671591014,-5.44214888274584E-16));
#57928=CARTESIAN_POINT('Ctrl Pts',(66.2762262188581,-33.8946295131778,-5.44214888274584E-16));
#57929=CARTESIAN_POINT('Ctrl Pts',(66.2778395165852,-33.9769512787351,-5.44214888274584E-16));
#57930=CARTESIAN_POINT('Ctrl Pts',(66.2585076236406,-34.0597557125863,-5.44214888274584E-16));
#57931=CARTESIAN_POINT('Ctrl Pts',(66.2207497120656,-34.1330090612018,-5.44214888274584E-16));
#57932=CARTESIAN_POINT('',(66.2207497120649,-34.1330090612013,12.));
#57933=CARTESIAN_POINT('Ctrl Pts',(66.2207497120656,-34.1330090612018,-5.55111512312578E-16));
#57934=CARTESIAN_POINT('Ctrl Pts',(66.2207497120656,-34.1330090612018,4.));
#57935=CARTESIAN_POINT('Ctrl Pts',(66.2207497120656,-34.1330090612017,8.));
#57936=CARTESIAN_POINT('Ctrl Pts',(66.2207497120656,-34.1330090612017,12.));
#57937=CARTESIAN_POINT('',(66.1657795405962,-33.590372266528,12.));
#57938=CARTESIAN_POINT('Ctrl Pts',(66.2207497120656,-34.1330090612017,12.));
#57939=CARTESIAN_POINT('Ctrl Pts',(66.2585076236405,-34.0597557125862,12.));
#57940=CARTESIAN_POINT('Ctrl Pts',(66.2778395165851,-33.976951278735,12.));
#57941=CARTESIAN_POINT('Ctrl Pts',(66.2762262188581,-33.8946295131777,12.));
#57942=CARTESIAN_POINT('Ctrl Pts',(66.2740751552219,-33.7848671591014,12.));
#57943=CARTESIAN_POINT('Ctrl Pts',(66.2346881970582,-33.675962881992,12.));
#57944=CARTESIAN_POINT('Ctrl Pts',(66.1657795405962,-33.590372266528,12.));
#57945=CARTESIAN_POINT('Ctrl Pts',(66.1657795405962,-33.590372266528,12.));
#57946=CARTESIAN_POINT('Ctrl Pts',(66.1657795405962,-33.590372266528,8.));
#57947=CARTESIAN_POINT('Ctrl Pts',(66.1657795405962,-33.590372266528,4.));
#57948=CARTESIAN_POINT('Ctrl Pts',(66.1657795405962,-33.590372266528,-5.55111512312578E-16));
#57949=CARTESIAN_POINT('Origin',(3.3253631270614E-10,-1.72995545227681E-10,
0.));
#57950=CARTESIAN_POINT('Origin',(3.3253631270614E-10,-1.72995545227681E-10,
12.));
#57951=CARTESIAN_POINT('Origin',(3.3253631270614E-10,-1.72995545227681E-10,
0.));
#57952=CARTESIAN_POINT('Ctrl Pts',(62.6704278106385,-40.2823469776966,0.));
#57953=CARTESIAN_POINT('Ctrl Pts',(62.6704278106385,-40.2823469776966,4.));
#57954=CARTESIAN_POINT('Ctrl Pts',(62.6704278106385,-40.2823469776966,8.));
#57955=CARTESIAN_POINT('Ctrl Pts',(62.6704278106385,-40.2823469776966,12.));
#57956=CARTESIAN_POINT('Ctrl Pts',(62.6110140705996,-40.374781624271,0.));
#57957=CARTESIAN_POINT('Ctrl Pts',(62.6110140705996,-40.374781624271,4.));
#57958=CARTESIAN_POINT('Ctrl Pts',(62.6110140705996,-40.374781624271,8.));
#57959=CARTESIAN_POINT('Ctrl Pts',(62.6110140705996,-40.374781624271,12.));
#57960=CARTESIAN_POINT('Ctrl Pts',(62.451999785206,-40.5004281293559,0.));
#57961=CARTESIAN_POINT('Ctrl Pts',(62.451999785206,-40.5004281293559,4.));
#57962=CARTESIAN_POINT('Ctrl Pts',(62.451999785206,-40.5004281293559,7.99999999999999));
#57963=CARTESIAN_POINT('Ctrl Pts',(62.451999785206,-40.5004281293559,12.));
#57964=CARTESIAN_POINT('Ctrl Pts',(62.2544389573111,-40.5187208145707,0.));
#57965=CARTESIAN_POINT('Ctrl Pts',(62.2544389573111,-40.5187208145707,4.));
#57966=CARTESIAN_POINT('Ctrl Pts',(62.2544389573111,-40.5187208145707,8.00000000000001));
#57967=CARTESIAN_POINT('Ctrl Pts',(62.2544389573111,-40.5187208145707,12.));
#57968=CARTESIAN_POINT('Ctrl Pts',(62.1730054756448,-40.506059810084,0.));
#57969=CARTESIAN_POINT('Ctrl Pts',(62.1730054756448,-40.506059810084,4.));
#57970=CARTESIAN_POINT('Ctrl Pts',(62.1730054756447,-40.506059810084,8.));
#57971=CARTESIAN_POINT('Ctrl Pts',(62.1730054756447,-40.506059810084,12.));
#57972=CARTESIAN_POINT('',(62.6704278106385,-40.2823469776966,0.));
#57973=CARTESIAN_POINT('',(62.1730054756448,-40.5060598100837,0.));
#57974=CARTESIAN_POINT('Ctrl Pts',(62.6704278106385,-40.2823469776966,0.));
#57975=CARTESIAN_POINT('Ctrl Pts',(62.6110140705996,-40.374781624271,0.));
#57976=CARTESIAN_POINT('Ctrl Pts',(62.5201487646604,-40.4465796271766,0.));
#57977=CARTESIAN_POINT('Ctrl Pts',(62.4166968325983,-40.4833233215533,0.));
#57978=CARTESIAN_POINT('Ctrl Pts',(62.3391078835518,-40.5108810923358,0.));
#57979=CARTESIAN_POINT('Ctrl Pts',(62.2544389573111,-40.5187208145707,0.));
#57980=CARTESIAN_POINT('Ctrl Pts',(62.1730054756448,-40.506059810084,0.));
#57981=CARTESIAN_POINT('',(62.1730054756448,-40.5060598100837,12.));
#57982=CARTESIAN_POINT('Ctrl Pts',(62.1730054756448,-40.506059810084,0.));
#57983=CARTESIAN_POINT('Ctrl Pts',(62.1730054756448,-40.506059810084,4.));
#57984=CARTESIAN_POINT('Ctrl Pts',(62.1730054756447,-40.506059810084,8.));
#57985=CARTESIAN_POINT('Ctrl Pts',(62.1730054756447,-40.506059810084,12.));
#57986=CARTESIAN_POINT('',(62.6704278106385,-40.2823469776966,12.));
#57987=CARTESIAN_POINT('Ctrl Pts',(62.1730054756447,-40.506059810084,12.));
#57988=CARTESIAN_POINT('Ctrl Pts',(62.2544389573111,-40.5187208145707,12.));
#57989=CARTESIAN_POINT('Ctrl Pts',(62.3391078835518,-40.5108810923358,12.));
#57990=CARTESIAN_POINT('Ctrl Pts',(62.4166968325983,-40.4833233215533,12.));
#57991=CARTESIAN_POINT('Ctrl Pts',(62.5201487646604,-40.4465796271767,12.));
#57992=CARTESIAN_POINT('Ctrl Pts',(62.6110140705996,-40.374781624271,12.));
#57993=CARTESIAN_POINT('Ctrl Pts',(62.6704278106385,-40.2823469776966,12.));
#57994=CARTESIAN_POINT('Ctrl Pts',(62.6704278106385,-40.2823469776966,12.));
#57995=CARTESIAN_POINT('Ctrl Pts',(62.6704278106385,-40.2823469776966,8.));
#57996=CARTESIAN_POINT('Ctrl Pts',(62.6704278106385,-40.2823469776966,4.));
#57997=CARTESIAN_POINT('Ctrl Pts',(62.6704278106385,-40.2823469776966,0.));
#57998=CARTESIAN_POINT('Ctrl Pts',(57.8261117662438,-39.4479504917287,0.));
#57999=CARTESIAN_POINT('Ctrl Pts',(57.8261117662438,-39.4479504917287,12.));
#58000=CARTESIAN_POINT('Ctrl Pts',(57.8297740100947,-39.4492429618443,0.));
#58001=CARTESIAN_POINT('Ctrl Pts',(57.8297740100947,-39.4492429618443,12.));
#58002=CARTESIAN_POINT('Ctrl Pts',(57.837104315141,-39.4518277003553,0.));
#58003=CARTESIAN_POINT('Ctrl Pts',(57.837104315141,-39.4518277003553,12.));
#58004=CARTESIAN_POINT('Ctrl Pts',(57.8481172247495,-39.4557042029652,0.));
#58005=CARTESIAN_POINT('Ctrl Pts',(57.8481172247495,-39.4557042029652,12.));
#58006=CARTESIAN_POINT('Ctrl Pts',(57.8628360096803,-39.4608716627118,0.));
#58007=CARTESIAN_POINT('Ctrl Pts',(57.8628360096803,-39.4608716627118,12.));
#58008=CARTESIAN_POINT('Ctrl Pts',(57.8812926637177,-39.4673289592259,0.));
#58009=CARTESIAN_POINT('Ctrl Pts',(57.8812926637177,-39.4673289592259,12.));
#58010=CARTESIAN_POINT('Ctrl Pts',(57.8998074670478,-39.473784194937,0.));
#58011=CARTESIAN_POINT('Ctrl Pts',(57.8998074670478,-39.473784194937,12.));
#58012=CARTESIAN_POINT('Ctrl Pts',(57.9183803632403,-39.4802373061058,0.));
#58013=CARTESIAN_POINT('Ctrl Pts',(57.9183803632403,-39.4802373061058,12.));
#58014=CARTESIAN_POINT('Ctrl Pts',(57.937011245663,-39.4866881842317,0.));
#58015=CARTESIAN_POINT('Ctrl Pts',(57.937011245663,-39.4866881842317,12.));
#58016=CARTESIAN_POINT('Ctrl Pts',(57.9556999583892,-39.4931366776714,0.));
#58017=CARTESIAN_POINT('Ctrl Pts',(57.9556999583892,-39.4931366776714,12.));
#58018=CARTESIAN_POINT('Ctrl Pts',(57.974446317937,-39.499582610674,0.));
#58019=CARTESIAN_POINT('Ctrl Pts',(57.974446317937,-39.499582610674,12.));
#58020=CARTESIAN_POINT('Ctrl Pts',(57.9932501298522,-39.5060257981225,0.));
#58021=CARTESIAN_POINT('Ctrl Pts',(57.9932501298522,-39.5060257981225,12.));
#58022=CARTESIAN_POINT('Ctrl Pts',(58.0121112067895,-39.5124660614976,0.));
#58023=CARTESIAN_POINT('Ctrl Pts',(58.0121112067895,-39.5124660614976,12.));
#58024=CARTESIAN_POINT('Ctrl Pts',(58.0310293875262,-39.5189032457184,0.));
#58025=CARTESIAN_POINT('Ctrl Pts',(58.0310293875262,-39.5189032457184,12.));
#58026=CARTESIAN_POINT('Ctrl Pts',(58.0500045308412,-39.5253372136887,0.));
#58027=CARTESIAN_POINT('Ctrl Pts',(58.0500045308412,-39.5253372136887,12.));
#58028=CARTESIAN_POINT('Ctrl Pts',(58.0690365065374,-39.5317678383217,0.));
#58029=CARTESIAN_POINT('Ctrl Pts',(58.0690365065374,-39.5317678383217,12.));
#58030=CARTESIAN_POINT('Ctrl Pts',(58.088125187992,-39.5381949959221,0.));
#58031=CARTESIAN_POINT('Ctrl Pts',(58.088125187992,-39.5381949959221,12.));
#58032=CARTESIAN_POINT('Ctrl Pts',(58.1072704428928,-39.5446185579638,0.));
#58033=CARTESIAN_POINT('Ctrl Pts',(58.1072704428928,-39.5446185579638,12.));
#58034=CARTESIAN_POINT('Ctrl Pts',(58.126472128574,-39.5510383869505,0.));
#58035=CARTESIAN_POINT('Ctrl Pts',(58.126472128574,-39.5510383869505,12.));
#58036=CARTESIAN_POINT('Ctrl Pts',(58.1457300968499,-39.5574543406982,0.));
#58037=CARTESIAN_POINT('Ctrl Pts',(58.1457300968499,-39.5574543406982,12.));
#58038=CARTESIAN_POINT('Ctrl Pts',(58.1650441970387,-39.563866275018,0.));
#58039=CARTESIAN_POINT('Ctrl Pts',(58.1650441970387,-39.563866275018,12.));
#58040=CARTESIAN_POINT('Ctrl Pts',(58.1844142794338,-39.5702740467999,0.));
#58041=CARTESIAN_POINT('Ctrl Pts',(58.1844142794338,-39.5702740467999,12.));
#58042=CARTESIAN_POINT('Ctrl Pts',(58.2038401992457,-39.57667751752,0.));
#58043=CARTESIAN_POINT('Ctrl Pts',(58.2038401992457,-39.57667751752,12.));
#58044=CARTESIAN_POINT('Ctrl Pts',(58.2233218164365,-39.5830765530891,0.));
#58045=CARTESIAN_POINT('Ctrl Pts',(58.2233218164365,-39.5830765530891,12.));
#58046=CARTESIAN_POINT('Ctrl Pts',(58.2428589938369,-39.5894710221713,0.));
#58047=CARTESIAN_POINT('Ctrl Pts',(58.2428589938369,-39.5894710221713,12.));
#58048=CARTESIAN_POINT('Ctrl Pts',(58.2624515958419,-39.5958607950239,0.));
#58049=CARTESIAN_POINT('Ctrl Pts',(58.2624515958419,-39.5958607950239,12.));
#58050=CARTESIAN_POINT('Ctrl Pts',(58.2820994868118,-39.602245742079,0.));
#58051=CARTESIAN_POINT('Ctrl Pts',(58.2820994868118,-39.602245742079,12.));
#58052=CARTESIAN_POINT('Ctrl Pts',(58.3018025297323,-39.6086257327583,0.));
#58053=CARTESIAN_POINT('Ctrl Pts',(58.3018025297323,-39.6086257327583,12.));
#58054=CARTESIAN_POINT('Ctrl Pts',(58.3215605869221,-39.6150006360915,0.));
#58055=CARTESIAN_POINT('Ctrl Pts',(58.3215605869221,-39.6150006360915,12.));
#58056=CARTESIAN_POINT('Ctrl Pts',(58.3413735206423,-39.6213703212531,0.));
#58057=CARTESIAN_POINT('Ctrl Pts',(58.3413735206423,-39.6213703212531,12.));
#58058=CARTESIAN_POINT('Ctrl Pts',(58.3612411936904,-39.6277346580892,0.));
#58059=CARTESIAN_POINT('Ctrl Pts',(58.3612411936904,-39.6277346580892,12.));
#58060=CARTESIAN_POINT('Ctrl Pts',(58.3811634701037,-39.6340935177476,0.));
#58061=CARTESIAN_POINT('Ctrl Pts',(58.3811634701037,-39.6340935177476,12.));
#58062=CARTESIAN_POINT('Ctrl Pts',(58.4011402154196,-39.6404467729094,0.));
#58063=CARTESIAN_POINT('Ctrl Pts',(58.4011402154196,-39.6404467729094,12.));
#58064=CARTESIAN_POINT('Ctrl Pts',(58.4211712963004,-39.6467942974451,0.));
#58065=CARTESIAN_POINT('Ctrl Pts',(58.4211712963004,-39.6467942974451,12.));
#58066=CARTESIAN_POINT('Ctrl Pts',(58.4412565802979,-39.653135966204,0.));
#58067=CARTESIAN_POINT('Ctrl Pts',(58.4412565802979,-39.653135966204,12.));
#58068=CARTESIAN_POINT('Ctrl Pts',(58.4613959355788,-39.6594716547689,0.));
#58069=CARTESIAN_POINT('Ctrl Pts',(58.4613959355788,-39.6594716547689,12.));
#58070=CARTESIAN_POINT('Ctrl Pts',(58.4815892306066,-39.6658012391815,0.));
#58071=CARTESIAN_POINT('Ctrl Pts',(58.4815892306066,-39.6658012391815,12.));
#58072=CARTESIAN_POINT('Ctrl Pts',(58.5018363341604,-39.6721245959531,0.));
#58073=CARTESIAN_POINT('Ctrl Pts',(58.5018363341604,-39.6721245959531,12.));
#58074=CARTESIAN_POINT('Ctrl Pts',(58.5221371154761,-39.6784416021826,0.));
#58075=CARTESIAN_POINT('Ctrl Pts',(58.5221371154761,-39.6784416021826,12.));
#58076=CARTESIAN_POINT('Ctrl Pts',(58.5424914443415,-39.6847521356395,0.));
#58077=CARTESIAN_POINT('Ctrl Pts',(58.5424914443415,-39.6847521356395,12.));
#58078=CARTESIAN_POINT('Ctrl Pts',(58.5628991912052,-39.6910560748629,0.));
#58079=CARTESIAN_POINT('Ctrl Pts',(58.5628991912052,-39.6910560748629,12.));
#58080=CARTESIAN_POINT('Ctrl Pts',(58.5833602272743,-39.697353299254,0.));
#58081=CARTESIAN_POINT('Ctrl Pts',(58.5833602272743,-39.697353299254,12.));
#58082=CARTESIAN_POINT('Ctrl Pts',(58.6038744244659,-39.7036436890233,0.));
#58083=CARTESIAN_POINT('Ctrl Pts',(58.6038744244659,-39.7036436890233,12.));
#58084=CARTESIAN_POINT('Ctrl Pts',(58.6244416553562,-39.7099271251413,0.));
#58085=CARTESIAN_POINT('Ctrl Pts',(58.6244416553562,-39.7099271251413,12.));
#58086=CARTESIAN_POINT('Ctrl Pts',(58.6450617931274,-39.71620348929,0.));
#58087=CARTESIAN_POINT('Ctrl Pts',(58.6450617931274,-39.71620348929,12.));
#58088=CARTESIAN_POINT('Ctrl Pts',(58.6657347115034,-39.7224726638101,0.));
#58089=CARTESIAN_POINT('Ctrl Pts',(58.6657347115034,-39.7224726638101,12.));
#58090=CARTESIAN_POINT('Ctrl Pts',(58.6864602847088,-39.7287345316681,0.));
#58091=CARTESIAN_POINT('Ctrl Pts',(58.6864602847088,-39.7287345316681,12.));
#58092=CARTESIAN_POINT('Ctrl Pts',(58.7072383875027,-39.734988976475,0.));
#58093=CARTESIAN_POINT('Ctrl Pts',(58.7072383875027,-39.734988976475,12.));
#58094=CARTESIAN_POINT('Ctrl Pts',(58.7280688951916,-39.7412358824953,0.));
#58095=CARTESIAN_POINT('Ctrl Pts',(58.7280688951916,-39.7412358824953,12.));
#58096=CARTESIAN_POINT('Ctrl Pts',(58.7489516836445,-39.7474751346599,0.));
#58097=CARTESIAN_POINT('Ctrl Pts',(58.7489516836445,-39.7474751346599,12.));
#58098=CARTESIAN_POINT('Ctrl Pts',(58.7698866293029,-39.7537066185813,0.));
#58099=CARTESIAN_POINT('Ctrl Pts',(58.7698866293029,-39.7537066185813,12.));
#58100=CARTESIAN_POINT('Ctrl Pts',(58.7908736091798,-39.7599302205521,0.));
#58101=CARTESIAN_POINT('Ctrl Pts',(58.7908736091798,-39.7599302205521,12.));
#58102=CARTESIAN_POINT('Ctrl Pts',(58.8119125008517,-39.7661458275274,0.));
#58103=CARTESIAN_POINT('Ctrl Pts',(58.8119125008517,-39.7661458275274,12.));
#58104=CARTESIAN_POINT('Ctrl Pts',(58.8330031824453,-39.772353327112,0.));
#58105=CARTESIAN_POINT('Ctrl Pts',(58.8330031824453,-39.772353327112,12.));
#58106=CARTESIAN_POINT('Ctrl Pts',(58.8541455326231,-39.7785526075479,0.));
#58107=CARTESIAN_POINT('Ctrl Pts',(58.8541455326231,-39.7785526075479,12.));
#58108=CARTESIAN_POINT('Ctrl Pts',(58.8753394305585,-39.7847435576997,0.));
#58109=CARTESIAN_POINT('Ctrl Pts',(58.8753394305585,-39.7847435576997,12.));
#58110=CARTESIAN_POINT('Ctrl Pts',(58.8965847559391,-39.7909260670517,0.));
#58111=CARTESIAN_POINT('Ctrl Pts',(58.8965847559391,-39.7909260670517,12.));
#58112=CARTESIAN_POINT('Ctrl Pts',(58.9178813889703,-39.7971000257044,0.));
#58113=CARTESIAN_POINT('Ctrl Pts',(58.9178813889703,-39.7971000257044,12.));
#58114=CARTESIAN_POINT('Ctrl Pts',(58.9392292103747,-39.8032653243712,0.));
#58115=CARTESIAN_POINT('Ctrl Pts',(58.9392292103747,-39.8032653243712,12.));
#58116=CARTESIAN_POINT('Ctrl Pts',(58.9606281013875,-39.8094218543782,0.));
#58117=CARTESIAN_POINT('Ctrl Pts',(58.9606281013875,-39.8094218543782,12.));
#58118=CARTESIAN_POINT('Ctrl Pts',(58.9820779437484,-39.8155695076626,0.));
#58119=CARTESIAN_POINT('Ctrl Pts',(58.9820779437484,-39.8155695076626,12.));
#58120=CARTESIAN_POINT('Ctrl Pts',(59.0035786197024,-39.821708176766,0.));
#58121=CARTESIAN_POINT('Ctrl Pts',(59.0035786197024,-39.821708176766,12.));
#58122=CARTESIAN_POINT('Ctrl Pts',(59.0251300119973,-39.8278377548262,0.));
#58123=CARTESIAN_POINT('Ctrl Pts',(59.0251300119973,-39.8278377548262,12.));
#58124=CARTESIAN_POINT('Ctrl Pts',(59.0467320038784,-39.8339581355716,0.));
#58125=CARTESIAN_POINT('Ctrl Pts',(59.0467320038784,-39.8339581355716,12.));
#58126=CARTESIAN_POINT('Ctrl Pts',(59.0683844790764,-39.8400692133139,0.));
#58127=CARTESIAN_POINT('Ctrl Pts',(59.0683844790764,-39.8400692133139,12.));
#58128=CARTESIAN_POINT('Ctrl Pts',(59.090087321798,-39.8461708829456,0.));
#58129=CARTESIAN_POINT('Ctrl Pts',(59.090087321798,-39.8461708829456,12.));
#58130=CARTESIAN_POINT('Ctrl Pts',(59.1118404167292,-39.8522630399328,0.));
#58131=CARTESIAN_POINT('Ctrl Pts',(59.1118404167292,-39.8522630399328,12.));
#58132=CARTESIAN_POINT('Ctrl Pts',(59.1336436490342,-39.8583455803105,0.));
#58133=CARTESIAN_POINT('Ctrl Pts',(59.1336436490342,-39.8583455803105,12.));
#58134=CARTESIAN_POINT('Ctrl Pts',(59.1554969043522,-39.8644184006787,0.));
#58135=CARTESIAN_POINT('Ctrl Pts',(59.1554969043522,-39.8644184006787,12.));
#58136=CARTESIAN_POINT('Ctrl Pts',(59.1774000687879,-39.8704813981989,0.));
#58137=CARTESIAN_POINT('Ctrl Pts',(59.1774000687879,-39.8704813981989,12.));
#58138=CARTESIAN_POINT('Ctrl Pts',(59.1993530289028,-39.876534470591,0.));
#58139=CARTESIAN_POINT('Ctrl Pts',(59.1993530289028,-39.876534470591,12.));
#58140=CARTESIAN_POINT('Ctrl Pts',(59.2213556717209,-39.8825775161267,0.));
#58141=CARTESIAN_POINT('Ctrl Pts',(59.2213556717209,-39.8825775161267,12.));
#58142=CARTESIAN_POINT('Ctrl Pts',(59.2434078847247,-39.8886104336242,0.));
#58143=CARTESIAN_POINT('Ctrl Pts',(59.2434078847247,-39.8886104336242,12.));
#58144=CARTESIAN_POINT('Ctrl Pts',(59.2655095558521,-39.8946331224438,0.));
#58145=CARTESIAN_POINT('Ctrl Pts',(59.2655095558521,-39.8946331224438,12.));
#58146=CARTESIAN_POINT('Ctrl Pts',(59.2876605734846,-39.9006454824845,0.));
#58147=CARTESIAN_POINT('Ctrl Pts',(59.2876605734846,-39.9006454824845,12.));
#58148=CARTESIAN_POINT('Ctrl Pts',(59.3098608264419,-39.9066474141803,0.));
#58149=CARTESIAN_POINT('Ctrl Pts',(59.3098608264419,-39.9066474141803,12.));
#58150=CARTESIAN_POINT('Ctrl Pts',(59.3321102039852,-39.9126388184936,0.));
#58151=CARTESIAN_POINT('Ctrl Pts',(59.3321102039852,-39.9126388184936,12.));
#58152=CARTESIAN_POINT('Ctrl Pts',(59.3544085958151,-39.9186195969104,0.));
#58153=CARTESIAN_POINT('Ctrl Pts',(59.3544085958151,-39.9186195969104,12.));
#58154=CARTESIAN_POINT('Ctrl Pts',(59.3767558920675,-39.9245896514367,0.));
#58155=CARTESIAN_POINT('Ctrl Pts',(59.3767558920675,-39.9245896514367,12.));
#58156=CARTESIAN_POINT('Ctrl Pts',(59.3991519833016,-39.9305488845958,0.));
#58157=CARTESIAN_POINT('Ctrl Pts',(59.3991519833016,-39.9305488845958,12.));
#58158=CARTESIAN_POINT('Ctrl Pts',(59.4215967604967,-39.9364971994242,0.));
#58159=CARTESIAN_POINT('Ctrl Pts',(59.4215967604967,-39.9364971994242,12.));
#58160=CARTESIAN_POINT('Ctrl Pts',(59.4440901150582,-39.9424344994673,0.));
#58161=CARTESIAN_POINT('Ctrl Pts',(59.4440901150582,-39.9424344994673,12.));
#58162=CARTESIAN_POINT('Ctrl Pts',(59.4666319388133,-39.9483606887738,0.));
#58163=CARTESIAN_POINT('Ctrl Pts',(59.4666319388133,-39.9483606887738,12.));
#58164=CARTESIAN_POINT('Ctrl Pts',(59.4892221240068,-39.9542756718922,0.));
#58165=CARTESIAN_POINT('Ctrl Pts',(59.4892221240068,-39.9542756718922,12.));
#58166=CARTESIAN_POINT('Ctrl Pts',(59.511860563289,-39.9601793538683,0.));
#58167=CARTESIAN_POINT('Ctrl Pts',(59.511860563289,-39.9601793538683,12.));
#58168=CARTESIAN_POINT('Ctrl Pts',(59.5345471497128,-39.9660716402403,0.));
#58169=CARTESIAN_POINT('Ctrl Pts',(59.5345471497128,-39.9660716402403,12.));
#58170=CARTESIAN_POINT('Ctrl Pts',(59.5572817767388,-39.9719524370346,0.));
#58171=CARTESIAN_POINT('Ctrl Pts',(59.5572817767388,-39.9719524370346,12.));
#58172=CARTESIAN_POINT('Ctrl Pts',(59.5800643382314,-39.9778216507605,0.));
#58173=CARTESIAN_POINT('Ctrl Pts',(59.5800643382314,-39.9778216507605,12.));
#58174=CARTESIAN_POINT('Ctrl Pts',(59.6028947284562,-39.9836791884079,0.));
#58175=CARTESIAN_POINT('Ctrl Pts',(59.6028947284562,-39.9836791884079,12.));
#58176=CARTESIAN_POINT('Ctrl Pts',(59.6257728420669,-39.9895249574448,0.));
#58177=CARTESIAN_POINT('Ctrl Pts',(59.6257728420669,-39.9895249574448,12.));
#58178=CARTESIAN_POINT('Ctrl Pts',(59.6486985741041,-39.9953588658132,0.));
#58179=CARTESIAN_POINT('Ctrl Pts',(59.6486985741041,-39.9953588658132,12.));
#58180=CARTESIAN_POINT('Ctrl Pts',(59.6716718200005,-40.0011808219241,0.));
#58181=CARTESIAN_POINT('Ctrl Pts',(59.6716718200005,-40.0011808219241,12.));
#58182=CARTESIAN_POINT('Ctrl Pts',(59.6946924755773,-40.0069907346538,0.));
#58183=CARTESIAN_POINT('Ctrl Pts',(59.6946924755773,-40.0069907346538,12.));
#58184=CARTESIAN_POINT('Ctrl Pts',(59.7177604370403,-40.0127885133403,0.));
#58185=CARTESIAN_POINT('Ctrl Pts',(59.7177604370403,-40.0127885133403,12.));
#58186=CARTESIAN_POINT('Ctrl Pts',(59.7408756009679,-40.0185740677821,0.));
#58187=CARTESIAN_POINT('Ctrl Pts',(59.7408756009679,-40.0185740677821,12.));
#58188=CARTESIAN_POINT('Ctrl Pts',(59.7640378643106,-40.0243473082337,0.));
#58189=CARTESIAN_POINT('Ctrl Pts',(59.7640378643106,-40.0243473082337,12.));
#58190=CARTESIAN_POINT('Ctrl Pts',(59.7872471243942,-40.0301081454002,0.));
#58191=CARTESIAN_POINT('Ctrl Pts',(59.7872471243942,-40.0301081454002,12.));
#58192=CARTESIAN_POINT('Ctrl Pts',(59.8105032789179,-40.0358564904341,0.));
#58193=CARTESIAN_POINT('Ctrl Pts',(59.8105032789179,-40.0358564904341,12.));
#58194=CARTESIAN_POINT('Ctrl Pts',(59.8338062259492,-40.0415922549315,0.));
#58195=CARTESIAN_POINT('Ctrl Pts',(59.8338062259492,-40.0415922549315,12.));
#58196=CARTESIAN_POINT('Ctrl Pts',(59.8571558639145,-40.0473153509324,0.));
#58197=CARTESIAN_POINT('Ctrl Pts',(59.8571558639145,-40.0473153509324,12.));
#58198=CARTESIAN_POINT('Ctrl Pts',(59.8805520915972,-40.0530256909161,0.));
#58199=CARTESIAN_POINT('Ctrl Pts',(59.8805520915972,-40.0530256909161,12.));
#58200=CARTESIAN_POINT('Ctrl Pts',(59.9039948081428,-40.0587231877959,0.));
#58201=CARTESIAN_POINT('Ctrl Pts',(59.9039948081428,-40.0587231877959,12.));
#58202=CARTESIAN_POINT('Ctrl Pts',(59.927483913055,-40.0644077549158,0.));
#58203=CARTESIAN_POINT('Ctrl Pts',(59.927483913055,-40.0644077549158,12.));
#58204=CARTESIAN_POINT('Ctrl Pts',(59.9510193061929,-40.0700793060475,0.));
#58205=CARTESIAN_POINT('Ctrl Pts',(59.9510193061929,-40.0700793060475,12.));
#58206=CARTESIAN_POINT('Ctrl Pts',(59.974600887759,-40.0757377553894,0.));
#58207=CARTESIAN_POINT('Ctrl Pts',(59.974600887759,-40.0757377553894,12.));
#58208=CARTESIAN_POINT('Ctrl Pts',(59.9982285582991,-40.0813830175629,0.));
#58209=CARTESIAN_POINT('Ctrl Pts',(59.9982285582991,-40.0813830175629,12.));
#58210=CARTESIAN_POINT('Ctrl Pts',(60.0219022187066,-40.0870150076078,0.));
#58211=CARTESIAN_POINT('Ctrl Pts',(60.0219022187066,-40.0870150076078,12.));
#58212=CARTESIAN_POINT('Ctrl Pts',(60.0456217702203,-40.0926336409787,0.));
#58213=CARTESIAN_POINT('Ctrl Pts',(60.0456217702203,-40.0926336409787,12.));
#58214=CARTESIAN_POINT('Ctrl Pts',(60.0693871144207,-40.0982388335421,0.));
#58215=CARTESIAN_POINT('Ctrl Pts',(60.0693871144207,-40.0982388335421,12.));
#58216=CARTESIAN_POINT('Ctrl Pts',(60.0931981532194,-40.1038305015764,0.));
#58217=CARTESIAN_POINT('Ctrl Pts',(60.0931981532194,-40.1038305015764,12.));
#58218=CARTESIAN_POINT('Ctrl Pts',(60.1170547888572,-40.1094085617672,0.));
#58219=CARTESIAN_POINT('Ctrl Pts',(60.1170547888572,-40.1094085617672,12.));
#58220=CARTESIAN_POINT('Ctrl Pts',(60.1409569239092,-40.1149729312036,0.));
#58221=CARTESIAN_POINT('Ctrl Pts',(60.1409569239092,-40.1149729312036,12.));
#58222=CARTESIAN_POINT('Ctrl Pts',(60.1649044612829,-40.120523527374,0.));
#58223=CARTESIAN_POINT('Ctrl Pts',(60.1649044612829,-40.120523527374,12.));
#58224=CARTESIAN_POINT('Ctrl Pts',(60.1888973042151,-40.1260602681644,0.));
#58225=CARTESIAN_POINT('Ctrl Pts',(60.1888973042151,-40.1260602681644,12.));
#58226=CARTESIAN_POINT('Ctrl Pts',(60.2129353562617,-40.1315830718575,0.));
#58227=CARTESIAN_POINT('Ctrl Pts',(60.2129353562617,-40.1315830718575,12.));
#58228=CARTESIAN_POINT('Ctrl Pts',(60.2370185212957,-40.13709185713,0.));
#58229=CARTESIAN_POINT('Ctrl Pts',(60.2370185212957,-40.13709185713,12.));
#58230=CARTESIAN_POINT('Ctrl Pts',(60.2611467035109,-40.1425865430468,0.));
#58231=CARTESIAN_POINT('Ctrl Pts',(60.2611467035109,-40.1425865430468,12.));
#58232=CARTESIAN_POINT('Ctrl Pts',(60.2853198074215,-40.1480670490583,0.));
#58233=CARTESIAN_POINT('Ctrl Pts',(60.2853198074215,-40.1480670490583,12.));
#58234=CARTESIAN_POINT('Ctrl Pts',(60.3095377378589,-40.1535332949978,0.));
#58235=CARTESIAN_POINT('Ctrl Pts',(60.3095377378589,-40.1535332949978,12.));
#58236=CARTESIAN_POINT('Ctrl Pts',(60.3338003999616,-40.1589852010811,0.));
#58237=CARTESIAN_POINT('Ctrl Pts',(60.3338003999616,-40.1589852010811,12.));
#58238=CARTESIAN_POINT('Ctrl Pts',(60.3581076991731,-40.1644226879043,0.));
#58239=CARTESIAN_POINT('Ctrl Pts',(60.3581076991731,-40.1644226879043,12.));
#58240=CARTESIAN_POINT('Ctrl Pts',(60.382459541246,-40.1698456764387,0.));
#58241=CARTESIAN_POINT('Ctrl Pts',(60.382459541246,-40.1698456764387,12.));
#58242=CARTESIAN_POINT('Ctrl Pts',(60.4068558322414,-40.1752540880273,0.));
#58243=CARTESIAN_POINT('Ctrl Pts',(60.4068558322414,-40.1752540880273,12.));
#58244=CARTESIAN_POINT('Ctrl Pts',(60.4312964785269,-40.1806478443829,0.));
#58245=CARTESIAN_POINT('Ctrl Pts',(60.4312964785269,-40.1806478443829,12.));
#58246=CARTESIAN_POINT('Ctrl Pts',(60.4557813867677,-40.1860268675876,0.));
#58247=CARTESIAN_POINT('Ctrl Pts',(60.4557813867677,-40.1860268675876,12.));
#58248=CARTESIAN_POINT('Ctrl Pts',(60.4803104639211,-40.1913910800912,0.));
#58249=CARTESIAN_POINT('Ctrl Pts',(60.4803104639211,-40.1913910800912,12.));
#58250=CARTESIAN_POINT('Ctrl Pts',(60.5048836172423,-40.1967404047055,0.));
#58251=CARTESIAN_POINT('Ctrl Pts',(60.5048836172423,-40.1967404047055,12.));
#58252=CARTESIAN_POINT('Ctrl Pts',(60.5295007542838,-40.2020747646012,0.));
#58253=CARTESIAN_POINT('Ctrl Pts',(60.5295007542838,-40.2020747646012,12.));
#58254=CARTESIAN_POINT('Ctrl Pts',(60.5541617828927,-40.2073940833054,0.));
#58255=CARTESIAN_POINT('Ctrl Pts',(60.5541617828927,-40.2073940833054,12.));
#58256=CARTESIAN_POINT('Ctrl Pts',(60.5788666112043,-40.2126982847012,0.));
#58257=CARTESIAN_POINT('Ctrl Pts',(60.5788666112043,-40.2126982847012,12.));
#58258=CARTESIAN_POINT('Ctrl Pts',(60.6036151476347,-40.2179872930272,0.));
#58259=CARTESIAN_POINT('Ctrl Pts',(60.6036151476347,-40.2179872930272,12.));
#58260=CARTESIAN_POINT('Ctrl Pts',(60.6284073008865,-40.2232610328717,0.));
#58261=CARTESIAN_POINT('Ctrl Pts',(60.6284073008865,-40.2232610328717,12.));
#58262=CARTESIAN_POINT('Ctrl Pts',(60.6532429799493,-40.2285194291702,0.));
#58263=CARTESIAN_POINT('Ctrl Pts',(60.6532429799493,-40.2285194291702,12.));
#58264=CARTESIAN_POINT('Ctrl Pts',(60.6781220940979,-40.2337624072029,0.));
#58265=CARTESIAN_POINT('Ctrl Pts',(60.6781220940979,-40.2337624072029,12.));
#58266=CARTESIAN_POINT('Ctrl Pts',(60.7030445528863,-40.2389898925937,0.));
#58267=CARTESIAN_POINT('Ctrl Pts',(60.7030445528863,-40.2389898925937,12.));
#58268=CARTESIAN_POINT('Ctrl Pts',(60.72801026614,-40.2442018113116,0.));
#58269=CARTESIAN_POINT('Ctrl Pts',(60.72801026614,-40.2442018113116,12.));
#58270=CARTESIAN_POINT('Ctrl Pts',(60.7530191439603,-40.2493980896646,0.));
#58271=CARTESIAN_POINT('Ctrl Pts',(60.7530191439603,-40.2493980896646,12.));
#58272=CARTESIAN_POINT('Ctrl Pts',(60.7780710967253,-40.2545786542957,0.));
#58273=CARTESIAN_POINT('Ctrl Pts',(60.7780710967253,-40.2545786542957,12.));
#58274=CARTESIAN_POINT('Ctrl Pts',(60.8031660350878,-40.2597434321804,0.));
#58275=CARTESIAN_POINT('Ctrl Pts',(60.8031660350878,-40.2597434321804,12.));
#58276=CARTESIAN_POINT('Ctrl Pts',(60.8283038699703,-40.2648923506245,0.));
#58277=CARTESIAN_POINT('Ctrl Pts',(60.8283038699703,-40.2648923506245,12.));
#58278=CARTESIAN_POINT('Ctrl Pts',(60.8534845125535,-40.2700253372644,0.));
#58279=CARTESIAN_POINT('Ctrl Pts',(60.8534845125535,-40.2700253372644,12.));
#58280=CARTESIAN_POINT('Ctrl Pts',(60.8787078742817,-40.2751423200637,0.));
#58281=CARTESIAN_POINT('Ctrl Pts',(60.8787078742817,-40.2751423200637,12.));
#58282=CARTESIAN_POINT('Ctrl Pts',(60.903973866867,-40.2802432273105,0.));
#58283=CARTESIAN_POINT('Ctrl Pts',(60.903973866867,-40.2802432273105,12.));
#58284=CARTESIAN_POINT('Ctrl Pts',(60.9292824022888,-40.2853279876162,0.));
#58285=CARTESIAN_POINT('Ctrl Pts',(60.9292824022888,-40.2853279876162,12.));
#58286=CARTESIAN_POINT('Ctrl Pts',(60.9546333927919,-40.2903965299155,0.));
#58287=CARTESIAN_POINT('Ctrl Pts',(60.9546333927919,-40.2903965299155,12.));
#58288=CARTESIAN_POINT('Ctrl Pts',(60.9800267508781,-40.2954487834688,0.));
#58289=CARTESIAN_POINT('Ctrl Pts',(60.9800267508781,-40.2954487834688,12.));
#58290=CARTESIAN_POINT('Ctrl Pts',(61.0054623893059,-40.3004846778577,0.));
#58291=CARTESIAN_POINT('Ctrl Pts',(61.0054623893059,-40.3004846778577,12.));
#58292=CARTESIAN_POINT('Ctrl Pts',(61.0309402210915,-40.3055041429772,0.));
#58293=CARTESIAN_POINT('Ctrl Pts',(61.0309402210915,-40.3055041429772,12.));
#58294=CARTESIAN_POINT('Ctrl Pts',(61.0564601595047,-40.3105071090308,0.));
#58295=CARTESIAN_POINT('Ctrl Pts',(61.0564601595047,-40.3105071090308,12.));
#58296=CARTESIAN_POINT('Ctrl Pts',(61.0820221180646,-40.3154935065264,0.));
#58297=CARTESIAN_POINT('Ctrl Pts',(61.0820221180646,-40.3154935065264,12.));
#58298=CARTESIAN_POINT('Ctrl Pts',(61.1076260105265,-40.3204632662729,0.));
#58299=CARTESIAN_POINT('Ctrl Pts',(61.1076260105265,-40.3204632662729,12.));
#58300=CARTESIAN_POINT('Ctrl Pts',(61.1332717508799,-40.3254163193806,0.));
#58301=CARTESIAN_POINT('Ctrl Pts',(61.1332717508799,-40.3254163193806,12.));
#58302=CARTESIAN_POINT('Ctrl Pts',(61.1589592533623,-40.3303525972621,0.));
#58303=CARTESIAN_POINT('Ctrl Pts',(61.1589592533623,-40.3303525972621,12.));
#58304=CARTESIAN_POINT('Ctrl Pts',(61.184688432465,-40.3352720316373,0.));
#58305=CARTESIAN_POINT('Ctrl Pts',(61.184688432465,-40.3352720316373,12.));
#58306=CARTESIAN_POINT('Ctrl Pts',(61.2104592029375,-40.3401745545369,0.));
#58307=CARTESIAN_POINT('Ctrl Pts',(61.2104592029375,-40.3401745545369,12.));
#58308=CARTESIAN_POINT('Ctrl Pts',(61.236271479789,-40.3450600983104,0.));
#58309=CARTESIAN_POINT('Ctrl Pts',(61.236271479789,-40.3450600983104,12.));
#58310=CARTESIAN_POINT('Ctrl Pts',(61.2621251782849,-40.3499285956297,0.));
#58311=CARTESIAN_POINT('Ctrl Pts',(61.2621251782849,-40.3499285956297,12.));
#58312=CARTESIAN_POINT('Ctrl Pts',(61.2880202139358,-40.3547799794672,0.));
#58313=CARTESIAN_POINT('Ctrl Pts',(61.2880202139358,-40.3547799794672,12.));
#58314=CARTESIAN_POINT('Ctrl Pts',(61.3139565024838,-40.3596141830786,0.));
#58315=CARTESIAN_POINT('Ctrl Pts',(61.3139565024838,-40.3596141830786,12.));
#58316=CARTESIAN_POINT('Ctrl Pts',(61.3399339598851,-40.3644311399861,0.));
#58317=CARTESIAN_POINT('Ctrl Pts',(61.3399339598851,-40.3644311399861,12.));
#58318=CARTESIAN_POINT('Ctrl Pts',(61.3659525022917,-40.3692307839642,0.));
#58319=CARTESIAN_POINT('Ctrl Pts',(61.3659525022917,-40.3692307839642,12.));
#58320=CARTESIAN_POINT('Ctrl Pts',(61.3920120460232,-40.3740130490233,0.));
#58321=CARTESIAN_POINT('Ctrl Pts',(61.3920120460232,-40.3740130490233,12.));
#58322=CARTESIAN_POINT('Ctrl Pts',(61.418112507605,-40.3787778694373,0.));
#58323=CARTESIAN_POINT('Ctrl Pts',(61.418112507605,-40.3787778694373,12.));
#58324=CARTESIAN_POINT('Ctrl Pts',(61.4442538038053,-40.3835251797726,0.));
#58325=CARTESIAN_POINT('Ctrl Pts',(61.4442538038053,-40.3835251797726,12.));
#58326=CARTESIAN_POINT('Ctrl Pts',(61.4704358516711,-40.3882549149229,0.));
#58327=CARTESIAN_POINT('Ctrl Pts',(61.4704358516711,-40.3882549149229,12.));
#58328=CARTESIAN_POINT('Ctrl Pts',(61.4966585685544,-40.3929670101363,0.));
#58329=CARTESIAN_POINT('Ctrl Pts',(61.4966585685544,-40.3929670101363,12.));
#58330=CARTESIAN_POINT('Ctrl Pts',(61.5229218721532,-40.3976614010648,0.));
#58331=CARTESIAN_POINT('Ctrl Pts',(61.5229218721532,-40.3976614010648,12.));
#58332=CARTESIAN_POINT('Ctrl Pts',(61.5492256804709,-40.4023380237227,0.));
#58333=CARTESIAN_POINT('Ctrl Pts',(61.5492256804709,-40.4023380237227,12.));
#58334=CARTESIAN_POINT('Ctrl Pts',(61.5755699117318,-40.4069968143953,0.));
#58335=CARTESIAN_POINT('Ctrl Pts',(61.5755699117318,-40.4069968143953,12.));
#58336=CARTESIAN_POINT('Ctrl Pts',(61.6019544843008,-40.4116377095595,0.));
#58337=CARTESIAN_POINT('Ctrl Pts',(61.6019544843008,-40.4116377095595,12.));
#58338=CARTESIAN_POINT('Ctrl Pts',(61.628379316608,-40.4162606458119,0.));
#58339=CARTESIAN_POINT('Ctrl Pts',(61.628379316608,-40.4162606458119,12.));
#58340=CARTESIAN_POINT('Ctrl Pts',(61.6548443270397,-40.420865559772,0.));
#58341=CARTESIAN_POINT('Ctrl Pts',(61.6548443270397,-40.420865559772,12.));
#58342=CARTESIAN_POINT('Ctrl Pts',(61.6813494339295,-40.4254523880766,0.));
#58343=CARTESIAN_POINT('Ctrl Pts',(61.6813494339295,-40.4254523880766,12.));
#58344=CARTESIAN_POINT('Ctrl Pts',(61.7078945557812,-40.4300210675848,0.));
#58345=CARTESIAN_POINT('Ctrl Pts',(61.7078945557812,-40.4300210675848,12.));
#58346=CARTESIAN_POINT('Ctrl Pts',(61.7344796114409,-40.4345715355411,0.));
#58347=CARTESIAN_POINT('Ctrl Pts',(61.7344796114409,-40.4345715355411,12.));
#58348=CARTESIAN_POINT('Ctrl Pts',(61.7611045202875,-40.439103729759,0.));
#58349=CARTESIAN_POINT('Ctrl Pts',(61.7611045202875,-40.439103729759,12.));
#58350=CARTESIAN_POINT('Ctrl Pts',(61.7877692024064,-40.4436175887943,0.));
#58351=CARTESIAN_POINT('Ctrl Pts',(61.7877692024064,-40.4436175887943,12.));
#58352=CARTESIAN_POINT('Ctrl Pts',(61.8144735787767,-40.448113052135,0.));
#58353=CARTESIAN_POINT('Ctrl Pts',(61.8144735787767,-40.448113052135,12.));
#58354=CARTESIAN_POINT('Ctrl Pts',(61.8412175708523,-40.4525900597877,0.));
#58355=CARTESIAN_POINT('Ctrl Pts',(61.8412175708523,-40.4525900597877,12.));
#58356=CARTESIAN_POINT('Ctrl Pts',(61.8680011001513,-40.4570485518735,0.));
#58357=CARTESIAN_POINT('Ctrl Pts',(61.8680011001513,-40.4570485518735,12.));
#58358=CARTESIAN_POINT('Ctrl Pts',(61.8948240877998,-40.4614884681884,0.));
#58359=CARTESIAN_POINT('Ctrl Pts',(61.8948240877998,-40.4614884681884,12.));
#58360=CARTESIAN_POINT('Ctrl Pts',(61.9216864541758,-40.4659097478595,0.));
#58361=CARTESIAN_POINT('Ctrl Pts',(61.9216864541758,-40.4659097478595,12.));
#58362=CARTESIAN_POINT('Ctrl Pts',(61.9485881182957,-40.4703123287642,0.));
#58363=CARTESIAN_POINT('Ctrl Pts',(61.9485881182957,-40.4703123287642,12.));
#58364=CARTESIAN_POINT('Ctrl Pts',(61.9755289983093,-40.4746961480045,0.));
#58365=CARTESIAN_POINT('Ctrl Pts',(61.9755289983093,-40.4746961480045,12.));
#58366=CARTESIAN_POINT('Ctrl Pts',(62.0025090126008,-40.4790611429613,0.));
#58367=CARTESIAN_POINT('Ctrl Pts',(62.0025090126008,-40.4790611429613,12.));
#58368=CARTESIAN_POINT('Ctrl Pts',(62.0295280807449,-40.4834072522182,0.));
#58369=CARTESIAN_POINT('Ctrl Pts',(62.0295280807449,-40.4834072522182,12.));
#58370=CARTESIAN_POINT('Ctrl Pts',(62.0565861244171,-40.4877344164407,0.));
#58371=CARTESIAN_POINT('Ctrl Pts',(62.0565861244171,-40.4877344164407,12.));
#58372=CARTESIAN_POINT('Ctrl Pts',(62.0836830685665,-40.4920425795184,0.));
#58373=CARTESIAN_POINT('Ctrl Pts',(62.0836830685665,-40.4920425795184,12.));
#58374=CARTESIAN_POINT('Ctrl Pts',(62.110818841691,-40.4963316888357,0.));
#58375=CARTESIAN_POINT('Ctrl Pts',(62.110818841691,-40.4963316888357,12.));
#58376=CARTESIAN_POINT('Ctrl Pts',(62.137993373242,-40.500601692749,0.));
#58377=CARTESIAN_POINT('Ctrl Pts',(62.137993373242,-40.500601692749,12.));
#58378=CARTESIAN_POINT('Ctrl Pts',(62.1652065915724,-40.5048525385985,0.));
#58379=CARTESIAN_POINT('Ctrl Pts',(62.1652065915724,-40.5048525385985,12.));
#58380=CARTESIAN_POINT('Ctrl Pts',(62.1924584215634,-40.5090841704111,0.));
#58381=CARTESIAN_POINT('Ctrl Pts',(62.1924584215634,-40.5090841704111,12.));
#58382=CARTESIAN_POINT('Ctrl Pts',(62.2197487826212,-40.5132965269679,0.));
#58383=CARTESIAN_POINT('Ctrl Pts',(62.2197487826212,-40.5132965269679,12.));
#58384=CARTESIAN_POINT('Ctrl Pts',(62.2470775858834,-40.5174895391059,0.));
#58385=CARTESIAN_POINT('Ctrl Pts',(62.2470775858834,-40.5174895391059,12.));
#58386=CARTESIAN_POINT('Ctrl Pts',(62.2744447382207,-40.5216631336335,0.));
#58387=CARTESIAN_POINT('Ctrl Pts',(62.2744447382207,-40.5216631336335,12.));
#58388=CARTESIAN_POINT('Ctrl Pts',(62.3018501471876,-40.5258172381565,0.));
#58389=CARTESIAN_POINT('Ctrl Pts',(62.3018501471876,-40.5258172381565,12.));
#58390=CARTESIAN_POINT('Ctrl Pts',(62.3292937258021,-40.5299517857793,0.));
#58391=CARTESIAN_POINT('Ctrl Pts',(62.3292937258021,-40.5299517857793,12.));
#58392=CARTESIAN_POINT('Ctrl Pts',(62.35677539702,-40.5340667194272,0.));
#58393=CARTESIAN_POINT('Ctrl Pts',(62.35677539702,-40.5340667194272,12.));
#58394=CARTESIAN_POINT('Ctrl Pts',(62.3842950992504,-40.5381619973972,0.));
#58395=CARTESIAN_POINT('Ctrl Pts',(62.3842950992504,-40.5381619973972,12.));
#58396=CARTESIAN_POINT('Ctrl Pts',(62.4118527880601,-40.5422375944697,0.));
#58397=CARTESIAN_POINT('Ctrl Pts',(62.4118527880601,-40.5422375944697,12.));
#58398=CARTESIAN_POINT('Ctrl Pts',(62.439448432904,-40.5462934972335,0.));
#58399=CARTESIAN_POINT('Ctrl Pts',(62.439448432904,-40.5462934972335,12.));
#58400=CARTESIAN_POINT('Ctrl Pts',(62.4615552986669,-40.5495224601437,0.));
#58401=CARTESIAN_POINT('Ctrl Pts',(62.4615552986669,-40.5495224601437,12.));
#58402=CARTESIAN_POINT('Ctrl Pts',(62.4781525155997,-40.5519353177058,0.));
#58403=CARTESIAN_POINT('Ctrl Pts',(62.4781525155997,-40.5519353177058,12.));
#58404=CARTESIAN_POINT('Ctrl Pts',(62.4892249121863,-40.5535399497449,0.));
#58405=CARTESIAN_POINT('Ctrl Pts',(62.4892249121863,-40.5535399497449,12.));
#58406=CARTESIAN_POINT('Ctrl Pts',(62.4947630068039,-40.554341280847,0.));
#58407=CARTESIAN_POINT('Ctrl Pts',(62.4947630068039,-40.554341280847,12.));
#58408=CARTESIAN_POINT('',(57.8261117662438,-39.4479504917287,0.));
#58409=CARTESIAN_POINT('Ctrl Pts',(57.8261117662438,-39.4479504917287,0.));
#58410=CARTESIAN_POINT('Ctrl Pts',(57.8297740100947,-39.4492429618443,0.));
#58411=CARTESIAN_POINT('Ctrl Pts',(57.837104315141,-39.4518277003553,0.));
#58412=CARTESIAN_POINT('Ctrl Pts',(57.8481172247495,-39.4557042029652,0.));
#58413=CARTESIAN_POINT('Ctrl Pts',(57.8628360096803,-39.4608716627118,0.));
#58414=CARTESIAN_POINT('Ctrl Pts',(57.8812926637177,-39.4673289592259,0.));
#58415=CARTESIAN_POINT('Ctrl Pts',(57.8998074670478,-39.473784194937,0.));
#58416=CARTESIAN_POINT('Ctrl Pts',(57.9183803632403,-39.4802373061058,0.));
#58417=CARTESIAN_POINT('Ctrl Pts',(57.937011245663,-39.4866881842317,0.));
#58418=CARTESIAN_POINT('Ctrl Pts',(57.9556999583892,-39.4931366776714,0.));
#58419=CARTESIAN_POINT('Ctrl Pts',(57.974446317937,-39.499582610674,0.));
#58420=CARTESIAN_POINT('Ctrl Pts',(57.9932501298522,-39.5060257981225,0.));
#58421=CARTESIAN_POINT('Ctrl Pts',(58.0121112067895,-39.5124660614976,0.));
#58422=CARTESIAN_POINT('Ctrl Pts',(58.0310293875262,-39.5189032457184,0.));
#58423=CARTESIAN_POINT('Ctrl Pts',(58.0500045308412,-39.5253372136887,0.));
#58424=CARTESIAN_POINT('Ctrl Pts',(58.0690365065374,-39.5317678383217,0.));
#58425=CARTESIAN_POINT('Ctrl Pts',(58.088125187992,-39.5381949959221,0.));
#58426=CARTESIAN_POINT('Ctrl Pts',(58.1072704428928,-39.5446185579638,0.));
#58427=CARTESIAN_POINT('Ctrl Pts',(58.126472128574,-39.5510383869505,0.));
#58428=CARTESIAN_POINT('Ctrl Pts',(58.1457300968499,-39.5574543406982,0.));
#58429=CARTESIAN_POINT('Ctrl Pts',(58.1650441970387,-39.563866275018,0.));
#58430=CARTESIAN_POINT('Ctrl Pts',(58.1844142794338,-39.5702740467999,0.));
#58431=CARTESIAN_POINT('Ctrl Pts',(58.2038401992457,-39.57667751752,0.));
#58432=CARTESIAN_POINT('Ctrl Pts',(58.2233218164365,-39.5830765530891,0.));
#58433=CARTESIAN_POINT('Ctrl Pts',(58.2428589938369,-39.5894710221713,0.));
#58434=CARTESIAN_POINT('Ctrl Pts',(58.2624515958419,-39.5958607950239,0.));
#58435=CARTESIAN_POINT('Ctrl Pts',(58.2820994868118,-39.602245742079,0.));
#58436=CARTESIAN_POINT('Ctrl Pts',(58.3018025297323,-39.6086257327583,0.));
#58437=CARTESIAN_POINT('Ctrl Pts',(58.3215605869221,-39.6150006360915,0.));
#58438=CARTESIAN_POINT('Ctrl Pts',(58.3413735206423,-39.6213703212531,0.));
#58439=CARTESIAN_POINT('Ctrl Pts',(58.3612411936904,-39.6277346580892,0.));
#58440=CARTESIAN_POINT('Ctrl Pts',(58.3811634701037,-39.6340935177476,0.));
#58441=CARTESIAN_POINT('Ctrl Pts',(58.4011402154196,-39.6404467729094,0.));
#58442=CARTESIAN_POINT('Ctrl Pts',(58.4211712963004,-39.6467942974451,0.));
#58443=CARTESIAN_POINT('Ctrl Pts',(58.4412565802979,-39.653135966204,0.));
#58444=CARTESIAN_POINT('Ctrl Pts',(58.4613959355788,-39.6594716547689,0.));
#58445=CARTESIAN_POINT('Ctrl Pts',(58.4815892306066,-39.6658012391815,0.));
#58446=CARTESIAN_POINT('Ctrl Pts',(58.5018363341604,-39.6721245959531,0.));
#58447=CARTESIAN_POINT('Ctrl Pts',(58.5221371154761,-39.6784416021826,0.));
#58448=CARTESIAN_POINT('Ctrl Pts',(58.5424914443415,-39.6847521356395,0.));
#58449=CARTESIAN_POINT('Ctrl Pts',(58.5628991912052,-39.6910560748629,0.));
#58450=CARTESIAN_POINT('Ctrl Pts',(58.5833602272743,-39.697353299254,0.));
#58451=CARTESIAN_POINT('Ctrl Pts',(58.6038744244659,-39.7036436890233,0.));
#58452=CARTESIAN_POINT('Ctrl Pts',(58.6244416553562,-39.7099271251413,0.));
#58453=CARTESIAN_POINT('Ctrl Pts',(58.6450617931274,-39.71620348929,0.));
#58454=CARTESIAN_POINT('Ctrl Pts',(58.6657347115034,-39.7224726638101,0.));
#58455=CARTESIAN_POINT('Ctrl Pts',(58.6864602847088,-39.7287345316681,0.));
#58456=CARTESIAN_POINT('Ctrl Pts',(58.7072383875027,-39.734988976475,0.));
#58457=CARTESIAN_POINT('Ctrl Pts',(58.7280688951916,-39.7412358824953,0.));
#58458=CARTESIAN_POINT('Ctrl Pts',(58.7489516836445,-39.7474751346599,0.));
#58459=CARTESIAN_POINT('Ctrl Pts',(58.7698866293029,-39.7537066185813,0.));
#58460=CARTESIAN_POINT('Ctrl Pts',(58.7908736091798,-39.7599302205521,0.));
#58461=CARTESIAN_POINT('Ctrl Pts',(58.8119125008517,-39.7661458275274,0.));
#58462=CARTESIAN_POINT('Ctrl Pts',(58.8330031824453,-39.772353327112,0.));
#58463=CARTESIAN_POINT('Ctrl Pts',(58.8541455326231,-39.7785526075479,0.));
#58464=CARTESIAN_POINT('Ctrl Pts',(58.8753394305585,-39.7847435576997,0.));
#58465=CARTESIAN_POINT('Ctrl Pts',(58.8965847559391,-39.7909260670517,0.));
#58466=CARTESIAN_POINT('Ctrl Pts',(58.9178813889703,-39.7971000257044,0.));
#58467=CARTESIAN_POINT('Ctrl Pts',(58.9392292103747,-39.8032653243712,0.));
#58468=CARTESIAN_POINT('Ctrl Pts',(58.9606281013875,-39.8094218543782,0.));
#58469=CARTESIAN_POINT('Ctrl Pts',(58.9820779437484,-39.8155695076626,0.));
#58470=CARTESIAN_POINT('Ctrl Pts',(59.0035786197024,-39.821708176766,0.));
#58471=CARTESIAN_POINT('Ctrl Pts',(59.0251300119973,-39.8278377548262,0.));
#58472=CARTESIAN_POINT('Ctrl Pts',(59.0467320038784,-39.8339581355716,0.));
#58473=CARTESIAN_POINT('Ctrl Pts',(59.0683844790764,-39.8400692133139,0.));
#58474=CARTESIAN_POINT('Ctrl Pts',(59.090087321798,-39.8461708829456,0.));
#58475=CARTESIAN_POINT('Ctrl Pts',(59.1118404167292,-39.8522630399328,0.));
#58476=CARTESIAN_POINT('Ctrl Pts',(59.1336436490342,-39.8583455803105,0.));
#58477=CARTESIAN_POINT('Ctrl Pts',(59.1554969043522,-39.8644184006787,0.));
#58478=CARTESIAN_POINT('Ctrl Pts',(59.1774000687879,-39.8704813981989,0.));
#58479=CARTESIAN_POINT('Ctrl Pts',(59.1993530289028,-39.876534470591,0.));
#58480=CARTESIAN_POINT('Ctrl Pts',(59.2213556717209,-39.8825775161267,0.));
#58481=CARTESIAN_POINT('Ctrl Pts',(59.2434078847247,-39.8886104336242,0.));
#58482=CARTESIAN_POINT('Ctrl Pts',(59.2655095558521,-39.8946331224438,0.));
#58483=CARTESIAN_POINT('Ctrl Pts',(59.2876605734846,-39.9006454824845,0.));
#58484=CARTESIAN_POINT('Ctrl Pts',(59.3098608264419,-39.9066474141803,0.));
#58485=CARTESIAN_POINT('Ctrl Pts',(59.3321102039852,-39.9126388184936,0.));
#58486=CARTESIAN_POINT('Ctrl Pts',(59.3544085958151,-39.9186195969104,0.));
#58487=CARTESIAN_POINT('Ctrl Pts',(59.3767558920675,-39.9245896514367,0.));
#58488=CARTESIAN_POINT('Ctrl Pts',(59.3991519833016,-39.9305488845958,0.));
#58489=CARTESIAN_POINT('Ctrl Pts',(59.4215967604967,-39.9364971994242,0.));
#58490=CARTESIAN_POINT('Ctrl Pts',(59.4440901150582,-39.9424344994673,0.));
#58491=CARTESIAN_POINT('Ctrl Pts',(59.4666319388133,-39.9483606887738,0.));
#58492=CARTESIAN_POINT('Ctrl Pts',(59.4892221240068,-39.9542756718922,0.));
#58493=CARTESIAN_POINT('Ctrl Pts',(59.511860563289,-39.9601793538683,0.));
#58494=CARTESIAN_POINT('Ctrl Pts',(59.5345471497128,-39.9660716402403,0.));
#58495=CARTESIAN_POINT('Ctrl Pts',(59.5572817767388,-39.9719524370346,0.));
#58496=CARTESIAN_POINT('Ctrl Pts',(59.5800643382314,-39.9778216507605,0.));
#58497=CARTESIAN_POINT('Ctrl Pts',(59.6028947284562,-39.9836791884079,0.));
#58498=CARTESIAN_POINT('Ctrl Pts',(59.6257728420669,-39.9895249574448,0.));
#58499=CARTESIAN_POINT('Ctrl Pts',(59.6486985741041,-39.9953588658132,0.));
#58500=CARTESIAN_POINT('Ctrl Pts',(59.6716718200005,-40.0011808219241,0.));
#58501=CARTESIAN_POINT('Ctrl Pts',(59.6946924755773,-40.0069907346538,0.));
#58502=CARTESIAN_POINT('Ctrl Pts',(59.7177604370403,-40.0127885133403,0.));
#58503=CARTESIAN_POINT('Ctrl Pts',(59.7408756009679,-40.0185740677821,0.));
#58504=CARTESIAN_POINT('Ctrl Pts',(59.7640378643106,-40.0243473082337,0.));
#58505=CARTESIAN_POINT('Ctrl Pts',(59.7872471243942,-40.0301081454002,0.));
#58506=CARTESIAN_POINT('Ctrl Pts',(59.8105032789179,-40.0358564904341,0.));
#58507=CARTESIAN_POINT('Ctrl Pts',(59.8338062259492,-40.0415922549315,0.));
#58508=CARTESIAN_POINT('Ctrl Pts',(59.8571558639145,-40.0473153509324,0.));
#58509=CARTESIAN_POINT('Ctrl Pts',(59.8805520915972,-40.0530256909161,0.));
#58510=CARTESIAN_POINT('Ctrl Pts',(59.9039948081428,-40.0587231877959,0.));
#58511=CARTESIAN_POINT('Ctrl Pts',(59.927483913055,-40.0644077549158,0.));
#58512=CARTESIAN_POINT('Ctrl Pts',(59.9510193061929,-40.0700793060475,0.));
#58513=CARTESIAN_POINT('Ctrl Pts',(59.974600887759,-40.0757377553894,0.));
#58514=CARTESIAN_POINT('Ctrl Pts',(59.9982285582991,-40.0813830175629,0.));
#58515=CARTESIAN_POINT('Ctrl Pts',(60.0219022187066,-40.0870150076078,0.));
#58516=CARTESIAN_POINT('Ctrl Pts',(60.0456217702203,-40.0926336409787,0.));
#58517=CARTESIAN_POINT('Ctrl Pts',(60.0693871144207,-40.0982388335421,0.));
#58518=CARTESIAN_POINT('Ctrl Pts',(60.0931981532194,-40.1038305015764,0.));
#58519=CARTESIAN_POINT('Ctrl Pts',(60.1170547888572,-40.1094085617672,0.));
#58520=CARTESIAN_POINT('Ctrl Pts',(60.1409569239092,-40.1149729312036,0.));
#58521=CARTESIAN_POINT('Ctrl Pts',(60.1649044612829,-40.120523527374,0.));
#58522=CARTESIAN_POINT('Ctrl Pts',(60.1888973042151,-40.1260602681644,0.));
#58523=CARTESIAN_POINT('Ctrl Pts',(60.2129353562617,-40.1315830718575,0.));
#58524=CARTESIAN_POINT('Ctrl Pts',(60.2370185212957,-40.13709185713,0.));
#58525=CARTESIAN_POINT('Ctrl Pts',(60.2611467035109,-40.1425865430468,0.));
#58526=CARTESIAN_POINT('Ctrl Pts',(60.2853198074215,-40.1480670490583,0.));
#58527=CARTESIAN_POINT('Ctrl Pts',(60.3095377378589,-40.1535332949978,0.));
#58528=CARTESIAN_POINT('Ctrl Pts',(60.3338003999616,-40.1589852010811,0.));
#58529=CARTESIAN_POINT('Ctrl Pts',(60.3581076991731,-40.1644226879043,0.));
#58530=CARTESIAN_POINT('Ctrl Pts',(60.382459541246,-40.1698456764387,0.));
#58531=CARTESIAN_POINT('Ctrl Pts',(60.4068558322414,-40.1752540880273,0.));
#58532=CARTESIAN_POINT('Ctrl Pts',(60.4312964785269,-40.1806478443829,0.));
#58533=CARTESIAN_POINT('Ctrl Pts',(60.4557813867677,-40.1860268675876,0.));
#58534=CARTESIAN_POINT('Ctrl Pts',(60.4803104639211,-40.1913910800912,0.));
#58535=CARTESIAN_POINT('Ctrl Pts',(60.5048836172423,-40.1967404047055,0.));
#58536=CARTESIAN_POINT('Ctrl Pts',(60.5295007542838,-40.2020747646012,0.));
#58537=CARTESIAN_POINT('Ctrl Pts',(60.5541617828927,-40.2073940833054,0.));
#58538=CARTESIAN_POINT('Ctrl Pts',(60.5788666112043,-40.2126982847012,0.));
#58539=CARTESIAN_POINT('Ctrl Pts',(60.6036151476347,-40.2179872930272,0.));
#58540=CARTESIAN_POINT('Ctrl Pts',(60.6284073008865,-40.2232610328717,0.));
#58541=CARTESIAN_POINT('Ctrl Pts',(60.6532429799493,-40.2285194291702,0.));
#58542=CARTESIAN_POINT('Ctrl Pts',(60.6781220940979,-40.2337624072029,0.));
#58543=CARTESIAN_POINT('Ctrl Pts',(60.7030445528863,-40.2389898925937,0.));
#58544=CARTESIAN_POINT('Ctrl Pts',(60.72801026614,-40.2442018113116,0.));
#58545=CARTESIAN_POINT('Ctrl Pts',(60.7530191439603,-40.2493980896646,0.));
#58546=CARTESIAN_POINT('Ctrl Pts',(60.7780710967253,-40.2545786542957,0.));
#58547=CARTESIAN_POINT('Ctrl Pts',(60.8031660350878,-40.2597434321804,0.));
#58548=CARTESIAN_POINT('Ctrl Pts',(60.8283038699703,-40.2648923506245,0.));
#58549=CARTESIAN_POINT('Ctrl Pts',(60.8534845125535,-40.2700253372644,0.));
#58550=CARTESIAN_POINT('Ctrl Pts',(60.8787078742817,-40.2751423200637,0.));
#58551=CARTESIAN_POINT('Ctrl Pts',(60.903973866867,-40.2802432273105,0.));
#58552=CARTESIAN_POINT('Ctrl Pts',(60.9292824022888,-40.2853279876162,0.));
#58553=CARTESIAN_POINT('Ctrl Pts',(60.9546333927919,-40.2903965299155,0.));
#58554=CARTESIAN_POINT('Ctrl Pts',(60.9800267508781,-40.2954487834688,0.));
#58555=CARTESIAN_POINT('Ctrl Pts',(61.0054623893059,-40.3004846778577,0.));
#58556=CARTESIAN_POINT('Ctrl Pts',(61.0309402210915,-40.3055041429772,0.));
#58557=CARTESIAN_POINT('Ctrl Pts',(61.0564601595047,-40.3105071090308,0.));
#58558=CARTESIAN_POINT('Ctrl Pts',(61.0820221180646,-40.3154935065264,0.));
#58559=CARTESIAN_POINT('Ctrl Pts',(61.1076260105265,-40.3204632662729,0.));
#58560=CARTESIAN_POINT('Ctrl Pts',(61.1332717508799,-40.3254163193806,0.));
#58561=CARTESIAN_POINT('Ctrl Pts',(61.1589592533623,-40.3303525972621,0.));
#58562=CARTESIAN_POINT('Ctrl Pts',(61.184688432465,-40.3352720316373,0.));
#58563=CARTESIAN_POINT('Ctrl Pts',(61.2104592029375,-40.3401745545369,0.));
#58564=CARTESIAN_POINT('Ctrl Pts',(61.236271479789,-40.3450600983104,0.));
#58565=CARTESIAN_POINT('Ctrl Pts',(61.2621251782849,-40.3499285956297,0.));
#58566=CARTESIAN_POINT('Ctrl Pts',(61.2880202139358,-40.3547799794672,0.));
#58567=CARTESIAN_POINT('Ctrl Pts',(61.3139565024838,-40.3596141830786,0.));
#58568=CARTESIAN_POINT('Ctrl Pts',(61.3399339598851,-40.3644311399861,0.));
#58569=CARTESIAN_POINT('Ctrl Pts',(61.3659525022917,-40.3692307839642,0.));
#58570=CARTESIAN_POINT('Ctrl Pts',(61.3920120460232,-40.3740130490233,0.));
#58571=CARTESIAN_POINT('Ctrl Pts',(61.418112507605,-40.3787778694373,0.));
#58572=CARTESIAN_POINT('Ctrl Pts',(61.4442538038053,-40.3835251797726,0.));
#58573=CARTESIAN_POINT('Ctrl Pts',(61.4704358516711,-40.3882549149229,0.));
#58574=CARTESIAN_POINT('Ctrl Pts',(61.4966585685544,-40.3929670101363,0.));
#58575=CARTESIAN_POINT('Ctrl Pts',(61.5229218721532,-40.3976614010648,0.));
#58576=CARTESIAN_POINT('Ctrl Pts',(61.5492256804709,-40.4023380237227,0.));
#58577=CARTESIAN_POINT('Ctrl Pts',(61.5755699117318,-40.4069968143953,0.));
#58578=CARTESIAN_POINT('Ctrl Pts',(61.6019544843008,-40.4116377095595,0.));
#58579=CARTESIAN_POINT('Ctrl Pts',(61.628379316608,-40.4162606458119,0.));
#58580=CARTESIAN_POINT('Ctrl Pts',(61.6548443270397,-40.420865559772,0.));
#58581=CARTESIAN_POINT('Ctrl Pts',(61.6813494339295,-40.4254523880766,0.));
#58582=CARTESIAN_POINT('Ctrl Pts',(61.7078945557812,-40.4300210675848,0.));
#58583=CARTESIAN_POINT('Ctrl Pts',(61.7344796114409,-40.4345715355411,0.));
#58584=CARTESIAN_POINT('Ctrl Pts',(61.7611045202875,-40.439103729759,0.));
#58585=CARTESIAN_POINT('Ctrl Pts',(61.7877692024064,-40.4436175887943,0.));
#58586=CARTESIAN_POINT('Ctrl Pts',(61.8144735787767,-40.448113052135,0.));
#58587=CARTESIAN_POINT('Ctrl Pts',(61.8412175708523,-40.4525900597877,0.));
#58588=CARTESIAN_POINT('Ctrl Pts',(61.8680011001513,-40.4570485518735,0.));
#58589=CARTESIAN_POINT('Ctrl Pts',(61.8948240877998,-40.4614884681884,0.));
#58590=CARTESIAN_POINT('Ctrl Pts',(61.9216864541758,-40.4659097478595,0.));
#58591=CARTESIAN_POINT('Ctrl Pts',(61.9485881182957,-40.4703123287642,0.));
#58592=CARTESIAN_POINT('Ctrl Pts',(61.9755289983093,-40.4746961480045,0.));
#58593=CARTESIAN_POINT('Ctrl Pts',(62.0025090126008,-40.4790611429613,0.));
#58594=CARTESIAN_POINT('Ctrl Pts',(62.0295280807449,-40.4834072522182,0.));
#58595=CARTESIAN_POINT('Ctrl Pts',(62.0565861244171,-40.4877344164407,0.));
#58596=CARTESIAN_POINT('Ctrl Pts',(62.0836830685665,-40.4920425795184,0.));
#58597=CARTESIAN_POINT('Ctrl Pts',(62.110818841691,-40.4963316888357,0.));
#58598=CARTESIAN_POINT('Ctrl Pts',(62.1341126810363,-40.499991909619,0.));
#58599=CARTESIAN_POINT('Ctrl Pts',(62.1519925002735,-40.5027877865723,0.));
#58600=CARTESIAN_POINT('Ctrl Pts',(62.1644411502527,-40.5047277935687,0.));
#58601=CARTESIAN_POINT('Ctrl Pts',(62.1714473137748,-40.5058175523045,0.));
#58602=CARTESIAN_POINT('Ctrl Pts',(62.1730054756448,-40.5060598100837,0.));
#58603=CARTESIAN_POINT('',(57.8261117662438,-39.4479504917287,12.));
#58604=CARTESIAN_POINT('',(57.8261117662438,-39.4479504917287,0.));
#58605=CARTESIAN_POINT('Ctrl Pts',(62.1730054756448,-40.5060598100837,12.));
#58606=CARTESIAN_POINT('Ctrl Pts',(62.1714473137748,-40.5058175523045,12.));
#58607=CARTESIAN_POINT('Ctrl Pts',(62.1644411502527,-40.5047277935687,12.));
#58608=CARTESIAN_POINT('Ctrl Pts',(62.1519925002735,-40.5027877865723,12.));
#58609=CARTESIAN_POINT('Ctrl Pts',(62.1341126810363,-40.499991909619,12.));
#58610=CARTESIAN_POINT('Ctrl Pts',(62.110818841691,-40.4963316888357,12.));
#58611=CARTESIAN_POINT('Ctrl Pts',(62.0836830685665,-40.4920425795184,12.));
#58612=CARTESIAN_POINT('Ctrl Pts',(62.0565861244171,-40.4877344164407,12.));
#58613=CARTESIAN_POINT('Ctrl Pts',(62.0295280807449,-40.4834072522182,12.));
#58614=CARTESIAN_POINT('Ctrl Pts',(62.0025090126008,-40.4790611429613,12.));
#58615=CARTESIAN_POINT('Ctrl Pts',(61.9755289983093,-40.4746961480045,12.));
#58616=CARTESIAN_POINT('Ctrl Pts',(61.9485881182957,-40.4703123287642,12.));
#58617=CARTESIAN_POINT('Ctrl Pts',(61.9216864541758,-40.4659097478595,12.));
#58618=CARTESIAN_POINT('Ctrl Pts',(61.8948240877998,-40.4614884681884,12.));
#58619=CARTESIAN_POINT('Ctrl Pts',(61.8680011001513,-40.4570485518735,12.));
#58620=CARTESIAN_POINT('Ctrl Pts',(61.8412175708523,-40.4525900597877,12.));
#58621=CARTESIAN_POINT('Ctrl Pts',(61.8144735787767,-40.448113052135,12.));
#58622=CARTESIAN_POINT('Ctrl Pts',(61.7877692024064,-40.4436175887943,12.));
#58623=CARTESIAN_POINT('Ctrl Pts',(61.7611045202875,-40.439103729759,12.));
#58624=CARTESIAN_POINT('Ctrl Pts',(61.7344796114409,-40.4345715355411,12.));
#58625=CARTESIAN_POINT('Ctrl Pts',(61.7078945557812,-40.4300210675848,12.));
#58626=CARTESIAN_POINT('Ctrl Pts',(61.6813494339295,-40.4254523880766,12.));
#58627=CARTESIAN_POINT('Ctrl Pts',(61.6548443270397,-40.420865559772,12.));
#58628=CARTESIAN_POINT('Ctrl Pts',(61.628379316608,-40.4162606458119,12.));
#58629=CARTESIAN_POINT('Ctrl Pts',(61.6019544843008,-40.4116377095595,12.));
#58630=CARTESIAN_POINT('Ctrl Pts',(61.5755699117318,-40.4069968143953,12.));
#58631=CARTESIAN_POINT('Ctrl Pts',(61.5492256804709,-40.4023380237227,12.));
#58632=CARTESIAN_POINT('Ctrl Pts',(61.5229218721532,-40.3976614010648,12.));
#58633=CARTESIAN_POINT('Ctrl Pts',(61.4966585685544,-40.3929670101363,12.));
#58634=CARTESIAN_POINT('Ctrl Pts',(61.4704358516711,-40.3882549149229,12.));
#58635=CARTESIAN_POINT('Ctrl Pts',(61.4442538038053,-40.3835251797726,12.));
#58636=CARTESIAN_POINT('Ctrl Pts',(61.418112507605,-40.3787778694373,12.));
#58637=CARTESIAN_POINT('Ctrl Pts',(61.3920120460232,-40.3740130490233,12.));
#58638=CARTESIAN_POINT('Ctrl Pts',(61.3659525022917,-40.3692307839642,12.));
#58639=CARTESIAN_POINT('Ctrl Pts',(61.3399339598851,-40.3644311399861,12.));
#58640=CARTESIAN_POINT('Ctrl Pts',(61.3139565024838,-40.3596141830786,12.));
#58641=CARTESIAN_POINT('Ctrl Pts',(61.2880202139358,-40.3547799794672,12.));
#58642=CARTESIAN_POINT('Ctrl Pts',(61.2621251782849,-40.3499285956297,12.));
#58643=CARTESIAN_POINT('Ctrl Pts',(61.236271479789,-40.3450600983104,12.));
#58644=CARTESIAN_POINT('Ctrl Pts',(61.2104592029375,-40.3401745545369,12.));
#58645=CARTESIAN_POINT('Ctrl Pts',(61.184688432465,-40.3352720316373,12.));
#58646=CARTESIAN_POINT('Ctrl Pts',(61.1589592533623,-40.3303525972621,12.));
#58647=CARTESIAN_POINT('Ctrl Pts',(61.1332717508799,-40.3254163193806,12.));
#58648=CARTESIAN_POINT('Ctrl Pts',(61.1076260105265,-40.3204632662729,12.));
#58649=CARTESIAN_POINT('Ctrl Pts',(61.0820221180646,-40.3154935065264,12.));
#58650=CARTESIAN_POINT('Ctrl Pts',(61.0564601595047,-40.3105071090308,12.));
#58651=CARTESIAN_POINT('Ctrl Pts',(61.0309402210915,-40.3055041429772,12.));
#58652=CARTESIAN_POINT('Ctrl Pts',(61.0054623893059,-40.3004846778577,12.));
#58653=CARTESIAN_POINT('Ctrl Pts',(60.9800267508781,-40.2954487834688,12.));
#58654=CARTESIAN_POINT('Ctrl Pts',(60.9546333927919,-40.2903965299155,12.));
#58655=CARTESIAN_POINT('Ctrl Pts',(60.9292824022888,-40.2853279876162,12.));
#58656=CARTESIAN_POINT('Ctrl Pts',(60.903973866867,-40.2802432273105,12.));
#58657=CARTESIAN_POINT('Ctrl Pts',(60.8787078742817,-40.2751423200637,12.));
#58658=CARTESIAN_POINT('Ctrl Pts',(60.8534845125535,-40.2700253372644,12.));
#58659=CARTESIAN_POINT('Ctrl Pts',(60.8283038699703,-40.2648923506245,12.));
#58660=CARTESIAN_POINT('Ctrl Pts',(60.8031660350878,-40.2597434321804,12.));
#58661=CARTESIAN_POINT('Ctrl Pts',(60.7780710967253,-40.2545786542957,12.));
#58662=CARTESIAN_POINT('Ctrl Pts',(60.7530191439603,-40.2493980896646,12.));
#58663=CARTESIAN_POINT('Ctrl Pts',(60.72801026614,-40.2442018113116,12.));
#58664=CARTESIAN_POINT('Ctrl Pts',(60.7030445528863,-40.2389898925937,12.));
#58665=CARTESIAN_POINT('Ctrl Pts',(60.6781220940979,-40.2337624072029,12.));
#58666=CARTESIAN_POINT('Ctrl Pts',(60.6532429799493,-40.2285194291702,12.));
#58667=CARTESIAN_POINT('Ctrl Pts',(60.6284073008865,-40.2232610328717,12.));
#58668=CARTESIAN_POINT('Ctrl Pts',(60.6036151476347,-40.2179872930272,12.));
#58669=CARTESIAN_POINT('Ctrl Pts',(60.5788666112043,-40.2126982847012,12.));
#58670=CARTESIAN_POINT('Ctrl Pts',(60.5541617828927,-40.2073940833054,12.));
#58671=CARTESIAN_POINT('Ctrl Pts',(60.5295007542838,-40.2020747646012,12.));
#58672=CARTESIAN_POINT('Ctrl Pts',(60.5048836172423,-40.1967404047055,12.));
#58673=CARTESIAN_POINT('Ctrl Pts',(60.4803104639211,-40.1913910800912,12.));
#58674=CARTESIAN_POINT('Ctrl Pts',(60.4557813867677,-40.1860268675876,12.));
#58675=CARTESIAN_POINT('Ctrl Pts',(60.4312964785269,-40.1806478443829,12.));
#58676=CARTESIAN_POINT('Ctrl Pts',(60.4068558322414,-40.1752540880273,12.));
#58677=CARTESIAN_POINT('Ctrl Pts',(60.382459541246,-40.1698456764387,12.));
#58678=CARTESIAN_POINT('Ctrl Pts',(60.3581076991731,-40.1644226879043,12.));
#58679=CARTESIAN_POINT('Ctrl Pts',(60.3338003999616,-40.1589852010811,12.));
#58680=CARTESIAN_POINT('Ctrl Pts',(60.3095377378589,-40.1535332949978,12.));
#58681=CARTESIAN_POINT('Ctrl Pts',(60.2853198074215,-40.1480670490583,12.));
#58682=CARTESIAN_POINT('Ctrl Pts',(60.2611467035109,-40.1425865430468,12.));
#58683=CARTESIAN_POINT('Ctrl Pts',(60.2370185212957,-40.13709185713,12.));
#58684=CARTESIAN_POINT('Ctrl Pts',(60.2129353562617,-40.1315830718575,12.));
#58685=CARTESIAN_POINT('Ctrl Pts',(60.1888973042151,-40.1260602681644,12.));
#58686=CARTESIAN_POINT('Ctrl Pts',(60.1649044612829,-40.120523527374,12.));
#58687=CARTESIAN_POINT('Ctrl Pts',(60.1409569239092,-40.1149729312036,12.));
#58688=CARTESIAN_POINT('Ctrl Pts',(60.1170547888572,-40.1094085617672,12.));
#58689=CARTESIAN_POINT('Ctrl Pts',(60.0931981532194,-40.1038305015764,12.));
#58690=CARTESIAN_POINT('Ctrl Pts',(60.0693871144207,-40.0982388335421,12.));
#58691=CARTESIAN_POINT('Ctrl Pts',(60.0456217702203,-40.0926336409787,12.));
#58692=CARTESIAN_POINT('Ctrl Pts',(60.0219022187066,-40.0870150076078,12.));
#58693=CARTESIAN_POINT('Ctrl Pts',(59.9982285582991,-40.0813830175629,12.));
#58694=CARTESIAN_POINT('Ctrl Pts',(59.974600887759,-40.0757377553894,12.));
#58695=CARTESIAN_POINT('Ctrl Pts',(59.9510193061929,-40.0700793060475,12.));
#58696=CARTESIAN_POINT('Ctrl Pts',(59.927483913055,-40.0644077549158,12.));
#58697=CARTESIAN_POINT('Ctrl Pts',(59.9039948081428,-40.0587231877959,12.));
#58698=CARTESIAN_POINT('Ctrl Pts',(59.8805520915972,-40.0530256909161,12.));
#58699=CARTESIAN_POINT('Ctrl Pts',(59.8571558639145,-40.0473153509324,12.));
#58700=CARTESIAN_POINT('Ctrl Pts',(59.8338062259492,-40.0415922549315,12.));
#58701=CARTESIAN_POINT('Ctrl Pts',(59.8105032789179,-40.0358564904341,12.));
#58702=CARTESIAN_POINT('Ctrl Pts',(59.7872471243942,-40.0301081454002,12.));
#58703=CARTESIAN_POINT('Ctrl Pts',(59.7640378643106,-40.0243473082337,12.));
#58704=CARTESIAN_POINT('Ctrl Pts',(59.7408756009679,-40.0185740677821,12.));
#58705=CARTESIAN_POINT('Ctrl Pts',(59.7177604370403,-40.0127885133403,12.));
#58706=CARTESIAN_POINT('Ctrl Pts',(59.6946924755773,-40.0069907346538,12.));
#58707=CARTESIAN_POINT('Ctrl Pts',(59.6716718200005,-40.0011808219241,12.));
#58708=CARTESIAN_POINT('Ctrl Pts',(59.6486985741041,-39.9953588658132,12.));
#58709=CARTESIAN_POINT('Ctrl Pts',(59.6257728420669,-39.9895249574448,12.));
#58710=CARTESIAN_POINT('Ctrl Pts',(59.6028947284562,-39.9836791884079,12.));
#58711=CARTESIAN_POINT('Ctrl Pts',(59.5800643382314,-39.9778216507605,12.));
#58712=CARTESIAN_POINT('Ctrl Pts',(59.5572817767388,-39.9719524370346,12.));
#58713=CARTESIAN_POINT('Ctrl Pts',(59.5345471497128,-39.9660716402403,12.));
#58714=CARTESIAN_POINT('Ctrl Pts',(59.511860563289,-39.9601793538683,12.));
#58715=CARTESIAN_POINT('Ctrl Pts',(59.4892221240068,-39.9542756718922,12.));
#58716=CARTESIAN_POINT('Ctrl Pts',(59.4666319388133,-39.9483606887738,12.));
#58717=CARTESIAN_POINT('Ctrl Pts',(59.4440901150582,-39.9424344994673,12.));
#58718=CARTESIAN_POINT('Ctrl Pts',(59.4215967604967,-39.9364971994242,12.));
#58719=CARTESIAN_POINT('Ctrl Pts',(59.3991519833016,-39.9305488845958,12.));
#58720=CARTESIAN_POINT('Ctrl Pts',(59.3767558920675,-39.9245896514367,12.));
#58721=CARTESIAN_POINT('Ctrl Pts',(59.3544085958151,-39.9186195969104,12.));
#58722=CARTESIAN_POINT('Ctrl Pts',(59.3321102039852,-39.9126388184936,12.));
#58723=CARTESIAN_POINT('Ctrl Pts',(59.3098608264419,-39.9066474141803,12.));
#58724=CARTESIAN_POINT('Ctrl Pts',(59.2876605734846,-39.9006454824845,12.));
#58725=CARTESIAN_POINT('Ctrl Pts',(59.2655095558521,-39.8946331224438,12.));
#58726=CARTESIAN_POINT('Ctrl Pts',(59.2434078847247,-39.8886104336242,12.));
#58727=CARTESIAN_POINT('Ctrl Pts',(59.2213556717209,-39.8825775161267,12.));
#58728=CARTESIAN_POINT('Ctrl Pts',(59.1993530289028,-39.876534470591,12.));
#58729=CARTESIAN_POINT('Ctrl Pts',(59.1774000687879,-39.8704813981989,12.));
#58730=CARTESIAN_POINT('Ctrl Pts',(59.1554969043522,-39.8644184006787,12.));
#58731=CARTESIAN_POINT('Ctrl Pts',(59.1336436490342,-39.8583455803105,12.));
#58732=CARTESIAN_POINT('Ctrl Pts',(59.1118404167292,-39.8522630399328,12.));
#58733=CARTESIAN_POINT('Ctrl Pts',(59.090087321798,-39.8461708829456,12.));
#58734=CARTESIAN_POINT('Ctrl Pts',(59.0683844790764,-39.8400692133139,12.));
#58735=CARTESIAN_POINT('Ctrl Pts',(59.0467320038784,-39.8339581355716,12.));
#58736=CARTESIAN_POINT('Ctrl Pts',(59.0251300119973,-39.8278377548262,12.));
#58737=CARTESIAN_POINT('Ctrl Pts',(59.0035786197024,-39.821708176766,12.));
#58738=CARTESIAN_POINT('Ctrl Pts',(58.9820779437484,-39.8155695076626,12.));
#58739=CARTESIAN_POINT('Ctrl Pts',(58.9606281013875,-39.8094218543782,12.));
#58740=CARTESIAN_POINT('Ctrl Pts',(58.9392292103747,-39.8032653243712,12.));
#58741=CARTESIAN_POINT('Ctrl Pts',(58.9178813889703,-39.7971000257044,12.));
#58742=CARTESIAN_POINT('Ctrl Pts',(58.8965847559391,-39.7909260670517,12.));
#58743=CARTESIAN_POINT('Ctrl Pts',(58.8753394305585,-39.7847435576997,12.));
#58744=CARTESIAN_POINT('Ctrl Pts',(58.8541455326231,-39.7785526075479,12.));
#58745=CARTESIAN_POINT('Ctrl Pts',(58.8330031824453,-39.772353327112,12.));
#58746=CARTESIAN_POINT('Ctrl Pts',(58.8119125008517,-39.7661458275274,12.));
#58747=CARTESIAN_POINT('Ctrl Pts',(58.7908736091798,-39.7599302205521,12.));
#58748=CARTESIAN_POINT('Ctrl Pts',(58.7698866293029,-39.7537066185813,12.));
#58749=CARTESIAN_POINT('Ctrl Pts',(58.7489516836445,-39.7474751346599,12.));
#58750=CARTESIAN_POINT('Ctrl Pts',(58.7280688951916,-39.7412358824953,12.));
#58751=CARTESIAN_POINT('Ctrl Pts',(58.7072383875027,-39.734988976475,12.));
#58752=CARTESIAN_POINT('Ctrl Pts',(58.6864602847088,-39.7287345316681,12.));
#58753=CARTESIAN_POINT('Ctrl Pts',(58.6657347115034,-39.7224726638101,12.));
#58754=CARTESIAN_POINT('Ctrl Pts',(58.6450617931274,-39.71620348929,12.));
#58755=CARTESIAN_POINT('Ctrl Pts',(58.6244416553562,-39.7099271251413,12.));
#58756=CARTESIAN_POINT('Ctrl Pts',(58.6038744244659,-39.7036436890233,12.));
#58757=CARTESIAN_POINT('Ctrl Pts',(58.5833602272743,-39.697353299254,12.));
#58758=CARTESIAN_POINT('Ctrl Pts',(58.5628991912052,-39.6910560748629,12.));
#58759=CARTESIAN_POINT('Ctrl Pts',(58.5424914443415,-39.6847521356395,12.));
#58760=CARTESIAN_POINT('Ctrl Pts',(58.5221371154761,-39.6784416021826,12.));
#58761=CARTESIAN_POINT('Ctrl Pts',(58.5018363341604,-39.6721245959531,12.));
#58762=CARTESIAN_POINT('Ctrl Pts',(58.4815892306066,-39.6658012391815,12.));
#58763=CARTESIAN_POINT('Ctrl Pts',(58.4613959355788,-39.6594716547689,12.));
#58764=CARTESIAN_POINT('Ctrl Pts',(58.4412565802979,-39.653135966204,12.));
#58765=CARTESIAN_POINT('Ctrl Pts',(58.4211712963004,-39.6467942974451,12.));
#58766=CARTESIAN_POINT('Ctrl Pts',(58.4011402154196,-39.6404467729094,12.));
#58767=CARTESIAN_POINT('Ctrl Pts',(58.3811634701037,-39.6340935177476,12.));
#58768=CARTESIAN_POINT('Ctrl Pts',(58.3612411936904,-39.6277346580892,12.));
#58769=CARTESIAN_POINT('Ctrl Pts',(58.3413735206423,-39.6213703212531,12.));
#58770=CARTESIAN_POINT('Ctrl Pts',(58.3215605869221,-39.6150006360915,12.));
#58771=CARTESIAN_POINT('Ctrl Pts',(58.3018025297323,-39.6086257327583,12.));
#58772=CARTESIAN_POINT('Ctrl Pts',(58.2820994868118,-39.602245742079,12.));
#58773=CARTESIAN_POINT('Ctrl Pts',(58.2624515958419,-39.5958607950239,12.));
#58774=CARTESIAN_POINT('Ctrl Pts',(58.2428589938369,-39.5894710221713,12.));
#58775=CARTESIAN_POINT('Ctrl Pts',(58.2233218164365,-39.5830765530891,12.));
#58776=CARTESIAN_POINT('Ctrl Pts',(58.2038401992457,-39.57667751752,12.));
#58777=CARTESIAN_POINT('Ctrl Pts',(58.1844142794338,-39.5702740467999,12.));
#58778=CARTESIAN_POINT('Ctrl Pts',(58.1650441970387,-39.563866275018,12.));
#58779=CARTESIAN_POINT('Ctrl Pts',(58.1457300968499,-39.5574543406982,12.));
#58780=CARTESIAN_POINT('Ctrl Pts',(58.126472128574,-39.5510383869505,12.));
#58781=CARTESIAN_POINT('Ctrl Pts',(58.1072704428928,-39.5446185579638,12.));
#58782=CARTESIAN_POINT('Ctrl Pts',(58.088125187992,-39.5381949959221,12.));
#58783=CARTESIAN_POINT('Ctrl Pts',(58.0690365065374,-39.5317678383217,12.));
#58784=CARTESIAN_POINT('Ctrl Pts',(58.0500045308412,-39.5253372136887,12.));
#58785=CARTESIAN_POINT('Ctrl Pts',(58.0310293875262,-39.5189032457184,12.));
#58786=CARTESIAN_POINT('Ctrl Pts',(58.0121112067895,-39.5124660614976,12.));
#58787=CARTESIAN_POINT('Ctrl Pts',(57.9932501298522,-39.5060257981225,12.));
#58788=CARTESIAN_POINT('Ctrl Pts',(57.974446317937,-39.499582610674,12.));
#58789=CARTESIAN_POINT('Ctrl Pts',(57.9556999583892,-39.4931366776714,12.));
#58790=CARTESIAN_POINT('Ctrl Pts',(57.937011245663,-39.4866881842317,12.));
#58791=CARTESIAN_POINT('Ctrl Pts',(57.9183803632403,-39.4802373061058,12.));
#58792=CARTESIAN_POINT('Ctrl Pts',(57.8998074670478,-39.473784194937,12.));
#58793=CARTESIAN_POINT('Ctrl Pts',(57.8812926637177,-39.4673289592259,12.));
#58794=CARTESIAN_POINT('Ctrl Pts',(57.8628360096803,-39.4608716627118,12.));
#58795=CARTESIAN_POINT('Ctrl Pts',(57.8481172247495,-39.4557042029652,12.));
#58796=CARTESIAN_POINT('Ctrl Pts',(57.837104315141,-39.4518277003553,12.));
#58797=CARTESIAN_POINT('Ctrl Pts',(57.8297740100947,-39.4492429618443,12.));
#58798=CARTESIAN_POINT('Ctrl Pts',(57.8261117662438,-39.4479504917287,12.));
#58799=CARTESIAN_POINT('Ctrl Pts',(62.9864049293894,-39.2292784191813,-5.55111512312578E-16));
#58800=CARTESIAN_POINT('Ctrl Pts',(62.9864049293894,-39.2292784191813,4.));
#58801=CARTESIAN_POINT('Ctrl Pts',(62.9864049293894,-39.2292784191812,8.));
#58802=CARTESIAN_POINT('Ctrl Pts',(62.9864049293894,-39.2292784191812,12.));
#58803=CARTESIAN_POINT('Ctrl Pts',(63.0475916539463,-39.3205491216485,-5.55111512312578E-16));
#58804=CARTESIAN_POINT('Ctrl Pts',(63.0475916539463,-39.3205491216485,4.));
#58805=CARTESIAN_POINT('Ctrl Pts',(63.0475916539463,-39.3205491216485,8.));
#58806=CARTESIAN_POINT('Ctrl Pts',(63.0475916539463,-39.3205491216485,12.));
#58807=CARTESIAN_POINT('Ctrl Pts',(63.0996457958581,-39.5164137621548,-5.55111512312578E-16));
#58808=CARTESIAN_POINT('Ctrl Pts',(63.0996457958581,-39.5164137621548,4.));
#58809=CARTESIAN_POINT('Ctrl Pts',(63.0996457958582,-39.5164137621548,7.99999999999999));
#58810=CARTESIAN_POINT('Ctrl Pts',(63.0996457958582,-39.5164137621548,12.));
#58811=CARTESIAN_POINT('Ctrl Pts',(63.0378706912073,-39.7049575044674,-5.55111512312578E-16));
#58812=CARTESIAN_POINT('Ctrl Pts',(63.0378706912073,-39.7049575044674,4.));
#58813=CARTESIAN_POINT('Ctrl Pts',(63.0378706912074,-39.7049575044674,8.00000000000001));
#58814=CARTESIAN_POINT('Ctrl Pts',(63.0378706912074,-39.7049575044674,12.));
#58815=CARTESIAN_POINT('Ctrl Pts',(62.9938720098781,-39.7746412831476,-5.55111512312578E-16));
#58816=CARTESIAN_POINT('Ctrl Pts',(62.9938720098781,-39.7746412831476,4.));
#58817=CARTESIAN_POINT('Ctrl Pts',(62.9938720098781,-39.7746412831477,8.));
#58818=CARTESIAN_POINT('Ctrl Pts',(62.9938720098781,-39.7746412831477,12.));
#58819=CARTESIAN_POINT('',(62.9864049293894,-39.2292784191813,2.77555756156289E-16));
#58820=CARTESIAN_POINT('',(62.9938720098782,-39.7746412831477,0.));
#58821=CARTESIAN_POINT('Ctrl Pts',(62.9864049293894,-39.2292784191813,-1.38777878078145E-16));
#58822=CARTESIAN_POINT('Ctrl Pts',(63.0475916539463,-39.3205491216485,-1.38777878078145E-16));
#58823=CARTESIAN_POINT('Ctrl Pts',(63.0773368778959,-39.4324717733664,-1.38777878078144E-16));
#58824=CARTESIAN_POINT('Ctrl Pts',(63.0699133682741,-39.5420039277149,-1.38777878078145E-16));
#58825=CARTESIAN_POINT('Ctrl Pts',(63.0643457360577,-39.6241530434763,-1.38777878078145E-16));
#58826=CARTESIAN_POINT('Ctrl Pts',(63.0378706912073,-39.7049575044674,-1.38777878078145E-16));
#58827=CARTESIAN_POINT('Ctrl Pts',(62.9938720098781,-39.7746412831476,-1.38777878078145E-16));
#58828=CARTESIAN_POINT('',(62.9938720098782,-39.7746412831478,12.));
#58829=CARTESIAN_POINT('Ctrl Pts',(62.9938720098781,-39.7746412831476,-5.55111512312578E-16));
#58830=CARTESIAN_POINT('Ctrl Pts',(62.9938720098781,-39.7746412831476,4.));
#58831=CARTESIAN_POINT('Ctrl Pts',(62.9938720098781,-39.7746412831477,8.));
#58832=CARTESIAN_POINT('Ctrl Pts',(62.9938720098781,-39.7746412831477,12.));
#58833=CARTESIAN_POINT('',(62.9864049293894,-39.2292784191812,12.));
#58834=CARTESIAN_POINT('Ctrl Pts',(62.9938720098781,-39.7746412831477,12.));
#58835=CARTESIAN_POINT('Ctrl Pts',(63.0378706912074,-39.7049575044674,12.));
#58836=CARTESIAN_POINT('Ctrl Pts',(63.0643457360577,-39.6241530434763,12.));
#58837=CARTESIAN_POINT('Ctrl Pts',(63.0699133682741,-39.5420039277149,12.));
#58838=CARTESIAN_POINT('Ctrl Pts',(63.077336877896,-39.4324717733664,12.));
#58839=CARTESIAN_POINT('Ctrl Pts',(63.0475916539463,-39.3205491216485,12.));
#58840=CARTESIAN_POINT('Ctrl Pts',(62.9864049293894,-39.2292784191812,12.));
#58841=CARTESIAN_POINT('Ctrl Pts',(62.9864049293894,-39.2292784191812,12.));
#58842=CARTESIAN_POINT('Ctrl Pts',(62.9864049293894,-39.2292784191812,8.));
#58843=CARTESIAN_POINT('Ctrl Pts',(62.9864049293894,-39.2292784191813,4.));
#58844=CARTESIAN_POINT('Ctrl Pts',(62.9864049293894,-39.2292784191813,-5.55111512312578E-16));
#58845=CARTESIAN_POINT('Origin',(3.16193356404481E-10,-2.01319694273778E-10,
0.));
#58846=CARTESIAN_POINT('Origin',(3.16193356404481E-10,-2.01319694273778E-10,
12.));
#58847=CARTESIAN_POINT('Origin',(3.16193356404481E-10,-2.01319694273778E-10,
0.));
#58848=CARTESIAN_POINT('Ctrl Pts',(58.9211100416397,-45.591148170023,-2.77555756156289E-15));
#58849=CARTESIAN_POINT('Ctrl Pts',(58.9211100416397,-45.591148170023,4.));
#58850=CARTESIAN_POINT('Ctrl Pts',(58.9211100416396,-45.591148170023,8.));
#58851=CARTESIAN_POINT('Ctrl Pts',(58.9211100416396,-45.591148170023,12.));
#58852=CARTESIAN_POINT('Ctrl Pts',(58.8538661785413,-45.6780528262178,-2.77555756156289E-15));
#58853=CARTESIAN_POINT('Ctrl Pts',(58.8538661785413,-45.6780528262178,4.));
#58854=CARTESIAN_POINT('Ctrl Pts',(58.8538661785413,-45.6780528262179,8.));
#58855=CARTESIAN_POINT('Ctrl Pts',(58.8538661785413,-45.6780528262179,12.));
#58856=CARTESIAN_POINT('Ctrl Pts',(58.6845061116498,-45.7893619681936,-2.55630692362817E-15));
#58857=CARTESIAN_POINT('Ctrl Pts',(58.6845061116498,-45.7893619681936,4.));
#58858=CARTESIAN_POINT('Ctrl Pts',(58.6845061116497,-45.7893619681937,7.99999999999999));
#58859=CARTESIAN_POINT('Ctrl Pts',(58.6845061116497,-45.7893619681937,12.));
#58860=CARTESIAN_POINT('Ctrl Pts',(58.4861028141709,-45.7903667155979,-2.0357240208649E-15));
#58861=CARTESIAN_POINT('Ctrl Pts',(58.4861028141709,-45.7903667155979,4.));
#58862=CARTESIAN_POINT('Ctrl Pts',(58.4861028141708,-45.790366715598,8.00000000000001));
#58863=CARTESIAN_POINT('Ctrl Pts',(58.4861028141708,-45.790366715598,12.));
#58864=CARTESIAN_POINT('Ctrl Pts',(58.4060826907377,-45.7706564944765,-1.78476208015248E-15));
#58865=CARTESIAN_POINT('Ctrl Pts',(58.4060826907377,-45.7706564944765,4.));
#58866=CARTESIAN_POINT('Ctrl Pts',(58.4060826907376,-45.7706564944766,8.));
#58867=CARTESIAN_POINT('Ctrl Pts',(58.4060826907376,-45.7706564944766,12.));
#58868=CARTESIAN_POINT('',(58.9211100416397,-45.591148170023,2.77555756156289E-16));
#58869=CARTESIAN_POINT('',(58.4060826907377,-45.7706564944766,0.));
#58870=CARTESIAN_POINT('Ctrl Pts',(58.9211100416397,-45.591148170023,-9.71445146547012E-16));
#58871=CARTESIAN_POINT('Ctrl Pts',(58.8538661785413,-45.6780528262178,-9.71445146547012E-16));
#58872=CARTESIAN_POINT('Ctrl Pts',(58.7570889974605,-45.741658050204,-8.46159067727172E-16));
#58873=CARTESIAN_POINT('Ctrl Pts',(58.6508283125143,-45.7692455126974,-6.22478779983725E-16));
#58874=CARTESIAN_POINT('Ctrl Pts',(58.5711327988047,-45.7899361095675,-4.5471856417614E-16));
#58875=CARTESIAN_POINT('Ctrl Pts',(58.4861028141709,-45.7903667155979,-2.31611605849026E-16));
#58876=CARTESIAN_POINT('Ctrl Pts',(58.4060826907377,-45.7706564944765,1.93503348634022E-17));
#58877=CARTESIAN_POINT('',(58.4060826907376,-45.7706564944766,12.));
#58878=CARTESIAN_POINT('Ctrl Pts',(58.4060826907377,-45.7706564944765,-1.78476208015248E-15));
#58879=CARTESIAN_POINT('Ctrl Pts',(58.4060826907377,-45.7706564944765,4.));
#58880=CARTESIAN_POINT('Ctrl Pts',(58.4060826907376,-45.7706564944766,8.));
#58881=CARTESIAN_POINT('Ctrl Pts',(58.4060826907376,-45.7706564944766,12.));
#58882=CARTESIAN_POINT('',(58.9211100416396,-45.591148170023,12.));
#58883=CARTESIAN_POINT('Ctrl Pts',(58.4060826907376,-45.7706564944766,12.));
#58884=CARTESIAN_POINT('Ctrl Pts',(58.4861028141708,-45.790366715598,12.));
#58885=CARTESIAN_POINT('Ctrl Pts',(58.5711327988046,-45.7899361095676,12.));
#58886=CARTESIAN_POINT('Ctrl Pts',(58.6508283125142,-45.7692455126975,12.));
#58887=CARTESIAN_POINT('Ctrl Pts',(58.7570889974604,-45.7416580502041,12.));
#58888=CARTESIAN_POINT('Ctrl Pts',(58.8538661785413,-45.6780528262179,12.));
#58889=CARTESIAN_POINT('Ctrl Pts',(58.9211100416396,-45.591148170023,12.));
#58890=CARTESIAN_POINT('Ctrl Pts',(58.9211100416396,-45.591148170023,12.));
#58891=CARTESIAN_POINT('Ctrl Pts',(58.9211100416396,-45.591148170023,8.));
#58892=CARTESIAN_POINT('Ctrl Pts',(58.9211100416397,-45.591148170023,4.));
#58893=CARTESIAN_POINT('Ctrl Pts',(58.9211100416397,-45.591148170023,-2.77555756156289E-15));
#58894=CARTESIAN_POINT('Ctrl Pts',(54.1679505278134,-44.3377168516418,0.));
#58895=CARTESIAN_POINT('Ctrl Pts',(54.1679505278134,-44.3377168516418,12.));
#58896=CARTESIAN_POINT('Ctrl Pts',(54.1714861895278,-44.3393235891014,0.));
#58897=CARTESIAN_POINT('Ctrl Pts',(54.1714861895278,-44.3393235891014,12.));
#58898=CARTESIAN_POINT('Ctrl Pts',(54.1785633257456,-44.3425373700829,0.));
#58899=CARTESIAN_POINT('Ctrl Pts',(54.1785633257456,-44.3425373700829,12.));
#58900=CARTESIAN_POINT('Ctrl Pts',(54.1891964684439,-44.3473589597468,0.));
#58901=CARTESIAN_POINT('Ctrl Pts',(54.1891964684439,-44.3473589597468,12.));
#58902=CARTESIAN_POINT('Ctrl Pts',(54.203408870162,-44.3537895823819,0.));
#58903=CARTESIAN_POINT('Ctrl Pts',(54.203408870162,-44.3537895823819,12.));
#58904=CARTESIAN_POINT('Ctrl Pts',(54.2212325005847,-44.3618309103245,0.));
#58905=CARTESIAN_POINT('Ctrl Pts',(54.2212325005847,-44.3618309103245,12.));
#58906=CARTESIAN_POINT('Ctrl Pts',(54.2391142386354,-44.369875253351,0.));
#58907=CARTESIAN_POINT('Ctrl Pts',(54.2391142386354,-44.369875253351,12.));
#58908=CARTESIAN_POINT('Ctrl Pts',(54.2570540336536,-44.3779225430461,0.));
#58909=CARTESIAN_POINT('Ctrl Pts',(54.2570540336536,-44.3779225430461,12.));
#58910=CARTESIAN_POINT('Ctrl Pts',(54.2750517888695,-44.3859726620288,0.));
#58911=CARTESIAN_POINT('Ctrl Pts',(54.2750517888695,-44.3859726620288,12.));
#58912=CARTESIAN_POINT('Ctrl Pts',(54.2931073621661,-44.3940254456427,0.));
#58913=CARTESIAN_POINT('Ctrl Pts',(54.2931073621661,-44.3940254456427,12.));
#58914=CARTESIAN_POINT('Ctrl Pts',(54.3112205860776,-44.4020807028144,0.));
#58915=CARTESIAN_POINT('Ctrl Pts',(54.3112205860776,-44.4020807028144,12.));
#58916=CARTESIAN_POINT('Ctrl Pts',(54.3293912830237,-44.4101382321834,0.));
#58917=CARTESIAN_POINT('Ctrl Pts',(54.3293912830237,-44.4101382321834,12.));
#58918=CARTESIAN_POINT('Ctrl Pts',(54.347619281931,-44.4181978395814,0.));
#58919=CARTESIAN_POINT('Ctrl Pts',(54.347619281931,-44.4181978395814,12.));
#58920=CARTESIAN_POINT('Ctrl Pts',(54.3659044357064,-44.4262593564664,0.));
#58921=CARTESIAN_POINT('Ctrl Pts',(54.3659044357064,-44.4262593564664,12.));
#58922=CARTESIAN_POINT('Ctrl Pts',(54.3842466156151,-44.4343226339555,0.));
#58923=CARTESIAN_POINT('Ctrl Pts',(54.3842466156151,-44.4343226339555,12.));
#58924=CARTESIAN_POINT('Ctrl Pts',(54.4026457030316,-44.442387534098,0.));
#58925=CARTESIAN_POINT('Ctrl Pts',(54.4026457030316,-44.442387534098,12.));
#58926=CARTESIAN_POINT('Ctrl Pts',(54.4211015825959,-44.4504539226336,0.));
#58927=CARTESIAN_POINT('Ctrl Pts',(54.4211015825959,-44.4504539226336,12.));
#58928=CARTESIAN_POINT('Ctrl Pts',(54.4396141337008,-44.4585216599933,0.));
#58929=CARTESIAN_POINT('Ctrl Pts',(54.4396141337008,-44.4585216599933,12.));
#58930=CARTESIAN_POINT('Ctrl Pts',(54.4581832262072,-44.4665905967701,0.));
#58931=CARTESIAN_POINT('Ctrl Pts',(54.4581832262072,-44.4665905967701,12.));
#58932=CARTESIAN_POINT('Ctrl Pts',(54.4768087248854,-44.4746605784056,0.));
#58933=CARTESIAN_POINT('Ctrl Pts',(54.4768087248854,-44.4746605784056,12.));
#58934=CARTESIAN_POINT('Ctrl Pts',(54.4954904921938,-44.4827314481271,0.));
#58935=CARTESIAN_POINT('Ctrl Pts',(54.4954904921938,-44.4827314481271,12.));
#58936=CARTESIAN_POINT('Ctrl Pts',(54.5142283914684,-44.4908030503209,0.));
#58937=CARTESIAN_POINT('Ctrl Pts',(54.5142283914684,-44.4908030503209,12.));
#58938=CARTESIAN_POINT('Ctrl Pts',(54.5330222905438,-44.4988752343715,0.));
#58939=CARTESIAN_POINT('Ctrl Pts',(54.5330222905438,-44.4988752343715,12.));
#58940=CARTESIAN_POINT('Ctrl Pts',(54.5518720616016,-44.5069478544945,0.));
#58941=CARTESIAN_POINT('Ctrl Pts',(54.5518720616016,-44.5069478544945,12.));
#58942=CARTESIAN_POINT('Ctrl Pts',(54.5707775794412,-44.5150207678988,0.));
#58943=CARTESIAN_POINT('Ctrl Pts',(54.5707775794412,-44.5150207678988,12.));
#58944=CARTESIAN_POINT('Ctrl Pts',(54.5897387202815,-44.5230938335167,0.));
#58945=CARTESIAN_POINT('Ctrl Pts',(54.5897387202815,-44.5230938335167,12.));
#58946=CARTESIAN_POINT('Ctrl Pts',(54.6087553602914,-44.5311669104515,0.));
#58947=CARTESIAN_POINT('Ctrl Pts',(54.6087553602914,-44.5311669104515,12.));
#58948=CARTESIAN_POINT('Ctrl Pts',(54.6278273743587,-44.5392398566802,0.));
#58949=CARTESIAN_POINT('Ctrl Pts',(54.6278273743587,-44.5392398566802,12.));
#58950=CARTESIAN_POINT('Ctrl Pts',(54.6469546367408,-44.5473125297312,0.));
#58951=CARTESIAN_POINT('Ctrl Pts',(54.6469546367408,-44.5473125297312,12.));
#58952=CARTESIAN_POINT('Ctrl Pts',(54.6661370216252,-44.5553847872721,0.));
#58953=CARTESIAN_POINT('Ctrl Pts',(54.6661370216252,-44.5553847872721,12.));
#58954=CARTESIAN_POINT('Ctrl Pts',(54.6853744036751,-44.5634564876863,0.));
#58955=CARTESIAN_POINT('Ctrl Pts',(54.6853744036751,-44.5634564876863,12.));
#58956=CARTESIAN_POINT('Ctrl Pts',(54.7046666586754,-44.5715274907619,0.));
#58957=CARTESIAN_POINT('Ctrl Pts',(54.7046666586754,-44.5715274907619,12.));
#58958=CARTESIAN_POINT('Ctrl Pts',(54.7240136637717,-44.5795976579454,0.));
#58959=CARTESIAN_POINT('Ctrl Pts',(54.7240136637717,-44.5795976579454,12.));
#58960=CARTESIAN_POINT('Ctrl Pts',(54.7434152971267,-44.5876668519661,0.));
#58961=CARTESIAN_POINT('Ctrl Pts',(54.7434152971267,-44.5876668519661,12.));
#58962=CARTESIAN_POINT('Ctrl Pts',(54.7628714377037,-44.5957349366059,0.));
#58963=CARTESIAN_POINT('Ctrl Pts',(54.7628714377037,-44.5957349366059,12.));
#58964=CARTESIAN_POINT('Ctrl Pts',(54.7823819650148,-44.603801776431,0.));
#58965=CARTESIAN_POINT('Ctrl Pts',(54.7823819650148,-44.603801776431,12.));
#58966=CARTESIAN_POINT('Ctrl Pts',(54.8019467588278,-44.6118672364906,0.));
#58967=CARTESIAN_POINT('Ctrl Pts',(54.8019467588278,-44.6118672364906,12.));
#58968=CARTESIAN_POINT('Ctrl Pts',(54.8215656991837,-44.6199311823293,0.));
#58969=CARTESIAN_POINT('Ctrl Pts',(54.8215656991837,-44.6199311823293,12.));
#58970=CARTESIAN_POINT('Ctrl Pts',(54.8412386665276,-44.6279934801169,0.));
#58971=CARTESIAN_POINT('Ctrl Pts',(54.8412386665276,-44.6279934801169,12.));
#58972=CARTESIAN_POINT('Ctrl Pts',(54.860965541796,-44.6360539967392,0.));
#58973=CARTESIAN_POINT('Ctrl Pts',(54.860965541796,-44.6360539967392,12.));
#58974=CARTESIAN_POINT('Ctrl Pts',(54.8807462065164,-44.6441125999063,0.));
#58975=CARTESIAN_POINT('Ctrl Pts',(54.8807462065164,-44.6441125999063,12.));
#58976=CARTESIAN_POINT('Ctrl Pts',(54.9005805428969,-44.6521691582534,0.));
#58977=CARTESIAN_POINT('Ctrl Pts',(54.9005805428969,-44.6521691582534,12.));
#58978=CARTESIAN_POINT('Ctrl Pts',(54.9204684337822,-44.6602235412836,0.));
#58979=CARTESIAN_POINT('Ctrl Pts',(54.9204684337822,-44.6602235412836,12.));
#58980=CARTESIAN_POINT('Ctrl Pts',(54.9404097626077,-44.6682756193147,0.));
#58981=CARTESIAN_POINT('Ctrl Pts',(54.9404097626077,-44.6682756193147,12.));
#58982=CARTESIAN_POINT('Ctrl Pts',(54.9604044133501,-44.6763252634259,0.));
#58983=CARTESIAN_POINT('Ctrl Pts',(54.9604044133501,-44.6763252634259,12.));
#58984=CARTESIAN_POINT('Ctrl Pts',(54.9804522704686,-44.6843723454,0.));
#58985=CARTESIAN_POINT('Ctrl Pts',(54.9804522704686,-44.6843723454,12.));
#58986=CARTESIAN_POINT('Ctrl Pts',(55.0005532188667,-44.6924167376869,0.));
#58987=CARTESIAN_POINT('Ctrl Pts',(55.0005532188667,-44.6924167376869,12.));
#58988=CARTESIAN_POINT('Ctrl Pts',(55.0207071439237,-44.7004583134249,0.));
#58989=CARTESIAN_POINT('Ctrl Pts',(55.0207071439237,-44.7004583134249,12.));
#58990=CARTESIAN_POINT('Ctrl Pts',(55.0409139315078,-44.7084969464513,0.));
#58991=CARTESIAN_POINT('Ctrl Pts',(55.0409139315078,-44.7084969464513,12.));
#58992=CARTESIAN_POINT('Ctrl Pts',(55.0611734679894,-44.716532511316,0.));
#58993=CARTESIAN_POINT('Ctrl Pts',(55.0611734679894,-44.716532511316,12.));
#58994=CARTESIAN_POINT('Ctrl Pts',(55.0814856402495,-44.7245648832979,0.));
#58995=CARTESIAN_POINT('Ctrl Pts',(55.0814856402495,-44.7245648832979,12.));
#58996=CARTESIAN_POINT('Ctrl Pts',(55.1018503356795,-44.7325939384035,0.));
#58997=CARTESIAN_POINT('Ctrl Pts',(55.1018503356795,-44.7325939384035,12.));
#58998=CARTESIAN_POINT('Ctrl Pts',(55.1222674421743,-44.740619553348,0.));
#58999=CARTESIAN_POINT('Ctrl Pts',(55.1222674421743,-44.740619553348,12.));
#59000=CARTESIAN_POINT('Ctrl Pts',(55.14273684812,-44.748641605542,0.));
#59001=CARTESIAN_POINT('Ctrl Pts',(55.14273684812,-44.748641605542,12.));
#59002=CARTESIAN_POINT('Ctrl Pts',(55.1632584423815,-44.7566599730773,0.));
#59003=CARTESIAN_POINT('Ctrl Pts',(55.1632584423815,-44.7566599730773,12.));
#59004=CARTESIAN_POINT('Ctrl Pts',(55.1838321142779,-44.7646745347109,0.));
#59005=CARTESIAN_POINT('Ctrl Pts',(55.1838321142779,-44.7646745347109,12.));
#59006=CARTESIAN_POINT('Ctrl Pts',(55.2044577535866,-44.7726851698619,0.));
#59007=CARTESIAN_POINT('Ctrl Pts',(55.2044577535866,-44.7726851698619,12.));
#59008=CARTESIAN_POINT('Ctrl Pts',(55.2251352505475,-44.7806917586077,0.));
#59009=CARTESIAN_POINT('Ctrl Pts',(55.2251352505475,-44.7806917586077,12.));
#59010=CARTESIAN_POINT('Ctrl Pts',(55.2458644958617,-44.7886941816823,0.));
#59011=CARTESIAN_POINT('Ctrl Pts',(55.2458644958617,-44.7886941816823,12.));
#59012=CARTESIAN_POINT('Ctrl Pts',(55.2666453806882,-44.7966923204741,0.));
#59013=CARTESIAN_POINT('Ctrl Pts',(55.2666453806882,-44.7966923204741,12.));
#59014=CARTESIAN_POINT('Ctrl Pts',(55.2874777966349,-44.8046860570245,0.));
#59015=CARTESIAN_POINT('Ctrl Pts',(55.2874777966349,-44.8046860570245,12.));
#59016=CARTESIAN_POINT('Ctrl Pts',(55.3083616357605,-44.812675274021,0.));
#59017=CARTESIAN_POINT('Ctrl Pts',(55.3083616357605,-44.812675274021,12.));
#59018=CARTESIAN_POINT('Ctrl Pts',(55.3292967905725,-44.8206598547889,0.));
#59019=CARTESIAN_POINT('Ctrl Pts',(55.3292967905725,-44.8206598547889,12.));
#59020=CARTESIAN_POINT('Ctrl Pts',(55.3502831540229,-44.8286396832849,0.));
#59021=CARTESIAN_POINT('Ctrl Pts',(55.3502831540229,-44.8286396832849,12.));
#59022=CARTESIAN_POINT('Ctrl Pts',(55.3713206194962,-44.8366146440896,0.));
#59023=CARTESIAN_POINT('Ctrl Pts',(55.3713206194962,-44.8366146440896,12.));
#59024=CARTESIAN_POINT('Ctrl Pts',(55.3924090808002,-44.8445846224034,0.));
#59025=CARTESIAN_POINT('Ctrl Pts',(55.3924090808002,-44.8445846224034,12.));
#59026=CARTESIAN_POINT('Ctrl Pts',(55.4135484321706,-44.8525495040398,0.));
#59027=CARTESIAN_POINT('Ctrl Pts',(55.4135484321706,-44.8525495040398,12.));
#59028=CARTESIAN_POINT('Ctrl Pts',(55.4347385682697,-44.8605091754208,0.));
#59029=CARTESIAN_POINT('Ctrl Pts',(55.4347385682697,-44.8605091754208,12.));
#59030=CARTESIAN_POINT('Ctrl Pts',(55.4559793841838,-44.8684635235727,0.));
#59031=CARTESIAN_POINT('Ctrl Pts',(55.4559793841838,-44.8684635235727,12.));
#59032=CARTESIAN_POINT('Ctrl Pts',(55.4772707754139,-44.8764124361218,0.));
#59033=CARTESIAN_POINT('Ctrl Pts',(55.4772707754139,-44.8764124361218,12.));
#59034=CARTESIAN_POINT('Ctrl Pts',(55.4986126378676,-44.8843558012903,0.));
#59035=CARTESIAN_POINT('Ctrl Pts',(55.4986126378676,-44.8843558012903,12.));
#59036=CARTESIAN_POINT('Ctrl Pts',(55.5200048678648,-44.8922935078905,0.));
#59037=CARTESIAN_POINT('Ctrl Pts',(55.5200048678648,-44.8922935078905,12.));
#59038=CARTESIAN_POINT('Ctrl Pts',(55.541447362135,-44.9002254453192,0.));
#59039=CARTESIAN_POINT('Ctrl Pts',(55.541447362135,-44.9002254453192,12.));
#59040=CARTESIAN_POINT('Ctrl Pts',(55.5629400178136,-44.9081515035526,0.));
#59041=CARTESIAN_POINT('Ctrl Pts',(55.5629400178136,-44.9081515035526,12.));
#59042=CARTESIAN_POINT('Ctrl Pts',(55.5844827324315,-44.9160715731425,0.));
#59043=CARTESIAN_POINT('Ctrl Pts',(55.5844827324315,-44.9160715731425,12.));
#59044=CARTESIAN_POINT('Ctrl Pts',(55.6060754039089,-44.9239855452119,0.));
#59045=CARTESIAN_POINT('Ctrl Pts',(55.6060754039089,-44.9239855452119,12.));
#59046=CARTESIAN_POINT('Ctrl Pts',(55.6277179305604,-44.9318933114483,0.));
#59047=CARTESIAN_POINT('Ctrl Pts',(55.6277179305604,-44.9318933114483,12.));
#59048=CARTESIAN_POINT('Ctrl Pts',(55.6494102110922,-44.9397947640996,0.));
#59049=CARTESIAN_POINT('Ctrl Pts',(55.6494102110922,-44.9397947640996,12.));
#59050=CARTESIAN_POINT('Ctrl Pts',(55.671152144599,-44.9476897959694,0.));
#59051=CARTESIAN_POINT('Ctrl Pts',(55.671152144599,-44.9476897959694,12.));
#59052=CARTESIAN_POINT('Ctrl Pts',(55.6929436305522,-44.9555783004133,0.));
#59053=CARTESIAN_POINT('Ctrl Pts',(55.6929436305522,-44.9555783004133,12.));
#59054=CARTESIAN_POINT('Ctrl Pts',(55.7147845687969,-44.9634601713352,0.));
#59055=CARTESIAN_POINT('Ctrl Pts',(55.7147845687969,-44.9634601713352,12.));
#59056=CARTESIAN_POINT('Ctrl Pts',(55.7366748595582,-44.9713353031827,0.));
#59057=CARTESIAN_POINT('Ctrl Pts',(55.7366748595582,-44.9713353031827,12.));
#59058=CARTESIAN_POINT('Ctrl Pts',(55.7586144034376,-44.979203590942,0.));
#59059=CARTESIAN_POINT('Ctrl Pts',(55.7586144034376,-44.979203590942,12.));
#59060=CARTESIAN_POINT('Ctrl Pts',(55.7806031014093,-44.9870649301333,0.));
#59061=CARTESIAN_POINT('Ctrl Pts',(55.7806031014093,-44.9870649301333,12.));
#59062=CARTESIAN_POINT('Ctrl Pts',(55.8026408548078,-44.9949192168073,0.));
#59063=CARTESIAN_POINT('Ctrl Pts',(55.8026408548078,-44.9949192168073,12.));
#59064=CARTESIAN_POINT('Ctrl Pts',(55.8247275653257,-45.002766347541,0.));
#59065=CARTESIAN_POINT('Ctrl Pts',(55.8247275653257,-45.002766347541,12.));
#59066=CARTESIAN_POINT('Ctrl Pts',(55.8468631350195,-45.0106062194325,0.));
#59067=CARTESIAN_POINT('Ctrl Pts',(55.8468631350195,-45.0106062194325,12.));
#59068=CARTESIAN_POINT('Ctrl Pts',(55.8690474663058,-45.0184387300968,0.));
#59069=CARTESIAN_POINT('Ctrl Pts',(55.8690474663058,-45.0184387300968,12.));
#59070=CARTESIAN_POINT('Ctrl Pts',(55.8912804619588,-45.0262637776623,0.));
#59071=CARTESIAN_POINT('Ctrl Pts',(55.8912804619588,-45.0262637776623,12.));
#59072=CARTESIAN_POINT('Ctrl Pts',(55.9135620250977,-45.0340812607676,0.));
#59073=CARTESIAN_POINT('Ctrl Pts',(55.9135620250977,-45.0340812607676,12.));
#59074=CARTESIAN_POINT('Ctrl Pts',(55.9358920591861,-45.041891078557,0.));
#59075=CARTESIAN_POINT('Ctrl Pts',(55.9358920591861,-45.041891078557,12.));
#59076=CARTESIAN_POINT('Ctrl Pts',(55.958270468037,-45.0496931306767,0.));
#59077=CARTESIAN_POINT('Ctrl Pts',(55.958270468037,-45.0496931306767,12.));
#59078=CARTESIAN_POINT('Ctrl Pts',(55.9806971558099,-45.0574873172696,0.));
#59079=CARTESIAN_POINT('Ctrl Pts',(55.9806971558099,-45.0574873172696,12.));
#59080=CARTESIAN_POINT('Ctrl Pts',(56.0031720270074,-45.0652735389729,0.));
#59081=CARTESIAN_POINT('Ctrl Pts',(56.0031720270074,-45.0652735389729,12.));
#59082=CARTESIAN_POINT('Ctrl Pts',(56.025694986463,-45.0730516969142,0.));
#59083=CARTESIAN_POINT('Ctrl Pts',(56.025694986463,-45.0730516969142,12.));
#59084=CARTESIAN_POINT('Ctrl Pts',(56.0482659393412,-45.0808216927082,0.));
#59085=CARTESIAN_POINT('Ctrl Pts',(56.0482659393412,-45.0808216927082,12.));
#59086=CARTESIAN_POINT('Ctrl Pts',(56.070884791141,-45.0885834284513,0.));
#59087=CARTESIAN_POINT('Ctrl Pts',(56.070884791141,-45.0885834284513,12.));
#59088=CARTESIAN_POINT('Ctrl Pts',(56.0935514476945,-45.0963368067177,0.));
#59089=CARTESIAN_POINT('Ctrl Pts',(56.0935514476945,-45.0963368067177,12.));
#59090=CARTESIAN_POINT('Ctrl Pts',(56.1162658151621,-45.1040817305563,0.));
#59091=CARTESIAN_POINT('Ctrl Pts',(56.1162658151621,-45.1040817305563,12.));
#59092=CARTESIAN_POINT('Ctrl Pts',(56.1390278000226,-45.1118181034888,0.));
#59093=CARTESIAN_POINT('Ctrl Pts',(56.1390278000226,-45.1118181034888,12.));
#59094=CARTESIAN_POINT('Ctrl Pts',(56.1618373090729,-45.119545829506,0.));
#59095=CARTESIAN_POINT('Ctrl Pts',(56.1618373090729,-45.119545829506,12.));
#59096=CARTESIAN_POINT('Ctrl Pts',(56.1846942494321,-45.1272648130627,0.));
#59097=CARTESIAN_POINT('Ctrl Pts',(56.1846942494321,-45.1272648130627,12.));
#59098=CARTESIAN_POINT('Ctrl Pts',(56.2075985285391,-45.1349749590736,0.));
#59099=CARTESIAN_POINT('Ctrl Pts',(56.2075985285391,-45.1349749590736,12.));
#59100=CARTESIAN_POINT('Ctrl Pts',(56.2305500541491,-45.1426761729107,0.));
#59101=CARTESIAN_POINT('Ctrl Pts',(56.2305500541491,-45.1426761729107,12.));
#59102=CARTESIAN_POINT('Ctrl Pts',(56.2535487343227,-45.150368360401,0.));
#59103=CARTESIAN_POINT('Ctrl Pts',(56.2535487343227,-45.150368360401,12.));
#59104=CARTESIAN_POINT('Ctrl Pts',(56.2765944774252,-45.158051427823,0.));
#59105=CARTESIAN_POINT('Ctrl Pts',(56.2765944774252,-45.158051427823,12.));
#59106=CARTESIAN_POINT('Ctrl Pts',(56.2996871921321,-45.1657252819018,0.));
#59107=CARTESIAN_POINT('Ctrl Pts',(56.2996871921321,-45.1657252819018,12.));
#59108=CARTESIAN_POINT('Ctrl Pts',(56.3228267874265,-45.1733898298062,0.));
#59109=CARTESIAN_POINT('Ctrl Pts',(56.3228267874265,-45.1733898298062,12.));
#59110=CARTESIAN_POINT('Ctrl Pts',(56.3460131725962,-45.1810449791451,0.));
#59111=CARTESIAN_POINT('Ctrl Pts',(56.3460131725962,-45.1810449791451,12.));
#59112=CARTESIAN_POINT('Ctrl Pts',(56.3692462572228,-45.1886906379664,0.));
#59113=CARTESIAN_POINT('Ctrl Pts',(56.3692462572228,-45.1886906379664,12.));
#59114=CARTESIAN_POINT('Ctrl Pts',(56.3925259511804,-45.1963267147527,0.));
#59115=CARTESIAN_POINT('Ctrl Pts',(56.3925259511804,-45.1963267147527,12.));
#59116=CARTESIAN_POINT('Ctrl Pts',(56.4158521646412,-45.2039531184172,0.));
#59117=CARTESIAN_POINT('Ctrl Pts',(56.4158521646412,-45.2039531184172,12.));
#59118=CARTESIAN_POINT('Ctrl Pts',(56.4392248080733,-45.2115697583002,0.));
#59119=CARTESIAN_POINT('Ctrl Pts',(56.4392248080733,-45.2115697583002,12.));
#59120=CARTESIAN_POINT('Ctrl Pts',(56.4626437922385,-45.2191765441666,0.));
#59121=CARTESIAN_POINT('Ctrl Pts',(56.4626437922385,-45.2191765441666,12.));
#59122=CARTESIAN_POINT('Ctrl Pts',(56.4861090281819,-45.2267733862046,0.));
#59123=CARTESIAN_POINT('Ctrl Pts',(56.4861090281819,-45.2267733862046,12.));
#59124=CARTESIAN_POINT('Ctrl Pts',(56.5096204272299,-45.2343601950222,0.));
#59125=CARTESIAN_POINT('Ctrl Pts',(56.5096204272299,-45.2343601950222,12.));
#59126=CARTESIAN_POINT('Ctrl Pts',(56.533177900995,-45.2419368816424,0.));
#59127=CARTESIAN_POINT('Ctrl Pts',(56.533177900995,-45.2419368816424,12.));
#59128=CARTESIAN_POINT('Ctrl Pts',(56.5567813613752,-45.2495033574997,0.));
#59129=CARTESIAN_POINT('Ctrl Pts',(56.5567813613752,-45.2495033574997,12.));
#59130=CARTESIAN_POINT('Ctrl Pts',(56.5804307205507,-45.2570595344382,0.));
#59131=CARTESIAN_POINT('Ctrl Pts',(56.5804307205507,-45.2570595344382,12.));
#59132=CARTESIAN_POINT('Ctrl Pts',(56.604125890975,-45.2646053247094,0.));
#59133=CARTESIAN_POINT('Ctrl Pts',(56.604125890975,-45.2646053247094,12.));
#59134=CARTESIAN_POINT('Ctrl Pts',(56.6278667853716,-45.2721406409707,0.));
#59135=CARTESIAN_POINT('Ctrl Pts',(56.6278667853716,-45.2721406409707,12.));
#59136=CARTESIAN_POINT('Ctrl Pts',(56.6516533167398,-45.2796653962796,0.));
#59137=CARTESIAN_POINT('Ctrl Pts',(56.6516533167398,-45.2796653962796,12.));
#59138=CARTESIAN_POINT('Ctrl Pts',(56.6754853983535,-45.2871795040912,0.));
#59139=CARTESIAN_POINT('Ctrl Pts',(56.6754853983535,-45.2871795040912,12.));
#59140=CARTESIAN_POINT('Ctrl Pts',(56.6993629437596,-45.2946828782557,0.));
#59141=CARTESIAN_POINT('Ctrl Pts',(56.6993629437596,-45.2946828782557,12.));
#59142=CARTESIAN_POINT('Ctrl Pts',(56.7232858667697,-45.3021754330169,0.));
#59143=CARTESIAN_POINT('Ctrl Pts',(56.7232858667697,-45.3021754330169,12.));
#59144=CARTESIAN_POINT('Ctrl Pts',(56.747254081454,-45.3096570830107,0.));
#59145=CARTESIAN_POINT('Ctrl Pts',(56.747254081454,-45.3096570830107,12.));
#59146=CARTESIAN_POINT('Ctrl Pts',(56.771267502148,-45.3171277432592,0.));
#59147=CARTESIAN_POINT('Ctrl Pts',(56.771267502148,-45.3171277432592,12.));
#59148=CARTESIAN_POINT('Ctrl Pts',(56.7953260434521,-45.3245873291682,0.));
#59149=CARTESIAN_POINT('Ctrl Pts',(56.7953260434521,-45.3245873291682,12.));
#59150=CARTESIAN_POINT('Ctrl Pts',(56.8194296202292,-45.3320357565241,0.));
#59151=CARTESIAN_POINT('Ctrl Pts',(56.8194296202292,-45.3320357565241,12.));
#59152=CARTESIAN_POINT('Ctrl Pts',(56.8435781475982,-45.3394729414932,0.));
#59153=CARTESIAN_POINT('Ctrl Pts',(56.8435781475982,-45.3394729414932,12.));
#59154=CARTESIAN_POINT('Ctrl Pts',(56.8677715409266,-45.3468988006202,0.));
#59155=CARTESIAN_POINT('Ctrl Pts',(56.8677715409266,-45.3468988006202,12.));
#59156=CARTESIAN_POINT('Ctrl Pts',(56.8920097158371,-45.3543132508234,0.));
#59157=CARTESIAN_POINT('Ctrl Pts',(56.8920097158371,-45.3543132508234,12.));
#59158=CARTESIAN_POINT('Ctrl Pts',(56.916292588208,-45.3617162093918,0.));
#59159=CARTESIAN_POINT('Ctrl Pts',(56.916292588208,-45.3617162093918,12.));
#59160=CARTESIAN_POINT('Ctrl Pts',(56.9406200741714,-45.3691075939827,0.));
#59161=CARTESIAN_POINT('Ctrl Pts',(56.9406200741714,-45.3691075939827,12.));
#59162=CARTESIAN_POINT('Ctrl Pts',(56.9649920901079,-45.3764873226202,0.));
#59163=CARTESIAN_POINT('Ctrl Pts',(56.9649920901079,-45.3764873226202,12.));
#59164=CARTESIAN_POINT('Ctrl Pts',(56.9894085526383,-45.3838553136957,0.));
#59165=CARTESIAN_POINT('Ctrl Pts',(56.9894085526383,-45.3838553136957,12.));
#59166=CARTESIAN_POINT('Ctrl Pts',(57.0138693786287,-45.3912114859625,0.));
#59167=CARTESIAN_POINT('Ctrl Pts',(57.0138693786287,-45.3912114859625,12.));
#59168=CARTESIAN_POINT('Ctrl Pts',(57.0383744851917,-45.3985557585316,0.));
#59169=CARTESIAN_POINT('Ctrl Pts',(57.0383744851917,-45.3985557585316,12.));
#59170=CARTESIAN_POINT('Ctrl Pts',(57.0629237896848,-45.4058880508693,0.));
#59171=CARTESIAN_POINT('Ctrl Pts',(57.0629237896848,-45.4058880508693,12.));
#59172=CARTESIAN_POINT('Ctrl Pts',(57.0875172097048,-45.4132082827945,0.));
#59173=CARTESIAN_POINT('Ctrl Pts',(57.0875172097048,-45.4132082827945,12.));
#59174=CARTESIAN_POINT('Ctrl Pts',(57.1121546630776,-45.4205163744778,0.));
#59175=CARTESIAN_POINT('Ctrl Pts',(57.1121546630776,-45.4205163744778,12.));
#59176=CARTESIAN_POINT('Ctrl Pts',(57.1368360678629,-45.4278122464387,0.));
#59177=CARTESIAN_POINT('Ctrl Pts',(57.1368360678629,-45.4278122464387,12.));
#59178=CARTESIAN_POINT('Ctrl Pts',(57.1615613423586,-45.4350958195434,0.));
#59179=CARTESIAN_POINT('Ctrl Pts',(57.1615613423586,-45.4350958195434,12.));
#59180=CARTESIAN_POINT('Ctrl Pts',(57.1863304051011,-45.4423670150035,0.));
#59181=CARTESIAN_POINT('Ctrl Pts',(57.1863304051011,-45.4423670150035,12.));
#59182=CARTESIAN_POINT('Ctrl Pts',(57.2111431748629,-45.4496257543759,0.));
#59183=CARTESIAN_POINT('Ctrl Pts',(57.2111431748629,-45.4496257543759,12.));
#59184=CARTESIAN_POINT('Ctrl Pts',(57.2359995706441,-45.4568719595639,0.));
#59185=CARTESIAN_POINT('Ctrl Pts',(57.2359995706441,-45.4568719595639,12.));
#59186=CARTESIAN_POINT('Ctrl Pts',(57.2608995116727,-45.4641055528138,0.));
#59187=CARTESIAN_POINT('Ctrl Pts',(57.2608995116727,-45.4641055528138,12.));
#59188=CARTESIAN_POINT('Ctrl Pts',(57.2858429174056,-45.4713264567059,0.));
#59189=CARTESIAN_POINT('Ctrl Pts',(57.2858429174056,-45.4713264567059,12.));
#59190=CARTESIAN_POINT('Ctrl Pts',(57.3108297075262,-45.4785345941506,0.));
#59191=CARTESIAN_POINT('Ctrl Pts',(57.3108297075262,-45.4785345941506,12.));
#59192=CARTESIAN_POINT('Ctrl Pts',(57.335859801939,-45.4857298883826,0.));
#59193=CARTESIAN_POINT('Ctrl Pts',(57.335859801939,-45.4857298883826,12.));
#59194=CARTESIAN_POINT('Ctrl Pts',(57.360933120758,-45.4929122629576,0.));
#59195=CARTESIAN_POINT('Ctrl Pts',(57.360933120758,-45.4929122629576,12.));
#59196=CARTESIAN_POINT('Ctrl Pts',(57.3860495843043,-45.5000816417516,0.));
#59197=CARTESIAN_POINT('Ctrl Pts',(57.3860495843043,-45.5000816417516,12.));
#59198=CARTESIAN_POINT('Ctrl Pts',(57.4112091131193,-45.5072379489637,0.));
#59199=CARTESIAN_POINT('Ctrl Pts',(57.4112091131193,-45.5072379489637,12.));
#59200=CARTESIAN_POINT('Ctrl Pts',(57.4364116279708,-45.5143811091209,0.));
#59201=CARTESIAN_POINT('Ctrl Pts',(57.4364116279708,-45.5143811091209,12.));
#59202=CARTESIAN_POINT('Ctrl Pts',(57.4616570498566,-45.5215110470825,0.));
#59203=CARTESIAN_POINT('Ctrl Pts',(57.4616570498566,-45.5215110470825,12.));
#59204=CARTESIAN_POINT('Ctrl Pts',(57.4869453000055,-45.5286276880479,0.));
#59205=CARTESIAN_POINT('Ctrl Pts',(57.4869453000055,-45.5286276880479,12.));
#59206=CARTESIAN_POINT('Ctrl Pts',(57.5122762998732,-45.5357309575603,0.));
#59207=CARTESIAN_POINT('Ctrl Pts',(57.5122762998732,-45.5357309575603,12.));
#59208=CARTESIAN_POINT('Ctrl Pts',(57.5376499711338,-45.5428207814832,0.));
#59209=CARTESIAN_POINT('Ctrl Pts',(57.5376499711338,-45.5428207814832,12.));
#59210=CARTESIAN_POINT('Ctrl Pts',(57.5630662356671,-45.5498970859829,0.));
#59211=CARTESIAN_POINT('Ctrl Pts',(57.5630662356671,-45.5498970859829,12.));
#59212=CARTESIAN_POINT('Ctrl Pts',(57.5885250155432,-45.5569597975096,0.));
#59213=CARTESIAN_POINT('Ctrl Pts',(57.5885250155432,-45.5569597975096,12.));
#59214=CARTESIAN_POINT('Ctrl Pts',(57.6140262330048,-45.5640088427819,0.));
#59215=CARTESIAN_POINT('Ctrl Pts',(57.6140262330048,-45.5640088427819,12.));
#59216=CARTESIAN_POINT('Ctrl Pts',(57.6395698104416,-45.5710441487683,0.));
#59217=CARTESIAN_POINT('Ctrl Pts',(57.6395698104416,-45.5710441487683,12.));
#59218=CARTESIAN_POINT('Ctrl Pts',(57.6651556704249,-45.5780656427173,0.));
#59219=CARTESIAN_POINT('Ctrl Pts',(57.6651556704249,-45.5780656427173,12.));
#59220=CARTESIAN_POINT('Ctrl Pts',(57.6907837357425,-45.5850732521902,0.));
#59221=CARTESIAN_POINT('Ctrl Pts',(57.6907837357425,-45.5850732521902,12.));
#59222=CARTESIAN_POINT('Ctrl Pts',(57.7164539294316,-45.5920669050988,0.));
#59223=CARTESIAN_POINT('Ctrl Pts',(57.7164539294316,-45.5920669050988,12.));
#59224=CARTESIAN_POINT('Ctrl Pts',(57.7421661748021,-45.5990465297341,0.));
#59225=CARTESIAN_POINT('Ctrl Pts',(57.7421661748021,-45.5990465297341,12.));
#59226=CARTESIAN_POINT('Ctrl Pts',(57.7679203954735,-45.6060120548199,0.));
#59227=CARTESIAN_POINT('Ctrl Pts',(57.7679203954735,-45.6060120548199,12.));
#59228=CARTESIAN_POINT('Ctrl Pts',(57.7937165153379,-45.6129634094678,0.));
#59229=CARTESIAN_POINT('Ctrl Pts',(57.7937165153379,-45.6129634094678,12.));
#59230=CARTESIAN_POINT('Ctrl Pts',(57.819554458484,-45.619900523078,0.));
#59231=CARTESIAN_POINT('Ctrl Pts',(57.819554458484,-45.619900523078,12.));
#59232=CARTESIAN_POINT('Ctrl Pts',(57.8454341491236,-45.6268233252543,0.));
#59233=CARTESIAN_POINT('Ctrl Pts',(57.8454341491236,-45.6268233252543,12.));
#59234=CARTESIAN_POINT('Ctrl Pts',(57.8713555115232,-45.6337317457253,0.));
#59235=CARTESIAN_POINT('Ctrl Pts',(57.8713555115232,-45.6337317457253,12.));
#59236=CARTESIAN_POINT('Ctrl Pts',(57.8973184699037,-45.6406257142385,0.));
#59237=CARTESIAN_POINT('Ctrl Pts',(57.8973184699037,-45.6406257142385,12.));
#59238=CARTESIAN_POINT('Ctrl Pts',(57.923322948432,-45.6475051605542,0.));
#59239=CARTESIAN_POINT('Ctrl Pts',(57.923322948432,-45.6475051605542,12.));
#59240=CARTESIAN_POINT('Ctrl Pts',(57.9493688714249,-45.6543700146689,0.));
#59241=CARTESIAN_POINT('Ctrl Pts',(57.9493688714249,-45.6543700146689,12.));
#59242=CARTESIAN_POINT('Ctrl Pts',(57.975456163507,-45.6612202069928,0.));
#59243=CARTESIAN_POINT('Ctrl Pts',(57.975456163507,-45.6612202069928,12.));
#59244=CARTESIAN_POINT('Ctrl Pts',(58.0015847497838,-45.6680556685494,0.));
#59245=CARTESIAN_POINT('Ctrl Pts',(58.0015847497838,-45.6680556685494,12.));
#59246=CARTESIAN_POINT('Ctrl Pts',(58.0277545560001,-45.6748763311635,0.));
#59247=CARTESIAN_POINT('Ctrl Pts',(58.0277545560001,-45.6748763311635,12.));
#59248=CARTESIAN_POINT('Ctrl Pts',(58.0539655087095,-45.6816821276662,0.));
#59249=CARTESIAN_POINT('Ctrl Pts',(58.0539655087095,-45.6816821276662,12.));
#59250=CARTESIAN_POINT('Ctrl Pts',(58.0802175348939,-45.6884729914465,0.));
#59251=CARTESIAN_POINT('Ctrl Pts',(58.0802175348939,-45.6884729914465,12.));
#59252=CARTESIAN_POINT('Ctrl Pts',(58.1065105615884,-45.6952488560134,0.));
#59253=CARTESIAN_POINT('Ctrl Pts',(58.1065105615884,-45.6952488560134,12.));
#59254=CARTESIAN_POINT('Ctrl Pts',(58.1328445154667,-45.7020096545174,0.));
#59255=CARTESIAN_POINT('Ctrl Pts',(58.1328445154667,-45.7020096545174,12.));
#59256=CARTESIAN_POINT('Ctrl Pts',(58.159219322515,-45.708755319378,0.));
#59257=CARTESIAN_POINT('Ctrl Pts',(58.159219322515,-45.708755319378,12.));
#59258=CARTESIAN_POINT('Ctrl Pts',(58.1856349074723,-45.7154857816507,0.));
#59259=CARTESIAN_POINT('Ctrl Pts',(58.1856349074723,-45.7154857816507,12.));
#59260=CARTESIAN_POINT('Ctrl Pts',(58.2120911942819,-45.7222009715431,0.));
#59261=CARTESIAN_POINT('Ctrl Pts',(58.2120911942819,-45.7222009715431,12.));
#59262=CARTESIAN_POINT('Ctrl Pts',(58.2385881070959,-45.7289008195612,0.));
#59263=CARTESIAN_POINT('Ctrl Pts',(58.2385881070959,-45.7289008195612,12.));
#59264=CARTESIAN_POINT('Ctrl Pts',(58.2651255711481,-45.7355852575127,0.));
#59265=CARTESIAN_POINT('Ctrl Pts',(58.2651255711481,-45.7355852575127,12.));
#59266=CARTESIAN_POINT('Ctrl Pts',(58.2917035135833,-45.7422542194625,0.));
#59267=CARTESIAN_POINT('Ctrl Pts',(58.2917035135833,-45.7422542194625,12.));
#59268=CARTESIAN_POINT('Ctrl Pts',(58.3183218645265,-45.7489076429725,0.));
#59269=CARTESIAN_POINT('Ctrl Pts',(58.3183218645265,-45.7489076429725,12.));
#59270=CARTESIAN_POINT('Ctrl Pts',(58.3449805573335,-45.7555454693956,0.));
#59271=CARTESIAN_POINT('Ctrl Pts',(58.3449805573335,-45.7555454693956,12.));
#59272=CARTESIAN_POINT('Ctrl Pts',(58.3716795262251,-45.7621676411361,0.));
#59273=CARTESIAN_POINT('Ctrl Pts',(58.3716795262251,-45.7621676411361,12.));
#59274=CARTESIAN_POINT('Ctrl Pts',(58.3984187044166,-45.76877409949,0.));
#59275=CARTESIAN_POINT('Ctrl Pts',(58.3984187044166,-45.76877409949,12.));
#59276=CARTESIAN_POINT('Ctrl Pts',(58.4251980219532,-45.77536478215,0.));
#59277=CARTESIAN_POINT('Ctrl Pts',(58.4251980219532,-45.77536478215,12.));
#59278=CARTESIAN_POINT('Ctrl Pts',(58.4520174038836,-45.7819396211062,0.));
#59279=CARTESIAN_POINT('Ctrl Pts',(58.4520174038836,-45.7819396211062,12.));
#59280=CARTESIAN_POINT('Ctrl Pts',(58.4788767677114,-45.7884985397138,0.));
#59281=CARTESIAN_POINT('Ctrl Pts',(58.4788767677114,-45.7884985397138,12.));
#59282=CARTESIAN_POINT('Ctrl Pts',(58.5057760270406,-45.7950414569431,0.));
#59283=CARTESIAN_POINT('Ctrl Pts',(58.5057760270406,-45.7950414569431,12.));
#59284=CARTESIAN_POINT('Ctrl Pts',(58.5327150960874,-45.801568292618,0.));
#59285=CARTESIAN_POINT('Ctrl Pts',(58.5327150960874,-45.801568292618,12.));
#59286=CARTESIAN_POINT('Ctrl Pts',(58.5596938940308,-45.8080789725167,0.));
#59287=CARTESIAN_POINT('Ctrl Pts',(58.5596938940308,-45.8080789725167,12.));
#59288=CARTESIAN_POINT('Ctrl Pts',(58.5867123490943,-45.8145734330666,0.));
#59289=CARTESIAN_POINT('Ctrl Pts',(58.5867123490943,-45.8145734330666,12.));
#59290=CARTESIAN_POINT('Ctrl Pts',(58.6137704035561,-45.8210516273556,0.));
#59291=CARTESIAN_POINT('Ctrl Pts',(58.6137704035561,-45.8210516273556,12.));
#59292=CARTESIAN_POINT('Ctrl Pts',(58.64086801535,-45.8275135263874,0.));
#59293=CARTESIAN_POINT('Ctrl Pts',(58.64086801535,-45.8275135263874,12.));
#59294=CARTESIAN_POINT('Ctrl Pts',(58.668005155216,-45.8339591141396,0.));
#59295=CARTESIAN_POINT('Ctrl Pts',(58.668005155216,-45.8339591141396,12.));
#59296=CARTESIAN_POINT('Ctrl Pts',(58.6897464750196,-45.8391025301766,0.));
#59297=CARTESIAN_POINT('Ctrl Pts',(58.6897464750196,-45.8391025301766,12.));
#59298=CARTESIAN_POINT('Ctrl Pts',(58.7060702401382,-45.8429527488565,0.));
#59299=CARTESIAN_POINT('Ctrl Pts',(58.7060702401382,-45.8429527488565,12.));
#59300=CARTESIAN_POINT('Ctrl Pts',(58.7169606500157,-45.8455162977347,0.));
#59301=CARTESIAN_POINT('Ctrl Pts',(58.7169606500157,-45.8455162977347,12.));
#59302=CARTESIAN_POINT('Ctrl Pts',(58.722407829904,-45.8467972562798,0.));
#59303=CARTESIAN_POINT('Ctrl Pts',(58.722407829904,-45.8467972562798,12.));
#59304=CARTESIAN_POINT('',(54.1679505278134,-44.3377168516418,0.));
#59305=CARTESIAN_POINT('Ctrl Pts',(54.1679505278134,-44.3377168516418,0.));
#59306=CARTESIAN_POINT('Ctrl Pts',(54.1714861895278,-44.3393235891014,0.));
#59307=CARTESIAN_POINT('Ctrl Pts',(54.1785633257456,-44.3425373700829,0.));
#59308=CARTESIAN_POINT('Ctrl Pts',(54.1891964684439,-44.3473589597468,0.));
#59309=CARTESIAN_POINT('Ctrl Pts',(54.203408870162,-44.3537895823819,0.));
#59310=CARTESIAN_POINT('Ctrl Pts',(54.2212325005847,-44.3618309103245,0.));
#59311=CARTESIAN_POINT('Ctrl Pts',(54.2391142386354,-44.369875253351,0.));
#59312=CARTESIAN_POINT('Ctrl Pts',(54.2570540336536,-44.3779225430461,0.));
#59313=CARTESIAN_POINT('Ctrl Pts',(54.2750517888695,-44.3859726620288,0.));
#59314=CARTESIAN_POINT('Ctrl Pts',(54.2931073621661,-44.3940254456427,0.));
#59315=CARTESIAN_POINT('Ctrl Pts',(54.3112205860776,-44.4020807028144,0.));
#59316=CARTESIAN_POINT('Ctrl Pts',(54.3293912830237,-44.4101382321834,0.));
#59317=CARTESIAN_POINT('Ctrl Pts',(54.347619281931,-44.4181978395814,0.));
#59318=CARTESIAN_POINT('Ctrl Pts',(54.3659044357064,-44.4262593564664,0.));
#59319=CARTESIAN_POINT('Ctrl Pts',(54.3842466156151,-44.4343226339555,0.));
#59320=CARTESIAN_POINT('Ctrl Pts',(54.4026457030316,-44.442387534098,0.));
#59321=CARTESIAN_POINT('Ctrl Pts',(54.4211015825959,-44.4504539226336,0.));
#59322=CARTESIAN_POINT('Ctrl Pts',(54.4396141337008,-44.4585216599933,0.));
#59323=CARTESIAN_POINT('Ctrl Pts',(54.4581832262072,-44.4665905967701,0.));
#59324=CARTESIAN_POINT('Ctrl Pts',(54.4768087248854,-44.4746605784056,0.));
#59325=CARTESIAN_POINT('Ctrl Pts',(54.4954904921938,-44.4827314481271,0.));
#59326=CARTESIAN_POINT('Ctrl Pts',(54.5142283914684,-44.4908030503209,0.));
#59327=CARTESIAN_POINT('Ctrl Pts',(54.5330222905438,-44.4988752343715,0.));
#59328=CARTESIAN_POINT('Ctrl Pts',(54.5518720616016,-44.5069478544945,0.));
#59329=CARTESIAN_POINT('Ctrl Pts',(54.5707775794412,-44.5150207678988,0.));
#59330=CARTESIAN_POINT('Ctrl Pts',(54.5897387202815,-44.5230938335167,0.));
#59331=CARTESIAN_POINT('Ctrl Pts',(54.6087553602914,-44.5311669104515,0.));
#59332=CARTESIAN_POINT('Ctrl Pts',(54.6278273743587,-44.5392398566802,0.));
#59333=CARTESIAN_POINT('Ctrl Pts',(54.6469546367408,-44.5473125297312,0.));
#59334=CARTESIAN_POINT('Ctrl Pts',(54.6661370216252,-44.5553847872721,0.));
#59335=CARTESIAN_POINT('Ctrl Pts',(54.6853744036751,-44.5634564876863,0.));
#59336=CARTESIAN_POINT('Ctrl Pts',(54.7046666586754,-44.5715274907619,0.));
#59337=CARTESIAN_POINT('Ctrl Pts',(54.7240136637717,-44.5795976579454,0.));
#59338=CARTESIAN_POINT('Ctrl Pts',(54.7434152971267,-44.5876668519661,0.));
#59339=CARTESIAN_POINT('Ctrl Pts',(54.7628714377037,-44.5957349366059,0.));
#59340=CARTESIAN_POINT('Ctrl Pts',(54.7823819650148,-44.603801776431,0.));
#59341=CARTESIAN_POINT('Ctrl Pts',(54.8019467588278,-44.6118672364906,0.));
#59342=CARTESIAN_POINT('Ctrl Pts',(54.8215656991837,-44.6199311823293,0.));
#59343=CARTESIAN_POINT('Ctrl Pts',(54.8412386665276,-44.6279934801169,0.));
#59344=CARTESIAN_POINT('Ctrl Pts',(54.860965541796,-44.6360539967392,0.));
#59345=CARTESIAN_POINT('Ctrl Pts',(54.8807462065164,-44.6441125999063,0.));
#59346=CARTESIAN_POINT('Ctrl Pts',(54.9005805428969,-44.6521691582534,0.));
#59347=CARTESIAN_POINT('Ctrl Pts',(54.9204684337822,-44.6602235412836,0.));
#59348=CARTESIAN_POINT('Ctrl Pts',(54.9404097626077,-44.6682756193147,0.));
#59349=CARTESIAN_POINT('Ctrl Pts',(54.9604044133501,-44.6763252634259,0.));
#59350=CARTESIAN_POINT('Ctrl Pts',(54.9804522704686,-44.6843723454,0.));
#59351=CARTESIAN_POINT('Ctrl Pts',(55.0005532188667,-44.6924167376869,0.));
#59352=CARTESIAN_POINT('Ctrl Pts',(55.0207071439237,-44.7004583134249,0.));
#59353=CARTESIAN_POINT('Ctrl Pts',(55.0409139315078,-44.7084969464513,0.));
#59354=CARTESIAN_POINT('Ctrl Pts',(55.0611734679894,-44.716532511316,0.));
#59355=CARTESIAN_POINT('Ctrl Pts',(55.0814856402495,-44.7245648832979,0.));
#59356=CARTESIAN_POINT('Ctrl Pts',(55.1018503356795,-44.7325939384035,0.));
#59357=CARTESIAN_POINT('Ctrl Pts',(55.1222674421743,-44.740619553348,0.));
#59358=CARTESIAN_POINT('Ctrl Pts',(55.14273684812,-44.748641605542,0.));
#59359=CARTESIAN_POINT('Ctrl Pts',(55.1632584423815,-44.7566599730773,0.));
#59360=CARTESIAN_POINT('Ctrl Pts',(55.1838321142779,-44.7646745347109,0.));
#59361=CARTESIAN_POINT('Ctrl Pts',(55.2044577535866,-44.7726851698619,0.));
#59362=CARTESIAN_POINT('Ctrl Pts',(55.2251352505475,-44.7806917586077,0.));
#59363=CARTESIAN_POINT('Ctrl Pts',(55.2458644958617,-44.7886941816823,0.));
#59364=CARTESIAN_POINT('Ctrl Pts',(55.2666453806882,-44.7966923204741,0.));
#59365=CARTESIAN_POINT('Ctrl Pts',(55.2874777966349,-44.8046860570245,0.));
#59366=CARTESIAN_POINT('Ctrl Pts',(55.3083616357605,-44.812675274021,0.));
#59367=CARTESIAN_POINT('Ctrl Pts',(55.3292967905725,-44.8206598547889,0.));
#59368=CARTESIAN_POINT('Ctrl Pts',(55.3502831540229,-44.8286396832849,0.));
#59369=CARTESIAN_POINT('Ctrl Pts',(55.3713206194962,-44.8366146440896,0.));
#59370=CARTESIAN_POINT('Ctrl Pts',(55.3924090808002,-44.8445846224034,0.));
#59371=CARTESIAN_POINT('Ctrl Pts',(55.4135484321706,-44.8525495040398,0.));
#59372=CARTESIAN_POINT('Ctrl Pts',(55.4347385682697,-44.8605091754208,0.));
#59373=CARTESIAN_POINT('Ctrl Pts',(55.4559793841838,-44.8684635235727,0.));
#59374=CARTESIAN_POINT('Ctrl Pts',(55.4772707754139,-44.8764124361218,0.));
#59375=CARTESIAN_POINT('Ctrl Pts',(55.4986126378676,-44.8843558012903,0.));
#59376=CARTESIAN_POINT('Ctrl Pts',(55.5200048678648,-44.8922935078905,0.));
#59377=CARTESIAN_POINT('Ctrl Pts',(55.541447362135,-44.9002254453192,0.));
#59378=CARTESIAN_POINT('Ctrl Pts',(55.5629400178136,-44.9081515035526,0.));
#59379=CARTESIAN_POINT('Ctrl Pts',(55.5844827324315,-44.9160715731425,0.));
#59380=CARTESIAN_POINT('Ctrl Pts',(55.6060754039089,-44.9239855452119,0.));
#59381=CARTESIAN_POINT('Ctrl Pts',(55.6277179305604,-44.9318933114483,0.));
#59382=CARTESIAN_POINT('Ctrl Pts',(55.6494102110922,-44.9397947640996,0.));
#59383=CARTESIAN_POINT('Ctrl Pts',(55.671152144599,-44.9476897959694,0.));
#59384=CARTESIAN_POINT('Ctrl Pts',(55.6929436305522,-44.9555783004133,0.));
#59385=CARTESIAN_POINT('Ctrl Pts',(55.7147845687969,-44.9634601713352,0.));
#59386=CARTESIAN_POINT('Ctrl Pts',(55.7366748595582,-44.9713353031827,0.));
#59387=CARTESIAN_POINT('Ctrl Pts',(55.7586144034376,-44.979203590942,0.));
#59388=CARTESIAN_POINT('Ctrl Pts',(55.7806031014093,-44.9870649301333,0.));
#59389=CARTESIAN_POINT('Ctrl Pts',(55.8026408548078,-44.9949192168073,0.));
#59390=CARTESIAN_POINT('Ctrl Pts',(55.8247275653257,-45.002766347541,0.));
#59391=CARTESIAN_POINT('Ctrl Pts',(55.8468631350195,-45.0106062194325,0.));
#59392=CARTESIAN_POINT('Ctrl Pts',(55.8690474663058,-45.0184387300968,0.));
#59393=CARTESIAN_POINT('Ctrl Pts',(55.8912804619588,-45.0262637776623,0.));
#59394=CARTESIAN_POINT('Ctrl Pts',(55.9135620250977,-45.0340812607676,0.));
#59395=CARTESIAN_POINT('Ctrl Pts',(55.9358920591861,-45.041891078557,0.));
#59396=CARTESIAN_POINT('Ctrl Pts',(55.958270468037,-45.0496931306767,0.));
#59397=CARTESIAN_POINT('Ctrl Pts',(55.9806971558099,-45.0574873172696,0.));
#59398=CARTESIAN_POINT('Ctrl Pts',(56.0031720270074,-45.0652735389729,0.));
#59399=CARTESIAN_POINT('Ctrl Pts',(56.025694986463,-45.0730516969142,0.));
#59400=CARTESIAN_POINT('Ctrl Pts',(56.0482659393412,-45.0808216927082,0.));
#59401=CARTESIAN_POINT('Ctrl Pts',(56.070884791141,-45.0885834284513,0.));
#59402=CARTESIAN_POINT('Ctrl Pts',(56.0935514476945,-45.0963368067177,0.));
#59403=CARTESIAN_POINT('Ctrl Pts',(56.1162658151621,-45.1040817305563,0.));
#59404=CARTESIAN_POINT('Ctrl Pts',(56.1390278000226,-45.1118181034888,0.));
#59405=CARTESIAN_POINT('Ctrl Pts',(56.1618373090729,-45.119545829506,0.));
#59406=CARTESIAN_POINT('Ctrl Pts',(56.1846942494321,-45.1272648130627,0.));
#59407=CARTESIAN_POINT('Ctrl Pts',(56.2075985285391,-45.1349749590736,0.));
#59408=CARTESIAN_POINT('Ctrl Pts',(56.2305500541491,-45.1426761729107,0.));
#59409=CARTESIAN_POINT('Ctrl Pts',(56.2535487343227,-45.150368360401,0.));
#59410=CARTESIAN_POINT('Ctrl Pts',(56.2765944774252,-45.158051427823,0.));
#59411=CARTESIAN_POINT('Ctrl Pts',(56.2996871921321,-45.1657252819018,0.));
#59412=CARTESIAN_POINT('Ctrl Pts',(56.3228267874265,-45.1733898298062,0.));
#59413=CARTESIAN_POINT('Ctrl Pts',(56.3460131725962,-45.1810449791451,0.));
#59414=CARTESIAN_POINT('Ctrl Pts',(56.3692462572228,-45.1886906379664,0.));
#59415=CARTESIAN_POINT('Ctrl Pts',(56.3925259511804,-45.1963267147527,0.));
#59416=CARTESIAN_POINT('Ctrl Pts',(56.4158521646412,-45.2039531184172,0.));
#59417=CARTESIAN_POINT('Ctrl Pts',(56.4392248080733,-45.2115697583002,0.));
#59418=CARTESIAN_POINT('Ctrl Pts',(56.4626437922385,-45.2191765441666,0.));
#59419=CARTESIAN_POINT('Ctrl Pts',(56.4861090281819,-45.2267733862046,0.));
#59420=CARTESIAN_POINT('Ctrl Pts',(56.5096204272299,-45.2343601950222,0.));
#59421=CARTESIAN_POINT('Ctrl Pts',(56.533177900995,-45.2419368816424,0.));
#59422=CARTESIAN_POINT('Ctrl Pts',(56.5567813613752,-45.2495033574997,0.));
#59423=CARTESIAN_POINT('Ctrl Pts',(56.5804307205507,-45.2570595344382,0.));
#59424=CARTESIAN_POINT('Ctrl Pts',(56.604125890975,-45.2646053247094,0.));
#59425=CARTESIAN_POINT('Ctrl Pts',(56.6278667853716,-45.2721406409707,0.));
#59426=CARTESIAN_POINT('Ctrl Pts',(56.6516533167398,-45.2796653962796,0.));
#59427=CARTESIAN_POINT('Ctrl Pts',(56.6754853983535,-45.2871795040912,0.));
#59428=CARTESIAN_POINT('Ctrl Pts',(56.6993629437596,-45.2946828782557,0.));
#59429=CARTESIAN_POINT('Ctrl Pts',(56.7232858667697,-45.3021754330169,0.));
#59430=CARTESIAN_POINT('Ctrl Pts',(56.747254081454,-45.3096570830107,0.));
#59431=CARTESIAN_POINT('Ctrl Pts',(56.771267502148,-45.3171277432592,0.));
#59432=CARTESIAN_POINT('Ctrl Pts',(56.7953260434521,-45.3245873291682,0.));
#59433=CARTESIAN_POINT('Ctrl Pts',(56.8194296202292,-45.3320357565241,0.));
#59434=CARTESIAN_POINT('Ctrl Pts',(56.8435781475982,-45.3394729414932,0.));
#59435=CARTESIAN_POINT('Ctrl Pts',(56.8677715409266,-45.3468988006202,0.));
#59436=CARTESIAN_POINT('Ctrl Pts',(56.8920097158371,-45.3543132508234,0.));
#59437=CARTESIAN_POINT('Ctrl Pts',(56.916292588208,-45.3617162093918,0.));
#59438=CARTESIAN_POINT('Ctrl Pts',(56.9406200741714,-45.3691075939827,0.));
#59439=CARTESIAN_POINT('Ctrl Pts',(56.9649920901079,-45.3764873226202,0.));
#59440=CARTESIAN_POINT('Ctrl Pts',(56.9894085526383,-45.3838553136957,0.));
#59441=CARTESIAN_POINT('Ctrl Pts',(57.0138693786287,-45.3912114859625,0.));
#59442=CARTESIAN_POINT('Ctrl Pts',(57.0383744851917,-45.3985557585316,0.));
#59443=CARTESIAN_POINT('Ctrl Pts',(57.0629237896848,-45.4058880508693,0.));
#59444=CARTESIAN_POINT('Ctrl Pts',(57.0875172097048,-45.4132082827945,0.));
#59445=CARTESIAN_POINT('Ctrl Pts',(57.1121546630776,-45.4205163744778,0.));
#59446=CARTESIAN_POINT('Ctrl Pts',(57.1368360678629,-45.4278122464387,0.));
#59447=CARTESIAN_POINT('Ctrl Pts',(57.1615613423586,-45.4350958195434,0.));
#59448=CARTESIAN_POINT('Ctrl Pts',(57.1863304051011,-45.4423670150035,0.));
#59449=CARTESIAN_POINT('Ctrl Pts',(57.2111431748629,-45.4496257543759,0.));
#59450=CARTESIAN_POINT('Ctrl Pts',(57.2359995706441,-45.4568719595639,0.));
#59451=CARTESIAN_POINT('Ctrl Pts',(57.2608995116727,-45.4641055528138,0.));
#59452=CARTESIAN_POINT('Ctrl Pts',(57.2858429174056,-45.4713264567059,0.));
#59453=CARTESIAN_POINT('Ctrl Pts',(57.3108297075262,-45.4785345941506,0.));
#59454=CARTESIAN_POINT('Ctrl Pts',(57.335859801939,-45.4857298883826,0.));
#59455=CARTESIAN_POINT('Ctrl Pts',(57.360933120758,-45.4929122629576,0.));
#59456=CARTESIAN_POINT('Ctrl Pts',(57.3860495843043,-45.5000816417516,0.));
#59457=CARTESIAN_POINT('Ctrl Pts',(57.4112091131193,-45.5072379489637,0.));
#59458=CARTESIAN_POINT('Ctrl Pts',(57.4364116279708,-45.5143811091209,0.));
#59459=CARTESIAN_POINT('Ctrl Pts',(57.4616570498566,-45.5215110470825,0.));
#59460=CARTESIAN_POINT('Ctrl Pts',(57.4869453000055,-45.5286276880479,0.));
#59461=CARTESIAN_POINT('Ctrl Pts',(57.5122762998732,-45.5357309575603,0.));
#59462=CARTESIAN_POINT('Ctrl Pts',(57.5376499711338,-45.5428207814832,0.));
#59463=CARTESIAN_POINT('Ctrl Pts',(57.5630662356671,-45.5498970859829,0.));
#59464=CARTESIAN_POINT('Ctrl Pts',(57.5885250155432,-45.5569597975096,0.));
#59465=CARTESIAN_POINT('Ctrl Pts',(57.6140262330048,-45.5640088427819,0.));
#59466=CARTESIAN_POINT('Ctrl Pts',(57.6395698104416,-45.5710441487683,0.));
#59467=CARTESIAN_POINT('Ctrl Pts',(57.6651556704249,-45.5780656427173,0.));
#59468=CARTESIAN_POINT('Ctrl Pts',(57.6907837357425,-45.5850732521902,0.));
#59469=CARTESIAN_POINT('Ctrl Pts',(57.7164539294316,-45.5920669050988,0.));
#59470=CARTESIAN_POINT('Ctrl Pts',(57.7421661748021,-45.5990465297341,0.));
#59471=CARTESIAN_POINT('Ctrl Pts',(57.7679203954735,-45.6060120548199,0.));
#59472=CARTESIAN_POINT('Ctrl Pts',(57.7937165153379,-45.6129634094678,0.));
#59473=CARTESIAN_POINT('Ctrl Pts',(57.819554458484,-45.619900523078,0.));
#59474=CARTESIAN_POINT('Ctrl Pts',(57.8454341491236,-45.6268233252543,0.));
#59475=CARTESIAN_POINT('Ctrl Pts',(57.8713555115232,-45.6337317457253,0.));
#59476=CARTESIAN_POINT('Ctrl Pts',(57.8973184699037,-45.6406257142385,0.));
#59477=CARTESIAN_POINT('Ctrl Pts',(57.923322948432,-45.6475051605542,0.));
#59478=CARTESIAN_POINT('Ctrl Pts',(57.9493688714249,-45.6543700146689,0.));
#59479=CARTESIAN_POINT('Ctrl Pts',(57.975456163507,-45.6612202069928,0.));
#59480=CARTESIAN_POINT('Ctrl Pts',(58.0015847497838,-45.6680556685494,0.));
#59481=CARTESIAN_POINT('Ctrl Pts',(58.0277545560001,-45.6748763311635,0.));
#59482=CARTESIAN_POINT('Ctrl Pts',(58.0539655087095,-45.6816821276662,0.));
#59483=CARTESIAN_POINT('Ctrl Pts',(58.0802175348939,-45.6884729914465,0.));
#59484=CARTESIAN_POINT('Ctrl Pts',(58.1065105615884,-45.6952488560134,0.));
#59485=CARTESIAN_POINT('Ctrl Pts',(58.1328445154667,-45.7020096545174,0.));
#59486=CARTESIAN_POINT('Ctrl Pts',(58.159219322515,-45.708755319378,0.));
#59487=CARTESIAN_POINT('Ctrl Pts',(58.1856349074723,-45.7154857816507,0.));
#59488=CARTESIAN_POINT('Ctrl Pts',(58.2120911942819,-45.7222009715431,0.));
#59489=CARTESIAN_POINT('Ctrl Pts',(58.2385881070959,-45.7289008195612,0.));
#59490=CARTESIAN_POINT('Ctrl Pts',(58.2651255711481,-45.7355852575127,0.));
#59491=CARTESIAN_POINT('Ctrl Pts',(58.2917035135833,-45.7422542194625,0.));
#59492=CARTESIAN_POINT('Ctrl Pts',(58.3183218645265,-45.7489076429725,0.));
#59493=CARTESIAN_POINT('Ctrl Pts',(58.3449805573335,-45.7555454693956,0.));
#59494=CARTESIAN_POINT('Ctrl Pts',(58.3678667473265,-45.7612219538034,0.));
#59495=CARTESIAN_POINT('Ctrl Pts',(58.3854348517209,-45.7655655205267,0.));
#59496=CARTESIAN_POINT('Ctrl Pts',(58.397667048078,-45.7685831165459,0.));
#59497=CARTESIAN_POINT('Ctrl Pts',(58.4045515723007,-45.7702793558063,0.));
#59498=CARTESIAN_POINT('Ctrl Pts',(58.4060826907377,-45.7706564944766,0.));
#59499=CARTESIAN_POINT('',(54.1679505278134,-44.3377168516418,12.));
#59500=CARTESIAN_POINT('',(54.1679505278134,-44.3377168516418,0.));
#59501=CARTESIAN_POINT('Ctrl Pts',(58.4060826907375,-45.7706564944766,12.));
#59502=CARTESIAN_POINT('Ctrl Pts',(58.4045515723006,-45.7702793558062,12.));
#59503=CARTESIAN_POINT('Ctrl Pts',(58.3976670480779,-45.7685831165459,12.));
#59504=CARTESIAN_POINT('Ctrl Pts',(58.3854348517209,-45.7655655205267,12.));
#59505=CARTESIAN_POINT('Ctrl Pts',(58.3678667473265,-45.7612219538034,12.));
#59506=CARTESIAN_POINT('Ctrl Pts',(58.3449805573335,-45.7555454693956,12.));
#59507=CARTESIAN_POINT('Ctrl Pts',(58.3183218645265,-45.7489076429725,12.));
#59508=CARTESIAN_POINT('Ctrl Pts',(58.2917035135833,-45.7422542194625,12.));
#59509=CARTESIAN_POINT('Ctrl Pts',(58.2651255711481,-45.7355852575127,12.));
#59510=CARTESIAN_POINT('Ctrl Pts',(58.2385881070959,-45.7289008195612,12.));
#59511=CARTESIAN_POINT('Ctrl Pts',(58.2120911942819,-45.7222009715431,12.));
#59512=CARTESIAN_POINT('Ctrl Pts',(58.1856349074723,-45.7154857816507,12.));
#59513=CARTESIAN_POINT('Ctrl Pts',(58.159219322515,-45.708755319378,12.));
#59514=CARTESIAN_POINT('Ctrl Pts',(58.1328445154667,-45.7020096545174,12.));
#59515=CARTESIAN_POINT('Ctrl Pts',(58.1065105615884,-45.6952488560134,12.));
#59516=CARTESIAN_POINT('Ctrl Pts',(58.0802175348939,-45.6884729914465,12.));
#59517=CARTESIAN_POINT('Ctrl Pts',(58.0539655087095,-45.6816821276662,12.));
#59518=CARTESIAN_POINT('Ctrl Pts',(58.0277545560001,-45.6748763311635,12.));
#59519=CARTESIAN_POINT('Ctrl Pts',(58.0015847497838,-45.6680556685494,12.));
#59520=CARTESIAN_POINT('Ctrl Pts',(57.975456163507,-45.6612202069928,12.));
#59521=CARTESIAN_POINT('Ctrl Pts',(57.9493688714249,-45.6543700146689,12.));
#59522=CARTESIAN_POINT('Ctrl Pts',(57.923322948432,-45.6475051605542,12.));
#59523=CARTESIAN_POINT('Ctrl Pts',(57.8973184699037,-45.6406257142385,12.));
#59524=CARTESIAN_POINT('Ctrl Pts',(57.8713555115232,-45.6337317457253,12.));
#59525=CARTESIAN_POINT('Ctrl Pts',(57.8454341491236,-45.6268233252543,12.));
#59526=CARTESIAN_POINT('Ctrl Pts',(57.819554458484,-45.619900523078,12.));
#59527=CARTESIAN_POINT('Ctrl Pts',(57.7937165153379,-45.6129634094678,12.));
#59528=CARTESIAN_POINT('Ctrl Pts',(57.7679203954735,-45.6060120548199,12.));
#59529=CARTESIAN_POINT('Ctrl Pts',(57.7421661748021,-45.5990465297341,12.));
#59530=CARTESIAN_POINT('Ctrl Pts',(57.7164539294316,-45.5920669050988,12.));
#59531=CARTESIAN_POINT('Ctrl Pts',(57.6907837357425,-45.5850732521902,12.));
#59532=CARTESIAN_POINT('Ctrl Pts',(57.6651556704249,-45.5780656427173,12.));
#59533=CARTESIAN_POINT('Ctrl Pts',(57.6395698104416,-45.5710441487683,12.));
#59534=CARTESIAN_POINT('Ctrl Pts',(57.6140262330048,-45.5640088427819,12.));
#59535=CARTESIAN_POINT('Ctrl Pts',(57.5885250155432,-45.5569597975096,12.));
#59536=CARTESIAN_POINT('Ctrl Pts',(57.5630662356671,-45.5498970859829,12.));
#59537=CARTESIAN_POINT('Ctrl Pts',(57.5376499711338,-45.5428207814832,12.));
#59538=CARTESIAN_POINT('Ctrl Pts',(57.5122762998732,-45.5357309575603,12.));
#59539=CARTESIAN_POINT('Ctrl Pts',(57.4869453000055,-45.5286276880479,12.));
#59540=CARTESIAN_POINT('Ctrl Pts',(57.4616570498566,-45.5215110470825,12.));
#59541=CARTESIAN_POINT('Ctrl Pts',(57.4364116279708,-45.5143811091209,12.));
#59542=CARTESIAN_POINT('Ctrl Pts',(57.4112091131193,-45.5072379489637,12.));
#59543=CARTESIAN_POINT('Ctrl Pts',(57.3860495843043,-45.5000816417516,12.));
#59544=CARTESIAN_POINT('Ctrl Pts',(57.360933120758,-45.4929122629576,12.));
#59545=CARTESIAN_POINT('Ctrl Pts',(57.335859801939,-45.4857298883826,12.));
#59546=CARTESIAN_POINT('Ctrl Pts',(57.3108297075262,-45.4785345941506,12.));
#59547=CARTESIAN_POINT('Ctrl Pts',(57.2858429174056,-45.4713264567059,12.));
#59548=CARTESIAN_POINT('Ctrl Pts',(57.2608995116727,-45.4641055528138,12.));
#59549=CARTESIAN_POINT('Ctrl Pts',(57.2359995706441,-45.4568719595639,12.));
#59550=CARTESIAN_POINT('Ctrl Pts',(57.2111431748629,-45.4496257543759,12.));
#59551=CARTESIAN_POINT('Ctrl Pts',(57.1863304051011,-45.4423670150035,12.));
#59552=CARTESIAN_POINT('Ctrl Pts',(57.1615613423586,-45.4350958195434,12.));
#59553=CARTESIAN_POINT('Ctrl Pts',(57.1368360678629,-45.4278122464387,12.));
#59554=CARTESIAN_POINT('Ctrl Pts',(57.1121546630776,-45.4205163744778,12.));
#59555=CARTESIAN_POINT('Ctrl Pts',(57.0875172097048,-45.4132082827945,12.));
#59556=CARTESIAN_POINT('Ctrl Pts',(57.0629237896848,-45.4058880508693,12.));
#59557=CARTESIAN_POINT('Ctrl Pts',(57.0383744851917,-45.3985557585316,12.));
#59558=CARTESIAN_POINT('Ctrl Pts',(57.0138693786287,-45.3912114859625,12.));
#59559=CARTESIAN_POINT('Ctrl Pts',(56.9894085526383,-45.3838553136957,12.));
#59560=CARTESIAN_POINT('Ctrl Pts',(56.9649920901079,-45.3764873226202,12.));
#59561=CARTESIAN_POINT('Ctrl Pts',(56.9406200741714,-45.3691075939827,12.));
#59562=CARTESIAN_POINT('Ctrl Pts',(56.916292588208,-45.3617162093918,12.));
#59563=CARTESIAN_POINT('Ctrl Pts',(56.8920097158371,-45.3543132508234,12.));
#59564=CARTESIAN_POINT('Ctrl Pts',(56.8677715409266,-45.3468988006202,12.));
#59565=CARTESIAN_POINT('Ctrl Pts',(56.8435781475982,-45.3394729414932,12.));
#59566=CARTESIAN_POINT('Ctrl Pts',(56.8194296202292,-45.3320357565241,12.));
#59567=CARTESIAN_POINT('Ctrl Pts',(56.7953260434521,-45.3245873291682,12.));
#59568=CARTESIAN_POINT('Ctrl Pts',(56.771267502148,-45.3171277432592,12.));
#59569=CARTESIAN_POINT('Ctrl Pts',(56.747254081454,-45.3096570830107,12.));
#59570=CARTESIAN_POINT('Ctrl Pts',(56.7232858667697,-45.3021754330169,12.));
#59571=CARTESIAN_POINT('Ctrl Pts',(56.6993629437596,-45.2946828782557,12.));
#59572=CARTESIAN_POINT('Ctrl Pts',(56.6754853983535,-45.2871795040912,12.));
#59573=CARTESIAN_POINT('Ctrl Pts',(56.6516533167398,-45.2796653962796,12.));
#59574=CARTESIAN_POINT('Ctrl Pts',(56.6278667853716,-45.2721406409707,12.));
#59575=CARTESIAN_POINT('Ctrl Pts',(56.604125890975,-45.2646053247094,12.));
#59576=CARTESIAN_POINT('Ctrl Pts',(56.5804307205507,-45.2570595344382,12.));
#59577=CARTESIAN_POINT('Ctrl Pts',(56.5567813613752,-45.2495033574997,12.));
#59578=CARTESIAN_POINT('Ctrl Pts',(56.533177900995,-45.2419368816424,12.));
#59579=CARTESIAN_POINT('Ctrl Pts',(56.5096204272299,-45.2343601950222,12.));
#59580=CARTESIAN_POINT('Ctrl Pts',(56.4861090281819,-45.2267733862046,12.));
#59581=CARTESIAN_POINT('Ctrl Pts',(56.4626437922385,-45.2191765441666,12.));
#59582=CARTESIAN_POINT('Ctrl Pts',(56.4392248080733,-45.2115697583002,12.));
#59583=CARTESIAN_POINT('Ctrl Pts',(56.4158521646412,-45.2039531184172,12.));
#59584=CARTESIAN_POINT('Ctrl Pts',(56.3925259511804,-45.1963267147527,12.));
#59585=CARTESIAN_POINT('Ctrl Pts',(56.3692462572228,-45.1886906379664,12.));
#59586=CARTESIAN_POINT('Ctrl Pts',(56.3460131725962,-45.1810449791451,12.));
#59587=CARTESIAN_POINT('Ctrl Pts',(56.3228267874265,-45.1733898298062,12.));
#59588=CARTESIAN_POINT('Ctrl Pts',(56.2996871921321,-45.1657252819018,12.));
#59589=CARTESIAN_POINT('Ctrl Pts',(56.2765944774252,-45.158051427823,12.));
#59590=CARTESIAN_POINT('Ctrl Pts',(56.2535487343227,-45.150368360401,12.));
#59591=CARTESIAN_POINT('Ctrl Pts',(56.2305500541491,-45.1426761729107,12.));
#59592=CARTESIAN_POINT('Ctrl Pts',(56.2075985285391,-45.1349749590736,12.));
#59593=CARTESIAN_POINT('Ctrl Pts',(56.1846942494321,-45.1272648130627,12.));
#59594=CARTESIAN_POINT('Ctrl Pts',(56.1618373090729,-45.119545829506,12.));
#59595=CARTESIAN_POINT('Ctrl Pts',(56.1390278000226,-45.1118181034888,12.));
#59596=CARTESIAN_POINT('Ctrl Pts',(56.1162658151621,-45.1040817305563,12.));
#59597=CARTESIAN_POINT('Ctrl Pts',(56.0935514476945,-45.0963368067177,12.));
#59598=CARTESIAN_POINT('Ctrl Pts',(56.070884791141,-45.0885834284513,12.));
#59599=CARTESIAN_POINT('Ctrl Pts',(56.0482659393412,-45.0808216927082,12.));
#59600=CARTESIAN_POINT('Ctrl Pts',(56.025694986463,-45.0730516969142,12.));
#59601=CARTESIAN_POINT('Ctrl Pts',(56.0031720270074,-45.0652735389729,12.));
#59602=CARTESIAN_POINT('Ctrl Pts',(55.9806971558099,-45.0574873172696,12.));
#59603=CARTESIAN_POINT('Ctrl Pts',(55.958270468037,-45.0496931306767,12.));
#59604=CARTESIAN_POINT('Ctrl Pts',(55.9358920591861,-45.041891078557,12.));
#59605=CARTESIAN_POINT('Ctrl Pts',(55.9135620250977,-45.0340812607676,12.));
#59606=CARTESIAN_POINT('Ctrl Pts',(55.8912804619588,-45.0262637776623,12.));
#59607=CARTESIAN_POINT('Ctrl Pts',(55.8690474663058,-45.0184387300968,12.));
#59608=CARTESIAN_POINT('Ctrl Pts',(55.8468631350195,-45.0106062194325,12.));
#59609=CARTESIAN_POINT('Ctrl Pts',(55.8247275653257,-45.002766347541,12.));
#59610=CARTESIAN_POINT('Ctrl Pts',(55.8026408548078,-44.9949192168073,12.));
#59611=CARTESIAN_POINT('Ctrl Pts',(55.7806031014093,-44.9870649301333,12.));
#59612=CARTESIAN_POINT('Ctrl Pts',(55.7586144034376,-44.979203590942,12.));
#59613=CARTESIAN_POINT('Ctrl Pts',(55.7366748595582,-44.9713353031827,12.));
#59614=CARTESIAN_POINT('Ctrl Pts',(55.7147845687969,-44.9634601713352,12.));
#59615=CARTESIAN_POINT('Ctrl Pts',(55.6929436305522,-44.9555783004133,12.));
#59616=CARTESIAN_POINT('Ctrl Pts',(55.671152144599,-44.9476897959694,12.));
#59617=CARTESIAN_POINT('Ctrl Pts',(55.6494102110922,-44.9397947640996,12.));
#59618=CARTESIAN_POINT('Ctrl Pts',(55.6277179305604,-44.9318933114483,12.));
#59619=CARTESIAN_POINT('Ctrl Pts',(55.6060754039089,-44.9239855452119,12.));
#59620=CARTESIAN_POINT('Ctrl Pts',(55.5844827324315,-44.9160715731425,12.));
#59621=CARTESIAN_POINT('Ctrl Pts',(55.5629400178136,-44.9081515035526,12.));
#59622=CARTESIAN_POINT('Ctrl Pts',(55.541447362135,-44.9002254453192,12.));
#59623=CARTESIAN_POINT('Ctrl Pts',(55.5200048678648,-44.8922935078905,12.));
#59624=CARTESIAN_POINT('Ctrl Pts',(55.4986126378676,-44.8843558012903,12.));
#59625=CARTESIAN_POINT('Ctrl Pts',(55.4772707754139,-44.8764124361218,12.));
#59626=CARTESIAN_POINT('Ctrl Pts',(55.4559793841838,-44.8684635235727,12.));
#59627=CARTESIAN_POINT('Ctrl Pts',(55.4347385682697,-44.8605091754208,12.));
#59628=CARTESIAN_POINT('Ctrl Pts',(55.4135484321706,-44.8525495040398,12.));
#59629=CARTESIAN_POINT('Ctrl Pts',(55.3924090808002,-44.8445846224034,12.));
#59630=CARTESIAN_POINT('Ctrl Pts',(55.3713206194962,-44.8366146440896,12.));
#59631=CARTESIAN_POINT('Ctrl Pts',(55.3502831540229,-44.8286396832849,12.));
#59632=CARTESIAN_POINT('Ctrl Pts',(55.3292967905725,-44.8206598547889,12.));
#59633=CARTESIAN_POINT('Ctrl Pts',(55.3083616357605,-44.812675274021,12.));
#59634=CARTESIAN_POINT('Ctrl Pts',(55.2874777966349,-44.8046860570245,12.));
#59635=CARTESIAN_POINT('Ctrl Pts',(55.2666453806882,-44.7966923204741,12.));
#59636=CARTESIAN_POINT('Ctrl Pts',(55.2458644958617,-44.7886941816823,12.));
#59637=CARTESIAN_POINT('Ctrl Pts',(55.2251352505475,-44.7806917586077,12.));
#59638=CARTESIAN_POINT('Ctrl Pts',(55.2044577535866,-44.7726851698619,12.));
#59639=CARTESIAN_POINT('Ctrl Pts',(55.1838321142779,-44.7646745347109,12.));
#59640=CARTESIAN_POINT('Ctrl Pts',(55.1632584423815,-44.7566599730773,12.));
#59641=CARTESIAN_POINT('Ctrl Pts',(55.14273684812,-44.748641605542,12.));
#59642=CARTESIAN_POINT('Ctrl Pts',(55.1222674421743,-44.740619553348,12.));
#59643=CARTESIAN_POINT('Ctrl Pts',(55.1018503356795,-44.7325939384035,12.));
#59644=CARTESIAN_POINT('Ctrl Pts',(55.0814856402495,-44.7245648832979,12.));
#59645=CARTESIAN_POINT('Ctrl Pts',(55.0611734679894,-44.716532511316,12.));
#59646=CARTESIAN_POINT('Ctrl Pts',(55.0409139315078,-44.7084969464513,12.));
#59647=CARTESIAN_POINT('Ctrl Pts',(55.0207071439237,-44.7004583134249,12.));
#59648=CARTESIAN_POINT('Ctrl Pts',(55.0005532188667,-44.6924167376869,12.));
#59649=CARTESIAN_POINT('Ctrl Pts',(54.9804522704686,-44.6843723454,12.));
#59650=CARTESIAN_POINT('Ctrl Pts',(54.9604044133501,-44.6763252634259,12.));
#59651=CARTESIAN_POINT('Ctrl Pts',(54.9404097626077,-44.6682756193147,12.));
#59652=CARTESIAN_POINT('Ctrl Pts',(54.9204684337822,-44.6602235412836,12.));
#59653=CARTESIAN_POINT('Ctrl Pts',(54.9005805428969,-44.6521691582534,12.));
#59654=CARTESIAN_POINT('Ctrl Pts',(54.8807462065164,-44.6441125999063,12.));
#59655=CARTESIAN_POINT('Ctrl Pts',(54.860965541796,-44.6360539967392,12.));
#59656=CARTESIAN_POINT('Ctrl Pts',(54.8412386665276,-44.6279934801169,12.));
#59657=CARTESIAN_POINT('Ctrl Pts',(54.8215656991837,-44.6199311823293,12.));
#59658=CARTESIAN_POINT('Ctrl Pts',(54.8019467588278,-44.6118672364906,12.));
#59659=CARTESIAN_POINT('Ctrl Pts',(54.7823819650148,-44.603801776431,12.));
#59660=CARTESIAN_POINT('Ctrl Pts',(54.7628714377037,-44.5957349366059,12.));
#59661=CARTESIAN_POINT('Ctrl Pts',(54.7434152971267,-44.5876668519661,12.));
#59662=CARTESIAN_POINT('Ctrl Pts',(54.7240136637717,-44.5795976579454,12.));
#59663=CARTESIAN_POINT('Ctrl Pts',(54.7046666586754,-44.5715274907619,12.));
#59664=CARTESIAN_POINT('Ctrl Pts',(54.6853744036751,-44.5634564876863,12.));
#59665=CARTESIAN_POINT('Ctrl Pts',(54.6661370216252,-44.5553847872721,12.));
#59666=CARTESIAN_POINT('Ctrl Pts',(54.6469546367408,-44.5473125297312,12.));
#59667=CARTESIAN_POINT('Ctrl Pts',(54.6278273743587,-44.5392398566802,12.));
#59668=CARTESIAN_POINT('Ctrl Pts',(54.6087553602914,-44.5311669104515,12.));
#59669=CARTESIAN_POINT('Ctrl Pts',(54.5897387202815,-44.5230938335167,12.));
#59670=CARTESIAN_POINT('Ctrl Pts',(54.5707775794412,-44.5150207678988,12.));
#59671=CARTESIAN_POINT('Ctrl Pts',(54.5518720616016,-44.5069478544945,12.));
#59672=CARTESIAN_POINT('Ctrl Pts',(54.5330222905438,-44.4988752343715,12.));
#59673=CARTESIAN_POINT('Ctrl Pts',(54.5142283914684,-44.4908030503209,12.));
#59674=CARTESIAN_POINT('Ctrl Pts',(54.4954904921938,-44.4827314481271,12.));
#59675=CARTESIAN_POINT('Ctrl Pts',(54.4768087248854,-44.4746605784056,12.));
#59676=CARTESIAN_POINT('Ctrl Pts',(54.4581832262072,-44.4665905967701,12.));
#59677=CARTESIAN_POINT('Ctrl Pts',(54.4396141337008,-44.4585216599933,12.));
#59678=CARTESIAN_POINT('Ctrl Pts',(54.4211015825959,-44.4504539226336,12.));
#59679=CARTESIAN_POINT('Ctrl Pts',(54.4026457030316,-44.442387534098,12.));
#59680=CARTESIAN_POINT('Ctrl Pts',(54.3842466156151,-44.4343226339555,12.));
#59681=CARTESIAN_POINT('Ctrl Pts',(54.3659044357064,-44.4262593564664,12.));
#59682=CARTESIAN_POINT('Ctrl Pts',(54.347619281931,-44.4181978395814,12.));
#59683=CARTESIAN_POINT('Ctrl Pts',(54.3293912830237,-44.4101382321834,12.));
#59684=CARTESIAN_POINT('Ctrl Pts',(54.3112205860776,-44.4020807028144,12.));
#59685=CARTESIAN_POINT('Ctrl Pts',(54.2931073621661,-44.3940254456427,12.));
#59686=CARTESIAN_POINT('Ctrl Pts',(54.2750517888695,-44.3859726620288,12.));
#59687=CARTESIAN_POINT('Ctrl Pts',(54.2570540336536,-44.3779225430461,12.));
#59688=CARTESIAN_POINT('Ctrl Pts',(54.2391142386354,-44.369875253351,12.));
#59689=CARTESIAN_POINT('Ctrl Pts',(54.2212325005847,-44.3618309103245,12.));
#59690=CARTESIAN_POINT('Ctrl Pts',(54.203408870162,-44.3537895823819,12.));
#59691=CARTESIAN_POINT('Ctrl Pts',(54.1891964684439,-44.3473589597468,12.));
#59692=CARTESIAN_POINT('Ctrl Pts',(54.1785633257456,-44.3425373700829,12.));
#59693=CARTESIAN_POINT('Ctrl Pts',(54.1714861895278,-44.3393235891014,12.));
#59694=CARTESIAN_POINT('Ctrl Pts',(54.1679505278134,-44.3377168516418,12.));
#59695=CARTESIAN_POINT('Ctrl Pts',(59.3276657444391,-44.569626075779,0.));
#59696=CARTESIAN_POINT('Ctrl Pts',(59.3276657444391,-44.569626075779,4.));
#59697=CARTESIAN_POINT('Ctrl Pts',(59.3276657444392,-44.5696260757792,8.));
#59698=CARTESIAN_POINT('Ctrl Pts',(59.3276657444392,-44.5696260757792,12.));
#59699=CARTESIAN_POINT('Ctrl Pts',(59.3806648691717,-44.6658822400931,0.));
#59700=CARTESIAN_POINT('Ctrl Pts',(59.3806648691717,-44.6658822400931,4.));
#59701=CARTESIAN_POINT('Ctrl Pts',(59.3806648691718,-44.6658822400932,8.00000000000001));
#59702=CARTESIAN_POINT('Ctrl Pts',(59.3806648691718,-44.6658822400932,12.));
#59703=CARTESIAN_POINT('Ctrl Pts',(59.4154499491515,-44.8655383388338,0.));
#59704=CARTESIAN_POINT('Ctrl Pts',(59.4154499491515,-44.8655383388338,4.));
#59705=CARTESIAN_POINT('Ctrl Pts',(59.4154499491515,-44.8655383388339,7.99999999999999));
#59706=CARTESIAN_POINT('Ctrl Pts',(59.4154499491515,-44.8655383388339,12.));
#59707=CARTESIAN_POINT('Ctrl Pts',(59.3374774995078,-45.0479805952316,0.));
#59708=CARTESIAN_POINT('Ctrl Pts',(59.3374774995078,-45.0479805952316,4.));
#59709=CARTESIAN_POINT('Ctrl Pts',(59.3374774995078,-45.0479805952316,8.00000000000001));
#59710=CARTESIAN_POINT('Ctrl Pts',(59.3374774995078,-45.0479805952316,12.));
#59711=CARTESIAN_POINT('Ctrl Pts',(59.2875729049562,-45.1135644683446,0.));
#59712=CARTESIAN_POINT('Ctrl Pts',(59.2875729049562,-45.1135644683446,4.));
#59713=CARTESIAN_POINT('Ctrl Pts',(59.2875729049562,-45.1135644683447,8.));
#59714=CARTESIAN_POINT('Ctrl Pts',(59.2875729049562,-45.1135644683447,12.));
#59715=CARTESIAN_POINT('',(59.3276657444391,-44.569626075779,0.));
#59716=CARTESIAN_POINT('',(59.2875729049563,-45.1135644683447,0.));
#59717=CARTESIAN_POINT('Ctrl Pts',(59.3276657444391,-44.569626075779,1.38777878078145E-16));
#59718=CARTESIAN_POINT('Ctrl Pts',(59.3806648691717,-44.6658822400931,1.38777878078145E-16));
#59719=CARTESIAN_POINT('Ctrl Pts',(59.4005420577316,-44.7799714393735,1.38777878078145E-16));
#59720=CARTESIAN_POINT('Ctrl Pts',(59.3836004611083,-44.8884397921746,1.38777878078145E-16));
#59721=CARTESIAN_POINT('Ctrl Pts',(59.3708942636408,-44.9697910567754,1.38777878078145E-16));
#59722=CARTESIAN_POINT('Ctrl Pts',(59.3374774995078,-45.0479805952316,1.38777878078144E-16));
#59723=CARTESIAN_POINT('Ctrl Pts',(59.2875729049562,-45.1135644683446,1.38777878078145E-16));
#59724=CARTESIAN_POINT('',(59.2875729049563,-45.1135644683447,12.));
#59725=CARTESIAN_POINT('Ctrl Pts',(59.2875729049562,-45.1135644683446,0.));
#59726=CARTESIAN_POINT('Ctrl Pts',(59.2875729049562,-45.1135644683446,4.));
#59727=CARTESIAN_POINT('Ctrl Pts',(59.2875729049562,-45.1135644683447,8.));
#59728=CARTESIAN_POINT('Ctrl Pts',(59.2875729049562,-45.1135644683447,12.));
#59729=CARTESIAN_POINT('',(59.3276657444392,-44.5696260757792,12.));
#59730=CARTESIAN_POINT('Ctrl Pts',(59.2875729049562,-45.1135644683447,12.));
#59731=CARTESIAN_POINT('Ctrl Pts',(59.3374774995078,-45.0479805952316,12.));
#59732=CARTESIAN_POINT('Ctrl Pts',(59.3708942636408,-44.9697910567755,12.));
#59733=CARTESIAN_POINT('Ctrl Pts',(59.3836004611083,-44.8884397921747,12.));
#59734=CARTESIAN_POINT('Ctrl Pts',(59.4005420577316,-44.7799714393736,12.));
#59735=CARTESIAN_POINT('Ctrl Pts',(59.3806648691718,-44.6658822400932,12.));
#59736=CARTESIAN_POINT('Ctrl Pts',(59.3276657444392,-44.5696260757792,12.));
#59737=CARTESIAN_POINT('Ctrl Pts',(59.3276657444392,-44.5696260757792,12.));
#59738=CARTESIAN_POINT('Ctrl Pts',(59.3276657444392,-44.5696260757792,8.));
#59739=CARTESIAN_POINT('Ctrl Pts',(59.3276657444391,-44.569626075779,4.));
#59740=CARTESIAN_POINT('Ctrl Pts',(59.3276657444391,-44.569626075779,0.));
#59741=CARTESIAN_POINT('Origin',(2.97443977737815E-10,-2.28111678886296E-10,
0.));
#59742=CARTESIAN_POINT('Origin',(2.97443977737815E-10,-2.28111678886296E-10,
12.));
#59743=CARTESIAN_POINT('Origin',(2.97443977737815E-10,-2.28111678886296E-10,
0.));
#59744=CARTESIAN_POINT('Ctrl Pts',(54.7233670476848,-50.5529731960877,0.));
#59745=CARTESIAN_POINT('Ctrl Pts',(54.7233670476848,-50.5529731960877,4.));
#59746=CARTESIAN_POINT('Ctrl Pts',(54.7233670476849,-50.5529731960877,8.));
#59747=CARTESIAN_POINT('Ctrl Pts',(54.7233670476849,-50.5529731960877,12.));
#59748=CARTESIAN_POINT('Ctrl Pts',(54.6488048279281,-50.6336864649949,0.));
#59749=CARTESIAN_POINT('Ctrl Pts',(54.6488048279281,-50.6336864649949,4.));
#59750=CARTESIAN_POINT('Ctrl Pts',(54.6488048279282,-50.6336864649949,8.));
#59751=CARTESIAN_POINT('Ctrl Pts',(54.6488048279282,-50.6336864649949,12.));
#59752=CARTESIAN_POINT('Ctrl Pts',(54.4703879751549,-50.7298112257547,0.));
#59753=CARTESIAN_POINT('Ctrl Pts',(54.4703879751549,-50.7298112257547,4.));
#59754=CARTESIAN_POINT('Ctrl Pts',(54.470387975155,-50.7298112257547,8.));
#59755=CARTESIAN_POINT('Ctrl Pts',(54.470387975155,-50.7298112257547,12.));
#59756=CARTESIAN_POINT('Ctrl Pts',(54.2726521137402,-50.7135202769403,0.));
#59757=CARTESIAN_POINT('Ctrl Pts',(54.2726521137402,-50.7135202769403,4.));
#59758=CARTESIAN_POINT('Ctrl Pts',(54.2726521137402,-50.7135202769403,8.00000000000001));
#59759=CARTESIAN_POINT('Ctrl Pts',(54.2726521137402,-50.7135202769403,12.));
#59760=CARTESIAN_POINT('Ctrl Pts',(54.194654349997,-50.6869108458685,0.));
#59761=CARTESIAN_POINT('Ctrl Pts',(54.194654349997,-50.6869108458685,4.));
#59762=CARTESIAN_POINT('Ctrl Pts',(54.194654349997,-50.6869108458684,8.));
#59763=CARTESIAN_POINT('Ctrl Pts',(54.194654349997,-50.6869108458684,12.));
#59764=CARTESIAN_POINT('',(54.7233670476848,-50.5529731960877,0.));
#59765=CARTESIAN_POINT('',(54.1946543499969,-50.6869108458685,0.));
#59766=CARTESIAN_POINT('Ctrl Pts',(54.7233670476848,-50.5529731960877,0.));
#59767=CARTESIAN_POINT('Ctrl Pts',(54.6488048279281,-50.6336864649949,0.));
#59768=CARTESIAN_POINT('Ctrl Pts',(54.5468523406292,-50.6886148997148,0.));
#59769=CARTESIAN_POINT('Ctrl Pts',(54.4385916056105,-50.7068361639615,0.));
#59770=CARTESIAN_POINT('Ctrl Pts',(54.3573960543465,-50.7205021121465,0.));
#59771=CARTESIAN_POINT('Ctrl Pts',(54.2726521137402,-50.7135202769403,0.));
#59772=CARTESIAN_POINT('Ctrl Pts',(54.194654349997,-50.6869108458685,0.));
#59773=CARTESIAN_POINT('',(54.1946543499969,-50.6869108458685,12.));
#59774=CARTESIAN_POINT('Ctrl Pts',(54.194654349997,-50.6869108458685,0.));
#59775=CARTESIAN_POINT('Ctrl Pts',(54.194654349997,-50.6869108458685,4.));
#59776=CARTESIAN_POINT('Ctrl Pts',(54.194654349997,-50.6869108458684,8.));
#59777=CARTESIAN_POINT('Ctrl Pts',(54.194654349997,-50.6869108458684,12.));
#59778=CARTESIAN_POINT('',(54.7233670476849,-50.5529731960877,12.));
#59779=CARTESIAN_POINT('Ctrl Pts',(54.194654349997,-50.6869108458684,12.));
#59780=CARTESIAN_POINT('Ctrl Pts',(54.2726521137402,-50.7135202769403,12.));
#59781=CARTESIAN_POINT('Ctrl Pts',(54.3573960543465,-50.7205021121465,12.));
#59782=CARTESIAN_POINT('Ctrl Pts',(54.4385916056105,-50.7068361639615,12.));
#59783=CARTESIAN_POINT('Ctrl Pts',(54.5468523406292,-50.6886148997148,12.));
#59784=CARTESIAN_POINT('Ctrl Pts',(54.6488048279282,-50.6336864649949,12.));
#59785=CARTESIAN_POINT('Ctrl Pts',(54.7233670476849,-50.5529731960877,12.));
#59786=CARTESIAN_POINT('Ctrl Pts',(54.7233670476849,-50.5529731960877,12.));
#59787=CARTESIAN_POINT('Ctrl Pts',(54.7233670476849,-50.5529731960877,8.));
#59788=CARTESIAN_POINT('Ctrl Pts',(54.7233670476848,-50.5529731960877,4.));
#59789=CARTESIAN_POINT('Ctrl Pts',(54.7233670476848,-50.5529731960877,0.));
#59790=CARTESIAN_POINT('Ctrl Pts',(50.0975384783634,-48.8900464144686,0.));
#59791=CARTESIAN_POINT('Ctrl Pts',(50.0975384783634,-48.8900464144686,12.));
#59792=CARTESIAN_POINT('Ctrl Pts',(50.1009206494209,-48.8919551910299,0.));
#59793=CARTESIAN_POINT('Ctrl Pts',(50.1009206494209,-48.8919551910299,12.));
#59794=CARTESIAN_POINT('Ctrl Pts',(50.1076907555303,-48.8957735556681,0.));
#59795=CARTESIAN_POINT('Ctrl Pts',(50.1076907555303,-48.8957735556681,12.));
#59796=CARTESIAN_POINT('Ctrl Pts',(50.1178632066821,-48.9015035371772,0.));
#59797=CARTESIAN_POINT('Ctrl Pts',(50.1178632066821,-48.9015035371772,12.));
#59798=CARTESIAN_POINT('Ctrl Pts',(50.1314610602286,-48.9091483817797,0.));
#59799=CARTESIAN_POINT('Ctrl Pts',(50.1314610602286,-48.9091483817797,12.));
#59800=CARTESIAN_POINT('Ctrl Pts',(50.148516018447,-48.9187125417897,0.));
#59801=CARTESIAN_POINT('Ctrl Pts',(50.148516018447,-48.9187125417897,12.));
#59802=CARTESIAN_POINT('Ctrl Pts',(50.1656286003943,-48.9282847698237,0.));
#59803=CARTESIAN_POINT('Ctrl Pts',(50.1656286003943,-48.9282847698237,12.));
#59804=CARTESIAN_POINT('Ctrl Pts',(50.1827987615659,-48.9378649933116,0.));
#59805=CARTESIAN_POINT('Ctrl Pts',(50.1827987615659,-48.9378649933116,12.));
#59806=CARTESIAN_POINT('Ctrl Pts',(50.2000264157903,-48.9474530868847,0.));
#59807=CARTESIAN_POINT('Ctrl Pts',(50.2000264157903,-48.9474530868847,12.));
#59808=CARTESIAN_POINT('Ctrl Pts',(50.2173114358423,-48.9570488741273,0.));
#59809=CARTESIAN_POINT('Ctrl Pts',(50.2173114358423,-48.9570488741273,12.));
#59810=CARTESIAN_POINT('Ctrl Pts',(50.2346536715465,-48.9666521500969,0.));
#59811=CARTESIAN_POINT('Ctrl Pts',(50.2346536715465,-48.9666521500969,12.));
#59812=CARTESIAN_POINT('Ctrl Pts',(50.252052963548,-48.9762626987227,0.));
#59813=CARTESIAN_POINT('Ctrl Pts',(50.252052963548,-48.9762626987227,12.));
#59814=CARTESIAN_POINT('Ctrl Pts',(50.2695091583472,-48.9858803116649,0.));
#59815=CARTESIAN_POINT('Ctrl Pts',(50.2695091583472,-48.9858803116649,12.));
#59816=CARTESIAN_POINT('Ctrl Pts',(50.2870221241003,-48.9955048082028,0.));
#59817=CARTESIAN_POINT('Ctrl Pts',(50.2870221241003,-48.9955048082028,12.));
#59818=CARTESIAN_POINT('Ctrl Pts',(50.3045917455383,-49.0051360288002,0.));
#59819=CARTESIAN_POINT('Ctrl Pts',(50.3045917455383,-49.0051360288002,12.));
#59820=CARTESIAN_POINT('Ctrl Pts',(50.3222179165102,-49.0147738256925,0.));
#59821=CARTESIAN_POINT('Ctrl Pts',(50.3222179165102,-49.0147738256925,12.));
#59822=CARTESIAN_POINT('Ctrl Pts',(50.3399005337967,-49.0244180550759,0.));
#59823=CARTESIAN_POINT('Ctrl Pts',(50.3399005337967,-49.0244180550759,12.));
#59824=CARTESIAN_POINT('Ctrl Pts',(50.3576394894136,-49.034068567401,0.));
#59825=CARTESIAN_POINT('Ctrl Pts',(50.3576394894136,-49.034068567401,12.));
#59826=CARTESIAN_POINT('Ctrl Pts',(50.3754346667389,-49.0437252024868,0.));
#59827=CARTESIAN_POINT('Ctrl Pts',(50.3754346667389,-49.0437252024868,12.));
#59828=CARTESIAN_POINT('Ctrl Pts',(50.393285944528,-49.0533877945771,0.));
#59829=CARTESIAN_POINT('Ctrl Pts',(50.393285944528,-49.0533877945771,12.));
#59830=CARTESIAN_POINT('Ctrl Pts',(50.4111931994264,-49.0630561755082,0.));
#59831=CARTESIAN_POINT('Ctrl Pts',(50.4111931994264,-49.0630561755082,12.));
#59832=CARTESIAN_POINT('Ctrl Pts',(50.4291563088528,-49.0727301783477,0.));
#59833=CARTESIAN_POINT('Ctrl Pts',(50.4291563088528,-49.0727301783477,12.));
#59834=CARTESIAN_POINT('Ctrl Pts',(50.4471751542717,-49.0824096415339,0.));
#59835=CARTESIAN_POINT('Ctrl Pts',(50.4471751542717,-49.0824096415339,12.));
#59836=CARTESIAN_POINT('Ctrl Pts',(50.465249621057,-49.0920944086973,0.));
#59837=CARTESIAN_POINT('Ctrl Pts',(50.465249621057,-49.0920944086973,12.));
#59838=CARTESIAN_POINT('Ctrl Pts',(50.4833795969296,-49.1017843266782,0.));
#59839=CARTESIAN_POINT('Ctrl Pts',(50.4833795969296,-49.1017843266782,12.));
#59840=CARTESIAN_POINT('Ctrl Pts',(50.5015649708742,-49.1114792441573,0.));
#59841=CARTESIAN_POINT('Ctrl Pts',(50.5015649708742,-49.1114792441573,12.));
#59842=CARTESIAN_POINT('Ctrl Pts',(50.5198056318111,-49.1211790099817,0.));
#59843=CARTESIAN_POINT('Ctrl Pts',(50.5198056318111,-49.1211790099817,12.));
#59844=CARTESIAN_POINT('Ctrl Pts',(50.5381014674822,-49.1308834717645,0.));
#59845=CARTESIAN_POINT('Ctrl Pts',(50.5381014674822,-49.1308834717645,12.));
#59846=CARTESIAN_POINT('Ctrl Pts',(50.5564523650406,-49.1405924766169,0.));
#59847=CARTESIAN_POINT('Ctrl Pts',(50.5564523650406,-49.1405924766169,12.));
#59848=CARTESIAN_POINT('Ctrl Pts',(50.5748582115575,-49.1503058717831,0.));
#59849=CARTESIAN_POINT('Ctrl Pts',(50.5748582115575,-49.1503058717831,12.));
#59850=CARTESIAN_POINT('Ctrl Pts',(50.593318894516,-49.1600235052613,0.));
#59851=CARTESIAN_POINT('Ctrl Pts',(50.593318894516,-49.1600235052613,12.));
#59852=CARTESIAN_POINT('Ctrl Pts',(50.6118343023937,-49.1697452265473,0.));
#59853=CARTESIAN_POINT('Ctrl Pts',(50.6118343023937,-49.1697452265473,12.));
#59854=CARTESIAN_POINT('Ctrl Pts',(50.6304043248796,-49.1794708869074,0.));
#59855=CARTESIAN_POINT('Ctrl Pts',(50.6304043248796,-49.1794708869074,12.));
#59856=CARTESIAN_POINT('Ctrl Pts',(50.6490288525639,-49.1892003389743,0.));
#59857=CARTESIAN_POINT('Ctrl Pts',(50.6490288525639,-49.1892003389743,12.));
#59858=CARTESIAN_POINT('Ctrl Pts',(50.6677077767427,-49.1989334364992,0.));
#59859=CARTESIAN_POINT('Ctrl Pts',(50.6677077767427,-49.1989334364992,12.));
#59860=CARTESIAN_POINT('Ctrl Pts',(50.6864409891905,-49.2086700340625,0.));
#59861=CARTESIAN_POINT('Ctrl Pts',(50.6864409891905,-49.2086700340625,12.));
#59862=CARTESIAN_POINT('Ctrl Pts',(50.7052283818941,-49.218409986748,0.));
#59863=CARTESIAN_POINT('Ctrl Pts',(50.7052283818941,-49.218409986748,12.));
#59864=CARTESIAN_POINT('Ctrl Pts',(50.7240698470698,-49.2281531501569,0.));
#59865=CARTESIAN_POINT('Ctrl Pts',(50.7240698470698,-49.2281531501569,12.));
#59866=CARTESIAN_POINT('Ctrl Pts',(50.7429652772816,-49.2378993805482,0.));
#59867=CARTESIAN_POINT('Ctrl Pts',(50.7429652772816,-49.2378993805482,12.));
#59868=CARTESIAN_POINT('Ctrl Pts',(50.7619145655207,-49.2476485349373,0.));
#59869=CARTESIAN_POINT('Ctrl Pts',(50.7619145655207,-49.2476485349373,12.));
#59870=CARTESIAN_POINT('Ctrl Pts',(50.7809176052954,-49.2574004712122,0.));
#59871=CARTESIAN_POINT('Ctrl Pts',(50.7809176052954,-49.2574004712122,12.));
#59872=CARTESIAN_POINT('Ctrl Pts',(50.799974290711,-49.2671550482415,0.));
#59873=CARTESIAN_POINT('Ctrl Pts',(50.799974290711,-49.2671550482415,12.));
#59874=CARTESIAN_POINT('Ctrl Pts',(50.8190845164319,-49.2769121258144,0.));
#59875=CARTESIAN_POINT('Ctrl Pts',(50.8190845164319,-49.2769121258144,12.));
#59876=CARTESIAN_POINT('Ctrl Pts',(50.8382481776392,-49.2866715645828,0.));
#59877=CARTESIAN_POINT('Ctrl Pts',(50.8382481776392,-49.2866715645828,12.));
#59878=CARTESIAN_POINT('Ctrl Pts',(50.8574651699877,-49.2964332260043,0.));
#59879=CARTESIAN_POINT('Ctrl Pts',(50.8574651699877,-49.2964332260043,12.));
#59880=CARTESIAN_POINT('Ctrl Pts',(50.8767353895509,-49.3061969722798,0.));
#59881=CARTESIAN_POINT('Ctrl Pts',(50.8767353895509,-49.3061969722798,12.));
#59882=CARTESIAN_POINT('Ctrl Pts',(50.8960587327869,-49.3159626663129,0.));
#59883=CARTESIAN_POINT('Ctrl Pts',(50.8960587327869,-49.3159626663129,12.));
#59884=CARTESIAN_POINT('Ctrl Pts',(50.9154350965681,-49.325730171735,0.));
#59885=CARTESIAN_POINT('Ctrl Pts',(50.9154350965681,-49.325730171735,12.));
#59886=CARTESIAN_POINT('Ctrl Pts',(50.9348643781928,-49.3354993529163,0.));
#59887=CARTESIAN_POINT('Ctrl Pts',(50.9348643781928,-49.3354993529163,12.));
#59888=CARTESIAN_POINT('Ctrl Pts',(50.9543464753974,-49.3452700749804,0.));
#59889=CARTESIAN_POINT('Ctrl Pts',(50.9543464753974,-49.3452700749804,12.));
#59890=CARTESIAN_POINT('Ctrl Pts',(50.9738812863635,-49.3550422038221,0.));
#59891=CARTESIAN_POINT('Ctrl Pts',(50.9738812863635,-49.3550422038221,12.));
#59892=CARTESIAN_POINT('Ctrl Pts',(50.9934687097179,-49.3648156061049,0.));
#59893=CARTESIAN_POINT('Ctrl Pts',(50.9934687097179,-49.3648156061049,12.));
#59894=CARTESIAN_POINT('Ctrl Pts',(51.0131086445268,-49.3745901492429,0.));
#59895=CARTESIAN_POINT('Ctrl Pts',(51.0131086445268,-49.3745901492429,12.));
#59896=CARTESIAN_POINT('Ctrl Pts',(51.0328009902857,-49.3843657013851,0.));
#59897=CARTESIAN_POINT('Ctrl Pts',(51.0328009902857,-49.3843657013851,12.));
#59898=CARTESIAN_POINT('Ctrl Pts',(51.0525456469072,-49.3941421314014,0.));
#59899=CARTESIAN_POINT('Ctrl Pts',(51.0525456469072,-49.3941421314014,12.));
#59900=CARTESIAN_POINT('Ctrl Pts',(51.0723425146987,-49.4039193088636,0.));
#59901=CARTESIAN_POINT('Ctrl Pts',(51.0723425146987,-49.4039193088636,12.));
#59902=CARTESIAN_POINT('Ctrl Pts',(51.0921914943663,-49.4136971040428,0.));
#59903=CARTESIAN_POINT('Ctrl Pts',(51.0921914943663,-49.4136971040428,12.));
#59904=CARTESIAN_POINT('Ctrl Pts',(51.1120924870196,-49.4234753879071,0.));
#59905=CARTESIAN_POINT('Ctrl Pts',(51.1120924870196,-49.4234753879071,12.));
#59906=CARTESIAN_POINT('Ctrl Pts',(51.1320453941702,-49.4332540321178,0.));
#59907=CARTESIAN_POINT('Ctrl Pts',(51.1320453941702,-49.4332540321178,12.));
#59908=CARTESIAN_POINT('Ctrl Pts',(51.1520501177291,-49.4430329090288,0.));
#59909=CARTESIAN_POINT('Ctrl Pts',(51.1520501177291,-49.4430329090288,12.));
#59910=CARTESIAN_POINT('Ctrl Pts',(51.1721065599972,-49.4528118916833,0.));
#59911=CARTESIAN_POINT('Ctrl Pts',(51.1721065599972,-49.4528118916833,12.));
#59912=CARTESIAN_POINT('Ctrl Pts',(51.1922146236686,-49.4625908538076,0.));
#59913=CARTESIAN_POINT('Ctrl Pts',(51.1922146236686,-49.4625908538076,12.));
#59914=CARTESIAN_POINT('Ctrl Pts',(51.2123742118288,-49.4723696698022,0.));
#59915=CARTESIAN_POINT('Ctrl Pts',(51.2123742118288,-49.4723696698022,12.));
#59916=CARTESIAN_POINT('Ctrl Pts',(51.2325852279507,-49.4821482147357,0.));
#59917=CARTESIAN_POINT('Ctrl Pts',(51.2325852279507,-49.4821482147357,12.));
#59918=CARTESIAN_POINT('Ctrl Pts',(51.2528475758841,-49.4919263643357,0.));
#59919=CARTESIAN_POINT('Ctrl Pts',(51.2528475758841,-49.4919263643357,12.));
#59920=CARTESIAN_POINT('Ctrl Pts',(51.2731611598465,-49.5017039949841,0.));
#59921=CARTESIAN_POINT('Ctrl Pts',(51.2731611598465,-49.5017039949841,12.));
#59922=CARTESIAN_POINT('Ctrl Pts',(51.2935258844278,-49.5114809837111,0.));
#59923=CARTESIAN_POINT('Ctrl Pts',(51.2935258844278,-49.5114809837111,12.));
#59924=CARTESIAN_POINT('Ctrl Pts',(51.3139416545903,-49.5212572081901,0.));
#59925=CARTESIAN_POINT('Ctrl Pts',(51.3139416545903,-49.5212572081901,12.));
#59926=CARTESIAN_POINT('Ctrl Pts',(51.3344083756659,-49.5310325467334,0.));
#59927=CARTESIAN_POINT('Ctrl Pts',(51.3344083756659,-49.5310325467334,12.));
#59928=CARTESIAN_POINT('Ctrl Pts',(51.354925953347,-49.5408068782871,0.));
#59929=CARTESIAN_POINT('Ctrl Pts',(51.354925953347,-49.5408068782871,12.));
#59930=CARTESIAN_POINT('Ctrl Pts',(51.3754942936796,-49.5505800824268,0.));
#59931=CARTESIAN_POINT('Ctrl Pts',(51.3754942936796,-49.5505800824268,12.));
#59932=CARTESIAN_POINT('Ctrl Pts',(51.3961133030688,-49.5603520393514,0.));
#59933=CARTESIAN_POINT('Ctrl Pts',(51.3961133030688,-49.5603520393514,12.));
#59934=CARTESIAN_POINT('Ctrl Pts',(51.4167828882765,-49.5701226298779,0.));
#59935=CARTESIAN_POINT('Ctrl Pts',(51.4167828882765,-49.5701226298779,12.));
#59936=CARTESIAN_POINT('Ctrl Pts',(51.4375029564191,-49.579891735436,0.));
#59937=CARTESIAN_POINT('Ctrl Pts',(51.4375029564191,-49.579891735436,12.));
#59938=CARTESIAN_POINT('Ctrl Pts',(51.4582734149562,-49.5896592380634,0.));
#59939=CARTESIAN_POINT('Ctrl Pts',(51.4582734149562,-49.5896592380634,12.));
#59940=CARTESIAN_POINT('Ctrl Pts',(51.4790941716859,-49.5994250204003,0.));
#59941=CARTESIAN_POINT('Ctrl Pts',(51.4790941716859,-49.5994250204003,12.));
#59942=CARTESIAN_POINT('Ctrl Pts',(51.4999651347496,-49.609188965684,0.));
#59943=CARTESIAN_POINT('Ctrl Pts',(51.4999651347496,-49.609188965684,12.));
#59944=CARTESIAN_POINT('Ctrl Pts',(51.5208862126303,-49.6189509577441,0.));
#59945=CARTESIAN_POINT('Ctrl Pts',(51.5208862126303,-49.6189509577441,12.));
#59946=CARTESIAN_POINT('Ctrl Pts',(51.5418573141494,-49.6287108809975,0.));
#59947=CARTESIAN_POINT('Ctrl Pts',(51.5418573141494,-49.6287108809975,12.));
#59948=CARTESIAN_POINT('Ctrl Pts',(51.5628783484556,-49.6384686204443,0.));
#59949=CARTESIAN_POINT('Ctrl Pts',(51.5628783484556,-49.6384686204443,12.));
#59950=CARTESIAN_POINT('Ctrl Pts',(51.5839492250218,-49.6482240616627,0.));
#59951=CARTESIAN_POINT('Ctrl Pts',(51.5839492250218,-49.6482240616627,12.));
#59952=CARTESIAN_POINT('Ctrl Pts',(51.6050698536525,-49.6579770908063,0.));
#59953=CARTESIAN_POINT('Ctrl Pts',(51.6050698536525,-49.6579770908063,12.));
#59954=CARTESIAN_POINT('Ctrl Pts',(51.6262401444799,-49.6677275945975,0.));
#59955=CARTESIAN_POINT('Ctrl Pts',(51.6262401444799,-49.6677275945975,12.));
#59956=CARTESIAN_POINT('Ctrl Pts',(51.6474600079611,-49.6774754603235,0.));
#59957=CARTESIAN_POINT('Ctrl Pts',(51.6474600079611,-49.6774754603235,12.));
#59958=CARTESIAN_POINT('Ctrl Pts',(51.6687293548656,-49.6872205758314,0.));
#59959=CARTESIAN_POINT('Ctrl Pts',(51.6687293548656,-49.6872205758314,12.));
#59960=CARTESIAN_POINT('Ctrl Pts',(51.6900480962743,-49.6969628295236,0.));
#59961=CARTESIAN_POINT('Ctrl Pts',(51.6900480962743,-49.6969628295236,12.));
#59962=CARTESIAN_POINT('Ctrl Pts',(51.7114161435847,-49.7067021103534,0.));
#59963=CARTESIAN_POINT('Ctrl Pts',(51.7114161435847,-49.7067021103534,12.));
#59964=CARTESIAN_POINT('Ctrl Pts',(51.7328334085084,-49.7164383078206,0.));
#59965=CARTESIAN_POINT('Ctrl Pts',(51.7328334085084,-49.7164383078206,12.));
#59966=CARTESIAN_POINT('Ctrl Pts',(51.7542998030679,-49.7261713119672,0.));
#59967=CARTESIAN_POINT('Ctrl Pts',(51.7542998030679,-49.7261713119672,12.));
#59968=CARTESIAN_POINT('Ctrl Pts',(51.7758152395857,-49.7359010133741,0.));
#59969=CARTESIAN_POINT('Ctrl Pts',(51.7758152395857,-49.7359010133741,12.));
#59970=CARTESIAN_POINT('Ctrl Pts',(51.7973796306826,-49.7456273031555,0.));
#59971=CARTESIAN_POINT('Ctrl Pts',(51.7973796306826,-49.7456273031555,12.));
#59972=CARTESIAN_POINT('Ctrl Pts',(51.8189928892841,-49.7553500729563,0.));
#59973=CARTESIAN_POINT('Ctrl Pts',(51.8189928892841,-49.7553500729563,12.));
#59974=CARTESIAN_POINT('Ctrl Pts',(51.8406549286176,-49.7650692149464,0.));
#59975=CARTESIAN_POINT('Ctrl Pts',(51.8406549286176,-49.7650692149464,12.));
#59976=CARTESIAN_POINT('Ctrl Pts',(51.8623656622092,-49.7747846218177,0.));
#59977=CARTESIAN_POINT('Ctrl Pts',(51.8623656622092,-49.7747846218177,12.));
#59978=CARTESIAN_POINT('Ctrl Pts',(51.8841250038716,-49.78449618678,0.));
#59979=CARTESIAN_POINT('Ctrl Pts',(51.8841250038716,-49.78449618678,12.));
#59980=CARTESIAN_POINT('Ctrl Pts',(51.9059328677051,-49.7942038035568,0.));
#59981=CARTESIAN_POINT('Ctrl Pts',(51.9059328677051,-49.7942038035568,12.));
#59982=CARTESIAN_POINT('Ctrl Pts',(51.9277891681013,-49.8039073663808,0.));
#59983=CARTESIAN_POINT('Ctrl Pts',(51.9277891681013,-49.8039073663808,12.));
#59984=CARTESIAN_POINT('Ctrl Pts',(51.9496938197418,-49.8136067699896,0.));
#59985=CARTESIAN_POINT('Ctrl Pts',(51.9496938197418,-49.8136067699896,12.));
#59986=CARTESIAN_POINT('Ctrl Pts',(51.9716467375938,-49.8233019096224,0.));
#59987=CARTESIAN_POINT('Ctrl Pts',(51.9716467375938,-49.8233019096224,12.));
#59988=CARTESIAN_POINT('Ctrl Pts',(51.9936478369008,-49.8329926810172,0.));
#59989=CARTESIAN_POINT('Ctrl Pts',(51.9936478369008,-49.8329926810172,12.));
#59990=CARTESIAN_POINT('Ctrl Pts',(52.015697033182,-49.8426789804068,0.));
#59991=CARTESIAN_POINT('Ctrl Pts',(52.015697033182,-49.8426789804068,12.));
#59992=CARTESIAN_POINT('Ctrl Pts',(52.0377942422373,-49.8523607045146,0.));
#59993=CARTESIAN_POINT('Ctrl Pts',(52.0377942422373,-49.8523607045146,12.));
#59994=CARTESIAN_POINT('Ctrl Pts',(52.059939380145,-49.8620377505498,0.));
#59995=CARTESIAN_POINT('Ctrl Pts',(52.059939380145,-49.8620377505498,12.));
#59996=CARTESIAN_POINT('Ctrl Pts',(52.0821323632588,-49.871710016205,0.));
#59997=CARTESIAN_POINT('Ctrl Pts',(52.0821323632588,-49.871710016205,12.));
#59998=CARTESIAN_POINT('Ctrl Pts',(52.1043731081968,-49.8813773996523,0.));
#59999=CARTESIAN_POINT('Ctrl Pts',(52.1043731081968,-49.8813773996523,12.));
#60000=CARTESIAN_POINT('Ctrl Pts',(52.1266615318414,-49.8910397995404,0.));
#60001=CARTESIAN_POINT('Ctrl Pts',(52.1266615318414,-49.8910397995404,12.));
#60002=CARTESIAN_POINT('Ctrl Pts',(52.1489975513449,-49.90069711499,0.));
#60003=CARTESIAN_POINT('Ctrl Pts',(52.1489975513449,-49.90069711499,12.));
#60004=CARTESIAN_POINT('Ctrl Pts',(52.1713810841277,-49.9103492455904,0.));
#60005=CARTESIAN_POINT('Ctrl Pts',(52.1713810841277,-49.9103492455904,12.));
#60006=CARTESIAN_POINT('Ctrl Pts',(52.1938120478752,-49.919996091396,0.));
#60007=CARTESIAN_POINT('Ctrl Pts',(52.1938120478752,-49.919996091396,12.));
#60008=CARTESIAN_POINT('Ctrl Pts',(52.2162903605272,-49.9296375529241,0.));
#60009=CARTESIAN_POINT('Ctrl Pts',(52.2162903605272,-49.9296375529241,12.));
#60010=CARTESIAN_POINT('Ctrl Pts',(52.238815940277,-49.9392735311507,0.));
#60011=CARTESIAN_POINT('Ctrl Pts',(52.238815940277,-49.9392735311507,12.));
#60012=CARTESIAN_POINT('Ctrl Pts',(52.2613887055773,-49.9489039275064,0.));
#60013=CARTESIAN_POINT('Ctrl Pts',(52.2613887055773,-49.9489039275064,12.));
#60014=CARTESIAN_POINT('Ctrl Pts',(52.2840085751385,-49.9585286438734,0.));
#60015=CARTESIAN_POINT('Ctrl Pts',(52.2840085751385,-49.9585286438734,12.));
#60016=CARTESIAN_POINT('Ctrl Pts',(52.3066754679264,-49.9681475825824,0.));
#60017=CARTESIAN_POINT('Ctrl Pts',(52.3066754679264,-49.9681475825824,12.));
#60018=CARTESIAN_POINT('Ctrl Pts',(52.3293893031524,-49.9777606464103,0.));
#60019=CARTESIAN_POINT('Ctrl Pts',(52.3293893031524,-49.9777606464103,12.));
#60020=CARTESIAN_POINT('Ctrl Pts',(52.3521500002711,-49.9873677385769,0.));
#60021=CARTESIAN_POINT('Ctrl Pts',(52.3521500002711,-49.9873677385769,12.));
#60022=CARTESIAN_POINT('Ctrl Pts',(52.3749574789865,-49.9969687627402,0.));
#60023=CARTESIAN_POINT('Ctrl Pts',(52.3749574789865,-49.9969687627402,12.));
#60024=CARTESIAN_POINT('Ctrl Pts',(52.3978116592505,-50.0065636229934,0.));
#60025=CARTESIAN_POINT('Ctrl Pts',(52.3978116592505,-50.0065636229934,12.));
#60026=CARTESIAN_POINT('Ctrl Pts',(52.420712461261,-50.0161522238619,0.));
#60027=CARTESIAN_POINT('Ctrl Pts',(52.420712461261,-50.0161522238619,12.));
#60028=CARTESIAN_POINT('Ctrl Pts',(52.4436598054523,-50.0257344703008,0.));
#60029=CARTESIAN_POINT('Ctrl Pts',(52.4436598054523,-50.0257344703008,12.));
#60030=CARTESIAN_POINT('Ctrl Pts',(52.4666536124926,-50.0353102676933,0.));
#60031=CARTESIAN_POINT('Ctrl Pts',(52.4666536124926,-50.0353102676933,12.));
#60032=CARTESIAN_POINT('Ctrl Pts',(52.4896938032896,-50.0448795218453,0.));
#60033=CARTESIAN_POINT('Ctrl Pts',(52.4896938032896,-50.0448795218453,12.));
#60034=CARTESIAN_POINT('Ctrl Pts',(52.5127802989903,-50.0544421389824,0.));
#60035=CARTESIAN_POINT('Ctrl Pts',(52.5127802989903,-50.0544421389824,12.));
#60036=CARTESIAN_POINT('Ctrl Pts',(52.5359130209789,-50.0639980257477,0.));
#60037=CARTESIAN_POINT('Ctrl Pts',(52.5359130209789,-50.0639980257477,12.));
#60038=CARTESIAN_POINT('Ctrl Pts',(52.5590918908691,-50.0735470891996,0.));
#60039=CARTESIAN_POINT('Ctrl Pts',(52.5590918908691,-50.0735470891996,12.));
#60040=CARTESIAN_POINT('Ctrl Pts',(52.5823168304981,-50.0830892368095,0.));
#60041=CARTESIAN_POINT('Ctrl Pts',(52.5823168304981,-50.0830892368095,12.));
#60042=CARTESIAN_POINT('Ctrl Pts',(52.6055877619338,-50.0926243764569,0.));
#60043=CARTESIAN_POINT('Ctrl Pts',(52.6055877619338,-50.0926243764569,12.));
#60044=CARTESIAN_POINT('Ctrl Pts',(52.6289046074743,-50.1021524164261,0.));
#60045=CARTESIAN_POINT('Ctrl Pts',(52.6289046074743,-50.1021524164261,12.));
#60046=CARTESIAN_POINT('Ctrl Pts',(52.6522672896462,-50.1116732654041,0.));
#60047=CARTESIAN_POINT('Ctrl Pts',(52.6522672896462,-50.1116732654041,12.));
#60048=CARTESIAN_POINT('Ctrl Pts',(52.6756757311979,-50.1211868324781,0.));
#60049=CARTESIAN_POINT('Ctrl Pts',(52.6756757311979,-50.1211868324781,12.));
#60050=CARTESIAN_POINT('Ctrl Pts',(52.6991298550928,-50.1306930271343,0.));
#60051=CARTESIAN_POINT('Ctrl Pts',(52.6991298550928,-50.1306930271343,12.));
#60052=CARTESIAN_POINT('Ctrl Pts',(52.7226295845155,-50.1401917592532,0.));
#60053=CARTESIAN_POINT('Ctrl Pts',(52.7226295845155,-50.1401917592532,12.));
#60054=CARTESIAN_POINT('Ctrl Pts',(52.7461748428733,-50.1496829391068,0.));
#60055=CARTESIAN_POINT('Ctrl Pts',(52.7461748428733,-50.1496829391068,12.));
#60056=CARTESIAN_POINT('Ctrl Pts',(52.769765553794,-50.1591664773561,0.));
#60057=CARTESIAN_POINT('Ctrl Pts',(52.769765553794,-50.1591664773561,12.));
#60058=CARTESIAN_POINT('Ctrl Pts',(52.793401641121,-50.1686422850493,0.));
#60059=CARTESIAN_POINT('Ctrl Pts',(52.793401641121,-50.1686422850493,12.));
#60060=CARTESIAN_POINT('Ctrl Pts',(52.8170830289052,-50.1781102736215,0.));
#60061=CARTESIAN_POINT('Ctrl Pts',(52.8170830289052,-50.1781102736215,12.));
#60062=CARTESIAN_POINT('Ctrl Pts',(52.8408096414101,-50.1875703548893,0.));
#60063=CARTESIAN_POINT('Ctrl Pts',(52.8408096414101,-50.1875703548893,12.));
#60064=CARTESIAN_POINT('Ctrl Pts',(52.8645814031137,-50.1970224410476,0.));
#60065=CARTESIAN_POINT('Ctrl Pts',(52.8645814031137,-50.1970224410476,12.));
#60066=CARTESIAN_POINT('Ctrl Pts',(52.8883982387068,-50.2064664446663,0.));
#60067=CARTESIAN_POINT('Ctrl Pts',(52.8883982387068,-50.2064664446663,12.));
#60068=CARTESIAN_POINT('Ctrl Pts',(52.9122600730882,-50.2159022786876,0.));
#60069=CARTESIAN_POINT('Ctrl Pts',(52.9122600730882,-50.2159022786876,12.));
#60070=CARTESIAN_POINT('Ctrl Pts',(52.9361668313539,-50.2253298564237,0.));
#60071=CARTESIAN_POINT('Ctrl Pts',(52.9361668313539,-50.2253298564237,12.));
#60072=CARTESIAN_POINT('Ctrl Pts',(52.9601184388027,-50.2347490915553,0.));
#60073=CARTESIAN_POINT('Ctrl Pts',(52.9601184388027,-50.2347490915553,12.));
#60074=CARTESIAN_POINT('Ctrl Pts',(52.9841148209404,-50.2441598981286,0.));
#60075=CARTESIAN_POINT('Ctrl Pts',(52.9841148209404,-50.2441598981286,12.));
#60076=CARTESIAN_POINT('Ctrl Pts',(53.0081559034802,-50.2535621905553,0.));
#60077=CARTESIAN_POINT('Ctrl Pts',(53.0081559034802,-50.2535621905553,12.));
#60078=CARTESIAN_POINT('Ctrl Pts',(53.0322416123404,-50.2629558836111,0.));
#60079=CARTESIAN_POINT('Ctrl Pts',(53.0322416123404,-50.2629558836111,12.));
#60080=CARTESIAN_POINT('Ctrl Pts',(53.0563718736361,-50.272340892437,0.));
#60081=CARTESIAN_POINT('Ctrl Pts',(53.0563718736361,-50.272340892437,12.));
#60082=CARTESIAN_POINT('Ctrl Pts',(53.0805466136791,-50.2817171325354,0.));
#60083=CARTESIAN_POINT('Ctrl Pts',(53.0805466136791,-50.2817171325354,12.));
#60084=CARTESIAN_POINT('Ctrl Pts',(53.1047657589806,-50.2910845197615,0.));
#60085=CARTESIAN_POINT('Ctrl Pts',(53.1047657589806,-50.2910845197615,12.));
#60086=CARTESIAN_POINT('Ctrl Pts',(53.1290292362482,-50.3004429703188,0.));
#60087=CARTESIAN_POINT('Ctrl Pts',(53.1290292362482,-50.3004429703188,12.));
#60088=CARTESIAN_POINT('Ctrl Pts',(53.153336972382,-50.3097924007536,0.));
#60089=CARTESIAN_POINT('Ctrl Pts',(53.153336972382,-50.3097924007536,12.));
#60090=CARTESIAN_POINT('Ctrl Pts',(53.1776888944622,-50.3191327279497,0.));
#60091=CARTESIAN_POINT('Ctrl Pts',(53.1776888944622,-50.3191327279497,12.));
#60092=CARTESIAN_POINT('Ctrl Pts',(53.202084929748,-50.3284638691285,0.));
#60093=CARTESIAN_POINT('Ctrl Pts',(53.202084929748,-50.3284638691285,12.));
#60094=CARTESIAN_POINT('Ctrl Pts',(53.2265250056896,-50.3377857418522,0.));
#60095=CARTESIAN_POINT('Ctrl Pts',(53.2265250056896,-50.3377857418522,12.));
#60096=CARTESIAN_POINT('Ctrl Pts',(53.2510090499341,-50.3470982640294,0.));
#60097=CARTESIAN_POINT('Ctrl Pts',(53.2510090499341,-50.3470982640294,12.));
#60098=CARTESIAN_POINT('Ctrl Pts',(53.2755369903291,-50.3564013539198,0.));
#60099=CARTESIAN_POINT('Ctrl Pts',(53.2755369903291,-50.3564013539198,12.));
#60100=CARTESIAN_POINT('Ctrl Pts',(53.3001087549222,-50.3656949301424,0.));
#60101=CARTESIAN_POINT('Ctrl Pts',(53.3001087549222,-50.3656949301424,12.));
#60102=CARTESIAN_POINT('Ctrl Pts',(53.3247242719575,-50.3749789116777,0.));
#60103=CARTESIAN_POINT('Ctrl Pts',(53.3247242719575,-50.3749789116777,12.));
#60104=CARTESIAN_POINT('Ctrl Pts',(53.3493834698685,-50.3842532178451,0.));
#60105=CARTESIAN_POINT('Ctrl Pts',(53.3493834698685,-50.3842532178451,12.));
#60106=CARTESIAN_POINT('Ctrl Pts',(53.3740862772673,-50.393517768283,0.));
#60107=CARTESIAN_POINT('Ctrl Pts',(53.3740862772673,-50.393517768283,12.));
#60108=CARTESIAN_POINT('Ctrl Pts',(53.3988326229308,-50.4027724829296,0.));
#60109=CARTESIAN_POINT('Ctrl Pts',(53.3988326229308,-50.4027724829296,12.));
#60110=CARTESIAN_POINT('Ctrl Pts',(53.4236224357846,-50.4120172820054,0.));
#60111=CARTESIAN_POINT('Ctrl Pts',(53.4236224357846,-50.4120172820054,12.));
#60112=CARTESIAN_POINT('Ctrl Pts',(53.4484556448787,-50.4212520859924,0.));
#60113=CARTESIAN_POINT('Ctrl Pts',(53.4484556448787,-50.4212520859924,12.));
#60114=CARTESIAN_POINT('Ctrl Pts',(53.4733321794199,-50.4304768156677,0.));
#60115=CARTESIAN_POINT('Ctrl Pts',(53.4733321794199,-50.4304768156677,12.));
#60116=CARTESIAN_POINT('Ctrl Pts',(53.4982519688032,-50.4396913921389,0.));
#60117=CARTESIAN_POINT('Ctrl Pts',(53.4982519688032,-50.4396913921389,12.));
#60118=CARTESIAN_POINT('Ctrl Pts',(53.5232149426415,-50.4488957368841,0.));
#60119=CARTESIAN_POINT('Ctrl Pts',(53.5232149426415,-50.4488957368841,12.));
#60120=CARTESIAN_POINT('Ctrl Pts',(53.5482210307864,-50.4580897717835,0.));
#60121=CARTESIAN_POINT('Ctrl Pts',(53.5482210307864,-50.4580897717835,12.));
#60122=CARTESIAN_POINT('Ctrl Pts',(53.5732701633602,-50.467273419175,0.));
#60123=CARTESIAN_POINT('Ctrl Pts',(53.5732701633602,-50.467273419175,12.));
#60124=CARTESIAN_POINT('Ctrl Pts',(53.5983622707231,-50.4764466018064,0.));
#60125=CARTESIAN_POINT('Ctrl Pts',(53.5983622707231,-50.4764466018064,12.));
#60126=CARTESIAN_POINT('Ctrl Pts',(53.6234972834055,-50.485609242731,0.));
#60127=CARTESIAN_POINT('Ctrl Pts',(53.6234972834055,-50.485609242731,12.));
#60128=CARTESIAN_POINT('Ctrl Pts',(53.6486751320434,-50.4947612652147,0.));
#60129=CARTESIAN_POINT('Ctrl Pts',(53.6486751320434,-50.4947612652147,12.));
#60130=CARTESIAN_POINT('Ctrl Pts',(53.6738957473158,-50.5039025926531,0.));
#60131=CARTESIAN_POINT('Ctrl Pts',(53.6738957473158,-50.5039025926531,12.));
#60132=CARTESIAN_POINT('Ctrl Pts',(53.6991590598551,-50.5130331484563,0.));
#60133=CARTESIAN_POINT('Ctrl Pts',(53.6991590598551,-50.5130331484563,12.));
#60134=CARTESIAN_POINT('Ctrl Pts',(53.7244650002382,-50.5221528560427,0.));
#60135=CARTESIAN_POINT('Ctrl Pts',(53.7244650002382,-50.5221528560427,12.));
#60136=CARTESIAN_POINT('Ctrl Pts',(53.7498134991714,-50.5312616390789,0.));
#60137=CARTESIAN_POINT('Ctrl Pts',(53.7498134991714,-50.5312616390789,12.));
#60138=CARTESIAN_POINT('Ctrl Pts',(53.7752044876312,-50.5403594216706,0.));
#60139=CARTESIAN_POINT('Ctrl Pts',(53.7752044876312,-50.5403594216706,12.));
#60140=CARTESIAN_POINT('Ctrl Pts',(53.8006378970198,-50.5494461285762,0.));
#60141=CARTESIAN_POINT('Ctrl Pts',(53.8006378970198,-50.5494461285762,12.));
#60142=CARTESIAN_POINT('Ctrl Pts',(53.8261136593064,-50.5585216854082,0.));
#60143=CARTESIAN_POINT('Ctrl Pts',(53.8261136593064,-50.5585216854082,12.));
#60144=CARTESIAN_POINT('Ctrl Pts',(53.8516317071783,-50.567586018852,0.));
#60145=CARTESIAN_POINT('Ctrl Pts',(53.8516317071783,-50.567586018852,12.));
#60146=CARTESIAN_POINT('Ctrl Pts',(53.8771919737007,-50.5766390561861,0.));
#60147=CARTESIAN_POINT('Ctrl Pts',(53.8771919737007,-50.5766390561861,12.));
#60148=CARTESIAN_POINT('Ctrl Pts',(53.9027943919814,-50.5856807248133,0.));
#60149=CARTESIAN_POINT('Ctrl Pts',(53.9027943919814,-50.5856807248133,12.));
#60150=CARTESIAN_POINT('Ctrl Pts',(53.9284388947996,-50.5947109517476,0.));
#60151=CARTESIAN_POINT('Ctrl Pts',(53.9284388947996,-50.5947109517476,12.));
#60152=CARTESIAN_POINT('Ctrl Pts',(53.954125414313,-50.603729663215,0.));
#60153=CARTESIAN_POINT('Ctrl Pts',(53.954125414313,-50.603729663215,12.));
#60154=CARTESIAN_POINT('Ctrl Pts',(53.9798538815561,-50.6127367839738,0.));
#60155=CARTESIAN_POINT('Ctrl Pts',(53.9798538815561,-50.6127367839738,12.));
#60156=CARTESIAN_POINT('Ctrl Pts',(54.0056242268443,-50.6217322378686,0.));
#60157=CARTESIAN_POINT('Ctrl Pts',(54.0056242268443,-50.6217322378686,12.));
#60158=CARTESIAN_POINT('Ctrl Pts',(54.0314363806751,-50.630715949059,0.));
#60159=CARTESIAN_POINT('Ctrl Pts',(54.0314363806751,-50.630715949059,12.));
#60160=CARTESIAN_POINT('Ctrl Pts',(54.0572902745101,-50.6396878430961,0.));
#60161=CARTESIAN_POINT('Ctrl Pts',(54.0572902745101,-50.6396878430961,12.));
#60162=CARTESIAN_POINT('Ctrl Pts',(54.0831858415182,-50.648647847946,0.));
#60163=CARTESIAN_POINT('Ctrl Pts',(54.0831858415182,-50.648647847946,12.));
#60164=CARTESIAN_POINT('Ctrl Pts',(54.1091230175319,-50.657595895318,0.));
#60165=CARTESIAN_POINT('Ctrl Pts',(54.1091230175319,-50.657595895318,12.));
#60166=CARTESIAN_POINT('Ctrl Pts',(54.1351017412721,-50.6665319209798,0.));
#60167=CARTESIAN_POINT('Ctrl Pts',(54.1351017412721,-50.6665319209798,12.));
#60168=CARTESIAN_POINT('Ctrl Pts',(54.1611219522299,-50.6754558618218,0.));
#60169=CARTESIAN_POINT('Ctrl Pts',(54.1611219522299,-50.6754558618218,12.));
#60170=CARTESIAN_POINT('Ctrl Pts',(54.1871835889908,-50.6843676535428,0.));
#60171=CARTESIAN_POINT('Ctrl Pts',(54.1871835889908,-50.6843676535428,12.));
#60172=CARTESIAN_POINT('Ctrl Pts',(54.2132865872968,-50.6932672279758,0.));
#60173=CARTESIAN_POINT('Ctrl Pts',(54.2132865872968,-50.6932672279758,12.));
#60174=CARTESIAN_POINT('Ctrl Pts',(54.2394308784093,-50.7021545108369,0.));
#60175=CARTESIAN_POINT('Ctrl Pts',(54.2394308784093,-50.7021545108369,12.));
#60176=CARTESIAN_POINT('Ctrl Pts',(54.2656163868258,-50.7110294185832,0.));
#60177=CARTESIAN_POINT('Ctrl Pts',(54.2656163868258,-50.7110294185832,12.));
#60178=CARTESIAN_POINT('Ctrl Pts',(54.2918430335414,-50.7198918629632,0.));
#60179=CARTESIAN_POINT('Ctrl Pts',(54.2918430335414,-50.7198918629632,12.));
#60180=CARTESIAN_POINT('Ctrl Pts',(54.3181107400862,-50.7287417566296,0.));
#60181=CARTESIAN_POINT('Ctrl Pts',(54.3181107400862,-50.7287417566296,12.));
#60182=CARTESIAN_POINT('Ctrl Pts',(54.344419432416,-50.7375790185988,0.));
#60183=CARTESIAN_POINT('Ctrl Pts',(54.344419432416,-50.7375790185988,12.));
#60184=CARTESIAN_POINT('Ctrl Pts',(54.3707690445679,-50.7464035792846,0.));
#60185=CARTESIAN_POINT('Ctrl Pts',(54.3707690445679,-50.7464035792846,12.));
#60186=CARTESIAN_POINT('Ctrl Pts',(54.3971595231285,-50.7552153869224,0.));
#60187=CARTESIAN_POINT('Ctrl Pts',(54.3971595231285,-50.7552153869224,12.));
#60188=CARTESIAN_POINT('Ctrl Pts',(54.4235908287188,-50.7640144089601,0.));
#60189=CARTESIAN_POINT('Ctrl Pts',(54.4235908287188,-50.7640144089601,12.));
#60190=CARTESIAN_POINT('Ctrl Pts',(54.4500629335867,-50.772800626886,0.));
#60191=CARTESIAN_POINT('Ctrl Pts',(54.4500629335867,-50.772800626886,12.));
#60192=CARTESIAN_POINT('Ctrl Pts',(54.4712732428597,-50.7798193515479,0.));
#60193=CARTESIAN_POINT('Ctrl Pts',(54.4712732428597,-50.7798193515479,12.));
#60194=CARTESIAN_POINT('Ctrl Pts',(54.4871993224549,-50.7850776288567,0.));
#60195=CARTESIAN_POINT('Ctrl Pts',(54.4871993224549,-50.7850776288567,12.));
#60196=CARTESIAN_POINT('Ctrl Pts',(54.4978248630284,-50.7885805844191,0.));
#60197=CARTESIAN_POINT('Ctrl Pts',(54.4978248630284,-50.7885805844191,12.));
#60198=CARTESIAN_POINT('Ctrl Pts',(54.5031396718592,-50.7903314215393,0.));
#60199=CARTESIAN_POINT('Ctrl Pts',(54.5031396718592,-50.7903314215393,12.));
#60200=CARTESIAN_POINT('',(50.0975384783634,-48.8900464144686,0.));
#60201=CARTESIAN_POINT('Ctrl Pts',(50.0975384783634,-48.8900464144686,0.));
#60202=CARTESIAN_POINT('Ctrl Pts',(50.1009206494209,-48.8919551910299,0.));
#60203=CARTESIAN_POINT('Ctrl Pts',(50.1076907555303,-48.8957735556681,0.));
#60204=CARTESIAN_POINT('Ctrl Pts',(50.1178632066821,-48.9015035371772,0.));
#60205=CARTESIAN_POINT('Ctrl Pts',(50.1314610602286,-48.9091483817797,0.));
#60206=CARTESIAN_POINT('Ctrl Pts',(50.148516018447,-48.9187125417897,0.));
#60207=CARTESIAN_POINT('Ctrl Pts',(50.1656286003943,-48.9282847698237,0.));
#60208=CARTESIAN_POINT('Ctrl Pts',(50.1827987615659,-48.9378649933116,0.));
#60209=CARTESIAN_POINT('Ctrl Pts',(50.2000264157903,-48.9474530868847,0.));
#60210=CARTESIAN_POINT('Ctrl Pts',(50.2173114358423,-48.9570488741273,0.));
#60211=CARTESIAN_POINT('Ctrl Pts',(50.2346536715465,-48.9666521500969,0.));
#60212=CARTESIAN_POINT('Ctrl Pts',(50.252052963548,-48.9762626987227,0.));
#60213=CARTESIAN_POINT('Ctrl Pts',(50.2695091583472,-48.9858803116649,0.));
#60214=CARTESIAN_POINT('Ctrl Pts',(50.2870221241003,-48.9955048082028,0.));
#60215=CARTESIAN_POINT('Ctrl Pts',(50.3045917455383,-49.0051360288002,0.));
#60216=CARTESIAN_POINT('Ctrl Pts',(50.3222179165102,-49.0147738256925,0.));
#60217=CARTESIAN_POINT('Ctrl Pts',(50.3399005337967,-49.0244180550759,0.));
#60218=CARTESIAN_POINT('Ctrl Pts',(50.3576394894136,-49.034068567401,0.));
#60219=CARTESIAN_POINT('Ctrl Pts',(50.3754346667389,-49.0437252024868,0.));
#60220=CARTESIAN_POINT('Ctrl Pts',(50.393285944528,-49.0533877945771,0.));
#60221=CARTESIAN_POINT('Ctrl Pts',(50.4111931994264,-49.0630561755082,0.));
#60222=CARTESIAN_POINT('Ctrl Pts',(50.4291563088528,-49.0727301783477,0.));
#60223=CARTESIAN_POINT('Ctrl Pts',(50.4471751542717,-49.0824096415339,0.));
#60224=CARTESIAN_POINT('Ctrl Pts',(50.465249621057,-49.0920944086973,0.));
#60225=CARTESIAN_POINT('Ctrl Pts',(50.4833795969296,-49.1017843266782,0.));
#60226=CARTESIAN_POINT('Ctrl Pts',(50.5015649708742,-49.1114792441573,0.));
#60227=CARTESIAN_POINT('Ctrl Pts',(50.5198056318111,-49.1211790099817,0.));
#60228=CARTESIAN_POINT('Ctrl Pts',(50.5381014674822,-49.1308834717645,0.));
#60229=CARTESIAN_POINT('Ctrl Pts',(50.5564523650406,-49.1405924766169,0.));
#60230=CARTESIAN_POINT('Ctrl Pts',(50.5748582115575,-49.1503058717831,0.));
#60231=CARTESIAN_POINT('Ctrl Pts',(50.593318894516,-49.1600235052613,0.));
#60232=CARTESIAN_POINT('Ctrl Pts',(50.6118343023937,-49.1697452265473,0.));
#60233=CARTESIAN_POINT('Ctrl Pts',(50.6304043248796,-49.1794708869074,0.));
#60234=CARTESIAN_POINT('Ctrl Pts',(50.6490288525639,-49.1892003389743,0.));
#60235=CARTESIAN_POINT('Ctrl Pts',(50.6677077767427,-49.1989334364992,0.));
#60236=CARTESIAN_POINT('Ctrl Pts',(50.6864409891905,-49.2086700340625,0.));
#60237=CARTESIAN_POINT('Ctrl Pts',(50.7052283818941,-49.218409986748,0.));
#60238=CARTESIAN_POINT('Ctrl Pts',(50.7240698470698,-49.2281531501569,0.));
#60239=CARTESIAN_POINT('Ctrl Pts',(50.7429652772816,-49.2378993805482,0.));
#60240=CARTESIAN_POINT('Ctrl Pts',(50.7619145655207,-49.2476485349373,0.));
#60241=CARTESIAN_POINT('Ctrl Pts',(50.7809176052954,-49.2574004712122,0.));
#60242=CARTESIAN_POINT('Ctrl Pts',(50.799974290711,-49.2671550482415,0.));
#60243=CARTESIAN_POINT('Ctrl Pts',(50.8190845164319,-49.2769121258144,0.));
#60244=CARTESIAN_POINT('Ctrl Pts',(50.8382481776392,-49.2866715645828,0.));
#60245=CARTESIAN_POINT('Ctrl Pts',(50.8574651699877,-49.2964332260043,0.));
#60246=CARTESIAN_POINT('Ctrl Pts',(50.8767353895509,-49.3061969722798,0.));
#60247=CARTESIAN_POINT('Ctrl Pts',(50.8960587327869,-49.3159626663129,0.));
#60248=CARTESIAN_POINT('Ctrl Pts',(50.9154350965681,-49.325730171735,0.));
#60249=CARTESIAN_POINT('Ctrl Pts',(50.9348643781928,-49.3354993529163,0.));
#60250=CARTESIAN_POINT('Ctrl Pts',(50.9543464753974,-49.3452700749804,0.));
#60251=CARTESIAN_POINT('Ctrl Pts',(50.9738812863635,-49.3550422038221,0.));
#60252=CARTESIAN_POINT('Ctrl Pts',(50.9934687097179,-49.3648156061049,0.));
#60253=CARTESIAN_POINT('Ctrl Pts',(51.0131086445268,-49.3745901492429,0.));
#60254=CARTESIAN_POINT('Ctrl Pts',(51.0328009902857,-49.3843657013851,0.));
#60255=CARTESIAN_POINT('Ctrl Pts',(51.0525456469072,-49.3941421314014,0.));
#60256=CARTESIAN_POINT('Ctrl Pts',(51.0723425146987,-49.4039193088636,0.));
#60257=CARTESIAN_POINT('Ctrl Pts',(51.0921914943663,-49.4136971040428,0.));
#60258=CARTESIAN_POINT('Ctrl Pts',(51.1120924870196,-49.4234753879071,0.));
#60259=CARTESIAN_POINT('Ctrl Pts',(51.1320453941702,-49.4332540321178,0.));
#60260=CARTESIAN_POINT('Ctrl Pts',(51.1520501177291,-49.4430329090288,0.));
#60261=CARTESIAN_POINT('Ctrl Pts',(51.1721065599972,-49.4528118916833,0.));
#60262=CARTESIAN_POINT('Ctrl Pts',(51.1922146236686,-49.4625908538076,0.));
#60263=CARTESIAN_POINT('Ctrl Pts',(51.2123742118288,-49.4723696698022,0.));
#60264=CARTESIAN_POINT('Ctrl Pts',(51.2325852279507,-49.4821482147357,0.));
#60265=CARTESIAN_POINT('Ctrl Pts',(51.2528475758841,-49.4919263643357,0.));
#60266=CARTESIAN_POINT('Ctrl Pts',(51.2731611598465,-49.5017039949841,0.));
#60267=CARTESIAN_POINT('Ctrl Pts',(51.2935258844278,-49.5114809837111,0.));
#60268=CARTESIAN_POINT('Ctrl Pts',(51.3139416545903,-49.5212572081901,0.));
#60269=CARTESIAN_POINT('Ctrl Pts',(51.3344083756659,-49.5310325467334,0.));
#60270=CARTESIAN_POINT('Ctrl Pts',(51.354925953347,-49.5408068782871,0.));
#60271=CARTESIAN_POINT('Ctrl Pts',(51.3754942936796,-49.5505800824268,0.));
#60272=CARTESIAN_POINT('Ctrl Pts',(51.3961133030688,-49.5603520393514,0.));
#60273=CARTESIAN_POINT('Ctrl Pts',(51.4167828882765,-49.5701226298779,0.));
#60274=CARTESIAN_POINT('Ctrl Pts',(51.4375029564191,-49.579891735436,0.));
#60275=CARTESIAN_POINT('Ctrl Pts',(51.4582734149562,-49.5896592380634,0.));
#60276=CARTESIAN_POINT('Ctrl Pts',(51.4790941716859,-49.5994250204003,0.));
#60277=CARTESIAN_POINT('Ctrl Pts',(51.4999651347496,-49.609188965684,0.));
#60278=CARTESIAN_POINT('Ctrl Pts',(51.5208862126303,-49.6189509577441,0.));
#60279=CARTESIAN_POINT('Ctrl Pts',(51.5418573141494,-49.6287108809975,0.));
#60280=CARTESIAN_POINT('Ctrl Pts',(51.5628783484556,-49.6384686204443,0.));
#60281=CARTESIAN_POINT('Ctrl Pts',(51.5839492250218,-49.6482240616627,0.));
#60282=CARTESIAN_POINT('Ctrl Pts',(51.6050698536525,-49.6579770908063,0.));
#60283=CARTESIAN_POINT('Ctrl Pts',(51.6262401444799,-49.6677275945975,0.));
#60284=CARTESIAN_POINT('Ctrl Pts',(51.6474600079611,-49.6774754603235,0.));
#60285=CARTESIAN_POINT('Ctrl Pts',(51.6687293548656,-49.6872205758314,0.));
#60286=CARTESIAN_POINT('Ctrl Pts',(51.6900480962743,-49.6969628295236,0.));
#60287=CARTESIAN_POINT('Ctrl Pts',(51.7114161435847,-49.7067021103534,0.));
#60288=CARTESIAN_POINT('Ctrl Pts',(51.7328334085084,-49.7164383078206,0.));
#60289=CARTESIAN_POINT('Ctrl Pts',(51.7542998030679,-49.7261713119672,0.));
#60290=CARTESIAN_POINT('Ctrl Pts',(51.7758152395857,-49.7359010133741,0.));
#60291=CARTESIAN_POINT('Ctrl Pts',(51.7973796306826,-49.7456273031555,0.));
#60292=CARTESIAN_POINT('Ctrl Pts',(51.8189928892841,-49.7553500729563,0.));
#60293=CARTESIAN_POINT('Ctrl Pts',(51.8406549286176,-49.7650692149464,0.));
#60294=CARTESIAN_POINT('Ctrl Pts',(51.8623656622092,-49.7747846218177,0.));
#60295=CARTESIAN_POINT('Ctrl Pts',(51.8841250038716,-49.78449618678,0.));
#60296=CARTESIAN_POINT('Ctrl Pts',(51.9059328677051,-49.7942038035568,0.));
#60297=CARTESIAN_POINT('Ctrl Pts',(51.9277891681013,-49.8039073663808,0.));
#60298=CARTESIAN_POINT('Ctrl Pts',(51.9496938197418,-49.8136067699896,0.));
#60299=CARTESIAN_POINT('Ctrl Pts',(51.9716467375938,-49.8233019096224,0.));
#60300=CARTESIAN_POINT('Ctrl Pts',(51.9936478369008,-49.8329926810172,0.));
#60301=CARTESIAN_POINT('Ctrl Pts',(52.015697033182,-49.8426789804068,0.));
#60302=CARTESIAN_POINT('Ctrl Pts',(52.0377942422373,-49.8523607045146,0.));
#60303=CARTESIAN_POINT('Ctrl Pts',(52.059939380145,-49.8620377505498,0.));
#60304=CARTESIAN_POINT('Ctrl Pts',(52.0821323632588,-49.871710016205,0.));
#60305=CARTESIAN_POINT('Ctrl Pts',(52.1043731081968,-49.8813773996523,0.));
#60306=CARTESIAN_POINT('Ctrl Pts',(52.1266615318414,-49.8910397995404,0.));
#60307=CARTESIAN_POINT('Ctrl Pts',(52.1489975513449,-49.90069711499,0.));
#60308=CARTESIAN_POINT('Ctrl Pts',(52.1713810841277,-49.9103492455904,0.));
#60309=CARTESIAN_POINT('Ctrl Pts',(52.1938120478752,-49.919996091396,0.));
#60310=CARTESIAN_POINT('Ctrl Pts',(52.2162903605272,-49.9296375529241,0.));
#60311=CARTESIAN_POINT('Ctrl Pts',(52.238815940277,-49.9392735311507,0.));
#60312=CARTESIAN_POINT('Ctrl Pts',(52.2613887055773,-49.9489039275064,0.));
#60313=CARTESIAN_POINT('Ctrl Pts',(52.2840085751385,-49.9585286438734,0.));
#60314=CARTESIAN_POINT('Ctrl Pts',(52.3066754679264,-49.9681475825824,0.));
#60315=CARTESIAN_POINT('Ctrl Pts',(52.3293893031524,-49.9777606464103,0.));
#60316=CARTESIAN_POINT('Ctrl Pts',(52.3521500002711,-49.9873677385769,0.));
#60317=CARTESIAN_POINT('Ctrl Pts',(52.3749574789865,-49.9969687627402,0.));
#60318=CARTESIAN_POINT('Ctrl Pts',(52.3978116592505,-50.0065636229934,0.));
#60319=CARTESIAN_POINT('Ctrl Pts',(52.420712461261,-50.0161522238619,0.));
#60320=CARTESIAN_POINT('Ctrl Pts',(52.4436598054523,-50.0257344703008,0.));
#60321=CARTESIAN_POINT('Ctrl Pts',(52.4666536124926,-50.0353102676933,0.));
#60322=CARTESIAN_POINT('Ctrl Pts',(52.4896938032896,-50.0448795218453,0.));
#60323=CARTESIAN_POINT('Ctrl Pts',(52.5127802989903,-50.0544421389824,0.));
#60324=CARTESIAN_POINT('Ctrl Pts',(52.5359130209789,-50.0639980257477,0.));
#60325=CARTESIAN_POINT('Ctrl Pts',(52.5590918908691,-50.0735470891996,0.));
#60326=CARTESIAN_POINT('Ctrl Pts',(52.5823168304981,-50.0830892368095,0.));
#60327=CARTESIAN_POINT('Ctrl Pts',(52.6055877619338,-50.0926243764569,0.));
#60328=CARTESIAN_POINT('Ctrl Pts',(52.6289046074743,-50.1021524164261,0.));
#60329=CARTESIAN_POINT('Ctrl Pts',(52.6522672896462,-50.1116732654041,0.));
#60330=CARTESIAN_POINT('Ctrl Pts',(52.6756757311979,-50.1211868324781,0.));
#60331=CARTESIAN_POINT('Ctrl Pts',(52.6991298550928,-50.1306930271343,0.));
#60332=CARTESIAN_POINT('Ctrl Pts',(52.7226295845155,-50.1401917592532,0.));
#60333=CARTESIAN_POINT('Ctrl Pts',(52.7461748428733,-50.1496829391068,0.));
#60334=CARTESIAN_POINT('Ctrl Pts',(52.769765553794,-50.1591664773561,0.));
#60335=CARTESIAN_POINT('Ctrl Pts',(52.793401641121,-50.1686422850493,0.));
#60336=CARTESIAN_POINT('Ctrl Pts',(52.8170830289052,-50.1781102736215,0.));
#60337=CARTESIAN_POINT('Ctrl Pts',(52.8408096414101,-50.1875703548893,0.));
#60338=CARTESIAN_POINT('Ctrl Pts',(52.8645814031137,-50.1970224410476,0.));
#60339=CARTESIAN_POINT('Ctrl Pts',(52.8883982387068,-50.2064664446663,0.));
#60340=CARTESIAN_POINT('Ctrl Pts',(52.9122600730882,-50.2159022786876,0.));
#60341=CARTESIAN_POINT('Ctrl Pts',(52.9361668313539,-50.2253298564237,0.));
#60342=CARTESIAN_POINT('Ctrl Pts',(52.9601184388027,-50.2347490915553,0.));
#60343=CARTESIAN_POINT('Ctrl Pts',(52.9841148209404,-50.2441598981286,0.));
#60344=CARTESIAN_POINT('Ctrl Pts',(53.0081559034802,-50.2535621905553,0.));
#60345=CARTESIAN_POINT('Ctrl Pts',(53.0322416123404,-50.2629558836111,0.));
#60346=CARTESIAN_POINT('Ctrl Pts',(53.0563718736361,-50.272340892437,0.));
#60347=CARTESIAN_POINT('Ctrl Pts',(53.0805466136791,-50.2817171325354,0.));
#60348=CARTESIAN_POINT('Ctrl Pts',(53.1047657589806,-50.2910845197615,0.));
#60349=CARTESIAN_POINT('Ctrl Pts',(53.1290292362482,-50.3004429703188,0.));
#60350=CARTESIAN_POINT('Ctrl Pts',(53.153336972382,-50.3097924007536,0.));
#60351=CARTESIAN_POINT('Ctrl Pts',(53.1776888944622,-50.3191327279497,0.));
#60352=CARTESIAN_POINT('Ctrl Pts',(53.202084929748,-50.3284638691285,0.));
#60353=CARTESIAN_POINT('Ctrl Pts',(53.2265250056896,-50.3377857418522,0.));
#60354=CARTESIAN_POINT('Ctrl Pts',(53.2510090499341,-50.3470982640294,0.));
#60355=CARTESIAN_POINT('Ctrl Pts',(53.2755369903291,-50.3564013539198,0.));
#60356=CARTESIAN_POINT('Ctrl Pts',(53.3001087549222,-50.3656949301424,0.));
#60357=CARTESIAN_POINT('Ctrl Pts',(53.3247242719575,-50.3749789116777,0.));
#60358=CARTESIAN_POINT('Ctrl Pts',(53.3493834698685,-50.3842532178451,0.));
#60359=CARTESIAN_POINT('Ctrl Pts',(53.3740862772673,-50.393517768283,0.));
#60360=CARTESIAN_POINT('Ctrl Pts',(53.3988326229308,-50.4027724829296,0.));
#60361=CARTESIAN_POINT('Ctrl Pts',(53.4236224357846,-50.4120172820054,0.));
#60362=CARTESIAN_POINT('Ctrl Pts',(53.4484556448787,-50.4212520859924,0.));
#60363=CARTESIAN_POINT('Ctrl Pts',(53.4733321794199,-50.4304768156677,0.));
#60364=CARTESIAN_POINT('Ctrl Pts',(53.4982519688032,-50.4396913921389,0.));
#60365=CARTESIAN_POINT('Ctrl Pts',(53.5232149426415,-50.4488957368841,0.));
#60366=CARTESIAN_POINT('Ctrl Pts',(53.5482210307864,-50.4580897717835,0.));
#60367=CARTESIAN_POINT('Ctrl Pts',(53.5732701633602,-50.467273419175,0.));
#60368=CARTESIAN_POINT('Ctrl Pts',(53.5983622707231,-50.4764466018064,0.));
#60369=CARTESIAN_POINT('Ctrl Pts',(53.6234972834055,-50.485609242731,0.));
#60370=CARTESIAN_POINT('Ctrl Pts',(53.6486751320434,-50.4947612652147,0.));
#60371=CARTESIAN_POINT('Ctrl Pts',(53.6738957473158,-50.5039025926531,0.));
#60372=CARTESIAN_POINT('Ctrl Pts',(53.6991590598551,-50.5130331484563,0.));
#60373=CARTESIAN_POINT('Ctrl Pts',(53.7244650002382,-50.5221528560427,0.));
#60374=CARTESIAN_POINT('Ctrl Pts',(53.7498134991714,-50.5312616390789,0.));
#60375=CARTESIAN_POINT('Ctrl Pts',(53.7752044876312,-50.5403594216706,0.));
#60376=CARTESIAN_POINT('Ctrl Pts',(53.8006378970198,-50.5494461285762,0.));
#60377=CARTESIAN_POINT('Ctrl Pts',(53.8261136593064,-50.5585216854082,0.));
#60378=CARTESIAN_POINT('Ctrl Pts',(53.8516317071783,-50.567586018852,0.));
#60379=CARTESIAN_POINT('Ctrl Pts',(53.8771919737007,-50.5766390561861,0.));
#60380=CARTESIAN_POINT('Ctrl Pts',(53.9027943919814,-50.5856807248133,0.));
#60381=CARTESIAN_POINT('Ctrl Pts',(53.9284388947996,-50.5947109517476,0.));
#60382=CARTESIAN_POINT('Ctrl Pts',(53.954125414313,-50.603729663215,0.));
#60383=CARTESIAN_POINT('Ctrl Pts',(53.9798538815561,-50.6127367839738,0.));
#60384=CARTESIAN_POINT('Ctrl Pts',(54.0056242268443,-50.6217322378686,0.));
#60385=CARTESIAN_POINT('Ctrl Pts',(54.0314363806751,-50.630715949059,0.));
#60386=CARTESIAN_POINT('Ctrl Pts',(54.0572902745101,-50.6396878430961,0.));
#60387=CARTESIAN_POINT('Ctrl Pts',(54.0831858415182,-50.648647847946,0.));
#60388=CARTESIAN_POINT('Ctrl Pts',(54.1091230175319,-50.657595895318,0.));
#60389=CARTESIAN_POINT('Ctrl Pts',(54.1351017412721,-50.6665319209798,0.));
#60390=CARTESIAN_POINT('Ctrl Pts',(54.157406104188,-50.6741814675381,0.));
#60391=CARTESIAN_POINT('Ctrl Pts',(54.1745287898573,-50.6800396668658,0.));
#60392=CARTESIAN_POINT('Ctrl Pts',(54.1864514381918,-50.6841118861801,0.));
#60393=CARTESIAN_POINT('Ctrl Pts',(54.1931619277288,-50.68640169656,0.));
#60394=CARTESIAN_POINT('Ctrl Pts',(54.1946543499969,-50.6869108458685,0.));
#60395=CARTESIAN_POINT('',(50.0975384783634,-48.8900464144686,12.));
#60396=CARTESIAN_POINT('',(50.0975384783634,-48.8900464144686,0.));
#60397=CARTESIAN_POINT('Ctrl Pts',(54.1946543499969,-50.6869108458685,12.));
#60398=CARTESIAN_POINT('Ctrl Pts',(54.1931619277288,-50.68640169656,12.));
#60399=CARTESIAN_POINT('Ctrl Pts',(54.1864514381918,-50.6841118861801,12.));
#60400=CARTESIAN_POINT('Ctrl Pts',(54.1745287898573,-50.6800396668658,12.));
#60401=CARTESIAN_POINT('Ctrl Pts',(54.157406104188,-50.6741814675381,12.));
#60402=CARTESIAN_POINT('Ctrl Pts',(54.1351017412721,-50.6665319209798,12.));
#60403=CARTESIAN_POINT('Ctrl Pts',(54.1091230175319,-50.657595895318,12.));
#60404=CARTESIAN_POINT('Ctrl Pts',(54.0831858415182,-50.648647847946,12.));
#60405=CARTESIAN_POINT('Ctrl Pts',(54.0572902745101,-50.6396878430961,12.));
#60406=CARTESIAN_POINT('Ctrl Pts',(54.0314363806751,-50.630715949059,12.));
#60407=CARTESIAN_POINT('Ctrl Pts',(54.0056242268443,-50.6217322378686,12.));
#60408=CARTESIAN_POINT('Ctrl Pts',(53.9798538815561,-50.6127367839738,12.));
#60409=CARTESIAN_POINT('Ctrl Pts',(53.954125414313,-50.603729663215,12.));
#60410=CARTESIAN_POINT('Ctrl Pts',(53.9284388947996,-50.5947109517476,12.));
#60411=CARTESIAN_POINT('Ctrl Pts',(53.9027943919814,-50.5856807248133,12.));
#60412=CARTESIAN_POINT('Ctrl Pts',(53.8771919737007,-50.5766390561861,12.));
#60413=CARTESIAN_POINT('Ctrl Pts',(53.8516317071783,-50.567586018852,12.));
#60414=CARTESIAN_POINT('Ctrl Pts',(53.8261136593064,-50.5585216854082,12.));
#60415=CARTESIAN_POINT('Ctrl Pts',(53.8006378970198,-50.5494461285762,12.));
#60416=CARTESIAN_POINT('Ctrl Pts',(53.7752044876312,-50.5403594216706,12.));
#60417=CARTESIAN_POINT('Ctrl Pts',(53.7498134991714,-50.5312616390789,12.));
#60418=CARTESIAN_POINT('Ctrl Pts',(53.7244650002382,-50.5221528560427,12.));
#60419=CARTESIAN_POINT('Ctrl Pts',(53.6991590598551,-50.5130331484563,12.));
#60420=CARTESIAN_POINT('Ctrl Pts',(53.6738957473158,-50.5039025926531,12.));
#60421=CARTESIAN_POINT('Ctrl Pts',(53.6486751320434,-50.4947612652147,12.));
#60422=CARTESIAN_POINT('Ctrl Pts',(53.6234972834055,-50.485609242731,12.));
#60423=CARTESIAN_POINT('Ctrl Pts',(53.5983622707231,-50.4764466018064,12.));
#60424=CARTESIAN_POINT('Ctrl Pts',(53.5732701633602,-50.467273419175,12.));
#60425=CARTESIAN_POINT('Ctrl Pts',(53.5482210307864,-50.4580897717835,12.));
#60426=CARTESIAN_POINT('Ctrl Pts',(53.5232149426415,-50.4488957368841,12.));
#60427=CARTESIAN_POINT('Ctrl Pts',(53.4982519688032,-50.4396913921389,12.));
#60428=CARTESIAN_POINT('Ctrl Pts',(53.4733321794199,-50.4304768156677,12.));
#60429=CARTESIAN_POINT('Ctrl Pts',(53.4484556448787,-50.4212520859924,12.));
#60430=CARTESIAN_POINT('Ctrl Pts',(53.4236224357846,-50.4120172820054,12.));
#60431=CARTESIAN_POINT('Ctrl Pts',(53.3988326229308,-50.4027724829296,12.));
#60432=CARTESIAN_POINT('Ctrl Pts',(53.3740862772673,-50.393517768283,12.));
#60433=CARTESIAN_POINT('Ctrl Pts',(53.3493834698685,-50.3842532178451,12.));
#60434=CARTESIAN_POINT('Ctrl Pts',(53.3247242719575,-50.3749789116777,12.));
#60435=CARTESIAN_POINT('Ctrl Pts',(53.3001087549222,-50.3656949301424,12.));
#60436=CARTESIAN_POINT('Ctrl Pts',(53.2755369903291,-50.3564013539198,12.));
#60437=CARTESIAN_POINT('Ctrl Pts',(53.2510090499341,-50.3470982640294,12.));
#60438=CARTESIAN_POINT('Ctrl Pts',(53.2265250056896,-50.3377857418522,12.));
#60439=CARTESIAN_POINT('Ctrl Pts',(53.202084929748,-50.3284638691285,12.));
#60440=CARTESIAN_POINT('Ctrl Pts',(53.1776888944622,-50.3191327279497,12.));
#60441=CARTESIAN_POINT('Ctrl Pts',(53.153336972382,-50.3097924007536,12.));
#60442=CARTESIAN_POINT('Ctrl Pts',(53.1290292362482,-50.3004429703188,12.));
#60443=CARTESIAN_POINT('Ctrl Pts',(53.1047657589806,-50.2910845197615,12.));
#60444=CARTESIAN_POINT('Ctrl Pts',(53.0805466136791,-50.2817171325354,12.));
#60445=CARTESIAN_POINT('Ctrl Pts',(53.0563718736361,-50.272340892437,12.));
#60446=CARTESIAN_POINT('Ctrl Pts',(53.0322416123404,-50.2629558836111,12.));
#60447=CARTESIAN_POINT('Ctrl Pts',(53.0081559034802,-50.2535621905553,12.));
#60448=CARTESIAN_POINT('Ctrl Pts',(52.9841148209404,-50.2441598981286,12.));
#60449=CARTESIAN_POINT('Ctrl Pts',(52.9601184388027,-50.2347490915553,12.));
#60450=CARTESIAN_POINT('Ctrl Pts',(52.9361668313539,-50.2253298564237,12.));
#60451=CARTESIAN_POINT('Ctrl Pts',(52.9122600730882,-50.2159022786876,12.));
#60452=CARTESIAN_POINT('Ctrl Pts',(52.8883982387068,-50.2064664446663,12.));
#60453=CARTESIAN_POINT('Ctrl Pts',(52.8645814031137,-50.1970224410476,12.));
#60454=CARTESIAN_POINT('Ctrl Pts',(52.8408096414101,-50.1875703548893,12.));
#60455=CARTESIAN_POINT('Ctrl Pts',(52.8170830289052,-50.1781102736215,12.));
#60456=CARTESIAN_POINT('Ctrl Pts',(52.793401641121,-50.1686422850493,12.));
#60457=CARTESIAN_POINT('Ctrl Pts',(52.769765553794,-50.1591664773561,12.));
#60458=CARTESIAN_POINT('Ctrl Pts',(52.7461748428733,-50.1496829391068,12.));
#60459=CARTESIAN_POINT('Ctrl Pts',(52.7226295845155,-50.1401917592532,12.));
#60460=CARTESIAN_POINT('Ctrl Pts',(52.6991298550928,-50.1306930271343,12.));
#60461=CARTESIAN_POINT('Ctrl Pts',(52.6756757311979,-50.1211868324781,12.));
#60462=CARTESIAN_POINT('Ctrl Pts',(52.6522672896462,-50.1116732654041,12.));
#60463=CARTESIAN_POINT('Ctrl Pts',(52.6289046074743,-50.1021524164261,12.));
#60464=CARTESIAN_POINT('Ctrl Pts',(52.6055877619338,-50.0926243764569,12.));
#60465=CARTESIAN_POINT('Ctrl Pts',(52.5823168304981,-50.0830892368095,12.));
#60466=CARTESIAN_POINT('Ctrl Pts',(52.5590918908691,-50.0735470891996,12.));
#60467=CARTESIAN_POINT('Ctrl Pts',(52.5359130209789,-50.0639980257477,12.));
#60468=CARTESIAN_POINT('Ctrl Pts',(52.5127802989903,-50.0544421389824,12.));
#60469=CARTESIAN_POINT('Ctrl Pts',(52.4896938032896,-50.0448795218453,12.));
#60470=CARTESIAN_POINT('Ctrl Pts',(52.4666536124926,-50.0353102676933,12.));
#60471=CARTESIAN_POINT('Ctrl Pts',(52.4436598054523,-50.0257344703008,12.));
#60472=CARTESIAN_POINT('Ctrl Pts',(52.420712461261,-50.0161522238619,12.));
#60473=CARTESIAN_POINT('Ctrl Pts',(52.3978116592505,-50.0065636229934,12.));
#60474=CARTESIAN_POINT('Ctrl Pts',(52.3749574789865,-49.9969687627402,12.));
#60475=CARTESIAN_POINT('Ctrl Pts',(52.3521500002711,-49.9873677385769,12.));
#60476=CARTESIAN_POINT('Ctrl Pts',(52.3293893031524,-49.9777606464103,12.));
#60477=CARTESIAN_POINT('Ctrl Pts',(52.3066754679264,-49.9681475825824,12.));
#60478=CARTESIAN_POINT('Ctrl Pts',(52.2840085751385,-49.9585286438734,12.));
#60479=CARTESIAN_POINT('Ctrl Pts',(52.2613887055773,-49.9489039275064,12.));
#60480=CARTESIAN_POINT('Ctrl Pts',(52.238815940277,-49.9392735311507,12.));
#60481=CARTESIAN_POINT('Ctrl Pts',(52.2162903605272,-49.9296375529241,12.));
#60482=CARTESIAN_POINT('Ctrl Pts',(52.1938120478752,-49.919996091396,12.));
#60483=CARTESIAN_POINT('Ctrl Pts',(52.1713810841277,-49.9103492455904,12.));
#60484=CARTESIAN_POINT('Ctrl Pts',(52.1489975513449,-49.90069711499,12.));
#60485=CARTESIAN_POINT('Ctrl Pts',(52.1266615318414,-49.8910397995404,12.));
#60486=CARTESIAN_POINT('Ctrl Pts',(52.1043731081968,-49.8813773996523,12.));
#60487=CARTESIAN_POINT('Ctrl Pts',(52.0821323632588,-49.871710016205,12.));
#60488=CARTESIAN_POINT('Ctrl Pts',(52.059939380145,-49.8620377505498,12.));
#60489=CARTESIAN_POINT('Ctrl Pts',(52.0377942422373,-49.8523607045146,12.));
#60490=CARTESIAN_POINT('Ctrl Pts',(52.015697033182,-49.8426789804068,12.));
#60491=CARTESIAN_POINT('Ctrl Pts',(51.9936478369008,-49.8329926810172,12.));
#60492=CARTESIAN_POINT('Ctrl Pts',(51.9716467375938,-49.8233019096224,12.));
#60493=CARTESIAN_POINT('Ctrl Pts',(51.9496938197418,-49.8136067699896,12.));
#60494=CARTESIAN_POINT('Ctrl Pts',(51.9277891681013,-49.8039073663808,12.));
#60495=CARTESIAN_POINT('Ctrl Pts',(51.9059328677051,-49.7942038035568,12.));
#60496=CARTESIAN_POINT('Ctrl Pts',(51.8841250038716,-49.78449618678,12.));
#60497=CARTESIAN_POINT('Ctrl Pts',(51.8623656622092,-49.7747846218177,12.));
#60498=CARTESIAN_POINT('Ctrl Pts',(51.8406549286176,-49.7650692149464,12.));
#60499=CARTESIAN_POINT('Ctrl Pts',(51.8189928892841,-49.7553500729563,12.));
#60500=CARTESIAN_POINT('Ctrl Pts',(51.7973796306826,-49.7456273031555,12.));
#60501=CARTESIAN_POINT('Ctrl Pts',(51.7758152395857,-49.7359010133741,12.));
#60502=CARTESIAN_POINT('Ctrl Pts',(51.7542998030679,-49.7261713119672,12.));
#60503=CARTESIAN_POINT('Ctrl Pts',(51.7328334085084,-49.7164383078206,12.));
#60504=CARTESIAN_POINT('Ctrl Pts',(51.7114161435847,-49.7067021103534,12.));
#60505=CARTESIAN_POINT('Ctrl Pts',(51.6900480962743,-49.6969628295236,12.));
#60506=CARTESIAN_POINT('Ctrl Pts',(51.6687293548656,-49.6872205758314,12.));
#60507=CARTESIAN_POINT('Ctrl Pts',(51.6474600079611,-49.6774754603235,12.));
#60508=CARTESIAN_POINT('Ctrl Pts',(51.6262401444799,-49.6677275945975,12.));
#60509=CARTESIAN_POINT('Ctrl Pts',(51.6050698536525,-49.6579770908063,12.));
#60510=CARTESIAN_POINT('Ctrl Pts',(51.5839492250218,-49.6482240616627,12.));
#60511=CARTESIAN_POINT('Ctrl Pts',(51.5628783484556,-49.6384686204443,12.));
#60512=CARTESIAN_POINT('Ctrl Pts',(51.5418573141494,-49.6287108809975,12.));
#60513=CARTESIAN_POINT('Ctrl Pts',(51.5208862126303,-49.6189509577441,12.));
#60514=CARTESIAN_POINT('Ctrl Pts',(51.4999651347496,-49.609188965684,12.));
#60515=CARTESIAN_POINT('Ctrl Pts',(51.4790941716859,-49.5994250204003,12.));
#60516=CARTESIAN_POINT('Ctrl Pts',(51.4582734149562,-49.5896592380634,12.));
#60517=CARTESIAN_POINT('Ctrl Pts',(51.4375029564191,-49.579891735436,12.));
#60518=CARTESIAN_POINT('Ctrl Pts',(51.4167828882765,-49.5701226298779,12.));
#60519=CARTESIAN_POINT('Ctrl Pts',(51.3961133030688,-49.5603520393514,12.));
#60520=CARTESIAN_POINT('Ctrl Pts',(51.3754942936796,-49.5505800824268,12.));
#60521=CARTESIAN_POINT('Ctrl Pts',(51.354925953347,-49.5408068782871,12.));
#60522=CARTESIAN_POINT('Ctrl Pts',(51.3344083756659,-49.5310325467334,12.));
#60523=CARTESIAN_POINT('Ctrl Pts',(51.3139416545903,-49.5212572081901,12.));
#60524=CARTESIAN_POINT('Ctrl Pts',(51.2935258844278,-49.5114809837111,12.));
#60525=CARTESIAN_POINT('Ctrl Pts',(51.2731611598465,-49.5017039949841,12.));
#60526=CARTESIAN_POINT('Ctrl Pts',(51.2528475758841,-49.4919263643357,12.));
#60527=CARTESIAN_POINT('Ctrl Pts',(51.2325852279507,-49.4821482147357,12.));
#60528=CARTESIAN_POINT('Ctrl Pts',(51.2123742118288,-49.4723696698022,12.));
#60529=CARTESIAN_POINT('Ctrl Pts',(51.1922146236686,-49.4625908538076,12.));
#60530=CARTESIAN_POINT('Ctrl Pts',(51.1721065599972,-49.4528118916833,12.));
#60531=CARTESIAN_POINT('Ctrl Pts',(51.1520501177291,-49.4430329090288,12.));
#60532=CARTESIAN_POINT('Ctrl Pts',(51.1320453941702,-49.4332540321178,12.));
#60533=CARTESIAN_POINT('Ctrl Pts',(51.1120924870196,-49.4234753879071,12.));
#60534=CARTESIAN_POINT('Ctrl Pts',(51.0921914943663,-49.4136971040428,12.));
#60535=CARTESIAN_POINT('Ctrl Pts',(51.0723425146987,-49.4039193088636,12.));
#60536=CARTESIAN_POINT('Ctrl Pts',(51.0525456469072,-49.3941421314014,12.));
#60537=CARTESIAN_POINT('Ctrl Pts',(51.0328009902857,-49.3843657013851,12.));
#60538=CARTESIAN_POINT('Ctrl Pts',(51.0131086445268,-49.3745901492429,12.));
#60539=CARTESIAN_POINT('Ctrl Pts',(50.9934687097179,-49.3648156061049,12.));
#60540=CARTESIAN_POINT('Ctrl Pts',(50.9738812863635,-49.3550422038221,12.));
#60541=CARTESIAN_POINT('Ctrl Pts',(50.9543464753974,-49.3452700749804,12.));
#60542=CARTESIAN_POINT('Ctrl Pts',(50.9348643781928,-49.3354993529163,12.));
#60543=CARTESIAN_POINT('Ctrl Pts',(50.9154350965681,-49.325730171735,12.));
#60544=CARTESIAN_POINT('Ctrl Pts',(50.8960587327869,-49.3159626663129,12.));
#60545=CARTESIAN_POINT('Ctrl Pts',(50.8767353895509,-49.3061969722798,12.));
#60546=CARTESIAN_POINT('Ctrl Pts',(50.8574651699877,-49.2964332260043,12.));
#60547=CARTESIAN_POINT('Ctrl Pts',(50.8382481776392,-49.2866715645828,12.));
#60548=CARTESIAN_POINT('Ctrl Pts',(50.8190845164319,-49.2769121258144,12.));
#60549=CARTESIAN_POINT('Ctrl Pts',(50.799974290711,-49.2671550482415,12.));
#60550=CARTESIAN_POINT('Ctrl Pts',(50.7809176052954,-49.2574004712122,12.));
#60551=CARTESIAN_POINT('Ctrl Pts',(50.7619145655207,-49.2476485349373,12.));
#60552=CARTESIAN_POINT('Ctrl Pts',(50.7429652772816,-49.2378993805482,12.));
#60553=CARTESIAN_POINT('Ctrl Pts',(50.7240698470698,-49.2281531501569,12.));
#60554=CARTESIAN_POINT('Ctrl Pts',(50.7052283818941,-49.218409986748,12.));
#60555=CARTESIAN_POINT('Ctrl Pts',(50.6864409891905,-49.2086700340625,12.));
#60556=CARTESIAN_POINT('Ctrl Pts',(50.6677077767427,-49.1989334364992,12.));
#60557=CARTESIAN_POINT('Ctrl Pts',(50.6490288525639,-49.1892003389743,12.));
#60558=CARTESIAN_POINT('Ctrl Pts',(50.6304043248796,-49.1794708869074,12.));
#60559=CARTESIAN_POINT('Ctrl Pts',(50.6118343023937,-49.1697452265473,12.));
#60560=CARTESIAN_POINT('Ctrl Pts',(50.593318894516,-49.1600235052613,12.));
#60561=CARTESIAN_POINT('Ctrl Pts',(50.5748582115575,-49.1503058717831,12.));
#60562=CARTESIAN_POINT('Ctrl Pts',(50.5564523650406,-49.1405924766169,12.));
#60563=CARTESIAN_POINT('Ctrl Pts',(50.5381014674822,-49.1308834717645,12.));
#60564=CARTESIAN_POINT('Ctrl Pts',(50.5198056318111,-49.1211790099817,12.));
#60565=CARTESIAN_POINT('Ctrl Pts',(50.5015649708742,-49.1114792441573,12.));
#60566=CARTESIAN_POINT('Ctrl Pts',(50.4833795969296,-49.1017843266782,12.));
#60567=CARTESIAN_POINT('Ctrl Pts',(50.465249621057,-49.0920944086973,12.));
#60568=CARTESIAN_POINT('Ctrl Pts',(50.4471751542717,-49.0824096415339,12.));
#60569=CARTESIAN_POINT('Ctrl Pts',(50.4291563088528,-49.0727301783477,12.));
#60570=CARTESIAN_POINT('Ctrl Pts',(50.4111931994264,-49.0630561755082,12.));
#60571=CARTESIAN_POINT('Ctrl Pts',(50.393285944528,-49.0533877945771,12.));
#60572=CARTESIAN_POINT('Ctrl Pts',(50.3754346667389,-49.0437252024868,12.));
#60573=CARTESIAN_POINT('Ctrl Pts',(50.3576394894136,-49.034068567401,12.));
#60574=CARTESIAN_POINT('Ctrl Pts',(50.3399005337967,-49.0244180550759,12.));
#60575=CARTESIAN_POINT('Ctrl Pts',(50.3222179165102,-49.0147738256925,12.));
#60576=CARTESIAN_POINT('Ctrl Pts',(50.3045917455383,-49.0051360288002,12.));
#60577=CARTESIAN_POINT('Ctrl Pts',(50.2870221241003,-48.9955048082028,12.));
#60578=CARTESIAN_POINT('Ctrl Pts',(50.2695091583472,-48.9858803116649,12.));
#60579=CARTESIAN_POINT('Ctrl Pts',(50.252052963548,-48.9762626987227,12.));
#60580=CARTESIAN_POINT('Ctrl Pts',(50.2346536715465,-48.9666521500969,12.));
#60581=CARTESIAN_POINT('Ctrl Pts',(50.2173114358423,-48.9570488741273,12.));
#60582=CARTESIAN_POINT('Ctrl Pts',(50.2000264157903,-48.9474530868847,12.));
#60583=CARTESIAN_POINT('Ctrl Pts',(50.1827987615659,-48.9378649933116,12.));
#60584=CARTESIAN_POINT('Ctrl Pts',(50.1656286003943,-48.9282847698237,12.));
#60585=CARTESIAN_POINT('Ctrl Pts',(50.148516018447,-48.9187125417897,12.));
#60586=CARTESIAN_POINT('Ctrl Pts',(50.1314610602286,-48.9091483817797,12.));
#60587=CARTESIAN_POINT('Ctrl Pts',(50.1178632066821,-48.9015035371772,12.));
#60588=CARTESIAN_POINT('Ctrl Pts',(50.1076907555303,-48.8957735556681,12.));
#60589=CARTESIAN_POINT('Ctrl Pts',(50.1009206494209,-48.8919551910299,12.));
#60590=CARTESIAN_POINT('Ctrl Pts',(50.0975384783634,-48.8900464144686,12.));
#60591=CARTESIAN_POINT('Ctrl Pts',(55.2174072001497,-49.5707719660643,-5.55111512312578E-16));
#60592=CARTESIAN_POINT('Ctrl Pts',(55.2174072001497,-49.5707719660643,4.));
#60593=CARTESIAN_POINT('Ctrl Pts',(55.2174072001497,-49.5707719660643,8.));
#60594=CARTESIAN_POINT('Ctrl Pts',(55.2174072001497,-49.5707719660643,12.));
#60595=CARTESIAN_POINT('Ctrl Pts',(55.2618153697169,-49.6712810246937,-5.55111512312578E-16));
#60596=CARTESIAN_POINT('Ctrl Pts',(55.2618153697169,-49.6712810246937,4.));
#60597=CARTESIAN_POINT('Ctrl Pts',(55.2618153697169,-49.6712810246937,8.));
#60598=CARTESIAN_POINT('Ctrl Pts',(55.2618153697169,-49.6712810246937,12.));
#60599=CARTESIAN_POINT('Ctrl Pts',(55.2790667815471,-49.8732090625343,-6.28195156302604E-16));
#60600=CARTESIAN_POINT('Ctrl Pts',(55.2790667815471,-49.8732090625343,4.));
#60601=CARTESIAN_POINT('Ctrl Pts',(55.2790667815471,-49.8732090625343,7.99999999999999));
#60602=CARTESIAN_POINT('Ctrl Pts',(55.2790667815471,-49.8732090625343,12.));
#60603=CARTESIAN_POINT('Ctrl Pts',(55.1854902750883,-50.0481613529515,-8.01722692509434E-16));
#60604=CARTESIAN_POINT('Ctrl Pts',(55.1854902750883,-50.0481613529515,4.));
#60605=CARTESIAN_POINT('Ctrl Pts',(55.1854902750883,-50.0481613529515,8.00000000000001));
#60606=CARTESIAN_POINT('Ctrl Pts',(55.1854902750883,-50.0481613529515,12.));
#60607=CARTESIAN_POINT('Ctrl Pts',(55.1300595714122,-50.1091461876223,-8.85376672737052E-16));
#60608=CARTESIAN_POINT('Ctrl Pts',(55.1300595714122,-50.1091461876223,4.));
#60609=CARTESIAN_POINT('Ctrl Pts',(55.1300595714122,-50.1091461876224,8.));
#60610=CARTESIAN_POINT('Ctrl Pts',(55.1300595714122,-50.1091461876224,12.));
#60611=CARTESIAN_POINT('',(55.2174072001497,-49.5707719660643,0.));
#60612=CARTESIAN_POINT('',(55.1300595714124,-50.1091461876225,0.));
#60613=CARTESIAN_POINT('Ctrl Pts',(55.2174072001497,-49.5707719660643,-4.91496295208056E-16));
#60614=CARTESIAN_POINT('Ctrl Pts',(55.2618153697169,-49.6712810246937,-4.91496295208056E-16));
#60615=CARTESIAN_POINT('Ctrl Pts',(55.2716733193341,-49.7866684748883,-5.3325837748807E-16));
#60616=CARTESIAN_POINT('Ctrl Pts',(55.2453425609387,-49.893247517761,-6.07818465389898E-16));
#60617=CARTESIAN_POINT('Ctrl Pts',(55.2255944921421,-49.9731817999155,-6.6373853131627E-16));
#60618=CARTESIAN_POINT('Ctrl Pts',(55.1854902750883,-50.0481613529515,-7.38107475404911E-16));
#60619=CARTESIAN_POINT('Ctrl Pts',(55.1300595714122,-50.1091461876223,-8.21761455632529E-16));
#60620=CARTESIAN_POINT('',(55.1300595714124,-50.1091461876225,12.));
#60621=CARTESIAN_POINT('Ctrl Pts',(55.1300595714122,-50.1091461876223,-8.85376672737052E-16));
#60622=CARTESIAN_POINT('Ctrl Pts',(55.1300595714122,-50.1091461876223,4.));
#60623=CARTESIAN_POINT('Ctrl Pts',(55.1300595714122,-50.1091461876224,8.));
#60624=CARTESIAN_POINT('Ctrl Pts',(55.1300595714122,-50.1091461876224,12.));
#60625=CARTESIAN_POINT('',(55.2174072001497,-49.5707719660643,12.));
#60626=CARTESIAN_POINT('Ctrl Pts',(55.1300595714122,-50.1091461876224,12.));
#60627=CARTESIAN_POINT('Ctrl Pts',(55.1854902750883,-50.0481613529515,12.));
#60628=CARTESIAN_POINT('Ctrl Pts',(55.2255944921421,-49.9731817999156,12.));
#60629=CARTESIAN_POINT('Ctrl Pts',(55.2453425609387,-49.893247517761,12.));
#60630=CARTESIAN_POINT('Ctrl Pts',(55.2716733193342,-49.7866684748883,12.));
#60631=CARTESIAN_POINT('Ctrl Pts',(55.2618153697169,-49.6712810246937,12.));
#60632=CARTESIAN_POINT('Ctrl Pts',(55.2174072001497,-49.5707719660643,12.));
#60633=CARTESIAN_POINT('Ctrl Pts',(55.2174072001497,-49.5707719660643,12.));
#60634=CARTESIAN_POINT('Ctrl Pts',(55.2174072001497,-49.5707719660643,8.));
#60635=CARTESIAN_POINT('Ctrl Pts',(55.2174072001497,-49.5707719660643,4.));
#60636=CARTESIAN_POINT('Ctrl Pts',(55.2174072001497,-49.5707719660643,-5.55111512312578E-16));
#60637=CARTESIAN_POINT('Origin',(2.7643087079898E-10,-2.53167595884892E-10,
0.));
#60638=CARTESIAN_POINT('Origin',(2.7643087079898E-10,-2.53167595884892E-10,
12.));
#60639=CARTESIAN_POINT('Origin',(2.7643087079898E-10,-2.53167595884892E-10,
0.));
#60640=CARTESIAN_POINT('Ctrl Pts',(50.1091461876248,-55.1300595714103,-5.55111512312578E-16));
#60641=CARTESIAN_POINT('Ctrl Pts',(50.1091461876248,-55.1300595714103,4.));
#60642=CARTESIAN_POINT('Ctrl Pts',(50.1091461876248,-55.1300595714103,8.));
#60643=CARTESIAN_POINT('Ctrl Pts',(50.1091461876248,-55.1300595714103,12.));
#60644=CARTESIAN_POINT('Ctrl Pts',(50.0278330747241,-55.2039671763175,-5.55111512312578E-16));
#60645=CARTESIAN_POINT('Ctrl Pts',(50.0278330747241,-55.2039671763175,4.));
#60646=CARTESIAN_POINT('Ctrl Pts',(50.0278330747241,-55.2039671763174,8.00000000000001));
#60647=CARTESIAN_POINT('Ctrl Pts',(50.0278330747241,-55.2039671763174,12.));
#60648=CARTESIAN_POINT('Ctrl Pts',(49.8417173275618,-55.2841761056302,-6.28195156314307E-16));
#60649=CARTESIAN_POINT('Ctrl Pts',(49.8417173275618,-55.2841761056302,4.00000000000001));
#60650=CARTESIAN_POINT('Ctrl Pts',(49.8417173275618,-55.2841761056302,7.99999999999999));
#60651=CARTESIAN_POINT('Ctrl Pts',(49.8417173275618,-55.2841761056302,12.));
#60652=CARTESIAN_POINT('Ctrl Pts',(49.6461537600011,-55.2507133273144,-8.01722692544929E-16));
#60653=CARTESIAN_POINT('Ctrl Pts',(49.6461537600011,-55.2507133273144,4.));
#60654=CARTESIAN_POINT('Ctrl Pts',(49.6461537600011,-55.2507133273144,8.00000000000001));
#60655=CARTESIAN_POINT('Ctrl Pts',(49.6461537600011,-55.2507133273144,12.));
#60656=CARTESIAN_POINT('Ctrl Pts',(49.5707719660263,-55.2174072001298,-8.85376672782319E-16));
#60657=CARTESIAN_POINT('Ctrl Pts',(49.5707719660263,-55.2174072001298,4.));
#60658=CARTESIAN_POINT('Ctrl Pts',(49.5707719660263,-55.2174072001297,8.));
#60659=CARTESIAN_POINT('Ctrl Pts',(49.5707719660263,-55.2174072001297,12.));
#60660=CARTESIAN_POINT('',(50.1091461876248,-55.1300595714103,0.));
#60661=CARTESIAN_POINT('',(49.5707719660262,-55.21740720013,0.));
#60662=CARTESIAN_POINT('Ctrl Pts',(50.1091461876248,-55.1300595714103,-5.27668960562141E-16));
#60663=CARTESIAN_POINT('Ctrl Pts',(50.0278330747241,-55.2039671763175,-5.27668960562141E-16));
#60664=CARTESIAN_POINT('Ctrl Pts',(49.9214812192028,-55.2498008502104,-5.69431042848843E-16));
#60665=CARTESIAN_POINT('Ctrl Pts',(49.8120443611024,-55.2585172318166,-6.43991130761306E-16));
#60666=CARTESIAN_POINT('Ctrl Pts',(49.7299667175271,-55.2650545180212,-6.99911196695654E-16));
#60667=CARTESIAN_POINT('Ctrl Pts',(49.6461537600011,-55.2507133273144,-7.74280140794491E-16));
#60668=CARTESIAN_POINT('Ctrl Pts',(49.5707719660263,-55.2174072001298,-8.57934121031881E-16));
#60669=CARTESIAN_POINT('',(49.5707719660262,-55.21740720013,12.));
#60670=CARTESIAN_POINT('Ctrl Pts',(49.5707719660263,-55.2174072001298,-8.85376672782319E-16));
#60671=CARTESIAN_POINT('Ctrl Pts',(49.5707719660263,-55.2174072001298,4.));
#60672=CARTESIAN_POINT('Ctrl Pts',(49.5707719660263,-55.2174072001297,8.));
#60673=CARTESIAN_POINT('Ctrl Pts',(49.5707719660263,-55.2174072001297,12.));
#60674=CARTESIAN_POINT('',(50.1091461876248,-55.1300595714103,12.));
#60675=CARTESIAN_POINT('Ctrl Pts',(49.5707719660263,-55.2174072001297,12.));
#60676=CARTESIAN_POINT('Ctrl Pts',(49.6461537600011,-55.2507133273144,12.));
#60677=CARTESIAN_POINT('Ctrl Pts',(49.7299667175271,-55.2650545180211,12.));
#60678=CARTESIAN_POINT('Ctrl Pts',(49.8120443611024,-55.2585172318165,12.));
#60679=CARTESIAN_POINT('Ctrl Pts',(49.9214812192028,-55.2498008502104,12.));
#60680=CARTESIAN_POINT('Ctrl Pts',(50.0278330747241,-55.2039671763174,12.));
#60681=CARTESIAN_POINT('Ctrl Pts',(50.1091461876248,-55.1300595714103,12.));
#60682=CARTESIAN_POINT('Ctrl Pts',(50.1091461876248,-55.1300595714103,12.));
#60683=CARTESIAN_POINT('Ctrl Pts',(50.1091461876248,-55.1300595714103,8.));
#60684=CARTESIAN_POINT('Ctrl Pts',(50.1091461876248,-55.1300595714103,4.));
#60685=CARTESIAN_POINT('Ctrl Pts',(50.1091461876248,-55.1300595714103,-5.55111512312578E-16));
#60686=CARTESIAN_POINT('Ctrl Pts',(45.6458539113724,-53.0702932034641,0.));
#60687=CARTESIAN_POINT('Ctrl Pts',(45.6458539113724,-53.0702932034641,12.));
#60688=CARTESIAN_POINT('Ctrl Pts',(45.6490568514089,-53.0724894921849,0.));
#60689=CARTESIAN_POINT('Ctrl Pts',(45.6490568514089,-53.0724894921849,12.));
#60690=CARTESIAN_POINT('Ctrl Pts',(45.6554684028145,-53.0768833804193,0.));
#60691=CARTESIAN_POINT('Ctrl Pts',(45.6554684028145,-53.0768833804193,12.));
#60692=CARTESIAN_POINT('Ctrl Pts',(45.6651027439241,-53.0834781451546,0.));
#60693=CARTESIAN_POINT('Ctrl Pts',(45.6651027439241,-53.0834781451546,12.));
#60694=CARTESIAN_POINT('Ctrl Pts',(45.6779825614231,-53.0922790298409,0.));
#60695=CARTESIAN_POINT('Ctrl Pts',(45.6779825614231,-53.0922790298409,12.));
#60696=CARTESIAN_POINT('Ctrl Pts',(45.694139048907,-53.1032932328857,0.));
#60697=CARTESIAN_POINT('Ctrl Pts',(45.694139048907,-53.1032932328857,12.));
#60698=CARTESIAN_POINT('Ctrl Pts',(45.7103522376696,-53.114320495492,0.));
#60699=CARTESIAN_POINT('Ctrl Pts',(45.7103522376696,-53.114320495492,12.));
#60700=CARTESIAN_POINT('Ctrl Pts',(45.7266220897003,-53.1253607414872,0.));
#60701=CARTESIAN_POINT('Ctrl Pts',(45.7266220897003,-53.1253607414872,12.));
#60702=CARTESIAN_POINT('Ctrl Pts',(45.7429485300823,-53.1364138384693,0.));
#60703=CARTESIAN_POINT('Ctrl Pts',(45.7429485300823,-53.1364138384693,12.));
#60704=CARTESIAN_POINT('Ctrl Pts',(45.7593314474501,-53.1474795996053,0.));
#60705=CARTESIAN_POINT('Ctrl Pts',(45.7593314474501,-53.1474795996053,12.));
#60706=CARTESIAN_POINT('Ctrl Pts',(45.7757707100618,-53.1585578076444,0.));
#60707=CARTESIAN_POINT('Ctrl Pts',(45.7757707100618,-53.1585578076444,12.));
#60708=CARTESIAN_POINT('Ctrl Pts',(45.7922661780005,-53.1696482334487,0.));
#60709=CARTESIAN_POINT('Ctrl Pts',(45.7922661780005,-53.1696482334487,12.));
#60710=CARTESIAN_POINT('Ctrl Pts',(45.8088177165089,-53.1807506560933,0.));
#60711=CARTESIAN_POINT('Ctrl Pts',(45.8088177165089,-53.1807506560933,12.));
#60712=CARTESIAN_POINT('Ctrl Pts',(45.8254252099957,-53.1918648840541,0.));
#60713=CARTESIAN_POINT('Ctrl Pts',(45.8254252099957,-53.1918648840541,12.));
#60714=CARTESIAN_POINT('Ctrl Pts',(45.8420885575349,-53.2029907483557,0.));
#60715=CARTESIAN_POINT('Ctrl Pts',(45.8420885575349,-53.2029907483557,12.));
#60716=CARTESIAN_POINT('Ctrl Pts',(45.8588076662582,-53.2141280925439,0.));
#60717=CARTESIAN_POINT('Ctrl Pts',(45.8588076662582,-53.2141280925439,12.));
#60718=CARTESIAN_POINT('Ctrl Pts',(45.8755824458722,-53.2252767643662,0.));
#60719=CARTESIAN_POINT('Ctrl Pts',(45.8755824458722,-53.2252767643662,12.));
#60720=CARTESIAN_POINT('Ctrl Pts',(45.8924128018379,-53.2364366054306,0.));
#60721=CARTESIAN_POINT('Ctrl Pts',(45.8924128018379,-53.2364366054306,12.));
#60722=CARTESIAN_POINT('Ctrl Pts',(45.9092986319377,-53.2476074460017,0.));
#60723=CARTESIAN_POINT('Ctrl Pts',(45.9092986319377,-53.2476074460017,12.));
#60724=CARTESIAN_POINT('Ctrl Pts',(45.9262398298349,-53.2587891103866,0.));
#60725=CARTESIAN_POINT('Ctrl Pts',(45.9262398298349,-53.2587891103866,12.));
#60726=CARTESIAN_POINT('Ctrl Pts',(45.9432362873008,-53.2699814203105,0.));
#60727=CARTESIAN_POINT('Ctrl Pts',(45.9432362873008,-53.2699814203105,12.));
#60728=CARTESIAN_POINT('Ctrl Pts',(45.9602878967698,-53.2811841987926,0.));
#60729=CARTESIAN_POINT('Ctrl Pts',(45.9602878967698,-53.2811841987926,12.));
#60730=CARTESIAN_POINT('Ctrl Pts',(45.9773945542384,-53.292397274555,0.));
#60731=CARTESIAN_POINT('Ctrl Pts',(45.9773945542384,-53.292397274555,12.));
#60732=CARTESIAN_POINT('Ctrl Pts',(45.9945561591453,-53.3036204818329,0.));
#60733=CARTESIAN_POINT('Ctrl Pts',(45.9945561591453,-53.3036204818329,12.));
#60734=CARTESIAN_POINT('Ctrl Pts',(46.0117726129873,-53.3148536582635,0.));
#60735=CARTESIAN_POINT('Ctrl Pts',(46.0117726129873,-53.3148536582635,12.));
#60736=CARTESIAN_POINT('Ctrl Pts',(46.02904381836,-53.326096643428,0.));
#60737=CARTESIAN_POINT('Ctrl Pts',(46.02904381836,-53.326096643428,12.));
#60738=CARTESIAN_POINT('Ctrl Pts',(46.0463696777801,-53.3373492770671,0.));
#60739=CARTESIAN_POINT('Ctrl Pts',(46.0463696777801,-53.3373492770671,12.));
#60740=CARTESIAN_POINT('Ctrl Pts',(46.0637500926982,-53.3486113975901,0.));
#60741=CARTESIAN_POINT('Ctrl Pts',(46.0637500926982,-53.3486113975901,12.));
#60742=CARTESIAN_POINT('Ctrl Pts',(46.0811849640218,-53.3598828428546,0.));
#60743=CARTESIAN_POINT('Ctrl Pts',(46.0811849640218,-53.3598828428546,12.));
#60744=CARTESIAN_POINT('Ctrl Pts',(46.0986741925656,-53.3711634508437,0.));
#60745=CARTESIAN_POINT('Ctrl Pts',(46.0986741925656,-53.3711634508437,12.));
#60746=CARTESIAN_POINT('Ctrl Pts',(46.1162176794884,-53.3824530603276,0.));
#60747=CARTESIAN_POINT('Ctrl Pts',(46.1162176794884,-53.3824530603276,12.));
#60748=CARTESIAN_POINT('Ctrl Pts',(46.1338153268097,-53.3937515116549,0.));
#60749=CARTESIAN_POINT('Ctrl Pts',(46.1338153268097,-53.3937515116549,12.));
#60750=CARTESIAN_POINT('Ctrl Pts',(46.1514670376012,-53.4050586470436,0.));
#60751=CARTESIAN_POINT('Ctrl Pts',(46.1514670376012,-53.4050586470436,12.));
#60752=CARTESIAN_POINT('Ctrl Pts',(46.1691727157134,-53.4163743101517,0.));
#60753=CARTESIAN_POINT('Ctrl Pts',(46.1691727157134,-53.4163743101517,12.));
#60754=CARTESIAN_POINT('Ctrl Pts',(46.1869322656023,-53.4276983458125,0.));
#60755=CARTESIAN_POINT('Ctrl Pts',(46.1869322656023,-53.4276983458125,12.));
#60756=CARTESIAN_POINT('Ctrl Pts',(46.2047455921286,-53.4390305997274,0.));
#60757=CARTESIAN_POINT('Ctrl Pts',(46.2047455921286,-53.4390305997274,12.));
#60758=CARTESIAN_POINT('Ctrl Pts',(46.2226126003202,-53.4503709181178,0.));
#60759=CARTESIAN_POINT('Ctrl Pts',(46.2226126003202,-53.4503709181178,12.));
#60760=CARTESIAN_POINT('Ctrl Pts',(46.2405331953889,-53.4617191477402,0.));
#60761=CARTESIAN_POINT('Ctrl Pts',(46.2405331953889,-53.4617191477402,12.));
#60762=CARTESIAN_POINT('Ctrl Pts',(46.2585072828353,-53.4730751360371,0.));
#60763=CARTESIAN_POINT('Ctrl Pts',(46.2585072828353,-53.4730751360371,12.));
#60764=CARTESIAN_POINT('Ctrl Pts',(46.2765347685198,-53.4844387312414,0.));
#60765=CARTESIAN_POINT('Ctrl Pts',(46.2765347685198,-53.4844387312414,12.));
#60766=CARTESIAN_POINT('Ctrl Pts',(46.2946155587417,-53.4958097825006,0.));
#60767=CARTESIAN_POINT('Ctrl Pts',(46.2946155587417,-53.4958097825006,12.));
#60768=CARTESIAN_POINT('Ctrl Pts',(46.3127495603098,-53.5071881399911,0.));
#60769=CARTESIAN_POINT('Ctrl Pts',(46.3127495603098,-53.5071881399911,12.));
#60770=CARTESIAN_POINT('Ctrl Pts',(46.3309366805093,-53.5185736548548,0.));
#60771=CARTESIAN_POINT('Ctrl Pts',(46.3309366805093,-53.5185736548548,12.));
#60772=CARTESIAN_POINT('Ctrl Pts',(46.3491768270655,-53.5299661791385,0.));
#60773=CARTESIAN_POINT('Ctrl Pts',(46.3491768270655,-53.5299661791385,12.));
#60774=CARTESIAN_POINT('Ctrl Pts',(46.3674699081046,-53.5413655657327,0.));
#60775=CARTESIAN_POINT('Ctrl Pts',(46.3674699081046,-53.5413655657327,12.));
#60776=CARTESIAN_POINT('Ctrl Pts',(46.3858158321059,-53.5527716683048,0.));
#60777=CARTESIAN_POINT('Ctrl Pts',(46.3858158321059,-53.5527716683048,12.));
#60778=CARTESIAN_POINT('Ctrl Pts',(46.4042145078701,-53.5641843412559,0.));
#60779=CARTESIAN_POINT('Ctrl Pts',(46.4042145078701,-53.5641843412559,12.));
#60780=CARTESIAN_POINT('Ctrl Pts',(46.4226658445474,-53.5756034397481,0.));
#60781=CARTESIAN_POINT('Ctrl Pts',(46.4226658445474,-53.5756034397481,12.));
#60782=CARTESIAN_POINT('Ctrl Pts',(46.4411697516478,-53.5870288197166,0.));
#60783=CARTESIAN_POINT('Ctrl Pts',(46.4411697516478,-53.5870288197166,12.));
#60784=CARTESIAN_POINT('Ctrl Pts',(46.459726139052,-53.5984603378855,0.));
#60785=CARTESIAN_POINT('Ctrl Pts',(46.459726139052,-53.5984603378855,12.));
#60786=CARTESIAN_POINT('Ctrl Pts',(46.4783349170173,-53.6098978517859,0.));
#60787=CARTESIAN_POINT('Ctrl Pts',(46.4783349170173,-53.6098978517859,12.));
#60788=CARTESIAN_POINT('Ctrl Pts',(46.496995996177,-53.6213412197533,0.));
#60789=CARTESIAN_POINT('Ctrl Pts',(46.496995996177,-53.6213412197533,12.));
#60790=CARTESIAN_POINT('Ctrl Pts',(46.5157092875373,-53.6327903009094,0.));
#60791=CARTESIAN_POINT('Ctrl Pts',(46.5157092875373,-53.6327903009094,12.));
#60792=CARTESIAN_POINT('Ctrl Pts',(46.5344747024676,-53.6442449551455,0.));
#60793=CARTESIAN_POINT('Ctrl Pts',(46.5344747024676,-53.6442449551455,12.));
#60794=CARTESIAN_POINT('Ctrl Pts',(46.5532921526901,-53.6557050431071,0.));
#60795=CARTESIAN_POINT('Ctrl Pts',(46.5532921526901,-53.6557050431071,12.));
#60796=CARTESIAN_POINT('Ctrl Pts',(46.5721615502591,-53.6671704261737,0.));
#60797=CARTESIAN_POINT('Ctrl Pts',(46.5721615502591,-53.6671704261737,12.));
#60798=CARTESIAN_POINT('Ctrl Pts',(46.5910828075653,-53.678640966456,0.));
#60799=CARTESIAN_POINT('Ctrl Pts',(46.5910828075653,-53.678640966456,12.));
#60800=CARTESIAN_POINT('Ctrl Pts',(46.6100558373402,-53.6901165267941,0.));
#60801=CARTESIAN_POINT('Ctrl Pts',(46.6100558373402,-53.6901165267941,12.));
#60802=CARTESIAN_POINT('Ctrl Pts',(46.6290805526559,-53.701596970754,0.));
#60803=CARTESIAN_POINT('Ctrl Pts',(46.6290805526559,-53.701596970754,12.));
#60804=CARTESIAN_POINT('Ctrl Pts',(46.6481568669216,-53.7130821626263,0.));
#60805=CARTESIAN_POINT('Ctrl Pts',(46.6481568669216,-53.7130821626263,12.));
#60806=CARTESIAN_POINT('Ctrl Pts',(46.6672846938752,-53.7245719674222,0.));
#60807=CARTESIAN_POINT('Ctrl Pts',(46.6672846938752,-53.7245719674222,12.));
#60808=CARTESIAN_POINT('Ctrl Pts',(46.6864639475863,-53.7360662508677,0.));
#60809=CARTESIAN_POINT('Ctrl Pts',(46.6864639475863,-53.7360662508677,12.));
#60810=CARTESIAN_POINT('Ctrl Pts',(46.7056945424559,-53.7475648793948,0.));
#60811=CARTESIAN_POINT('Ctrl Pts',(46.7056945424559,-53.7475648793948,12.));
#60812=CARTESIAN_POINT('Ctrl Pts',(46.724976393213,-53.7590677201344,0.));
#60813=CARTESIAN_POINT('Ctrl Pts',(46.724976393213,-53.7590677201344,12.));
#60814=CARTESIAN_POINT('Ctrl Pts',(46.7443094149041,-53.770574640907,0.));
#60815=CARTESIAN_POINT('Ctrl Pts',(46.7443094149041,-53.770574640907,12.));
#60816=CARTESIAN_POINT('Ctrl Pts',(46.7636935228851,-53.782085510217,0.));
#60817=CARTESIAN_POINT('Ctrl Pts',(46.7636935228851,-53.782085510217,12.));
#60818=CARTESIAN_POINT('Ctrl Pts',(46.7831286328268,-53.7936001972468,0.));
#60819=CARTESIAN_POINT('Ctrl Pts',(46.7831286328268,-53.7936001972468,12.));
#60820=CARTESIAN_POINT('Ctrl Pts',(46.8026146607144,-53.8051185718525,0.));
#60821=CARTESIAN_POINT('Ctrl Pts',(46.8026146607144,-53.8051185718525,12.));
#60822=CARTESIAN_POINT('Ctrl Pts',(46.8221515228459,-53.8166405045582,0.));
#60823=CARTESIAN_POINT('Ctrl Pts',(46.8221515228459,-53.8166405045582,12.));
#60824=CARTESIAN_POINT('Ctrl Pts',(46.8417391358231,-53.8281658665517,0.));
#60825=CARTESIAN_POINT('Ctrl Pts',(46.8417391358231,-53.8281658665517,12.));
#60826=CARTESIAN_POINT('Ctrl Pts',(46.8613774165452,-53.8396945296777,0.));
#60827=CARTESIAN_POINT('Ctrl Pts',(46.8613774165452,-53.8396945296777,12.));
#60828=CARTESIAN_POINT('Ctrl Pts',(46.8810662822146,-53.851226366434,0.));
#60829=CARTESIAN_POINT('Ctrl Pts',(46.8810662822146,-53.851226366434,12.));
#60830=CARTESIAN_POINT('Ctrl Pts',(46.900805650336,-53.8627612499648,0.));
#60831=CARTESIAN_POINT('Ctrl Pts',(46.900805650336,-53.8627612499648,12.));
#60832=CARTESIAN_POINT('Ctrl Pts',(46.9205954387128,-53.8742990540557,0.));
#60833=CARTESIAN_POINT('Ctrl Pts',(46.9205954387128,-53.8742990540557,12.));
#60834=CARTESIAN_POINT('Ctrl Pts',(46.9404355654381,-53.8858396531277,0.));
#60835=CARTESIAN_POINT('Ctrl Pts',(46.9404355654381,-53.8858396531277,12.));
#60836=CARTESIAN_POINT('Ctrl Pts',(46.9603259488894,-53.8973829222317,0.));
#60837=CARTESIAN_POINT('Ctrl Pts',(46.9603259488894,-53.8973829222317,12.));
#60838=CARTESIAN_POINT('Ctrl Pts',(46.9802665077342,-53.9089287370436,0.));
#60839=CARTESIAN_POINT('Ctrl Pts',(46.9802665077342,-53.9089287370436,12.));
#60840=CARTESIAN_POINT('Ctrl Pts',(47.0002571609286,-53.9204769738584,0.));
#60841=CARTESIAN_POINT('Ctrl Pts',(47.0002571609286,-53.9204769738584,12.));
#60842=CARTESIAN_POINT('Ctrl Pts',(47.0202978277148,-53.9320275095864,0.));
#60843=CARTESIAN_POINT('Ctrl Pts',(47.0202978277148,-53.9320275095864,12.));
#60844=CARTESIAN_POINT('Ctrl Pts',(47.04038842761,-53.9435802217468,0.));
#60845=CARTESIAN_POINT('Ctrl Pts',(47.04038842761,-53.9435802217468,12.));
#60846=CARTESIAN_POINT('Ctrl Pts',(47.0605288804042,-53.9551349884637,0.));
#60847=CARTESIAN_POINT('Ctrl Pts',(47.0605288804042,-53.9551349884637,12.));
#60848=CARTESIAN_POINT('Ctrl Pts',(47.0807191061673,-53.9666916884624,0.));
#60849=CARTESIAN_POINT('Ctrl Pts',(47.0807191061673,-53.9666916884624,12.));
#60850=CARTESIAN_POINT('Ctrl Pts',(47.1009590252466,-53.9782502010642,0.));
#60851=CARTESIAN_POINT('Ctrl Pts',(47.1009590252466,-53.9782502010642,12.));
#60852=CARTESIAN_POINT('Ctrl Pts',(47.1212485582632,-53.9898104061809,0.));
#60853=CARTESIAN_POINT('Ctrl Pts',(47.1212485582632,-53.9898104061809,12.));
#60854=CARTESIAN_POINT('Ctrl Pts',(47.1415876261012,-54.0013721843094,0.));
#60855=CARTESIAN_POINT('Ctrl Pts',(47.1415876261012,-54.0013721843094,12.));
#60856=CARTESIAN_POINT('Ctrl Pts',(47.161976149906,-54.0129354165269,0.));
#60857=CARTESIAN_POINT('Ctrl Pts',(47.161976149906,-54.0129354165269,12.));
#60858=CARTESIAN_POINT('Ctrl Pts',(47.1824140510906,-54.0244999844872,0.));
#60859=CARTESIAN_POINT('Ctrl Pts',(47.1824140510906,-54.0244999844872,12.));
#60860=CARTESIAN_POINT('Ctrl Pts',(47.2029012513334,-54.0360657704156,0.));
#60861=CARTESIAN_POINT('Ctrl Pts',(47.2029012513334,-54.0360657704156,12.));
#60862=CARTESIAN_POINT('Ctrl Pts',(47.2234376725752,-54.047632657105,0.));
#60863=CARTESIAN_POINT('Ctrl Pts',(47.2234376725752,-54.047632657105,12.));
#60864=CARTESIAN_POINT('Ctrl Pts',(47.2440232370085,-54.0592005279108,0.));
#60865=CARTESIAN_POINT('Ctrl Pts',(47.2440232370085,-54.0592005279108,12.));
#60866=CARTESIAN_POINT('Ctrl Pts',(47.2646578670767,-54.0707692667461,0.));
#60867=CARTESIAN_POINT('Ctrl Pts',(47.2646578670767,-54.0707692667461,12.));
#60868=CARTESIAN_POINT('Ctrl Pts',(47.2853414854805,-54.082338758079,0.));
#60869=CARTESIAN_POINT('Ctrl Pts',(47.2853414854805,-54.082338758079,12.));
#60870=CARTESIAN_POINT('Ctrl Pts',(47.3060740151754,-54.0939088869271,0.));
#60871=CARTESIAN_POINT('Ctrl Pts',(47.3060740151754,-54.0939088869271,12.));
#60872=CARTESIAN_POINT('Ctrl Pts',(47.326855379369,-54.1054795388538,0.));
#60873=CARTESIAN_POINT('Ctrl Pts',(47.326855379369,-54.1054795388538,12.));
#60874=CARTESIAN_POINT('Ctrl Pts',(47.3476855015095,-54.1170505999637,0.));
#60875=CARTESIAN_POINT('Ctrl Pts',(47.3476855015095,-54.1170505999637,12.));
#60876=CARTESIAN_POINT('Ctrl Pts',(47.3685643052867,-54.1286219568981,0.));
#60877=CARTESIAN_POINT('Ctrl Pts',(47.3685643052867,-54.1286219568981,12.));
#60878=CARTESIAN_POINT('Ctrl Pts',(47.3894917146361,-54.1401934968306,0.));
#60879=CARTESIAN_POINT('Ctrl Pts',(47.3894917146361,-54.1401934968306,12.));
#60880=CARTESIAN_POINT('Ctrl Pts',(47.4104676537381,-54.1517651074638,0.));
#60881=CARTESIAN_POINT('Ctrl Pts',(47.4104676537381,-54.1517651074638,12.));
#60882=CARTESIAN_POINT('Ctrl Pts',(47.4314920470142,-54.163336677024,0.));
#60883=CARTESIAN_POINT('Ctrl Pts',(47.4314920470142,-54.163336677024,12.));
#60884=CARTESIAN_POINT('Ctrl Pts',(47.4525648191173,-54.1749080942593,0.));
#60885=CARTESIAN_POINT('Ctrl Pts',(47.4525648191173,-54.1749080942593,12.));
#60886=CARTESIAN_POINT('Ctrl Pts',(47.473685894932,-54.1864792484343,0.));
#60887=CARTESIAN_POINT('Ctrl Pts',(47.473685894932,-54.1864792484343,12.));
#60888=CARTESIAN_POINT('Ctrl Pts',(47.4948551995798,-54.1980500293267,0.));
#60889=CARTESIAN_POINT('Ctrl Pts',(47.4948551995798,-54.1980500293267,12.));
#60890=CARTESIAN_POINT('Ctrl Pts',(47.5160726584172,-54.2096203272228,0.));
#60891=CARTESIAN_POINT('Ctrl Pts',(47.5160726584172,-54.2096203272228,12.));
#60892=CARTESIAN_POINT('Ctrl Pts',(47.5373381970328,-54.2211900329141,0.));
#60893=CARTESIAN_POINT('Ctrl Pts',(47.5373381970328,-54.2211900329141,12.));
#60894=CARTESIAN_POINT('Ctrl Pts',(47.5586517412368,-54.232759037693,0.));
#60895=CARTESIAN_POINT('Ctrl Pts',(47.5586517412368,-54.232759037693,12.));
#60896=CARTESIAN_POINT('Ctrl Pts',(47.5800132170614,-54.2443272333498,0.));
#60897=CARTESIAN_POINT('Ctrl Pts',(47.5800132170614,-54.2443272333498,12.));
#60898=CARTESIAN_POINT('Ctrl Pts',(47.6014225507663,-54.2558945121684,0.));
#60899=CARTESIAN_POINT('Ctrl Pts',(47.6014225507663,-54.2558945121684,12.));
#60900=CARTESIAN_POINT('Ctrl Pts',(47.6228796688376,-54.2674607669228,0.));
#60901=CARTESIAN_POINT('Ctrl Pts',(47.6228796688376,-54.2674607669228,12.));
#60902=CARTESIAN_POINT('Ctrl Pts',(47.6443844979846,-54.2790258908736,0.));
#60903=CARTESIAN_POINT('Ctrl Pts',(47.6443844979846,-54.2790258908736,12.));
#60904=CARTESIAN_POINT('Ctrl Pts',(47.6659369651299,-54.2905897777647,0.));
#60905=CARTESIAN_POINT('Ctrl Pts',(47.6659369651299,-54.2905897777647,12.));
#60906=CARTESIAN_POINT('Ctrl Pts',(47.6875369974086,-54.3021523218188,0.));
#60907=CARTESIAN_POINT('Ctrl Pts',(47.6875369974086,-54.3021523218188,12.));
#60908=CARTESIAN_POINT('Ctrl Pts',(47.7091845221747,-54.3137134177345,0.));
#60909=CARTESIAN_POINT('Ctrl Pts',(47.7091845221747,-54.3137134177345,12.));
#60910=CARTESIAN_POINT('Ctrl Pts',(47.7308794669994,-54.3252729606824,0.));
#60911=CARTESIAN_POINT('Ctrl Pts',(47.7308794669994,-54.3252729606824,12.));
#60912=CARTESIAN_POINT('Ctrl Pts',(47.7526217596694,-54.3368308463023,0.));
#60913=CARTESIAN_POINT('Ctrl Pts',(47.7526217596694,-54.3368308463023,12.));
#60914=CARTESIAN_POINT('Ctrl Pts',(47.7744113281767,-54.3483869706998,0.));
#60915=CARTESIAN_POINT('Ctrl Pts',(47.7744113281767,-54.3483869706998,12.));
#60916=CARTESIAN_POINT('Ctrl Pts',(47.7962481007179,-54.3599412304431,0.));
#60917=CARTESIAN_POINT('Ctrl Pts',(47.7962481007179,-54.3599412304431,12.));
#60918=CARTESIAN_POINT('Ctrl Pts',(47.8181320056988,-54.3714935225585,0.));
#60919=CARTESIAN_POINT('Ctrl Pts',(47.8181320056988,-54.3714935225585,12.));
#60920=CARTESIAN_POINT('Ctrl Pts',(47.8400629717352,-54.3830437445275,0.));
#60921=CARTESIAN_POINT('Ctrl Pts',(47.8400629717352,-54.3830437445275,12.));
#60922=CARTESIAN_POINT('Ctrl Pts',(47.8620409276495,-54.3945917942835,0.));
#60923=CARTESIAN_POINT('Ctrl Pts',(47.8620409276495,-54.3945917942835,12.));
#60924=CARTESIAN_POINT('Ctrl Pts',(47.8840658024626,-54.4061375702088,0.));
#60925=CARTESIAN_POINT('Ctrl Pts',(47.8840658024626,-54.4061375702088,12.));
#60926=CARTESIAN_POINT('Ctrl Pts',(47.9061375253909,-54.4176809711324,0.));
#60927=CARTESIAN_POINT('Ctrl Pts',(47.9061375253909,-54.4176809711324,12.));
#60928=CARTESIAN_POINT('Ctrl Pts',(47.9282560258528,-54.4292218963253,0.));
#60929=CARTESIAN_POINT('Ctrl Pts',(47.9282560258528,-54.4292218963253,12.));
#60930=CARTESIAN_POINT('Ctrl Pts',(47.9504212334681,-54.4407602454974,0.));
#60931=CARTESIAN_POINT('Ctrl Pts',(47.9504212334681,-54.4407602454974,12.));
#60932=CARTESIAN_POINT('Ctrl Pts',(47.972633078057,-54.4522959187952,0.));
#60933=CARTESIAN_POINT('Ctrl Pts',(47.972633078057,-54.4522959187952,12.));
#60934=CARTESIAN_POINT('Ctrl Pts',(47.9948914896316,-54.4638288167991,0.));
#60935=CARTESIAN_POINT('Ctrl Pts',(47.9948914896316,-54.4638288167991,12.));
#60936=CARTESIAN_POINT('Ctrl Pts',(48.0171963983912,-54.4753588405202,0.));
#60937=CARTESIAN_POINT('Ctrl Pts',(48.0171963983912,-54.4753588405202,12.));
#60938=CARTESIAN_POINT('Ctrl Pts',(48.039547734729,-54.4868858913961,0.));
#60939=CARTESIAN_POINT('Ctrl Pts',(48.039547734729,-54.4868858913961,12.));
#60940=CARTESIAN_POINT('Ctrl Pts',(48.0619454292321,-54.4984098712883,0.));
#60941=CARTESIAN_POINT('Ctrl Pts',(48.0619454292321,-54.4984098712883,12.));
#60942=CARTESIAN_POINT('Ctrl Pts',(48.0843894126807,-54.5099306824788,0.));
#60943=CARTESIAN_POINT('Ctrl Pts',(48.0843894126807,-54.5099306824788,12.));
#60944=CARTESIAN_POINT('Ctrl Pts',(48.1068796160406,-54.5214482276679,0.));
#60945=CARTESIAN_POINT('Ctrl Pts',(48.1068796160406,-54.5214482276679,12.));
#60946=CARTESIAN_POINT('Ctrl Pts',(48.1294159704571,-54.5329624099719,0.));
#60947=CARTESIAN_POINT('Ctrl Pts',(48.1294159704571,-54.5329624099719,12.));
#60948=CARTESIAN_POINT('Ctrl Pts',(48.1519984072617,-54.5444731329196,0.));
#60949=CARTESIAN_POINT('Ctrl Pts',(48.1519984072617,-54.5444731329196,12.));
#60950=CARTESIAN_POINT('Ctrl Pts',(48.1746268579732,-54.5559803004487,0.));
#60951=CARTESIAN_POINT('Ctrl Pts',(48.1746268579732,-54.5559803004487,12.));
#60952=CARTESIAN_POINT('Ctrl Pts',(48.1973012542966,-54.5674838169041,0.));
#60953=CARTESIAN_POINT('Ctrl Pts',(48.1973012542966,-54.5674838169041,12.));
#60954=CARTESIAN_POINT('Ctrl Pts',(48.2200215281178,-54.5789835870348,0.));
#60955=CARTESIAN_POINT('Ctrl Pts',(48.2200215281178,-54.5789835870348,12.));
#60956=CARTESIAN_POINT('Ctrl Pts',(48.2427876114955,-54.5904795159936,0.));
#60957=CARTESIAN_POINT('Ctrl Pts',(48.2427876114955,-54.5904795159936,12.));
#60958=CARTESIAN_POINT('Ctrl Pts',(48.2655994366672,-54.6019715093319,0.));
#60959=CARTESIAN_POINT('Ctrl Pts',(48.2655994366672,-54.6019715093319,12.));
#60960=CARTESIAN_POINT('Ctrl Pts',(48.288456936051,-54.6134594729964,0.));
#60961=CARTESIAN_POINT('Ctrl Pts',(48.288456936051,-54.6134594729964,12.));
#60962=CARTESIAN_POINT('Ctrl Pts',(48.3113600422443,-54.6249433133262,0.));
#60963=CARTESIAN_POINT('Ctrl Pts',(48.3113600422443,-54.6249433133262,12.));
#60964=CARTESIAN_POINT('Ctrl Pts',(48.3343086880192,-54.636422937049,0.));
#60965=CARTESIAN_POINT('Ctrl Pts',(48.3343086880192,-54.636422937049,12.));
#60966=CARTESIAN_POINT('Ctrl Pts',(48.3573028063121,-54.647898251279,0.));
#60967=CARTESIAN_POINT('Ctrl Pts',(48.3573028063121,-54.647898251279,12.));
#60968=CARTESIAN_POINT('Ctrl Pts',(48.3803423302294,-54.6593691635143,0.));
#60969=CARTESIAN_POINT('Ctrl Pts',(48.3803423302294,-54.6593691635143,12.));
#60970=CARTESIAN_POINT('Ctrl Pts',(48.4034271930516,-54.6708355816359,0.));
#60971=CARTESIAN_POINT('Ctrl Pts',(48.4034271930516,-54.6708355816359,12.));
#60972=CARTESIAN_POINT('Ctrl Pts',(48.4265573282341,-54.6822974139065,0.));
#60973=CARTESIAN_POINT('Ctrl Pts',(48.4265573282341,-54.6822974139065,12.));
#60974=CARTESIAN_POINT('Ctrl Pts',(48.4497326694051,-54.6937545689694,0.));
#60975=CARTESIAN_POINT('Ctrl Pts',(48.4497326694051,-54.6937545689694,12.));
#60976=CARTESIAN_POINT('Ctrl Pts',(48.4729531503565,-54.7052069558493,0.));
#60977=CARTESIAN_POINT('Ctrl Pts',(48.4729531503565,-54.7052069558493,12.));
#60978=CARTESIAN_POINT('Ctrl Pts',(48.4962187050451,-54.7166544839475,0.));
#60979=CARTESIAN_POINT('Ctrl Pts',(48.4962187050451,-54.7166544839475,12.));
#60980=CARTESIAN_POINT('Ctrl Pts',(48.5195292675955,-54.7280970630346,0.));
#60981=CARTESIAN_POINT('Ctrl Pts',(48.5195292675955,-54.7280970630346,12.));
#60982=CARTESIAN_POINT('Ctrl Pts',(48.5428847722974,-54.7395346032451,0.));
#60983=CARTESIAN_POINT('Ctrl Pts',(48.5428847722974,-54.7395346032451,12.));
#60984=CARTESIAN_POINT('Ctrl Pts',(48.5662851536027,-54.7509670150716,0.));
#60985=CARTESIAN_POINT('Ctrl Pts',(48.5662851536027,-54.7509670150716,12.));
#60986=CARTESIAN_POINT('Ctrl Pts',(48.5897303461131,-54.7623942093591,0.));
#60987=CARTESIAN_POINT('Ctrl Pts',(48.5897303461131,-54.7623942093591,12.));
#60988=CARTESIAN_POINT('Ctrl Pts',(48.6132202845792,-54.773816097304,0.));
#60989=CARTESIAN_POINT('Ctrl Pts',(48.6132202845792,-54.773816097304,12.));
#60990=CARTESIAN_POINT('Ctrl Pts',(48.6367549039121,-54.7852325904591,0.));
#60991=CARTESIAN_POINT('Ctrl Pts',(48.6367549039121,-54.7852325904591,12.));
#60992=CARTESIAN_POINT('Ctrl Pts',(48.6603341391891,-54.7966436007395,0.));
#60993=CARTESIAN_POINT('Ctrl Pts',(48.6603341391891,-54.7966436007395,12.));
#60994=CARTESIAN_POINT('Ctrl Pts',(48.6839579256565,-54.8080490404274,0.));
#60995=CARTESIAN_POINT('Ctrl Pts',(48.6839579256565,-54.8080490404274,12.));
#60996=CARTESIAN_POINT('Ctrl Pts',(48.7076261987284,-54.8194488221803,0.));
#60997=CARTESIAN_POINT('Ctrl Pts',(48.7076261987284,-54.8194488221803,12.));
#60998=CARTESIAN_POINT('Ctrl Pts',(48.7313388939834,-54.8308428590334,0.));
#60999=CARTESIAN_POINT('Ctrl Pts',(48.7313388939834,-54.8308428590334,12.));
#61000=CARTESIAN_POINT('Ctrl Pts',(48.755095947159,-54.8422310643752,0.));
#61001=CARTESIAN_POINT('Ctrl Pts',(48.755095947159,-54.8422310643752,12.));
#61002=CARTESIAN_POINT('Ctrl Pts',(48.7788972941431,-54.8536133519285,0.));
#61003=CARTESIAN_POINT('Ctrl Pts',(48.7788972941431,-54.8536133519285,12.));
#61004=CARTESIAN_POINT('Ctrl Pts',(48.8027428709613,-54.8649896357284,0.));
#61005=CARTESIAN_POINT('Ctrl Pts',(48.8027428709613,-54.8649896357284,12.));
#61006=CARTESIAN_POINT('Ctrl Pts',(48.8266326137629,-54.8763598301045,0.));
#61007=CARTESIAN_POINT('Ctrl Pts',(48.8266326137629,-54.8763598301045,12.));
#61008=CARTESIAN_POINT('Ctrl Pts',(48.8505664587984,-54.8877238496577,0.));
#61009=CARTESIAN_POINT('Ctrl Pts',(48.8505664587984,-54.8877238496577,12.));
#61010=CARTESIAN_POINT('Ctrl Pts',(48.8745443424488,-54.8990816092964,0.));
#61011=CARTESIAN_POINT('Ctrl Pts',(48.8745443424488,-54.8990816092964,12.));
#61012=CARTESIAN_POINT('Ctrl Pts',(48.8985662012535,-54.910433024275,0.));
#61013=CARTESIAN_POINT('Ctrl Pts',(48.8985662012535,-54.910433024275,12.));
#61014=CARTESIAN_POINT('Ctrl Pts',(48.922631971937,-54.9217780102357,0.));
#61015=CARTESIAN_POINT('Ctrl Pts',(48.922631971937,-54.9217780102357,12.));
#61016=CARTESIAN_POINT('Ctrl Pts',(48.9467415914266,-54.933116483242,0.));
#61017=CARTESIAN_POINT('Ctrl Pts',(48.9467415914266,-54.933116483242,12.));
#61018=CARTESIAN_POINT('Ctrl Pts',(48.9708949968789,-54.9444483598372,0.));
#61019=CARTESIAN_POINT('Ctrl Pts',(48.9708949968789,-54.9444483598372,12.));
#61020=CARTESIAN_POINT('Ctrl Pts',(48.995092125652,-54.9557735569936,0.));
#61021=CARTESIAN_POINT('Ctrl Pts',(48.995092125652,-54.9557735569936,12.));
#61022=CARTESIAN_POINT('Ctrl Pts',(49.0193329152475,-54.9670919920024,0.));
#61023=CARTESIAN_POINT('Ctrl Pts',(49.0193329152475,-54.9670919920024,12.));
#61024=CARTESIAN_POINT('Ctrl Pts',(49.0436173032527,-54.9784035823764,0.));
#61025=CARTESIAN_POINT('Ctrl Pts',(49.0436173032527,-54.9784035823764,12.));
#61026=CARTESIAN_POINT('Ctrl Pts',(49.0679452272871,-54.9897082457607,0.));
#61027=CARTESIAN_POINT('Ctrl Pts',(49.0679452272871,-54.9897082457607,12.));
#61028=CARTESIAN_POINT('Ctrl Pts',(49.0923166249222,-55.0010058998111,0.));
#61029=CARTESIAN_POINT('Ctrl Pts',(49.0923166249222,-55.0010058998111,12.));
#61030=CARTESIAN_POINT('Ctrl Pts',(49.1167314336737,-55.0122964621868,0.));
#61031=CARTESIAN_POINT('Ctrl Pts',(49.1167314336737,-55.0122964621868,12.));
#61032=CARTESIAN_POINT('Ctrl Pts',(49.1411895911645,-55.0235798508056,0.));
#61033=CARTESIAN_POINT('Ctrl Pts',(49.1411895911645,-55.0235798508056,12.));
#61034=CARTESIAN_POINT('Ctrl Pts',(49.1656910352484,-55.0348559840462,0.));
#61035=CARTESIAN_POINT('Ctrl Pts',(49.1656910352484,-55.0348559840462,12.));
#61036=CARTESIAN_POINT('Ctrl Pts',(49.1902357041462,-55.0461247809745,0.));
#61037=CARTESIAN_POINT('Ctrl Pts',(49.1902357041462,-55.0461247809745,12.));
#61038=CARTESIAN_POINT('Ctrl Pts',(49.2148235365694,-55.0573861615569,0.));
#61039=CARTESIAN_POINT('Ctrl Pts',(49.2148235365694,-55.0573861615569,12.));
#61040=CARTESIAN_POINT('Ctrl Pts',(49.2394544718512,-55.0686400468911,0.));
#61041=CARTESIAN_POINT('Ctrl Pts',(49.2394544718512,-55.0686400468911,12.));
#61042=CARTESIAN_POINT('Ctrl Pts',(49.2641284496496,-55.0798863586986,0.));
#61043=CARTESIAN_POINT('Ctrl Pts',(49.2641284496496,-55.0798863586986,12.));
#61044=CARTESIAN_POINT('Ctrl Pts',(49.2888454096544,-55.0911250188282,0.));
#61045=CARTESIAN_POINT('Ctrl Pts',(49.2888454096544,-55.0911250188282,12.));
#61046=CARTESIAN_POINT('Ctrl Pts',(49.3136052912614,-55.1023559487133,0.));
#61047=CARTESIAN_POINT('Ctrl Pts',(49.3136052912614,-55.1023559487133,12.));
#61048=CARTESIAN_POINT('Ctrl Pts',(49.3384080333166,-55.1135790689475,0.));
#61049=CARTESIAN_POINT('Ctrl Pts',(49.3384080333166,-55.1135790689475,12.));
#61050=CARTESIAN_POINT('Ctrl Pts',(49.3632535736744,-55.1247942985649,0.));
#61051=CARTESIAN_POINT('Ctrl Pts',(49.3632535736744,-55.1247942985649,12.));
#61052=CARTESIAN_POINT('Ctrl Pts',(49.3881418495529,-55.1360015556262,0.));
#61053=CARTESIAN_POINT('Ctrl Pts',(49.3881418495529,-55.1360015556262,12.));
#61054=CARTESIAN_POINT('Ctrl Pts',(49.413072798324,-55.1472007585224,0.));
#61055=CARTESIAN_POINT('Ctrl Pts',(49.413072798324,-55.1472007585224,12.));
#61056=CARTESIAN_POINT('Ctrl Pts',(49.4380463581989,-55.158391827114,0.));
#61057=CARTESIAN_POINT('Ctrl Pts',(49.4380463581989,-55.158391827114,12.));
#61058=CARTESIAN_POINT('Ctrl Pts',(49.4630624688787,-55.1695746838168,0.));
#61059=CARTESIAN_POINT('Ctrl Pts',(49.4630624688787,-55.1695746838168,12.));
#61060=CARTESIAN_POINT('Ctrl Pts',(49.4881210723921,-55.1807492550073,0.));
#61061=CARTESIAN_POINT('Ctrl Pts',(49.4881210723921,-55.1807492550073,12.));
#61062=CARTESIAN_POINT('Ctrl Pts',(49.5132221132916,-55.1919154713569,0.));
#61063=CARTESIAN_POINT('Ctrl Pts',(49.5132221132916,-55.1919154713569,12.));
#61064=CARTESIAN_POINT('Ctrl Pts',(49.5383655367987,-55.2030732647222,0.));
#61065=CARTESIAN_POINT('Ctrl Pts',(49.5383655367987,-55.2030732647222,12.));
#61066=CARTESIAN_POINT('Ctrl Pts',(49.5635512873368,-55.2142225656943,0.));
#61067=CARTESIAN_POINT('Ctrl Pts',(49.5635512873368,-55.2142225656943,12.));
#61068=CARTESIAN_POINT('Ctrl Pts',(49.5887793068337,-55.225363300765,0.));
#61069=CARTESIAN_POINT('Ctrl Pts',(49.5887793068337,-55.225363300765,12.));
#61070=CARTESIAN_POINT('Ctrl Pts',(49.6140495332865,-55.2364953899423,0.));
#61071=CARTESIAN_POINT('Ctrl Pts',(49.6140495332865,-55.2364953899423,12.));
#61072=CARTESIAN_POINT('Ctrl Pts',(49.6393618987614,-55.2476187434204,0.));
#61073=CARTESIAN_POINT('Ctrl Pts',(49.6393618987614,-55.2476187434204,12.));
#61074=CARTESIAN_POINT('Ctrl Pts',(49.6647163322457,-55.2587332663982,0.));
#61075=CARTESIAN_POINT('Ctrl Pts',(49.6647163322457,-55.2587332663982,12.));
#61076=CARTESIAN_POINT('Ctrl Pts',(49.690112763181,-55.2698388650215,0.));
#61077=CARTESIAN_POINT('Ctrl Pts',(49.690112763181,-55.2698388650215,12.));
#61078=CARTESIAN_POINT('Ctrl Pts',(49.7155511248629,-55.2809354521616,0.));
#61079=CARTESIAN_POINT('Ctrl Pts',(49.7155511248629,-55.2809354521616,12.));
#61080=CARTESIAN_POINT('Ctrl Pts',(49.7410313576444,-55.292022952748,0.));
#61081=CARTESIAN_POINT('Ctrl Pts',(49.7410313576444,-55.292022952748,12.));
#61082=CARTESIAN_POINT('Ctrl Pts',(49.7665534128269,-55.3031013105578,0.));
#61083=CARTESIAN_POINT('Ctrl Pts',(49.7665534128269,-55.3031013105578,12.));
#61084=CARTESIAN_POINT('Ctrl Pts',(49.7921172540185,-55.3141704897307,0.));
#61085=CARTESIAN_POINT('Ctrl Pts',(49.7921172540185,-55.3141704897307,12.));
#61086=CARTESIAN_POINT('Ctrl Pts',(49.817722855186,-55.3252304694066,0.));
#61087=CARTESIAN_POINT('Ctrl Pts',(49.817722855186,-55.3252304694066,12.));
#61088=CARTESIAN_POINT('Ctrl Pts',(49.8382407306675,-55.3340710859607,0.));
#61089=CARTESIAN_POINT('Ctrl Pts',(49.8382407306675,-55.3340710859607,12.));
#61090=CARTESIAN_POINT('Ctrl Pts',(49.8536479176573,-55.340697403233,0.));
#61091=CARTESIAN_POINT('Ctrl Pts',(49.8536479176573,-55.340697403233,12.));
#61092=CARTESIAN_POINT('Ctrl Pts',(49.8639277221471,-55.3451131058727,0.));
#61093=CARTESIAN_POINT('Ctrl Pts',(49.8639277221471,-55.3451131058727,12.));
#61094=CARTESIAN_POINT('Ctrl Pts',(49.869069711016,-55.3473204966403,0.));
#61095=CARTESIAN_POINT('Ctrl Pts',(49.869069711016,-55.3473204966403,12.));
#61096=CARTESIAN_POINT('',(45.6458539113724,-53.0702932034641,0.));
#61097=CARTESIAN_POINT('Ctrl Pts',(45.6458539113724,-53.0702932034641,0.));
#61098=CARTESIAN_POINT('Ctrl Pts',(45.6490568514089,-53.0724894921849,0.));
#61099=CARTESIAN_POINT('Ctrl Pts',(45.6554684028145,-53.0768833804193,0.));
#61100=CARTESIAN_POINT('Ctrl Pts',(45.6651027439241,-53.0834781451546,0.));
#61101=CARTESIAN_POINT('Ctrl Pts',(45.6779825614231,-53.0922790298409,0.));
#61102=CARTESIAN_POINT('Ctrl Pts',(45.694139048907,-53.1032932328857,0.));
#61103=CARTESIAN_POINT('Ctrl Pts',(45.7103522376696,-53.114320495492,0.));
#61104=CARTESIAN_POINT('Ctrl Pts',(45.7266220897003,-53.1253607414872,0.));
#61105=CARTESIAN_POINT('Ctrl Pts',(45.7429485300823,-53.1364138384693,0.));
#61106=CARTESIAN_POINT('Ctrl Pts',(45.7593314474501,-53.1474795996053,0.));
#61107=CARTESIAN_POINT('Ctrl Pts',(45.7757707100618,-53.1585578076444,0.));
#61108=CARTESIAN_POINT('Ctrl Pts',(45.7922661780005,-53.1696482334487,0.));
#61109=CARTESIAN_POINT('Ctrl Pts',(45.8088177165089,-53.1807506560933,0.));
#61110=CARTESIAN_POINT('Ctrl Pts',(45.8254252099957,-53.1918648840541,0.));
#61111=CARTESIAN_POINT('Ctrl Pts',(45.8420885575349,-53.2029907483557,0.));
#61112=CARTESIAN_POINT('Ctrl Pts',(45.8588076662582,-53.2141280925439,0.));
#61113=CARTESIAN_POINT('Ctrl Pts',(45.8755824458722,-53.2252767643662,0.));
#61114=CARTESIAN_POINT('Ctrl Pts',(45.8924128018379,-53.2364366054306,0.));
#61115=CARTESIAN_POINT('Ctrl Pts',(45.9092986319377,-53.2476074460017,0.));
#61116=CARTESIAN_POINT('Ctrl Pts',(45.9262398298349,-53.2587891103866,0.));
#61117=CARTESIAN_POINT('Ctrl Pts',(45.9432362873008,-53.2699814203105,0.));
#61118=CARTESIAN_POINT('Ctrl Pts',(45.9602878967698,-53.2811841987926,0.));
#61119=CARTESIAN_POINT('Ctrl Pts',(45.9773945542384,-53.292397274555,0.));
#61120=CARTESIAN_POINT('Ctrl Pts',(45.9945561591453,-53.3036204818329,0.));
#61121=CARTESIAN_POINT('Ctrl Pts',(46.0117726129873,-53.3148536582635,0.));
#61122=CARTESIAN_POINT('Ctrl Pts',(46.02904381836,-53.326096643428,0.));
#61123=CARTESIAN_POINT('Ctrl Pts',(46.0463696777801,-53.3373492770671,0.));
#61124=CARTESIAN_POINT('Ctrl Pts',(46.0637500926982,-53.3486113975901,0.));
#61125=CARTESIAN_POINT('Ctrl Pts',(46.0811849640218,-53.3598828428546,0.));
#61126=CARTESIAN_POINT('Ctrl Pts',(46.0986741925656,-53.3711634508437,0.));
#61127=CARTESIAN_POINT('Ctrl Pts',(46.1162176794884,-53.3824530603276,0.));
#61128=CARTESIAN_POINT('Ctrl Pts',(46.1338153268097,-53.3937515116549,0.));
#61129=CARTESIAN_POINT('Ctrl Pts',(46.1514670376012,-53.4050586470436,0.));
#61130=CARTESIAN_POINT('Ctrl Pts',(46.1691727157134,-53.4163743101517,0.));
#61131=CARTESIAN_POINT('Ctrl Pts',(46.1869322656023,-53.4276983458125,0.));
#61132=CARTESIAN_POINT('Ctrl Pts',(46.2047455921286,-53.4390305997274,0.));
#61133=CARTESIAN_POINT('Ctrl Pts',(46.2226126003202,-53.4503709181178,0.));
#61134=CARTESIAN_POINT('Ctrl Pts',(46.2405331953889,-53.4617191477402,0.));
#61135=CARTESIAN_POINT('Ctrl Pts',(46.2585072828353,-53.4730751360371,0.));
#61136=CARTESIAN_POINT('Ctrl Pts',(46.2765347685198,-53.4844387312414,0.));
#61137=CARTESIAN_POINT('Ctrl Pts',(46.2946155587417,-53.4958097825006,0.));
#61138=CARTESIAN_POINT('Ctrl Pts',(46.3127495603098,-53.5071881399911,0.));
#61139=CARTESIAN_POINT('Ctrl Pts',(46.3309366805093,-53.5185736548548,0.));
#61140=CARTESIAN_POINT('Ctrl Pts',(46.3491768270655,-53.5299661791385,0.));
#61141=CARTESIAN_POINT('Ctrl Pts',(46.3674699081046,-53.5413655657327,0.));
#61142=CARTESIAN_POINT('Ctrl Pts',(46.3858158321059,-53.5527716683048,0.));
#61143=CARTESIAN_POINT('Ctrl Pts',(46.4042145078701,-53.5641843412559,0.));
#61144=CARTESIAN_POINT('Ctrl Pts',(46.4226658445474,-53.5756034397481,0.));
#61145=CARTESIAN_POINT('Ctrl Pts',(46.4411697516478,-53.5870288197166,0.));
#61146=CARTESIAN_POINT('Ctrl Pts',(46.459726139052,-53.5984603378855,0.));
#61147=CARTESIAN_POINT('Ctrl Pts',(46.4783349170173,-53.6098978517859,0.));
#61148=CARTESIAN_POINT('Ctrl Pts',(46.496995996177,-53.6213412197533,0.));
#61149=CARTESIAN_POINT('Ctrl Pts',(46.5157092875373,-53.6327903009094,0.));
#61150=CARTESIAN_POINT('Ctrl Pts',(46.5344747024676,-53.6442449551455,0.));
#61151=CARTESIAN_POINT('Ctrl Pts',(46.5532921526901,-53.6557050431071,0.));
#61152=CARTESIAN_POINT('Ctrl Pts',(46.5721615502591,-53.6671704261737,0.));
#61153=CARTESIAN_POINT('Ctrl Pts',(46.5910828075653,-53.678640966456,0.));
#61154=CARTESIAN_POINT('Ctrl Pts',(46.6100558373402,-53.6901165267941,0.));
#61155=CARTESIAN_POINT('Ctrl Pts',(46.6290805526559,-53.701596970754,0.));
#61156=CARTESIAN_POINT('Ctrl Pts',(46.6481568669216,-53.7130821626263,0.));
#61157=CARTESIAN_POINT('Ctrl Pts',(46.6672846938752,-53.7245719674222,0.));
#61158=CARTESIAN_POINT('Ctrl Pts',(46.6864639475863,-53.7360662508677,0.));
#61159=CARTESIAN_POINT('Ctrl Pts',(46.7056945424559,-53.7475648793948,0.));
#61160=CARTESIAN_POINT('Ctrl Pts',(46.724976393213,-53.7590677201344,0.));
#61161=CARTESIAN_POINT('Ctrl Pts',(46.7443094149041,-53.770574640907,0.));
#61162=CARTESIAN_POINT('Ctrl Pts',(46.7636935228851,-53.782085510217,0.));
#61163=CARTESIAN_POINT('Ctrl Pts',(46.7831286328268,-53.7936001972468,0.));
#61164=CARTESIAN_POINT('Ctrl Pts',(46.8026146607144,-53.8051185718525,0.));
#61165=CARTESIAN_POINT('Ctrl Pts',(46.8221515228459,-53.8166405045582,0.));
#61166=CARTESIAN_POINT('Ctrl Pts',(46.8417391358231,-53.8281658665517,0.));
#61167=CARTESIAN_POINT('Ctrl Pts',(46.8613774165452,-53.8396945296777,0.));
#61168=CARTESIAN_POINT('Ctrl Pts',(46.8810662822146,-53.851226366434,0.));
#61169=CARTESIAN_POINT('Ctrl Pts',(46.900805650336,-53.8627612499648,0.));
#61170=CARTESIAN_POINT('Ctrl Pts',(46.9205954387128,-53.8742990540557,0.));
#61171=CARTESIAN_POINT('Ctrl Pts',(46.9404355654381,-53.8858396531277,0.));
#61172=CARTESIAN_POINT('Ctrl Pts',(46.9603259488894,-53.8973829222317,0.));
#61173=CARTESIAN_POINT('Ctrl Pts',(46.9802665077342,-53.9089287370436,0.));
#61174=CARTESIAN_POINT('Ctrl Pts',(47.0002571609286,-53.9204769738584,0.));
#61175=CARTESIAN_POINT('Ctrl Pts',(47.0202978277148,-53.9320275095864,0.));
#61176=CARTESIAN_POINT('Ctrl Pts',(47.04038842761,-53.9435802217468,0.));
#61177=CARTESIAN_POINT('Ctrl Pts',(47.0605288804042,-53.9551349884637,0.));
#61178=CARTESIAN_POINT('Ctrl Pts',(47.0807191061673,-53.9666916884624,0.));
#61179=CARTESIAN_POINT('Ctrl Pts',(47.1009590252466,-53.9782502010642,0.));
#61180=CARTESIAN_POINT('Ctrl Pts',(47.1212485582632,-53.9898104061809,0.));
#61181=CARTESIAN_POINT('Ctrl Pts',(47.1415876261012,-54.0013721843094,0.));
#61182=CARTESIAN_POINT('Ctrl Pts',(47.161976149906,-54.0129354165269,0.));
#61183=CARTESIAN_POINT('Ctrl Pts',(47.1824140510906,-54.0244999844872,0.));
#61184=CARTESIAN_POINT('Ctrl Pts',(47.2029012513334,-54.0360657704156,0.));
#61185=CARTESIAN_POINT('Ctrl Pts',(47.2234376725752,-54.047632657105,0.));
#61186=CARTESIAN_POINT('Ctrl Pts',(47.2440232370085,-54.0592005279108,0.));
#61187=CARTESIAN_POINT('Ctrl Pts',(47.2646578670767,-54.0707692667461,0.));
#61188=CARTESIAN_POINT('Ctrl Pts',(47.2853414854805,-54.082338758079,0.));
#61189=CARTESIAN_POINT('Ctrl Pts',(47.3060740151754,-54.0939088869271,0.));
#61190=CARTESIAN_POINT('Ctrl Pts',(47.326855379369,-54.1054795388538,0.));
#61191=CARTESIAN_POINT('Ctrl Pts',(47.3476855015095,-54.1170505999637,0.));
#61192=CARTESIAN_POINT('Ctrl Pts',(47.3685643052867,-54.1286219568981,0.));
#61193=CARTESIAN_POINT('Ctrl Pts',(47.3894917146361,-54.1401934968306,0.));
#61194=CARTESIAN_POINT('Ctrl Pts',(47.4104676537381,-54.1517651074638,0.));
#61195=CARTESIAN_POINT('Ctrl Pts',(47.4314920470142,-54.163336677024,0.));
#61196=CARTESIAN_POINT('Ctrl Pts',(47.4525648191173,-54.1749080942593,0.));
#61197=CARTESIAN_POINT('Ctrl Pts',(47.473685894932,-54.1864792484343,0.));
#61198=CARTESIAN_POINT('Ctrl Pts',(47.4948551995798,-54.1980500293267,0.));
#61199=CARTESIAN_POINT('Ctrl Pts',(47.5160726584172,-54.2096203272228,0.));
#61200=CARTESIAN_POINT('Ctrl Pts',(47.5373381970328,-54.2211900329141,0.));
#61201=CARTESIAN_POINT('Ctrl Pts',(47.5586517412368,-54.232759037693,0.));
#61202=CARTESIAN_POINT('Ctrl Pts',(47.5800132170614,-54.2443272333498,0.));
#61203=CARTESIAN_POINT('Ctrl Pts',(47.6014225507663,-54.2558945121684,0.));
#61204=CARTESIAN_POINT('Ctrl Pts',(47.6228796688376,-54.2674607669228,0.));
#61205=CARTESIAN_POINT('Ctrl Pts',(47.6443844979846,-54.2790258908736,0.));
#61206=CARTESIAN_POINT('Ctrl Pts',(47.6659369651299,-54.2905897777647,0.));
#61207=CARTESIAN_POINT('Ctrl Pts',(47.6875369974086,-54.3021523218188,0.));
#61208=CARTESIAN_POINT('Ctrl Pts',(47.7091845221747,-54.3137134177345,0.));
#61209=CARTESIAN_POINT('Ctrl Pts',(47.7308794669994,-54.3252729606824,0.));
#61210=CARTESIAN_POINT('Ctrl Pts',(47.7526217596694,-54.3368308463023,0.));
#61211=CARTESIAN_POINT('Ctrl Pts',(47.7744113281767,-54.3483869706998,0.));
#61212=CARTESIAN_POINT('Ctrl Pts',(47.7962481007179,-54.3599412304431,0.));
#61213=CARTESIAN_POINT('Ctrl Pts',(47.8181320056988,-54.3714935225585,0.));
#61214=CARTESIAN_POINT('Ctrl Pts',(47.8400629717352,-54.3830437445275,0.));
#61215=CARTESIAN_POINT('Ctrl Pts',(47.8620409276495,-54.3945917942835,0.));
#61216=CARTESIAN_POINT('Ctrl Pts',(47.8840658024626,-54.4061375702088,0.));
#61217=CARTESIAN_POINT('Ctrl Pts',(47.9061375253909,-54.4176809711324,0.));
#61218=CARTESIAN_POINT('Ctrl Pts',(47.9282560258528,-54.4292218963253,0.));
#61219=CARTESIAN_POINT('Ctrl Pts',(47.9504212334681,-54.4407602454974,0.));
#61220=CARTESIAN_POINT('Ctrl Pts',(47.972633078057,-54.4522959187952,0.));
#61221=CARTESIAN_POINT('Ctrl Pts',(47.9948914896316,-54.4638288167991,0.));
#61222=CARTESIAN_POINT('Ctrl Pts',(48.0171963983912,-54.4753588405202,0.));
#61223=CARTESIAN_POINT('Ctrl Pts',(48.039547734729,-54.4868858913961,0.));
#61224=CARTESIAN_POINT('Ctrl Pts',(48.0619454292321,-54.4984098712883,0.));
#61225=CARTESIAN_POINT('Ctrl Pts',(48.0843894126807,-54.5099306824788,0.));
#61226=CARTESIAN_POINT('Ctrl Pts',(48.1068796160406,-54.5214482276679,0.));
#61227=CARTESIAN_POINT('Ctrl Pts',(48.1294159704571,-54.5329624099719,0.));
#61228=CARTESIAN_POINT('Ctrl Pts',(48.1519984072617,-54.5444731329196,0.));
#61229=CARTESIAN_POINT('Ctrl Pts',(48.1746268579732,-54.5559803004487,0.));
#61230=CARTESIAN_POINT('Ctrl Pts',(48.1973012542966,-54.5674838169041,0.));
#61231=CARTESIAN_POINT('Ctrl Pts',(48.2200215281178,-54.5789835870348,0.));
#61232=CARTESIAN_POINT('Ctrl Pts',(48.2427876114955,-54.5904795159936,0.));
#61233=CARTESIAN_POINT('Ctrl Pts',(48.2655994366672,-54.6019715093319,0.));
#61234=CARTESIAN_POINT('Ctrl Pts',(48.288456936051,-54.6134594729964,0.));
#61235=CARTESIAN_POINT('Ctrl Pts',(48.3113600422443,-54.6249433133262,0.));
#61236=CARTESIAN_POINT('Ctrl Pts',(48.3343086880192,-54.636422937049,0.));
#61237=CARTESIAN_POINT('Ctrl Pts',(48.3573028063121,-54.647898251279,0.));
#61238=CARTESIAN_POINT('Ctrl Pts',(48.3803423302294,-54.6593691635143,0.));
#61239=CARTESIAN_POINT('Ctrl Pts',(48.4034271930516,-54.6708355816359,0.));
#61240=CARTESIAN_POINT('Ctrl Pts',(48.4265573282341,-54.6822974139065,0.));
#61241=CARTESIAN_POINT('Ctrl Pts',(48.4497326694051,-54.6937545689694,0.));
#61242=CARTESIAN_POINT('Ctrl Pts',(48.4729531503565,-54.7052069558493,0.));
#61243=CARTESIAN_POINT('Ctrl Pts',(48.4962187050451,-54.7166544839475,0.));
#61244=CARTESIAN_POINT('Ctrl Pts',(48.5195292675955,-54.7280970630346,0.));
#61245=CARTESIAN_POINT('Ctrl Pts',(48.5428847722974,-54.7395346032451,0.));
#61246=CARTESIAN_POINT('Ctrl Pts',(48.5662851536027,-54.7509670150716,0.));
#61247=CARTESIAN_POINT('Ctrl Pts',(48.5897303461131,-54.7623942093591,0.));
#61248=CARTESIAN_POINT('Ctrl Pts',(48.6132202845792,-54.773816097304,0.));
#61249=CARTESIAN_POINT('Ctrl Pts',(48.6367549039121,-54.7852325904591,0.));
#61250=CARTESIAN_POINT('Ctrl Pts',(48.6603341391891,-54.7966436007395,0.));
#61251=CARTESIAN_POINT('Ctrl Pts',(48.6839579256565,-54.8080490404274,0.));
#61252=CARTESIAN_POINT('Ctrl Pts',(48.7076261987284,-54.8194488221803,0.));
#61253=CARTESIAN_POINT('Ctrl Pts',(48.7313388939834,-54.8308428590334,0.));
#61254=CARTESIAN_POINT('Ctrl Pts',(48.755095947159,-54.8422310643752,0.));
#61255=CARTESIAN_POINT('Ctrl Pts',(48.7788972941431,-54.8536133519285,0.));
#61256=CARTESIAN_POINT('Ctrl Pts',(48.8027428709613,-54.8649896357284,0.));
#61257=CARTESIAN_POINT('Ctrl Pts',(48.8266326137629,-54.8763598301045,0.));
#61258=CARTESIAN_POINT('Ctrl Pts',(48.8505664587984,-54.8877238496577,0.));
#61259=CARTESIAN_POINT('Ctrl Pts',(48.8745443424488,-54.8990816092964,0.));
#61260=CARTESIAN_POINT('Ctrl Pts',(48.8985662012535,-54.910433024275,0.));
#61261=CARTESIAN_POINT('Ctrl Pts',(48.922631971937,-54.9217780102357,0.));
#61262=CARTESIAN_POINT('Ctrl Pts',(48.9467415914266,-54.933116483242,0.));
#61263=CARTESIAN_POINT('Ctrl Pts',(48.9708949968789,-54.9444483598372,0.));
#61264=CARTESIAN_POINT('Ctrl Pts',(48.995092125652,-54.9557735569936,0.));
#61265=CARTESIAN_POINT('Ctrl Pts',(49.0193329152475,-54.9670919920024,0.));
#61266=CARTESIAN_POINT('Ctrl Pts',(49.0436173032527,-54.9784035823764,0.));
#61267=CARTESIAN_POINT('Ctrl Pts',(49.0679452272871,-54.9897082457607,0.));
#61268=CARTESIAN_POINT('Ctrl Pts',(49.0923166249222,-55.0010058998111,0.));
#61269=CARTESIAN_POINT('Ctrl Pts',(49.1167314336737,-55.0122964621868,0.));
#61270=CARTESIAN_POINT('Ctrl Pts',(49.1411895911645,-55.0235798508056,0.));
#61271=CARTESIAN_POINT('Ctrl Pts',(49.1656910352484,-55.0348559840462,0.));
#61272=CARTESIAN_POINT('Ctrl Pts',(49.1902357041462,-55.0461247809745,0.));
#61273=CARTESIAN_POINT('Ctrl Pts',(49.2148235365694,-55.0573861615569,0.));
#61274=CARTESIAN_POINT('Ctrl Pts',(49.2394544718512,-55.0686400468911,0.));
#61275=CARTESIAN_POINT('Ctrl Pts',(49.2641284496496,-55.0798863586986,0.));
#61276=CARTESIAN_POINT('Ctrl Pts',(49.2888454096544,-55.0911250188282,0.));
#61277=CARTESIAN_POINT('Ctrl Pts',(49.3136052912614,-55.1023559487133,0.));
#61278=CARTESIAN_POINT('Ctrl Pts',(49.3384080333166,-55.1135790689475,0.));
#61279=CARTESIAN_POINT('Ctrl Pts',(49.3632535736744,-55.1247942985649,0.));
#61280=CARTESIAN_POINT('Ctrl Pts',(49.3881418495529,-55.1360015556262,0.));
#61281=CARTESIAN_POINT('Ctrl Pts',(49.413072798324,-55.1472007585224,0.));
#61282=CARTESIAN_POINT('Ctrl Pts',(49.4380463581989,-55.158391827114,0.));
#61283=CARTESIAN_POINT('Ctrl Pts',(49.4630624688787,-55.1695746838168,0.));
#61284=CARTESIAN_POINT('Ctrl Pts',(49.4881210723921,-55.1807492550073,0.));
#61285=CARTESIAN_POINT('Ctrl Pts',(49.5132221132916,-55.1919154713569,0.));
#61286=CARTESIAN_POINT('Ctrl Pts',(49.5347748994608,-55.2014798623976,0.));
#61287=CARTESIAN_POINT('Ctrl Pts',(49.5513218524282,-55.2088081098956,0.));
#61288=CARTESIAN_POINT('Ctrl Pts',(49.5628442141874,-55.2139039604571,0.));
#61289=CARTESIAN_POINT('Ctrl Pts',(49.5693295981614,-55.216769915117,0.));
#61290=CARTESIAN_POINT('Ctrl Pts',(49.5707719660262,-55.21740720013,0.));
#61291=CARTESIAN_POINT('',(45.6458539113724,-53.0702932034641,12.));
#61292=CARTESIAN_POINT('',(45.6458539113724,-53.0702932034641,0.));
#61293=CARTESIAN_POINT('Ctrl Pts',(49.5707719660262,-55.21740720013,12.));
#61294=CARTESIAN_POINT('Ctrl Pts',(49.5693295981614,-55.216769915117,12.));
#61295=CARTESIAN_POINT('Ctrl Pts',(49.5628442141874,-55.2139039604571,12.));
#61296=CARTESIAN_POINT('Ctrl Pts',(49.5513218524282,-55.2088081098956,12.));
#61297=CARTESIAN_POINT('Ctrl Pts',(49.5347748994608,-55.2014798623976,12.));
#61298=CARTESIAN_POINT('Ctrl Pts',(49.5132221132916,-55.1919154713569,12.));
#61299=CARTESIAN_POINT('Ctrl Pts',(49.4881210723921,-55.1807492550073,12.));
#61300=CARTESIAN_POINT('Ctrl Pts',(49.4630624688787,-55.1695746838168,12.));
#61301=CARTESIAN_POINT('Ctrl Pts',(49.4380463581989,-55.158391827114,12.));
#61302=CARTESIAN_POINT('Ctrl Pts',(49.413072798324,-55.1472007585224,12.));
#61303=CARTESIAN_POINT('Ctrl Pts',(49.3881418495529,-55.1360015556262,12.));
#61304=CARTESIAN_POINT('Ctrl Pts',(49.3632535736744,-55.1247942985649,12.));
#61305=CARTESIAN_POINT('Ctrl Pts',(49.3384080333166,-55.1135790689475,12.));
#61306=CARTESIAN_POINT('Ctrl Pts',(49.3136052912614,-55.1023559487133,12.));
#61307=CARTESIAN_POINT('Ctrl Pts',(49.2888454096544,-55.0911250188282,12.));
#61308=CARTESIAN_POINT('Ctrl Pts',(49.2641284496496,-55.0798863586986,12.));
#61309=CARTESIAN_POINT('Ctrl Pts',(49.2394544718512,-55.0686400468911,12.));
#61310=CARTESIAN_POINT('Ctrl Pts',(49.2148235365694,-55.0573861615569,12.));
#61311=CARTESIAN_POINT('Ctrl Pts',(49.1902357041462,-55.0461247809745,12.));
#61312=CARTESIAN_POINT('Ctrl Pts',(49.1656910352484,-55.0348559840462,12.));
#61313=CARTESIAN_POINT('Ctrl Pts',(49.1411895911645,-55.0235798508056,12.));
#61314=CARTESIAN_POINT('Ctrl Pts',(49.1167314336737,-55.0122964621868,12.));
#61315=CARTESIAN_POINT('Ctrl Pts',(49.0923166249222,-55.0010058998111,12.));
#61316=CARTESIAN_POINT('Ctrl Pts',(49.0679452272871,-54.9897082457607,12.));
#61317=CARTESIAN_POINT('Ctrl Pts',(49.0436173032527,-54.9784035823764,12.));
#61318=CARTESIAN_POINT('Ctrl Pts',(49.0193329152475,-54.9670919920024,12.));
#61319=CARTESIAN_POINT('Ctrl Pts',(48.995092125652,-54.9557735569936,12.));
#61320=CARTESIAN_POINT('Ctrl Pts',(48.9708949968789,-54.9444483598372,12.));
#61321=CARTESIAN_POINT('Ctrl Pts',(48.9467415914266,-54.933116483242,12.));
#61322=CARTESIAN_POINT('Ctrl Pts',(48.922631971937,-54.9217780102357,12.));
#61323=CARTESIAN_POINT('Ctrl Pts',(48.8985662012535,-54.910433024275,12.));
#61324=CARTESIAN_POINT('Ctrl Pts',(48.8745443424488,-54.8990816092964,12.));
#61325=CARTESIAN_POINT('Ctrl Pts',(48.8505664587984,-54.8877238496577,12.));
#61326=CARTESIAN_POINT('Ctrl Pts',(48.8266326137629,-54.8763598301045,12.));
#61327=CARTESIAN_POINT('Ctrl Pts',(48.8027428709613,-54.8649896357284,12.));
#61328=CARTESIAN_POINT('Ctrl Pts',(48.7788972941431,-54.8536133519285,12.));
#61329=CARTESIAN_POINT('Ctrl Pts',(48.755095947159,-54.8422310643752,12.));
#61330=CARTESIAN_POINT('Ctrl Pts',(48.7313388939834,-54.8308428590334,12.));
#61331=CARTESIAN_POINT('Ctrl Pts',(48.7076261987284,-54.8194488221803,12.));
#61332=CARTESIAN_POINT('Ctrl Pts',(48.6839579256565,-54.8080490404274,12.));
#61333=CARTESIAN_POINT('Ctrl Pts',(48.6603341391891,-54.7966436007395,12.));
#61334=CARTESIAN_POINT('Ctrl Pts',(48.6367549039121,-54.7852325904591,12.));
#61335=CARTESIAN_POINT('Ctrl Pts',(48.6132202845792,-54.773816097304,12.));
#61336=CARTESIAN_POINT('Ctrl Pts',(48.5897303461131,-54.7623942093591,12.));
#61337=CARTESIAN_POINT('Ctrl Pts',(48.5662851536027,-54.7509670150716,12.));
#61338=CARTESIAN_POINT('Ctrl Pts',(48.5428847722974,-54.7395346032451,12.));
#61339=CARTESIAN_POINT('Ctrl Pts',(48.5195292675955,-54.7280970630346,12.));
#61340=CARTESIAN_POINT('Ctrl Pts',(48.4962187050451,-54.7166544839475,12.));
#61341=CARTESIAN_POINT('Ctrl Pts',(48.4729531503565,-54.7052069558493,12.));
#61342=CARTESIAN_POINT('Ctrl Pts',(48.4497326694051,-54.6937545689694,12.));
#61343=CARTESIAN_POINT('Ctrl Pts',(48.4265573282341,-54.6822974139065,12.));
#61344=CARTESIAN_POINT('Ctrl Pts',(48.4034271930516,-54.6708355816359,12.));
#61345=CARTESIAN_POINT('Ctrl Pts',(48.3803423302294,-54.6593691635143,12.));
#61346=CARTESIAN_POINT('Ctrl Pts',(48.3573028063121,-54.647898251279,12.));
#61347=CARTESIAN_POINT('Ctrl Pts',(48.3343086880192,-54.636422937049,12.));
#61348=CARTESIAN_POINT('Ctrl Pts',(48.3113600422443,-54.6249433133262,12.));
#61349=CARTESIAN_POINT('Ctrl Pts',(48.288456936051,-54.6134594729964,12.));
#61350=CARTESIAN_POINT('Ctrl Pts',(48.2655994366672,-54.6019715093319,12.));
#61351=CARTESIAN_POINT('Ctrl Pts',(48.2427876114955,-54.5904795159936,12.));
#61352=CARTESIAN_POINT('Ctrl Pts',(48.2200215281178,-54.5789835870348,12.));
#61353=CARTESIAN_POINT('Ctrl Pts',(48.1973012542966,-54.5674838169041,12.));
#61354=CARTESIAN_POINT('Ctrl Pts',(48.1746268579732,-54.5559803004487,12.));
#61355=CARTESIAN_POINT('Ctrl Pts',(48.1519984072617,-54.5444731329196,12.));
#61356=CARTESIAN_POINT('Ctrl Pts',(48.1294159704571,-54.5329624099719,12.));
#61357=CARTESIAN_POINT('Ctrl Pts',(48.1068796160406,-54.5214482276679,12.));
#61358=CARTESIAN_POINT('Ctrl Pts',(48.0843894126807,-54.5099306824788,12.));
#61359=CARTESIAN_POINT('Ctrl Pts',(48.0619454292321,-54.4984098712883,12.));
#61360=CARTESIAN_POINT('Ctrl Pts',(48.039547734729,-54.4868858913961,12.));
#61361=CARTESIAN_POINT('Ctrl Pts',(48.0171963983912,-54.4753588405202,12.));
#61362=CARTESIAN_POINT('Ctrl Pts',(47.9948914896316,-54.4638288167991,12.));
#61363=CARTESIAN_POINT('Ctrl Pts',(47.972633078057,-54.4522959187952,12.));
#61364=CARTESIAN_POINT('Ctrl Pts',(47.9504212334681,-54.4407602454974,12.));
#61365=CARTESIAN_POINT('Ctrl Pts',(47.9282560258528,-54.4292218963253,12.));
#61366=CARTESIAN_POINT('Ctrl Pts',(47.9061375253909,-54.4176809711324,12.));
#61367=CARTESIAN_POINT('Ctrl Pts',(47.8840658024626,-54.4061375702088,12.));
#61368=CARTESIAN_POINT('Ctrl Pts',(47.8620409276495,-54.3945917942835,12.));
#61369=CARTESIAN_POINT('Ctrl Pts',(47.8400629717352,-54.3830437445275,12.));
#61370=CARTESIAN_POINT('Ctrl Pts',(47.8181320056988,-54.3714935225585,12.));
#61371=CARTESIAN_POINT('Ctrl Pts',(47.7962481007179,-54.3599412304431,12.));
#61372=CARTESIAN_POINT('Ctrl Pts',(47.7744113281767,-54.3483869706998,12.));
#61373=CARTESIAN_POINT('Ctrl Pts',(47.7526217596694,-54.3368308463023,12.));
#61374=CARTESIAN_POINT('Ctrl Pts',(47.7308794669994,-54.3252729606824,12.));
#61375=CARTESIAN_POINT('Ctrl Pts',(47.7091845221747,-54.3137134177345,12.));
#61376=CARTESIAN_POINT('Ctrl Pts',(47.6875369974086,-54.3021523218188,12.));
#61377=CARTESIAN_POINT('Ctrl Pts',(47.6659369651299,-54.2905897777647,12.));
#61378=CARTESIAN_POINT('Ctrl Pts',(47.6443844979846,-54.2790258908736,12.));
#61379=CARTESIAN_POINT('Ctrl Pts',(47.6228796688376,-54.2674607669228,12.));
#61380=CARTESIAN_POINT('Ctrl Pts',(47.6014225507663,-54.2558945121684,12.));
#61381=CARTESIAN_POINT('Ctrl Pts',(47.5800132170614,-54.2443272333498,12.));
#61382=CARTESIAN_POINT('Ctrl Pts',(47.5586517412368,-54.232759037693,12.));
#61383=CARTESIAN_POINT('Ctrl Pts',(47.5373381970328,-54.2211900329141,12.));
#61384=CARTESIAN_POINT('Ctrl Pts',(47.5160726584172,-54.2096203272228,12.));
#61385=CARTESIAN_POINT('Ctrl Pts',(47.4948551995798,-54.1980500293267,12.));
#61386=CARTESIAN_POINT('Ctrl Pts',(47.473685894932,-54.1864792484343,12.));
#61387=CARTESIAN_POINT('Ctrl Pts',(47.4525648191173,-54.1749080942593,12.));
#61388=CARTESIAN_POINT('Ctrl Pts',(47.4314920470142,-54.163336677024,12.));
#61389=CARTESIAN_POINT('Ctrl Pts',(47.4104676537381,-54.1517651074638,12.));
#61390=CARTESIAN_POINT('Ctrl Pts',(47.3894917146361,-54.1401934968306,12.));
#61391=CARTESIAN_POINT('Ctrl Pts',(47.3685643052867,-54.1286219568981,12.));
#61392=CARTESIAN_POINT('Ctrl Pts',(47.3476855015095,-54.1170505999637,12.));
#61393=CARTESIAN_POINT('Ctrl Pts',(47.326855379369,-54.1054795388538,12.));
#61394=CARTESIAN_POINT('Ctrl Pts',(47.3060740151754,-54.0939088869271,12.));
#61395=CARTESIAN_POINT('Ctrl Pts',(47.2853414854805,-54.082338758079,12.));
#61396=CARTESIAN_POINT('Ctrl Pts',(47.2646578670767,-54.0707692667461,12.));
#61397=CARTESIAN_POINT('Ctrl Pts',(47.2440232370085,-54.0592005279108,12.));
#61398=CARTESIAN_POINT('Ctrl Pts',(47.2234376725752,-54.047632657105,12.));
#61399=CARTESIAN_POINT('Ctrl Pts',(47.2029012513334,-54.0360657704156,12.));
#61400=CARTESIAN_POINT('Ctrl Pts',(47.1824140510906,-54.0244999844872,12.));
#61401=CARTESIAN_POINT('Ctrl Pts',(47.161976149906,-54.0129354165269,12.));
#61402=CARTESIAN_POINT('Ctrl Pts',(47.1415876261012,-54.0013721843094,12.));
#61403=CARTESIAN_POINT('Ctrl Pts',(47.1212485582632,-53.9898104061809,12.));
#61404=CARTESIAN_POINT('Ctrl Pts',(47.1009590252466,-53.9782502010642,12.));
#61405=CARTESIAN_POINT('Ctrl Pts',(47.0807191061673,-53.9666916884624,12.));
#61406=CARTESIAN_POINT('Ctrl Pts',(47.0605288804042,-53.9551349884637,12.));
#61407=CARTESIAN_POINT('Ctrl Pts',(47.04038842761,-53.9435802217468,12.));
#61408=CARTESIAN_POINT('Ctrl Pts',(47.0202978277148,-53.9320275095864,12.));
#61409=CARTESIAN_POINT('Ctrl Pts',(47.0002571609286,-53.9204769738584,12.));
#61410=CARTESIAN_POINT('Ctrl Pts',(46.9802665077342,-53.9089287370436,12.));
#61411=CARTESIAN_POINT('Ctrl Pts',(46.9603259488894,-53.8973829222317,12.));
#61412=CARTESIAN_POINT('Ctrl Pts',(46.9404355654381,-53.8858396531277,12.));
#61413=CARTESIAN_POINT('Ctrl Pts',(46.9205954387128,-53.8742990540557,12.));
#61414=CARTESIAN_POINT('Ctrl Pts',(46.900805650336,-53.8627612499648,12.));
#61415=CARTESIAN_POINT('Ctrl Pts',(46.8810662822146,-53.851226366434,12.));
#61416=CARTESIAN_POINT('Ctrl Pts',(46.8613774165452,-53.8396945296777,12.));
#61417=CARTESIAN_POINT('Ctrl Pts',(46.8417391358231,-53.8281658665517,12.));
#61418=CARTESIAN_POINT('Ctrl Pts',(46.8221515228459,-53.8166405045582,12.));
#61419=CARTESIAN_POINT('Ctrl Pts',(46.8026146607144,-53.8051185718525,12.));
#61420=CARTESIAN_POINT('Ctrl Pts',(46.7831286328268,-53.7936001972468,12.));
#61421=CARTESIAN_POINT('Ctrl Pts',(46.7636935228851,-53.782085510217,12.));
#61422=CARTESIAN_POINT('Ctrl Pts',(46.7443094149041,-53.770574640907,12.));
#61423=CARTESIAN_POINT('Ctrl Pts',(46.724976393213,-53.7590677201344,12.));
#61424=CARTESIAN_POINT('Ctrl Pts',(46.7056945424559,-53.7475648793948,12.));
#61425=CARTESIAN_POINT('Ctrl Pts',(46.6864639475863,-53.7360662508677,12.));
#61426=CARTESIAN_POINT('Ctrl Pts',(46.6672846938752,-53.7245719674222,12.));
#61427=CARTESIAN_POINT('Ctrl Pts',(46.6481568669216,-53.7130821626263,12.));
#61428=CARTESIAN_POINT('Ctrl Pts',(46.6290805526559,-53.701596970754,12.));
#61429=CARTESIAN_POINT('Ctrl Pts',(46.6100558373402,-53.6901165267941,12.));
#61430=CARTESIAN_POINT('Ctrl Pts',(46.5910828075653,-53.678640966456,12.));
#61431=CARTESIAN_POINT('Ctrl Pts',(46.5721615502591,-53.6671704261737,12.));
#61432=CARTESIAN_POINT('Ctrl Pts',(46.5532921526901,-53.6557050431071,12.));
#61433=CARTESIAN_POINT('Ctrl Pts',(46.5344747024676,-53.6442449551455,12.));
#61434=CARTESIAN_POINT('Ctrl Pts',(46.5157092875373,-53.6327903009094,12.));
#61435=CARTESIAN_POINT('Ctrl Pts',(46.496995996177,-53.6213412197533,12.));
#61436=CARTESIAN_POINT('Ctrl Pts',(46.4783349170173,-53.6098978517859,12.));
#61437=CARTESIAN_POINT('Ctrl Pts',(46.459726139052,-53.5984603378855,12.));
#61438=CARTESIAN_POINT('Ctrl Pts',(46.4411697516478,-53.5870288197166,12.));
#61439=CARTESIAN_POINT('Ctrl Pts',(46.4226658445474,-53.5756034397481,12.));
#61440=CARTESIAN_POINT('Ctrl Pts',(46.4042145078701,-53.5641843412559,12.));
#61441=CARTESIAN_POINT('Ctrl Pts',(46.3858158321059,-53.5527716683048,12.));
#61442=CARTESIAN_POINT('Ctrl Pts',(46.3674699081046,-53.5413655657327,12.));
#61443=CARTESIAN_POINT('Ctrl Pts',(46.3491768270655,-53.5299661791385,12.));
#61444=CARTESIAN_POINT('Ctrl Pts',(46.3309366805093,-53.5185736548548,12.));
#61445=CARTESIAN_POINT('Ctrl Pts',(46.3127495603098,-53.5071881399911,12.));
#61446=CARTESIAN_POINT('Ctrl Pts',(46.2946155587417,-53.4958097825006,12.));
#61447=CARTESIAN_POINT('Ctrl Pts',(46.2765347685198,-53.4844387312414,12.));
#61448=CARTESIAN_POINT('Ctrl Pts',(46.2585072828353,-53.4730751360371,12.));
#61449=CARTESIAN_POINT('Ctrl Pts',(46.2405331953889,-53.4617191477402,12.));
#61450=CARTESIAN_POINT('Ctrl Pts',(46.2226126003202,-53.4503709181178,12.));
#61451=CARTESIAN_POINT('Ctrl Pts',(46.2047455921286,-53.4390305997274,12.));
#61452=CARTESIAN_POINT('Ctrl Pts',(46.1869322656023,-53.4276983458125,12.));
#61453=CARTESIAN_POINT('Ctrl Pts',(46.1691727157134,-53.4163743101517,12.));
#61454=CARTESIAN_POINT('Ctrl Pts',(46.1514670376012,-53.4050586470436,12.));
#61455=CARTESIAN_POINT('Ctrl Pts',(46.1338153268097,-53.3937515116549,12.));
#61456=CARTESIAN_POINT('Ctrl Pts',(46.1162176794884,-53.3824530603276,12.));
#61457=CARTESIAN_POINT('Ctrl Pts',(46.0986741925656,-53.3711634508437,12.));
#61458=CARTESIAN_POINT('Ctrl Pts',(46.0811849640218,-53.3598828428546,12.));
#61459=CARTESIAN_POINT('Ctrl Pts',(46.0637500926982,-53.3486113975901,12.));
#61460=CARTESIAN_POINT('Ctrl Pts',(46.0463696777801,-53.3373492770671,12.));
#61461=CARTESIAN_POINT('Ctrl Pts',(46.02904381836,-53.326096643428,12.));
#61462=CARTESIAN_POINT('Ctrl Pts',(46.0117726129873,-53.3148536582635,12.));
#61463=CARTESIAN_POINT('Ctrl Pts',(45.9945561591453,-53.3036204818329,12.));
#61464=CARTESIAN_POINT('Ctrl Pts',(45.9773945542384,-53.292397274555,12.));
#61465=CARTESIAN_POINT('Ctrl Pts',(45.9602878967698,-53.2811841987926,12.));
#61466=CARTESIAN_POINT('Ctrl Pts',(45.9432362873008,-53.2699814203105,12.));
#61467=CARTESIAN_POINT('Ctrl Pts',(45.9262398298349,-53.2587891103866,12.));
#61468=CARTESIAN_POINT('Ctrl Pts',(45.9092986319377,-53.2476074460017,12.));
#61469=CARTESIAN_POINT('Ctrl Pts',(45.8924128018379,-53.2364366054306,12.));
#61470=CARTESIAN_POINT('Ctrl Pts',(45.8755824458722,-53.2252767643662,12.));
#61471=CARTESIAN_POINT('Ctrl Pts',(45.8588076662582,-53.2141280925439,12.));
#61472=CARTESIAN_POINT('Ctrl Pts',(45.8420885575349,-53.2029907483557,12.));
#61473=CARTESIAN_POINT('Ctrl Pts',(45.8254252099957,-53.1918648840541,12.));
#61474=CARTESIAN_POINT('Ctrl Pts',(45.8088177165089,-53.1807506560933,12.));
#61475=CARTESIAN_POINT('Ctrl Pts',(45.7922661780005,-53.1696482334487,12.));
#61476=CARTESIAN_POINT('Ctrl Pts',(45.7757707100618,-53.1585578076444,12.));
#61477=CARTESIAN_POINT('Ctrl Pts',(45.7593314474501,-53.1474795996053,12.));
#61478=CARTESIAN_POINT('Ctrl Pts',(45.7429485300823,-53.1364138384693,12.));
#61479=CARTESIAN_POINT('Ctrl Pts',(45.7266220897003,-53.1253607414872,12.));
#61480=CARTESIAN_POINT('Ctrl Pts',(45.7103522376696,-53.114320495492,12.));
#61481=CARTESIAN_POINT('Ctrl Pts',(45.694139048907,-53.1032932328857,12.));
#61482=CARTESIAN_POINT('Ctrl Pts',(45.6779825614231,-53.0922790298409,12.));
#61483=CARTESIAN_POINT('Ctrl Pts',(45.6651027439241,-53.0834781451546,12.));
#61484=CARTESIAN_POINT('Ctrl Pts',(45.6554684028145,-53.0768833804193,12.));
#61485=CARTESIAN_POINT('Ctrl Pts',(45.6490568514089,-53.0724894921849,12.));
#61486=CARTESIAN_POINT('Ctrl Pts',(45.6458539113724,-53.0702932034641,12.));
#61487=CARTESIAN_POINT('Ctrl Pts',(50.6869108458849,-54.1946543500368,0.));
#61488=CARTESIAN_POINT('Ctrl Pts',(50.6869108458849,-54.1946543500368,4.));
#61489=CARTESIAN_POINT('Ctrl Pts',(50.6869108458849,-54.1946543500368,8.));
#61490=CARTESIAN_POINT('Ctrl Pts',(50.6869108458849,-54.1946543500368,12.));
#61491=CARTESIAN_POINT('Ctrl Pts',(50.722390087302,-54.2986513683562,0.));
#61492=CARTESIAN_POINT('Ctrl Pts',(50.722390087302,-54.2986513683562,4.));
#61493=CARTESIAN_POINT('Ctrl Pts',(50.722390087302,-54.2986513683562,8.));
#61494=CARTESIAN_POINT('Ctrl Pts',(50.722390087302,-54.2986513683562,12.));
#61495=CARTESIAN_POINT('Ctrl Pts',(50.7219766588193,-54.501314566926,0.));
#61496=CARTESIAN_POINT('Ctrl Pts',(50.7219766588193,-54.501314566926,4.));
#61497=CARTESIAN_POINT('Ctrl Pts',(50.7219766588193,-54.5013145669259,7.99999999999999));
#61498=CARTESIAN_POINT('Ctrl Pts',(50.7219766588193,-54.5013145669259,12.));
#61499=CARTESIAN_POINT('Ctrl Pts',(50.6135081477654,-54.6674453828693,0.));
#61500=CARTESIAN_POINT('Ctrl Pts',(50.6135081477654,-54.6674453828693,4.));
#61501=CARTESIAN_POINT('Ctrl Pts',(50.6135081477654,-54.6674453828692,8.00000000000001));
#61502=CARTESIAN_POINT('Ctrl Pts',(50.6135081477654,-54.6674453828692,12.));
#61503=CARTESIAN_POINT('Ctrl Pts',(50.5529731960897,-54.7233670476825,0.));
#61504=CARTESIAN_POINT('Ctrl Pts',(50.5529731960897,-54.7233670476825,4.));
#61505=CARTESIAN_POINT('Ctrl Pts',(50.5529731960896,-54.7233670476824,8.));
#61506=CARTESIAN_POINT('Ctrl Pts',(50.5529731960896,-54.7233670476824,12.));
#61507=CARTESIAN_POINT('',(50.6869108458849,-54.1946543500368,0.));
#61508=CARTESIAN_POINT('',(50.5529731960899,-54.7233670476828,0.));
#61509=CARTESIAN_POINT('Ctrl Pts',(50.6869108458849,-54.1946543500368,7.52391395153922E-35));
#61510=CARTESIAN_POINT('Ctrl Pts',(50.722390087302,-54.2986513683562,7.52391395153921E-35));
#61511=CARTESIAN_POINT('Ctrl Pts',(50.7221538424548,-54.4144589103961,7.52391395153922E-35));
#61512=CARTESIAN_POINT('Ctrl Pts',(50.6866343053394,-54.5183375111702,7.52391395153922E-35));
#61513=CARTESIAN_POINT('Ctrl Pts',(50.6599946525028,-54.5962464617507,7.52391395153922E-35));
#61514=CARTESIAN_POINT('Ctrl Pts',(50.6135081477654,-54.6674453828693,7.52391395153921E-35));
#61515=CARTESIAN_POINT('Ctrl Pts',(50.5529731960897,-54.7233670476825,7.52391395153922E-35));
#61516=CARTESIAN_POINT('',(50.55297319609,-54.7233670476827,12.));
#61517=CARTESIAN_POINT('Ctrl Pts',(50.5529731960897,-54.7233670476825,0.));
#61518=CARTESIAN_POINT('Ctrl Pts',(50.5529731960897,-54.7233670476825,4.));
#61519=CARTESIAN_POINT('Ctrl Pts',(50.5529731960896,-54.7233670476824,8.));
#61520=CARTESIAN_POINT('Ctrl Pts',(50.5529731960896,-54.7233670476824,12.));
#61521=CARTESIAN_POINT('',(50.6869108458849,-54.1946543500368,12.));
#61522=CARTESIAN_POINT('Ctrl Pts',(50.5529731960896,-54.7233670476824,12.));
#61523=CARTESIAN_POINT('Ctrl Pts',(50.6135081477654,-54.6674453828692,12.));
#61524=CARTESIAN_POINT('Ctrl Pts',(50.6599946525028,-54.5962464617507,12.));
#61525=CARTESIAN_POINT('Ctrl Pts',(50.6866343053393,-54.5183375111701,12.));
#61526=CARTESIAN_POINT('Ctrl Pts',(50.7221538424547,-54.414458910396,12.));
#61527=CARTESIAN_POINT('Ctrl Pts',(50.722390087302,-54.2986513683562,12.));
#61528=CARTESIAN_POINT('Ctrl Pts',(50.6869108458849,-54.1946543500368,12.));
#61529=CARTESIAN_POINT('Ctrl Pts',(50.6869108458849,-54.1946543500368,12.));
#61530=CARTESIAN_POINT('Ctrl Pts',(50.6869108458849,-54.1946543500368,8.));
#61531=CARTESIAN_POINT('Ctrl Pts',(50.6869108458849,-54.1946543500368,4.));
#61532=CARTESIAN_POINT('Ctrl Pts',(50.6869108458849,-54.1946543500368,0.));
#61533=CARTESIAN_POINT('Origin',(2.53313958019842E-10,-2.7629675461203E-10,
0.));
#61534=CARTESIAN_POINT('Origin',(2.53313958019842E-10,-2.7629675461203E-10,
12.));
#61535=CARTESIAN_POINT('Origin',(2.53313958019842E-10,-2.7629675461203E-10,
0.));
#61536=CARTESIAN_POINT('Ctrl Pts',(45.1135644683471,-59.2875729049545,0.));
#61537=CARTESIAN_POINT('Ctrl Pts',(45.1135644683471,-59.2875729049545,4.));
#61538=CARTESIAN_POINT('Ctrl Pts',(45.1135644683471,-59.2875729049545,8.));
#61539=CARTESIAN_POINT('Ctrl Pts',(45.1135644683471,-59.2875729049545,12.));
#61540=CARTESIAN_POINT('Ctrl Pts',(45.0261193041895,-59.3541123643618,0.));
#61541=CARTESIAN_POINT('Ctrl Pts',(45.0261193041895,-59.3541123643618,4.));
#61542=CARTESIAN_POINT('Ctrl Pts',(45.0261193041895,-59.3541123643618,8.));
#61543=CARTESIAN_POINT('Ctrl Pts',(45.0261193041895,-59.3541123643618,12.));
#61544=CARTESIAN_POINT('Ctrl Pts',(44.8337211159575,-59.4177951463802,0.));
#61545=CARTESIAN_POINT('Ctrl Pts',(44.8337211159575,-59.4177951463802,4.00000000000001));
#61546=CARTESIAN_POINT('Ctrl Pts',(44.8337211159575,-59.4177951463802,8.));
#61547=CARTESIAN_POINT('Ctrl Pts',(44.8337211159575,-59.4177951463802,12.));
#61548=CARTESIAN_POINT('Ctrl Pts',(44.6418181989799,-59.3674150879748,0.));
#61549=CARTESIAN_POINT('Ctrl Pts',(44.6418181989799,-59.3674150879748,4.));
#61550=CARTESIAN_POINT('Ctrl Pts',(44.6418181989798,-59.3674150879747,8.00000000000001));
#61551=CARTESIAN_POINT('Ctrl Pts',(44.6418181989798,-59.3674150879747,12.));
#61552=CARTESIAN_POINT('Ctrl Pts',(44.5696260757423,-59.3276657444157,0.));
#61553=CARTESIAN_POINT('Ctrl Pts',(44.5696260757423,-59.3276657444157,4.));
#61554=CARTESIAN_POINT('Ctrl Pts',(44.5696260757423,-59.3276657444157,8.));
#61555=CARTESIAN_POINT('Ctrl Pts',(44.5696260757423,-59.3276657444157,12.));
#61556=CARTESIAN_POINT('',(45.1135644683471,-59.2875729049545,0.));
#61557=CARTESIAN_POINT('',(44.5696260757422,-59.3276657444159,0.));
#61558=CARTESIAN_POINT('Ctrl Pts',(45.1135644683471,-59.2875729049545,0.));
#61559=CARTESIAN_POINT('Ctrl Pts',(45.0261193041895,-59.3541123643618,0.));
#61560=CARTESIAN_POINT('Ctrl Pts',(44.9161774823427,-59.3905025255151,0.));
#61561=CARTESIAN_POINT('Ctrl Pts',(44.8063973817217,-59.3896476775505,0.));
#61562=CARTESIAN_POINT('Ctrl Pts',(44.724062306256,-59.3890065415771,0.));
#61563=CARTESIAN_POINT('Ctrl Pts',(44.6418181989799,-59.3674150879748,0.));
#61564=CARTESIAN_POINT('Ctrl Pts',(44.5696260757423,-59.3276657444157,0.));
#61565=CARTESIAN_POINT('',(44.5696260757422,-59.3276657444159,12.));
#61566=CARTESIAN_POINT('Ctrl Pts',(44.5696260757423,-59.3276657444157,0.));
#61567=CARTESIAN_POINT('Ctrl Pts',(44.5696260757423,-59.3276657444157,4.));
#61568=CARTESIAN_POINT('Ctrl Pts',(44.5696260757423,-59.3276657444157,8.));
#61569=CARTESIAN_POINT('Ctrl Pts',(44.5696260757423,-59.3276657444157,12.));
#61570=CARTESIAN_POINT('',(45.1135644683471,-59.2875729049545,12.));
#61571=CARTESIAN_POINT('Ctrl Pts',(44.5696260757423,-59.3276657444157,12.));
#61572=CARTESIAN_POINT('Ctrl Pts',(44.6418181989798,-59.3674150879747,12.));
#61573=CARTESIAN_POINT('Ctrl Pts',(44.724062306256,-59.3890065415771,12.));
#61574=CARTESIAN_POINT('Ctrl Pts',(44.8063973817217,-59.3896476775505,12.));
#61575=CARTESIAN_POINT('Ctrl Pts',(44.9161774823427,-59.3905025255151,12.));
#61576=CARTESIAN_POINT('Ctrl Pts',(45.0261193041895,-59.3541123643618,12.));
#61577=CARTESIAN_POINT('Ctrl Pts',(45.1135644683471,-59.2875729049545,12.));
#61578=CARTESIAN_POINT('Ctrl Pts',(45.1135644683471,-59.2875729049545,12.));
#61579=CARTESIAN_POINT('Ctrl Pts',(45.1135644683471,-59.2875729049545,8.));
#61580=CARTESIAN_POINT('Ctrl Pts',(45.1135644683471,-59.2875729049545,4.));
#61581=CARTESIAN_POINT('Ctrl Pts',(45.1135644683471,-59.2875729049545,0.));
#61582=CARTESIAN_POINT('Ctrl Pts',(40.8467768343956,-56.8466430164621,0.));
#61583=CARTESIAN_POINT('Ctrl Pts',(40.8467768343956,-56.8466430164621,12.));
#61584=CARTESIAN_POINT('Ctrl Pts',(40.8497761671036,-56.8491101022591,0.));
#61585=CARTESIAN_POINT('Ctrl Pts',(40.8497761671036,-56.8491101022591,12.));
#61586=CARTESIAN_POINT('Ctrl Pts',(40.8557803680278,-56.8540460739472,0.));
#61587=CARTESIAN_POINT('Ctrl Pts',(40.8557803680278,-56.8540460739472,12.));
#61588=CARTESIAN_POINT('Ctrl Pts',(40.864803275942,-56.8614554317668,0.));
#61589=CARTESIAN_POINT('Ctrl Pts',(40.864803275942,-56.8614554317668,12.));
#61590=CARTESIAN_POINT('Ctrl Pts',(40.8768670342052,-56.8713453764905,0.));
#61591=CARTESIAN_POINT('Ctrl Pts',(40.8768670342052,-56.8713453764905,12.));
#61592=CARTESIAN_POINT('Ctrl Pts',(40.8920020903293,-56.8837257978343,0.));
#61593=CARTESIAN_POINT('Ctrl Pts',(40.8920020903293,-56.8837257978343,12.));
#61594=CARTESIAN_POINT('Ctrl Pts',(40.9071924937508,-56.8961241708861,0.));
#61595=CARTESIAN_POINT('Ctrl Pts',(40.9071924937508,-56.8961241708861,12.));
#61596=CARTESIAN_POINT('Ctrl Pts',(40.9224382132427,-56.9085404164502,0.));
#61597=CARTESIAN_POINT('Ctrl Pts',(40.9224382132427,-56.9085404164502,12.));
#61598=CARTESIAN_POINT('Ctrl Pts',(40.9377391857129,-56.9209743960992,0.));
#61599=CARTESIAN_POINT('Ctrl Pts',(40.9377391857129,-56.9209743960992,12.));
#61600=CARTESIAN_POINT('Ctrl Pts',(40.9530953165031,-56.9334259140049,0.));
#61601=CARTESIAN_POINT('Ctrl Pts',(40.9530953165031,-56.9334259140049,12.));
#61602=CARTESIAN_POINT('Ctrl Pts',(40.9685064933074,-56.9458947422608,0.));
#61603=CARTESIAN_POINT('Ctrl Pts',(40.9685064933074,-56.9458947422608,12.));
#61604=CARTESIAN_POINT('Ctrl Pts',(40.9839725967121,-56.9583806404069,0.));
#61605=CARTESIAN_POINT('Ctrl Pts',(40.9839725967121,-56.9583806404069,12.));
#61606=CARTESIAN_POINT('Ctrl Pts',(40.9994935117276,-56.9708833766137,0.));
#61607=CARTESIAN_POINT('Ctrl Pts',(40.9994935117276,-56.9708833766137,12.));
#61608=CARTESIAN_POINT('Ctrl Pts',(41.0150691398947,-56.9834027500117,0.));
#61609=CARTESIAN_POINT('Ctrl Pts',(41.0150691398947,-56.9834027500117,12.));
#61610=CARTESIAN_POINT('Ctrl Pts',(41.0306993953989,-56.995938583472,0.));
#61611=CARTESIAN_POINT('Ctrl Pts',(41.0306993953989,-56.995938583472,12.));
#61612=CARTESIAN_POINT('Ctrl Pts',(41.0463841993608,-57.008490713042,0.));
#61613=CARTESIAN_POINT('Ctrl Pts',(41.0463841993608,-57.008490713042,12.));
#61614=CARTESIAN_POINT('Ctrl Pts',(41.0621234751007,-57.0210589791788,0.));
#61615=CARTESIAN_POINT('Ctrl Pts',(41.0621234751007,-57.0210589791788,12.));
#61616=CARTESIAN_POINT('Ctrl Pts',(41.0779171422438,-57.0336432158536,0.));
#61617=CARTESIAN_POINT('Ctrl Pts',(41.0779171422438,-57.0336432158536,12.));
#61618=CARTESIAN_POINT('Ctrl Pts',(41.0937651137549,-57.046243245068,0.));
#61619=CARTESIAN_POINT('Ctrl Pts',(41.0937651137549,-57.046243245068,12.));
#61620=CARTESIAN_POINT('Ctrl Pts',(41.1096672990148,-57.0588588825298,0.));
#61621=CARTESIAN_POINT('Ctrl Pts',(41.1096672990148,-57.0588588825298,12.));
#61622=CARTESIAN_POINT('Ctrl Pts',(41.1256236057443,-57.0714899412099,0.));
#61623=CARTESIAN_POINT('Ctrl Pts',(41.1256236057443,-57.0714899412099,12.));
#61624=CARTESIAN_POINT('Ctrl Pts',(41.1416339422117,-57.084136235426,0.));
#61625=CARTESIAN_POINT('Ctrl Pts',(41.1416339422117,-57.084136235426,12.));
#61626=CARTESIAN_POINT('Ctrl Pts',(41.1576982197375,-57.0967975854874,0.));
#61627=CARTESIAN_POINT('Ctrl Pts',(41.1576982197375,-57.0967975854874,12.));
#61628=CARTESIAN_POINT('Ctrl Pts',(41.1738163525902,-57.1094738174957,0.));
#61629=CARTESIAN_POINT('Ctrl Pts',(41.1738163525902,-57.1094738174957,12.));
#61630=CARTESIAN_POINT('Ctrl Pts',(41.1899882567923,-57.1221647611207,0.));
#61631=CARTESIAN_POINT('Ctrl Pts',(41.1899882567923,-57.1221647611207,12.));
#61632=CARTESIAN_POINT('Ctrl Pts',(41.2062138492915,-57.1348702480647,0.));
#61633=CARTESIAN_POINT('Ctrl Pts',(41.2062138492915,-57.1348702480647,12.));
#61634=CARTESIAN_POINT('Ctrl Pts',(41.222493046943,-57.147590110182,0.));
#61635=CARTESIAN_POINT('Ctrl Pts',(41.222493046943,-57.147590110182,12.));
#61636=CARTESIAN_POINT('Ctrl Pts',(41.2388257656559,-57.1603241779077,0.));
#61637=CARTESIAN_POINT('Ctrl Pts',(41.2388257656559,-57.1603241779077,12.));
#61638=CARTESIAN_POINT('Ctrl Pts',(41.2552119208466,-57.17307228108,0.));
#61639=CARTESIAN_POINT('Ctrl Pts',(41.2552119208466,-57.17307228108,12.));
#61640=CARTESIAN_POINT('Ctrl Pts',(41.2716514278276,-57.1858342496538,0.));
#61641=CARTESIAN_POINT('Ctrl Pts',(41.2716514278276,-57.1858342496538,12.));
#61642=CARTESIAN_POINT('Ctrl Pts',(41.2881442021863,-57.1986099143983,0.));
#61643=CARTESIAN_POINT('Ctrl Pts',(41.2881442021863,-57.1986099143983,12.));
#61644=CARTESIAN_POINT('Ctrl Pts',(41.3046901602293,-57.2113991077302,0.));
#61645=CARTESIAN_POINT('Ctrl Pts',(41.3046901602293,-57.2113991077302,12.));
#61646=CARTESIAN_POINT('Ctrl Pts',(41.321289219149,-57.2242016640198,0.));
#61647=CARTESIAN_POINT('Ctrl Pts',(41.321289219149,-57.2242016640198,12.));
#61648=CARTESIAN_POINT('Ctrl Pts',(41.3379412967875,-57.2370174191401,0.));
#61649=CARTESIAN_POINT('Ctrl Pts',(41.3379412967875,-57.2370174191401,12.));
#61650=CARTESIAN_POINT('Ctrl Pts',(41.3546463114885,-57.2498462101879,0.));
#61651=CARTESIAN_POINT('Ctrl Pts',(41.3546463114885,-57.2498462101879,12.));
#61652=CARTESIAN_POINT('Ctrl Pts',(41.3714041819224,-57.2626878751596,0.));
#61653=CARTESIAN_POINT('Ctrl Pts',(41.3714041819224,-57.2626878751596,12.));
#61654=CARTESIAN_POINT('Ctrl Pts',(41.3882148268814,-57.2755422525844,0.));
#61655=CARTESIAN_POINT('Ctrl Pts',(41.3882148268814,-57.2755422525844,12.));
#61656=CARTESIAN_POINT('Ctrl Pts',(41.4050781652938,-57.2884091815406,0.));
#61657=CARTESIAN_POINT('Ctrl Pts',(41.4050781652938,-57.2884091815406,12.));
#61658=CARTESIAN_POINT('Ctrl Pts',(41.4219941163163,-57.3012885018151,0.));
#61659=CARTESIAN_POINT('Ctrl Pts',(41.4219941163163,-57.3012885018151,12.));
#61660=CARTESIAN_POINT('Ctrl Pts',(41.4389625993948,-57.3141800540137,0.));
#61661=CARTESIAN_POINT('Ctrl Pts',(41.4389625993948,-57.3141800540137,12.));
#61662=CARTESIAN_POINT('Ctrl Pts',(41.4559835343328,-57.3270836796911,0.));
#61663=CARTESIAN_POINT('Ctrl Pts',(41.4559835343328,-57.3270836796911,12.));
#61664=CARTESIAN_POINT('Ctrl Pts',(41.4730568413518,-57.3399992214717,0.));
#61665=CARTESIAN_POINT('Ctrl Pts',(41.4730568413518,-57.3399992214717,12.));
#61666=CARTESIAN_POINT('Ctrl Pts',(41.4901824410637,-57.3529265229835,0.));
#61667=CARTESIAN_POINT('Ctrl Pts',(41.4901824410637,-57.3529265229835,12.));
#61668=CARTESIAN_POINT('Ctrl Pts',(41.5073602544396,-57.3658654287937,0.));
#61669=CARTESIAN_POINT('Ctrl Pts',(41.5073602544396,-57.3658654287937,12.));
#61670=CARTESIAN_POINT('Ctrl Pts',(41.5245902027771,-57.3788157843454,0.));
#61671=CARTESIAN_POINT('Ctrl Pts',(41.5245902027771,-57.3788157843454,12.));
#61672=CARTESIAN_POINT('Ctrl Pts',(41.5418722076572,-57.3917774358863,0.));
#61673=CARTESIAN_POINT('Ctrl Pts',(41.5418722076572,-57.3917774358863,12.));
#61674=CARTESIAN_POINT('Ctrl Pts',(41.5592061909176,-57.4047502304231,0.));
#61675=CARTESIAN_POINT('Ctrl Pts',(41.5592061909176,-57.4047502304231,12.));
#61676=CARTESIAN_POINT('Ctrl Pts',(41.5765920746777,-57.4177340157508,0.));
#61677=CARTESIAN_POINT('Ctrl Pts',(41.5765920746777,-57.4177340157508,12.));
#61678=CARTESIAN_POINT('Ctrl Pts',(41.5940297813477,-57.4307286404662,0.));
#61679=CARTESIAN_POINT('Ctrl Pts',(41.5940297813477,-57.4307286404662,12.));
#61680=CARTESIAN_POINT('Ctrl Pts',(41.6115192336388,-57.4437339539841,0.));
#61681=CARTESIAN_POINT('Ctrl Pts',(41.6115192336388,-57.4437339539841,12.));
#61682=CARTESIAN_POINT('Ctrl Pts',(41.6290603545666,-57.4567498065562,0.));
#61683=CARTESIAN_POINT('Ctrl Pts',(41.6290603545666,-57.4567498065562,12.));
#61684=CARTESIAN_POINT('Ctrl Pts',(41.6466530674515,-57.4697760492683,0.));
#61685=CARTESIAN_POINT('Ctrl Pts',(41.6466530674515,-57.4697760492683,12.));
#61686=CARTESIAN_POINT('Ctrl Pts',(41.6642972959165,-57.4828125340218,0.));
#61687=CARTESIAN_POINT('Ctrl Pts',(41.6642972959165,-57.4828125340218,12.));
#61688=CARTESIAN_POINT('Ctrl Pts',(41.6819929638797,-57.4958591135165,0.));
#61689=CARTESIAN_POINT('Ctrl Pts',(41.6819929638797,-57.4958591135165,12.));
#61690=CARTESIAN_POINT('Ctrl Pts',(41.6997399955447,-57.5089156412343,0.));
#61691=CARTESIAN_POINT('Ctrl Pts',(41.6997399955447,-57.5089156412343,12.));
#61692=CARTESIAN_POINT('Ctrl Pts',(41.7175383153821,-57.5219819714171,0.));
#61693=CARTESIAN_POINT('Ctrl Pts',(41.7175383153821,-57.5219819714171,12.));
#61694=CARTESIAN_POINT('Ctrl Pts',(41.7353878481337,-57.5350579590649,0.));
#61695=CARTESIAN_POINT('Ctrl Pts',(41.7353878481337,-57.5350579590649,12.));
#61696=CARTESIAN_POINT('Ctrl Pts',(41.7532885188175,-57.5481434599335,0.));
#61697=CARTESIAN_POINT('Ctrl Pts',(41.7532885188175,-57.5481434599335,12.));
#61698=CARTESIAN_POINT('Ctrl Pts',(41.7712402527273,-57.561238330532,0.));
#61699=CARTESIAN_POINT('Ctrl Pts',(41.7712402527273,-57.561238330532,12.));
#61700=CARTESIAN_POINT('Ctrl Pts',(41.7892429754297,-57.5743424281204,0.));
#61701=CARTESIAN_POINT('Ctrl Pts',(41.7892429754297,-57.5743424281204,12.));
#61702=CARTESIAN_POINT('Ctrl Pts',(41.8072966127558,-57.5874556107056,0.));
#61703=CARTESIAN_POINT('Ctrl Pts',(41.8072966127558,-57.5874556107056,12.));
#61704=CARTESIAN_POINT('Ctrl Pts',(41.8254010908051,-57.6005777370349,0.));
#61705=CARTESIAN_POINT('Ctrl Pts',(41.8254010908051,-57.6005777370349,12.));
#61706=CARTESIAN_POINT('Ctrl Pts',(41.8435563359456,-57.6137086665882,0.));
#61707=CARTESIAN_POINT('Ctrl Pts',(41.8435563359456,-57.6137086665882,12.));
#61708=CARTESIAN_POINT('Ctrl Pts',(41.8617622748108,-57.6268482595702,0.));
#61709=CARTESIAN_POINT('Ctrl Pts',(41.8617622748108,-57.6268482595702,12.));
#61710=CARTESIAN_POINT('Ctrl Pts',(41.8800188342909,-57.6399963769003,0.));
#61711=CARTESIAN_POINT('Ctrl Pts',(41.8800188342909,-57.6399963769003,12.));
#61712=CARTESIAN_POINT('Ctrl Pts',(41.8983259415245,-57.6531528802059,0.));
#61713=CARTESIAN_POINT('Ctrl Pts',(41.8983259415245,-57.6531528802059,12.));
#61714=CARTESIAN_POINT('Ctrl Pts',(41.9166835239046,-57.6663176318176,0.));
#61715=CARTESIAN_POINT('Ctrl Pts',(41.9166835239046,-57.6663176318176,12.));
#61716=CARTESIAN_POINT('Ctrl Pts',(41.9350915090791,-57.6794904947641,0.));
#61717=CARTESIAN_POINT('Ctrl Pts',(41.9350915090791,-57.6794904947641,12.));
#61718=CARTESIAN_POINT('Ctrl Pts',(41.9535498249489,-57.6926713327674,0.));
#61719=CARTESIAN_POINT('Ctrl Pts',(41.9535498249489,-57.6926713327674,12.));
#61720=CARTESIAN_POINT('Ctrl Pts',(41.9720583996601,-57.7058600102365,0.));
#61721=CARTESIAN_POINT('Ctrl Pts',(41.9720583996601,-57.7058600102365,12.));
#61722=CARTESIAN_POINT('Ctrl Pts',(41.9906171615975,-57.7190563922614,0.));
#61723=CARTESIAN_POINT('Ctrl Pts',(41.9906171615975,-57.7190563922614,12.));
#61724=CARTESIAN_POINT('Ctrl Pts',(42.0092260393911,-57.7322603446086,0.));
#61725=CARTESIAN_POINT('Ctrl Pts',(42.0092260393911,-57.7322603446086,12.));
#61726=CARTESIAN_POINT('Ctrl Pts',(42.0278849619156,-57.7454717337151,0.));
#61727=CARTESIAN_POINT('Ctrl Pts',(42.0278849619156,-57.7454717337151,12.));
#61728=CARTESIAN_POINT('Ctrl Pts',(42.0465938582878,-57.7586904266828,0.));
#61729=CARTESIAN_POINT('Ctrl Pts',(42.0465938582878,-57.7586904266828,12.));
#61730=CARTESIAN_POINT('Ctrl Pts',(42.0653526578571,-57.7719162912721,0.));
#61731=CARTESIAN_POINT('Ctrl Pts',(42.0653526578571,-57.7719162912721,12.));
#61732=CARTESIAN_POINT('Ctrl Pts',(42.0841612902018,-57.7851491958954,0.));
#61733=CARTESIAN_POINT('Ctrl Pts',(42.0841612902018,-57.7851491958954,12.));
#61734=CARTESIAN_POINT('Ctrl Pts',(42.1030196851344,-57.798389009613,0.));
#61735=CARTESIAN_POINT('Ctrl Pts',(42.1030196851344,-57.798389009613,12.));
#61736=CARTESIAN_POINT('Ctrl Pts',(42.121927772701,-57.8116356021274,0.));
#61737=CARTESIAN_POINT('Ctrl Pts',(42.121927772701,-57.8116356021274,12.));
#61738=CARTESIAN_POINT('Ctrl Pts',(42.1408854831792,-57.8248888437787,0.));
#61739=CARTESIAN_POINT('Ctrl Pts',(42.1408854831792,-57.8248888437787,12.));
#61740=CARTESIAN_POINT('Ctrl Pts',(42.1598927470671,-57.8381486055376,0.));
#61741=CARTESIAN_POINT('Ctrl Pts',(42.1598927470671,-57.8381486055376,12.));
#61742=CARTESIAN_POINT('Ctrl Pts',(42.1789494950824,-57.8514147590012,0.));
#61743=CARTESIAN_POINT('Ctrl Pts',(42.1789494950824,-57.8514147590012,12.));
#61744=CARTESIAN_POINT('Ctrl Pts',(42.1980556581689,-57.86468717639,0.));
#61745=CARTESIAN_POINT('Ctrl Pts',(42.1980556581689,-57.86468717639,12.));
#61746=CARTESIAN_POINT('Ctrl Pts',(42.2172111674946,-57.8779657305422,0.));
#61747=CARTESIAN_POINT('Ctrl Pts',(42.2172111674946,-57.8779657305422,12.));
#61748=CARTESIAN_POINT('Ctrl Pts',(42.2364159544492,-57.8912502949084,0.));
#61749=CARTESIAN_POINT('Ctrl Pts',(42.2364159544492,-57.8912502949084,12.));
#61750=CARTESIAN_POINT('Ctrl Pts',(42.2556699506332,-57.9045407435447,0.));
#61751=CARTESIAN_POINT('Ctrl Pts',(42.2556699506332,-57.9045407435447,12.));
#61752=CARTESIAN_POINT('Ctrl Pts',(42.274973087857,-57.9178369511084,0.));
#61753=CARTESIAN_POINT('Ctrl Pts',(42.274973087857,-57.9178369511084,12.));
#61754=CARTESIAN_POINT('Ctrl Pts',(42.2943252981471,-57.9311387928541,0.));
#61755=CARTESIAN_POINT('Ctrl Pts',(42.2943252981471,-57.9311387928541,12.));
#61756=CARTESIAN_POINT('Ctrl Pts',(42.3137265137446,-57.9444461446292,0.));
#61757=CARTESIAN_POINT('Ctrl Pts',(42.3137265137446,-57.9444461446292,12.));
#61758=CARTESIAN_POINT('Ctrl Pts',(42.3331766671028,-57.9577588828693,0.));
#61759=CARTESIAN_POINT('Ctrl Pts',(42.3331766671028,-57.9577588828693,12.));
#61760=CARTESIAN_POINT('Ctrl Pts',(42.3526756908764,-57.9710768845923,0.));
#61761=CARTESIAN_POINT('Ctrl Pts',(42.3526756908764,-57.9710768845923,12.));
#61762=CARTESIAN_POINT('Ctrl Pts',(42.3722235179216,-57.9844000273936,0.));
#61763=CARTESIAN_POINT('Ctrl Pts',(42.3722235179216,-57.9844000273936,12.));
#61764=CARTESIAN_POINT('Ctrl Pts',(42.3918200813025,-57.9977281894437,0.));
#61765=CARTESIAN_POINT('Ctrl Pts',(42.3918200813025,-57.9977281894437,12.));
#61766=CARTESIAN_POINT('Ctrl Pts',(42.4114653142891,-58.011061249483,0.));
#61767=CARTESIAN_POINT('Ctrl Pts',(42.4114653142891,-58.011061249483,12.));
#61768=CARTESIAN_POINT('Ctrl Pts',(42.4311591503551,-58.0243990868175,0.));
#61769=CARTESIAN_POINT('Ctrl Pts',(42.4311591503551,-58.0243990868175,12.));
#61770=CARTESIAN_POINT('Ctrl Pts',(42.4509015231668,-58.0377415813132,0.));
#61771=CARTESIAN_POINT('Ctrl Pts',(42.4509015231668,-58.0377415813132,12.));
#61772=CARTESIAN_POINT('Ctrl Pts',(42.4706923665838,-58.0510886133917,0.));
#61773=CARTESIAN_POINT('Ctrl Pts',(42.4706923665838,-58.0510886133917,12.));
#61774=CARTESIAN_POINT('Ctrl Pts',(42.490531614665,-58.064440064027,0.));
#61775=CARTESIAN_POINT('Ctrl Pts',(42.490531614665,-58.064440064027,12.));
#61776=CARTESIAN_POINT('Ctrl Pts',(42.5104192016664,-58.0777958147404,0.));
#61777=CARTESIAN_POINT('Ctrl Pts',(42.5104192016664,-58.0777958147404,12.));
#61778=CARTESIAN_POINT('Ctrl Pts',(42.5303550620388,-58.0911557475967,0.));
#61779=CARTESIAN_POINT('Ctrl Pts',(42.5303550620388,-58.0911557475967,12.));
#61780=CARTESIAN_POINT('Ctrl Pts',(42.5503391304183,-58.1045197452003,0.));
#61781=CARTESIAN_POINT('Ctrl Pts',(42.5503391304183,-58.1045197452003,12.));
#61782=CARTESIAN_POINT('Ctrl Pts',(42.5703713416263,-58.1178876906905,0.));
#61783=CARTESIAN_POINT('Ctrl Pts',(42.5703713416263,-58.1178876906905,12.));
#61784=CARTESIAN_POINT('Ctrl Pts',(42.5904516306759,-58.1312594677383,0.));
#61785=CARTESIAN_POINT('Ctrl Pts',(42.5904516306759,-58.1312594677383,12.));
#61786=CARTESIAN_POINT('Ctrl Pts',(42.6105799327697,-58.1446349605419,0.));
#61787=CARTESIAN_POINT('Ctrl Pts',(42.6105799327697,-58.1446349605419,12.));
#61788=CARTESIAN_POINT('Ctrl Pts',(42.6307561832978,-58.158014053823,0.));
#61789=CARTESIAN_POINT('Ctrl Pts',(42.6307561832978,-58.158014053823,12.));
#61790=CARTESIAN_POINT('Ctrl Pts',(42.650980317827,-58.1713966328217,0.));
#61791=CARTESIAN_POINT('Ctrl Pts',(42.650980317827,-58.1713966328217,12.));
#61792=CARTESIAN_POINT('Ctrl Pts',(42.6712522721021,-58.1847825832932,0.));
#61793=CARTESIAN_POINT('Ctrl Pts',(42.6712522721021,-58.1847825832932,12.));
#61794=CARTESIAN_POINT('Ctrl Pts',(42.6915719820517,-58.1981717915043,0.));
#61795=CARTESIAN_POINT('Ctrl Pts',(42.6915719820517,-58.1981717915043,12.));
#61796=CARTESIAN_POINT('Ctrl Pts',(42.7119393837867,-58.2115641442302,0.));
#61797=CARTESIAN_POINT('Ctrl Pts',(42.7119393837867,-58.2115641442302,12.));
#61798=CARTESIAN_POINT('Ctrl Pts',(42.7323544135983,-58.2249595287497,0.));
#61799=CARTESIAN_POINT('Ctrl Pts',(42.7323544135983,-58.2249595287497,12.));
#61800=CARTESIAN_POINT('Ctrl Pts',(42.7528170079482,-58.238357832842,0.));
#61801=CARTESIAN_POINT('Ctrl Pts',(42.7528170079482,-58.238357832842,12.));
#61802=CARTESIAN_POINT('Ctrl Pts',(42.7733271034679,-58.2517589447818,0.));
#61803=CARTESIAN_POINT('Ctrl Pts',(42.7733271034679,-58.2517589447818,12.));
#61804=CARTESIAN_POINT('Ctrl Pts',(42.7938846369651,-58.2651627533368,0.));
#61805=CARTESIAN_POINT('Ctrl Pts',(42.7938846369651,-58.2651627533368,12.));
#61806=CARTESIAN_POINT('Ctrl Pts',(42.8144895454234,-58.278569147764,0.));
#61807=CARTESIAN_POINT('Ctrl Pts',(42.8144895454234,-58.278569147764,12.));
#61808=CARTESIAN_POINT('Ctrl Pts',(42.8351417659998,-58.2919780178063,0.));
#61809=CARTESIAN_POINT('Ctrl Pts',(42.8351417659998,-58.2919780178063,12.));
#61810=CARTESIAN_POINT('Ctrl Pts',(42.8558412360154,-58.305389253689,0.));
#61811=CARTESIAN_POINT('Ctrl Pts',(42.8558412360154,-58.305389253689,12.));
#61812=CARTESIAN_POINT('Ctrl Pts',(42.8765878929545,-58.3188027461157,0.));
#61813=CARTESIAN_POINT('Ctrl Pts',(42.8765878929545,-58.3188027461157,12.));
#61814=CARTESIAN_POINT('Ctrl Pts',(42.8973816744703,-58.3322183862647,0.));
#61815=CARTESIAN_POINT('Ctrl Pts',(42.8973816744703,-58.3322183862647,12.));
#61816=CARTESIAN_POINT('Ctrl Pts',(42.9182225183851,-58.3456360657861,0.));
#61817=CARTESIAN_POINT('Ctrl Pts',(42.9182225183851,-58.3456360657861,12.));
#61818=CARTESIAN_POINT('Ctrl Pts',(42.9391103626881,-58.3590556767981,0.));
#61819=CARTESIAN_POINT('Ctrl Pts',(42.9391103626881,-58.3590556767981,12.));
#61820=CARTESIAN_POINT('Ctrl Pts',(42.9600451455267,-58.3724771118835,0.));
#61821=CARTESIAN_POINT('Ctrl Pts',(42.9600451455267,-58.3724771118835,12.));
#61822=CARTESIAN_POINT('Ctrl Pts',(42.9810268052043,-58.3859002640871,0.));
#61823=CARTESIAN_POINT('Ctrl Pts',(42.9810268052043,-58.3859002640871,12.));
#61824=CARTESIAN_POINT('Ctrl Pts',(43.002055280187,-58.3993250269115,0.));
#61825=CARTESIAN_POINT('Ctrl Pts',(43.002055280187,-58.3993250269115,12.));
#61826=CARTESIAN_POINT('Ctrl Pts',(43.0231305091033,-58.4127512943144,0.));
#61827=CARTESIAN_POINT('Ctrl Pts',(43.0231305091033,-58.4127512943144,12.));
#61828=CARTESIAN_POINT('Ctrl Pts',(43.0442524307432,-58.4261789607055,0.));
#61829=CARTESIAN_POINT('Ctrl Pts',(43.0442524307432,-58.4261789607055,12.));
#61830=CARTESIAN_POINT('Ctrl Pts',(43.0654209840502,-58.4396079209438,0.));
#61831=CARTESIAN_POINT('Ctrl Pts',(43.0654209840502,-58.4396079209438,12.));
#61832=CARTESIAN_POINT('Ctrl Pts',(43.0866361081166,-58.4530380703335,0.));
#61833=CARTESIAN_POINT('Ctrl Pts',(43.0866361081166,-58.4530380703335,12.));
#61834=CARTESIAN_POINT('Ctrl Pts',(43.1078977421908,-58.4664693046206,0.));
#61835=CARTESIAN_POINT('Ctrl Pts',(43.1078977421908,-58.4664693046206,12.));
#61836=CARTESIAN_POINT('Ctrl Pts',(43.1292058256774,-58.4799015199904,0.));
#61837=CARTESIAN_POINT('Ctrl Pts',(43.1292058256774,-58.4799015199904,12.));
#61838=CARTESIAN_POINT('Ctrl Pts',(43.1505602981366,-58.4933346130638,0.));
#61839=CARTESIAN_POINT('Ctrl Pts',(43.1505602981366,-58.4933346130638,12.));
#61840=CARTESIAN_POINT('Ctrl Pts',(43.1719610992772,-58.5067684808946,0.));
#61841=CARTESIAN_POINT('Ctrl Pts',(43.1719610992772,-58.5067684808946,12.));
#61842=CARTESIAN_POINT('Ctrl Pts',(43.1934081689504,-58.5202030209667,0.));
#61843=CARTESIAN_POINT('Ctrl Pts',(43.1934081689504,-58.5202030209667,12.));
#61844=CARTESIAN_POINT('Ctrl Pts',(43.214901447157,-58.5336381311911,0.));
#61845=CARTESIAN_POINT('Ctrl Pts',(43.214901447157,-58.5336381311911,12.));
#61846=CARTESIAN_POINT('Ctrl Pts',(43.2364408740489,-58.5470737099027,0.));
#61847=CARTESIAN_POINT('Ctrl Pts',(43.2364408740489,-58.5470737099027,12.));
#61848=CARTESIAN_POINT('Ctrl Pts',(43.2580263899278,-58.5605096558578,0.));
#61849=CARTESIAN_POINT('Ctrl Pts',(43.2580263899278,-58.5605096558578,12.));
#61850=CARTESIAN_POINT('Ctrl Pts',(43.2796579352405,-58.5739458682317,0.));
#61851=CARTESIAN_POINT('Ctrl Pts',(43.2796579352405,-58.5739458682317,12.));
#61852=CARTESIAN_POINT('Ctrl Pts',(43.3013354505708,-58.5873822466163,0.));
#61853=CARTESIAN_POINT('Ctrl Pts',(43.3013354505708,-58.5873822466163,12.));
#61854=CARTESIAN_POINT('Ctrl Pts',(43.3230588766456,-58.6008186910166,0.));
#61855=CARTESIAN_POINT('Ctrl Pts',(43.3230588766456,-58.6008186910166,12.));
#61856=CARTESIAN_POINT('Ctrl Pts',(43.3448281543375,-58.6142551018473,0.));
#61857=CARTESIAN_POINT('Ctrl Pts',(43.3448281543375,-58.6142551018473,12.));
#61858=CARTESIAN_POINT('Ctrl Pts',(43.3666432246635,-58.627691379929,0.));
#61859=CARTESIAN_POINT('Ctrl Pts',(43.3666432246635,-58.627691379929,12.));
#61860=CARTESIAN_POINT('Ctrl Pts',(43.3885040287808,-58.6411274264854,0.));
#61861=CARTESIAN_POINT('Ctrl Pts',(43.3885040287808,-58.6411274264854,12.));
#61862=CARTESIAN_POINT('Ctrl Pts',(43.4104105079766,-58.6545631431388,0.));
#61863=CARTESIAN_POINT('Ctrl Pts',(43.4104105079766,-58.6545631431388,12.));
#61864=CARTESIAN_POINT('Ctrl Pts',(43.4323626036736,-58.6679984319095,0.));
#61865=CARTESIAN_POINT('Ctrl Pts',(43.4323626036736,-58.6679984319095,12.));
#61866=CARTESIAN_POINT('Ctrl Pts',(43.4543602574352,-58.6814331952138,0.));
#61867=CARTESIAN_POINT('Ctrl Pts',(43.4543602574352,-58.6814331952138,12.));
#61868=CARTESIAN_POINT('Ctrl Pts',(43.4764034109655,-58.6948673358639,0.));
#61869=CARTESIAN_POINT('Ctrl Pts',(43.4764034109655,-58.6948673358639,12.));
#61870=CARTESIAN_POINT('Ctrl Pts',(43.4984920061071,-58.708300757066,0.));
#61871=CARTESIAN_POINT('Ctrl Pts',(43.4984920061071,-58.708300757066,12.));
#61872=CARTESIAN_POINT('Ctrl Pts',(43.5206259848333,-58.7217333624206,0.));
#61873=CARTESIAN_POINT('Ctrl Pts',(43.5206259848333,-58.7217333624206,12.));
#61874=CARTESIAN_POINT('Ctrl Pts',(43.5428052892483,-58.7351650559176,0.));
#61875=CARTESIAN_POINT('Ctrl Pts',(43.5428052892483,-58.7351650559176,12.));
#61876=CARTESIAN_POINT('Ctrl Pts',(43.5650298615912,-58.7485957419296,0.));
#61877=CARTESIAN_POINT('Ctrl Pts',(43.5650298615912,-58.7485957419296,12.));
#61878=CARTESIAN_POINT('Ctrl Pts',(43.5872996442343,-58.7620253252059,0.));
#61879=CARTESIAN_POINT('Ctrl Pts',(43.5872996442343,-58.7620253252059,12.));
#61880=CARTESIAN_POINT('Ctrl Pts',(43.6096145796798,-58.7754537108672,0.));
#61881=CARTESIAN_POINT('Ctrl Pts',(43.6096145796798,-58.7754537108672,12.));
#61882=CARTESIAN_POINT('Ctrl Pts',(43.6319746105488,-58.7888808043976,0.));
#61883=CARTESIAN_POINT('Ctrl Pts',(43.6319746105488,-58.7888808043976,12.));
#61884=CARTESIAN_POINT('Ctrl Pts',(43.6543796795797,-58.8023065116446,0.));
#61885=CARTESIAN_POINT('Ctrl Pts',(43.6543796795797,-58.8023065116446,12.));
#61886=CARTESIAN_POINT('Ctrl Pts',(43.6768297296403,-58.8157307388247,0.));
#61887=CARTESIAN_POINT('Ctrl Pts',(43.6768297296403,-58.8157307388247,12.));
#61888=CARTESIAN_POINT('Ctrl Pts',(43.6993247037318,-58.8291533925299,0.));
#61889=CARTESIAN_POINT('Ctrl Pts',(43.6993247037318,-58.8291533925299,12.));
#61890=CARTESIAN_POINT('Ctrl Pts',(43.7218645449921,-58.8425743797325,0.));
#61891=CARTESIAN_POINT('Ctrl Pts',(43.7218645449921,-58.8425743797325,12.));
#61892=CARTESIAN_POINT('Ctrl Pts',(43.7444491966935,-58.8559936077933,0.));
#61893=CARTESIAN_POINT('Ctrl Pts',(43.7444491966935,-58.8559936077933,12.));
#61894=CARTESIAN_POINT('Ctrl Pts',(43.7670786022392,-58.8694109844636,0.));
#61895=CARTESIAN_POINT('Ctrl Pts',(43.7670786022392,-58.8694109844636,12.));
#61896=CARTESIAN_POINT('Ctrl Pts',(43.7897527051599,-58.882826417861,0.));
#61897=CARTESIAN_POINT('Ctrl Pts',(43.7897527051599,-58.882826417861,12.));
#61898=CARTESIAN_POINT('Ctrl Pts',(43.812471449107,-58.8962398164486,0.));
#61899=CARTESIAN_POINT('Ctrl Pts',(43.812471449107,-58.8962398164486,12.));
#61900=CARTESIAN_POINT('Ctrl Pts',(43.8352347778419,-58.9096510890128,0.));
#61901=CARTESIAN_POINT('Ctrl Pts',(43.8352347778419,-58.9096510890128,12.));
#61902=CARTESIAN_POINT('Ctrl Pts',(43.8580426352236,-58.9230601446445,0.));
#61903=CARTESIAN_POINT('Ctrl Pts',(43.8580426352236,-58.9230601446445,12.));
#61904=CARTESIAN_POINT('Ctrl Pts',(43.8808949651882,-58.9364668927132,0.));
#61905=CARTESIAN_POINT('Ctrl Pts',(43.8808949651882,-58.9364668927132,12.));
#61906=CARTESIAN_POINT('Ctrl Pts',(43.9037917117749,-58.9498712429066,0.));
#61907=CARTESIAN_POINT('Ctrl Pts',(43.9037917117749,-58.9498712429066,12.));
#61908=CARTESIAN_POINT('Ctrl Pts',(43.9267328191508,-58.9632731052704,0.));
#61909=CARTESIAN_POINT('Ctrl Pts',(43.9267328191508,-58.9632731052704,12.));
#61910=CARTESIAN_POINT('Ctrl Pts',(43.9497182316333,-58.9766723902531,0.));
#61911=CARTESIAN_POINT('Ctrl Pts',(43.9497182316333,-58.9766723902531,12.));
#61912=CARTESIAN_POINT('Ctrl Pts',(43.9727478937053,-58.9900690087404,0.));
#61913=CARTESIAN_POINT('Ctrl Pts',(43.9727478937053,-58.9900690087404,12.));
#61914=CARTESIAN_POINT('Ctrl Pts',(43.9958217500364,-59.0034628721161,0.));
#61915=CARTESIAN_POINT('Ctrl Pts',(43.9958217500364,-59.0034628721161,12.));
#61916=CARTESIAN_POINT('Ctrl Pts',(44.0189397454593,-59.0168538922087,0.));
#61917=CARTESIAN_POINT('Ctrl Pts',(44.0189397454593,-59.0168538922087,12.));
#61918=CARTESIAN_POINT('Ctrl Pts',(44.0421018249219,-59.0302419811772,0.));
#61919=CARTESIAN_POINT('Ctrl Pts',(44.0421018249219,-59.0302419811772,12.));
#61920=CARTESIAN_POINT('Ctrl Pts',(44.0653079334384,-59.0436270514085,0.));
#61921=CARTESIAN_POINT('Ctrl Pts',(44.0653079334384,-59.0436270514085,12.));
#61922=CARTESIAN_POINT('Ctrl Pts',(44.0885580160433,-59.0570090154243,0.));
#61923=CARTESIAN_POINT('Ctrl Pts',(44.0885580160433,-59.0570090154243,12.));
#61924=CARTESIAN_POINT('Ctrl Pts',(44.1118520177224,-59.0703877857529,0.));
#61925=CARTESIAN_POINT('Ctrl Pts',(44.1118520177224,-59.0703877857529,12.));
#61926=CARTESIAN_POINT('Ctrl Pts',(44.1351898834057,-59.0837632749209,0.));
#61927=CARTESIAN_POINT('Ctrl Pts',(44.1351898834057,-59.0837632749209,12.));
#61928=CARTESIAN_POINT('Ctrl Pts',(44.1585715581074,-59.0971353957218,0.));
#61929=CARTESIAN_POINT('Ctrl Pts',(44.1585715581074,-59.0971353957218,12.));
#61930=CARTESIAN_POINT('Ctrl Pts',(44.1819969870314,-59.1105040614285,0.));
#61931=CARTESIAN_POINT('Ctrl Pts',(44.1819969870314,-59.1105040614285,12.));
#61932=CARTESIAN_POINT('Ctrl Pts',(44.2054661156876,-59.1238691860307,0.));
#61933=CARTESIAN_POINT('Ctrl Pts',(44.2054661156876,-59.1238691860307,12.));
#61934=CARTESIAN_POINT('Ctrl Pts',(44.2289788899962,-59.1372306844575,0.));
#61935=CARTESIAN_POINT('Ctrl Pts',(44.2289788899962,-59.1372306844575,12.));
#61936=CARTESIAN_POINT('Ctrl Pts',(44.2525352563979,-59.1505884728194,0.));
#61937=CARTESIAN_POINT('Ctrl Pts',(44.2525352563979,-59.1505884728194,12.));
#61938=CARTESIAN_POINT('Ctrl Pts',(44.2761351616027,-59.1639424678766,0.));
#61939=CARTESIAN_POINT('Ctrl Pts',(44.2761351616027,-59.1639424678766,12.));
#61940=CARTESIAN_POINT('Ctrl Pts',(44.2997785523413,-59.1772925865191,0.));
#61941=CARTESIAN_POINT('Ctrl Pts',(44.2997785523413,-59.1772925865191,12.));
#61942=CARTESIAN_POINT('Ctrl Pts',(44.3234653750877,-59.1906387451971,0.));
#61943=CARTESIAN_POINT('Ctrl Pts',(44.3234653750877,-59.1906387451971,12.));
#61944=CARTESIAN_POINT('Ctrl Pts',(44.3471955758412,-59.2039808594765,0.));
#61945=CARTESIAN_POINT('Ctrl Pts',(44.3471955758412,-59.2039808594765,12.));
#61946=CARTESIAN_POINT('Ctrl Pts',(44.3709690997495,-59.217318843283,0.));
#61947=CARTESIAN_POINT('Ctrl Pts',(44.3709690997495,-59.217318843283,12.));
#61948=CARTESIAN_POINT('Ctrl Pts',(44.394785891411,-59.2306526095175,0.));
#61949=CARTESIAN_POINT('Ctrl Pts',(44.394785891411,-59.2306526095175,12.));
#61950=CARTESIAN_POINT('Ctrl Pts',(44.4186458955486,-59.2439820714231,0.));
#61951=CARTESIAN_POINT('Ctrl Pts',(44.4186458955486,-59.2439820714231,12.));
#61952=CARTESIAN_POINT('Ctrl Pts',(44.4425490575932,-59.2573071437801,0.));
#61953=CARTESIAN_POINT('Ctrl Pts',(44.4425490575932,-59.2573071437801,12.));
#61954=CARTESIAN_POINT('Ctrl Pts',(44.4664953242373,-59.2706277440438,0.));
#61955=CARTESIAN_POINT('Ctrl Pts',(44.4664953242373,-59.2706277440438,12.));
#61956=CARTESIAN_POINT('Ctrl Pts',(44.490484644147,-59.2839437938187,0.));
#61957=CARTESIAN_POINT('Ctrl Pts',(44.490484644147,-59.2839437938187,12.));
#61958=CARTESIAN_POINT('Ctrl Pts',(44.514516968128,-59.2972552192072,0.));
#61959=CARTESIAN_POINT('Ctrl Pts',(44.514516968128,-59.2972552192072,12.));
#61960=CARTESIAN_POINT('Ctrl Pts',(44.5385922475494,-59.3105619475512,0.));
#61961=CARTESIAN_POINT('Ctrl Pts',(44.5385922475494,-59.3105619475512,12.));
#61962=CARTESIAN_POINT('Ctrl Pts',(44.5627104330956,-59.3238639048618,0.));
#61963=CARTESIAN_POINT('Ctrl Pts',(44.5627104330956,-59.3238639048618,12.));
#61964=CARTESIAN_POINT('Ctrl Pts',(44.586871473322,-59.3371610128494,0.));
#61965=CARTESIAN_POINT('Ctrl Pts',(44.586871473322,-59.3371610128494,12.));
#61966=CARTESIAN_POINT('Ctrl Pts',(44.6110753134333,-59.3504531864223,0.));
#61967=CARTESIAN_POINT('Ctrl Pts',(44.6110753134333,-59.3504531864223,12.));
#61968=CARTESIAN_POINT('Ctrl Pts',(44.6353218935813,-59.3637403301959,0.));
#61969=CARTESIAN_POINT('Ctrl Pts',(44.6353218935813,-59.3637403301959,12.));
#61970=CARTESIAN_POINT('Ctrl Pts',(44.6596111512861,-59.3770223435405,0.));
#61971=CARTESIAN_POINT('Ctrl Pts',(44.6596111512861,-59.3770223435405,12.));
#61972=CARTESIAN_POINT('Ctrl Pts',(44.6839430244376,-59.3902991268094,0.));
#61973=CARTESIAN_POINT('Ctrl Pts',(44.6839430244376,-59.3902991268094,12.));
#61974=CARTESIAN_POINT('Ctrl Pts',(44.708317454179,-59.403570587392,0.));
#61975=CARTESIAN_POINT('Ctrl Pts',(44.708317454179,-59.403570587392,12.));
#61976=CARTESIAN_POINT('Ctrl Pts',(44.7327343876333,-59.4168366453047,0.));
#61977=CARTESIAN_POINT('Ctrl Pts',(44.7327343876333,-59.4168366453047,12.));
#61978=CARTESIAN_POINT('Ctrl Pts',(44.7571937811872,-59.4300972402943,0.));
#61979=CARTESIAN_POINT('Ctrl Pts',(44.7571937811872,-59.4300972402943,12.));
#61980=CARTESIAN_POINT('Ctrl Pts',(44.7816956017127,-59.4433523334651,0.));
#61981=CARTESIAN_POINT('Ctrl Pts',(44.7816956017127,-59.4433523334651,12.));
#61982=CARTESIAN_POINT('Ctrl Pts',(44.8062398250937,-59.4566019017674,0.));
#61983=CARTESIAN_POINT('Ctrl Pts',(44.8062398250937,-59.4566019017674,12.));
#61984=CARTESIAN_POINT('Ctrl Pts',(44.8259091133624,-59.4671971277837,0.));
#61985=CARTESIAN_POINT('Ctrl Pts',(44.8259091133624,-59.4671971277837,12.));
#61986=CARTESIAN_POINT('Ctrl Pts',(44.8406801497506,-59.475141054744,0.));
#61987=CARTESIAN_POINT('Ctrl Pts',(44.8406801497506,-59.475141054744,12.));
#61988=CARTESIAN_POINT('Ctrl Pts',(44.8505359826374,-59.4804358982977,0.));
#61989=CARTESIAN_POINT('Ctrl Pts',(44.8505359826374,-59.4804358982977,12.));
#61990=CARTESIAN_POINT('Ctrl Pts',(44.8554660179045,-59.483083043136,0.));
#61991=CARTESIAN_POINT('Ctrl Pts',(44.8554660179045,-59.483083043136,12.));
#61992=CARTESIAN_POINT('',(40.8467768343956,-56.8466430164621,0.));
#61993=CARTESIAN_POINT('Ctrl Pts',(40.8467768343956,-56.8466430164621,0.));
#61994=CARTESIAN_POINT('Ctrl Pts',(40.8497761671036,-56.8491101022591,0.));
#61995=CARTESIAN_POINT('Ctrl Pts',(40.8557803680278,-56.8540460739472,0.));
#61996=CARTESIAN_POINT('Ctrl Pts',(40.864803275942,-56.8614554317668,0.));
#61997=CARTESIAN_POINT('Ctrl Pts',(40.8768670342052,-56.8713453764905,0.));
#61998=CARTESIAN_POINT('Ctrl Pts',(40.8920020903293,-56.8837257978343,0.));
#61999=CARTESIAN_POINT('Ctrl Pts',(40.9071924937508,-56.8961241708861,0.));
#62000=CARTESIAN_POINT('Ctrl Pts',(40.9224382132427,-56.9085404164502,0.));
#62001=CARTESIAN_POINT('Ctrl Pts',(40.9377391857129,-56.9209743960992,0.));
#62002=CARTESIAN_POINT('Ctrl Pts',(40.9530953165031,-56.9334259140049,0.));
#62003=CARTESIAN_POINT('Ctrl Pts',(40.9685064933074,-56.9458947422608,0.));
#62004=CARTESIAN_POINT('Ctrl Pts',(40.9839725967121,-56.9583806404069,0.));
#62005=CARTESIAN_POINT('Ctrl Pts',(40.9994935117276,-56.9708833766137,0.));
#62006=CARTESIAN_POINT('Ctrl Pts',(41.0150691398947,-56.9834027500117,0.));
#62007=CARTESIAN_POINT('Ctrl Pts',(41.0306993953989,-56.995938583472,0.));
#62008=CARTESIAN_POINT('Ctrl Pts',(41.0463841993608,-57.008490713042,0.));
#62009=CARTESIAN_POINT('Ctrl Pts',(41.0621234751007,-57.0210589791788,0.));
#62010=CARTESIAN_POINT('Ctrl Pts',(41.0779171422438,-57.0336432158536,0.));
#62011=CARTESIAN_POINT('Ctrl Pts',(41.0937651137549,-57.046243245068,0.));
#62012=CARTESIAN_POINT('Ctrl Pts',(41.1096672990148,-57.0588588825298,0.));
#62013=CARTESIAN_POINT('Ctrl Pts',(41.1256236057443,-57.0714899412099,0.));
#62014=CARTESIAN_POINT('Ctrl Pts',(41.1416339422117,-57.084136235426,0.));
#62015=CARTESIAN_POINT('Ctrl Pts',(41.1576982197375,-57.0967975854874,0.));
#62016=CARTESIAN_POINT('Ctrl Pts',(41.1738163525902,-57.1094738174957,0.));
#62017=CARTESIAN_POINT('Ctrl Pts',(41.1899882567923,-57.1221647611207,0.));
#62018=CARTESIAN_POINT('Ctrl Pts',(41.2062138492915,-57.1348702480647,0.));
#62019=CARTESIAN_POINT('Ctrl Pts',(41.222493046943,-57.147590110182,0.));
#62020=CARTESIAN_POINT('Ctrl Pts',(41.2388257656559,-57.1603241779077,0.));
#62021=CARTESIAN_POINT('Ctrl Pts',(41.2552119208466,-57.17307228108,0.));
#62022=CARTESIAN_POINT('Ctrl Pts',(41.2716514278276,-57.1858342496538,0.));
#62023=CARTESIAN_POINT('Ctrl Pts',(41.2881442021863,-57.1986099143983,0.));
#62024=CARTESIAN_POINT('Ctrl Pts',(41.3046901602293,-57.2113991077302,0.));
#62025=CARTESIAN_POINT('Ctrl Pts',(41.321289219149,-57.2242016640198,0.));
#62026=CARTESIAN_POINT('Ctrl Pts',(41.3379412967875,-57.2370174191401,0.));
#62027=CARTESIAN_POINT('Ctrl Pts',(41.3546463114885,-57.2498462101879,0.));
#62028=CARTESIAN_POINT('Ctrl Pts',(41.3714041819224,-57.2626878751596,0.));
#62029=CARTESIAN_POINT('Ctrl Pts',(41.3882148268814,-57.2755422525844,0.));
#62030=CARTESIAN_POINT('Ctrl Pts',(41.4050781652938,-57.2884091815406,0.));
#62031=CARTESIAN_POINT('Ctrl Pts',(41.4219941163163,-57.3012885018151,0.));
#62032=CARTESIAN_POINT('Ctrl Pts',(41.4389625993948,-57.3141800540137,0.));
#62033=CARTESIAN_POINT('Ctrl Pts',(41.4559835343328,-57.3270836796911,0.));
#62034=CARTESIAN_POINT('Ctrl Pts',(41.4730568413518,-57.3399992214717,0.));
#62035=CARTESIAN_POINT('Ctrl Pts',(41.4901824410637,-57.3529265229835,0.));
#62036=CARTESIAN_POINT('Ctrl Pts',(41.5073602544396,-57.3658654287937,0.));
#62037=CARTESIAN_POINT('Ctrl Pts',(41.5245902027771,-57.3788157843454,0.));
#62038=CARTESIAN_POINT('Ctrl Pts',(41.5418722076572,-57.3917774358863,0.));
#62039=CARTESIAN_POINT('Ctrl Pts',(41.5592061909176,-57.4047502304231,0.));
#62040=CARTESIAN_POINT('Ctrl Pts',(41.5765920746777,-57.4177340157508,0.));
#62041=CARTESIAN_POINT('Ctrl Pts',(41.5940297813477,-57.4307286404662,0.));
#62042=CARTESIAN_POINT('Ctrl Pts',(41.6115192336388,-57.4437339539841,0.));
#62043=CARTESIAN_POINT('Ctrl Pts',(41.6290603545666,-57.4567498065562,0.));
#62044=CARTESIAN_POINT('Ctrl Pts',(41.6466530674515,-57.4697760492683,0.));
#62045=CARTESIAN_POINT('Ctrl Pts',(41.6642972959165,-57.4828125340218,0.));
#62046=CARTESIAN_POINT('Ctrl Pts',(41.6819929638797,-57.4958591135165,0.));
#62047=CARTESIAN_POINT('Ctrl Pts',(41.6997399955447,-57.5089156412343,0.));
#62048=CARTESIAN_POINT('Ctrl Pts',(41.7175383153821,-57.5219819714171,0.));
#62049=CARTESIAN_POINT('Ctrl Pts',(41.7353878481337,-57.5350579590649,0.));
#62050=CARTESIAN_POINT('Ctrl Pts',(41.7532885188175,-57.5481434599335,0.));
#62051=CARTESIAN_POINT('Ctrl Pts',(41.7712402527273,-57.561238330532,0.));
#62052=CARTESIAN_POINT('Ctrl Pts',(41.7892429754297,-57.5743424281204,0.));
#62053=CARTESIAN_POINT('Ctrl Pts',(41.8072966127558,-57.5874556107056,0.));
#62054=CARTESIAN_POINT('Ctrl Pts',(41.8254010908051,-57.6005777370349,0.));
#62055=CARTESIAN_POINT('Ctrl Pts',(41.8435563359456,-57.6137086665882,0.));
#62056=CARTESIAN_POINT('Ctrl Pts',(41.8617622748108,-57.6268482595702,0.));
#62057=CARTESIAN_POINT('Ctrl Pts',(41.8800188342909,-57.6399963769003,0.));
#62058=CARTESIAN_POINT('Ctrl Pts',(41.8983259415245,-57.6531528802059,0.));
#62059=CARTESIAN_POINT('Ctrl Pts',(41.9166835239046,-57.6663176318176,0.));
#62060=CARTESIAN_POINT('Ctrl Pts',(41.9350915090791,-57.6794904947641,0.));
#62061=CARTESIAN_POINT('Ctrl Pts',(41.9535498249489,-57.6926713327674,0.));
#62062=CARTESIAN_POINT('Ctrl Pts',(41.9720583996601,-57.7058600102365,0.));
#62063=CARTESIAN_POINT('Ctrl Pts',(41.9906171615975,-57.7190563922614,0.));
#62064=CARTESIAN_POINT('Ctrl Pts',(42.0092260393911,-57.7322603446086,0.));
#62065=CARTESIAN_POINT('Ctrl Pts',(42.0278849619156,-57.7454717337151,0.));
#62066=CARTESIAN_POINT('Ctrl Pts',(42.0465938582878,-57.7586904266828,0.));
#62067=CARTESIAN_POINT('Ctrl Pts',(42.0653526578571,-57.7719162912721,0.));
#62068=CARTESIAN_POINT('Ctrl Pts',(42.0841612902018,-57.7851491958954,0.));
#62069=CARTESIAN_POINT('Ctrl Pts',(42.1030196851344,-57.798389009613,0.));
#62070=CARTESIAN_POINT('Ctrl Pts',(42.121927772701,-57.8116356021274,0.));
#62071=CARTESIAN_POINT('Ctrl Pts',(42.1408854831792,-57.8248888437787,0.));
#62072=CARTESIAN_POINT('Ctrl Pts',(42.1598927470671,-57.8381486055376,0.));
#62073=CARTESIAN_POINT('Ctrl Pts',(42.1789494950824,-57.8514147590012,0.));
#62074=CARTESIAN_POINT('Ctrl Pts',(42.1980556581689,-57.86468717639,0.));
#62075=CARTESIAN_POINT('Ctrl Pts',(42.2172111674946,-57.8779657305422,0.));
#62076=CARTESIAN_POINT('Ctrl Pts',(42.2364159544492,-57.8912502949084,0.));
#62077=CARTESIAN_POINT('Ctrl Pts',(42.2556699506332,-57.9045407435447,0.));
#62078=CARTESIAN_POINT('Ctrl Pts',(42.274973087857,-57.9178369511084,0.));
#62079=CARTESIAN_POINT('Ctrl Pts',(42.2943252981471,-57.9311387928541,0.));
#62080=CARTESIAN_POINT('Ctrl Pts',(42.3137265137446,-57.9444461446292,0.));
#62081=CARTESIAN_POINT('Ctrl Pts',(42.3331766671028,-57.9577588828693,0.));
#62082=CARTESIAN_POINT('Ctrl Pts',(42.3526756908764,-57.9710768845923,0.));
#62083=CARTESIAN_POINT('Ctrl Pts',(42.3722235179216,-57.9844000273936,0.));
#62084=CARTESIAN_POINT('Ctrl Pts',(42.3918200813025,-57.9977281894437,0.));
#62085=CARTESIAN_POINT('Ctrl Pts',(42.4114653142891,-58.011061249483,0.));
#62086=CARTESIAN_POINT('Ctrl Pts',(42.4311591503551,-58.0243990868175,0.));
#62087=CARTESIAN_POINT('Ctrl Pts',(42.4509015231668,-58.0377415813132,0.));
#62088=CARTESIAN_POINT('Ctrl Pts',(42.4706923665838,-58.0510886133917,0.));
#62089=CARTESIAN_POINT('Ctrl Pts',(42.490531614665,-58.064440064027,0.));
#62090=CARTESIAN_POINT('Ctrl Pts',(42.5104192016664,-58.0777958147404,0.));
#62091=CARTESIAN_POINT('Ctrl Pts',(42.5303550620388,-58.0911557475967,0.));
#62092=CARTESIAN_POINT('Ctrl Pts',(42.5503391304183,-58.1045197452003,0.));
#62093=CARTESIAN_POINT('Ctrl Pts',(42.5703713416263,-58.1178876906905,0.));
#62094=CARTESIAN_POINT('Ctrl Pts',(42.5904516306759,-58.1312594677383,0.));
#62095=CARTESIAN_POINT('Ctrl Pts',(42.6105799327697,-58.1446349605419,0.));
#62096=CARTESIAN_POINT('Ctrl Pts',(42.6307561832978,-58.158014053823,0.));
#62097=CARTESIAN_POINT('Ctrl Pts',(42.650980317827,-58.1713966328217,0.));
#62098=CARTESIAN_POINT('Ctrl Pts',(42.6712522721021,-58.1847825832932,0.));
#62099=CARTESIAN_POINT('Ctrl Pts',(42.6915719820517,-58.1981717915043,0.));
#62100=CARTESIAN_POINT('Ctrl Pts',(42.7119393837867,-58.2115641442302,0.));
#62101=CARTESIAN_POINT('Ctrl Pts',(42.7323544135983,-58.2249595287497,0.));
#62102=CARTESIAN_POINT('Ctrl Pts',(42.7528170079482,-58.238357832842,0.));
#62103=CARTESIAN_POINT('Ctrl Pts',(42.7733271034679,-58.2517589447818,0.));
#62104=CARTESIAN_POINT('Ctrl Pts',(42.7938846369651,-58.2651627533368,0.));
#62105=CARTESIAN_POINT('Ctrl Pts',(42.8144895454234,-58.278569147764,0.));
#62106=CARTESIAN_POINT('Ctrl Pts',(42.8351417659998,-58.2919780178063,0.));
#62107=CARTESIAN_POINT('Ctrl Pts',(42.8558412360154,-58.305389253689,0.));
#62108=CARTESIAN_POINT('Ctrl Pts',(42.8765878929545,-58.3188027461157,0.));
#62109=CARTESIAN_POINT('Ctrl Pts',(42.8973816744703,-58.3322183862647,0.));
#62110=CARTESIAN_POINT('Ctrl Pts',(42.9182225183851,-58.3456360657861,0.));
#62111=CARTESIAN_POINT('Ctrl Pts',(42.9391103626881,-58.3590556767981,0.));
#62112=CARTESIAN_POINT('Ctrl Pts',(42.9600451455267,-58.3724771118835,0.));
#62113=CARTESIAN_POINT('Ctrl Pts',(42.9810268052043,-58.3859002640871,0.));
#62114=CARTESIAN_POINT('Ctrl Pts',(43.002055280187,-58.3993250269115,0.));
#62115=CARTESIAN_POINT('Ctrl Pts',(43.0231305091033,-58.4127512943144,0.));
#62116=CARTESIAN_POINT('Ctrl Pts',(43.0442524307432,-58.4261789607055,0.));
#62117=CARTESIAN_POINT('Ctrl Pts',(43.0654209840502,-58.4396079209438,0.));
#62118=CARTESIAN_POINT('Ctrl Pts',(43.0866361081166,-58.4530380703335,0.));
#62119=CARTESIAN_POINT('Ctrl Pts',(43.1078977421908,-58.4664693046206,0.));
#62120=CARTESIAN_POINT('Ctrl Pts',(43.1292058256774,-58.4799015199904,0.));
#62121=CARTESIAN_POINT('Ctrl Pts',(43.1505602981366,-58.4933346130638,0.));
#62122=CARTESIAN_POINT('Ctrl Pts',(43.1719610992772,-58.5067684808946,0.));
#62123=CARTESIAN_POINT('Ctrl Pts',(43.1934081689504,-58.5202030209667,0.));
#62124=CARTESIAN_POINT('Ctrl Pts',(43.214901447157,-58.5336381311911,0.));
#62125=CARTESIAN_POINT('Ctrl Pts',(43.2364408740489,-58.5470737099027,0.));
#62126=CARTESIAN_POINT('Ctrl Pts',(43.2580263899278,-58.5605096558578,0.));
#62127=CARTESIAN_POINT('Ctrl Pts',(43.2796579352405,-58.5739458682317,0.));
#62128=CARTESIAN_POINT('Ctrl Pts',(43.3013354505708,-58.5873822466163,0.));
#62129=CARTESIAN_POINT('Ctrl Pts',(43.3230588766456,-58.6008186910166,0.));
#62130=CARTESIAN_POINT('Ctrl Pts',(43.3448281543375,-58.6142551018473,0.));
#62131=CARTESIAN_POINT('Ctrl Pts',(43.3666432246635,-58.627691379929,0.));
#62132=CARTESIAN_POINT('Ctrl Pts',(43.3885040287808,-58.6411274264854,0.));
#62133=CARTESIAN_POINT('Ctrl Pts',(43.4104105079766,-58.6545631431388,0.));
#62134=CARTESIAN_POINT('Ctrl Pts',(43.4323626036736,-58.6679984319095,0.));
#62135=CARTESIAN_POINT('Ctrl Pts',(43.4543602574352,-58.6814331952138,0.));
#62136=CARTESIAN_POINT('Ctrl Pts',(43.4764034109655,-58.6948673358639,0.));
#62137=CARTESIAN_POINT('Ctrl Pts',(43.4984920061071,-58.708300757066,0.));
#62138=CARTESIAN_POINT('Ctrl Pts',(43.5206259848333,-58.7217333624206,0.));
#62139=CARTESIAN_POINT('Ctrl Pts',(43.5428052892483,-58.7351650559176,0.));
#62140=CARTESIAN_POINT('Ctrl Pts',(43.5650298615912,-58.7485957419296,0.));
#62141=CARTESIAN_POINT('Ctrl Pts',(43.5872996442343,-58.7620253252059,0.));
#62142=CARTESIAN_POINT('Ctrl Pts',(43.6096145796798,-58.7754537108672,0.));
#62143=CARTESIAN_POINT('Ctrl Pts',(43.6319746105488,-58.7888808043976,0.));
#62144=CARTESIAN_POINT('Ctrl Pts',(43.6543796795797,-58.8023065116446,0.));
#62145=CARTESIAN_POINT('Ctrl Pts',(43.6768297296403,-58.8157307388247,0.));
#62146=CARTESIAN_POINT('Ctrl Pts',(43.6993247037318,-58.8291533925299,0.));
#62147=CARTESIAN_POINT('Ctrl Pts',(43.7218645449921,-58.8425743797325,0.));
#62148=CARTESIAN_POINT('Ctrl Pts',(43.7444491966935,-58.8559936077933,0.));
#62149=CARTESIAN_POINT('Ctrl Pts',(43.7670786022392,-58.8694109844636,0.));
#62150=CARTESIAN_POINT('Ctrl Pts',(43.7897527051599,-58.882826417861,0.));
#62151=CARTESIAN_POINT('Ctrl Pts',(43.812471449107,-58.8962398164486,0.));
#62152=CARTESIAN_POINT('Ctrl Pts',(43.8352347778419,-58.9096510890128,0.));
#62153=CARTESIAN_POINT('Ctrl Pts',(43.8580426352236,-58.9230601446445,0.));
#62154=CARTESIAN_POINT('Ctrl Pts',(43.8808949651882,-58.9364668927132,0.));
#62155=CARTESIAN_POINT('Ctrl Pts',(43.9037917117749,-58.9498712429066,0.));
#62156=CARTESIAN_POINT('Ctrl Pts',(43.9267328191508,-58.9632731052704,0.));
#62157=CARTESIAN_POINT('Ctrl Pts',(43.9497182316333,-58.9766723902531,0.));
#62158=CARTESIAN_POINT('Ctrl Pts',(43.9727478937053,-58.9900690087404,0.));
#62159=CARTESIAN_POINT('Ctrl Pts',(43.9958217500364,-59.0034628721161,0.));
#62160=CARTESIAN_POINT('Ctrl Pts',(44.0189397454593,-59.0168538922087,0.));
#62161=CARTESIAN_POINT('Ctrl Pts',(44.0421018249219,-59.0302419811772,0.));
#62162=CARTESIAN_POINT('Ctrl Pts',(44.0653079334384,-59.0436270514085,0.));
#62163=CARTESIAN_POINT('Ctrl Pts',(44.0885580160433,-59.0570090154243,0.));
#62164=CARTESIAN_POINT('Ctrl Pts',(44.1118520177224,-59.0703877857529,0.));
#62165=CARTESIAN_POINT('Ctrl Pts',(44.1351898834057,-59.0837632749209,0.));
#62166=CARTESIAN_POINT('Ctrl Pts',(44.1585715581074,-59.0971353957218,0.));
#62167=CARTESIAN_POINT('Ctrl Pts',(44.1819969870314,-59.1105040614285,0.));
#62168=CARTESIAN_POINT('Ctrl Pts',(44.2054661156876,-59.1238691860307,0.));
#62169=CARTESIAN_POINT('Ctrl Pts',(44.2289788899962,-59.1372306844575,0.));
#62170=CARTESIAN_POINT('Ctrl Pts',(44.2525352563979,-59.1505884728194,0.));
#62171=CARTESIAN_POINT('Ctrl Pts',(44.2761351616027,-59.1639424678766,0.));
#62172=CARTESIAN_POINT('Ctrl Pts',(44.2997785523413,-59.1772925865191,0.));
#62173=CARTESIAN_POINT('Ctrl Pts',(44.3234653750877,-59.1906387451971,0.));
#62174=CARTESIAN_POINT('Ctrl Pts',(44.3471955758412,-59.2039808594765,0.));
#62175=CARTESIAN_POINT('Ctrl Pts',(44.3709690997495,-59.217318843283,0.));
#62176=CARTESIAN_POINT('Ctrl Pts',(44.394785891411,-59.2306526095175,0.));
#62177=CARTESIAN_POINT('Ctrl Pts',(44.4186458955486,-59.2439820714231,0.));
#62178=CARTESIAN_POINT('Ctrl Pts',(44.4425490575932,-59.2573071437801,0.));
#62179=CARTESIAN_POINT('Ctrl Pts',(44.4664953242373,-59.2706277440438,0.));
#62180=CARTESIAN_POINT('Ctrl Pts',(44.490484644147,-59.2839437938187,0.));
#62181=CARTESIAN_POINT('Ctrl Pts',(44.514516968128,-59.2972552192072,0.));
#62182=CARTESIAN_POINT('Ctrl Pts',(44.5351541478336,-59.3086616639392,0.));
#62183=CARTESIAN_POINT('Ctrl Pts',(44.5509994357954,-59.317404187219,0.));
#62184=CARTESIAN_POINT('Ctrl Pts',(44.5620338188487,-59.3234848865279,0.));
#62185=CARTESIAN_POINT('Ctrl Pts',(44.5682447395714,-59.3269051738223,0.));
#62186=CARTESIAN_POINT('Ctrl Pts',(44.5696260757422,-59.3276657444159,0.));
#62187=CARTESIAN_POINT('',(40.8467768343956,-56.8466430164621,12.));
#62188=CARTESIAN_POINT('',(40.8467768343956,-56.8466430164621,0.));
#62189=CARTESIAN_POINT('Ctrl Pts',(44.5696260757422,-59.3276657444159,12.));
#62190=CARTESIAN_POINT('Ctrl Pts',(44.5682447395714,-59.3269051738223,12.));
#62191=CARTESIAN_POINT('Ctrl Pts',(44.5620338188486,-59.3234848865279,12.));
#62192=CARTESIAN_POINT('Ctrl Pts',(44.5509994357954,-59.317404187219,12.));
#62193=CARTESIAN_POINT('Ctrl Pts',(44.5351541478336,-59.3086616639392,12.));
#62194=CARTESIAN_POINT('Ctrl Pts',(44.514516968128,-59.2972552192072,12.));
#62195=CARTESIAN_POINT('Ctrl Pts',(44.490484644147,-59.2839437938187,12.));
#62196=CARTESIAN_POINT('Ctrl Pts',(44.4664953242373,-59.2706277440438,12.));
#62197=CARTESIAN_POINT('Ctrl Pts',(44.4425490575932,-59.2573071437801,12.));
#62198=CARTESIAN_POINT('Ctrl Pts',(44.4186458955486,-59.2439820714231,12.));
#62199=CARTESIAN_POINT('Ctrl Pts',(44.394785891411,-59.2306526095175,12.));
#62200=CARTESIAN_POINT('Ctrl Pts',(44.3709690997495,-59.217318843283,12.));
#62201=CARTESIAN_POINT('Ctrl Pts',(44.3471955758412,-59.2039808594765,12.));
#62202=CARTESIAN_POINT('Ctrl Pts',(44.3234653750877,-59.1906387451971,12.));
#62203=CARTESIAN_POINT('Ctrl Pts',(44.2997785523413,-59.1772925865191,12.));
#62204=CARTESIAN_POINT('Ctrl Pts',(44.2761351616027,-59.1639424678766,12.));
#62205=CARTESIAN_POINT('Ctrl Pts',(44.2525352563979,-59.1505884728194,12.));
#62206=CARTESIAN_POINT('Ctrl Pts',(44.2289788899962,-59.1372306844575,12.));
#62207=CARTESIAN_POINT('Ctrl Pts',(44.2054661156876,-59.1238691860307,12.));
#62208=CARTESIAN_POINT('Ctrl Pts',(44.1819969870314,-59.1105040614285,12.));
#62209=CARTESIAN_POINT('Ctrl Pts',(44.1585715581074,-59.0971353957218,12.));
#62210=CARTESIAN_POINT('Ctrl Pts',(44.1351898834057,-59.0837632749209,12.));
#62211=CARTESIAN_POINT('Ctrl Pts',(44.1118520177224,-59.0703877857529,12.));
#62212=CARTESIAN_POINT('Ctrl Pts',(44.0885580160433,-59.0570090154243,12.));
#62213=CARTESIAN_POINT('Ctrl Pts',(44.0653079334384,-59.0436270514085,12.));
#62214=CARTESIAN_POINT('Ctrl Pts',(44.0421018249219,-59.0302419811772,12.));
#62215=CARTESIAN_POINT('Ctrl Pts',(44.0189397454593,-59.0168538922087,12.));
#62216=CARTESIAN_POINT('Ctrl Pts',(43.9958217500364,-59.0034628721161,12.));
#62217=CARTESIAN_POINT('Ctrl Pts',(43.9727478937053,-58.9900690087404,12.));
#62218=CARTESIAN_POINT('Ctrl Pts',(43.9497182316333,-58.9766723902531,12.));
#62219=CARTESIAN_POINT('Ctrl Pts',(43.9267328191508,-58.9632731052704,12.));
#62220=CARTESIAN_POINT('Ctrl Pts',(43.9037917117749,-58.9498712429066,12.));
#62221=CARTESIAN_POINT('Ctrl Pts',(43.8808949651882,-58.9364668927132,12.));
#62222=CARTESIAN_POINT('Ctrl Pts',(43.8580426352236,-58.9230601446445,12.));
#62223=CARTESIAN_POINT('Ctrl Pts',(43.8352347778419,-58.9096510890128,12.));
#62224=CARTESIAN_POINT('Ctrl Pts',(43.812471449107,-58.8962398164486,12.));
#62225=CARTESIAN_POINT('Ctrl Pts',(43.7897527051599,-58.882826417861,12.));
#62226=CARTESIAN_POINT('Ctrl Pts',(43.7670786022392,-58.8694109844636,12.));
#62227=CARTESIAN_POINT('Ctrl Pts',(43.7444491966935,-58.8559936077933,12.));
#62228=CARTESIAN_POINT('Ctrl Pts',(43.7218645449921,-58.8425743797325,12.));
#62229=CARTESIAN_POINT('Ctrl Pts',(43.6993247037318,-58.8291533925299,12.));
#62230=CARTESIAN_POINT('Ctrl Pts',(43.6768297296403,-58.8157307388247,12.));
#62231=CARTESIAN_POINT('Ctrl Pts',(43.6543796795797,-58.8023065116446,12.));
#62232=CARTESIAN_POINT('Ctrl Pts',(43.6319746105488,-58.7888808043976,12.));
#62233=CARTESIAN_POINT('Ctrl Pts',(43.6096145796798,-58.7754537108672,12.));
#62234=CARTESIAN_POINT('Ctrl Pts',(43.5872996442343,-58.7620253252059,12.));
#62235=CARTESIAN_POINT('Ctrl Pts',(43.5650298615912,-58.7485957419296,12.));
#62236=CARTESIAN_POINT('Ctrl Pts',(43.5428052892483,-58.7351650559176,12.));
#62237=CARTESIAN_POINT('Ctrl Pts',(43.5206259848333,-58.7217333624206,12.));
#62238=CARTESIAN_POINT('Ctrl Pts',(43.4984920061071,-58.708300757066,12.));
#62239=CARTESIAN_POINT('Ctrl Pts',(43.4764034109655,-58.6948673358639,12.));
#62240=CARTESIAN_POINT('Ctrl Pts',(43.4543602574352,-58.6814331952138,12.));
#62241=CARTESIAN_POINT('Ctrl Pts',(43.4323626036736,-58.6679984319095,12.));
#62242=CARTESIAN_POINT('Ctrl Pts',(43.4104105079766,-58.6545631431388,12.));
#62243=CARTESIAN_POINT('Ctrl Pts',(43.3885040287808,-58.6411274264854,12.));
#62244=CARTESIAN_POINT('Ctrl Pts',(43.3666432246635,-58.627691379929,12.));
#62245=CARTESIAN_POINT('Ctrl Pts',(43.3448281543375,-58.6142551018473,12.));
#62246=CARTESIAN_POINT('Ctrl Pts',(43.3230588766456,-58.6008186910166,12.));
#62247=CARTESIAN_POINT('Ctrl Pts',(43.3013354505708,-58.5873822466163,12.));
#62248=CARTESIAN_POINT('Ctrl Pts',(43.2796579352405,-58.5739458682317,12.));
#62249=CARTESIAN_POINT('Ctrl Pts',(43.2580263899278,-58.5605096558578,12.));
#62250=CARTESIAN_POINT('Ctrl Pts',(43.2364408740489,-58.5470737099027,12.));
#62251=CARTESIAN_POINT('Ctrl Pts',(43.214901447157,-58.5336381311911,12.));
#62252=CARTESIAN_POINT('Ctrl Pts',(43.1934081689504,-58.5202030209667,12.));
#62253=CARTESIAN_POINT('Ctrl Pts',(43.1719610992772,-58.5067684808946,12.));
#62254=CARTESIAN_POINT('Ctrl Pts',(43.1505602981366,-58.4933346130638,12.));
#62255=CARTESIAN_POINT('Ctrl Pts',(43.1292058256774,-58.4799015199904,12.));
#62256=CARTESIAN_POINT('Ctrl Pts',(43.1078977421908,-58.4664693046206,12.));
#62257=CARTESIAN_POINT('Ctrl Pts',(43.0866361081166,-58.4530380703335,12.));
#62258=CARTESIAN_POINT('Ctrl Pts',(43.0654209840502,-58.4396079209438,12.));
#62259=CARTESIAN_POINT('Ctrl Pts',(43.0442524307432,-58.4261789607055,12.));
#62260=CARTESIAN_POINT('Ctrl Pts',(43.0231305091033,-58.4127512943144,12.));
#62261=CARTESIAN_POINT('Ctrl Pts',(43.002055280187,-58.3993250269115,12.));
#62262=CARTESIAN_POINT('Ctrl Pts',(42.9810268052043,-58.3859002640871,12.));
#62263=CARTESIAN_POINT('Ctrl Pts',(42.9600451455267,-58.3724771118835,12.));
#62264=CARTESIAN_POINT('Ctrl Pts',(42.9391103626881,-58.3590556767981,12.));
#62265=CARTESIAN_POINT('Ctrl Pts',(42.9182225183851,-58.3456360657861,12.));
#62266=CARTESIAN_POINT('Ctrl Pts',(42.8973816744703,-58.3322183862647,12.));
#62267=CARTESIAN_POINT('Ctrl Pts',(42.8765878929545,-58.3188027461157,12.));
#62268=CARTESIAN_POINT('Ctrl Pts',(42.8558412360154,-58.305389253689,12.));
#62269=CARTESIAN_POINT('Ctrl Pts',(42.8351417659998,-58.2919780178063,12.));
#62270=CARTESIAN_POINT('Ctrl Pts',(42.8144895454234,-58.278569147764,12.));
#62271=CARTESIAN_POINT('Ctrl Pts',(42.7938846369651,-58.2651627533368,12.));
#62272=CARTESIAN_POINT('Ctrl Pts',(42.7733271034679,-58.2517589447818,12.));
#62273=CARTESIAN_POINT('Ctrl Pts',(42.7528170079482,-58.238357832842,12.));
#62274=CARTESIAN_POINT('Ctrl Pts',(42.7323544135983,-58.2249595287497,12.));
#62275=CARTESIAN_POINT('Ctrl Pts',(42.7119393837867,-58.2115641442302,12.));
#62276=CARTESIAN_POINT('Ctrl Pts',(42.6915719820517,-58.1981717915043,12.));
#62277=CARTESIAN_POINT('Ctrl Pts',(42.6712522721021,-58.1847825832932,12.));
#62278=CARTESIAN_POINT('Ctrl Pts',(42.650980317827,-58.1713966328217,12.));
#62279=CARTESIAN_POINT('Ctrl Pts',(42.6307561832978,-58.158014053823,12.));
#62280=CARTESIAN_POINT('Ctrl Pts',(42.6105799327697,-58.1446349605419,12.));
#62281=CARTESIAN_POINT('Ctrl Pts',(42.5904516306759,-58.1312594677383,12.));
#62282=CARTESIAN_POINT('Ctrl Pts',(42.5703713416263,-58.1178876906905,12.));
#62283=CARTESIAN_POINT('Ctrl Pts',(42.5503391304183,-58.1045197452003,12.));
#62284=CARTESIAN_POINT('Ctrl Pts',(42.5303550620388,-58.0911557475967,12.));
#62285=CARTESIAN_POINT('Ctrl Pts',(42.5104192016664,-58.0777958147404,12.));
#62286=CARTESIAN_POINT('Ctrl Pts',(42.490531614665,-58.064440064027,12.));
#62287=CARTESIAN_POINT('Ctrl Pts',(42.4706923665838,-58.0510886133917,12.));
#62288=CARTESIAN_POINT('Ctrl Pts',(42.4509015231668,-58.0377415813132,12.));
#62289=CARTESIAN_POINT('Ctrl Pts',(42.4311591503551,-58.0243990868175,12.));
#62290=CARTESIAN_POINT('Ctrl Pts',(42.4114653142891,-58.011061249483,12.));
#62291=CARTESIAN_POINT('Ctrl Pts',(42.3918200813025,-57.9977281894437,12.));
#62292=CARTESIAN_POINT('Ctrl Pts',(42.3722235179216,-57.9844000273936,12.));
#62293=CARTESIAN_POINT('Ctrl Pts',(42.3526756908764,-57.9710768845923,12.));
#62294=CARTESIAN_POINT('Ctrl Pts',(42.3331766671028,-57.9577588828693,12.));
#62295=CARTESIAN_POINT('Ctrl Pts',(42.3137265137446,-57.9444461446292,12.));
#62296=CARTESIAN_POINT('Ctrl Pts',(42.2943252981471,-57.9311387928541,12.));
#62297=CARTESIAN_POINT('Ctrl Pts',(42.274973087857,-57.9178369511084,12.));
#62298=CARTESIAN_POINT('Ctrl Pts',(42.2556699506332,-57.9045407435447,12.));
#62299=CARTESIAN_POINT('Ctrl Pts',(42.2364159544492,-57.8912502949084,12.));
#62300=CARTESIAN_POINT('Ctrl Pts',(42.2172111674946,-57.8779657305422,12.));
#62301=CARTESIAN_POINT('Ctrl Pts',(42.1980556581689,-57.86468717639,12.));
#62302=CARTESIAN_POINT('Ctrl Pts',(42.1789494950824,-57.8514147590012,12.));
#62303=CARTESIAN_POINT('Ctrl Pts',(42.1598927470671,-57.8381486055376,12.));
#62304=CARTESIAN_POINT('Ctrl Pts',(42.1408854831792,-57.8248888437787,12.));
#62305=CARTESIAN_POINT('Ctrl Pts',(42.121927772701,-57.8116356021274,12.));
#62306=CARTESIAN_POINT('Ctrl Pts',(42.1030196851344,-57.798389009613,12.));
#62307=CARTESIAN_POINT('Ctrl Pts',(42.0841612902018,-57.7851491958954,12.));
#62308=CARTESIAN_POINT('Ctrl Pts',(42.0653526578571,-57.7719162912721,12.));
#62309=CARTESIAN_POINT('Ctrl Pts',(42.0465938582878,-57.7586904266828,12.));
#62310=CARTESIAN_POINT('Ctrl Pts',(42.0278849619156,-57.7454717337151,12.));
#62311=CARTESIAN_POINT('Ctrl Pts',(42.0092260393911,-57.7322603446086,12.));
#62312=CARTESIAN_POINT('Ctrl Pts',(41.9906171615975,-57.7190563922614,12.));
#62313=CARTESIAN_POINT('Ctrl Pts',(41.9720583996601,-57.7058600102365,12.));
#62314=CARTESIAN_POINT('Ctrl Pts',(41.9535498249489,-57.6926713327674,12.));
#62315=CARTESIAN_POINT('Ctrl Pts',(41.9350915090791,-57.6794904947641,12.));
#62316=CARTESIAN_POINT('Ctrl Pts',(41.9166835239046,-57.6663176318176,12.));
#62317=CARTESIAN_POINT('Ctrl Pts',(41.8983259415245,-57.6531528802059,12.));
#62318=CARTESIAN_POINT('Ctrl Pts',(41.8800188342909,-57.6399963769003,12.));
#62319=CARTESIAN_POINT('Ctrl Pts',(41.8617622748108,-57.6268482595702,12.));
#62320=CARTESIAN_POINT('Ctrl Pts',(41.8435563359456,-57.6137086665882,12.));
#62321=CARTESIAN_POINT('Ctrl Pts',(41.8254010908051,-57.6005777370349,12.));
#62322=CARTESIAN_POINT('Ctrl Pts',(41.8072966127558,-57.5874556107056,12.));
#62323=CARTESIAN_POINT('Ctrl Pts',(41.7892429754297,-57.5743424281204,12.));
#62324=CARTESIAN_POINT('Ctrl Pts',(41.7712402527273,-57.561238330532,12.));
#62325=CARTESIAN_POINT('Ctrl Pts',(41.7532885188175,-57.5481434599335,12.));
#62326=CARTESIAN_POINT('Ctrl Pts',(41.7353878481337,-57.5350579590649,12.));
#62327=CARTESIAN_POINT('Ctrl Pts',(41.7175383153821,-57.5219819714171,12.));
#62328=CARTESIAN_POINT('Ctrl Pts',(41.6997399955447,-57.5089156412343,12.));
#62329=CARTESIAN_POINT('Ctrl Pts',(41.6819929638797,-57.4958591135165,12.));
#62330=CARTESIAN_POINT('Ctrl Pts',(41.6642972959165,-57.4828125340218,12.));
#62331=CARTESIAN_POINT('Ctrl Pts',(41.6466530674515,-57.4697760492683,12.));
#62332=CARTESIAN_POINT('Ctrl Pts',(41.6290603545666,-57.4567498065562,12.));
#62333=CARTESIAN_POINT('Ctrl Pts',(41.6115192336388,-57.4437339539841,12.));
#62334=CARTESIAN_POINT('Ctrl Pts',(41.5940297813477,-57.4307286404662,12.));
#62335=CARTESIAN_POINT('Ctrl Pts',(41.5765920746777,-57.4177340157508,12.));
#62336=CARTESIAN_POINT('Ctrl Pts',(41.5592061909176,-57.4047502304231,12.));
#62337=CARTESIAN_POINT('Ctrl Pts',(41.5418722076572,-57.3917774358863,12.));
#62338=CARTESIAN_POINT('Ctrl Pts',(41.5245902027771,-57.3788157843454,12.));
#62339=CARTESIAN_POINT('Ctrl Pts',(41.5073602544396,-57.3658654287937,12.));
#62340=CARTESIAN_POINT('Ctrl Pts',(41.4901824410637,-57.3529265229835,12.));
#62341=CARTESIAN_POINT('Ctrl Pts',(41.4730568413518,-57.3399992214717,12.));
#62342=CARTESIAN_POINT('Ctrl Pts',(41.4559835343328,-57.3270836796911,12.));
#62343=CARTESIAN_POINT('Ctrl Pts',(41.4389625993948,-57.3141800540137,12.));
#62344=CARTESIAN_POINT('Ctrl Pts',(41.4219941163163,-57.3012885018151,12.));
#62345=CARTESIAN_POINT('Ctrl Pts',(41.4050781652938,-57.2884091815406,12.));
#62346=CARTESIAN_POINT('Ctrl Pts',(41.3882148268814,-57.2755422525844,12.));
#62347=CARTESIAN_POINT('Ctrl Pts',(41.3714041819224,-57.2626878751596,12.));
#62348=CARTESIAN_POINT('Ctrl Pts',(41.3546463114885,-57.2498462101879,12.));
#62349=CARTESIAN_POINT('Ctrl Pts',(41.3379412967875,-57.2370174191401,12.));
#62350=CARTESIAN_POINT('Ctrl Pts',(41.321289219149,-57.2242016640198,12.));
#62351=CARTESIAN_POINT('Ctrl Pts',(41.3046901602293,-57.2113991077302,12.));
#62352=CARTESIAN_POINT('Ctrl Pts',(41.2881442021863,-57.1986099143983,12.));
#62353=CARTESIAN_POINT('Ctrl Pts',(41.2716514278276,-57.1858342496538,12.));
#62354=CARTESIAN_POINT('Ctrl Pts',(41.2552119208466,-57.17307228108,12.));
#62355=CARTESIAN_POINT('Ctrl Pts',(41.2388257656559,-57.1603241779077,12.));
#62356=CARTESIAN_POINT('Ctrl Pts',(41.222493046943,-57.147590110182,12.));
#62357=CARTESIAN_POINT('Ctrl Pts',(41.2062138492915,-57.1348702480647,12.));
#62358=CARTESIAN_POINT('Ctrl Pts',(41.1899882567923,-57.1221647611207,12.));
#62359=CARTESIAN_POINT('Ctrl Pts',(41.1738163525902,-57.1094738174957,12.));
#62360=CARTESIAN_POINT('Ctrl Pts',(41.1576982197375,-57.0967975854874,12.));
#62361=CARTESIAN_POINT('Ctrl Pts',(41.1416339422117,-57.084136235426,12.));
#62362=CARTESIAN_POINT('Ctrl Pts',(41.1256236057443,-57.0714899412099,12.));
#62363=CARTESIAN_POINT('Ctrl Pts',(41.1096672990148,-57.0588588825298,12.));
#62364=CARTESIAN_POINT('Ctrl Pts',(41.0937651137549,-57.046243245068,12.));
#62365=CARTESIAN_POINT('Ctrl Pts',(41.0779171422438,-57.0336432158536,12.));
#62366=CARTESIAN_POINT('Ctrl Pts',(41.0621234751007,-57.0210589791788,12.));
#62367=CARTESIAN_POINT('Ctrl Pts',(41.0463841993608,-57.008490713042,12.));
#62368=CARTESIAN_POINT('Ctrl Pts',(41.0306993953989,-56.995938583472,12.));
#62369=CARTESIAN_POINT('Ctrl Pts',(41.0150691398947,-56.9834027500117,12.));
#62370=CARTESIAN_POINT('Ctrl Pts',(40.9994935117276,-56.9708833766137,12.));
#62371=CARTESIAN_POINT('Ctrl Pts',(40.9839725967121,-56.9583806404069,12.));
#62372=CARTESIAN_POINT('Ctrl Pts',(40.9685064933074,-56.9458947422608,12.));
#62373=CARTESIAN_POINT('Ctrl Pts',(40.9530953165031,-56.9334259140049,12.));
#62374=CARTESIAN_POINT('Ctrl Pts',(40.9377391857129,-56.9209743960992,12.));
#62375=CARTESIAN_POINT('Ctrl Pts',(40.9224382132427,-56.9085404164502,12.));
#62376=CARTESIAN_POINT('Ctrl Pts',(40.9071924937508,-56.8961241708861,12.));
#62377=CARTESIAN_POINT('Ctrl Pts',(40.8920020903293,-56.8837257978343,12.));
#62378=CARTESIAN_POINT('Ctrl Pts',(40.8768670342052,-56.8713453764905,12.));
#62379=CARTESIAN_POINT('Ctrl Pts',(40.864803275942,-56.8614554317668,12.));
#62380=CARTESIAN_POINT('Ctrl Pts',(40.8557803680278,-56.8540460739472,12.));
#62381=CARTESIAN_POINT('Ctrl Pts',(40.8497761671036,-56.8491101022591,12.));
#62382=CARTESIAN_POINT('Ctrl Pts',(40.8467768343956,-56.8466430164621,12.));
#62383=CARTESIAN_POINT('Ctrl Pts',(45.7706564944895,-58.4060826907792,-5.55111512312578E-16));
#62384=CARTESIAN_POINT('Ctrl Pts',(45.7706564944895,-58.4060826907792,4.));
#62385=CARTESIAN_POINT('Ctrl Pts',(45.7706564944895,-58.4060826907792,8.));
#62386=CARTESIAN_POINT('Ctrl Pts',(45.7706564944895,-58.4060826907792,12.));
#62387=CARTESIAN_POINT('Ctrl Pts',(45.7969367893064,-58.5127761886842,-5.55111512312578E-16));
#62388=CARTESIAN_POINT('Ctrl Pts',(45.7969367893064,-58.5127761886842,4.));
#62389=CARTESIAN_POINT('Ctrl Pts',(45.7969367893065,-58.5127761886843,8.00000000000001));
#62390=CARTESIAN_POINT('Ctrl Pts',(45.7969367893065,-58.5127761886843,12.));
#62391=CARTESIAN_POINT('Ctrl Pts',(45.7788617791412,-58.7146322050558,-5.55111512312578E-16));
#62392=CARTESIAN_POINT('Ctrl Pts',(45.7788617791412,-58.7146322050558,4.));
#62393=CARTESIAN_POINT('Ctrl Pts',(45.7788617791413,-58.7146322050559,7.99999999999999));
#62394=CARTESIAN_POINT('Ctrl Pts',(45.7788617791413,-58.7146322050559,12.));
#62395=CARTESIAN_POINT('Ctrl Pts',(45.6563266621664,-58.870677144318,-5.55111512312578E-16));
#62396=CARTESIAN_POINT('Ctrl Pts',(45.6563266621664,-58.870677144318,4.));
#62397=CARTESIAN_POINT('Ctrl Pts',(45.6563266621664,-58.870677144318,8.00000000000001));
#62398=CARTESIAN_POINT('Ctrl Pts',(45.6563266621664,-58.870677144318,12.));
#62399=CARTESIAN_POINT('Ctrl Pts',(45.5911481700253,-58.9211100416379,-5.55111512312578E-16));
#62400=CARTESIAN_POINT('Ctrl Pts',(45.5911481700253,-58.9211100416379,4.));
#62401=CARTESIAN_POINT('Ctrl Pts',(45.5911481700253,-58.9211100416379,8.));
#62402=CARTESIAN_POINT('Ctrl Pts',(45.5911481700253,-58.9211100416379,12.));
#62403=CARTESIAN_POINT('',(45.7706564944895,-58.4060826907792,2.77555756156289E-16));
#62404=CARTESIAN_POINT('',(45.5911481700253,-58.9211100416379,0.));
#62405=CARTESIAN_POINT('Ctrl Pts',(45.7706564944895,-58.4060826907792,-1.38777878078145E-16));
#62406=CARTESIAN_POINT('Ctrl Pts',(45.7969367893064,-58.5127761886842,-1.38777878078145E-16));
#62407=CARTESIAN_POINT('Ctrl Pts',(45.7866082120692,-58.6281224837537,-1.38777878078144E-16));
#62408=CARTESIAN_POINT('Ctrl Pts',(45.7421702122002,-58.7285100597671,-1.38777878078145E-16));
#62409=CARTESIAN_POINT('Ctrl Pts',(45.7088417122985,-58.8038007417771,-1.38777878078145E-16));
#62410=CARTESIAN_POINT('Ctrl Pts',(45.6563266621664,-58.870677144318,-1.38777878078145E-16));
#62411=CARTESIAN_POINT('Ctrl Pts',(45.5911481700253,-58.9211100416379,-1.38777878078145E-16));
#62412=CARTESIAN_POINT('',(45.5911481700253,-58.9211100416379,12.));
#62413=CARTESIAN_POINT('Ctrl Pts',(45.5911481700253,-58.9211100416379,-5.55111512312578E-16));
#62414=CARTESIAN_POINT('Ctrl Pts',(45.5911481700253,-58.9211100416379,4.));
#62415=CARTESIAN_POINT('Ctrl Pts',(45.5911481700253,-58.9211100416379,8.));
#62416=CARTESIAN_POINT('Ctrl Pts',(45.5911481700253,-58.9211100416379,12.));
#62417=CARTESIAN_POINT('',(45.7706564944895,-58.4060826907792,12.));
#62418=CARTESIAN_POINT('Ctrl Pts',(45.5911481700253,-58.9211100416379,12.));
#62419=CARTESIAN_POINT('Ctrl Pts',(45.6563266621664,-58.870677144318,12.));
#62420=CARTESIAN_POINT('Ctrl Pts',(45.7088417122985,-58.8038007417771,12.));
#62421=CARTESIAN_POINT('Ctrl Pts',(45.7421702122002,-58.7285100597671,12.));
#62422=CARTESIAN_POINT('Ctrl Pts',(45.7866082120692,-58.6281224837538,12.));
#62423=CARTESIAN_POINT('Ctrl Pts',(45.7969367893065,-58.5127761886843,12.));
#62424=CARTESIAN_POINT('Ctrl Pts',(45.7706564944895,-58.4060826907792,12.));
#62425=CARTESIAN_POINT('Ctrl Pts',(45.7706564944895,-58.4060826907792,12.));
#62426=CARTESIAN_POINT('Ctrl Pts',(45.7706564944895,-58.4060826907792,8.));
#62427=CARTESIAN_POINT('Ctrl Pts',(45.7706564944895,-58.4060826907792,4.));
#62428=CARTESIAN_POINT('Ctrl Pts',(45.7706564944895,-58.4060826907792,-5.55111512312578E-16));
#62429=CARTESIAN_POINT('Origin',(2.28269173065022E-10,-2.97323128204029E-10,
0.));
#62430=CARTESIAN_POINT('Origin',(2.28269173065022E-10,-2.97323128204029E-10,
12.));
#62431=CARTESIAN_POINT('Origin',(2.28269173065022E-10,-2.97323128204029E-10,
0.));
#62432=CARTESIAN_POINT('Ctrl Pts',(39.7746412831502,-62.9938720098767,0.));
#62433=CARTESIAN_POINT('Ctrl Pts',(39.7746412831502,-62.9938720098767,4.));
#62434=CARTESIAN_POINT('Ctrl Pts',(39.7746412831501,-62.9938720098767,8.));
#62435=CARTESIAN_POINT('Ctrl Pts',(39.7746412831501,-62.9938720098767,12.));
#62436=CARTESIAN_POINT('Ctrl Pts',(39.681729578236,-63.0525369183203,0.));
#62437=CARTESIAN_POINT('Ctrl Pts',(39.681729578236,-63.0525369183203,4.));
#62438=CARTESIAN_POINT('Ctrl Pts',(39.6817295782359,-63.0525369183203,8.00000000000001));
#62439=CARTESIAN_POINT('Ctrl Pts',(39.6817295782359,-63.0525369183203,12.));
#62440=CARTESIAN_POINT('Ctrl Pts',(39.4845131830967,-63.0992090147608,-7.30833037966997E-17));
#62441=CARTESIAN_POINT('Ctrl Pts',(39.4845131830967,-63.0992090147608,4.00000000000001));
#62442=CARTESIAN_POINT('Ctrl Pts',(39.4845131830966,-63.0992090147609,7.99999999999999));
#62443=CARTESIAN_POINT('Ctrl Pts',(39.4845131830966,-63.0992090147609,12.));
#62444=CARTESIAN_POINT('Ctrl Pts',(39.2977314459981,-63.0322949727904,-2.46611180233029E-16));
#62445=CARTESIAN_POINT('Ctrl Pts',(39.2977314459981,-63.0322949727904,3.99999999999999));
#62446=CARTESIAN_POINT('Ctrl Pts',(39.2977314459979,-63.0322949727905,8.00000000000001));
#62447=CARTESIAN_POINT('Ctrl Pts',(39.2977314459979,-63.0322949727905,12.));
#62448=CARTESIAN_POINT('Ctrl Pts',(39.2292784191464,-62.9864049293629,-3.30265160470605E-16));
#62449=CARTESIAN_POINT('Ctrl Pts',(39.2292784191464,-62.9864049293629,4.));
#62450=CARTESIAN_POINT('Ctrl Pts',(39.2292784191463,-62.986404929363,8.));
#62451=CARTESIAN_POINT('Ctrl Pts',(39.2292784191463,-62.986404929363,12.));
#62452=CARTESIAN_POINT('',(39.7746412831502,-62.9938720098767,0.));
#62453=CARTESIAN_POINT('',(39.2292784191464,-62.9864049293629,0.));
#62454=CARTESIAN_POINT('Ctrl Pts',(39.7746412831502,-62.9938720098767,2.74425517504384E-17));
#62455=CARTESIAN_POINT('Ctrl Pts',(39.681729578236,-63.0525369183203,2.74425517504384E-17));
#62456=CARTESIAN_POINT('Ctrl Pts',(39.5690344952992,-63.0792066877149,-1.431933613339E-17));
#62457=CARTESIAN_POINT('Ctrl Pts',(39.4597466476411,-63.0687871057916,-8.88794518179137E-17));
#62458=CARTESIAN_POINT('Ctrl Pts',(39.3777807618975,-63.0609724193492,-1.44799538581306E-16));
#62459=CARTESIAN_POINT('Ctrl Pts',(39.2977314459981,-63.0322949727904,-2.1916862848259E-16));
#62460=CARTESIAN_POINT('Ctrl Pts',(39.2292784191464,-62.9864049293629,-3.02822608720167E-16));
#62461=CARTESIAN_POINT('',(39.2292784191464,-62.9864049293629,12.));
#62462=CARTESIAN_POINT('Ctrl Pts',(39.2292784191464,-62.9864049293629,-3.30265160470605E-16));
#62463=CARTESIAN_POINT('Ctrl Pts',(39.2292784191464,-62.9864049293629,4.));
#62464=CARTESIAN_POINT('Ctrl Pts',(39.2292784191463,-62.986404929363,8.));
#62465=CARTESIAN_POINT('Ctrl Pts',(39.2292784191463,-62.986404929363,12.));
#62466=CARTESIAN_POINT('',(39.7746412831501,-62.9938720098767,12.));
#62467=CARTESIAN_POINT('Ctrl Pts',(39.2292784191463,-62.986404929363,12.));
#62468=CARTESIAN_POINT('Ctrl Pts',(39.2977314459979,-63.0322949727905,12.));
#62469=CARTESIAN_POINT('Ctrl Pts',(39.3777807618974,-63.0609724193492,12.));
#62470=CARTESIAN_POINT('Ctrl Pts',(39.459746647641,-63.0687871057917,12.));
#62471=CARTESIAN_POINT('Ctrl Pts',(39.5690344952991,-63.079206687715,12.));
#62472=CARTESIAN_POINT('Ctrl Pts',(39.6817295782359,-63.0525369183203,12.));
#62473=CARTESIAN_POINT('Ctrl Pts',(39.7746412831501,-62.9938720098767,12.));
#62474=CARTESIAN_POINT('Ctrl Pts',(39.7746412831501,-62.9938720098767,12.));
#62475=CARTESIAN_POINT('Ctrl Pts',(39.7746412831501,-62.9938720098767,8.));
#62476=CARTESIAN_POINT('Ctrl Pts',(39.7746412831502,-62.9938720098767,4.));
#62477=CARTESIAN_POINT('Ctrl Pts',(39.7746412831502,-62.9938720098767,0.));
#62478=CARTESIAN_POINT('Ctrl Pts',(35.7368311217509,-60.1903555511633,0.));
#62479=CARTESIAN_POINT('Ctrl Pts',(35.7368311217509,-60.1903555511633,12.));
#62480=CARTESIAN_POINT('Ctrl Pts',(35.7396040203974,-60.1930746580239,0.));
#62481=CARTESIAN_POINT('Ctrl Pts',(35.7396040203974,-60.1930746580239,12.));
#62482=CARTESIAN_POINT('Ctrl Pts',(35.7451551752456,-60.1985151474406,0.));
#62483=CARTESIAN_POINT('Ctrl Pts',(35.7451551752456,-60.1985151474406,12.));
#62484=CARTESIAN_POINT('Ctrl Pts',(35.7534979801871,-60.2066827086579,0.));
#62485=CARTESIAN_POINT('Ctrl Pts',(35.7534979801871,-60.2066827086579,12.));
#62486=CARTESIAN_POINT('Ctrl Pts',(35.7646538667299,-60.2175864449678,0.));
#62487=CARTESIAN_POINT('Ctrl Pts',(35.7646538667299,-60.2175864449678,12.));
#62488=CARTESIAN_POINT('Ctrl Pts',(35.7786523045783,-60.2312388621286,0.));
#62489=CARTESIAN_POINT('Ctrl Pts',(35.7786523045783,-60.2312388621286,12.));
#62490=CARTESIAN_POINT('Ctrl Pts',(35.7927043145165,-60.2449139865206,0.));
#62491=CARTESIAN_POINT('Ctrl Pts',(35.7927043145165,-60.2449139865206,12.));
#62492=CARTESIAN_POINT('Ctrl Pts',(35.8068098723386,-60.2586117365278,0.));
#62493=CARTESIAN_POINT('Ctrl Pts',(35.8068098723386,-60.2586117365278,12.));
#62494=CARTESIAN_POINT('Ctrl Pts',(35.8209689272574,-60.2723319687507,0.));
#62495=CARTESIAN_POINT('Ctrl Pts',(35.8209689272574,-60.2723319687507,12.));
#62496=CARTESIAN_POINT('Ctrl Pts',(35.8351814020424,-60.2860744798563,0.));
#62497=CARTESIAN_POINT('Ctrl Pts',(35.8351814020424,-60.2860744798563,12.));
#62498=CARTESIAN_POINT('Ctrl Pts',(35.8494472046784,-60.2998390330173,0.));
#62499=CARTESIAN_POINT('Ctrl Pts',(35.8494472046784,-60.2998390330173,12.));
#62500=CARTESIAN_POINT('Ctrl Pts',(35.8637662371635,-60.313625378281,0.));
#62501=CARTESIAN_POINT('Ctrl Pts',(35.8637662371635,-60.313625378281,12.));
#62502=CARTESIAN_POINT('Ctrl Pts',(35.878138405151,-60.3274332746781,0.));
#62503=CARTESIAN_POINT('Ctrl Pts',(35.878138405151,-60.3274332746781,12.));
#62504=CARTESIAN_POINT('Ctrl Pts',(35.8925636280633,-60.3412625135223,0.));
#62505=CARTESIAN_POINT('Ctrl Pts',(35.8925636280633,-60.3412625135223,12.));
#62506=CARTESIAN_POINT('Ctrl Pts',(35.9070418358501,-60.3551129108794,0.));
#62507=CARTESIAN_POINT('Ctrl Pts',(35.9070418358501,-60.3551129108794,12.));
#62508=CARTESIAN_POINT('Ctrl Pts',(35.9215729642219,-60.368984296546,0.));
#62509=CARTESIAN_POINT('Ctrl Pts',(35.9215729642219,-60.368984296546,12.));
#62510=CARTESIAN_POINT('Ctrl Pts',(35.9361569506956,-60.3828765049031,0.));
#62511=CARTESIAN_POINT('Ctrl Pts',(35.9361569506956,-60.3828765049031,12.));
#62512=CARTESIAN_POINT('Ctrl Pts',(35.9507937296727,-60.3967893635487,0.));
#62513=CARTESIAN_POINT('Ctrl Pts',(35.9507937296727,-60.3967893635487,12.));
#62514=CARTESIAN_POINT('Ctrl Pts',(35.9654832299627,-60.4107226875759,0.));
#62515=CARTESIAN_POINT('Ctrl Pts',(35.9654832299627,-60.4107226875759,12.));
#62516=CARTESIAN_POINT('Ctrl Pts',(35.9802253773535,-60.424676285496,0.));
#62517=CARTESIAN_POINT('Ctrl Pts',(35.9802253773535,-60.424676285496,12.));
#62518=CARTESIAN_POINT('Ctrl Pts',(35.9950200962175,-60.438649962949,0.));
#62519=CARTESIAN_POINT('Ctrl Pts',(35.9950200962175,-60.438649962949,12.));
#62520=CARTESIAN_POINT('Ctrl Pts',(36.0098673113557,-60.452643526964,0.));
#62521=CARTESIAN_POINT('Ctrl Pts',(36.0098673113557,-60.452643526964,12.));
#62522=CARTESIAN_POINT('Ctrl Pts',(36.0247669500867,-60.4666567908053,0.));
#62523=CARTESIAN_POINT('Ctrl Pts',(36.0247669500867,-60.4666567908053,12.));
#62524=CARTESIAN_POINT('Ctrl Pts',(36.0397189421617,-60.4806895737643,0.));
#62525=CARTESIAN_POINT('Ctrl Pts',(36.0397189421617,-60.4806895737643,12.));
#62526=CARTESIAN_POINT('Ctrl Pts',(36.0547232187682,-60.4947416988396,0.));
#62527=CARTESIAN_POINT('Ctrl Pts',(36.0547232187682,-60.4947416988396,12.));
#62528=CARTESIAN_POINT('Ctrl Pts',(36.0697797118377,-60.5088129911357,0.));
#62529=CARTESIAN_POINT('Ctrl Pts',(36.0697797118377,-60.5088129911357,12.));
#62530=CARTESIAN_POINT('Ctrl Pts',(36.0848883531969,-60.5229032759001,0.));
#62531=CARTESIAN_POINT('Ctrl Pts',(36.0848883531969,-60.5229032759001,12.));
#62532=CARTESIAN_POINT('Ctrl Pts',(36.1000490738532,-60.5370123768841,0.));
#62533=CARTESIAN_POINT('Ctrl Pts',(36.1000490738532,-60.5370123768841,12.));
#62534=CARTESIAN_POINT('Ctrl Pts',(36.1152618043757,-60.5511401172014,0.));
#62535=CARTESIAN_POINT('Ctrl Pts',(36.1152618043757,-60.5511401172014,12.));
#62536=CARTESIAN_POINT('Ctrl Pts',(36.1305264752195,-60.5652863200732,0.));
#62537=CARTESIAN_POINT('Ctrl Pts',(36.1305264752195,-60.5652863200732,12.));
#62538=CARTESIAN_POINT('Ctrl Pts',(36.1458430170425,-60.5794508095555,0.));
#62539=CARTESIAN_POINT('Ctrl Pts',(36.1458430170425,-60.5794508095555,12.));
#62540=CARTESIAN_POINT('Ctrl Pts',(36.1612113610758,-60.5936334114082,0.));
#62541=CARTESIAN_POINT('Ctrl Pts',(36.1612113610758,-60.5936334114082,12.));
#62542=CARTESIAN_POINT('Ctrl Pts',(36.1766314392624,-60.6078339534151,0.));
#62543=CARTESIAN_POINT('Ctrl Pts',(36.1766314392624,-60.6078339534151,12.));
#62544=CARTESIAN_POINT('Ctrl Pts',(36.1921031840618,-60.6220522649129,0.));
#62545=CARTESIAN_POINT('Ctrl Pts',(36.1921031840618,-60.6220522649129,12.));
#62546=CARTESIAN_POINT('Ctrl Pts',(36.2076265283261,-60.6362881765014,0.));
#62547=CARTESIAN_POINT('Ctrl Pts',(36.2076265283261,-60.6362881765014,12.));
#62548=CARTESIAN_POINT('Ctrl Pts',(36.2232014051549,-60.6505415197054,0.));
#62549=CARTESIAN_POINT('Ctrl Pts',(36.2232014051549,-60.6505415197054,12.));
#62550=CARTESIAN_POINT('Ctrl Pts',(36.2388277477225,-60.6648121265907,0.));
#62551=CARTESIAN_POINT('Ctrl Pts',(36.2388277477225,-60.6648121265907,12.));
#62552=CARTESIAN_POINT('Ctrl Pts',(36.2545054892911,-60.6790998297823,0.));
#62553=CARTESIAN_POINT('Ctrl Pts',(36.2545054892911,-60.6790998297823,12.));
#62554=CARTESIAN_POINT('Ctrl Pts',(36.2702345632883,-60.6934044626304,0.));
#62555=CARTESIAN_POINT('Ctrl Pts',(36.2702345632883,-60.6934044626304,12.));
#62556=CARTESIAN_POINT('Ctrl Pts',(36.2860149033587,-60.7077258593268,0.));
#62557=CARTESIAN_POINT('Ctrl Pts',(36.2860149033587,-60.7077258593268,12.));
#62558=CARTESIAN_POINT('Ctrl Pts',(36.3018464434204,-60.7220638550396,0.));
#62559=CARTESIAN_POINT('Ctrl Pts',(36.3018464434204,-60.7220638550396,12.));
#62560=CARTESIAN_POINT('Ctrl Pts',(36.3177291177148,-60.7364182860388,0.));
#62561=CARTESIAN_POINT('Ctrl Pts',(36.3177291177148,-60.7364182860388,12.));
#62562=CARTESIAN_POINT('Ctrl Pts',(36.3336628607844,-60.7507889896283,0.));
#62563=CARTESIAN_POINT('Ctrl Pts',(36.3336628607844,-60.7507889896283,12.));
#62564=CARTESIAN_POINT('Ctrl Pts',(36.349647607448,-60.7651758040791,0.));
#62565=CARTESIAN_POINT('Ctrl Pts',(36.349647607448,-60.7651758040791,12.));
#62566=CARTESIAN_POINT('Ctrl Pts',(36.3656832927733,-60.779578568563,0.));
#62567=CARTESIAN_POINT('Ctrl Pts',(36.3656832927733,-60.779578568563,12.));
#62568=CARTESIAN_POINT('Ctrl Pts',(36.38176985204,-60.7939971230781,0.));
#62569=CARTESIAN_POINT('Ctrl Pts',(36.38176985204,-60.7939971230781,12.));
#62570=CARTESIAN_POINT('Ctrl Pts',(36.3979072207175,-60.8084313084009,0.));
#62571=CARTESIAN_POINT('Ctrl Pts',(36.3979072207175,-60.8084313084009,12.));
#62572=CARTESIAN_POINT('Ctrl Pts',(36.414095334487,-60.8228809661179,0.));
#62573=CARTESIAN_POINT('Ctrl Pts',(36.414095334487,-60.8228809661179,12.));
#62574=CARTESIAN_POINT('Ctrl Pts',(36.4303341292497,-60.8373459386397,0.));
#62575=CARTESIAN_POINT('Ctrl Pts',(36.4303341292497,-60.8373459386397,12.));
#62576=CARTESIAN_POINT('Ctrl Pts',(36.4466235411353,-60.851826069218,0.));
#62577=CARTESIAN_POINT('Ctrl Pts',(36.4466235411353,-60.851826069218,12.));
#62578=CARTESIAN_POINT('Ctrl Pts',(36.4629635065038,-60.8663212019645,0.));
#62579=CARTESIAN_POINT('Ctrl Pts',(36.4629635065038,-60.8663212019645,12.));
#62580=CARTESIAN_POINT('Ctrl Pts',(36.4793539619459,-60.8808311818488,0.));
#62581=CARTESIAN_POINT('Ctrl Pts',(36.4793539619459,-60.8808311818488,12.));
#62582=CARTESIAN_POINT('Ctrl Pts',(36.4957948442832,-60.8953558546791,0.));
#62583=CARTESIAN_POINT('Ctrl Pts',(36.4957948442832,-60.8953558546791,12.));
#62584=CARTESIAN_POINT('Ctrl Pts',(36.5122860905611,-60.9098950670847,0.));
#62585=CARTESIAN_POINT('Ctrl Pts',(36.5122860905611,-60.9098950670847,12.));
#62586=CARTESIAN_POINT('Ctrl Pts',(36.5288276380417,-60.9244486664989,0.));
#62587=CARTESIAN_POINT('Ctrl Pts',(36.5288276380417,-60.9244486664989,12.));
#62588=CARTESIAN_POINT('Ctrl Pts',(36.5454194241866,-60.9390165011357,0.));
#62589=CARTESIAN_POINT('Ctrl Pts',(36.5454194241866,-60.9390165011357,12.));
#62590=CARTESIAN_POINT('Ctrl Pts',(36.5620613866616,-60.9535984199874,0.));
#62591=CARTESIAN_POINT('Ctrl Pts',(36.5620613866616,-60.9535984199874,12.));
#62592=CARTESIAN_POINT('Ctrl Pts',(36.5787534633416,-60.9681942728237,0.));
#62593=CARTESIAN_POINT('Ctrl Pts',(36.5787534633416,-60.9681942728237,12.));
#62594=CARTESIAN_POINT('Ctrl Pts',(36.5954955923109,-60.9828039101887,0.));
#62595=CARTESIAN_POINT('Ctrl Pts',(36.5954955923109,-60.9828039101887,12.));
#62596=CARTESIAN_POINT('Ctrl Pts',(36.61228771186,-60.9974271833981,0.));
#62597=CARTESIAN_POINT('Ctrl Pts',(36.61228771186,-60.9974271833981,12.));
#62598=CARTESIAN_POINT('Ctrl Pts',(36.6291297604775,-61.012063944535,0.));
#62599=CARTESIAN_POINT('Ctrl Pts',(36.6291297604775,-61.012063944535,12.));
#62600=CARTESIAN_POINT('Ctrl Pts',(36.6460216768553,-61.0267140464434,0.));
#62601=CARTESIAN_POINT('Ctrl Pts',(36.6460216768553,-61.0267140464434,12.));
#62602=CARTESIAN_POINT('Ctrl Pts',(36.6629633998886,-61.0413773427204,0.));
#62603=CARTESIAN_POINT('Ctrl Pts',(36.6629633998886,-61.0413773427204,12.));
#62604=CARTESIAN_POINT('Ctrl Pts',(36.6799548686741,-61.0560536877084,0.));
#62605=CARTESIAN_POINT('Ctrl Pts',(36.6799548686741,-61.0560536877084,12.));
#62606=CARTESIAN_POINT('Ctrl Pts',(36.6969960225019,-61.0707429364841,0.));
#62607=CARTESIAN_POINT('Ctrl Pts',(36.6969960225019,-61.0707429364841,12.));
#62608=CARTESIAN_POINT('Ctrl Pts',(36.7140868008479,-61.085444944851,0.));
#62609=CARTESIAN_POINT('Ctrl Pts',(36.7140868008479,-61.085444944851,12.));
#62610=CARTESIAN_POINT('Ctrl Pts',(36.7312271433799,-61.1001595693357,0.));
#62611=CARTESIAN_POINT('Ctrl Pts',(36.7312271433799,-61.1001595693357,12.));
#62612=CARTESIAN_POINT('Ctrl Pts',(36.7484169899591,-61.114886667182,0.));
#62613=CARTESIAN_POINT('Ctrl Pts',(36.7484169899591,-61.114886667182,12.));
#62614=CARTESIAN_POINT('Ctrl Pts',(36.7656562806381,-61.1296260963468,0.));
#62615=CARTESIAN_POINT('Ctrl Pts',(36.7656562806381,-61.1296260963468,12.));
#62616=CARTESIAN_POINT('Ctrl Pts',(36.782944955654,-61.1443777154926,0.));
#62617=CARTESIAN_POINT('Ctrl Pts',(36.782944955654,-61.1443777154926,12.));
#62618=CARTESIAN_POINT('Ctrl Pts',(36.8002829554221,-61.1591413839809,0.));
#62619=CARTESIAN_POINT('Ctrl Pts',(36.8002829554221,-61.1591413839809,12.));
#62620=CARTESIAN_POINT('Ctrl Pts',(36.8176702205436,-61.1739169618688,0.));
#62621=CARTESIAN_POINT('Ctrl Pts',(36.8176702205436,-61.1739169618688,12.));
#62622=CARTESIAN_POINT('Ctrl Pts',(36.8351066918043,-61.1887043099026,0.));
#62623=CARTESIAN_POINT('Ctrl Pts',(36.8351066918043,-61.1887043099026,12.));
#62624=CARTESIAN_POINT('Ctrl Pts',(36.8525923101736,-61.2035032895121,0.));
#62625=CARTESIAN_POINT('Ctrl Pts',(36.8525923101736,-61.2035032895121,12.));
#62626=CARTESIAN_POINT('Ctrl Pts',(36.8701270167954,-61.2183137628031,0.));
#62627=CARTESIAN_POINT('Ctrl Pts',(36.8701270167954,-61.2183137628031,12.));
#62628=CARTESIAN_POINT('Ctrl Pts',(36.8877107529844,-61.2331355925513,0.));
#62629=CARTESIAN_POINT('Ctrl Pts',(36.8877107529844,-61.2331355925513,12.));
#62630=CARTESIAN_POINT('Ctrl Pts',(36.9053434602324,-61.2479686421979,0.));
#62631=CARTESIAN_POINT('Ctrl Pts',(36.9053434602324,-61.2479686421979,12.));
#62632=CARTESIAN_POINT('Ctrl Pts',(36.9230250802079,-61.2628127758443,0.));
#62633=CARTESIAN_POINT('Ctrl Pts',(36.9230250802079,-61.2628127758443,12.));
#62634=CARTESIAN_POINT('Ctrl Pts',(36.9407555547542,-61.2776678582473,0.));
#62635=CARTESIAN_POINT('Ctrl Pts',(36.9407555547542,-61.2776678582473,12.));
#62636=CARTESIAN_POINT('Ctrl Pts',(36.9585348258798,-61.2925337548113,0.));
#62637=CARTESIAN_POINT('Ctrl Pts',(36.9585348258798,-61.2925337548113,12.));
#62638=CARTESIAN_POINT('Ctrl Pts',(36.976362835757,-61.3074103315834,0.));
#62639=CARTESIAN_POINT('Ctrl Pts',(36.976362835757,-61.3074103315834,12.));
#62640=CARTESIAN_POINT('Ctrl Pts',(36.994239526729,-61.3222974552519,0.));
#62641=CARTESIAN_POINT('Ctrl Pts',(36.994239526729,-61.3222974552519,12.));
#62642=CARTESIAN_POINT('Ctrl Pts',(37.0121648413088,-61.3371949931396,0.));
#62643=CARTESIAN_POINT('Ctrl Pts',(37.0121648413088,-61.3371949931396,12.));
#62644=CARTESIAN_POINT('Ctrl Pts',(37.0301387221766,-61.352102813199,0.));
#62645=CARTESIAN_POINT('Ctrl Pts',(37.0301387221766,-61.352102813199,12.));
#62646=CARTESIAN_POINT('Ctrl Pts',(37.0481611121698,-61.367020784004,0.));
#62647=CARTESIAN_POINT('Ctrl Pts',(37.0481611121698,-61.367020784004,12.));
#62648=CARTESIAN_POINT('Ctrl Pts',(37.0662319542827,-61.3819487747458,0.));
#62649=CARTESIAN_POINT('Ctrl Pts',(37.0662319542827,-61.3819487747458,12.));
#62650=CARTESIAN_POINT('Ctrl Pts',(37.0843511916729,-61.3968866552294,0.));
#62651=CARTESIAN_POINT('Ctrl Pts',(37.0843511916729,-61.3968866552294,12.));
#62652=CARTESIAN_POINT('Ctrl Pts',(37.1025187676597,-61.411834295869,0.));
#62653=CARTESIAN_POINT('Ctrl Pts',(37.1025187676597,-61.411834295869,12.));
#62654=CARTESIAN_POINT('Ctrl Pts',(37.1207346257229,-61.4267915676833,0.));
#62655=CARTESIAN_POINT('Ctrl Pts',(37.1207346257229,-61.4267915676833,12.));
#62656=CARTESIAN_POINT('Ctrl Pts',(37.138998709492,-61.4417583422888,0.));
#62657=CARTESIAN_POINT('Ctrl Pts',(37.138998709492,-61.4417583422888,12.));
#62658=CARTESIAN_POINT('Ctrl Pts',(37.157310962747,-61.4567344918946,0.));
#62659=CARTESIAN_POINT('Ctrl Pts',(37.157310962747,-61.4567344918946,12.));
#62660=CARTESIAN_POINT('Ctrl Pts',(37.175671329425,-61.471719889301,0.));
#62661=CARTESIAN_POINT('Ctrl Pts',(37.175671329425,-61.471719889301,12.));
#62662=CARTESIAN_POINT('Ctrl Pts',(37.1940797536182,-61.4867144078939,0.));
#62663=CARTESIAN_POINT('Ctrl Pts',(37.1940797536182,-61.4867144078939,12.));
#62664=CARTESIAN_POINT('Ctrl Pts',(37.2125361795727,-61.5017179216404,0.));
#62665=CARTESIAN_POINT('Ctrl Pts',(37.2125361795727,-61.5017179216404,12.));
#62666=CARTESIAN_POINT('Ctrl Pts',(37.2310405516775,-61.5167303050823,0.));
#62667=CARTESIAN_POINT('Ctrl Pts',(37.2310405516775,-61.5167303050823,12.));
#62668=CARTESIAN_POINT('Ctrl Pts',(37.2495928144661,-61.5317514333319,0.));
#62669=CARTESIAN_POINT('Ctrl Pts',(37.2495928144661,-61.5317514333319,12.));
#62670=CARTESIAN_POINT('Ctrl Pts',(37.2681929126218,-61.5467811820685,0.));
#62671=CARTESIAN_POINT('Ctrl Pts',(37.2681929126218,-61.5467811820685,12.));
#62672=CARTESIAN_POINT('Ctrl Pts',(37.286840790977,-61.5618194275348,0.));
#62673=CARTESIAN_POINT('Ctrl Pts',(37.286840790977,-61.5618194275348,12.));
#62674=CARTESIAN_POINT('Ctrl Pts',(37.3055363945108,-61.5768660465313,0.));
#62675=CARTESIAN_POINT('Ctrl Pts',(37.3055363945108,-61.5768660465313,12.));
#62676=CARTESIAN_POINT('Ctrl Pts',(37.3242796683395,-61.591920916412,0.));
#62677=CARTESIAN_POINT('Ctrl Pts',(37.3242796683395,-61.591920916412,12.));
#62678=CARTESIAN_POINT('Ctrl Pts',(37.3430705577178,-61.6069839150804,0.));
#62679=CARTESIAN_POINT('Ctrl Pts',(37.3430705577178,-61.6069839150804,12.));
#62680=CARTESIAN_POINT('Ctrl Pts',(37.3619090080447,-61.6220549209862,0.));
#62681=CARTESIAN_POINT('Ctrl Pts',(37.3619090080447,-61.6220549209862,12.));
#62682=CARTESIAN_POINT('Ctrl Pts',(37.3807949648623,-61.6371338131208,0.));
#62683=CARTESIAN_POINT('Ctrl Pts',(37.3807949648623,-61.6371338131208,12.));
#62684=CARTESIAN_POINT('Ctrl Pts',(37.3997283738534,-61.6522204710133,0.));
#62685=CARTESIAN_POINT('Ctrl Pts',(37.3997283738534,-61.6522204710133,12.));
#62686=CARTESIAN_POINT('Ctrl Pts',(37.4187091808324,-61.6673147747249,0.));
#62687=CARTESIAN_POINT('Ctrl Pts',(37.4187091808324,-61.6673147747249,12.));
#62688=CARTESIAN_POINT('Ctrl Pts',(37.4377373317456,-61.6824166048453,0.));
#62689=CARTESIAN_POINT('Ctrl Pts',(37.4377373317456,-61.6824166048453,12.));
#62690=CARTESIAN_POINT('Ctrl Pts',(37.4568127726776,-61.69752584249,0.));
#62691=CARTESIAN_POINT('Ctrl Pts',(37.4568127726776,-61.69752584249,12.));
#62692=CARTESIAN_POINT('Ctrl Pts',(37.475935449851,-61.7126423692965,0.));
#62693=CARTESIAN_POINT('Ctrl Pts',(37.475935449851,-61.7126423692965,12.));
#62694=CARTESIAN_POINT('Ctrl Pts',(37.4951053096235,-61.7277660674203,0.));
#62695=CARTESIAN_POINT('Ctrl Pts',(37.4951053096235,-61.7277660674203,12.));
#62696=CARTESIAN_POINT('Ctrl Pts',(37.5143222984794,-61.7428968195295,0.));
#62697=CARTESIAN_POINT('Ctrl Pts',(37.5143222984794,-61.7428968195295,12.));
#62698=CARTESIAN_POINT('Ctrl Pts',(37.5335863630286,-61.7580345088013,0.));
#62699=CARTESIAN_POINT('Ctrl Pts',(37.5335863630286,-61.7580345088013,12.));
#62700=CARTESIAN_POINT('Ctrl Pts',(37.5528974500142,-61.7731790189191,0.));
#62701=CARTESIAN_POINT('Ctrl Pts',(37.5528974500142,-61.7731790189191,12.));
#62702=CARTESIAN_POINT('Ctrl Pts',(37.5722555063112,-61.7883302340689,0.));
#62703=CARTESIAN_POINT('Ctrl Pts',(37.5722555063112,-61.7883302340689,12.));
#62704=CARTESIAN_POINT('Ctrl Pts',(37.5916604789252,-61.8034880389362,0.));
#62705=CARTESIAN_POINT('Ctrl Pts',(37.5916604789252,-61.8034880389362,12.));
#62706=CARTESIAN_POINT('Ctrl Pts',(37.6111123149836,-61.8186523187011,0.));
#62707=CARTESIAN_POINT('Ctrl Pts',(37.6111123149836,-61.8186523187011,12.));
#62708=CARTESIAN_POINT('Ctrl Pts',(37.6306109617341,-61.8338229590345,0.));
#62709=CARTESIAN_POINT('Ctrl Pts',(37.6306109617341,-61.8338229590345,12.));
#62710=CARTESIAN_POINT('Ctrl Pts',(37.6501563665518,-61.848999846095,0.));
#62711=CARTESIAN_POINT('Ctrl Pts',(37.6501563665518,-61.848999846095,12.));
#62712=CARTESIAN_POINT('Ctrl Pts',(37.6697484769389,-61.8641828665257,0.));
#62713=CARTESIAN_POINT('Ctrl Pts',(37.6697484769389,-61.8641828665257,12.));
#62714=CARTESIAN_POINT('Ctrl Pts',(37.689387240523,-61.879371907451,0.));
#62715=CARTESIAN_POINT('Ctrl Pts',(37.689387240523,-61.879371907451,12.));
#62716=CARTESIAN_POINT('Ctrl Pts',(37.7090726050489,-61.8945668564714,0.));
#62717=CARTESIAN_POINT('Ctrl Pts',(37.7090726050489,-61.8945668564714,12.));
#62718=CARTESIAN_POINT('Ctrl Pts',(37.7288045183765,-61.9097676016616,0.));
#62719=CARTESIAN_POINT('Ctrl Pts',(37.7288045183765,-61.9097676016616,12.));
#62720=CARTESIAN_POINT('Ctrl Pts',(37.748582928488,-61.9249740315664,0.));
#62721=CARTESIAN_POINT('Ctrl Pts',(37.748582928488,-61.9249740315664,12.));
#62722=CARTESIAN_POINT('Ctrl Pts',(37.7684077834877,-61.940186035198,0.));
#62723=CARTESIAN_POINT('Ctrl Pts',(37.7684077834877,-61.940186035198,12.));
#62724=CARTESIAN_POINT('Ctrl Pts',(37.7882790316012,-61.9554035020334,0.));
#62725=CARTESIAN_POINT('Ctrl Pts',(37.7882790316012,-61.9554035020334,12.));
#62726=CARTESIAN_POINT('Ctrl Pts',(37.808196621168,-61.9706263220101,0.));
#62727=CARTESIAN_POINT('Ctrl Pts',(37.808196621168,-61.9706263220101,12.));
#62728=CARTESIAN_POINT('Ctrl Pts',(37.8281605006371,-61.9858543855221,0.));
#62729=CARTESIAN_POINT('Ctrl Pts',(37.8281605006371,-61.9858543855221,12.));
#62730=CARTESIAN_POINT('Ctrl Pts',(37.8481706185742,-62.0010875834176,0.));
#62731=CARTESIAN_POINT('Ctrl Pts',(37.8481706185742,-62.0010875834176,12.));
#62732=CARTESIAN_POINT('Ctrl Pts',(37.8682269236628,-62.0163258069954,0.));
#62733=CARTESIAN_POINT('Ctrl Pts',(37.8682269236628,-62.0163258069954,12.));
#62734=CARTESIAN_POINT('Ctrl Pts',(37.888329364703,-62.0315689480022,0.));
#62735=CARTESIAN_POINT('Ctrl Pts',(37.888329364703,-62.0315689480022,12.));
#62736=CARTESIAN_POINT('Ctrl Pts',(37.9084778906054,-62.0468168986289,0.));
#62737=CARTESIAN_POINT('Ctrl Pts',(37.9084778906054,-62.0468168986289,12.));
#62738=CARTESIAN_POINT('Ctrl Pts',(37.9286724503849,-62.0620695515072,0.));
#62739=CARTESIAN_POINT('Ctrl Pts',(37.9286724503849,-62.0620695515072,12.));
#62740=CARTESIAN_POINT('Ctrl Pts',(37.9489129931685,-62.0773267997072,0.));
#62741=CARTESIAN_POINT('Ctrl Pts',(37.9489129931685,-62.0773267997072,12.));
#62742=CARTESIAN_POINT('Ctrl Pts',(37.9691994681963,-62.0925885367346,0.));
#62743=CARTESIAN_POINT('Ctrl Pts',(37.9691994681963,-62.0925885367346,12.));
#62744=CARTESIAN_POINT('Ctrl Pts',(37.9895318248212,-62.107854656528,0.));
#62745=CARTESIAN_POINT('Ctrl Pts',(37.9895318248212,-62.107854656528,12.));
#62746=CARTESIAN_POINT('Ctrl Pts',(38.0099100125041,-62.1231250534558,0.));
#62747=CARTESIAN_POINT('Ctrl Pts',(38.0099100125041,-62.1231250534558,12.));
#62748=CARTESIAN_POINT('Ctrl Pts',(38.0303339808059,-62.1383996223136,0.));
#62749=CARTESIAN_POINT('Ctrl Pts',(38.0303339808059,-62.1383996223136,12.));
#62750=CARTESIAN_POINT('Ctrl Pts',(38.0508036793944,-62.153678258321,0.));
#62751=CARTESIAN_POINT('Ctrl Pts',(38.0508036793944,-62.153678258321,12.));
#62752=CARTESIAN_POINT('Ctrl Pts',(38.0713190580466,-62.1689608571182,0.));
#62753=CARTESIAN_POINT('Ctrl Pts',(38.0713190580466,-62.1689608571182,12.));
#62754=CARTESIAN_POINT('Ctrl Pts',(38.0918800666479,-62.1842473147626,0.));
#62755=CARTESIAN_POINT('Ctrl Pts',(38.0918800666479,-62.1842473147626,12.));
#62756=CARTESIAN_POINT('Ctrl Pts',(38.1124866551884,-62.1995375277253,0.));
#62757=CARTESIAN_POINT('Ctrl Pts',(38.1124866551884,-62.1995375277253,12.));
#62758=CARTESIAN_POINT('Ctrl Pts',(38.1331387737528,-62.2148313928859,0.));
#62759=CARTESIAN_POINT('Ctrl Pts',(38.1331387737528,-62.2148313928859,12.));
#62760=CARTESIAN_POINT('Ctrl Pts',(38.1538363725264,-62.2301288075318,0.));
#62761=CARTESIAN_POINT('Ctrl Pts',(38.1538363725264,-62.2301288075318,12.));
#62762=CARTESIAN_POINT('Ctrl Pts',(38.1745794017997,-62.245429669358,0.));
#62763=CARTESIAN_POINT('Ctrl Pts',(38.1745794017997,-62.245429669358,12.));
#62764=CARTESIAN_POINT('Ctrl Pts',(38.1953678119692,-62.2607338764655,0.));
#62765=CARTESIAN_POINT('Ctrl Pts',(38.1953678119692,-62.2607338764655,12.));
#62766=CARTESIAN_POINT('Ctrl Pts',(38.2162015535351,-62.2760413273601,0.));
#62767=CARTESIAN_POINT('Ctrl Pts',(38.2162015535351,-62.2760413273601,12.));
#62768=CARTESIAN_POINT('Ctrl Pts',(38.2370805770931,-62.2913519209517,0.));
#62769=CARTESIAN_POINT('Ctrl Pts',(38.2370805770931,-62.2913519209517,12.));
#62770=CARTESIAN_POINT('Ctrl Pts',(38.2580048333356,-62.3066655565497,0.));
#62771=CARTESIAN_POINT('Ctrl Pts',(38.2580048333356,-62.3066655565497,12.));
#62772=CARTESIAN_POINT('Ctrl Pts',(38.2789742730559,-62.3219821338564,0.));
#62773=CARTESIAN_POINT('Ctrl Pts',(38.2789742730559,-62.3219821338564,12.));
#62774=CARTESIAN_POINT('Ctrl Pts',(38.2999888471474,-62.337301552961,0.));
#62775=CARTESIAN_POINT('Ctrl Pts',(38.2999888471474,-62.337301552961,12.));
#62776=CARTESIAN_POINT('Ctrl Pts',(38.3210485066003,-62.3526237143338,0.));
#62777=CARTESIAN_POINT('Ctrl Pts',(38.3210485066003,-62.3526237143338,12.));
#62778=CARTESIAN_POINT('Ctrl Pts',(38.3421532024915,-62.3679485188178,0.));
#62779=CARTESIAN_POINT('Ctrl Pts',(38.3421532024915,-62.3679485188178,12.));
#62780=CARTESIAN_POINT('Ctrl Pts',(38.3633028859835,-62.3832758676281,0.));
#62781=CARTESIAN_POINT('Ctrl Pts',(38.3633028859835,-62.3832758676281,12.));
#62782=CARTESIAN_POINT('Ctrl Pts',(38.384497508335,-62.3986056623587,0.));
#62783=CARTESIAN_POINT('Ctrl Pts',(38.384497508335,-62.3986056623587,12.));
#62784=CARTESIAN_POINT('Ctrl Pts',(38.4057370209054,-62.4139378049891,0.));
#62785=CARTESIAN_POINT('Ctrl Pts',(38.4057370209054,-62.4139378049891,12.));
#62786=CARTESIAN_POINT('Ctrl Pts',(38.4270213751567,-62.42927219789,0.));
#62787=CARTESIAN_POINT('Ctrl Pts',(38.4270213751567,-62.42927219789,12.));
#62788=CARTESIAN_POINT('Ctrl Pts',(38.4483505226512,-62.4446087438304,0.));
#62789=CARTESIAN_POINT('Ctrl Pts',(38.4483505226512,-62.4446087438304,12.));
#62790=CARTESIAN_POINT('Ctrl Pts',(38.4697244150473,-62.4599473459799,0.));
#62791=CARTESIAN_POINT('Ctrl Pts',(38.4697244150473,-62.4599473459799,12.));
#62792=CARTESIAN_POINT('Ctrl Pts',(38.4911430040988,-62.4752879078842,0.));
#62793=CARTESIAN_POINT('Ctrl Pts',(38.4911430040988,-62.4752879078842,12.));
#62794=CARTESIAN_POINT('Ctrl Pts',(38.5126062416496,-62.4906303334435,0.));
#62795=CARTESIAN_POINT('Ctrl Pts',(38.5126062416496,-62.4906303334435,12.));
#62796=CARTESIAN_POINT('Ctrl Pts',(38.5341140796247,-62.5059745268899,0.));
#62797=CARTESIAN_POINT('Ctrl Pts',(38.5341140796247,-62.5059745268899,12.));
#62798=CARTESIAN_POINT('Ctrl Pts',(38.5556664700201,-62.5213203927672,0.));
#62799=CARTESIAN_POINT('Ctrl Pts',(38.5556664700201,-62.5213203927672,12.));
#62800=CARTESIAN_POINT('Ctrl Pts',(38.5772633648841,-62.5366678359035,0.));
#62801=CARTESIAN_POINT('Ctrl Pts',(38.5772633648841,-62.5366678359035,12.));
#62802=CARTESIAN_POINT('Ctrl Pts',(38.5989047163401,-62.5520167614529,0.));
#62803=CARTESIAN_POINT('Ctrl Pts',(38.5989047163401,-62.5520167614529,12.));
#62804=CARTESIAN_POINT('Ctrl Pts',(38.6205904766078,-62.567367074937,0.));
#62805=CARTESIAN_POINT('Ctrl Pts',(38.6205904766078,-62.567367074937,12.));
#62806=CARTESIAN_POINT('Ctrl Pts',(38.6423205980214,-62.5827186822923,0.));
#62807=CARTESIAN_POINT('Ctrl Pts',(38.6423205980214,-62.5827186822923,12.));
#62808=CARTESIAN_POINT('Ctrl Pts',(38.6640950330418,-62.5980714899048,0.));
#62809=CARTESIAN_POINT('Ctrl Pts',(38.6640950330418,-62.5980714899048,12.));
#62810=CARTESIAN_POINT('Ctrl Pts',(38.6859137342726,-62.6134254046731,0.));
#62811=CARTESIAN_POINT('Ctrl Pts',(38.6859137342726,-62.6134254046731,12.));
#62812=CARTESIAN_POINT('Ctrl Pts',(38.7077766544411,-62.6287803339534,0.));
#62813=CARTESIAN_POINT('Ctrl Pts',(38.7077766544411,-62.6287803339534,12.));
#62814=CARTESIAN_POINT('Ctrl Pts',(38.7296837463605,-62.6441361854406,0.));
#62815=CARTESIAN_POINT('Ctrl Pts',(38.7296837463605,-62.6441361854406,12.));
#62816=CARTESIAN_POINT('Ctrl Pts',(38.7516349628902,-62.6594928670626,0.));
#62817=CARTESIAN_POINT('Ctrl Pts',(38.7516349628902,-62.6594928670626,12.));
#62818=CARTESIAN_POINT('Ctrl Pts',(38.7736302568982,-62.6748502868836,0.));
#62819=CARTESIAN_POINT('Ctrl Pts',(38.7736302568982,-62.6748502868836,12.));
#62820=CARTESIAN_POINT('Ctrl Pts',(38.7956695812032,-62.6902083529698,0.));
#62821=CARTESIAN_POINT('Ctrl Pts',(38.7956695812032,-62.6902083529698,12.));
#62822=CARTESIAN_POINT('Ctrl Pts',(38.8177528885687,-62.7055669733811,0.));
#62823=CARTESIAN_POINT('Ctrl Pts',(38.8177528885687,-62.7055669733811,12.));
#62824=CARTESIAN_POINT('Ctrl Pts',(38.8398801318185,-62.7209260564505,0.));
#62825=CARTESIAN_POINT('Ctrl Pts',(38.8398801318185,-62.7209260564505,12.));
#62826=CARTESIAN_POINT('Ctrl Pts',(38.8620512639239,-62.7362855110052,0.));
#62827=CARTESIAN_POINT('Ctrl Pts',(38.8620512639239,-62.7362855110052,12.));
#62828=CARTESIAN_POINT('Ctrl Pts',(38.8842662380984,-62.7516452466129,0.));
#62829=CARTESIAN_POINT('Ctrl Pts',(38.8842662380984,-62.7516452466129,12.));
#62830=CARTESIAN_POINT('Ctrl Pts',(38.9065250078824,-62.7670051738131,0.));
#62831=CARTESIAN_POINT('Ctrl Pts',(38.9065250078824,-62.7670051738131,12.));
#62832=CARTESIAN_POINT('Ctrl Pts',(38.928827527232,-62.7823652043677,0.));
#62833=CARTESIAN_POINT('Ctrl Pts',(38.928827527232,-62.7823652043677,12.));
#62834=CARTESIAN_POINT('Ctrl Pts',(38.9511737503146,-62.797725250709,0.));
#62835=CARTESIAN_POINT('Ctrl Pts',(38.9511737503146,-62.797725250709,12.));
#62836=CARTESIAN_POINT('Ctrl Pts',(38.9735636313073,-62.8130852254004,0.));
#62837=CARTESIAN_POINT('Ctrl Pts',(38.9735636313073,-62.8130852254004,12.));
#62838=CARTESIAN_POINT('Ctrl Pts',(38.9959971241695,-62.8284450405451,0.));
#62839=CARTESIAN_POINT('Ctrl Pts',(38.9959971241695,-62.8284450405451,12.));
#62840=CARTESIAN_POINT('Ctrl Pts',(39.018474182465,-62.8438046073237,0.));
#62841=CARTESIAN_POINT('Ctrl Pts',(39.018474182465,-62.8438046073237,12.));
#62842=CARTESIAN_POINT('Ctrl Pts',(39.0409947590519,-62.859163835209,0.));
#62843=CARTESIAN_POINT('Ctrl Pts',(39.0409947590519,-62.859163835209,12.));
#62844=CARTESIAN_POINT('Ctrl Pts',(39.0635588063309,-62.8745226326046,0.));
#62845=CARTESIAN_POINT('Ctrl Pts',(39.0635588063309,-62.8745226326046,12.));
#62846=CARTESIAN_POINT('Ctrl Pts',(39.0861662767964,-62.8898809082658,0.));
#62847=CARTESIAN_POINT('Ctrl Pts',(39.0861662767964,-62.8898809082658,12.));
#62848=CARTESIAN_POINT('Ctrl Pts',(39.1088171235144,-62.9052385725416,0.));
#62849=CARTESIAN_POINT('Ctrl Pts',(39.1088171235144,-62.9052385725416,12.));
#62850=CARTESIAN_POINT('Ctrl Pts',(39.1315113005745,-62.9205955385551,0.));
#62851=CARTESIAN_POINT('Ctrl Pts',(39.1315113005745,-62.9205955385551,12.));
#62852=CARTESIAN_POINT('Ctrl Pts',(39.1542487636708,-62.9359517237352,0.));
#62853=CARTESIAN_POINT('Ctrl Pts',(39.1542487636708,-62.9359517237352,12.));
#62854=CARTESIAN_POINT('Ctrl Pts',(39.1770294702367,-62.9513070501777,0.));
#62855=CARTESIAN_POINT('Ctrl Pts',(39.1770294702367,-62.9513070501777,12.));
#62856=CARTESIAN_POINT('Ctrl Pts',(39.199853378159,-62.9666614412627,0.));
#62857=CARTESIAN_POINT('Ctrl Pts',(39.199853378159,-62.9666614412627,12.));
#62858=CARTESIAN_POINT('Ctrl Pts',(39.2227204447583,-62.9820148189849,0.));
#62859=CARTESIAN_POINT('Ctrl Pts',(39.2227204447583,-62.9820148189849,12.));
#62860=CARTESIAN_POINT('Ctrl Pts',(39.2456306256092,-62.9973671008685,0.));
#62861=CARTESIAN_POINT('Ctrl Pts',(39.2456306256092,-62.9973671008685,12.));
#62862=CARTESIAN_POINT('Ctrl Pts',(39.2685838735411,-63.0127181973702,0.));
#62863=CARTESIAN_POINT('Ctrl Pts',(39.2685838735411,-63.0127181973702,12.));
#62864=CARTESIAN_POINT('Ctrl Pts',(39.2915801372468,-63.0280680082522,0.));
#62865=CARTESIAN_POINT('Ctrl Pts',(39.2915801372468,-63.0280680082522,12.));
#62866=CARTESIAN_POINT('Ctrl Pts',(39.3146193632546,-63.0434164278221,0.));
#62867=CARTESIAN_POINT('Ctrl Pts',(39.3146193632546,-63.0434164278221,12.));
#62868=CARTESIAN_POINT('Ctrl Pts',(39.3377014983757,-63.0587633513993,0.));
#62869=CARTESIAN_POINT('Ctrl Pts',(39.3377014983757,-63.0587633513993,12.));
#62870=CARTESIAN_POINT('Ctrl Pts',(39.3608264920487,-63.0741086815957,0.));
#62871=CARTESIAN_POINT('Ctrl Pts',(39.3608264920487,-63.0741086815957,12.));
#62872=CARTESIAN_POINT('Ctrl Pts',(39.3839942985688,-63.0894523341238,0.));
#62873=CARTESIAN_POINT('Ctrl Pts',(39.3839942985688,-63.0894523341238,12.));
#62874=CARTESIAN_POINT('Ctrl Pts',(39.4072048797401,-63.1047942451583,0.));
#62875=CARTESIAN_POINT('Ctrl Pts',(39.4072048797401,-63.1047942451583,12.));
#62876=CARTESIAN_POINT('Ctrl Pts',(39.4304582059507,-63.1201343730643,0.));
#62877=CARTESIAN_POINT('Ctrl Pts',(39.4304582059507,-63.1201343730643,12.));
#62878=CARTESIAN_POINT('Ctrl Pts',(39.4537542551852,-63.1354726927781,0.));
#62879=CARTESIAN_POINT('Ctrl Pts',(39.4537542551852,-63.1354726927781,12.));
#62880=CARTESIAN_POINT('Ctrl Pts',(39.4724252610807,-63.1477418921889,0.));
#62881=CARTESIAN_POINT('Ctrl Pts',(39.4724252610807,-63.1477418921889,12.));
#62882=CARTESIAN_POINT('Ctrl Pts',(39.4864477303614,-63.1569429707564,0.));
#62883=CARTESIAN_POINT('Ctrl Pts',(39.4864477303614,-63.1569429707564,12.));
#62884=CARTESIAN_POINT('Ctrl Pts',(39.4958045828059,-63.1630766582674,0.));
#62885=CARTESIAN_POINT('Ctrl Pts',(39.4958045828059,-63.1630766582674,12.));
#62886=CARTESIAN_POINT('Ctrl Pts',(39.5004851439258,-63.1661434108059,0.));
#62887=CARTESIAN_POINT('Ctrl Pts',(39.5004851439258,-63.1661434108059,12.));
#62888=CARTESIAN_POINT('',(35.7368311217509,-60.1903555511633,0.));
#62889=CARTESIAN_POINT('Ctrl Pts',(35.7368311217509,-60.1903555511633,0.));
#62890=CARTESIAN_POINT('Ctrl Pts',(35.7396040203974,-60.1930746580239,0.));
#62891=CARTESIAN_POINT('Ctrl Pts',(35.7451551752456,-60.1985151474406,0.));
#62892=CARTESIAN_POINT('Ctrl Pts',(35.7534979801871,-60.2066827086579,0.));
#62893=CARTESIAN_POINT('Ctrl Pts',(35.7646538667299,-60.2175864449678,0.));
#62894=CARTESIAN_POINT('Ctrl Pts',(35.7786523045783,-60.2312388621286,0.));
#62895=CARTESIAN_POINT('Ctrl Pts',(35.7927043145165,-60.2449139865206,0.));
#62896=CARTESIAN_POINT('Ctrl Pts',(35.8068098723386,-60.2586117365278,0.));
#62897=CARTESIAN_POINT('Ctrl Pts',(35.8209689272574,-60.2723319687507,0.));
#62898=CARTESIAN_POINT('Ctrl Pts',(35.8351814020424,-60.2860744798563,0.));
#62899=CARTESIAN_POINT('Ctrl Pts',(35.8494472046784,-60.2998390330173,0.));
#62900=CARTESIAN_POINT('Ctrl Pts',(35.8637662371635,-60.313625378281,0.));
#62901=CARTESIAN_POINT('Ctrl Pts',(35.878138405151,-60.3274332746781,0.));
#62902=CARTESIAN_POINT('Ctrl Pts',(35.8925636280633,-60.3412625135223,0.));
#62903=CARTESIAN_POINT('Ctrl Pts',(35.9070418358501,-60.3551129108794,0.));
#62904=CARTESIAN_POINT('Ctrl Pts',(35.9215729642219,-60.368984296546,0.));
#62905=CARTESIAN_POINT('Ctrl Pts',(35.9361569506956,-60.3828765049031,0.));
#62906=CARTESIAN_POINT('Ctrl Pts',(35.9507937296727,-60.3967893635487,0.));
#62907=CARTESIAN_POINT('Ctrl Pts',(35.9654832299627,-60.4107226875759,0.));
#62908=CARTESIAN_POINT('Ctrl Pts',(35.9802253773535,-60.424676285496,0.));
#62909=CARTESIAN_POINT('Ctrl Pts',(35.9950200962175,-60.438649962949,0.));
#62910=CARTESIAN_POINT('Ctrl Pts',(36.0098673113557,-60.452643526964,0.));
#62911=CARTESIAN_POINT('Ctrl Pts',(36.0247669500867,-60.4666567908053,0.));
#62912=CARTESIAN_POINT('Ctrl Pts',(36.0397189421617,-60.4806895737643,0.));
#62913=CARTESIAN_POINT('Ctrl Pts',(36.0547232187682,-60.4947416988396,0.));
#62914=CARTESIAN_POINT('Ctrl Pts',(36.0697797118377,-60.5088129911357,0.));
#62915=CARTESIAN_POINT('Ctrl Pts',(36.0848883531969,-60.5229032759001,0.));
#62916=CARTESIAN_POINT('Ctrl Pts',(36.1000490738532,-60.5370123768841,0.));
#62917=CARTESIAN_POINT('Ctrl Pts',(36.1152618043757,-60.5511401172014,0.));
#62918=CARTESIAN_POINT('Ctrl Pts',(36.1305264752195,-60.5652863200732,0.));
#62919=CARTESIAN_POINT('Ctrl Pts',(36.1458430170425,-60.5794508095555,0.));
#62920=CARTESIAN_POINT('Ctrl Pts',(36.1612113610758,-60.5936334114082,0.));
#62921=CARTESIAN_POINT('Ctrl Pts',(36.1766314392624,-60.6078339534151,0.));
#62922=CARTESIAN_POINT('Ctrl Pts',(36.1921031840618,-60.6220522649129,0.));
#62923=CARTESIAN_POINT('Ctrl Pts',(36.2076265283261,-60.6362881765014,0.));
#62924=CARTESIAN_POINT('Ctrl Pts',(36.2232014051549,-60.6505415197054,0.));
#62925=CARTESIAN_POINT('Ctrl Pts',(36.2388277477225,-60.6648121265907,0.));
#62926=CARTESIAN_POINT('Ctrl Pts',(36.2545054892911,-60.6790998297823,0.));
#62927=CARTESIAN_POINT('Ctrl Pts',(36.2702345632883,-60.6934044626304,0.));
#62928=CARTESIAN_POINT('Ctrl Pts',(36.2860149033587,-60.7077258593268,0.));
#62929=CARTESIAN_POINT('Ctrl Pts',(36.3018464434204,-60.7220638550396,0.));
#62930=CARTESIAN_POINT('Ctrl Pts',(36.3177291177148,-60.7364182860388,0.));
#62931=CARTESIAN_POINT('Ctrl Pts',(36.3336628607844,-60.7507889896283,0.));
#62932=CARTESIAN_POINT('Ctrl Pts',(36.349647607448,-60.7651758040791,0.));
#62933=CARTESIAN_POINT('Ctrl Pts',(36.3656832927733,-60.779578568563,0.));
#62934=CARTESIAN_POINT('Ctrl Pts',(36.38176985204,-60.7939971230781,0.));
#62935=CARTESIAN_POINT('Ctrl Pts',(36.3979072207175,-60.8084313084009,0.));
#62936=CARTESIAN_POINT('Ctrl Pts',(36.414095334487,-60.8228809661179,0.));
#62937=CARTESIAN_POINT('Ctrl Pts',(36.4303341292497,-60.8373459386397,0.));
#62938=CARTESIAN_POINT('Ctrl Pts',(36.4466235411353,-60.851826069218,0.));
#62939=CARTESIAN_POINT('Ctrl Pts',(36.4629635065038,-60.8663212019645,0.));
#62940=CARTESIAN_POINT('Ctrl Pts',(36.4793539619459,-60.8808311818488,0.));
#62941=CARTESIAN_POINT('Ctrl Pts',(36.4957948442832,-60.8953558546791,0.));
#62942=CARTESIAN_POINT('Ctrl Pts',(36.5122860905611,-60.9098950670847,0.));
#62943=CARTESIAN_POINT('Ctrl Pts',(36.5288276380417,-60.9244486664989,0.));
#62944=CARTESIAN_POINT('Ctrl Pts',(36.5454194241866,-60.9390165011357,0.));
#62945=CARTESIAN_POINT('Ctrl Pts',(36.5620613866616,-60.9535984199874,0.));
#62946=CARTESIAN_POINT('Ctrl Pts',(36.5787534633416,-60.9681942728237,0.));
#62947=CARTESIAN_POINT('Ctrl Pts',(36.5954955923109,-60.9828039101887,0.));
#62948=CARTESIAN_POINT('Ctrl Pts',(36.61228771186,-60.9974271833981,0.));
#62949=CARTESIAN_POINT('Ctrl Pts',(36.6291297604775,-61.012063944535,0.));
#62950=CARTESIAN_POINT('Ctrl Pts',(36.6460216768553,-61.0267140464434,0.));
#62951=CARTESIAN_POINT('Ctrl Pts',(36.6629633998886,-61.0413773427204,0.));
#62952=CARTESIAN_POINT('Ctrl Pts',(36.6799548686741,-61.0560536877084,0.));
#62953=CARTESIAN_POINT('Ctrl Pts',(36.6969960225019,-61.0707429364841,0.));
#62954=CARTESIAN_POINT('Ctrl Pts',(36.7140868008479,-61.085444944851,0.));
#62955=CARTESIAN_POINT('Ctrl Pts',(36.7312271433799,-61.1001595693357,0.));
#62956=CARTESIAN_POINT('Ctrl Pts',(36.7484169899591,-61.114886667182,0.));
#62957=CARTESIAN_POINT('Ctrl Pts',(36.7656562806381,-61.1296260963468,0.));
#62958=CARTESIAN_POINT('Ctrl Pts',(36.782944955654,-61.1443777154926,0.));
#62959=CARTESIAN_POINT('Ctrl Pts',(36.8002829554221,-61.1591413839809,0.));
#62960=CARTESIAN_POINT('Ctrl Pts',(36.8176702205436,-61.1739169618688,0.));
#62961=CARTESIAN_POINT('Ctrl Pts',(36.8351066918043,-61.1887043099026,0.));
#62962=CARTESIAN_POINT('Ctrl Pts',(36.8525923101736,-61.2035032895121,0.));
#62963=CARTESIAN_POINT('Ctrl Pts',(36.8701270167954,-61.2183137628031,0.));
#62964=CARTESIAN_POINT('Ctrl Pts',(36.8877107529844,-61.2331355925513,0.));
#62965=CARTESIAN_POINT('Ctrl Pts',(36.9053434602324,-61.2479686421979,0.));
#62966=CARTESIAN_POINT('Ctrl Pts',(36.9230250802079,-61.2628127758443,0.));
#62967=CARTESIAN_POINT('Ctrl Pts',(36.9407555547542,-61.2776678582473,0.));
#62968=CARTESIAN_POINT('Ctrl Pts',(36.9585348258798,-61.2925337548113,0.));
#62969=CARTESIAN_POINT('Ctrl Pts',(36.976362835757,-61.3074103315834,0.));
#62970=CARTESIAN_POINT('Ctrl Pts',(36.994239526729,-61.3222974552519,0.));
#62971=CARTESIAN_POINT('Ctrl Pts',(37.0121648413088,-61.3371949931396,0.));
#62972=CARTESIAN_POINT('Ctrl Pts',(37.0301387221766,-61.352102813199,0.));
#62973=CARTESIAN_POINT('Ctrl Pts',(37.0481611121698,-61.367020784004,0.));
#62974=CARTESIAN_POINT('Ctrl Pts',(37.0662319542827,-61.3819487747458,0.));
#62975=CARTESIAN_POINT('Ctrl Pts',(37.0843511916729,-61.3968866552294,0.));
#62976=CARTESIAN_POINT('Ctrl Pts',(37.1025187676597,-61.411834295869,0.));
#62977=CARTESIAN_POINT('Ctrl Pts',(37.1207346257229,-61.4267915676833,0.));
#62978=CARTESIAN_POINT('Ctrl Pts',(37.138998709492,-61.4417583422888,0.));
#62979=CARTESIAN_POINT('Ctrl Pts',(37.157310962747,-61.4567344918946,0.));
#62980=CARTESIAN_POINT('Ctrl Pts',(37.175671329425,-61.471719889301,0.));
#62981=CARTESIAN_POINT('Ctrl Pts',(37.1940797536182,-61.4867144078939,0.));
#62982=CARTESIAN_POINT('Ctrl Pts',(37.2125361795727,-61.5017179216404,0.));
#62983=CARTESIAN_POINT('Ctrl Pts',(37.2310405516775,-61.5167303050823,0.));
#62984=CARTESIAN_POINT('Ctrl Pts',(37.2495928144661,-61.5317514333319,0.));
#62985=CARTESIAN_POINT('Ctrl Pts',(37.2681929126218,-61.5467811820685,0.));
#62986=CARTESIAN_POINT('Ctrl Pts',(37.286840790977,-61.5618194275348,0.));
#62987=CARTESIAN_POINT('Ctrl Pts',(37.3055363945108,-61.5768660465313,0.));
#62988=CARTESIAN_POINT('Ctrl Pts',(37.3242796683395,-61.591920916412,0.));
#62989=CARTESIAN_POINT('Ctrl Pts',(37.3430705577178,-61.6069839150804,0.));
#62990=CARTESIAN_POINT('Ctrl Pts',(37.3619090080447,-61.6220549209862,0.));
#62991=CARTESIAN_POINT('Ctrl Pts',(37.3807949648623,-61.6371338131208,0.));
#62992=CARTESIAN_POINT('Ctrl Pts',(37.3997283738534,-61.6522204710133,0.));
#62993=CARTESIAN_POINT('Ctrl Pts',(37.4187091808324,-61.6673147747249,0.));
#62994=CARTESIAN_POINT('Ctrl Pts',(37.4377373317456,-61.6824166048453,0.));
#62995=CARTESIAN_POINT('Ctrl Pts',(37.4568127726776,-61.69752584249,0.));
#62996=CARTESIAN_POINT('Ctrl Pts',(37.475935449851,-61.7126423692965,0.));
#62997=CARTESIAN_POINT('Ctrl Pts',(37.4951053096235,-61.7277660674203,0.));
#62998=CARTESIAN_POINT('Ctrl Pts',(37.5143222984794,-61.7428968195295,0.));
#62999=CARTESIAN_POINT('Ctrl Pts',(37.5335863630286,-61.7580345088013,0.));
#63000=CARTESIAN_POINT('Ctrl Pts',(37.5528974500142,-61.7731790189191,0.));
#63001=CARTESIAN_POINT('Ctrl Pts',(37.5722555063112,-61.7883302340689,0.));
#63002=CARTESIAN_POINT('Ctrl Pts',(37.5916604789252,-61.8034880389362,0.));
#63003=CARTESIAN_POINT('Ctrl Pts',(37.6111123149836,-61.8186523187011,0.));
#63004=CARTESIAN_POINT('Ctrl Pts',(37.6306109617341,-61.8338229590345,0.));
#63005=CARTESIAN_POINT('Ctrl Pts',(37.6501563665518,-61.848999846095,0.));
#63006=CARTESIAN_POINT('Ctrl Pts',(37.6697484769389,-61.8641828665257,0.));
#63007=CARTESIAN_POINT('Ctrl Pts',(37.689387240523,-61.879371907451,0.));
#63008=CARTESIAN_POINT('Ctrl Pts',(37.7090726050489,-61.8945668564714,0.));
#63009=CARTESIAN_POINT('Ctrl Pts',(37.7288045183765,-61.9097676016616,0.));
#63010=CARTESIAN_POINT('Ctrl Pts',(37.748582928488,-61.9249740315664,0.));
#63011=CARTESIAN_POINT('Ctrl Pts',(37.7684077834877,-61.940186035198,0.));
#63012=CARTESIAN_POINT('Ctrl Pts',(37.7882790316012,-61.9554035020334,0.));
#63013=CARTESIAN_POINT('Ctrl Pts',(37.808196621168,-61.9706263220101,0.));
#63014=CARTESIAN_POINT('Ctrl Pts',(37.8281605006371,-61.9858543855221,0.));
#63015=CARTESIAN_POINT('Ctrl Pts',(37.8481706185742,-62.0010875834176,0.));
#63016=CARTESIAN_POINT('Ctrl Pts',(37.8682269236628,-62.0163258069954,0.));
#63017=CARTESIAN_POINT('Ctrl Pts',(37.888329364703,-62.0315689480022,0.));
#63018=CARTESIAN_POINT('Ctrl Pts',(37.9084778906054,-62.0468168986289,0.));
#63019=CARTESIAN_POINT('Ctrl Pts',(37.9286724503849,-62.0620695515072,0.));
#63020=CARTESIAN_POINT('Ctrl Pts',(37.9489129931685,-62.0773267997072,0.));
#63021=CARTESIAN_POINT('Ctrl Pts',(37.9691994681963,-62.0925885367346,0.));
#63022=CARTESIAN_POINT('Ctrl Pts',(37.9895318248212,-62.107854656528,0.));
#63023=CARTESIAN_POINT('Ctrl Pts',(38.0099100125041,-62.1231250534558,0.));
#63024=CARTESIAN_POINT('Ctrl Pts',(38.0303339808059,-62.1383996223136,0.));
#63025=CARTESIAN_POINT('Ctrl Pts',(38.0508036793944,-62.153678258321,0.));
#63026=CARTESIAN_POINT('Ctrl Pts',(38.0713190580466,-62.1689608571182,0.));
#63027=CARTESIAN_POINT('Ctrl Pts',(38.0918800666479,-62.1842473147626,0.));
#63028=CARTESIAN_POINT('Ctrl Pts',(38.1124866551884,-62.1995375277253,0.));
#63029=CARTESIAN_POINT('Ctrl Pts',(38.1331387737528,-62.2148313928859,0.));
#63030=CARTESIAN_POINT('Ctrl Pts',(38.1538363725264,-62.2301288075318,0.));
#63031=CARTESIAN_POINT('Ctrl Pts',(38.1745794017997,-62.245429669358,0.));
#63032=CARTESIAN_POINT('Ctrl Pts',(38.1953678119692,-62.2607338764655,0.));
#63033=CARTESIAN_POINT('Ctrl Pts',(38.2162015535351,-62.2760413273601,0.));
#63034=CARTESIAN_POINT('Ctrl Pts',(38.2370805770931,-62.2913519209517,0.));
#63035=CARTESIAN_POINT('Ctrl Pts',(38.2580048333356,-62.3066655565497,0.));
#63036=CARTESIAN_POINT('Ctrl Pts',(38.2789742730559,-62.3219821338564,0.));
#63037=CARTESIAN_POINT('Ctrl Pts',(38.2999888471474,-62.337301552961,0.));
#63038=CARTESIAN_POINT('Ctrl Pts',(38.3210485066003,-62.3526237143338,0.));
#63039=CARTESIAN_POINT('Ctrl Pts',(38.3421532024915,-62.3679485188178,0.));
#63040=CARTESIAN_POINT('Ctrl Pts',(38.3633028859835,-62.3832758676281,0.));
#63041=CARTESIAN_POINT('Ctrl Pts',(38.384497508335,-62.3986056623587,0.));
#63042=CARTESIAN_POINT('Ctrl Pts',(38.4057370209054,-62.4139378049891,0.));
#63043=CARTESIAN_POINT('Ctrl Pts',(38.4270213751567,-62.42927219789,0.));
#63044=CARTESIAN_POINT('Ctrl Pts',(38.4483505226512,-62.4446087438304,0.));
#63045=CARTESIAN_POINT('Ctrl Pts',(38.4697244150473,-62.4599473459799,0.));
#63046=CARTESIAN_POINT('Ctrl Pts',(38.4911430040988,-62.4752879078842,0.));
#63047=CARTESIAN_POINT('Ctrl Pts',(38.5126062416496,-62.4906303334435,0.));
#63048=CARTESIAN_POINT('Ctrl Pts',(38.5341140796247,-62.5059745268899,0.));
#63049=CARTESIAN_POINT('Ctrl Pts',(38.5556664700201,-62.5213203927672,0.));
#63050=CARTESIAN_POINT('Ctrl Pts',(38.5772633648841,-62.5366678359035,0.));
#63051=CARTESIAN_POINT('Ctrl Pts',(38.5989047163401,-62.5520167614529,0.));
#63052=CARTESIAN_POINT('Ctrl Pts',(38.6205904766078,-62.567367074937,0.));
#63053=CARTESIAN_POINT('Ctrl Pts',(38.6423205980214,-62.5827186822923,0.));
#63054=CARTESIAN_POINT('Ctrl Pts',(38.6640950330418,-62.5980714899048,0.));
#63055=CARTESIAN_POINT('Ctrl Pts',(38.6859137342726,-62.6134254046731,0.));
#63056=CARTESIAN_POINT('Ctrl Pts',(38.7077766544411,-62.6287803339534,0.));
#63057=CARTESIAN_POINT('Ctrl Pts',(38.7296837463605,-62.6441361854406,0.));
#63058=CARTESIAN_POINT('Ctrl Pts',(38.7516349628902,-62.6594928670626,0.));
#63059=CARTESIAN_POINT('Ctrl Pts',(38.7736302568982,-62.6748502868836,0.));
#63060=CARTESIAN_POINT('Ctrl Pts',(38.7956695812032,-62.6902083529698,0.));
#63061=CARTESIAN_POINT('Ctrl Pts',(38.8177528885687,-62.7055669733811,0.));
#63062=CARTESIAN_POINT('Ctrl Pts',(38.8398801318185,-62.7209260564505,0.));
#63063=CARTESIAN_POINT('Ctrl Pts',(38.8620512639239,-62.7362855110052,0.));
#63064=CARTESIAN_POINT('Ctrl Pts',(38.8842662380984,-62.7516452466129,0.));
#63065=CARTESIAN_POINT('Ctrl Pts',(38.9065250078824,-62.7670051738131,0.));
#63066=CARTESIAN_POINT('Ctrl Pts',(38.928827527232,-62.7823652043677,0.));
#63067=CARTESIAN_POINT('Ctrl Pts',(38.9511737503146,-62.797725250709,0.));
#63068=CARTESIAN_POINT('Ctrl Pts',(38.9735636313073,-62.8130852254004,0.));
#63069=CARTESIAN_POINT('Ctrl Pts',(38.9959971241695,-62.8284450405451,0.));
#63070=CARTESIAN_POINT('Ctrl Pts',(39.018474182465,-62.8438046073237,0.));
#63071=CARTESIAN_POINT('Ctrl Pts',(39.0409947590519,-62.859163835209,0.));
#63072=CARTESIAN_POINT('Ctrl Pts',(39.0635588063309,-62.8745226326046,0.));
#63073=CARTESIAN_POINT('Ctrl Pts',(39.0861662767964,-62.8898809082658,0.));
#63074=CARTESIAN_POINT('Ctrl Pts',(39.1088171235144,-62.9052385725416,0.));
#63075=CARTESIAN_POINT('Ctrl Pts',(39.1315113005745,-62.9205955385551,0.));
#63076=CARTESIAN_POINT('Ctrl Pts',(39.1542487636708,-62.9359517237352,0.));
#63077=CARTESIAN_POINT('Ctrl Pts',(39.1770294702367,-62.9513070501777,0.));
#63078=CARTESIAN_POINT('Ctrl Pts',(39.1965939820803,-62.9644687386693,0.));
#63079=CARTESIAN_POINT('Ctrl Pts',(39.2116170128276,-62.9745590018499,0.));
#63080=CARTESIAN_POINT('Ctrl Pts',(39.2220794388572,-62.9815782721128,0.));
#63081=CARTESIAN_POINT('Ctrl Pts',(39.2279686274718,-62.9855268615901,0.));
#63082=CARTESIAN_POINT('Ctrl Pts',(39.2292784191464,-62.9864049293629,0.));
#63083=CARTESIAN_POINT('',(35.7368311217509,-60.1903555511633,12.));
#63084=CARTESIAN_POINT('',(35.7368311217509,-60.1903555511633,0.));
#63085=CARTESIAN_POINT('Ctrl Pts',(39.2292784191464,-62.9864049293629,12.));
#63086=CARTESIAN_POINT('Ctrl Pts',(39.2279686274718,-62.9855268615901,12.));
#63087=CARTESIAN_POINT('Ctrl Pts',(39.2220794388571,-62.9815782721128,12.));
#63088=CARTESIAN_POINT('Ctrl Pts',(39.2116170128275,-62.9745590018499,12.));
#63089=CARTESIAN_POINT('Ctrl Pts',(39.1965939820803,-62.9644687386693,12.));
#63090=CARTESIAN_POINT('Ctrl Pts',(39.1770294702367,-62.9513070501777,12.));
#63091=CARTESIAN_POINT('Ctrl Pts',(39.1542487636708,-62.9359517237352,12.));
#63092=CARTESIAN_POINT('Ctrl Pts',(39.1315113005745,-62.9205955385551,12.));
#63093=CARTESIAN_POINT('Ctrl Pts',(39.1088171235144,-62.9052385725416,12.));
#63094=CARTESIAN_POINT('Ctrl Pts',(39.0861662767964,-62.8898809082658,12.));
#63095=CARTESIAN_POINT('Ctrl Pts',(39.0635588063309,-62.8745226326046,12.));
#63096=CARTESIAN_POINT('Ctrl Pts',(39.0409947590519,-62.859163835209,12.));
#63097=CARTESIAN_POINT('Ctrl Pts',(39.018474182465,-62.8438046073237,12.));
#63098=CARTESIAN_POINT('Ctrl Pts',(38.9959971241695,-62.8284450405451,12.));
#63099=CARTESIAN_POINT('Ctrl Pts',(38.9735636313073,-62.8130852254004,12.));
#63100=CARTESIAN_POINT('Ctrl Pts',(38.9511737503146,-62.797725250709,12.));
#63101=CARTESIAN_POINT('Ctrl Pts',(38.928827527232,-62.7823652043677,12.));
#63102=CARTESIAN_POINT('Ctrl Pts',(38.9065250078824,-62.7670051738131,12.));
#63103=CARTESIAN_POINT('Ctrl Pts',(38.8842662380984,-62.7516452466129,12.));
#63104=CARTESIAN_POINT('Ctrl Pts',(38.8620512639239,-62.7362855110052,12.));
#63105=CARTESIAN_POINT('Ctrl Pts',(38.8398801318185,-62.7209260564505,12.));
#63106=CARTESIAN_POINT('Ctrl Pts',(38.8177528885687,-62.7055669733811,12.));
#63107=CARTESIAN_POINT('Ctrl Pts',(38.7956695812032,-62.6902083529698,12.));
#63108=CARTESIAN_POINT('Ctrl Pts',(38.7736302568982,-62.6748502868836,12.));
#63109=CARTESIAN_POINT('Ctrl Pts',(38.7516349628902,-62.6594928670626,12.));
#63110=CARTESIAN_POINT('Ctrl Pts',(38.7296837463605,-62.6441361854406,12.));
#63111=CARTESIAN_POINT('Ctrl Pts',(38.7077766544411,-62.6287803339534,12.));
#63112=CARTESIAN_POINT('Ctrl Pts',(38.6859137342726,-62.6134254046731,12.));
#63113=CARTESIAN_POINT('Ctrl Pts',(38.6640950330418,-62.5980714899048,12.));
#63114=CARTESIAN_POINT('Ctrl Pts',(38.6423205980214,-62.5827186822923,12.));
#63115=CARTESIAN_POINT('Ctrl Pts',(38.6205904766078,-62.567367074937,12.));
#63116=CARTESIAN_POINT('Ctrl Pts',(38.5989047163401,-62.5520167614529,12.));
#63117=CARTESIAN_POINT('Ctrl Pts',(38.5772633648841,-62.5366678359035,12.));
#63118=CARTESIAN_POINT('Ctrl Pts',(38.5556664700201,-62.5213203927672,12.));
#63119=CARTESIAN_POINT('Ctrl Pts',(38.5341140796247,-62.5059745268899,12.));
#63120=CARTESIAN_POINT('Ctrl Pts',(38.5126062416496,-62.4906303334435,12.));
#63121=CARTESIAN_POINT('Ctrl Pts',(38.4911430040988,-62.4752879078842,12.));
#63122=CARTESIAN_POINT('Ctrl Pts',(38.4697244150473,-62.4599473459799,12.));
#63123=CARTESIAN_POINT('Ctrl Pts',(38.4483505226512,-62.4446087438304,12.));
#63124=CARTESIAN_POINT('Ctrl Pts',(38.4270213751567,-62.42927219789,12.));
#63125=CARTESIAN_POINT('Ctrl Pts',(38.4057370209054,-62.4139378049891,12.));
#63126=CARTESIAN_POINT('Ctrl Pts',(38.384497508335,-62.3986056623587,12.));
#63127=CARTESIAN_POINT('Ctrl Pts',(38.3633028859835,-62.3832758676281,12.));
#63128=CARTESIAN_POINT('Ctrl Pts',(38.3421532024915,-62.3679485188178,12.));
#63129=CARTESIAN_POINT('Ctrl Pts',(38.3210485066003,-62.3526237143338,12.));
#63130=CARTESIAN_POINT('Ctrl Pts',(38.2999888471474,-62.337301552961,12.));
#63131=CARTESIAN_POINT('Ctrl Pts',(38.2789742730559,-62.3219821338564,12.));
#63132=CARTESIAN_POINT('Ctrl Pts',(38.2580048333356,-62.3066655565497,12.));
#63133=CARTESIAN_POINT('Ctrl Pts',(38.2370805770931,-62.2913519209517,12.));
#63134=CARTESIAN_POINT('Ctrl Pts',(38.2162015535351,-62.2760413273601,12.));
#63135=CARTESIAN_POINT('Ctrl Pts',(38.1953678119692,-62.2607338764655,12.));
#63136=CARTESIAN_POINT('Ctrl Pts',(38.1745794017997,-62.245429669358,12.));
#63137=CARTESIAN_POINT('Ctrl Pts',(38.1538363725264,-62.2301288075318,12.));
#63138=CARTESIAN_POINT('Ctrl Pts',(38.1331387737528,-62.2148313928859,12.));
#63139=CARTESIAN_POINT('Ctrl Pts',(38.1124866551884,-62.1995375277253,12.));
#63140=CARTESIAN_POINT('Ctrl Pts',(38.0918800666479,-62.1842473147626,12.));
#63141=CARTESIAN_POINT('Ctrl Pts',(38.0713190580466,-62.1689608571182,12.));
#63142=CARTESIAN_POINT('Ctrl Pts',(38.0508036793944,-62.153678258321,12.));
#63143=CARTESIAN_POINT('Ctrl Pts',(38.0303339808059,-62.1383996223136,12.));
#63144=CARTESIAN_POINT('Ctrl Pts',(38.0099100125041,-62.1231250534558,12.));
#63145=CARTESIAN_POINT('Ctrl Pts',(37.9895318248212,-62.107854656528,12.));
#63146=CARTESIAN_POINT('Ctrl Pts',(37.9691994681963,-62.0925885367346,12.));
#63147=CARTESIAN_POINT('Ctrl Pts',(37.9489129931685,-62.0773267997072,12.));
#63148=CARTESIAN_POINT('Ctrl Pts',(37.9286724503849,-62.0620695515072,12.));
#63149=CARTESIAN_POINT('Ctrl Pts',(37.9084778906054,-62.0468168986289,12.));
#63150=CARTESIAN_POINT('Ctrl Pts',(37.888329364703,-62.0315689480022,12.));
#63151=CARTESIAN_POINT('Ctrl Pts',(37.8682269236628,-62.0163258069954,12.));
#63152=CARTESIAN_POINT('Ctrl Pts',(37.8481706185742,-62.0010875834176,12.));
#63153=CARTESIAN_POINT('Ctrl Pts',(37.8281605006371,-61.9858543855221,12.));
#63154=CARTESIAN_POINT('Ctrl Pts',(37.808196621168,-61.9706263220101,12.));
#63155=CARTESIAN_POINT('Ctrl Pts',(37.7882790316012,-61.9554035020334,12.));
#63156=CARTESIAN_POINT('Ctrl Pts',(37.7684077834877,-61.940186035198,12.));
#63157=CARTESIAN_POINT('Ctrl Pts',(37.748582928488,-61.9249740315664,12.));
#63158=CARTESIAN_POINT('Ctrl Pts',(37.7288045183765,-61.9097676016616,12.));
#63159=CARTESIAN_POINT('Ctrl Pts',(37.7090726050489,-61.8945668564714,12.));
#63160=CARTESIAN_POINT('Ctrl Pts',(37.689387240523,-61.879371907451,12.));
#63161=CARTESIAN_POINT('Ctrl Pts',(37.6697484769389,-61.8641828665257,12.));
#63162=CARTESIAN_POINT('Ctrl Pts',(37.6501563665518,-61.848999846095,12.));
#63163=CARTESIAN_POINT('Ctrl Pts',(37.6306109617341,-61.8338229590345,12.));
#63164=CARTESIAN_POINT('Ctrl Pts',(37.6111123149836,-61.8186523187011,12.));
#63165=CARTESIAN_POINT('Ctrl Pts',(37.5916604789252,-61.8034880389362,12.));
#63166=CARTESIAN_POINT('Ctrl Pts',(37.5722555063112,-61.7883302340689,12.));
#63167=CARTESIAN_POINT('Ctrl Pts',(37.5528974500142,-61.7731790189191,12.));
#63168=CARTESIAN_POINT('Ctrl Pts',(37.5335863630286,-61.7580345088013,12.));
#63169=CARTESIAN_POINT('Ctrl Pts',(37.5143222984794,-61.7428968195295,12.));
#63170=CARTESIAN_POINT('Ctrl Pts',(37.4951053096235,-61.7277660674203,12.));
#63171=CARTESIAN_POINT('Ctrl Pts',(37.475935449851,-61.7126423692965,12.));
#63172=CARTESIAN_POINT('Ctrl Pts',(37.4568127726776,-61.69752584249,12.));
#63173=CARTESIAN_POINT('Ctrl Pts',(37.4377373317456,-61.6824166048453,12.));
#63174=CARTESIAN_POINT('Ctrl Pts',(37.4187091808324,-61.6673147747249,12.));
#63175=CARTESIAN_POINT('Ctrl Pts',(37.3997283738534,-61.6522204710133,12.));
#63176=CARTESIAN_POINT('Ctrl Pts',(37.3807949648623,-61.6371338131208,12.));
#63177=CARTESIAN_POINT('Ctrl Pts',(37.3619090080447,-61.6220549209862,12.));
#63178=CARTESIAN_POINT('Ctrl Pts',(37.3430705577178,-61.6069839150804,12.));
#63179=CARTESIAN_POINT('Ctrl Pts',(37.3242796683395,-61.591920916412,12.));
#63180=CARTESIAN_POINT('Ctrl Pts',(37.3055363945108,-61.5768660465313,12.));
#63181=CARTESIAN_POINT('Ctrl Pts',(37.286840790977,-61.5618194275348,12.));
#63182=CARTESIAN_POINT('Ctrl Pts',(37.2681929126218,-61.5467811820685,12.));
#63183=CARTESIAN_POINT('Ctrl Pts',(37.2495928144661,-61.5317514333319,12.));
#63184=CARTESIAN_POINT('Ctrl Pts',(37.2310405516775,-61.5167303050823,12.));
#63185=CARTESIAN_POINT('Ctrl Pts',(37.2125361795727,-61.5017179216404,12.));
#63186=CARTESIAN_POINT('Ctrl Pts',(37.1940797536182,-61.4867144078939,12.));
#63187=CARTESIAN_POINT('Ctrl Pts',(37.175671329425,-61.471719889301,12.));
#63188=CARTESIAN_POINT('Ctrl Pts',(37.157310962747,-61.4567344918946,12.));
#63189=CARTESIAN_POINT('Ctrl Pts',(37.138998709492,-61.4417583422888,12.));
#63190=CARTESIAN_POINT('Ctrl Pts',(37.1207346257229,-61.4267915676833,12.));
#63191=CARTESIAN_POINT('Ctrl Pts',(37.1025187676597,-61.411834295869,12.));
#63192=CARTESIAN_POINT('Ctrl Pts',(37.0843511916729,-61.3968866552294,12.));
#63193=CARTESIAN_POINT('Ctrl Pts',(37.0662319542827,-61.3819487747458,12.));
#63194=CARTESIAN_POINT('Ctrl Pts',(37.0481611121698,-61.367020784004,12.));
#63195=CARTESIAN_POINT('Ctrl Pts',(37.0301387221766,-61.352102813199,12.));
#63196=CARTESIAN_POINT('Ctrl Pts',(37.0121648413088,-61.3371949931396,12.));
#63197=CARTESIAN_POINT('Ctrl Pts',(36.994239526729,-61.3222974552519,12.));
#63198=CARTESIAN_POINT('Ctrl Pts',(36.976362835757,-61.3074103315834,12.));
#63199=CARTESIAN_POINT('Ctrl Pts',(36.9585348258798,-61.2925337548113,12.));
#63200=CARTESIAN_POINT('Ctrl Pts',(36.9407555547542,-61.2776678582473,12.));
#63201=CARTESIAN_POINT('Ctrl Pts',(36.9230250802079,-61.2628127758443,12.));
#63202=CARTESIAN_POINT('Ctrl Pts',(36.9053434602324,-61.2479686421979,12.));
#63203=CARTESIAN_POINT('Ctrl Pts',(36.8877107529844,-61.2331355925513,12.));
#63204=CARTESIAN_POINT('Ctrl Pts',(36.8701270167954,-61.2183137628031,12.));
#63205=CARTESIAN_POINT('Ctrl Pts',(36.8525923101736,-61.2035032895121,12.));
#63206=CARTESIAN_POINT('Ctrl Pts',(36.8351066918043,-61.1887043099026,12.));
#63207=CARTESIAN_POINT('Ctrl Pts',(36.8176702205436,-61.1739169618688,12.));
#63208=CARTESIAN_POINT('Ctrl Pts',(36.8002829554221,-61.1591413839809,12.));
#63209=CARTESIAN_POINT('Ctrl Pts',(36.782944955654,-61.1443777154926,12.));
#63210=CARTESIAN_POINT('Ctrl Pts',(36.7656562806381,-61.1296260963468,12.));
#63211=CARTESIAN_POINT('Ctrl Pts',(36.7484169899591,-61.114886667182,12.));
#63212=CARTESIAN_POINT('Ctrl Pts',(36.7312271433799,-61.1001595693357,12.));
#63213=CARTESIAN_POINT('Ctrl Pts',(36.7140868008479,-61.085444944851,12.));
#63214=CARTESIAN_POINT('Ctrl Pts',(36.6969960225019,-61.0707429364841,12.));
#63215=CARTESIAN_POINT('Ctrl Pts',(36.6799548686741,-61.0560536877084,12.));
#63216=CARTESIAN_POINT('Ctrl Pts',(36.6629633998886,-61.0413773427204,12.));
#63217=CARTESIAN_POINT('Ctrl Pts',(36.6460216768553,-61.0267140464434,12.));
#63218=CARTESIAN_POINT('Ctrl Pts',(36.6291297604775,-61.012063944535,12.));
#63219=CARTESIAN_POINT('Ctrl Pts',(36.61228771186,-60.9974271833981,12.));
#63220=CARTESIAN_POINT('Ctrl Pts',(36.5954955923109,-60.9828039101887,12.));
#63221=CARTESIAN_POINT('Ctrl Pts',(36.5787534633416,-60.9681942728237,12.));
#63222=CARTESIAN_POINT('Ctrl Pts',(36.5620613866616,-60.9535984199874,12.));
#63223=CARTESIAN_POINT('Ctrl Pts',(36.5454194241866,-60.9390165011357,12.));
#63224=CARTESIAN_POINT('Ctrl Pts',(36.5288276380417,-60.9244486664989,12.));
#63225=CARTESIAN_POINT('Ctrl Pts',(36.5122860905611,-60.9098950670847,12.));
#63226=CARTESIAN_POINT('Ctrl Pts',(36.4957948442832,-60.8953558546791,12.));
#63227=CARTESIAN_POINT('Ctrl Pts',(36.4793539619459,-60.8808311818488,12.));
#63228=CARTESIAN_POINT('Ctrl Pts',(36.4629635065038,-60.8663212019645,12.));
#63229=CARTESIAN_POINT('Ctrl Pts',(36.4466235411353,-60.851826069218,12.));
#63230=CARTESIAN_POINT('Ctrl Pts',(36.4303341292497,-60.8373459386397,12.));
#63231=CARTESIAN_POINT('Ctrl Pts',(36.414095334487,-60.8228809661179,12.));
#63232=CARTESIAN_POINT('Ctrl Pts',(36.3979072207175,-60.8084313084009,12.));
#63233=CARTESIAN_POINT('Ctrl Pts',(36.38176985204,-60.7939971230781,12.));
#63234=CARTESIAN_POINT('Ctrl Pts',(36.3656832927733,-60.779578568563,12.));
#63235=CARTESIAN_POINT('Ctrl Pts',(36.349647607448,-60.7651758040791,12.));
#63236=CARTESIAN_POINT('Ctrl Pts',(36.3336628607844,-60.7507889896283,12.));
#63237=CARTESIAN_POINT('Ctrl Pts',(36.3177291177148,-60.7364182860388,12.));
#63238=CARTESIAN_POINT('Ctrl Pts',(36.3018464434204,-60.7220638550396,12.));
#63239=CARTESIAN_POINT('Ctrl Pts',(36.2860149033587,-60.7077258593268,12.));
#63240=CARTESIAN_POINT('Ctrl Pts',(36.2702345632883,-60.6934044626304,12.));
#63241=CARTESIAN_POINT('Ctrl Pts',(36.2545054892911,-60.6790998297823,12.));
#63242=CARTESIAN_POINT('Ctrl Pts',(36.2388277477225,-60.6648121265907,12.));
#63243=CARTESIAN_POINT('Ctrl Pts',(36.2232014051549,-60.6505415197054,12.));
#63244=CARTESIAN_POINT('Ctrl Pts',(36.2076265283261,-60.6362881765014,12.));
#63245=CARTESIAN_POINT('Ctrl Pts',(36.1921031840618,-60.6220522649129,12.));
#63246=CARTESIAN_POINT('Ctrl Pts',(36.1766314392624,-60.6078339534151,12.));
#63247=CARTESIAN_POINT('Ctrl Pts',(36.1612113610758,-60.5936334114082,12.));
#63248=CARTESIAN_POINT('Ctrl Pts',(36.1458430170425,-60.5794508095555,12.));
#63249=CARTESIAN_POINT('Ctrl Pts',(36.1305264752195,-60.5652863200732,12.));
#63250=CARTESIAN_POINT('Ctrl Pts',(36.1152618043757,-60.5511401172014,12.));
#63251=CARTESIAN_POINT('Ctrl Pts',(36.1000490738532,-60.5370123768841,12.));
#63252=CARTESIAN_POINT('Ctrl Pts',(36.0848883531969,-60.5229032759001,12.));
#63253=CARTESIAN_POINT('Ctrl Pts',(36.0697797118377,-60.5088129911357,12.));
#63254=CARTESIAN_POINT('Ctrl Pts',(36.0547232187682,-60.4947416988396,12.));
#63255=CARTESIAN_POINT('Ctrl Pts',(36.0397189421617,-60.4806895737643,12.));
#63256=CARTESIAN_POINT('Ctrl Pts',(36.0247669500867,-60.4666567908053,12.));
#63257=CARTESIAN_POINT('Ctrl Pts',(36.0098673113557,-60.452643526964,12.));
#63258=CARTESIAN_POINT('Ctrl Pts',(35.9950200962175,-60.438649962949,12.));
#63259=CARTESIAN_POINT('Ctrl Pts',(35.9802253773535,-60.424676285496,12.));
#63260=CARTESIAN_POINT('Ctrl Pts',(35.9654832299627,-60.4107226875759,12.));
#63261=CARTESIAN_POINT('Ctrl Pts',(35.9507937296727,-60.3967893635487,12.));
#63262=CARTESIAN_POINT('Ctrl Pts',(35.9361569506956,-60.3828765049031,12.));
#63263=CARTESIAN_POINT('Ctrl Pts',(35.9215729642219,-60.368984296546,12.));
#63264=CARTESIAN_POINT('Ctrl Pts',(35.9070418358501,-60.3551129108794,12.));
#63265=CARTESIAN_POINT('Ctrl Pts',(35.8925636280633,-60.3412625135223,12.));
#63266=CARTESIAN_POINT('Ctrl Pts',(35.878138405151,-60.3274332746781,12.));
#63267=CARTESIAN_POINT('Ctrl Pts',(35.8637662371635,-60.313625378281,12.));
#63268=CARTESIAN_POINT('Ctrl Pts',(35.8494472046784,-60.2998390330173,12.));
#63269=CARTESIAN_POINT('Ctrl Pts',(35.8351814020424,-60.2860744798563,12.));
#63270=CARTESIAN_POINT('Ctrl Pts',(35.8209689272574,-60.2723319687507,12.));
#63271=CARTESIAN_POINT('Ctrl Pts',(35.8068098723386,-60.2586117365278,12.));
#63272=CARTESIAN_POINT('Ctrl Pts',(35.7927043145165,-60.2449139865206,12.));
#63273=CARTESIAN_POINT('Ctrl Pts',(35.7786523045783,-60.2312388621286,12.));
#63274=CARTESIAN_POINT('Ctrl Pts',(35.7646538667299,-60.2175864449678,12.));
#63275=CARTESIAN_POINT('Ctrl Pts',(35.7534979801871,-60.2066827086579,12.));
#63276=CARTESIAN_POINT('Ctrl Pts',(35.7451551752456,-60.1985151474406,12.));
#63277=CARTESIAN_POINT('Ctrl Pts',(35.7396040203974,-60.1930746580239,12.));
#63278=CARTESIAN_POINT('Ctrl Pts',(35.7368311217509,-60.1903555511633,12.));
#63279=CARTESIAN_POINT('Ctrl Pts',(40.506059810093,-62.1730054756874,-5.55111512312578E-16));
#63280=CARTESIAN_POINT('Ctrl Pts',(40.506059810093,-62.1730054756874,4.));
#63281=CARTESIAN_POINT('Ctrl Pts',(40.506059810093,-62.1730054756875,8.));
#63282=CARTESIAN_POINT('Ctrl Pts',(40.506059810093,-62.1730054756875,12.));
#63283=CARTESIAN_POINT('Ctrl Pts',(40.5229411493977,-62.2815834512357,-5.55111512312578E-16));
#63284=CARTESIAN_POINT('Ctrl Pts',(40.5229411493977,-62.2815834512357,4.));
#63285=CARTESIAN_POINT('Ctrl Pts',(40.5229411493977,-62.2815834512358,8.));
#63286=CARTESIAN_POINT('Ctrl Pts',(40.5229411493977,-62.2815834512358,12.));
#63287=CARTESIAN_POINT('Ctrl Pts',(40.4873422218647,-62.4810961163746,-5.55111512312578E-16));
#63288=CARTESIAN_POINT('Ctrl Pts',(40.4873422218647,-62.4810961163746,4.));
#63289=CARTESIAN_POINT('Ctrl Pts',(40.4873422218647,-62.4810961163747,7.99999999999999));
#63290=CARTESIAN_POINT('Ctrl Pts',(40.4873422218647,-62.4810961163747,12.));
#63291=CARTESIAN_POINT('Ctrl Pts',(40.3516729626244,-62.6258675056116,-5.55111512312578E-16));
#63292=CARTESIAN_POINT('Ctrl Pts',(40.3516729626244,-62.6258675056116,4.));
#63293=CARTESIAN_POINT('Ctrl Pts',(40.3516729626244,-62.6258675056116,8.00000000000001));
#63294=CARTESIAN_POINT('Ctrl Pts',(40.3516729626244,-62.6258675056116,12.));
#63295=CARTESIAN_POINT('Ctrl Pts',(40.282346977699,-62.6704278106373,-5.55111512312578E-16));
#63296=CARTESIAN_POINT('Ctrl Pts',(40.282346977699,-62.6704278106373,4.));
#63297=CARTESIAN_POINT('Ctrl Pts',(40.282346977699,-62.6704278106374,8.));
#63298=CARTESIAN_POINT('Ctrl Pts',(40.282346977699,-62.6704278106374,12.));
#63299=CARTESIAN_POINT('',(40.506059810093,-62.1730054756875,2.77555756156289E-16));
#63300=CARTESIAN_POINT('',(40.2823469776988,-62.6704278106371,0.));
#63301=CARTESIAN_POINT('Ctrl Pts',(40.506059810093,-62.1730054756874,-5.55111512312578E-16));
#63302=CARTESIAN_POINT('Ctrl Pts',(40.5229411493977,-62.2815834512357,-5.55111512312578E-16));
#63303=CARTESIAN_POINT('Ctrl Pts',(40.5025989050931,-62.395590688458,-5.55111512312578E-16));
#63304=CARTESIAN_POINT('Ctrl Pts',(40.4495806341086,-62.4917232233449,-5.55111512312578E-16));
#63305=CARTESIAN_POINT('Ctrl Pts',(40.4098169308703,-62.56382262451,-5.55111512312578E-16));
#63306=CARTESIAN_POINT('Ctrl Pts',(40.3516729626244,-62.6258675056116,-5.55111512312578E-16));
#63307=CARTESIAN_POINT('Ctrl Pts',(40.282346977699,-62.6704278106373,-5.55111512312578E-16));
#63308=CARTESIAN_POINT('',(40.2823469776988,-62.6704278106371,12.));
#63309=CARTESIAN_POINT('Ctrl Pts',(40.282346977699,-62.6704278106373,-5.55111512312578E-16));
#63310=CARTESIAN_POINT('Ctrl Pts',(40.282346977699,-62.6704278106373,4.));
#63311=CARTESIAN_POINT('Ctrl Pts',(40.282346977699,-62.6704278106374,8.));
#63312=CARTESIAN_POINT('Ctrl Pts',(40.282346977699,-62.6704278106374,12.));
#63313=CARTESIAN_POINT('',(40.506059810093,-62.1730054756875,12.));
#63314=CARTESIAN_POINT('Ctrl Pts',(40.282346977699,-62.6704278106374,12.));
#63315=CARTESIAN_POINT('Ctrl Pts',(40.3516729626244,-62.6258675056116,12.));
#63316=CARTESIAN_POINT('Ctrl Pts',(40.4098169308703,-62.5638226245101,12.));
#63317=CARTESIAN_POINT('Ctrl Pts',(40.4495806341086,-62.4917232233449,12.));
#63318=CARTESIAN_POINT('Ctrl Pts',(40.5025989050932,-62.395590688458,12.));
#63319=CARTESIAN_POINT('Ctrl Pts',(40.5229411493977,-62.2815834512358,12.));
#63320=CARTESIAN_POINT('Ctrl Pts',(40.506059810093,-62.1730054756875,12.));
#63321=CARTESIAN_POINT('Ctrl Pts',(40.506059810093,-62.1730054756875,12.));
#63322=CARTESIAN_POINT('Ctrl Pts',(40.506059810093,-62.1730054756875,8.));
#63323=CARTESIAN_POINT('Ctrl Pts',(40.506059810093,-62.1730054756874,4.));
#63324=CARTESIAN_POINT('Ctrl Pts',(40.506059810093,-62.1730054756874,-5.55111512312578E-16));
#63325=CARTESIAN_POINT('Origin',(2.01487121870483E-10,-3.16086693261782E-10,
0.));
#63326=CARTESIAN_POINT('Origin',(2.01487121870483E-10,-3.16086693261782E-10,
12.));
#63327=CARTESIAN_POINT('Origin',(2.01487121870483E-10,-3.16086693261782E-10,
0.));
#63328=CARTESIAN_POINT('Ctrl Pts',(34.1330090612035,-66.2207497120638,0.));
#63329=CARTESIAN_POINT('Ctrl Pts',(34.1330090612035,-66.2207497120638,4.));
#63330=CARTESIAN_POINT('Ctrl Pts',(34.1330090612035,-66.2207497120638,8.));
#63331=CARTESIAN_POINT('Ctrl Pts',(34.1330090612035,-66.2207497120638,12.));
#63332=CARTESIAN_POINT('Ctrl Pts',(34.0353379297088,-66.2710935941676,0.));
#63333=CARTESIAN_POINT('Ctrl Pts',(34.0353379297088,-66.2710935941676,4.));
#63334=CARTESIAN_POINT('Ctrl Pts',(34.0353379297088,-66.2710935941676,8.));
#63335=CARTESIAN_POINT('Ctrl Pts',(34.0353379297088,-66.2710935941676,12.));
#63336=CARTESIAN_POINT('Ctrl Pts',(33.8348041971631,-66.3003999311009,0.));
#63337=CARTESIAN_POINT('Ctrl Pts',(33.8348041971631,-66.3003999311009,4.00000000000001));
#63338=CARTESIAN_POINT('Ctrl Pts',(33.8348041971632,-66.3003999311009,8.));
#63339=CARTESIAN_POINT('Ctrl Pts',(33.8348041971632,-66.3003999311009,12.));
#63340=CARTESIAN_POINT('Ctrl Pts',(33.6545652280937,-66.2174610329229,0.));
#63341=CARTESIAN_POINT('Ctrl Pts',(33.6545652280937,-66.2174610329229,3.99999999999999));
#63342=CARTESIAN_POINT('Ctrl Pts',(33.6545652280938,-66.2174610329229,8.));
#63343=CARTESIAN_POINT('Ctrl Pts',(33.6545652280938,-66.2174610329229,12.));
#63344=CARTESIAN_POINT('Ctrl Pts',(33.5903722664954,-66.1657795405668,0.));
#63345=CARTESIAN_POINT('Ctrl Pts',(33.5903722664954,-66.1657795405668,4.));
#63346=CARTESIAN_POINT('Ctrl Pts',(33.5903722664955,-66.1657795405668,8.));
#63347=CARTESIAN_POINT('Ctrl Pts',(33.5903722664955,-66.1657795405668,12.));
#63348=CARTESIAN_POINT('',(34.1330090612035,-66.2207497120638,0.));
#63349=CARTESIAN_POINT('',(33.5903722664955,-66.1657795405667,0.));
#63350=CARTESIAN_POINT('Ctrl Pts',(34.1330090612035,-66.2207497120638,0.));
#63351=CARTESIAN_POINT('Ctrl Pts',(34.0353379297088,-66.2710935941676,0.));
#63352=CARTESIAN_POINT('Ctrl Pts',(33.920747225397,-66.2878400724152,0.));
#63353=CARTESIAN_POINT('Ctrl Pts',(33.8127833826284,-66.2679350453204,0.));
#63354=CARTESIAN_POINT('Ctrl Pts',(33.731810500552,-66.2530062749992,0.));
#63355=CARTESIAN_POINT('Ctrl Pts',(33.6545652280937,-66.2174610329229,0.));
#63356=CARTESIAN_POINT('Ctrl Pts',(33.5903722664954,-66.1657795405668,0.));
#63357=CARTESIAN_POINT('',(33.5903722664955,-66.1657795405668,12.));
#63358=CARTESIAN_POINT('Ctrl Pts',(33.5903722664954,-66.1657795405668,0.));
#63359=CARTESIAN_POINT('Ctrl Pts',(33.5903722664954,-66.1657795405668,4.));
#63360=CARTESIAN_POINT('Ctrl Pts',(33.5903722664955,-66.1657795405668,8.));
#63361=CARTESIAN_POINT('Ctrl Pts',(33.5903722664955,-66.1657795405668,12.));
#63362=CARTESIAN_POINT('',(34.1330090612035,-66.2207497120638,12.));
#63363=CARTESIAN_POINT('Ctrl Pts',(33.5903722664955,-66.1657795405668,12.));
#63364=CARTESIAN_POINT('Ctrl Pts',(33.6545652280938,-66.2174610329229,12.));
#63365=CARTESIAN_POINT('Ctrl Pts',(33.7318105005521,-66.2530062749992,12.));
#63366=CARTESIAN_POINT('Ctrl Pts',(33.8127833826285,-66.2679350453203,12.));
#63367=CARTESIAN_POINT('Ctrl Pts',(33.920747225397,-66.2878400724152,12.));
#63368=CARTESIAN_POINT('Ctrl Pts',(34.0353379297088,-66.2710935941676,12.));
#63369=CARTESIAN_POINT('Ctrl Pts',(34.1330090612035,-66.2207497120638,12.));
#63370=CARTESIAN_POINT('Ctrl Pts',(34.1330090612035,-66.2207497120638,12.));
#63371=CARTESIAN_POINT('Ctrl Pts',(34.1330090612035,-66.2207497120638,8.));
#63372=CARTESIAN_POINT('Ctrl Pts',(34.1330090612035,-66.2207497120638,4.));
#63373=CARTESIAN_POINT('Ctrl Pts',(34.1330090612035,-66.2207497120638,0.));
#63374=CARTESIAN_POINT('Ctrl Pts',(30.354906545781,-63.0759831361898,0.));
#63375=CARTESIAN_POINT('Ctrl Pts',(30.354906545781,-63.0759831361898,12.));
#63376=CARTESIAN_POINT('Ctrl Pts',(30.3574319069329,-63.078933570069,0.));
#63377=CARTESIAN_POINT('Ctrl Pts',(30.3574319069329,-63.078933570069,12.));
#63378=CARTESIAN_POINT('Ctrl Pts',(30.362487768065,-63.0848371718048,0.));
#63379=CARTESIAN_POINT('Ctrl Pts',(30.362487768065,-63.0848371718048,12.));
#63380=CARTESIAN_POINT('Ctrl Pts',(30.3700869762507,-63.0937007763471,0.));
#63381=CARTESIAN_POINT('Ctrl Pts',(30.3700869762507,-63.0937007763471,12.));
#63382=CARTESIAN_POINT('Ctrl Pts',(30.3802500880402,-63.105535320226,0.));
#63383=CARTESIAN_POINT('Ctrl Pts',(30.3802500880402,-63.105535320226,12.));
#63384=CARTESIAN_POINT('Ctrl Pts',(30.3930053710484,-63.1203558300657,0.));
#63385=CARTESIAN_POINT('Ctrl Pts',(30.3930053710484,-63.1203558300657,12.));
#63386=CARTESIAN_POINT('Ctrl Pts',(30.4058120432228,-63.1352036298441,0.));
#63387=CARTESIAN_POINT('Ctrl Pts',(30.4058120432228,-63.1352036298441,12.));
#63388=CARTESIAN_POINT('Ctrl Pts',(30.418670087563,-63.1500786361459,0.));
#63389=CARTESIAN_POINT('Ctrl Pts',(30.418670087563,-63.1500786361459,12.));
#63390=CARTESIAN_POINT('Ctrl Pts',(30.431579465973,-63.164980701691,0.));
#63391=CARTESIAN_POINT('Ctrl Pts',(30.431579465973,-63.164980701691,12.));
#63392=CARTESIAN_POINT('Ctrl Pts',(30.444540119238,-63.179909617189,0.));
#63393=CARTESIAN_POINT('Ctrl Pts',(30.444540119238,-63.179909617189,12.));
#63394=CARTESIAN_POINT('Ctrl Pts',(30.4575519763336,-63.1948651386942,0.));
#63395=CARTESIAN_POINT('Ctrl Pts',(30.4575519763336,-63.1948651386942,12.));
#63396=CARTESIAN_POINT('Ctrl Pts',(30.4706149614159,-63.2098470086636,0.));
#63397=CARTESIAN_POINT('Ctrl Pts',(30.4706149614159,-63.2098470086636,12.));
#63398=CARTESIAN_POINT('Ctrl Pts',(30.4837290014989,-63.2248549788222,0.));
#63399=CARTESIAN_POINT('Ctrl Pts',(30.4837290014989,-63.2248549788222,12.));
#63400=CARTESIAN_POINT('Ctrl Pts',(30.4968940344997,-63.2398888342546,0.));
#63401=CARTESIAN_POINT('Ctrl Pts',(30.4968940344997,-63.2398888342546,12.));
#63402=CARTESIAN_POINT('Ctrl Pts',(30.5101100066659,-63.2549483856215,0.));
#63403=CARTESIAN_POINT('Ctrl Pts',(30.5101100066659,-63.2549483856215,12.));
#63404=CARTESIAN_POINT('Ctrl Pts',(30.5233768687864,-63.2700334577639,0.));
#63405=CARTESIAN_POINT('Ctrl Pts',(30.5233768687864,-63.2700334577639,12.));
#63406=CARTESIAN_POINT('Ctrl Pts',(30.5366945730508,-63.2851438802474,0.));
#63407=CARTESIAN_POINT('Ctrl Pts',(30.5366945730508,-63.2851438802474,12.));
#63408=CARTESIAN_POINT('Ctrl Pts',(30.5500630691359,-63.3002794756086,0.));
#63409=CARTESIAN_POINT('Ctrl Pts',(30.5500630691359,-63.3002794756086,12.));
#63410=CARTESIAN_POINT('Ctrl Pts',(30.5634823022379,-63.3154400534397,0.));
#63411=CARTESIAN_POINT('Ctrl Pts',(30.5634823022379,-63.3154400534397,12.));
#63412=CARTESIAN_POINT('Ctrl Pts',(30.5769522151163,-63.3306254165126,0.));
#63413=CARTESIAN_POINT('Ctrl Pts',(30.5769522151163,-63.3306254165126,12.));
#63414=CARTESIAN_POINT('Ctrl Pts',(30.5904727493711,-63.3458353646154,0.));
#63415=CARTESIAN_POINT('Ctrl Pts',(30.5904727493711,-63.3458353646154,12.));
#63416=CARTESIAN_POINT('Ctrl Pts',(30.6040438469078,-63.3610696989577,0.));
#63417=CARTESIAN_POINT('Ctrl Pts',(30.6040438469078,-63.3610696989577,12.));
#63418=CARTESIAN_POINT('Ctrl Pts',(30.6176654515967,-63.3763282271796,0.));
#63419=CARTESIAN_POINT('Ctrl Pts',(30.6176654515967,-63.3763282271796,12.));
#63420=CARTESIAN_POINT('Ctrl Pts',(30.6313375092062,-63.3916107631376,0.));
#63421=CARTESIAN_POINT('Ctrl Pts',(30.6313375092062,-63.3916107631376,12.));
#63422=CARTESIAN_POINT('Ctrl Pts',(30.645059966612,-63.4069171245067,0.));
#63423=CARTESIAN_POINT('Ctrl Pts',(30.645059966612,-63.4069171245067,12.));
#63424=CARTESIAN_POINT('Ctrl Pts',(30.6588327712483,-63.422247131124,0.));
#63425=CARTESIAN_POINT('Ctrl Pts',(30.6588327712483,-63.422247131124,12.));
#63426=CARTESIAN_POINT('Ctrl Pts',(30.6726558704315,-63.4376006029604,0.));
#63427=CARTESIAN_POINT('Ctrl Pts',(30.6726558704315,-63.4376006029604,12.));
#63428=CARTESIAN_POINT('Ctrl Pts',(30.6865292107929,-63.4529773584249,0.));
#63429=CARTESIAN_POINT('Ctrl Pts',(30.6865292107929,-63.4529773584249,12.));
#63430=CARTESIAN_POINT('Ctrl Pts',(30.7004527385821,-63.468377215253,0.));
#63431=CARTESIAN_POINT('Ctrl Pts',(30.7004527385821,-63.468377215253,12.));
#63432=CARTESIAN_POINT('Ctrl Pts',(30.7144263999265,-63.4837999912772,0.));
#63433=CARTESIAN_POINT('Ctrl Pts',(30.7144263999265,-63.4837999912772,12.));
#63434=CARTESIAN_POINT('Ctrl Pts',(30.7284501410822,-63.4992455051795,0.));
#63435=CARTESIAN_POINT('Ctrl Pts',(30.7284501410822,-63.4992455051795,12.));
#63436=CARTESIAN_POINT('Ctrl Pts',(30.7425239087281,-63.5147135773894,0.));
#63437=CARTESIAN_POINT('Ctrl Pts',(30.7425239087281,-63.5147135773894,12.));
#63438=CARTESIAN_POINT('Ctrl Pts',(30.7566476500757,-63.5302040304142,0.));
#63439=CARTESIAN_POINT('Ctrl Pts',(30.7566476500757,-63.5302040304142,12.));
#63440=CARTESIAN_POINT('Ctrl Pts',(30.7708213127158,-63.5457166883537,0.));
#63441=CARTESIAN_POINT('Ctrl Pts',(30.7708213127158,-63.5457166883537,12.));
#63442=CARTESIAN_POINT('Ctrl Pts',(30.7850448445204,-63.5612513766,0.));
#63443=CARTESIAN_POINT('Ctrl Pts',(30.7850448445204,-63.5612513766,12.));
#63444=CARTESIAN_POINT('Ctrl Pts',(30.7993181935271,-63.5768079214882,0.));
#63445=CARTESIAN_POINT('Ctrl Pts',(30.7993181935271,-63.5768079214882,12.));
#63446=CARTESIAN_POINT('Ctrl Pts',(30.813641307801,-63.5923861498988,0.));
#63447=CARTESIAN_POINT('Ctrl Pts',(30.813641307801,-63.5923861498988,12.));
#63448=CARTESIAN_POINT('Ctrl Pts',(30.8280141354458,-63.6079858892771,0.));
#63449=CARTESIAN_POINT('Ctrl Pts',(30.8280141354458,-63.6079858892771,12.));
#63450=CARTESIAN_POINT('Ctrl Pts',(30.8424366246671,-63.6236069678055,0.));
#63451=CARTESIAN_POINT('Ctrl Pts',(30.8424366246671,-63.6236069678055,12.));
#63452=CARTESIAN_POINT('Ctrl Pts',(30.8569087238131,-63.6392492145233,0.));
#63453=CARTESIAN_POINT('Ctrl Pts',(30.8569087238131,-63.6392492145233,12.));
#63454=CARTESIAN_POINT('Ctrl Pts',(30.8714303814194,-63.6549124594666,0.));
#63455=CARTESIAN_POINT('Ctrl Pts',(30.8714303814194,-63.6549124594666,12.));
#63456=CARTESIAN_POINT('Ctrl Pts',(30.8860015462475,-63.6705965337971,0.));
#63457=CARTESIAN_POINT('Ctrl Pts',(30.8860015462475,-63.6705965337971,12.));
#63458=CARTESIAN_POINT('Ctrl Pts',(30.900622167269,-63.6863012697328,0.));
#63459=CARTESIAN_POINT('Ctrl Pts',(30.900622167269,-63.6863012697328,12.));
#63460=CARTESIAN_POINT('Ctrl Pts',(30.9152921936464,-63.7020265004792,0.));
#63461=CARTESIAN_POINT('Ctrl Pts',(30.9152921936464,-63.7020265004792,12.));
#63462=CARTESIAN_POINT('Ctrl Pts',(30.9300115747115,-63.717772060161,0.));
#63463=CARTESIAN_POINT('Ctrl Pts',(30.9300115747115,-63.717772060161,12.));
#63464=CARTESIAN_POINT('Ctrl Pts',(30.9447802599354,-63.7335377837441,0.));
#63465=CARTESIAN_POINT('Ctrl Pts',(30.9447802599354,-63.7335377837441,12.));
#63466=CARTESIAN_POINT('Ctrl Pts',(30.9595981989103,-63.7493235069871,0.));
#63467=CARTESIAN_POINT('Ctrl Pts',(30.9595981989103,-63.7493235069871,12.));
#63468=CARTESIAN_POINT('Ctrl Pts',(30.9744653413688,-63.7651290664733,0.));
#63469=CARTESIAN_POINT('Ctrl Pts',(30.9744653413688,-63.7651290664733,12.));
#63470=CARTESIAN_POINT('Ctrl Pts',(30.9893816371909,-63.7809542996264,0.));
#63471=CARTESIAN_POINT('Ctrl Pts',(30.9893816371909,-63.7809542996264,12.));
#63472=CARTESIAN_POINT('Ctrl Pts',(31.0043470364108,-63.796799044728,0.));
#63473=CARTESIAN_POINT('Ctrl Pts',(31.0043470364108,-63.796799044728,12.));
#63474=CARTESIAN_POINT('Ctrl Pts',(31.019361489217,-63.8126631409364,0.));
#63475=CARTESIAN_POINT('Ctrl Pts',(31.019361489217,-63.8126631409364,12.));
#63476=CARTESIAN_POINT('Ctrl Pts',(31.0344249459538,-63.8285464282846,0.));
#63477=CARTESIAN_POINT('Ctrl Pts',(31.0344249459538,-63.8285464282846,12.));
#63478=CARTESIAN_POINT('Ctrl Pts',(31.0495373571214,-63.8444487476611,0.));
#63479=CARTESIAN_POINT('Ctrl Pts',(31.0495373571214,-63.8444487476611,12.));
#63480=CARTESIAN_POINT('Ctrl Pts',(31.0646986733723,-63.8603699407922,0.));
#63481=CARTESIAN_POINT('Ctrl Pts',(31.0646986733723,-63.8603699407922,12.));
#63482=CARTESIAN_POINT('Ctrl Pts',(31.0799088455041,-63.8763098502237,0.));
#63483=CARTESIAN_POINT('Ctrl Pts',(31.0799088455041,-63.8763098502237,12.));
#63484=CARTESIAN_POINT('Ctrl Pts',(31.0951678244455,-63.8922683192965,0.));
#63485=CARTESIAN_POINT('Ctrl Pts',(31.0951678244455,-63.8922683192965,12.));
#63486=CARTESIAN_POINT('Ctrl Pts',(31.1104755612607,-63.9082451921448,0.));
#63487=CARTESIAN_POINT('Ctrl Pts',(31.1104755612607,-63.9082451921448,12.));
#63488=CARTESIAN_POINT('Ctrl Pts',(31.1258320071545,-63.9242403136955,0.));
#63489=CARTESIAN_POINT('Ctrl Pts',(31.1258320071545,-63.9242403136955,12.));
#63490=CARTESIAN_POINT('Ctrl Pts',(31.1412371134727,-63.9402535296651,0.));
#63491=CARTESIAN_POINT('Ctrl Pts',(31.1412371134727,-63.9402535296651,12.));
#63492=CARTESIAN_POINT('Ctrl Pts',(31.1566908316991,-63.9562846865567,0.));
#63493=CARTESIAN_POINT('Ctrl Pts',(31.1566908316991,-63.9562846865567,12.));
#63494=CARTESIAN_POINT('Ctrl Pts',(31.1721931134487,-63.9723336316551,0.));
#63495=CARTESIAN_POINT('Ctrl Pts',(31.1721931134487,-63.9723336316551,12.));
#63496=CARTESIAN_POINT('Ctrl Pts',(31.1877439104716,-63.9884002130211,0.));
#63497=CARTESIAN_POINT('Ctrl Pts',(31.1877439104716,-63.9884002130211,12.));
#63498=CARTESIAN_POINT('Ctrl Pts',(31.2033431746558,-64.0044842794832,0.));
#63499=CARTESIAN_POINT('Ctrl Pts',(31.2033431746558,-64.0044842794832,12.));
#63500=CARTESIAN_POINT('Ctrl Pts',(31.2189908580245,-64.02058568063,0.));
#63501=CARTESIAN_POINT('Ctrl Pts',(31.2189908580245,-64.02058568063,12.));
#63502=CARTESIAN_POINT('Ctrl Pts',(31.2346869127297,-64.0367042667984,0.));
#63503=CARTESIAN_POINT('Ctrl Pts',(31.2346869127297,-64.0367042667984,12.));
#63504=CARTESIAN_POINT('Ctrl Pts',(31.2504312910451,-64.0528398890657,0.));
#63505=CARTESIAN_POINT('Ctrl Pts',(31.2504312910451,-64.0528398890657,12.));
#63506=CARTESIAN_POINT('Ctrl Pts',(31.2662239453728,-64.0689923992461,0.));
#63507=CARTESIAN_POINT('Ctrl Pts',(31.2662239453728,-64.0689923992461,12.));
#63508=CARTESIAN_POINT('Ctrl Pts',(31.2820648282447,-64.0851616498853,0.));
#63509=CARTESIAN_POINT('Ctrl Pts',(31.2820648282447,-64.0851616498853,12.));
#63510=CARTESIAN_POINT('Ctrl Pts',(31.2979538923214,-64.1013474942557,0.));
#63511=CARTESIAN_POINT('Ctrl Pts',(31.2979538923214,-64.1013474942557,12.));
#63512=CARTESIAN_POINT('Ctrl Pts',(31.3138910903858,-64.1175497863491,0.));
#63513=CARTESIAN_POINT('Ctrl Pts',(31.3138910903858,-64.1175497863491,12.));
#63514=CARTESIAN_POINT('Ctrl Pts',(31.3298763753376,-64.1337683808691,0.));
#63515=CARTESIAN_POINT('Ctrl Pts',(31.3298763753376,-64.1337683808691,12.));
#63516=CARTESIAN_POINT('Ctrl Pts',(31.3459097002006,-64.1500031332282,0.));
#63517=CARTESIAN_POINT('Ctrl Pts',(31.3459097002006,-64.1500031332282,12.));
#63518=CARTESIAN_POINT('Ctrl Pts',(31.3619910181228,-64.166253899542,0.));
#63519=CARTESIAN_POINT('Ctrl Pts',(31.3619910181228,-64.166253899542,12.));
#63520=CARTESIAN_POINT('Ctrl Pts',(31.3781202823754,-64.1825205366225,0.));
#63521=CARTESIAN_POINT('Ctrl Pts',(31.3781202823754,-64.1825205366225,12.));
#63522=CARTESIAN_POINT('Ctrl Pts',(31.3942974463445,-64.1988029019707,0.));
#63523=CARTESIAN_POINT('Ctrl Pts',(31.3942974463445,-64.1988029019707,12.));
#63524=CARTESIAN_POINT('Ctrl Pts',(31.410522463528,-64.2151008537697,0.));
#63525=CARTESIAN_POINT('Ctrl Pts',(31.410522463528,-64.2151008537697,12.));
#63526=CARTESIAN_POINT('Ctrl Pts',(31.4267952875423,-64.231414250881,0.));
#63527=CARTESIAN_POINT('Ctrl Pts',(31.4267952875423,-64.231414250881,12.));
#63528=CARTESIAN_POINT('Ctrl Pts',(31.4431158721221,-64.2477429528393,0.));
#63529=CARTESIAN_POINT('Ctrl Pts',(31.4431158721221,-64.2477429528393,12.));
#63530=CARTESIAN_POINT('Ctrl Pts',(31.4594841711194,-64.2640868198473,0.));
#63531=CARTESIAN_POINT('Ctrl Pts',(31.4594841711194,-64.2640868198473,12.));
#63532=CARTESIAN_POINT('Ctrl Pts',(31.4759001384941,-64.2804457127671,0.));
#63533=CARTESIAN_POINT('Ctrl Pts',(31.4759001384941,-64.2804457127671,12.));
#63534=CARTESIAN_POINT('Ctrl Pts',(31.4923637283131,-64.2968194931158,0.));
#63535=CARTESIAN_POINT('Ctrl Pts',(31.4923637283131,-64.2968194931158,12.));
#63536=CARTESIAN_POINT('Ctrl Pts',(31.5088748947582,-64.3132080230637,0.));
#63537=CARTESIAN_POINT('Ctrl Pts',(31.5088748947582,-64.3132080230637,12.));
#63538=CARTESIAN_POINT('Ctrl Pts',(31.5254335921245,-64.3296111654283,0.));
#63539=CARTESIAN_POINT('Ctrl Pts',(31.5254335921245,-64.3296111654283,12.));
#63540=CARTESIAN_POINT('Ctrl Pts',(31.5420397748191,-64.3460287836687,0.));
#63541=CARTESIAN_POINT('Ctrl Pts',(31.5420397748191,-64.3460287836687,12.));
#63542=CARTESIAN_POINT('Ctrl Pts',(31.5586933973515,-64.3624607418769,0.));
#63543=CARTESIAN_POINT('Ctrl Pts',(31.5586933973515,-64.3624607418769,12.));
#63544=CARTESIAN_POINT('Ctrl Pts',(31.5753944143336,-64.3789069047734,0.));
#63545=CARTESIAN_POINT('Ctrl Pts',(31.5753944143336,-64.3789069047734,12.));
#63546=CARTESIAN_POINT('Ctrl Pts',(31.5921427804865,-64.3953671377046,0.));
#63547=CARTESIAN_POINT('Ctrl Pts',(31.5921427804865,-64.3953671377046,12.));
#63548=CARTESIAN_POINT('Ctrl Pts',(31.6089384506395,-64.4118413066378,0.));
#63549=CARTESIAN_POINT('Ctrl Pts',(31.6089384506395,-64.4118413066378,12.));
#63550=CARTESIAN_POINT('Ctrl Pts',(31.6257813797287,-64.4283292781565,0.));
#63551=CARTESIAN_POINT('Ctrl Pts',(31.6257813797287,-64.4283292781565,12.));
#63552=CARTESIAN_POINT('Ctrl Pts',(31.6426715227878,-64.4448309194525,0.));
#63553=CARTESIAN_POINT('Ctrl Pts',(31.6426715227878,-64.4448309194525,12.));
#63554=CARTESIAN_POINT('Ctrl Pts',(31.6596088349481,-64.4613460983214,0.));
#63555=CARTESIAN_POINT('Ctrl Pts',(31.6596088349481,-64.4613460983214,12.));
#63556=CARTESIAN_POINT('Ctrl Pts',(31.6765932714464,-64.4778746831614,0.));
#63557=CARTESIAN_POINT('Ctrl Pts',(31.6765932714464,-64.4778746831614,12.));
#63558=CARTESIAN_POINT('Ctrl Pts',(31.6936247876228,-64.4944165429675,0.));
#63559=CARTESIAN_POINT('Ctrl Pts',(31.6936247876228,-64.4944165429675,12.));
#63560=CARTESIAN_POINT('Ctrl Pts',(31.71070333892,-64.510971547327,0.));
#63561=CARTESIAN_POINT('Ctrl Pts',(31.71070333892,-64.510971547327,12.));
#63562=CARTESIAN_POINT('Ctrl Pts',(31.7278288808731,-64.5275395664124,0.));
#63563=CARTESIAN_POINT('Ctrl Pts',(31.7278288808731,-64.5275395664124,12.));
#63564=CARTESIAN_POINT('Ctrl Pts',(31.7450013691111,-64.544120470977,0.));
#63565=CARTESIAN_POINT('Ctrl Pts',(31.7450013691111,-64.544120470977,12.));
#63566=CARTESIAN_POINT('Ctrl Pts',(31.7622207593634,-64.5607141323521,0.));
#63567=CARTESIAN_POINT('Ctrl Pts',(31.7622207593634,-64.5607141323521,12.));
#63568=CARTESIAN_POINT('Ctrl Pts',(31.7794870074583,-64.5773204224429,0.));
#63569=CARTESIAN_POINT('Ctrl Pts',(31.7794870074583,-64.5773204224429,12.));
#63570=CARTESIAN_POINT('Ctrl Pts',(31.7968000693218,-64.5939392137235,0.));
#63571=CARTESIAN_POINT('Ctrl Pts',(31.7968000693218,-64.5939392137235,12.));
#63572=CARTESIAN_POINT('Ctrl Pts',(31.8141599009684,-64.6105703792312,0.));
#63573=CARTESIAN_POINT('Ctrl Pts',(31.8141599009684,-64.6105703792312,12.));
#63574=CARTESIAN_POINT('Ctrl Pts',(31.8315664585025,-64.6272137925627,0.));
#63575=CARTESIAN_POINT('Ctrl Pts',(31.8315664585025,-64.6272137925627,12.));
#63576=CARTESIAN_POINT('Ctrl Pts',(31.8490196981248,-64.6438693278714,0.));
#63577=CARTESIAN_POINT('Ctrl Pts',(31.8490196981248,-64.6438693278714,12.));
#63578=CARTESIAN_POINT('Ctrl Pts',(31.866519576131,-64.6605368598629,0.));
#63579=CARTESIAN_POINT('Ctrl Pts',(31.866519576131,-64.6605368598629,12.));
#63580=CARTESIAN_POINT('Ctrl Pts',(31.8840660489106,-64.6772162637907,0.));
#63581=CARTESIAN_POINT('Ctrl Pts',(31.8840660489106,-64.6772162637907,12.));
#63582=CARTESIAN_POINT('Ctrl Pts',(31.9016590729373,-64.6939074154498,0.));
#63583=CARTESIAN_POINT('Ctrl Pts',(31.9016590729373,-64.6939074154498,12.));
#63584=CARTESIAN_POINT('Ctrl Pts',(31.9192986047705,-64.7106101911732,0.));
#63585=CARTESIAN_POINT('Ctrl Pts',(31.9192986047705,-64.7106101911732,12.));
#63586=CARTESIAN_POINT('Ctrl Pts',(31.9369846010615,-64.7273244678297,0.));
#63587=CARTESIAN_POINT('Ctrl Pts',(31.9369846010615,-64.7273244678297,12.));
#63588=CARTESIAN_POINT('Ctrl Pts',(31.9547170185533,-64.7440501228203,0.));
#63589=CARTESIAN_POINT('Ctrl Pts',(31.9547170185533,-64.7440501228203,12.));
#63590=CARTESIAN_POINT('Ctrl Pts',(31.9724958140789,-64.7607870340735,0.));
#63591=CARTESIAN_POINT('Ctrl Pts',(31.9724958140789,-64.7607870340735,12.));
#63592=CARTESIAN_POINT('Ctrl Pts',(31.9903209445519,-64.7775350800401,0.));
#63593=CARTESIAN_POINT('Ctrl Pts',(31.9903209445519,-64.7775350800401,12.));
#63594=CARTESIAN_POINT('Ctrl Pts',(32.0081923669676,-64.7942941396881,0.));
#63595=CARTESIAN_POINT('Ctrl Pts',(32.0081923669676,-64.7942941396881,12.));
#63596=CARTESIAN_POINT('Ctrl Pts',(32.0261100384092,-64.8110640925021,0.));
#63597=CARTESIAN_POINT('Ctrl Pts',(32.0261100384092,-64.8110640925021,12.));
#63598=CARTESIAN_POINT('Ctrl Pts',(32.0440739160477,-64.8278448184787,0.));
#63599=CARTESIAN_POINT('Ctrl Pts',(32.0440739160477,-64.8278448184787,12.));
#63600=CARTESIAN_POINT('Ctrl Pts',(32.0620839571408,-64.8446361981234,0.));
#63601=CARTESIAN_POINT('Ctrl Pts',(32.0620839571408,-64.8446361981234,12.));
#63602=CARTESIAN_POINT('Ctrl Pts',(32.0801401190241,-64.861438112445,0.));
#63603=CARTESIAN_POINT('Ctrl Pts',(32.0801401190241,-64.861438112445,12.));
#63604=CARTESIAN_POINT('Ctrl Pts',(32.0982423591108,-64.878250442952,0.));
#63605=CARTESIAN_POINT('Ctrl Pts',(32.0982423591108,-64.878250442952,12.));
#63606=CARTESIAN_POINT('Ctrl Pts',(32.1163906348979,-64.8950730716493,0.));
#63607=CARTESIAN_POINT('Ctrl Pts',(32.1163906348979,-64.8950730716493,12.));
#63608=CARTESIAN_POINT('Ctrl Pts',(32.1345849039671,-64.9119058810362,0.));
#63609=CARTESIAN_POINT('Ctrl Pts',(32.1345849039671,-64.9119058810362,12.));
#63610=CARTESIAN_POINT('Ctrl Pts',(32.1528251239831,-64.9287487541019,0.));
#63611=CARTESIAN_POINT('Ctrl Pts',(32.1528251239831,-64.9287487541019,12.));
#63612=CARTESIAN_POINT('Ctrl Pts',(32.1711112526859,-64.9456015743203,0.));
#63613=CARTESIAN_POINT('Ctrl Pts',(32.1711112526859,-64.9456015743203,12.));
#63614=CARTESIAN_POINT('Ctrl Pts',(32.1894432478888,-64.9624642256478,0.));
#63615=CARTESIAN_POINT('Ctrl Pts',(32.1894432478888,-64.9624642256478,12.));
#63616=CARTESIAN_POINT('Ctrl Pts',(32.2078210674857,-64.9793365925194,0.));
#63617=CARTESIAN_POINT('Ctrl Pts',(32.2078210674857,-64.9793365925194,12.));
#63618=CARTESIAN_POINT('Ctrl Pts',(32.2262446694516,-64.996218559847,0.));
#63619=CARTESIAN_POINT('Ctrl Pts',(32.2262446694516,-64.996218559847,12.));
#63620=CARTESIAN_POINT('Ctrl Pts',(32.244714011842,-65.0131100130155,0.));
#63621=CARTESIAN_POINT('Ctrl Pts',(32.244714011842,-65.0131100130155,12.));
#63622=CARTESIAN_POINT('Ctrl Pts',(32.2632290527854,-65.0300108378786,0.));
#63623=CARTESIAN_POINT('Ctrl Pts',(32.2632290527854,-65.0300108378786,12.));
#63624=CARTESIAN_POINT('Ctrl Pts',(32.2817897504799,-65.0469209207548,0.));
#63625=CARTESIAN_POINT('Ctrl Pts',(32.2817897504799,-65.0469209207548,12.));
#63626=CARTESIAN_POINT('Ctrl Pts',(32.3003960632,-65.0638401484245,0.));
#63627=CARTESIAN_POINT('Ctrl Pts',(32.3003960632,-65.0638401484245,12.));
#63628=CARTESIAN_POINT('Ctrl Pts',(32.3190479492985,-65.0807684081278,0.));
#63629=CARTESIAN_POINT('Ctrl Pts',(32.3190479492985,-65.0807684081278,12.));
#63630=CARTESIAN_POINT('Ctrl Pts',(32.3377453672051,-65.097705587561,0.));
#63631=CARTESIAN_POINT('Ctrl Pts',(32.3377453672051,-65.097705587561,12.));
#63632=CARTESIAN_POINT('Ctrl Pts',(32.3564882754212,-65.1146515748723,0.));
#63633=CARTESIAN_POINT('Ctrl Pts',(32.3564882754212,-65.1146515748723,12.));
#63634=CARTESIAN_POINT('Ctrl Pts',(32.3752766325134,-65.1316062586586,0.));
#63635=CARTESIAN_POINT('Ctrl Pts',(32.3752766325134,-65.1316062586586,12.));
#63636=CARTESIAN_POINT('Ctrl Pts',(32.3941103971218,-65.1485695279628,0.));
#63637=CARTESIAN_POINT('Ctrl Pts',(32.3941103971218,-65.1485695279628,12.));
#63638=CARTESIAN_POINT('Ctrl Pts',(32.4129895279612,-65.165541272272,0.));
#63639=CARTESIAN_POINT('Ctrl Pts',(32.4129895279612,-65.165541272272,12.));
#63640=CARTESIAN_POINT('Ctrl Pts',(32.4319139838212,-65.182521381514,0.));
#63641=CARTESIAN_POINT('Ctrl Pts',(32.4319139838212,-65.182521381514,12.));
#63642=CARTESIAN_POINT('Ctrl Pts',(32.4508837235613,-65.1995097460546,0.));
#63643=CARTESIAN_POINT('Ctrl Pts',(32.4508837235613,-65.1995097460546,12.));
#63644=CARTESIAN_POINT('Ctrl Pts',(32.4698987061036,-65.2165062566936,0.));
#63645=CARTESIAN_POINT('Ctrl Pts',(32.4698987061036,-65.2165062566936,12.));
#63646=CARTESIAN_POINT('Ctrl Pts',(32.4889588904396,-65.2335108046625,0.));
#63647=CARTESIAN_POINT('Ctrl Pts',(32.4889588904396,-65.2335108046625,12.));
#63648=CARTESIAN_POINT('Ctrl Pts',(32.508064235633,-65.2505232816215,0.));
#63649=CARTESIAN_POINT('Ctrl Pts',(32.508064235633,-65.2505232816215,12.));
#63650=CARTESIAN_POINT('Ctrl Pts',(32.527214700819,-65.2675435796558,0.));
#63651=CARTESIAN_POINT('Ctrl Pts',(32.527214700819,-65.2675435796558,12.));
#63652=CARTESIAN_POINT('Ctrl Pts',(32.5464102452013,-65.2845715912717,0.));
#63653=CARTESIAN_POINT('Ctrl Pts',(32.5464102452013,-65.2845715912717,12.));
#63654=CARTESIAN_POINT('Ctrl Pts',(32.565650828042,-65.3016072093908,0.));
#63655=CARTESIAN_POINT('Ctrl Pts',(32.565650828042,-65.3016072093908,12.));
#63656=CARTESIAN_POINT('Ctrl Pts',(32.5849364086678,-65.3186503273498,0.));
#63657=CARTESIAN_POINT('Ctrl Pts',(32.5849364086678,-65.3186503273498,12.));
#63658=CARTESIAN_POINT('Ctrl Pts',(32.6042669464751,-65.3357008389005,0.));
#63659=CARTESIAN_POINT('Ctrl Pts',(32.6042669464751,-65.3357008389005,12.));
#63660=CARTESIAN_POINT('Ctrl Pts',(32.6236424009301,-65.3527586382082,0.));
#63661=CARTESIAN_POINT('Ctrl Pts',(32.6236424009301,-65.3527586382082,12.));
#63662=CARTESIAN_POINT('Ctrl Pts',(32.6430627315672,-65.3698236198512,0.));
#63663=CARTESIAN_POINT('Ctrl Pts',(32.6430627315672,-65.3698236198512,12.));
#63664=CARTESIAN_POINT('Ctrl Pts',(32.6625278979807,-65.3868956788178,0.));
#63665=CARTESIAN_POINT('Ctrl Pts',(32.6625278979807,-65.3868956788178,12.));
#63666=CARTESIAN_POINT('Ctrl Pts',(32.6820378598262,-65.4039747105033,0.));
#63667=CARTESIAN_POINT('Ctrl Pts',(32.6820378598262,-65.4039747105033,12.));
#63668=CARTESIAN_POINT('Ctrl Pts',(32.701592576826,-65.421060610703,0.));
#63669=CARTESIAN_POINT('Ctrl Pts',(32.701592576826,-65.421060610703,12.));
#63670=CARTESIAN_POINT('Ctrl Pts',(32.7211920087681,-65.4381532756063,0.));
#63671=CARTESIAN_POINT('Ctrl Pts',(32.7211920087681,-65.4381532756063,12.));
#63672=CARTESIAN_POINT('Ctrl Pts',(32.7408361155037,-65.4552526017907,0.));
#63673=CARTESIAN_POINT('Ctrl Pts',(32.7408361155037,-65.4552526017907,12.));
#63674=CARTESIAN_POINT('Ctrl Pts',(32.7605248569382,-65.4723584862129,0.));
#63675=CARTESIAN_POINT('Ctrl Pts',(32.7605248569382,-65.4723584862129,12.));
#63676=CARTESIAN_POINT('Ctrl Pts',(32.7802581930293,-65.4894708262071,0.));
#63677=CARTESIAN_POINT('Ctrl Pts',(32.7802581930293,-65.4894708262071,12.));
#63678=CARTESIAN_POINT('Ctrl Pts',(32.800036083798,-65.5065895194939,0.));
#63679=CARTESIAN_POINT('Ctrl Pts',(32.800036083798,-65.5065895194939,12.));
#63680=CARTESIAN_POINT('Ctrl Pts',(32.8198584893318,-65.5237144641864,0.));
#63681=CARTESIAN_POINT('Ctrl Pts',(32.8198584893318,-65.5237144641864,12.));
#63682=CARTESIAN_POINT('Ctrl Pts',(32.8397253697864,-65.5408455587963,0.));
#63683=CARTESIAN_POINT('Ctrl Pts',(32.8397253697864,-65.5408455587963,12.));
#63684=CARTESIAN_POINT('Ctrl Pts',(32.8596366853826,-65.5579827022413,0.));
#63685=CARTESIAN_POINT('Ctrl Pts',(32.8596366853826,-65.5579827022413,12.));
#63686=CARTESIAN_POINT('Ctrl Pts',(32.8795923964021,-65.575125793846,0.));
#63687=CARTESIAN_POINT('Ctrl Pts',(32.8795923964021,-65.575125793846,12.));
#63688=CARTESIAN_POINT('Ctrl Pts',(32.899592463189,-65.5922747333182,0.));
#63689=CARTESIAN_POINT('Ctrl Pts',(32.899592463189,-65.5922747333182,12.));
#63690=CARTESIAN_POINT('Ctrl Pts',(32.9196368461457,-65.6094294207267,0.));
#63691=CARTESIAN_POINT('Ctrl Pts',(32.9196368461457,-65.6094294207267,12.));
#63692=CARTESIAN_POINT('Ctrl Pts',(32.9397255057273,-65.6265897564782,0.));
#63693=CARTESIAN_POINT('Ctrl Pts',(32.9397255057273,-65.6265897564782,12.));
#63694=CARTESIAN_POINT('Ctrl Pts',(32.9598584024317,-65.6437556412956,0.));
#63695=CARTESIAN_POINT('Ctrl Pts',(32.9598584024317,-65.6437556412956,12.));
#63696=CARTESIAN_POINT('Ctrl Pts',(32.9800354967846,-65.6609269761902,0.));
#63697=CARTESIAN_POINT('Ctrl Pts',(32.9800354967846,-65.6609269761902,12.));
#63698=CARTESIAN_POINT('Ctrl Pts',(33.000256749358,-65.6781036625041,0.));
#63699=CARTESIAN_POINT('Ctrl Pts',(33.000256749358,-65.6781036625041,12.));
#63700=CARTESIAN_POINT('Ctrl Pts',(33.0205221207877,-65.6952856019542,0.));
#63701=CARTESIAN_POINT('Ctrl Pts',(33.0205221207877,-65.6952856019542,12.));
#63702=CARTESIAN_POINT('Ctrl Pts',(33.0408315717874,-65.7124726966805,0.));
#63703=CARTESIAN_POINT('Ctrl Pts',(33.0408315717874,-65.7124726966805,12.));
#63704=CARTESIAN_POINT('Ctrl Pts',(33.0611850631579,-65.729664849282,0.));
#63705=CARTESIAN_POINT('Ctrl Pts',(33.0611850631579,-65.729664849282,12.));
#63706=CARTESIAN_POINT('Ctrl Pts',(33.0815825557976,-65.7468619628808,0.));
#63707=CARTESIAN_POINT('Ctrl Pts',(33.0815825557976,-65.7468619628808,12.));
#63708=CARTESIAN_POINT('Ctrl Pts',(33.102024010688,-65.7640639410653,0.));
#63709=CARTESIAN_POINT('Ctrl Pts',(33.102024010688,-65.7640639410653,12.));
#63710=CARTESIAN_POINT('Ctrl Pts',(33.1225093888668,-65.7812706877691,0.));
#63711=CARTESIAN_POINT('Ctrl Pts',(33.1225093888668,-65.7812706877691,12.));
#63712=CARTESIAN_POINT('Ctrl Pts',(33.1430386513975,-65.7984821071622,0.));
#63713=CARTESIAN_POINT('Ctrl Pts',(33.1430386513975,-65.7984821071622,12.));
#63714=CARTESIAN_POINT('Ctrl Pts',(33.16361175934,-65.8156981035504,0.));
#63715=CARTESIAN_POINT('Ctrl Pts',(33.16361175934,-65.8156981035504,12.));
#63716=CARTESIAN_POINT('Ctrl Pts',(33.1842286737053,-65.8329185812379,0.));
#63717=CARTESIAN_POINT('Ctrl Pts',(33.1842286737053,-65.8329185812379,12.));
#63718=CARTESIAN_POINT('Ctrl Pts',(33.2048893554495,-65.8501434445174,0.));
#63719=CARTESIAN_POINT('Ctrl Pts',(33.2048893554495,-65.8501434445174,12.));
#63720=CARTESIAN_POINT('Ctrl Pts',(33.2255937655655,-65.8673725979591,0.));
#63721=CARTESIAN_POINT('Ctrl Pts',(33.2255937655655,-65.8673725979591,12.));
#63722=CARTESIAN_POINT('Ctrl Pts',(33.2463418651497,-65.8846059466382,0.));
#63723=CARTESIAN_POINT('Ctrl Pts',(33.2463418651497,-65.8846059466382,12.));
#63724=CARTESIAN_POINT('Ctrl Pts',(33.2671336154754,-65.901843396389,0.));
#63725=CARTESIAN_POINT('Ctrl Pts',(33.2671336154754,-65.901843396389,12.));
#63726=CARTESIAN_POINT('Ctrl Pts',(33.2879689780566,-65.9190848540422,0.));
#63727=CARTESIAN_POINT('Ctrl Pts',(33.2879689780566,-65.9190848540422,12.));
#63728=CARTESIAN_POINT('Ctrl Pts',(33.308847914715,-65.9363302276822,0.));
#63729=CARTESIAN_POINT('Ctrl Pts',(33.308847914715,-65.9363302276822,12.));
#63730=CARTESIAN_POINT('Ctrl Pts',(33.3297703874249,-65.9535794260802,0.));
#63731=CARTESIAN_POINT('Ctrl Pts',(33.3297703874249,-65.9535794260802,12.));
#63732=CARTESIAN_POINT('Ctrl Pts',(33.3507363581578,-65.9708323581386,0.));
#63733=CARTESIAN_POINT('Ctrl Pts',(33.3507363581578,-65.9708323581386,12.));
#63734=CARTESIAN_POINT('Ctrl Pts',(33.3717457887094,-65.9880889322822,0.));
#63735=CARTESIAN_POINT('Ctrl Pts',(33.3717457887094,-65.9880889322822,12.));
#63736=CARTESIAN_POINT('Ctrl Pts',(33.3927986405612,-66.0053490559826,0.));
#63737=CARTESIAN_POINT('Ctrl Pts',(33.3927986405612,-66.0053490559826,12.));
#63738=CARTESIAN_POINT('Ctrl Pts',(33.4138948746407,-66.0226126349482,0.));
#63739=CARTESIAN_POINT('Ctrl Pts',(33.4138948746407,-66.0226126349482,12.));
#63740=CARTESIAN_POINT('Ctrl Pts',(33.4350344515128,-66.0398795737827,0.));
#63741=CARTESIAN_POINT('Ctrl Pts',(33.4350344515128,-66.0398795737827,12.));
#63742=CARTESIAN_POINT('Ctrl Pts',(33.4562173318052,-66.0571497774484,0.));
#63743=CARTESIAN_POINT('Ctrl Pts',(33.4562173318052,-66.0571497774484,12.));
#63744=CARTESIAN_POINT('Ctrl Pts',(33.4774434765761,-66.0744231525445,0.));
#63745=CARTESIAN_POINT('Ctrl Pts',(33.4774434765761,-66.0744231525445,12.));
#63746=CARTESIAN_POINT('Ctrl Pts',(33.4987128476617,-66.0916996085237,0.));
#63747=CARTESIAN_POINT('Ctrl Pts',(33.4987128476617,-66.0916996085237,12.));
#63748=CARTESIAN_POINT('Ctrl Pts',(33.5200254081212,-66.1089790592673,0.));
#63749=CARTESIAN_POINT('Ctrl Pts',(33.5200254081212,-66.1089790592673,12.));
#63750=CARTESIAN_POINT('Ctrl Pts',(33.5413811223397,-66.1262614234579,0.));
#63751=CARTESIAN_POINT('Ctrl Pts',(33.5413811223397,-66.1262614234579,12.));
#63752=CARTESIAN_POINT('Ctrl Pts',(33.5627799550422,-66.1435466210967,0.));
#63753=CARTESIAN_POINT('Ctrl Pts',(33.5627799550422,-66.1435466210967,12.));
#63754=CARTESIAN_POINT('Ctrl Pts',(33.5842218705103,-66.1608345707552,0.));
#63755=CARTESIAN_POINT('Ctrl Pts',(33.5842218705103,-66.1608345707552,12.));
#63756=CARTESIAN_POINT('Ctrl Pts',(33.6057068316758,-66.1781251863998,0.));
#63757=CARTESIAN_POINT('Ctrl Pts',(33.6057068316758,-66.1781251863998,12.));
#63758=CARTESIAN_POINT('Ctrl Pts',(33.6272347993519,-66.1954183747167,0.));
#63759=CARTESIAN_POINT('Ctrl Pts',(33.6272347993519,-66.1954183747167,12.));
#63760=CARTESIAN_POINT('Ctrl Pts',(33.648805731163,-66.2127140313777,0.));
#63761=CARTESIAN_POINT('Ctrl Pts',(33.648805731163,-66.2127140313777,12.));
#63762=CARTESIAN_POINT('Ctrl Pts',(33.6704195830525,-66.2300120464323,0.));
#63763=CARTESIAN_POINT('Ctrl Pts',(33.6704195830525,-66.2300120464323,12.));
#63764=CARTESIAN_POINT('Ctrl Pts',(33.6920763111575,-66.2473123109627,0.));
#63765=CARTESIAN_POINT('Ctrl Pts',(33.6920763111575,-66.2473123109627,12.));
#63766=CARTESIAN_POINT('Ctrl Pts',(33.713775873597,-66.2646147235444,0.));
#63767=CARTESIAN_POINT('Ctrl Pts',(33.713775873597,-66.2646147235444,12.));
#63768=CARTESIAN_POINT('Ctrl Pts',(33.7355182321862,-66.2819191962273,0.));
#63769=CARTESIAN_POINT('Ctrl Pts',(33.7355182321862,-66.2819191962273,12.));
#63770=CARTESIAN_POINT('Ctrl Pts',(33.7573033544373,-66.2992256621001,0.));
#63771=CARTESIAN_POINT('Ctrl Pts',(33.7573033544373,-66.2992256621001,12.));
#63772=CARTESIAN_POINT('Ctrl Pts',(33.7791312144798,-66.3165340771053,0.));
#63773=CARTESIAN_POINT('Ctrl Pts',(33.7791312144798,-66.3165340771053,12.));
#63774=CARTESIAN_POINT('Ctrl Pts',(33.8010017925666,-66.333844414356,0.));
#63775=CARTESIAN_POINT('Ctrl Pts',(33.8010017925666,-66.333844414356,12.));
#63776=CARTESIAN_POINT('Ctrl Pts',(33.8185324184601,-66.3476942111456,0.));
#63777=CARTESIAN_POINT('Ctrl Pts',(33.8185324184601,-66.3476942111456,12.));
#63778=CARTESIAN_POINT('Ctrl Pts',(33.831699601175,-66.3580824155565,0.));
#63779=CARTESIAN_POINT('Ctrl Pts',(33.831699601175,-66.3580824155565,12.));
#63780=CARTESIAN_POINT('Ctrl Pts',(33.8404862618803,-66.3650082659593,0.));
#63781=CARTESIAN_POINT('Ctrl Pts',(33.8404862618803,-66.3650082659593,12.));
#63782=CARTESIAN_POINT('Ctrl Pts',(33.8448817269567,-66.3684712863594,0.));
#63783=CARTESIAN_POINT('Ctrl Pts',(33.8448817269567,-66.3684712863594,12.));
#63784=CARTESIAN_POINT('',(30.354906545781,-63.0759831361898,0.));
#63785=CARTESIAN_POINT('Ctrl Pts',(30.354906545781,-63.0759831361898,0.));
#63786=CARTESIAN_POINT('Ctrl Pts',(30.3574319069329,-63.078933570069,0.));
#63787=CARTESIAN_POINT('Ctrl Pts',(30.362487768065,-63.0848371718048,0.));
#63788=CARTESIAN_POINT('Ctrl Pts',(30.3700869762507,-63.0937007763471,0.));
#63789=CARTESIAN_POINT('Ctrl Pts',(30.3802500880402,-63.105535320226,0.));
#63790=CARTESIAN_POINT('Ctrl Pts',(30.3930053710484,-63.1203558300657,0.));
#63791=CARTESIAN_POINT('Ctrl Pts',(30.4058120432228,-63.1352036298441,0.));
#63792=CARTESIAN_POINT('Ctrl Pts',(30.418670087563,-63.1500786361459,0.));
#63793=CARTESIAN_POINT('Ctrl Pts',(30.431579465973,-63.164980701691,0.));
#63794=CARTESIAN_POINT('Ctrl Pts',(30.444540119238,-63.179909617189,0.));
#63795=CARTESIAN_POINT('Ctrl Pts',(30.4575519763336,-63.1948651386942,0.));
#63796=CARTESIAN_POINT('Ctrl Pts',(30.4706149614159,-63.2098470086636,0.));
#63797=CARTESIAN_POINT('Ctrl Pts',(30.4837290014989,-63.2248549788222,0.));
#63798=CARTESIAN_POINT('Ctrl Pts',(30.4968940344997,-63.2398888342546,0.));
#63799=CARTESIAN_POINT('Ctrl Pts',(30.5101100066659,-63.2549483856215,0.));
#63800=CARTESIAN_POINT('Ctrl Pts',(30.5233768687864,-63.2700334577639,0.));
#63801=CARTESIAN_POINT('Ctrl Pts',(30.5366945730508,-63.2851438802474,0.));
#63802=CARTESIAN_POINT('Ctrl Pts',(30.5500630691359,-63.3002794756086,0.));
#63803=CARTESIAN_POINT('Ctrl Pts',(30.5634823022379,-63.3154400534397,0.));
#63804=CARTESIAN_POINT('Ctrl Pts',(30.5769522151163,-63.3306254165126,0.));
#63805=CARTESIAN_POINT('Ctrl Pts',(30.5904727493711,-63.3458353646154,0.));
#63806=CARTESIAN_POINT('Ctrl Pts',(30.6040438469078,-63.3610696989577,0.));
#63807=CARTESIAN_POINT('Ctrl Pts',(30.6176654515967,-63.3763282271796,0.));
#63808=CARTESIAN_POINT('Ctrl Pts',(30.6313375092062,-63.3916107631376,0.));
#63809=CARTESIAN_POINT('Ctrl Pts',(30.645059966612,-63.4069171245067,0.));
#63810=CARTESIAN_POINT('Ctrl Pts',(30.6588327712483,-63.422247131124,0.));
#63811=CARTESIAN_POINT('Ctrl Pts',(30.6726558704315,-63.4376006029604,0.));
#63812=CARTESIAN_POINT('Ctrl Pts',(30.6865292107929,-63.4529773584249,0.));
#63813=CARTESIAN_POINT('Ctrl Pts',(30.7004527385821,-63.468377215253,0.));
#63814=CARTESIAN_POINT('Ctrl Pts',(30.7144263999265,-63.4837999912772,0.));
#63815=CARTESIAN_POINT('Ctrl Pts',(30.7284501410822,-63.4992455051795,0.));
#63816=CARTESIAN_POINT('Ctrl Pts',(30.7425239087281,-63.5147135773894,0.));
#63817=CARTESIAN_POINT('Ctrl Pts',(30.7566476500757,-63.5302040304142,0.));
#63818=CARTESIAN_POINT('Ctrl Pts',(30.7708213127158,-63.5457166883537,0.));
#63819=CARTESIAN_POINT('Ctrl Pts',(30.7850448445204,-63.5612513766,0.));
#63820=CARTESIAN_POINT('Ctrl Pts',(30.7993181935271,-63.5768079214882,0.));
#63821=CARTESIAN_POINT('Ctrl Pts',(30.813641307801,-63.5923861498988,0.));
#63822=CARTESIAN_POINT('Ctrl Pts',(30.8280141354458,-63.6079858892771,0.));
#63823=CARTESIAN_POINT('Ctrl Pts',(30.8424366246671,-63.6236069678055,0.));
#63824=CARTESIAN_POINT('Ctrl Pts',(30.8569087238131,-63.6392492145233,0.));
#63825=CARTESIAN_POINT('Ctrl Pts',(30.8714303814194,-63.6549124594666,0.));
#63826=CARTESIAN_POINT('Ctrl Pts',(30.8860015462475,-63.6705965337971,0.));
#63827=CARTESIAN_POINT('Ctrl Pts',(30.900622167269,-63.6863012697328,0.));
#63828=CARTESIAN_POINT('Ctrl Pts',(30.9152921936464,-63.7020265004792,0.));
#63829=CARTESIAN_POINT('Ctrl Pts',(30.9300115747115,-63.717772060161,0.));
#63830=CARTESIAN_POINT('Ctrl Pts',(30.9447802599354,-63.7335377837441,0.));
#63831=CARTESIAN_POINT('Ctrl Pts',(30.9595981989103,-63.7493235069871,0.));
#63832=CARTESIAN_POINT('Ctrl Pts',(30.9744653413688,-63.7651290664733,0.));
#63833=CARTESIAN_POINT('Ctrl Pts',(30.9893816371909,-63.7809542996264,0.));
#63834=CARTESIAN_POINT('Ctrl Pts',(31.0043470364108,-63.796799044728,0.));
#63835=CARTESIAN_POINT('Ctrl Pts',(31.019361489217,-63.8126631409364,0.));
#63836=CARTESIAN_POINT('Ctrl Pts',(31.0344249459538,-63.8285464282846,0.));
#63837=CARTESIAN_POINT('Ctrl Pts',(31.0495373571214,-63.8444487476611,0.));
#63838=CARTESIAN_POINT('Ctrl Pts',(31.0646986733723,-63.8603699407922,0.));
#63839=CARTESIAN_POINT('Ctrl Pts',(31.0799088455041,-63.8763098502237,0.));
#63840=CARTESIAN_POINT('Ctrl Pts',(31.0951678244455,-63.8922683192965,0.));
#63841=CARTESIAN_POINT('Ctrl Pts',(31.1104755612607,-63.9082451921448,0.));
#63842=CARTESIAN_POINT('Ctrl Pts',(31.1258320071545,-63.9242403136955,0.));
#63843=CARTESIAN_POINT('Ctrl Pts',(31.1412371134727,-63.9402535296651,0.));
#63844=CARTESIAN_POINT('Ctrl Pts',(31.1566908316991,-63.9562846865567,0.));
#63845=CARTESIAN_POINT('Ctrl Pts',(31.1721931134487,-63.9723336316551,0.));
#63846=CARTESIAN_POINT('Ctrl Pts',(31.1877439104716,-63.9884002130211,0.));
#63847=CARTESIAN_POINT('Ctrl Pts',(31.2033431746558,-64.0044842794832,0.));
#63848=CARTESIAN_POINT('Ctrl Pts',(31.2189908580245,-64.02058568063,0.));
#63849=CARTESIAN_POINT('Ctrl Pts',(31.2346869127297,-64.0367042667984,0.));
#63850=CARTESIAN_POINT('Ctrl Pts',(31.2504312910451,-64.0528398890657,0.));
#63851=CARTESIAN_POINT('Ctrl Pts',(31.2662239453728,-64.0689923992461,0.));
#63852=CARTESIAN_POINT('Ctrl Pts',(31.2820648282447,-64.0851616498853,0.));
#63853=CARTESIAN_POINT('Ctrl Pts',(31.2979538923214,-64.1013474942557,0.));
#63854=CARTESIAN_POINT('Ctrl Pts',(31.3138910903858,-64.1175497863491,0.));
#63855=CARTESIAN_POINT('Ctrl Pts',(31.3298763753376,-64.1337683808691,0.));
#63856=CARTESIAN_POINT('Ctrl Pts',(31.3459097002006,-64.1500031332282,0.));
#63857=CARTESIAN_POINT('Ctrl Pts',(31.3619910181228,-64.166253899542,0.));
#63858=CARTESIAN_POINT('Ctrl Pts',(31.3781202823754,-64.1825205366225,0.));
#63859=CARTESIAN_POINT('Ctrl Pts',(31.3942974463445,-64.1988029019707,0.));
#63860=CARTESIAN_POINT('Ctrl Pts',(31.410522463528,-64.2151008537697,0.));
#63861=CARTESIAN_POINT('Ctrl Pts',(31.4267952875423,-64.231414250881,0.));
#63862=CARTESIAN_POINT('Ctrl Pts',(31.4431158721221,-64.2477429528393,0.));
#63863=CARTESIAN_POINT('Ctrl Pts',(31.4594841711194,-64.2640868198473,0.));
#63864=CARTESIAN_POINT('Ctrl Pts',(31.4759001384941,-64.2804457127671,0.));
#63865=CARTESIAN_POINT('Ctrl Pts',(31.4923637283131,-64.2968194931158,0.));
#63866=CARTESIAN_POINT('Ctrl Pts',(31.5088748947582,-64.3132080230637,0.));
#63867=CARTESIAN_POINT('Ctrl Pts',(31.5254335921245,-64.3296111654283,0.));
#63868=CARTESIAN_POINT('Ctrl Pts',(31.5420397748191,-64.3460287836687,0.));
#63869=CARTESIAN_POINT('Ctrl Pts',(31.5586933973515,-64.3624607418769,0.));
#63870=CARTESIAN_POINT('Ctrl Pts',(31.5753944143336,-64.3789069047734,0.));
#63871=CARTESIAN_POINT('Ctrl Pts',(31.5921427804865,-64.3953671377046,0.));
#63872=CARTESIAN_POINT('Ctrl Pts',(31.6089384506395,-64.4118413066378,0.));
#63873=CARTESIAN_POINT('Ctrl Pts',(31.6257813797287,-64.4283292781565,0.));
#63874=CARTESIAN_POINT('Ctrl Pts',(31.6426715227878,-64.4448309194525,0.));
#63875=CARTESIAN_POINT('Ctrl Pts',(31.6596088349481,-64.4613460983214,0.));
#63876=CARTESIAN_POINT('Ctrl Pts',(31.6765932714464,-64.4778746831614,0.));
#63877=CARTESIAN_POINT('Ctrl Pts',(31.6936247876228,-64.4944165429675,0.));
#63878=CARTESIAN_POINT('Ctrl Pts',(31.71070333892,-64.510971547327,0.));
#63879=CARTESIAN_POINT('Ctrl Pts',(31.7278288808731,-64.5275395664124,0.));
#63880=CARTESIAN_POINT('Ctrl Pts',(31.7450013691111,-64.544120470977,0.));
#63881=CARTESIAN_POINT('Ctrl Pts',(31.7622207593634,-64.5607141323521,0.));
#63882=CARTESIAN_POINT('Ctrl Pts',(31.7794870074583,-64.5773204224429,0.));
#63883=CARTESIAN_POINT('Ctrl Pts',(31.7968000693218,-64.5939392137235,0.));
#63884=CARTESIAN_POINT('Ctrl Pts',(31.8141599009684,-64.6105703792312,0.));
#63885=CARTESIAN_POINT('Ctrl Pts',(31.8315664585025,-64.6272137925627,0.));
#63886=CARTESIAN_POINT('Ctrl Pts',(31.8490196981248,-64.6438693278714,0.));
#63887=CARTESIAN_POINT('Ctrl Pts',(31.866519576131,-64.6605368598629,0.));
#63888=CARTESIAN_POINT('Ctrl Pts',(31.8840660489106,-64.6772162637907,0.));
#63889=CARTESIAN_POINT('Ctrl Pts',(31.9016590729373,-64.6939074154498,0.));
#63890=CARTESIAN_POINT('Ctrl Pts',(31.9192986047705,-64.7106101911732,0.));
#63891=CARTESIAN_POINT('Ctrl Pts',(31.9369846010615,-64.7273244678297,0.));
#63892=CARTESIAN_POINT('Ctrl Pts',(31.9547170185533,-64.7440501228203,0.));
#63893=CARTESIAN_POINT('Ctrl Pts',(31.9724958140789,-64.7607870340735,0.));
#63894=CARTESIAN_POINT('Ctrl Pts',(31.9903209445519,-64.7775350800401,0.));
#63895=CARTESIAN_POINT('Ctrl Pts',(32.0081923669676,-64.7942941396881,0.));
#63896=CARTESIAN_POINT('Ctrl Pts',(32.0261100384092,-64.8110640925021,0.));
#63897=CARTESIAN_POINT('Ctrl Pts',(32.0440739160477,-64.8278448184787,0.));
#63898=CARTESIAN_POINT('Ctrl Pts',(32.0620839571408,-64.8446361981234,0.));
#63899=CARTESIAN_POINT('Ctrl Pts',(32.0801401190241,-64.861438112445,0.));
#63900=CARTESIAN_POINT('Ctrl Pts',(32.0982423591108,-64.878250442952,0.));
#63901=CARTESIAN_POINT('Ctrl Pts',(32.1163906348979,-64.8950730716493,0.));
#63902=CARTESIAN_POINT('Ctrl Pts',(32.1345849039671,-64.9119058810362,0.));
#63903=CARTESIAN_POINT('Ctrl Pts',(32.1528251239831,-64.9287487541019,0.));
#63904=CARTESIAN_POINT('Ctrl Pts',(32.1711112526859,-64.9456015743203,0.));
#63905=CARTESIAN_POINT('Ctrl Pts',(32.1894432478888,-64.9624642256478,0.));
#63906=CARTESIAN_POINT('Ctrl Pts',(32.2078210674857,-64.9793365925194,0.));
#63907=CARTESIAN_POINT('Ctrl Pts',(32.2262446694516,-64.996218559847,0.));
#63908=CARTESIAN_POINT('Ctrl Pts',(32.244714011842,-65.0131100130155,0.));
#63909=CARTESIAN_POINT('Ctrl Pts',(32.2632290527854,-65.0300108378786,0.));
#63910=CARTESIAN_POINT('Ctrl Pts',(32.2817897504799,-65.0469209207548,0.));
#63911=CARTESIAN_POINT('Ctrl Pts',(32.3003960632,-65.0638401484245,0.));
#63912=CARTESIAN_POINT('Ctrl Pts',(32.3190479492985,-65.0807684081278,0.));
#63913=CARTESIAN_POINT('Ctrl Pts',(32.3377453672051,-65.097705587561,0.));
#63914=CARTESIAN_POINT('Ctrl Pts',(32.3564882754212,-65.1146515748723,0.));
#63915=CARTESIAN_POINT('Ctrl Pts',(32.3752766325134,-65.1316062586586,0.));
#63916=CARTESIAN_POINT('Ctrl Pts',(32.3941103971218,-65.1485695279628,0.));
#63917=CARTESIAN_POINT('Ctrl Pts',(32.4129895279612,-65.165541272272,0.));
#63918=CARTESIAN_POINT('Ctrl Pts',(32.4319139838212,-65.182521381514,0.));
#63919=CARTESIAN_POINT('Ctrl Pts',(32.4508837235613,-65.1995097460546,0.));
#63920=CARTESIAN_POINT('Ctrl Pts',(32.4698987061036,-65.2165062566936,0.));
#63921=CARTESIAN_POINT('Ctrl Pts',(32.4889588904396,-65.2335108046625,0.));
#63922=CARTESIAN_POINT('Ctrl Pts',(32.508064235633,-65.2505232816215,0.));
#63923=CARTESIAN_POINT('Ctrl Pts',(32.527214700819,-65.2675435796558,0.));
#63924=CARTESIAN_POINT('Ctrl Pts',(32.5464102452013,-65.2845715912717,0.));
#63925=CARTESIAN_POINT('Ctrl Pts',(32.565650828042,-65.3016072093908,0.));
#63926=CARTESIAN_POINT('Ctrl Pts',(32.5849364086678,-65.3186503273498,0.));
#63927=CARTESIAN_POINT('Ctrl Pts',(32.6042669464751,-65.3357008389005,0.));
#63928=CARTESIAN_POINT('Ctrl Pts',(32.6236424009301,-65.3527586382082,0.));
#63929=CARTESIAN_POINT('Ctrl Pts',(32.6430627315672,-65.3698236198512,0.));
#63930=CARTESIAN_POINT('Ctrl Pts',(32.6625278979807,-65.3868956788178,0.));
#63931=CARTESIAN_POINT('Ctrl Pts',(32.6820378598262,-65.4039747105033,0.));
#63932=CARTESIAN_POINT('Ctrl Pts',(32.701592576826,-65.421060610703,0.));
#63933=CARTESIAN_POINT('Ctrl Pts',(32.7211920087681,-65.4381532756063,0.));
#63934=CARTESIAN_POINT('Ctrl Pts',(32.7408361155037,-65.4552526017907,0.));
#63935=CARTESIAN_POINT('Ctrl Pts',(32.7605248569382,-65.4723584862129,0.));
#63936=CARTESIAN_POINT('Ctrl Pts',(32.7802581930293,-65.4894708262071,0.));
#63937=CARTESIAN_POINT('Ctrl Pts',(32.800036083798,-65.5065895194939,0.));
#63938=CARTESIAN_POINT('Ctrl Pts',(32.8198584893318,-65.5237144641864,0.));
#63939=CARTESIAN_POINT('Ctrl Pts',(32.8397253697864,-65.5408455587963,0.));
#63940=CARTESIAN_POINT('Ctrl Pts',(32.8596366853826,-65.5579827022413,0.));
#63941=CARTESIAN_POINT('Ctrl Pts',(32.8795923964021,-65.575125793846,0.));
#63942=CARTESIAN_POINT('Ctrl Pts',(32.899592463189,-65.5922747333182,0.));
#63943=CARTESIAN_POINT('Ctrl Pts',(32.9196368461457,-65.6094294207267,0.));
#63944=CARTESIAN_POINT('Ctrl Pts',(32.9397255057273,-65.6265897564782,0.));
#63945=CARTESIAN_POINT('Ctrl Pts',(32.9598584024317,-65.6437556412956,0.));
#63946=CARTESIAN_POINT('Ctrl Pts',(32.9800354967846,-65.6609269761902,0.));
#63947=CARTESIAN_POINT('Ctrl Pts',(33.000256749358,-65.6781036625041,0.));
#63948=CARTESIAN_POINT('Ctrl Pts',(33.0205221207877,-65.6952856019542,0.));
#63949=CARTESIAN_POINT('Ctrl Pts',(33.0408315717874,-65.7124726966805,0.));
#63950=CARTESIAN_POINT('Ctrl Pts',(33.0611850631579,-65.729664849282,0.));
#63951=CARTESIAN_POINT('Ctrl Pts',(33.0815825557976,-65.7468619628808,0.));
#63952=CARTESIAN_POINT('Ctrl Pts',(33.102024010688,-65.7640639410653,0.));
#63953=CARTESIAN_POINT('Ctrl Pts',(33.1225093888668,-65.7812706877691,0.));
#63954=CARTESIAN_POINT('Ctrl Pts',(33.1430386513975,-65.7984821071622,0.));
#63955=CARTESIAN_POINT('Ctrl Pts',(33.16361175934,-65.8156981035504,0.));
#63956=CARTESIAN_POINT('Ctrl Pts',(33.1842286737053,-65.8329185812379,0.));
#63957=CARTESIAN_POINT('Ctrl Pts',(33.2048893554495,-65.8501434445174,0.));
#63958=CARTESIAN_POINT('Ctrl Pts',(33.2255937655655,-65.8673725979591,0.));
#63959=CARTESIAN_POINT('Ctrl Pts',(33.2463418651497,-65.8846059466382,0.));
#63960=CARTESIAN_POINT('Ctrl Pts',(33.2671336154754,-65.901843396389,0.));
#63961=CARTESIAN_POINT('Ctrl Pts',(33.2879689780566,-65.9190848540422,0.));
#63962=CARTESIAN_POINT('Ctrl Pts',(33.308847914715,-65.9363302276822,0.));
#63963=CARTESIAN_POINT('Ctrl Pts',(33.3297703874249,-65.9535794260802,0.));
#63964=CARTESIAN_POINT('Ctrl Pts',(33.3507363581578,-65.9708323581386,0.));
#63965=CARTESIAN_POINT('Ctrl Pts',(33.3717457887094,-65.9880889322822,0.));
#63966=CARTESIAN_POINT('Ctrl Pts',(33.3927986405612,-66.0053490559826,0.));
#63967=CARTESIAN_POINT('Ctrl Pts',(33.4138948746407,-66.0226126349482,0.));
#63968=CARTESIAN_POINT('Ctrl Pts',(33.4350344515128,-66.0398795737827,0.));
#63969=CARTESIAN_POINT('Ctrl Pts',(33.4562173318052,-66.0571497774484,0.));
#63970=CARTESIAN_POINT('Ctrl Pts',(33.4774434765761,-66.0744231525445,0.));
#63971=CARTESIAN_POINT('Ctrl Pts',(33.4987128476617,-66.0916996085237,0.));
#63972=CARTESIAN_POINT('Ctrl Pts',(33.5200254081212,-66.1089790592673,0.));
#63973=CARTESIAN_POINT('Ctrl Pts',(33.5413811223397,-66.1262614234579,0.));
#63974=CARTESIAN_POINT('Ctrl Pts',(33.5597240685728,-66.1410781873124,0.));
#63975=CARTESIAN_POINT('Ctrl Pts',(33.5738105077705,-66.1524393973985,0.));
#63976=CARTESIAN_POINT('Ctrl Pts',(33.5836213513971,-66.1603438177304,0.));
#63977=CARTESIAN_POINT('Ctrl Pts',(33.5891439876225,-66.1647906582406,0.));
#63978=CARTESIAN_POINT('Ctrl Pts',(33.5903722664954,-66.1657795405667,0.));
#63979=CARTESIAN_POINT('',(30.354906545781,-63.0759831361898,12.));
#63980=CARTESIAN_POINT('',(30.354906545781,-63.0759831361898,0.));
#63981=CARTESIAN_POINT('Ctrl Pts',(33.5903722664955,-66.1657795405668,12.));
#63982=CARTESIAN_POINT('Ctrl Pts',(33.5891439876225,-66.1647906582407,12.));
#63983=CARTESIAN_POINT('Ctrl Pts',(33.5836213513971,-66.1603438177305,12.));
#63984=CARTESIAN_POINT('Ctrl Pts',(33.5738105077705,-66.1524393973985,12.));
#63985=CARTESIAN_POINT('Ctrl Pts',(33.5597240685728,-66.1410781873124,12.));
#63986=CARTESIAN_POINT('Ctrl Pts',(33.5413811223397,-66.1262614234579,12.));
#63987=CARTESIAN_POINT('Ctrl Pts',(33.5200254081212,-66.1089790592673,12.));
#63988=CARTESIAN_POINT('Ctrl Pts',(33.4987128476617,-66.0916996085237,12.));
#63989=CARTESIAN_POINT('Ctrl Pts',(33.4774434765761,-66.0744231525445,12.));
#63990=CARTESIAN_POINT('Ctrl Pts',(33.4562173318052,-66.0571497774484,12.));
#63991=CARTESIAN_POINT('Ctrl Pts',(33.4350344515128,-66.0398795737827,12.));
#63992=CARTESIAN_POINT('Ctrl Pts',(33.4138948746407,-66.0226126349482,12.));
#63993=CARTESIAN_POINT('Ctrl Pts',(33.3927986405612,-66.0053490559826,12.));
#63994=CARTESIAN_POINT('Ctrl Pts',(33.3717457887094,-65.9880889322822,12.));
#63995=CARTESIAN_POINT('Ctrl Pts',(33.3507363581578,-65.9708323581386,12.));
#63996=CARTESIAN_POINT('Ctrl Pts',(33.3297703874249,-65.9535794260802,12.));
#63997=CARTESIAN_POINT('Ctrl Pts',(33.308847914715,-65.9363302276822,12.));
#63998=CARTESIAN_POINT('Ctrl Pts',(33.2879689780566,-65.9190848540422,12.));
#63999=CARTESIAN_POINT('Ctrl Pts',(33.2671336154754,-65.901843396389,12.));
#64000=CARTESIAN_POINT('Ctrl Pts',(33.2463418651497,-65.8846059466382,12.));
#64001=CARTESIAN_POINT('Ctrl Pts',(33.2255937655655,-65.8673725979591,12.));
#64002=CARTESIAN_POINT('Ctrl Pts',(33.2048893554495,-65.8501434445174,12.));
#64003=CARTESIAN_POINT('Ctrl Pts',(33.1842286737053,-65.8329185812379,12.));
#64004=CARTESIAN_POINT('Ctrl Pts',(33.16361175934,-65.8156981035504,12.));
#64005=CARTESIAN_POINT('Ctrl Pts',(33.1430386513975,-65.7984821071622,12.));
#64006=CARTESIAN_POINT('Ctrl Pts',(33.1225093888668,-65.7812706877691,12.));
#64007=CARTESIAN_POINT('Ctrl Pts',(33.102024010688,-65.7640639410653,12.));
#64008=CARTESIAN_POINT('Ctrl Pts',(33.0815825557976,-65.7468619628808,12.));
#64009=CARTESIAN_POINT('Ctrl Pts',(33.0611850631579,-65.729664849282,12.));
#64010=CARTESIAN_POINT('Ctrl Pts',(33.0408315717874,-65.7124726966805,12.));
#64011=CARTESIAN_POINT('Ctrl Pts',(33.0205221207877,-65.6952856019542,12.));
#64012=CARTESIAN_POINT('Ctrl Pts',(33.000256749358,-65.6781036625041,12.));
#64013=CARTESIAN_POINT('Ctrl Pts',(32.9800354967846,-65.6609269761902,12.));
#64014=CARTESIAN_POINT('Ctrl Pts',(32.9598584024317,-65.6437556412956,12.));
#64015=CARTESIAN_POINT('Ctrl Pts',(32.9397255057273,-65.6265897564782,12.));
#64016=CARTESIAN_POINT('Ctrl Pts',(32.9196368461457,-65.6094294207267,12.));
#64017=CARTESIAN_POINT('Ctrl Pts',(32.899592463189,-65.5922747333182,12.));
#64018=CARTESIAN_POINT('Ctrl Pts',(32.8795923964021,-65.575125793846,12.));
#64019=CARTESIAN_POINT('Ctrl Pts',(32.8596366853826,-65.5579827022413,12.));
#64020=CARTESIAN_POINT('Ctrl Pts',(32.8397253697864,-65.5408455587963,12.));
#64021=CARTESIAN_POINT('Ctrl Pts',(32.8198584893318,-65.5237144641864,12.));
#64022=CARTESIAN_POINT('Ctrl Pts',(32.800036083798,-65.5065895194939,12.));
#64023=CARTESIAN_POINT('Ctrl Pts',(32.7802581930293,-65.4894708262071,12.));
#64024=CARTESIAN_POINT('Ctrl Pts',(32.7605248569382,-65.4723584862129,12.));
#64025=CARTESIAN_POINT('Ctrl Pts',(32.7408361155037,-65.4552526017907,12.));
#64026=CARTESIAN_POINT('Ctrl Pts',(32.7211920087681,-65.4381532756063,12.));
#64027=CARTESIAN_POINT('Ctrl Pts',(32.701592576826,-65.421060610703,12.));
#64028=CARTESIAN_POINT('Ctrl Pts',(32.6820378598262,-65.4039747105033,12.));
#64029=CARTESIAN_POINT('Ctrl Pts',(32.6625278979807,-65.3868956788178,12.));
#64030=CARTESIAN_POINT('Ctrl Pts',(32.6430627315672,-65.3698236198512,12.));
#64031=CARTESIAN_POINT('Ctrl Pts',(32.6236424009301,-65.3527586382082,12.));
#64032=CARTESIAN_POINT('Ctrl Pts',(32.6042669464751,-65.3357008389005,12.));
#64033=CARTESIAN_POINT('Ctrl Pts',(32.5849364086678,-65.3186503273498,12.));
#64034=CARTESIAN_POINT('Ctrl Pts',(32.565650828042,-65.3016072093908,12.));
#64035=CARTESIAN_POINT('Ctrl Pts',(32.5464102452013,-65.2845715912717,12.));
#64036=CARTESIAN_POINT('Ctrl Pts',(32.527214700819,-65.2675435796558,12.));
#64037=CARTESIAN_POINT('Ctrl Pts',(32.508064235633,-65.2505232816215,12.));
#64038=CARTESIAN_POINT('Ctrl Pts',(32.4889588904396,-65.2335108046625,12.));
#64039=CARTESIAN_POINT('Ctrl Pts',(32.4698987061036,-65.2165062566936,12.));
#64040=CARTESIAN_POINT('Ctrl Pts',(32.4508837235613,-65.1995097460546,12.));
#64041=CARTESIAN_POINT('Ctrl Pts',(32.4319139838212,-65.182521381514,12.));
#64042=CARTESIAN_POINT('Ctrl Pts',(32.4129895279612,-65.165541272272,12.));
#64043=CARTESIAN_POINT('Ctrl Pts',(32.3941103971218,-65.1485695279628,12.));
#64044=CARTESIAN_POINT('Ctrl Pts',(32.3752766325134,-65.1316062586586,12.));
#64045=CARTESIAN_POINT('Ctrl Pts',(32.3564882754212,-65.1146515748723,12.));
#64046=CARTESIAN_POINT('Ctrl Pts',(32.3377453672051,-65.097705587561,12.));
#64047=CARTESIAN_POINT('Ctrl Pts',(32.3190479492985,-65.0807684081278,12.));
#64048=CARTESIAN_POINT('Ctrl Pts',(32.3003960632,-65.0638401484245,12.));
#64049=CARTESIAN_POINT('Ctrl Pts',(32.2817897504799,-65.0469209207548,12.));
#64050=CARTESIAN_POINT('Ctrl Pts',(32.2632290527854,-65.0300108378786,12.));
#64051=CARTESIAN_POINT('Ctrl Pts',(32.244714011842,-65.0131100130155,12.));
#64052=CARTESIAN_POINT('Ctrl Pts',(32.2262446694516,-64.996218559847,12.));
#64053=CARTESIAN_POINT('Ctrl Pts',(32.2078210674857,-64.9793365925194,12.));
#64054=CARTESIAN_POINT('Ctrl Pts',(32.1894432478888,-64.9624642256478,12.));
#64055=CARTESIAN_POINT('Ctrl Pts',(32.1711112526859,-64.9456015743203,12.));
#64056=CARTESIAN_POINT('Ctrl Pts',(32.1528251239831,-64.9287487541019,12.));
#64057=CARTESIAN_POINT('Ctrl Pts',(32.1345849039671,-64.9119058810362,12.));
#64058=CARTESIAN_POINT('Ctrl Pts',(32.1163906348979,-64.8950730716493,12.));
#64059=CARTESIAN_POINT('Ctrl Pts',(32.0982423591108,-64.878250442952,12.));
#64060=CARTESIAN_POINT('Ctrl Pts',(32.0801401190241,-64.861438112445,12.));
#64061=CARTESIAN_POINT('Ctrl Pts',(32.0620839571408,-64.8446361981234,12.));
#64062=CARTESIAN_POINT('Ctrl Pts',(32.0440739160477,-64.8278448184787,12.));
#64063=CARTESIAN_POINT('Ctrl Pts',(32.0261100384092,-64.8110640925021,12.));
#64064=CARTESIAN_POINT('Ctrl Pts',(32.0081923669676,-64.7942941396881,12.));
#64065=CARTESIAN_POINT('Ctrl Pts',(31.9903209445519,-64.7775350800401,12.));
#64066=CARTESIAN_POINT('Ctrl Pts',(31.9724958140789,-64.7607870340735,12.));
#64067=CARTESIAN_POINT('Ctrl Pts',(31.9547170185533,-64.7440501228203,12.));
#64068=CARTESIAN_POINT('Ctrl Pts',(31.9369846010615,-64.7273244678297,12.));
#64069=CARTESIAN_POINT('Ctrl Pts',(31.9192986047705,-64.7106101911732,12.));
#64070=CARTESIAN_POINT('Ctrl Pts',(31.9016590729373,-64.6939074154498,12.));
#64071=CARTESIAN_POINT('Ctrl Pts',(31.8840660489106,-64.6772162637907,12.));
#64072=CARTESIAN_POINT('Ctrl Pts',(31.866519576131,-64.6605368598629,12.));
#64073=CARTESIAN_POINT('Ctrl Pts',(31.8490196981248,-64.6438693278714,12.));
#64074=CARTESIAN_POINT('Ctrl Pts',(31.8315664585025,-64.6272137925627,12.));
#64075=CARTESIAN_POINT('Ctrl Pts',(31.8141599009684,-64.6105703792312,12.));
#64076=CARTESIAN_POINT('Ctrl Pts',(31.7968000693218,-64.5939392137235,12.));
#64077=CARTESIAN_POINT('Ctrl Pts',(31.7794870074583,-64.5773204224429,12.));
#64078=CARTESIAN_POINT('Ctrl Pts',(31.7622207593634,-64.5607141323521,12.));
#64079=CARTESIAN_POINT('Ctrl Pts',(31.7450013691111,-64.544120470977,12.));
#64080=CARTESIAN_POINT('Ctrl Pts',(31.7278288808731,-64.5275395664124,12.));
#64081=CARTESIAN_POINT('Ctrl Pts',(31.71070333892,-64.510971547327,12.));
#64082=CARTESIAN_POINT('Ctrl Pts',(31.6936247876228,-64.4944165429675,12.));
#64083=CARTESIAN_POINT('Ctrl Pts',(31.6765932714464,-64.4778746831614,12.));
#64084=CARTESIAN_POINT('Ctrl Pts',(31.6596088349481,-64.4613460983214,12.));
#64085=CARTESIAN_POINT('Ctrl Pts',(31.6426715227878,-64.4448309194525,12.));
#64086=CARTESIAN_POINT('Ctrl Pts',(31.6257813797287,-64.4283292781565,12.));
#64087=CARTESIAN_POINT('Ctrl Pts',(31.6089384506395,-64.4118413066378,12.));
#64088=CARTESIAN_POINT('Ctrl Pts',(31.5921427804865,-64.3953671377046,12.));
#64089=CARTESIAN_POINT('Ctrl Pts',(31.5753944143336,-64.3789069047734,12.));
#64090=CARTESIAN_POINT('Ctrl Pts',(31.5586933973515,-64.3624607418769,12.));
#64091=CARTESIAN_POINT('Ctrl Pts',(31.5420397748191,-64.3460287836687,12.));
#64092=CARTESIAN_POINT('Ctrl Pts',(31.5254335921245,-64.3296111654283,12.));
#64093=CARTESIAN_POINT('Ctrl Pts',(31.5088748947582,-64.3132080230637,12.));
#64094=CARTESIAN_POINT('Ctrl Pts',(31.4923637283131,-64.2968194931158,12.));
#64095=CARTESIAN_POINT('Ctrl Pts',(31.4759001384941,-64.2804457127671,12.));
#64096=CARTESIAN_POINT('Ctrl Pts',(31.4594841711194,-64.2640868198473,12.));
#64097=CARTESIAN_POINT('Ctrl Pts',(31.4431158721221,-64.2477429528393,12.));
#64098=CARTESIAN_POINT('Ctrl Pts',(31.4267952875423,-64.231414250881,12.));
#64099=CARTESIAN_POINT('Ctrl Pts',(31.410522463528,-64.2151008537697,12.));
#64100=CARTESIAN_POINT('Ctrl Pts',(31.3942974463445,-64.1988029019707,12.));
#64101=CARTESIAN_POINT('Ctrl Pts',(31.3781202823754,-64.1825205366225,12.));
#64102=CARTESIAN_POINT('Ctrl Pts',(31.3619910181228,-64.166253899542,12.));
#64103=CARTESIAN_POINT('Ctrl Pts',(31.3459097002006,-64.1500031332282,12.));
#64104=CARTESIAN_POINT('Ctrl Pts',(31.3298763753376,-64.1337683808691,12.));
#64105=CARTESIAN_POINT('Ctrl Pts',(31.3138910903858,-64.1175497863491,12.));
#64106=CARTESIAN_POINT('Ctrl Pts',(31.2979538923214,-64.1013474942557,12.));
#64107=CARTESIAN_POINT('Ctrl Pts',(31.2820648282447,-64.0851616498853,12.));
#64108=CARTESIAN_POINT('Ctrl Pts',(31.2662239453728,-64.0689923992461,12.));
#64109=CARTESIAN_POINT('Ctrl Pts',(31.2504312910451,-64.0528398890657,12.));
#64110=CARTESIAN_POINT('Ctrl Pts',(31.2346869127297,-64.0367042667984,12.));
#64111=CARTESIAN_POINT('Ctrl Pts',(31.2189908580245,-64.02058568063,12.));
#64112=CARTESIAN_POINT('Ctrl Pts',(31.2033431746558,-64.0044842794832,12.));
#64113=CARTESIAN_POINT('Ctrl Pts',(31.1877439104716,-63.9884002130211,12.));
#64114=CARTESIAN_POINT('Ctrl Pts',(31.1721931134487,-63.9723336316551,12.));
#64115=CARTESIAN_POINT('Ctrl Pts',(31.1566908316991,-63.9562846865567,12.));
#64116=CARTESIAN_POINT('Ctrl Pts',(31.1412371134727,-63.9402535296651,12.));
#64117=CARTESIAN_POINT('Ctrl Pts',(31.1258320071545,-63.9242403136955,12.));
#64118=CARTESIAN_POINT('Ctrl Pts',(31.1104755612607,-63.9082451921448,12.));
#64119=CARTESIAN_POINT('Ctrl Pts',(31.0951678244455,-63.8922683192965,12.));
#64120=CARTESIAN_POINT('Ctrl Pts',(31.0799088455041,-63.8763098502237,12.));
#64121=CARTESIAN_POINT('Ctrl Pts',(31.0646986733723,-63.8603699407922,12.));
#64122=CARTESIAN_POINT('Ctrl Pts',(31.0495373571214,-63.8444487476611,12.));
#64123=CARTESIAN_POINT('Ctrl Pts',(31.0344249459538,-63.8285464282846,12.));
#64124=CARTESIAN_POINT('Ctrl Pts',(31.019361489217,-63.8126631409364,12.));
#64125=CARTESIAN_POINT('Ctrl Pts',(31.0043470364108,-63.796799044728,12.));
#64126=CARTESIAN_POINT('Ctrl Pts',(30.9893816371909,-63.7809542996264,12.));
#64127=CARTESIAN_POINT('Ctrl Pts',(30.9744653413688,-63.7651290664733,12.));
#64128=CARTESIAN_POINT('Ctrl Pts',(30.9595981989103,-63.7493235069871,12.));
#64129=CARTESIAN_POINT('Ctrl Pts',(30.9447802599354,-63.7335377837441,12.));
#64130=CARTESIAN_POINT('Ctrl Pts',(30.9300115747115,-63.717772060161,12.));
#64131=CARTESIAN_POINT('Ctrl Pts',(30.9152921936464,-63.7020265004792,12.));
#64132=CARTESIAN_POINT('Ctrl Pts',(30.900622167269,-63.6863012697328,12.));
#64133=CARTESIAN_POINT('Ctrl Pts',(30.8860015462475,-63.6705965337971,12.));
#64134=CARTESIAN_POINT('Ctrl Pts',(30.8714303814194,-63.6549124594666,12.));
#64135=CARTESIAN_POINT('Ctrl Pts',(30.8569087238131,-63.6392492145233,12.));
#64136=CARTESIAN_POINT('Ctrl Pts',(30.8424366246671,-63.6236069678055,12.));
#64137=CARTESIAN_POINT('Ctrl Pts',(30.8280141354458,-63.6079858892771,12.));
#64138=CARTESIAN_POINT('Ctrl Pts',(30.813641307801,-63.5923861498988,12.));
#64139=CARTESIAN_POINT('Ctrl Pts',(30.7993181935271,-63.5768079214882,12.));
#64140=CARTESIAN_POINT('Ctrl Pts',(30.7850448445204,-63.5612513766,12.));
#64141=CARTESIAN_POINT('Ctrl Pts',(30.7708213127158,-63.5457166883537,12.));
#64142=CARTESIAN_POINT('Ctrl Pts',(30.7566476500757,-63.5302040304142,12.));
#64143=CARTESIAN_POINT('Ctrl Pts',(30.7425239087281,-63.5147135773894,12.));
#64144=CARTESIAN_POINT('Ctrl Pts',(30.7284501410822,-63.4992455051795,12.));
#64145=CARTESIAN_POINT('Ctrl Pts',(30.7144263999265,-63.4837999912772,12.));
#64146=CARTESIAN_POINT('Ctrl Pts',(30.7004527385821,-63.468377215253,12.));
#64147=CARTESIAN_POINT('Ctrl Pts',(30.6865292107929,-63.4529773584249,12.));
#64148=CARTESIAN_POINT('Ctrl Pts',(30.6726558704315,-63.4376006029604,12.));
#64149=CARTESIAN_POINT('Ctrl Pts',(30.6588327712483,-63.422247131124,12.));
#64150=CARTESIAN_POINT('Ctrl Pts',(30.645059966612,-63.4069171245067,12.));
#64151=CARTESIAN_POINT('Ctrl Pts',(30.6313375092062,-63.3916107631376,12.));
#64152=CARTESIAN_POINT('Ctrl Pts',(30.6176654515967,-63.3763282271796,12.));
#64153=CARTESIAN_POINT('Ctrl Pts',(30.6040438469078,-63.3610696989577,12.));
#64154=CARTESIAN_POINT('Ctrl Pts',(30.5904727493711,-63.3458353646154,12.));
#64155=CARTESIAN_POINT('Ctrl Pts',(30.5769522151163,-63.3306254165126,12.));
#64156=CARTESIAN_POINT('Ctrl Pts',(30.5634823022379,-63.3154400534397,12.));
#64157=CARTESIAN_POINT('Ctrl Pts',(30.5500630691359,-63.3002794756086,12.));
#64158=CARTESIAN_POINT('Ctrl Pts',(30.5366945730508,-63.2851438802474,12.));
#64159=CARTESIAN_POINT('Ctrl Pts',(30.5233768687864,-63.2700334577639,12.));
#64160=CARTESIAN_POINT('Ctrl Pts',(30.5101100066659,-63.2549483856215,12.));
#64161=CARTESIAN_POINT('Ctrl Pts',(30.4968940344997,-63.2398888342546,12.));
#64162=CARTESIAN_POINT('Ctrl Pts',(30.4837290014989,-63.2248549788222,12.));
#64163=CARTESIAN_POINT('Ctrl Pts',(30.4706149614159,-63.2098470086636,12.));
#64164=CARTESIAN_POINT('Ctrl Pts',(30.4575519763336,-63.1948651386942,12.));
#64165=CARTESIAN_POINT('Ctrl Pts',(30.444540119238,-63.179909617189,12.));
#64166=CARTESIAN_POINT('Ctrl Pts',(30.431579465973,-63.164980701691,12.));
#64167=CARTESIAN_POINT('Ctrl Pts',(30.418670087563,-63.1500786361459,12.));
#64168=CARTESIAN_POINT('Ctrl Pts',(30.4058120432228,-63.1352036298441,12.));
#64169=CARTESIAN_POINT('Ctrl Pts',(30.3930053710484,-63.1203558300657,12.));
#64170=CARTESIAN_POINT('Ctrl Pts',(30.3802500880402,-63.105535320226,12.));
#64171=CARTESIAN_POINT('Ctrl Pts',(30.3700869762507,-63.0937007763471,12.));
#64172=CARTESIAN_POINT('Ctrl Pts',(30.362487768065,-63.0848371718048,12.));
#64173=CARTESIAN_POINT('Ctrl Pts',(30.3574319069329,-63.078933570069,12.));
#64174=CARTESIAN_POINT('Ctrl Pts',(30.354906545781,-63.0759831361898,12.));
#64175=CARTESIAN_POINT('Ctrl Pts',(34.933187552314,-65.4667541478395,-5.55111512312578E-16));
#64176=CARTESIAN_POINT('Ctrl Pts',(34.933187552314,-65.4667541478395,4.));
#64177=CARTESIAN_POINT('Ctrl Pts',(34.933187552314,-65.4667541478394,8.));
#64178=CARTESIAN_POINT('Ctrl Pts',(34.933187552314,-65.4667541478394,12.));
#64179=CARTESIAN_POINT('Ctrl Pts',(34.940541458921,-65.5763902570758,-5.55111512312578E-16));
#64180=CARTESIAN_POINT('Ctrl Pts',(34.940541458921,-65.5763902570758,4.));
#64181=CARTESIAN_POINT('Ctrl Pts',(34.940541458921,-65.5763902570757,8.00000000000001));
#64182=CARTESIAN_POINT('Ctrl Pts',(34.940541458921,-65.5763902570757,12.));
#64183=CARTESIAN_POINT('Ctrl Pts',(34.8876896346298,-65.7720412680595,-5.55111512312578E-16));
#64184=CARTESIAN_POINT('Ctrl Pts',(34.8876896346298,-65.7720412680595,4.));
#64185=CARTESIAN_POINT('Ctrl Pts',(34.8876896346298,-65.7720412680595,7.99999999999999));
#64186=CARTESIAN_POINT('Ctrl Pts',(34.8876896346298,-65.7720412680595,12.));
#64187=CARTESIAN_POINT('Ctrl Pts',(34.7399186668304,-65.9044372006549,-5.55111512312578E-16));
#64188=CARTESIAN_POINT('Ctrl Pts',(34.7399186668304,-65.9044372006549,4.));
#64189=CARTESIAN_POINT('Ctrl Pts',(34.7399186668304,-65.9044372006548,8.00000000000001));
#64190=CARTESIAN_POINT('Ctrl Pts',(34.7399186668304,-65.9044372006548,12.));
#64191=CARTESIAN_POINT('Ctrl Pts',(34.6669728017261,-65.9427857825589,-5.55111512312578E-16));
#64192=CARTESIAN_POINT('Ctrl Pts',(34.6669728017261,-65.9427857825589,4.));
#64193=CARTESIAN_POINT('Ctrl Pts',(34.6669728017261,-65.9427857825589,8.));
#64194=CARTESIAN_POINT('Ctrl Pts',(34.6669728017261,-65.9427857825589,12.));
#64195=CARTESIAN_POINT('',(34.933187552314,-65.4667541478395,2.77555756156289E-16));
#64196=CARTESIAN_POINT('',(34.6669728017259,-65.9427857825585,0.));
#64197=CARTESIAN_POINT('Ctrl Pts',(34.933187552314,-65.4667541478395,-1.38777878078145E-16));
#64198=CARTESIAN_POINT('Ctrl Pts',(34.940541458921,-65.5763902570758,-1.38777878078145E-16));
#64199=CARTESIAN_POINT('Ctrl Pts',(34.9103404164689,-65.6881908347808,-1.38777878078144E-16));
#64200=CARTESIAN_POINT('Ctrl Pts',(34.8491453679733,-65.779336693012,-1.38777878078145E-16));
#64201=CARTESIAN_POINT('Ctrl Pts',(34.8032490816015,-65.8476960866854,-1.38777878078145E-16));
#64202=CARTESIAN_POINT('Ctrl Pts',(34.7399186668304,-65.9044372006549,-1.38777878078145E-16));
#64203=CARTESIAN_POINT('Ctrl Pts',(34.6669728017261,-65.9427857825589,-1.38777878078145E-16));
#64204=CARTESIAN_POINT('',(34.6669728017259,-65.9427857825585,12.));
#64205=CARTESIAN_POINT('Ctrl Pts',(34.6669728017261,-65.9427857825589,-5.55111512312578E-16));
#64206=CARTESIAN_POINT('Ctrl Pts',(34.6669728017261,-65.9427857825589,4.));
#64207=CARTESIAN_POINT('Ctrl Pts',(34.6669728017261,-65.9427857825589,8.));
#64208=CARTESIAN_POINT('Ctrl Pts',(34.6669728017261,-65.9427857825589,12.));
#64209=CARTESIAN_POINT('',(34.933187552314,-65.4667541478394,12.));
#64210=CARTESIAN_POINT('Ctrl Pts',(34.6669728017261,-65.9427857825589,12.));
#64211=CARTESIAN_POINT('Ctrl Pts',(34.7399186668304,-65.9044372006548,12.));
#64212=CARTESIAN_POINT('Ctrl Pts',(34.8032490816015,-65.8476960866854,12.));
#64213=CARTESIAN_POINT('Ctrl Pts',(34.8491453679733,-65.779336693012,12.));
#64214=CARTESIAN_POINT('Ctrl Pts',(34.9103404164689,-65.6881908347807,12.));
#64215=CARTESIAN_POINT('Ctrl Pts',(34.940541458921,-65.5763902570757,12.));
#64216=CARTESIAN_POINT('Ctrl Pts',(34.933187552314,-65.4667541478394,12.));
#64217=CARTESIAN_POINT('Ctrl Pts',(34.933187552314,-65.4667541478394,12.));
#64218=CARTESIAN_POINT('Ctrl Pts',(34.933187552314,-65.4667541478394,8.));
#64219=CARTESIAN_POINT('Ctrl Pts',(34.933187552314,-65.4667541478395,4.));
#64220=CARTESIAN_POINT('Ctrl Pts',(34.933187552314,-65.4667541478395,-5.55111512312578E-16));
#64221=CARTESIAN_POINT('Origin',(1.73171632017258E-10,-3.32444647725449E-10,
0.));
#64222=CARTESIAN_POINT('Origin',(1.73171632017258E-10,-3.32444647725449E-10,
12.));
#64223=CARTESIAN_POINT('Origin',(1.73171632017258E-10,-3.32444647725449E-10,
0.));
#64224=CARTESIAN_POINT('Ctrl Pts',(28.2316040302268,-68.9436475237602,0.));
#64225=CARTESIAN_POINT('Ctrl Pts',(28.2316040302268,-68.9436475237602,4.));
#64226=CARTESIAN_POINT('Ctrl Pts',(28.2316040302268,-68.9436475237602,8.));
#64227=CARTESIAN_POINT('Ctrl Pts',(28.2316040302268,-68.9436475237602,12.));
#64228=CARTESIAN_POINT('Ctrl Pts',(28.1299168084376,-68.9852872321829,0.));
#64229=CARTESIAN_POINT('Ctrl Pts',(28.1299168084376,-68.9852872321829,4.));
#64230=CARTESIAN_POINT('Ctrl Pts',(28.1299168084376,-68.9852872321829,8.));
#64231=CARTESIAN_POINT('Ctrl Pts',(28.1299168084376,-68.9852872321829,12.));
#64232=CARTESIAN_POINT('Ctrl Pts',(27.9275918177428,-68.9970049015576,0.));
#64233=CARTESIAN_POINT('Ctrl Pts',(27.9275918177428,-68.9970049015576,4.));
#64234=CARTESIAN_POINT('Ctrl Pts',(27.9275918177428,-68.9970049015576,7.99999999999999));
#64235=CARTESIAN_POINT('Ctrl Pts',(27.9275918177428,-68.9970049015576,12.));
#64236=CARTESIAN_POINT('Ctrl Pts',(27.7552674476217,-68.8986722313987,0.));
#64237=CARTESIAN_POINT('Ctrl Pts',(27.7552674476217,-68.8986722313987,4.));
#64238=CARTESIAN_POINT('Ctrl Pts',(27.7552674476217,-68.8986722313987,8.00000000000001));
#64239=CARTESIAN_POINT('Ctrl Pts',(27.7552674476217,-68.8986722313987,12.));
#64240=CARTESIAN_POINT('Ctrl Pts',(27.6958230984752,-68.8415926174768,0.));
#64241=CARTESIAN_POINT('Ctrl Pts',(27.6958230984752,-68.8415926174768,4.));
#64242=CARTESIAN_POINT('Ctrl Pts',(27.6958230984752,-68.8415926174768,8.));
#64243=CARTESIAN_POINT('Ctrl Pts',(27.6958230984752,-68.8415926174768,12.));
#64244=CARTESIAN_POINT('',(28.2316040302268,-68.9436475237602,0.));
#64245=CARTESIAN_POINT('',(27.6958230984751,-68.8415926174769,0.));
#64246=CARTESIAN_POINT('Ctrl Pts',(28.2316040302268,-68.9436475237602,0.));
#64247=CARTESIAN_POINT('Ctrl Pts',(28.1299168084376,-68.9852872321829,0.));
#64248=CARTESIAN_POINT('Ctrl Pts',(28.0143025280406,-68.9919830432541,0.));
#64249=CARTESIAN_POINT('Ctrl Pts',(27.9084843686472,-68.9627440495797,0.));
#64250=CARTESIAN_POINT('Ctrl Pts',(27.8291207491021,-68.9408148043239,0.));
#64251=CARTESIAN_POINT('Ctrl Pts',(27.7552674476217,-68.8986722313987,0.));
#64252=CARTESIAN_POINT('Ctrl Pts',(27.6958230984752,-68.8415926174768,0.));
#64253=CARTESIAN_POINT('',(27.6958230984751,-68.8415926174769,12.));
#64254=CARTESIAN_POINT('Ctrl Pts',(27.6958230984752,-68.8415926174768,0.));
#64255=CARTESIAN_POINT('Ctrl Pts',(27.6958230984752,-68.8415926174768,4.));
#64256=CARTESIAN_POINT('Ctrl Pts',(27.6958230984752,-68.8415926174768,8.));
#64257=CARTESIAN_POINT('Ctrl Pts',(27.6958230984752,-68.8415926174768,12.));
#64258=CARTESIAN_POINT('',(28.2316040302268,-68.9436475237602,12.));
#64259=CARTESIAN_POINT('Ctrl Pts',(27.6958230984752,-68.8415926174768,12.));
#64260=CARTESIAN_POINT('Ctrl Pts',(27.7552674476217,-68.8986722313987,12.));
#64261=CARTESIAN_POINT('Ctrl Pts',(27.8291207491021,-68.9408148043239,12.));
#64262=CARTESIAN_POINT('Ctrl Pts',(27.9084843686472,-68.9627440495797,12.));
#64263=CARTESIAN_POINT('Ctrl Pts',(28.0143025280406,-68.9919830432541,12.));
#64264=CARTESIAN_POINT('Ctrl Pts',(28.1299168084376,-68.9852872321829,12.));
#64265=CARTESIAN_POINT('Ctrl Pts',(28.2316040302268,-68.9436475237602,12.));
#64266=CARTESIAN_POINT('Ctrl Pts',(28.2316040302268,-68.9436475237602,12.));
#64267=CARTESIAN_POINT('Ctrl Pts',(28.2316040302268,-68.9436475237602,8.));
#64268=CARTESIAN_POINT('Ctrl Pts',(28.2316040302268,-68.9436475237602,4.));
#64269=CARTESIAN_POINT('Ctrl Pts',(28.2316040302268,-68.9436475237602,0.));
#64270=CARTESIAN_POINT('Ctrl Pts',(24.7419628022041,-65.4815644032299,0.));
#64271=CARTESIAN_POINT('Ctrl Pts',(24.7419628022041,-65.4815644032299,12.));
#64272=CARTESIAN_POINT('Ctrl Pts',(24.7442214063382,-65.4847237095443,0.));
#64273=CARTESIAN_POINT('Ctrl Pts',(24.7442214063382,-65.4847237095443,12.));
#64274=CARTESIAN_POINT('Ctrl Pts',(24.7487434955981,-65.4910454936254,0.));
#64275=CARTESIAN_POINT('Ctrl Pts',(24.7487434955981,-65.4910454936254,12.));
#64276=CARTESIAN_POINT('Ctrl Pts',(24.7555412724651,-65.5005376841101,0.));
#64277=CARTESIAN_POINT('Ctrl Pts',(24.7555412724651,-65.5005376841101,12.));
#64278=CARTESIAN_POINT('Ctrl Pts',(24.7646342620841,-65.5132129675333,0.));
#64279=CARTESIAN_POINT('Ctrl Pts',(24.7646342620841,-65.5132129675333,12.));
#64280=CARTESIAN_POINT('Ctrl Pts',(24.7760493148465,-65.5290887770232,0.));
#64281=CARTESIAN_POINT('Ctrl Pts',(24.7760493148465,-65.5290887770232,12.));
#64282=CARTESIAN_POINT('Ctrl Pts',(24.787513182749,-65.5449962514662,0.));
#64283=CARTESIAN_POINT('Ctrl Pts',(24.787513182749,-65.5449962514662,12.));
#64284=CARTESIAN_POINT('Ctrl Pts',(24.7990258561259,-65.5609353062829,0.));
#64285=CARTESIAN_POINT('Ctrl Pts',(24.7990258561259,-65.5609353062829,12.));
#64286=CARTESIAN_POINT('Ctrl Pts',(24.8105873098626,-65.5769057914333,0.));
#64287=CARTESIAN_POINT('Ctrl Pts',(24.8105873098626,-65.5769057914333,12.));
#64288=CARTESIAN_POINT('Ctrl Pts',(24.8221975032103,-65.5929074932624,0.));
#64289=CARTESIAN_POINT('Ctrl Pts',(24.8221975032103,-65.5929074932624,12.));
#64290=CARTESIAN_POINT('Ctrl Pts',(24.8338563866763,-65.6089401625628,0.));
#64291=CARTESIAN_POINT('Ctrl Pts',(24.8338563866763,-65.6089401625628,12.));
#64292=CARTESIAN_POINT('Ctrl Pts',(24.8455639071516,-65.6250035361612,0.));
#64293=CARTESIAN_POINT('Ctrl Pts',(24.8455639071516,-65.6250035361612,12.));
#64294=CARTESIAN_POINT('Ctrl Pts',(24.8573200135665,-65.6410973603661,0.));
#64295=CARTESIAN_POINT('Ctrl Pts',(24.8573200135665,-65.6410973603661,12.));
#64296=CARTESIAN_POINT('Ctrl Pts',(24.8691246628056,-65.6572214156692,0.));
#64297=CARTESIAN_POINT('Ctrl Pts',(24.8691246628056,-65.6572214156692,12.));
#64298=CARTESIAN_POINT('Ctrl Pts',(24.8809778178228,-65.6733755087669,0.));
#64299=CARTESIAN_POINT('Ctrl Pts',(24.8809778178228,-65.6733755087669,12.));
#64300=CARTESIAN_POINT('Ctrl Pts',(24.8928794448607,-65.6895594608776,0.));
#64301=CARTESIAN_POINT('Ctrl Pts',(24.8928794448607,-65.6895594608776,12.));
#64302=CARTESIAN_POINT('Ctrl Pts',(24.9048295111448,-65.7057730980483,0.));
#64303=CARTESIAN_POINT('Ctrl Pts',(24.9048295111448,-65.7057730980483,12.));
#64304=CARTESIAN_POINT('Ctrl Pts',(24.9168279820106,-65.7220162391054,0.));
#64305=CARTESIAN_POINT('Ctrl Pts',(24.9168279820106,-65.7220162391054,12.));
#64306=CARTESIAN_POINT('Ctrl Pts',(24.928874819458,-65.7382886895888,0.));
#64307=CARTESIAN_POINT('Ctrl Pts',(24.928874819458,-65.7382886895888,12.));
#64308=CARTESIAN_POINT('Ctrl Pts',(24.9409699836537,-65.7545902480323,0.));
#64309=CARTESIAN_POINT('Ctrl Pts',(24.9409699836537,-65.7545902480323,12.));
#64310=CARTESIAN_POINT('Ctrl Pts',(24.9531134338696,-65.7709207098959,0.));
#64311=CARTESIAN_POINT('Ctrl Pts',(24.9531134338696,-65.7709207098959,12.));
#64312=CARTESIAN_POINT('Ctrl Pts',(24.965305129558,-65.7872798720823,0.));
#64313=CARTESIAN_POINT('Ctrl Pts',(24.965305129558,-65.7872798720823,12.));
#64314=CARTESIAN_POINT('Ctrl Pts',(24.9775450315682,-65.8036675380718,0.));
#64315=CARTESIAN_POINT('Ctrl Pts',(24.9775450315682,-65.8036675380718,12.));
#64316=CARTESIAN_POINT('Ctrl Pts',(24.9898331020983,-65.8200835177024,0.));
#64317=CARTESIAN_POINT('Ctrl Pts',(24.9898331020983,-65.8200835177024,12.));
#64318=CARTESIAN_POINT('Ctrl Pts',(25.0021693041169,-65.8365276247128,0.));
#64319=CARTESIAN_POINT('Ctrl Pts',(25.0021693041169,-65.8365276247128,12.));
#64320=CARTESIAN_POINT('Ctrl Pts',(25.0145536009604,-65.8529996750445,0.));
#64321=CARTESIAN_POINT('Ctrl Pts',(25.0145536009604,-65.8529996750445,12.));
#64322=CARTESIAN_POINT('Ctrl Pts',(25.0269859558362,-65.8694994847617,0.));
#64323=CARTESIAN_POINT('Ctrl Pts',(25.0269859558362,-65.8694994847617,12.));
#64324=CARTESIAN_POINT('Ctrl Pts',(25.0394663314055,-65.8860268683128,0.));
#64325=CARTESIAN_POINT('Ctrl Pts',(25.0394663314055,-65.8860268683128,12.));
#64326=CARTESIAN_POINT('Ctrl Pts',(25.0519946900078,-65.9025816394424,0.));
#64327=CARTESIAN_POINT('Ctrl Pts',(25.0519946900078,-65.9025816394424,12.));
#64328=CARTESIAN_POINT('Ctrl Pts',(25.0645709938524,-65.919163611981,0.));
#64329=CARTESIAN_POINT('Ctrl Pts',(25.0645709938524,-65.919163611981,12.));
#64330=CARTESIAN_POINT('Ctrl Pts',(25.0771952052028,-65.9357726006163,0.));
#64331=CARTESIAN_POINT('Ctrl Pts',(25.0771952052028,-65.9357726006163,12.));
#64332=CARTESIAN_POINT('Ctrl Pts',(25.0898672865915,-65.952408421814,0.));
#64333=CARTESIAN_POINT('Ctrl Pts',(25.0898672865915,-65.952408421814,12.));
#64334=CARTESIAN_POINT('Ctrl Pts',(25.1025872009003,-65.9690708941558,0.));
#64335=CARTESIAN_POINT('Ctrl Pts',(25.1025872009003,-65.9690708941558,12.));
#64336=CARTESIAN_POINT('Ctrl Pts',(25.1153549112503,-65.9857598378433,0.));
#64337=CARTESIAN_POINT('Ctrl Pts',(25.1153549112503,-65.9857598378433,12.));
#64338=CARTESIAN_POINT('Ctrl Pts',(25.1281703809297,-66.0024750743897,0.));
#64339=CARTESIAN_POINT('Ctrl Pts',(25.1281703809297,-66.0024750743897,12.));
#64340=CARTESIAN_POINT('Ctrl Pts',(25.1410335733098,-66.0192164262621,0.));
#64341=CARTESIAN_POINT('Ctrl Pts',(25.1410335733098,-66.0192164262621,12.));
#64342=CARTESIAN_POINT('Ctrl Pts',(25.1539444517418,-66.0359837164734,0.));
#64343=CARTESIAN_POINT('Ctrl Pts',(25.1539444517418,-66.0359837164734,12.));
#64344=CARTESIAN_POINT('Ctrl Pts',(25.166902979566,-66.0527767686025,0.));
#64345=CARTESIAN_POINT('Ctrl Pts',(25.166902979566,-66.0527767686025,12.));
#64346=CARTESIAN_POINT('Ctrl Pts',(25.1799091201599,-66.0695954069713,0.));
#64347=CARTESIAN_POINT('Ctrl Pts',(25.1799091201599,-66.0695954069713,12.));
#64348=CARTESIAN_POINT('Ctrl Pts',(25.1929628369684,-66.086439456768,0.));
#64349=CARTESIAN_POINT('Ctrl Pts',(25.1929628369684,-66.086439456768,12.));
#64350=CARTESIAN_POINT('Ctrl Pts',(25.2060640935365,-66.10330874419,0.));
#64351=CARTESIAN_POINT('Ctrl Pts',(25.2060640935365,-66.10330874419,12.));
#64352=CARTESIAN_POINT('Ctrl Pts',(25.2192128535357,-66.1202030965759,0.));
#64353=CARTESIAN_POINT('Ctrl Pts',(25.2192128535357,-66.1202030965759,12.));
#64354=CARTESIAN_POINT('Ctrl Pts',(25.2324090807549,-66.1371223423345,0.));
#64355=CARTESIAN_POINT('Ctrl Pts',(25.2324090807549,-66.1371223423345,12.));
#64356=CARTESIAN_POINT('Ctrl Pts',(25.2456527390874,-66.1540663108754,0.));
#64357=CARTESIAN_POINT('Ctrl Pts',(25.2456527390874,-66.1540663108754,12.));
#64358=CARTESIAN_POINT('Ctrl Pts',(25.2589437925146,-66.1710348325384,0.));
#64359=CARTESIAN_POINT('Ctrl Pts',(25.2589437925146,-66.1710348325384,12.));
#64360=CARTESIAN_POINT('Ctrl Pts',(25.2722822050836,-66.1880277385136,0.));
#64361=CARTESIAN_POINT('Ctrl Pts',(25.2722822050836,-66.1880277385136,12.));
#64362=CARTESIAN_POINT('Ctrl Pts',(25.285667940893,-66.2050448607911,0.));
#64363=CARTESIAN_POINT('Ctrl Pts',(25.285667940893,-66.2050448607911,12.));
#64364=CARTESIAN_POINT('Ctrl Pts',(25.2991009641094,-66.2220860321952,0.));
#64365=CARTESIAN_POINT('Ctrl Pts',(25.2991009641094,-66.2220860321952,12.));
#64366=CARTESIAN_POINT('Ctrl Pts',(25.3125812389729,-66.2391510863998,0.));
#64367=CARTESIAN_POINT('Ctrl Pts',(25.3125812389729,-66.2391510863998,12.));
#64368=CARTESIAN_POINT('Ctrl Pts',(25.3261087298026,-66.2562398579471,0.));
#64369=CARTESIAN_POINT('Ctrl Pts',(25.3261087298026,-66.2562398579471,12.));
#64370=CARTESIAN_POINT('Ctrl Pts',(25.3396834009949,-66.2733521822662,0.));
#64371=CARTESIAN_POINT('Ctrl Pts',(25.3396834009949,-66.2733521822662,12.));
#64372=CARTESIAN_POINT('Ctrl Pts',(25.3533052170248,-66.290487895671,0.));
#64373=CARTESIAN_POINT('Ctrl Pts',(25.3533052170248,-66.290487895671,12.));
#64374=CARTESIAN_POINT('Ctrl Pts',(25.3669741424488,-66.3076468353413,0.));
#64375=CARTESIAN_POINT('Ctrl Pts',(25.3669741424488,-66.3076468353413,12.));
#64376=CARTESIAN_POINT('Ctrl Pts',(25.3806901419012,-66.3248288393046,0.));
#64377=CARTESIAN_POINT('Ctrl Pts',(25.3806901419012,-66.3248288393046,12.));
#64378=CARTESIAN_POINT('Ctrl Pts',(25.3944531800901,-66.3420337464178,0.));
#64379=CARTESIAN_POINT('Ctrl Pts',(25.3944531800901,-66.3420337464178,12.));
#64380=CARTESIAN_POINT('Ctrl Pts',(25.4082632217847,-66.359261396341,0.));
#64381=CARTESIAN_POINT('Ctrl Pts',(25.4082632217847,-66.359261396341,12.));
#64382=CARTESIAN_POINT('Ctrl Pts',(25.4221202318199,-66.3765116295365,0.));
#64383=CARTESIAN_POINT('Ctrl Pts',(25.4221202318199,-66.3765116295365,12.));
#64384=CARTESIAN_POINT('Ctrl Pts',(25.4360241751017,-66.3937842872685,0.));
#64385=CARTESIAN_POINT('Ctrl Pts',(25.4360241751017,-66.3937842872685,12.));
#64386=CARTESIAN_POINT('Ctrl Pts',(25.4499750166078,-66.4110792116,0.));
#64387=CARTESIAN_POINT('Ctrl Pts',(25.4499750166078,-66.4110792116,12.));
#64388=CARTESIAN_POINT('Ctrl Pts',(25.4639727213849,-66.4283962453899,0.));
#64389=CARTESIAN_POINT('Ctrl Pts',(25.4639727213849,-66.4283962453899,12.));
#64390=CARTESIAN_POINT('Ctrl Pts',(25.4780172545417,-66.4457352322871,0.));
#64391=CARTESIAN_POINT('Ctrl Pts',(25.4780172545417,-66.4457352322871,12.));
#64392=CARTESIAN_POINT('Ctrl Pts',(25.4921085812547,-66.4630960167252,0.));
#64393=CARTESIAN_POINT('Ctrl Pts',(25.4921085812547,-66.4630960167252,12.));
#64394=CARTESIAN_POINT('Ctrl Pts',(25.5062466667702,-66.4804784439148,0.));
#64395=CARTESIAN_POINT('Ctrl Pts',(25.5062466667702,-66.4804784439148,12.));
#64396=CARTESIAN_POINT('Ctrl Pts',(25.5204314764033,-66.4978823598354,0.));
#64397=CARTESIAN_POINT('Ctrl Pts',(25.5204314764033,-66.4978823598354,12.));
#64398=CARTESIAN_POINT('Ctrl Pts',(25.534662975532,-66.5153076112231,0.));
#64399=CARTESIAN_POINT('Ctrl Pts',(25.534662975532,-66.5153076112231,12.));
#64400=CARTESIAN_POINT('Ctrl Pts',(25.5489411295911,-66.5327540455624,0.));
#64401=CARTESIAN_POINT('Ctrl Pts',(25.5489411295911,-66.5327540455624,12.));
#64402=CARTESIAN_POINT('Ctrl Pts',(25.5632659040792,-66.5502215110829,0.));
#64403=CARTESIAN_POINT('Ctrl Pts',(25.5632659040792,-66.5502215110829,12.));
#64404=CARTESIAN_POINT('Ctrl Pts',(25.5776372645601,-66.5677098567542,0.));
#64405=CARTESIAN_POINT('Ctrl Pts',(25.5776372645601,-66.5677098567542,12.));
#64406=CARTESIAN_POINT('Ctrl Pts',(25.5920551766629,-66.5852189322813,0.));
#64407=CARTESIAN_POINT('Ctrl Pts',(25.5920551766629,-66.5852189322813,12.));
#64408=CARTESIAN_POINT('Ctrl Pts',(25.6065196060755,-66.6027485880963,0.));
#64409=CARTESIAN_POINT('Ctrl Pts',(25.6065196060755,-66.6027485880963,12.));
#64410=CARTESIAN_POINT('Ctrl Pts',(25.6210305185403,-66.6202986753507,0.));
#64411=CARTESIAN_POINT('Ctrl Pts',(25.6210305185403,-66.6202986753507,12.));
#64412=CARTESIAN_POINT('Ctrl Pts',(25.6355878798613,-66.6378690459129,0.));
#64413=CARTESIAN_POINT('Ctrl Pts',(25.6355878798613,-66.6378690459129,12.));
#64414=CARTESIAN_POINT('Ctrl Pts',(25.6501916559055,-66.6554595523624,0.));
#64415=CARTESIAN_POINT('Ctrl Pts',(25.6501916559055,-66.6554595523624,12.));
#64416=CARTESIAN_POINT('Ctrl Pts',(25.6648418126013,-66.6730700479837,0.));
#64417=CARTESIAN_POINT('Ctrl Pts',(25.6648418126013,-66.6730700479837,12.));
#64418=CARTESIAN_POINT('Ctrl Pts',(25.6795383159319,-66.6907003867572,0.));
#64419=CARTESIAN_POINT('Ctrl Pts',(25.6795383159319,-66.6907003867572,12.));
#64420=CARTESIAN_POINT('Ctrl Pts',(25.6942811319322,-66.7083504233529,0.));
#64421=CARTESIAN_POINT('Ctrl Pts',(25.6942811319322,-66.7083504233529,12.));
#64422=CARTESIAN_POINT('Ctrl Pts',(25.7090702266962,-66.7260200131266,0.));
#64423=CARTESIAN_POINT('Ctrl Pts',(25.7090702266962,-66.7260200131266,12.));
#64424=CARTESIAN_POINT('Ctrl Pts',(25.7239055663772,-66.7437090121153,0.));
#64425=CARTESIAN_POINT('Ctrl Pts',(25.7239055663772,-66.7437090121153,12.));
#64426=CARTESIAN_POINT('Ctrl Pts',(25.7387871171866,-66.7614172770316,0.));
#64427=CARTESIAN_POINT('Ctrl Pts',(25.7387871171866,-66.7614172770316,12.));
#64428=CARTESIAN_POINT('Ctrl Pts',(25.7537148453863,-66.7791446652545,0.));
#64429=CARTESIAN_POINT('Ctrl Pts',(25.7537148453863,-66.7791446652545,12.));
#64430=CARTESIAN_POINT('Ctrl Pts',(25.7686887172877,-66.7968910348245,0.));
#64431=CARTESIAN_POINT('Ctrl Pts',(25.7686887172877,-66.7968910348245,12.));
#64432=CARTESIAN_POINT('Ctrl Pts',(25.7837086992594,-66.8146562444433,0.));
#64433=CARTESIAN_POINT('Ctrl Pts',(25.7837086992594,-66.8146562444433,12.));
#64434=CARTESIAN_POINT('Ctrl Pts',(25.7987747577269,-66.8324401534668,0.));
#64435=CARTESIAN_POINT('Ctrl Pts',(25.7987747577269,-66.8324401534668,12.));
#64436=CARTESIAN_POINT('Ctrl Pts',(25.8138868591709,-66.8502426219001,0.));
#64437=CARTESIAN_POINT('Ctrl Pts',(25.8138868591709,-66.8502426219001,12.));
#64438=CARTESIAN_POINT('Ctrl Pts',(25.8290449701192,-66.8680635103876,0.));
#64439=CARTESIAN_POINT('Ctrl Pts',(25.8290449701192,-66.8680635103876,12.));
#64440=CARTESIAN_POINT('Ctrl Pts',(25.844249057147,-66.8859026802088,0.));
#64441=CARTESIAN_POINT('Ctrl Pts',(25.844249057147,-66.8859026802088,12.));
#64442=CARTESIAN_POINT('Ctrl Pts',(25.8594990868833,-66.9037599932761,0.));
#64443=CARTESIAN_POINT('Ctrl Pts',(25.8594990868833,-66.9037599932761,12.));
#64444=CARTESIAN_POINT('Ctrl Pts',(25.874795026011,-66.92163531213,0.));
#64445=CARTESIAN_POINT('Ctrl Pts',(25.874795026011,-66.92163531213,12.));
#64446=CARTESIAN_POINT('Ctrl Pts',(25.890136841266,-66.939528499934,0.));
#64447=CARTESIAN_POINT('Ctrl Pts',(25.890136841266,-66.939528499934,12.));
#64448=CARTESIAN_POINT('Ctrl Pts',(25.9055244994277,-66.9574394204663,0.));
#64449=CARTESIAN_POINT('Ctrl Pts',(25.9055244994277,-66.9574394204663,12.));
#64450=CARTESIAN_POINT('Ctrl Pts',(25.9209579673209,-66.975367938115,0.));
#64451=CARTESIAN_POINT('Ctrl Pts',(25.9209579673209,-66.975367938115,12.));
#64452=CARTESIAN_POINT('Ctrl Pts',(25.9364372118222,-66.9933139178778,0.));
#64453=CARTESIAN_POINT('Ctrl Pts',(25.9364372118222,-66.9933139178778,12.));
#64454=CARTESIAN_POINT('Ctrl Pts',(25.9519621998598,-67.0112772253556,0.));
#64455=CARTESIAN_POINT('Ctrl Pts',(25.9519621998598,-67.0112772253556,12.));
#64456=CARTESIAN_POINT('Ctrl Pts',(25.967532898412,-67.0292577267489,0.));
#64457=CARTESIAN_POINT('Ctrl Pts',(25.967532898412,-67.0292577267489,12.));
#64458=CARTESIAN_POINT('Ctrl Pts',(25.9831492744983,-67.0472552888485,0.));
#64459=CARTESIAN_POINT('Ctrl Pts',(25.9831492744983,-67.0472552888485,12.));
#64460=CARTESIAN_POINT('Ctrl Pts',(25.9988112951814,-67.0652697790325,0.));
#64461=CARTESIAN_POINT('Ctrl Pts',(25.9988112951814,-67.0652697790325,12.));
#64462=CARTESIAN_POINT('Ctrl Pts',(26.014518927573,-67.0833010652634,0.));
#64463=CARTESIAN_POINT('Ctrl Pts',(26.014518927573,-67.0833010652634,12.));
#64464=CARTESIAN_POINT('Ctrl Pts',(26.0302721388339,-67.101349016084,0.));
#64465=CARTESIAN_POINT('Ctrl Pts',(26.0302721388339,-67.101349016084,12.));
#64466=CARTESIAN_POINT('Ctrl Pts',(26.0460708961725,-67.1194135006124,0.));
#64467=CARTESIAN_POINT('Ctrl Pts',(26.0460708961725,-67.1194135006124,12.));
#64468=CARTESIAN_POINT('Ctrl Pts',(26.061915166836,-67.1374943885354,0.));
#64469=CARTESIAN_POINT('Ctrl Pts',(26.061915166836,-67.1374943885354,12.));
#64470=CARTESIAN_POINT('Ctrl Pts',(26.0778049181128,-67.1555915501049,0.));
#64471=CARTESIAN_POINT('Ctrl Pts',(26.0778049181128,-67.1555915501049,12.));
#64472=CARTESIAN_POINT('Ctrl Pts',(26.0937401173383,-67.173704856136,0.));
#64473=CARTESIAN_POINT('Ctrl Pts',(26.0937401173383,-67.173704856136,12.));
#64474=CARTESIAN_POINT('Ctrl Pts',(26.1097207318949,-67.1918341780018,0.));
#64475=CARTESIAN_POINT('Ctrl Pts',(26.1097207318949,-67.1918341780018,12.));
#64476=CARTESIAN_POINT('Ctrl Pts',(26.1257467292102,-67.2099793876297,0.));
#64477=CARTESIAN_POINT('Ctrl Pts',(26.1257467292102,-67.2099793876297,12.));
#64478=CARTESIAN_POINT('Ctrl Pts',(26.1418180767489,-67.2281403574938,0.));
#64479=CARTESIAN_POINT('Ctrl Pts',(26.1418180767489,-67.2281403574938,12.));
#64480=CARTESIAN_POINT('Ctrl Pts',(26.1579347420138,-67.2463169606115,0.));
#64481=CARTESIAN_POINT('Ctrl Pts',(26.1579347420138,-67.2463169606115,12.));
#64482=CARTESIAN_POINT('Ctrl Pts',(26.1740966925528,-67.2645090705421,0.));
#64483=CARTESIAN_POINT('Ctrl Pts',(26.1740966925528,-67.2645090705421,12.));
#64484=CARTESIAN_POINT('Ctrl Pts',(26.1903038959589,-67.282716561383,0.));
#64485=CARTESIAN_POINT('Ctrl Pts',(26.1903038959589,-67.282716561383,12.));
#64486=CARTESIAN_POINT('Ctrl Pts',(26.2065563198683,-67.3009393077652,0.));
#64487=CARTESIAN_POINT('Ctrl Pts',(26.2065563198683,-67.3009393077652,12.));
#64488=CARTESIAN_POINT('Ctrl Pts',(26.2228539319526,-67.3191771848464,0.));
#64489=CARTESIAN_POINT('Ctrl Pts',(26.2228539319526,-67.3191771848464,12.));
#64490=CARTESIAN_POINT('Ctrl Pts',(26.2391966999191,-67.3374300683074,0.));
#64491=CARTESIAN_POINT('Ctrl Pts',(26.2391966999191,-67.3374300683074,12.));
#64492=CARTESIAN_POINT('Ctrl Pts',(26.255584591518,-67.3556978343507,0.));
#64493=CARTESIAN_POINT('Ctrl Pts',(26.255584591518,-67.3556978343507,12.));
#64494=CARTESIAN_POINT('Ctrl Pts',(26.2720175745423,-67.3739803596969,0.));
#64495=CARTESIAN_POINT('Ctrl Pts',(26.2720175745423,-67.3739803596969,12.));
#64496=CARTESIAN_POINT('Ctrl Pts',(26.2884956168269,-67.392277521581,0.));
#64497=CARTESIAN_POINT('Ctrl Pts',(26.2884956168269,-67.392277521581,12.));
#64498=CARTESIAN_POINT('Ctrl Pts',(26.3050186862407,-67.4105891977461,0.));
#64499=CARTESIAN_POINT('Ctrl Pts',(26.3050186862407,-67.4105891977461,12.));
#64500=CARTESIAN_POINT('Ctrl Pts',(26.321586750686,-67.4289152664398,0.));
#64501=CARTESIAN_POINT('Ctrl Pts',(26.321586750686,-67.4289152664398,12.));
#64502=CARTESIAN_POINT('Ctrl Pts',(26.3381997781055,-67.4472556064119,0.));
#64503=CARTESIAN_POINT('Ctrl Pts',(26.3381997781055,-67.4472556064119,12.));
#64504=CARTESIAN_POINT('Ctrl Pts',(26.3548577364833,-67.4656100969116,0.));
#64505=CARTESIAN_POINT('Ctrl Pts',(26.3548577364833,-67.4656100969116,12.));
#64506=CARTESIAN_POINT('Ctrl Pts',(26.3715605938432,-67.4839786176836,0.));
#64507=CARTESIAN_POINT('Ctrl Pts',(26.3715605938432,-67.4839786176836,12.));
#64508=CARTESIAN_POINT('Ctrl Pts',(26.3883083182421,-67.5023610489622,0.));
#64509=CARTESIAN_POINT('Ctrl Pts',(26.3883083182421,-67.5023610489622,12.));
#64510=CARTESIAN_POINT('Ctrl Pts',(26.4051008777675,-67.5207572714683,0.));
#64511=CARTESIAN_POINT('Ctrl Pts',(26.4051008777675,-67.5207572714683,12.));
#64512=CARTESIAN_POINT('Ctrl Pts',(26.4219382405458,-67.5391671664072,0.));
#64513=CARTESIAN_POINT('Ctrl Pts',(26.4219382405458,-67.5391671664072,12.));
#64514=CARTESIAN_POINT('Ctrl Pts',(26.4388203747425,-67.5575906154657,0.));
#64515=CARTESIAN_POINT('Ctrl Pts',(26.4388203747425,-67.5575906154657,12.));
#64516=CARTESIAN_POINT('Ctrl Pts',(26.455747248562,-67.5760275008093,0.));
#64517=CARTESIAN_POINT('Ctrl Pts',(26.455747248562,-67.5760275008093,12.));
#64518=CARTESIAN_POINT('Ctrl Pts',(26.4727188302409,-67.5944777050768,0.));
#64519=CARTESIAN_POINT('Ctrl Pts',(26.4727188302409,-67.5944777050768,12.));
#64520=CARTESIAN_POINT('Ctrl Pts',(26.4897350880439,-67.6129411113758,0.));
#64521=CARTESIAN_POINT('Ctrl Pts',(26.4897350880439,-67.6129411113758,12.));
#64522=CARTESIAN_POINT('Ctrl Pts',(26.5067959902725,-67.6314176032811,0.));
#64523=CARTESIAN_POINT('Ctrl Pts',(26.5067959902725,-67.6314176032811,12.));
#64524=CARTESIAN_POINT('Ctrl Pts',(26.5239015052653,-67.649907064832,0.));
#64525=CARTESIAN_POINT('Ctrl Pts',(26.5239015052653,-67.649907064832,12.));
#64526=CARTESIAN_POINT('Ctrl Pts',(26.5410516013984,-67.6684093805291,0.));
#64527=CARTESIAN_POINT('Ctrl Pts',(26.5410516013984,-67.6684093805291,12.));
#64528=CARTESIAN_POINT('Ctrl Pts',(26.5582462470794,-67.6869244353294,0.));
#64529=CARTESIAN_POINT('Ctrl Pts',(26.5582462470794,-67.6869244353294,12.));
#64530=CARTESIAN_POINT('Ctrl Pts',(26.5754854107421,-67.7054521146425,0.));
#64531=CARTESIAN_POINT('Ctrl Pts',(26.5754854107421,-67.7054521146425,12.));
#64532=CARTESIAN_POINT('Ctrl Pts',(26.5927690608543,-67.7239923043288,0.));
#64533=CARTESIAN_POINT('Ctrl Pts',(26.5927690608543,-67.7239923043288,12.));
#64534=CARTESIAN_POINT('Ctrl Pts',(26.6100971659201,-67.7425448906977,0.));
#64535=CARTESIAN_POINT('Ctrl Pts',(26.6100971659201,-67.7425448906977,12.));
#64536=CARTESIAN_POINT('Ctrl Pts',(26.6274696944792,-67.7611097605042,0.));
#64537=CARTESIAN_POINT('Ctrl Pts',(26.6274696944792,-67.7611097605042,12.));
#64538=CARTESIAN_POINT('Ctrl Pts',(26.6448866151029,-67.7796868009455,0.));
#64539=CARTESIAN_POINT('Ctrl Pts',(26.6448866151029,-67.7796868009455,12.));
#64540=CARTESIAN_POINT('Ctrl Pts',(26.662347896387,-67.798275899657,0.));
#64541=CARTESIAN_POINT('Ctrl Pts',(26.662347896387,-67.798275899657,12.));
#64542=CARTESIAN_POINT('Ctrl Pts',(26.6798535069589,-67.8168769447098,0.));
#64543=CARTESIAN_POINT('Ctrl Pts',(26.6798535069589,-67.8168769447098,12.));
#64544=CARTESIAN_POINT('Ctrl Pts',(26.6974034154804,-67.8354898246086,0.));
#64545=CARTESIAN_POINT('Ctrl Pts',(26.6974034154804,-67.8354898246086,12.));
#64546=CARTESIAN_POINT('Ctrl Pts',(26.7149975906477,-67.8541144282875,0.));
#64547=CARTESIAN_POINT('Ctrl Pts',(26.7149975906477,-67.8541144282875,12.));
#64548=CARTESIAN_POINT('Ctrl Pts',(26.7326360011884,-67.8727506451064,0.));
#64549=CARTESIAN_POINT('Ctrl Pts',(26.7326360011884,-67.8727506451064,12.));
#64550=CARTESIAN_POINT('Ctrl Pts',(26.7503186158522,-67.8913983648437,0.));
#64551=CARTESIAN_POINT('Ctrl Pts',(26.7503186158522,-67.8913983648437,12.));
#64552=CARTESIAN_POINT('Ctrl Pts',(26.7680454034168,-67.9100574776972,0.));
#64553=CARTESIAN_POINT('Ctrl Pts',(26.7680454034168,-67.9100574776972,12.));
#64554=CARTESIAN_POINT('Ctrl Pts',(26.7858163326933,-67.928727874284,0.));
#64555=CARTESIAN_POINT('Ctrl Pts',(26.7858163326933,-67.928727874284,12.));
#64556=CARTESIAN_POINT('Ctrl Pts',(26.8036313725262,-67.9474094456396,0.));
#64557=CARTESIAN_POINT('Ctrl Pts',(26.8036313725262,-67.9474094456396,12.));
#64558=CARTESIAN_POINT('Ctrl Pts',(26.821490491792,-67.9661020832164,0.));
#64559=CARTESIAN_POINT('Ctrl Pts',(26.821490491792,-67.9661020832164,12.));
#64560=CARTESIAN_POINT('Ctrl Pts',(26.8393936593911,-67.9848056788809,0.));
#64561=CARTESIAN_POINT('Ctrl Pts',(26.8393936593911,-67.9848056788809,12.));
#64562=CARTESIAN_POINT('Ctrl Pts',(26.8573408442496,-68.0035201249102,0.));
#64563=CARTESIAN_POINT('Ctrl Pts',(26.8573408442496,-68.0035201249102,12.));
#64564=CARTESIAN_POINT('Ctrl Pts',(26.8753320153251,-68.0222453139856,0.));
#64565=CARTESIAN_POINT('Ctrl Pts',(26.8753320153251,-68.0222453139856,12.));
#64566=CARTESIAN_POINT('Ctrl Pts',(26.8933671416062,-68.0409811391869,0.));
#64567=CARTESIAN_POINT('Ctrl Pts',(26.8933671416062,-68.0409811391869,12.));
#64568=CARTESIAN_POINT('Ctrl Pts',(26.9114461921109,-68.0597274939859,0.));
#64569=CARTESIAN_POINT('Ctrl Pts',(26.9114461921109,-68.0597274939859,12.));
#64570=CARTESIAN_POINT('Ctrl Pts',(26.9295691358778,-68.0784842722369,0.));
#64571=CARTESIAN_POINT('Ctrl Pts',(26.9295691358778,-68.0784842722369,12.));
#64572=CARTESIAN_POINT('Ctrl Pts',(26.9477359419651,-68.0972513681751,0.));
#64573=CARTESIAN_POINT('Ctrl Pts',(26.9477359419651,-68.0972513681751,12.));
#64574=CARTESIAN_POINT('Ctrl Pts',(26.9659465794601,-68.1160286764255,0.));
#64575=CARTESIAN_POINT('Ctrl Pts',(26.9659465794601,-68.1160286764255,12.));
#64576=CARTESIAN_POINT('Ctrl Pts',(26.9842010174821,-68.1348160920107,0.));
#64577=CARTESIAN_POINT('Ctrl Pts',(26.9842010174821,-68.1348160920107,12.));
#64578=CARTESIAN_POINT('Ctrl Pts',(27.0024992251838,-68.1536135103557,0.));
#64579=CARTESIAN_POINT('Ctrl Pts',(27.0024992251838,-68.1536135103557,12.));
#64580=CARTESIAN_POINT('Ctrl Pts',(27.0208411717472,-68.1724208272958,0.));
#64581=CARTESIAN_POINT('Ctrl Pts',(27.0208411717472,-68.1724208272958,12.));
#64582=CARTESIAN_POINT('Ctrl Pts',(27.0392268263797,-68.1912379390773,0.));
#64583=CARTESIAN_POINT('Ctrl Pts',(27.0392268263797,-68.1912379390773,12.));
#64584=CARTESIAN_POINT('Ctrl Pts',(27.0576561583172,-68.2100647423332,0.));
#64585=CARTESIAN_POINT('Ctrl Pts',(27.0576561583172,-68.2100647423332,12.));
#64586=CARTESIAN_POINT('Ctrl Pts',(27.0761291368225,-68.2289011340615,0.));
#64587=CARTESIAN_POINT('Ctrl Pts',(27.0761291368225,-68.2289011340615,12.));
#64588=CARTESIAN_POINT('Ctrl Pts',(27.0946457311812,-68.2477470116013,0.));
#64589=CARTESIAN_POINT('Ctrl Pts',(27.0946457311812,-68.2477470116013,12.));
#64590=CARTESIAN_POINT('Ctrl Pts',(27.1132059106943,-68.2666022726104,0.));
#64591=CARTESIAN_POINT('Ctrl Pts',(27.1132059106943,-68.2666022726104,12.));
#64592=CARTESIAN_POINT('Ctrl Pts',(27.1318096446648,-68.2854668150364,0.));
#64593=CARTESIAN_POINT('Ctrl Pts',(27.1318096446648,-68.2854668150364,12.));
#64594=CARTESIAN_POINT('Ctrl Pts',(27.1504569024136,-68.3043405371603,0.));
#64595=CARTESIAN_POINT('Ctrl Pts',(27.1504569024136,-68.3043405371603,12.));
#64596=CARTESIAN_POINT('Ctrl Pts',(27.1691476532921,-68.3232233376425,0.));
#64597=CARTESIAN_POINT('Ctrl Pts',(27.1691476532921,-68.3232233376425,12.));
#64598=CARTESIAN_POINT('Ctrl Pts',(27.1878818666926,-68.3421151155711,0.));
#64599=CARTESIAN_POINT('Ctrl Pts',(27.1878818666926,-68.3421151155711,12.));
#64600=CARTESIAN_POINT('Ctrl Pts',(27.2066595120541,-68.3610157704994,0.));
#64601=CARTESIAN_POINT('Ctrl Pts',(27.2066595120541,-68.3610157704994,12.));
#64602=CARTESIAN_POINT('Ctrl Pts',(27.2254805588673,-68.3799252025102,0.));
#64603=CARTESIAN_POINT('Ctrl Pts',(27.2254805588673,-68.3799252025102,12.));
#64604=CARTESIAN_POINT('Ctrl Pts',(27.244344976665,-68.3988433121581,0.));
#64605=CARTESIAN_POINT('Ctrl Pts',(27.244344976665,-68.3988433121581,12.));
#64606=CARTESIAN_POINT('Ctrl Pts',(27.2632527350059,-68.4177700003465,0.));
#64607=CARTESIAN_POINT('Ctrl Pts',(27.2632527350059,-68.4177700003465,12.));
#64608=CARTESIAN_POINT('Ctrl Pts',(27.2822038034538,-68.4367051682164,0.));
#64609=CARTESIAN_POINT('Ctrl Pts',(27.2822038034538,-68.4367051682164,12.));
#64610=CARTESIAN_POINT('Ctrl Pts',(27.301198151557,-68.4556487170441,0.));
#64611=CARTESIAN_POINT('Ctrl Pts',(27.301198151557,-68.4556487170441,12.));
#64612=CARTESIAN_POINT('Ctrl Pts',(27.3202357488154,-68.4746005480997,0.));
#64613=CARTESIAN_POINT('Ctrl Pts',(27.3202357488154,-68.4746005480997,12.));
#64614=CARTESIAN_POINT('Ctrl Pts',(27.3393165646751,-68.4935605626372,0.));
#64615=CARTESIAN_POINT('Ctrl Pts',(27.3393165646751,-68.4935605626372,12.));
#64616=CARTESIAN_POINT('Ctrl Pts',(27.3584405685947,-68.5125286621902,0.));
#64617=CARTESIAN_POINT('Ctrl Pts',(27.3584405685947,-68.5125286621902,12.));
#64618=CARTESIAN_POINT('Ctrl Pts',(27.3776077300918,-68.5315047488046,0.));
#64619=CARTESIAN_POINT('Ctrl Pts',(27.3776077300918,-68.5315047488046,12.));
#64620=CARTESIAN_POINT('Ctrl Pts',(27.3968180187941,-68.5504887252976,0.));
#64621=CARTESIAN_POINT('Ctrl Pts',(27.3968180187941,-68.5504887252976,12.));
#64622=CARTESIAN_POINT('Ctrl Pts',(27.4160714044825,-68.5694804955002,0.));
#64623=CARTESIAN_POINT('Ctrl Pts',(27.4160714044825,-68.5694804955002,12.));
#64624=CARTESIAN_POINT('Ctrl Pts',(27.4353678571349,-68.5884799645193,0.));
#64625=CARTESIAN_POINT('Ctrl Pts',(27.4353678571349,-68.5884799645193,12.));
#64626=CARTESIAN_POINT('Ctrl Pts',(27.4547073468212,-68.6074870381588,0.));
#64627=CARTESIAN_POINT('Ctrl Pts',(27.4547073468212,-68.6074870381588,12.));
#64628=CARTESIAN_POINT('Ctrl Pts',(27.4740898435976,-68.6265016223536,0.));
#64629=CARTESIAN_POINT('Ctrl Pts',(27.4740898435976,-68.6265016223536,12.));
#64630=CARTESIAN_POINT('Ctrl Pts',(27.4935153173863,-68.6455236225471,0.));
#64631=CARTESIAN_POINT('Ctrl Pts',(27.4935153173863,-68.6455236225471,12.));
#64632=CARTESIAN_POINT('Ctrl Pts',(27.5129837378797,-68.664552943206,0.));
#64633=CARTESIAN_POINT('Ctrl Pts',(27.5129837378797,-68.664552943206,12.));
#64634=CARTESIAN_POINT('Ctrl Pts',(27.5324950743722,-68.683589486992,0.));
#64635=CARTESIAN_POINT('Ctrl Pts',(27.5324950743722,-68.683589486992,12.));
#64636=CARTESIAN_POINT('Ctrl Pts',(27.552049295893,-68.7026331554349,0.));
#64637=CARTESIAN_POINT('Ctrl Pts',(27.552049295893,-68.7026331554349,12.));
#64638=CARTESIAN_POINT('Ctrl Pts',(27.5716463715027,-68.721683850427,0.));
#64639=CARTESIAN_POINT('Ctrl Pts',(27.5716463715027,-68.721683850427,12.));
#64640=CARTESIAN_POINT('Ctrl Pts',(27.5912862705482,-68.7407414755291,0.));
#64641=CARTESIAN_POINT('Ctrl Pts',(27.5912862705482,-68.7407414755291,12.));
#64642=CARTESIAN_POINT('Ctrl Pts',(27.6109689629025,-68.7598059372121,0.));
#64643=CARTESIAN_POINT('Ctrl Pts',(27.6109689629025,-68.7598059372121,12.));
#64644=CARTESIAN_POINT('Ctrl Pts',(27.6306944192711,-68.7788771464655,0.));
#64645=CARTESIAN_POINT('Ctrl Pts',(27.6306944192711,-68.7788771464655,12.));
#64646=CARTESIAN_POINT('Ctrl Pts',(27.6504626112621,-68.7979550191773,0.));
#64647=CARTESIAN_POINT('Ctrl Pts',(27.6504626112621,-68.7979550191773,12.));
#64648=CARTESIAN_POINT('Ctrl Pts',(27.6702735107069,-68.8170394725786,0.));
#64649=CARTESIAN_POINT('Ctrl Pts',(27.6702735107069,-68.8170394725786,12.));
#64650=CARTESIAN_POINT('Ctrl Pts',(27.6901270891201,-68.8361304224378,0.));
#64651=CARTESIAN_POINT('Ctrl Pts',(27.6901270891201,-68.8361304224378,12.));
#64652=CARTESIAN_POINT('Ctrl Pts',(27.7100233170728,-68.8552277798181,0.));
#64653=CARTESIAN_POINT('Ctrl Pts',(27.7100233170728,-68.8552277798181,12.));
#64654=CARTESIAN_POINT('Ctrl Pts',(27.7299621636602,-68.8743314483451,0.));
#64655=CARTESIAN_POINT('Ctrl Pts',(27.7299621636602,-68.8743314483451,12.));
#64656=CARTESIAN_POINT('Ctrl Pts',(27.7499435957607,-68.8934413203945,0.));
#64657=CARTESIAN_POINT('Ctrl Pts',(27.7499435957607,-68.8934413203945,12.));
#64658=CARTESIAN_POINT('Ctrl Pts',(27.7699675790683,-68.9125572825946,0.));
#64659=CARTESIAN_POINT('Ctrl Pts',(27.7699675790683,-68.9125572825946,12.));
#64660=CARTESIAN_POINT('Ctrl Pts',(27.7900340793796,-68.9316792226187,0.));
#64661=CARTESIAN_POINT('Ctrl Pts',(27.7900340793796,-68.9316792226187,12.));
#64662=CARTESIAN_POINT('Ctrl Pts',(27.8101430638128,-68.9508070357786,0.));
#64663=CARTESIAN_POINT('Ctrl Pts',(27.8101430638128,-68.9508070357786,12.));
#64664=CARTESIAN_POINT('Ctrl Pts',(27.8302945019938,-68.9699406311305,0.));
#64665=CARTESIAN_POINT('Ctrl Pts',(27.8302945019938,-68.9699406311305,12.));
#64666=CARTESIAN_POINT('Ctrl Pts',(27.8504883673902,-68.9890799391863,0.));
#64667=CARTESIAN_POINT('Ctrl Pts',(27.8504883673902,-68.9890799391863,12.));
#64668=CARTESIAN_POINT('Ctrl Pts',(27.8707246380697,-69.0082249138015,0.));
#64669=CARTESIAN_POINT('Ctrl Pts',(27.8707246380697,-69.0082249138015,12.));
#64670=CARTESIAN_POINT('Ctrl Pts',(27.8910032967036,-69.0273755264702,0.));
#64671=CARTESIAN_POINT('Ctrl Pts',(27.8910032967036,-69.0273755264702,12.));
#64672=CARTESIAN_POINT('Ctrl Pts',(27.9072601239469,-69.0427005153223,0.));
#64673=CARTESIAN_POINT('Ctrl Pts',(27.9072601239469,-69.0427005153223,12.));
#64674=CARTESIAN_POINT('Ctrl Pts',(27.919471809885,-69.0541967850685,0.));
#64675=CARTESIAN_POINT('Ctrl Pts',(27.919471809885,-69.0541967850685,12.));
#64676=CARTESIAN_POINT('Ctrl Pts',(27.9276214070575,-69.0618620884596,0.));
#64677=CARTESIAN_POINT('Ctrl Pts',(27.9276214070575,-69.0618620884596,12.));
#64678=CARTESIAN_POINT('Ctrl Pts',(27.9316983239472,-69.065695021045,0.));
#64679=CARTESIAN_POINT('Ctrl Pts',(27.9316983239472,-69.065695021045,12.));
#64680=CARTESIAN_POINT('',(24.7419628022041,-65.4815644032299,0.));
#64681=CARTESIAN_POINT('Ctrl Pts',(24.7419628022041,-65.4815644032299,0.));
#64682=CARTESIAN_POINT('Ctrl Pts',(24.7442214063382,-65.4847237095443,0.));
#64683=CARTESIAN_POINT('Ctrl Pts',(24.7487434955981,-65.4910454936254,0.));
#64684=CARTESIAN_POINT('Ctrl Pts',(24.7555412724651,-65.5005376841101,0.));
#64685=CARTESIAN_POINT('Ctrl Pts',(24.7646342620841,-65.5132129675333,0.));
#64686=CARTESIAN_POINT('Ctrl Pts',(24.7760493148465,-65.5290887770232,0.));
#64687=CARTESIAN_POINT('Ctrl Pts',(24.787513182749,-65.5449962514662,0.));
#64688=CARTESIAN_POINT('Ctrl Pts',(24.7990258561259,-65.5609353062829,0.));
#64689=CARTESIAN_POINT('Ctrl Pts',(24.8105873098626,-65.5769057914333,0.));
#64690=CARTESIAN_POINT('Ctrl Pts',(24.8221975032103,-65.5929074932624,0.));
#64691=CARTESIAN_POINT('Ctrl Pts',(24.8338563866763,-65.6089401625628,0.));
#64692=CARTESIAN_POINT('Ctrl Pts',(24.8455639071516,-65.6250035361612,0.));
#64693=CARTESIAN_POINT('Ctrl Pts',(24.8573200135665,-65.6410973603661,0.));
#64694=CARTESIAN_POINT('Ctrl Pts',(24.8691246628056,-65.6572214156692,0.));
#64695=CARTESIAN_POINT('Ctrl Pts',(24.8809778178228,-65.6733755087669,0.));
#64696=CARTESIAN_POINT('Ctrl Pts',(24.8928794448607,-65.6895594608776,0.));
#64697=CARTESIAN_POINT('Ctrl Pts',(24.9048295111448,-65.7057730980483,0.));
#64698=CARTESIAN_POINT('Ctrl Pts',(24.9168279820106,-65.7220162391054,0.));
#64699=CARTESIAN_POINT('Ctrl Pts',(24.928874819458,-65.7382886895888,0.));
#64700=CARTESIAN_POINT('Ctrl Pts',(24.9409699836537,-65.7545902480323,0.));
#64701=CARTESIAN_POINT('Ctrl Pts',(24.9531134338696,-65.7709207098959,0.));
#64702=CARTESIAN_POINT('Ctrl Pts',(24.965305129558,-65.7872798720823,0.));
#64703=CARTESIAN_POINT('Ctrl Pts',(24.9775450315682,-65.8036675380718,0.));
#64704=CARTESIAN_POINT('Ctrl Pts',(24.9898331020983,-65.8200835177024,0.));
#64705=CARTESIAN_POINT('Ctrl Pts',(25.0021693041169,-65.8365276247128,0.));
#64706=CARTESIAN_POINT('Ctrl Pts',(25.0145536009604,-65.8529996750445,0.));
#64707=CARTESIAN_POINT('Ctrl Pts',(25.0269859558362,-65.8694994847617,0.));
#64708=CARTESIAN_POINT('Ctrl Pts',(25.0394663314055,-65.8860268683128,0.));
#64709=CARTESIAN_POINT('Ctrl Pts',(25.0519946900078,-65.9025816394424,0.));
#64710=CARTESIAN_POINT('Ctrl Pts',(25.0645709938524,-65.919163611981,0.));
#64711=CARTESIAN_POINT('Ctrl Pts',(25.0771952052028,-65.9357726006163,0.));
#64712=CARTESIAN_POINT('Ctrl Pts',(25.0898672865915,-65.952408421814,0.));
#64713=CARTESIAN_POINT('Ctrl Pts',(25.1025872009003,-65.9690708941558,0.));
#64714=CARTESIAN_POINT('Ctrl Pts',(25.1153549112503,-65.9857598378433,0.));
#64715=CARTESIAN_POINT('Ctrl Pts',(25.1281703809297,-66.0024750743897,0.));
#64716=CARTESIAN_POINT('Ctrl Pts',(25.1410335733098,-66.0192164262621,0.));
#64717=CARTESIAN_POINT('Ctrl Pts',(25.1539444517418,-66.0359837164734,0.));
#64718=CARTESIAN_POINT('Ctrl Pts',(25.166902979566,-66.0527767686025,0.));
#64719=CARTESIAN_POINT('Ctrl Pts',(25.1799091201599,-66.0695954069713,0.));
#64720=CARTESIAN_POINT('Ctrl Pts',(25.1929628369684,-66.086439456768,0.));
#64721=CARTESIAN_POINT('Ctrl Pts',(25.2060640935365,-66.10330874419,0.));
#64722=CARTESIAN_POINT('Ctrl Pts',(25.2192128535357,-66.1202030965759,0.));
#64723=CARTESIAN_POINT('Ctrl Pts',(25.2324090807549,-66.1371223423345,0.));
#64724=CARTESIAN_POINT('Ctrl Pts',(25.2456527390874,-66.1540663108754,0.));
#64725=CARTESIAN_POINT('Ctrl Pts',(25.2589437925146,-66.1710348325384,0.));
#64726=CARTESIAN_POINT('Ctrl Pts',(25.2722822050836,-66.1880277385136,0.));
#64727=CARTESIAN_POINT('Ctrl Pts',(25.285667940893,-66.2050448607911,0.));
#64728=CARTESIAN_POINT('Ctrl Pts',(25.2991009641094,-66.2220860321952,0.));
#64729=CARTESIAN_POINT('Ctrl Pts',(25.3125812389729,-66.2391510863998,0.));
#64730=CARTESIAN_POINT('Ctrl Pts',(25.3261087298026,-66.2562398579471,0.));
#64731=CARTESIAN_POINT('Ctrl Pts',(25.3396834009949,-66.2733521822662,0.));
#64732=CARTESIAN_POINT('Ctrl Pts',(25.3533052170248,-66.290487895671,0.));
#64733=CARTESIAN_POINT('Ctrl Pts',(25.3669741424488,-66.3076468353413,0.));
#64734=CARTESIAN_POINT('Ctrl Pts',(25.3806901419012,-66.3248288393046,0.));
#64735=CARTESIAN_POINT('Ctrl Pts',(25.3944531800901,-66.3420337464178,0.));
#64736=CARTESIAN_POINT('Ctrl Pts',(25.4082632217847,-66.359261396341,0.));
#64737=CARTESIAN_POINT('Ctrl Pts',(25.4221202318199,-66.3765116295365,0.));
#64738=CARTESIAN_POINT('Ctrl Pts',(25.4360241751017,-66.3937842872685,0.));
#64739=CARTESIAN_POINT('Ctrl Pts',(25.4499750166078,-66.4110792116,0.));
#64740=CARTESIAN_POINT('Ctrl Pts',(25.4639727213849,-66.4283962453899,0.));
#64741=CARTESIAN_POINT('Ctrl Pts',(25.4780172545417,-66.4457352322871,0.));
#64742=CARTESIAN_POINT('Ctrl Pts',(25.4921085812547,-66.4630960167252,0.));
#64743=CARTESIAN_POINT('Ctrl Pts',(25.5062466667702,-66.4804784439148,0.));
#64744=CARTESIAN_POINT('Ctrl Pts',(25.5204314764033,-66.4978823598354,0.));
#64745=CARTESIAN_POINT('Ctrl Pts',(25.534662975532,-66.5153076112231,0.));
#64746=CARTESIAN_POINT('Ctrl Pts',(25.5489411295911,-66.5327540455624,0.));
#64747=CARTESIAN_POINT('Ctrl Pts',(25.5632659040792,-66.5502215110829,0.));
#64748=CARTESIAN_POINT('Ctrl Pts',(25.5776372645601,-66.5677098567542,0.));
#64749=CARTESIAN_POINT('Ctrl Pts',(25.5920551766629,-66.5852189322813,0.));
#64750=CARTESIAN_POINT('Ctrl Pts',(25.6065196060755,-66.6027485880963,0.));
#64751=CARTESIAN_POINT('Ctrl Pts',(25.6210305185403,-66.6202986753507,0.));
#64752=CARTESIAN_POINT('Ctrl Pts',(25.6355878798613,-66.6378690459129,0.));
#64753=CARTESIAN_POINT('Ctrl Pts',(25.6501916559055,-66.6554595523624,0.));
#64754=CARTESIAN_POINT('Ctrl Pts',(25.6648418126013,-66.6730700479837,0.));
#64755=CARTESIAN_POINT('Ctrl Pts',(25.6795383159319,-66.6907003867572,0.));
#64756=CARTESIAN_POINT('Ctrl Pts',(25.6942811319322,-66.7083504233529,0.));
#64757=CARTESIAN_POINT('Ctrl Pts',(25.7090702266962,-66.7260200131266,0.));
#64758=CARTESIAN_POINT('Ctrl Pts',(25.7239055663772,-66.7437090121153,0.));
#64759=CARTESIAN_POINT('Ctrl Pts',(25.7387871171866,-66.7614172770316,0.));
#64760=CARTESIAN_POINT('Ctrl Pts',(25.7537148453863,-66.7791446652545,0.));
#64761=CARTESIAN_POINT('Ctrl Pts',(25.7686887172877,-66.7968910348245,0.));
#64762=CARTESIAN_POINT('Ctrl Pts',(25.7837086992594,-66.8146562444433,0.));
#64763=CARTESIAN_POINT('Ctrl Pts',(25.7987747577269,-66.8324401534668,0.));
#64764=CARTESIAN_POINT('Ctrl Pts',(25.8138868591709,-66.8502426219001,0.));
#64765=CARTESIAN_POINT('Ctrl Pts',(25.8290449701192,-66.8680635103876,0.));
#64766=CARTESIAN_POINT('Ctrl Pts',(25.844249057147,-66.8859026802088,0.));
#64767=CARTESIAN_POINT('Ctrl Pts',(25.8594990868833,-66.9037599932761,0.));
#64768=CARTESIAN_POINT('Ctrl Pts',(25.874795026011,-66.92163531213,0.));
#64769=CARTESIAN_POINT('Ctrl Pts',(25.890136841266,-66.939528499934,0.));
#64770=CARTESIAN_POINT('Ctrl Pts',(25.9055244994277,-66.9574394204663,0.));
#64771=CARTESIAN_POINT('Ctrl Pts',(25.9209579673209,-66.975367938115,0.));
#64772=CARTESIAN_POINT('Ctrl Pts',(25.9364372118222,-66.9933139178778,0.));
#64773=CARTESIAN_POINT('Ctrl Pts',(25.9519621998598,-67.0112772253556,0.));
#64774=CARTESIAN_POINT('Ctrl Pts',(25.967532898412,-67.0292577267489,0.));
#64775=CARTESIAN_POINT('Ctrl Pts',(25.9831492744983,-67.0472552888485,0.));
#64776=CARTESIAN_POINT('Ctrl Pts',(25.9988112951814,-67.0652697790325,0.));
#64777=CARTESIAN_POINT('Ctrl Pts',(26.014518927573,-67.0833010652634,0.));
#64778=CARTESIAN_POINT('Ctrl Pts',(26.0302721388339,-67.101349016084,0.));
#64779=CARTESIAN_POINT('Ctrl Pts',(26.0460708961725,-67.1194135006124,0.));
#64780=CARTESIAN_POINT('Ctrl Pts',(26.061915166836,-67.1374943885354,0.));
#64781=CARTESIAN_POINT('Ctrl Pts',(26.0778049181128,-67.1555915501049,0.));
#64782=CARTESIAN_POINT('Ctrl Pts',(26.0937401173383,-67.173704856136,0.));
#64783=CARTESIAN_POINT('Ctrl Pts',(26.1097207318949,-67.1918341780018,0.));
#64784=CARTESIAN_POINT('Ctrl Pts',(26.1257467292102,-67.2099793876297,0.));
#64785=CARTESIAN_POINT('Ctrl Pts',(26.1418180767489,-67.2281403574938,0.));
#64786=CARTESIAN_POINT('Ctrl Pts',(26.1579347420138,-67.2463169606115,0.));
#64787=CARTESIAN_POINT('Ctrl Pts',(26.1740966925528,-67.2645090705421,0.));
#64788=CARTESIAN_POINT('Ctrl Pts',(26.1903038959589,-67.282716561383,0.));
#64789=CARTESIAN_POINT('Ctrl Pts',(26.2065563198683,-67.3009393077652,0.));
#64790=CARTESIAN_POINT('Ctrl Pts',(26.2228539319526,-67.3191771848464,0.));
#64791=CARTESIAN_POINT('Ctrl Pts',(26.2391966999191,-67.3374300683074,0.));
#64792=CARTESIAN_POINT('Ctrl Pts',(26.255584591518,-67.3556978343507,0.));
#64793=CARTESIAN_POINT('Ctrl Pts',(26.2720175745423,-67.3739803596969,0.));
#64794=CARTESIAN_POINT('Ctrl Pts',(26.2884956168269,-67.392277521581,0.));
#64795=CARTESIAN_POINT('Ctrl Pts',(26.3050186862407,-67.4105891977461,0.));
#64796=CARTESIAN_POINT('Ctrl Pts',(26.321586750686,-67.4289152664398,0.));
#64797=CARTESIAN_POINT('Ctrl Pts',(26.3381997781055,-67.4472556064119,0.));
#64798=CARTESIAN_POINT('Ctrl Pts',(26.3548577364833,-67.4656100969116,0.));
#64799=CARTESIAN_POINT('Ctrl Pts',(26.3715605938432,-67.4839786176836,0.));
#64800=CARTESIAN_POINT('Ctrl Pts',(26.3883083182421,-67.5023610489622,0.));
#64801=CARTESIAN_POINT('Ctrl Pts',(26.4051008777675,-67.5207572714683,0.));
#64802=CARTESIAN_POINT('Ctrl Pts',(26.4219382405458,-67.5391671664072,0.));
#64803=CARTESIAN_POINT('Ctrl Pts',(26.4388203747425,-67.5575906154657,0.));
#64804=CARTESIAN_POINT('Ctrl Pts',(26.455747248562,-67.5760275008093,0.));
#64805=CARTESIAN_POINT('Ctrl Pts',(26.4727188302409,-67.5944777050768,0.));
#64806=CARTESIAN_POINT('Ctrl Pts',(26.4897350880439,-67.6129411113758,0.));
#64807=CARTESIAN_POINT('Ctrl Pts',(26.5067959902725,-67.6314176032811,0.));
#64808=CARTESIAN_POINT('Ctrl Pts',(26.5239015052653,-67.649907064832,0.));
#64809=CARTESIAN_POINT('Ctrl Pts',(26.5410516013984,-67.6684093805291,0.));
#64810=CARTESIAN_POINT('Ctrl Pts',(26.5582462470794,-67.6869244353294,0.));
#64811=CARTESIAN_POINT('Ctrl Pts',(26.5754854107421,-67.7054521146425,0.));
#64812=CARTESIAN_POINT('Ctrl Pts',(26.5927690608543,-67.7239923043288,0.));
#64813=CARTESIAN_POINT('Ctrl Pts',(26.6100971659201,-67.7425448906977,0.));
#64814=CARTESIAN_POINT('Ctrl Pts',(26.6274696944792,-67.7611097605042,0.));
#64815=CARTESIAN_POINT('Ctrl Pts',(26.6448866151029,-67.7796868009455,0.));
#64816=CARTESIAN_POINT('Ctrl Pts',(26.662347896387,-67.798275899657,0.));
#64817=CARTESIAN_POINT('Ctrl Pts',(26.6798535069589,-67.8168769447098,0.));
#64818=CARTESIAN_POINT('Ctrl Pts',(26.6974034154804,-67.8354898246086,0.));
#64819=CARTESIAN_POINT('Ctrl Pts',(26.7149975906477,-67.8541144282875,0.));
#64820=CARTESIAN_POINT('Ctrl Pts',(26.7326360011884,-67.8727506451064,0.));
#64821=CARTESIAN_POINT('Ctrl Pts',(26.7503186158522,-67.8913983648437,0.));
#64822=CARTESIAN_POINT('Ctrl Pts',(26.7680454034168,-67.9100574776972,0.));
#64823=CARTESIAN_POINT('Ctrl Pts',(26.7858163326933,-67.928727874284,0.));
#64824=CARTESIAN_POINT('Ctrl Pts',(26.8036313725262,-67.9474094456396,0.));
#64825=CARTESIAN_POINT('Ctrl Pts',(26.821490491792,-67.9661020832164,0.));
#64826=CARTESIAN_POINT('Ctrl Pts',(26.8393936593911,-67.9848056788809,0.));
#64827=CARTESIAN_POINT('Ctrl Pts',(26.8573408442496,-68.0035201249102,0.));
#64828=CARTESIAN_POINT('Ctrl Pts',(26.8753320153251,-68.0222453139856,0.));
#64829=CARTESIAN_POINT('Ctrl Pts',(26.8933671416062,-68.0409811391869,0.));
#64830=CARTESIAN_POINT('Ctrl Pts',(26.9114461921109,-68.0597274939859,0.));
#64831=CARTESIAN_POINT('Ctrl Pts',(26.9295691358778,-68.0784842722369,0.));
#64832=CARTESIAN_POINT('Ctrl Pts',(26.9477359419651,-68.0972513681751,0.));
#64833=CARTESIAN_POINT('Ctrl Pts',(26.9659465794601,-68.1160286764255,0.));
#64834=CARTESIAN_POINT('Ctrl Pts',(26.9842010174821,-68.1348160920107,0.));
#64835=CARTESIAN_POINT('Ctrl Pts',(27.0024992251838,-68.1536135103557,0.));
#64836=CARTESIAN_POINT('Ctrl Pts',(27.0208411717472,-68.1724208272958,0.));
#64837=CARTESIAN_POINT('Ctrl Pts',(27.0392268263797,-68.1912379390773,0.));
#64838=CARTESIAN_POINT('Ctrl Pts',(27.0576561583172,-68.2100647423332,0.));
#64839=CARTESIAN_POINT('Ctrl Pts',(27.0761291368225,-68.2289011340615,0.));
#64840=CARTESIAN_POINT('Ctrl Pts',(27.0946457311812,-68.2477470116013,0.));
#64841=CARTESIAN_POINT('Ctrl Pts',(27.1132059106943,-68.2666022726104,0.));
#64842=CARTESIAN_POINT('Ctrl Pts',(27.1318096446648,-68.2854668150364,0.));
#64843=CARTESIAN_POINT('Ctrl Pts',(27.1504569024136,-68.3043405371603,0.));
#64844=CARTESIAN_POINT('Ctrl Pts',(27.1691476532921,-68.3232233376425,0.));
#64845=CARTESIAN_POINT('Ctrl Pts',(27.1878818666926,-68.3421151155711,0.));
#64846=CARTESIAN_POINT('Ctrl Pts',(27.2066595120541,-68.3610157704994,0.));
#64847=CARTESIAN_POINT('Ctrl Pts',(27.2254805588673,-68.3799252025102,0.));
#64848=CARTESIAN_POINT('Ctrl Pts',(27.244344976665,-68.3988433121581,0.));
#64849=CARTESIAN_POINT('Ctrl Pts',(27.2632527350059,-68.4177700003465,0.));
#64850=CARTESIAN_POINT('Ctrl Pts',(27.2822038034538,-68.4367051682164,0.));
#64851=CARTESIAN_POINT('Ctrl Pts',(27.301198151557,-68.4556487170441,0.));
#64852=CARTESIAN_POINT('Ctrl Pts',(27.3202357488154,-68.4746005480997,0.));
#64853=CARTESIAN_POINT('Ctrl Pts',(27.3393165646751,-68.4935605626372,0.));
#64854=CARTESIAN_POINT('Ctrl Pts',(27.3584405685947,-68.5125286621902,0.));
#64855=CARTESIAN_POINT('Ctrl Pts',(27.3776077300918,-68.5315047488046,0.));
#64856=CARTESIAN_POINT('Ctrl Pts',(27.3968180187941,-68.5504887252976,0.));
#64857=CARTESIAN_POINT('Ctrl Pts',(27.4160714044825,-68.5694804955002,0.));
#64858=CARTESIAN_POINT('Ctrl Pts',(27.4353678571349,-68.5884799645193,0.));
#64859=CARTESIAN_POINT('Ctrl Pts',(27.4547073468212,-68.6074870381588,0.));
#64860=CARTESIAN_POINT('Ctrl Pts',(27.4740898435976,-68.6265016223536,0.));
#64861=CARTESIAN_POINT('Ctrl Pts',(27.4935153173863,-68.6455236225471,0.));
#64862=CARTESIAN_POINT('Ctrl Pts',(27.5129837378797,-68.664552943206,0.));
#64863=CARTESIAN_POINT('Ctrl Pts',(27.5324950743722,-68.683589486992,0.));
#64864=CARTESIAN_POINT('Ctrl Pts',(27.552049295893,-68.7026331554349,0.));
#64865=CARTESIAN_POINT('Ctrl Pts',(27.5716463715027,-68.721683850427,0.));
#64866=CARTESIAN_POINT('Ctrl Pts',(27.5912862705482,-68.7407414755291,0.));
#64867=CARTESIAN_POINT('Ctrl Pts',(27.6109689629025,-68.7598059372121,0.));
#64868=CARTESIAN_POINT('Ctrl Pts',(27.6306944192711,-68.7788771464655,0.));
#64869=CARTESIAN_POINT('Ctrl Pts',(27.6504626112621,-68.7979550191773,0.));
#64870=CARTESIAN_POINT('Ctrl Pts',(27.667444390988,-68.8143140938752,0.));
#64871=CARTESIAN_POINT('Ctrl Pts',(27.6804870323283,-68.8268597851978,0.));
#64872=CARTESIAN_POINT('Ctrl Pts',(27.689571627108,-68.8355891981874,0.));
#64873=CARTESIAN_POINT('Ctrl Pts',(27.6946856803477,-68.8405004465891,0.));
#64874=CARTESIAN_POINT('Ctrl Pts',(27.6958230984751,-68.8415926174769,0.));
#64875=CARTESIAN_POINT('',(24.7419628022041,-65.4815644032299,12.));
#64876=CARTESIAN_POINT('',(24.7419628022041,-65.4815644032299,0.));
#64877=CARTESIAN_POINT('Ctrl Pts',(27.6958230984751,-68.8415926174769,12.));
#64878=CARTESIAN_POINT('Ctrl Pts',(27.6946856803477,-68.8405004465891,12.));
#64879=CARTESIAN_POINT('Ctrl Pts',(27.689571627108,-68.8355891981874,12.));
#64880=CARTESIAN_POINT('Ctrl Pts',(27.6804870323283,-68.8268597851978,12.));
#64881=CARTESIAN_POINT('Ctrl Pts',(27.667444390988,-68.8143140938752,12.));
#64882=CARTESIAN_POINT('Ctrl Pts',(27.6504626112621,-68.7979550191773,12.));
#64883=CARTESIAN_POINT('Ctrl Pts',(27.6306944192711,-68.7788771464655,12.));
#64884=CARTESIAN_POINT('Ctrl Pts',(27.6109689629025,-68.7598059372121,12.));
#64885=CARTESIAN_POINT('Ctrl Pts',(27.5912862705482,-68.7407414755291,12.));
#64886=CARTESIAN_POINT('Ctrl Pts',(27.5716463715027,-68.721683850427,12.));
#64887=CARTESIAN_POINT('Ctrl Pts',(27.552049295893,-68.7026331554349,12.));
#64888=CARTESIAN_POINT('Ctrl Pts',(27.5324950743722,-68.683589486992,12.));
#64889=CARTESIAN_POINT('Ctrl Pts',(27.5129837378797,-68.664552943206,12.));
#64890=CARTESIAN_POINT('Ctrl Pts',(27.4935153173863,-68.6455236225471,12.));
#64891=CARTESIAN_POINT('Ctrl Pts',(27.4740898435976,-68.6265016223536,12.));
#64892=CARTESIAN_POINT('Ctrl Pts',(27.4547073468212,-68.6074870381588,12.));
#64893=CARTESIAN_POINT('Ctrl Pts',(27.4353678571349,-68.5884799645193,12.));
#64894=CARTESIAN_POINT('Ctrl Pts',(27.4160714044825,-68.5694804955002,12.));
#64895=CARTESIAN_POINT('Ctrl Pts',(27.3968180187941,-68.5504887252976,12.));
#64896=CARTESIAN_POINT('Ctrl Pts',(27.3776077300918,-68.5315047488046,12.));
#64897=CARTESIAN_POINT('Ctrl Pts',(27.3584405685947,-68.5125286621902,12.));
#64898=CARTESIAN_POINT('Ctrl Pts',(27.3393165646751,-68.4935605626372,12.));
#64899=CARTESIAN_POINT('Ctrl Pts',(27.3202357488154,-68.4746005480997,12.));
#64900=CARTESIAN_POINT('Ctrl Pts',(27.301198151557,-68.4556487170441,12.));
#64901=CARTESIAN_POINT('Ctrl Pts',(27.2822038034538,-68.4367051682164,12.));
#64902=CARTESIAN_POINT('Ctrl Pts',(27.2632527350059,-68.4177700003465,12.));
#64903=CARTESIAN_POINT('Ctrl Pts',(27.244344976665,-68.3988433121581,12.));
#64904=CARTESIAN_POINT('Ctrl Pts',(27.2254805588673,-68.3799252025102,12.));
#64905=CARTESIAN_POINT('Ctrl Pts',(27.2066595120541,-68.3610157704994,12.));
#64906=CARTESIAN_POINT('Ctrl Pts',(27.1878818666926,-68.3421151155711,12.));
#64907=CARTESIAN_POINT('Ctrl Pts',(27.1691476532921,-68.3232233376425,12.));
#64908=CARTESIAN_POINT('Ctrl Pts',(27.1504569024136,-68.3043405371603,12.));
#64909=CARTESIAN_POINT('Ctrl Pts',(27.1318096446648,-68.2854668150364,12.));
#64910=CARTESIAN_POINT('Ctrl Pts',(27.1132059106943,-68.2666022726104,12.));
#64911=CARTESIAN_POINT('Ctrl Pts',(27.0946457311812,-68.2477470116013,12.));
#64912=CARTESIAN_POINT('Ctrl Pts',(27.0761291368225,-68.2289011340615,12.));
#64913=CARTESIAN_POINT('Ctrl Pts',(27.0576561583172,-68.2100647423332,12.));
#64914=CARTESIAN_POINT('Ctrl Pts',(27.0392268263797,-68.1912379390773,12.));
#64915=CARTESIAN_POINT('Ctrl Pts',(27.0208411717472,-68.1724208272958,12.));
#64916=CARTESIAN_POINT('Ctrl Pts',(27.0024992251838,-68.1536135103557,12.));
#64917=CARTESIAN_POINT('Ctrl Pts',(26.9842010174821,-68.1348160920107,12.));
#64918=CARTESIAN_POINT('Ctrl Pts',(26.9659465794601,-68.1160286764255,12.));
#64919=CARTESIAN_POINT('Ctrl Pts',(26.9477359419651,-68.0972513681751,12.));
#64920=CARTESIAN_POINT('Ctrl Pts',(26.9295691358778,-68.0784842722369,12.));
#64921=CARTESIAN_POINT('Ctrl Pts',(26.9114461921109,-68.0597274939859,12.));
#64922=CARTESIAN_POINT('Ctrl Pts',(26.8933671416062,-68.0409811391869,12.));
#64923=CARTESIAN_POINT('Ctrl Pts',(26.8753320153251,-68.0222453139856,12.));
#64924=CARTESIAN_POINT('Ctrl Pts',(26.8573408442496,-68.0035201249102,12.));
#64925=CARTESIAN_POINT('Ctrl Pts',(26.8393936593911,-67.9848056788809,12.));
#64926=CARTESIAN_POINT('Ctrl Pts',(26.821490491792,-67.9661020832164,12.));
#64927=CARTESIAN_POINT('Ctrl Pts',(26.8036313725262,-67.9474094456396,12.));
#64928=CARTESIAN_POINT('Ctrl Pts',(26.7858163326933,-67.928727874284,12.));
#64929=CARTESIAN_POINT('Ctrl Pts',(26.7680454034168,-67.9100574776972,12.));
#64930=CARTESIAN_POINT('Ctrl Pts',(26.7503186158522,-67.8913983648437,12.));
#64931=CARTESIAN_POINT('Ctrl Pts',(26.7326360011884,-67.8727506451064,12.));
#64932=CARTESIAN_POINT('Ctrl Pts',(26.7149975906477,-67.8541144282875,12.));
#64933=CARTESIAN_POINT('Ctrl Pts',(26.6974034154804,-67.8354898246086,12.));
#64934=CARTESIAN_POINT('Ctrl Pts',(26.6798535069589,-67.8168769447098,12.));
#64935=CARTESIAN_POINT('Ctrl Pts',(26.662347896387,-67.798275899657,12.));
#64936=CARTESIAN_POINT('Ctrl Pts',(26.6448866151029,-67.7796868009455,12.));
#64937=CARTESIAN_POINT('Ctrl Pts',(26.6274696944792,-67.7611097605042,12.));
#64938=CARTESIAN_POINT('Ctrl Pts',(26.6100971659201,-67.7425448906977,12.));
#64939=CARTESIAN_POINT('Ctrl Pts',(26.5927690608543,-67.7239923043288,12.));
#64940=CARTESIAN_POINT('Ctrl Pts',(26.5754854107421,-67.7054521146425,12.));
#64941=CARTESIAN_POINT('Ctrl Pts',(26.5582462470794,-67.6869244353294,12.));
#64942=CARTESIAN_POINT('Ctrl Pts',(26.5410516013984,-67.6684093805291,12.));
#64943=CARTESIAN_POINT('Ctrl Pts',(26.5239015052653,-67.649907064832,12.));
#64944=CARTESIAN_POINT('Ctrl Pts',(26.5067959902725,-67.6314176032811,12.));
#64945=CARTESIAN_POINT('Ctrl Pts',(26.4897350880439,-67.6129411113758,12.));
#64946=CARTESIAN_POINT('Ctrl Pts',(26.4727188302409,-67.5944777050768,12.));
#64947=CARTESIAN_POINT('Ctrl Pts',(26.455747248562,-67.5760275008093,12.));
#64948=CARTESIAN_POINT('Ctrl Pts',(26.4388203747425,-67.5575906154657,12.));
#64949=CARTESIAN_POINT('Ctrl Pts',(26.4219382405458,-67.5391671664072,12.));
#64950=CARTESIAN_POINT('Ctrl Pts',(26.4051008777675,-67.5207572714683,12.));
#64951=CARTESIAN_POINT('Ctrl Pts',(26.3883083182421,-67.5023610489622,12.));
#64952=CARTESIAN_POINT('Ctrl Pts',(26.3715605938432,-67.4839786176836,12.));
#64953=CARTESIAN_POINT('Ctrl Pts',(26.3548577364833,-67.4656100969116,12.));
#64954=CARTESIAN_POINT('Ctrl Pts',(26.3381997781055,-67.4472556064119,12.));
#64955=CARTESIAN_POINT('Ctrl Pts',(26.321586750686,-67.4289152664398,12.));
#64956=CARTESIAN_POINT('Ctrl Pts',(26.3050186862407,-67.4105891977461,12.));
#64957=CARTESIAN_POINT('Ctrl Pts',(26.2884956168269,-67.392277521581,12.));
#64958=CARTESIAN_POINT('Ctrl Pts',(26.2720175745423,-67.3739803596969,12.));
#64959=CARTESIAN_POINT('Ctrl Pts',(26.255584591518,-67.3556978343507,12.));
#64960=CARTESIAN_POINT('Ctrl Pts',(26.2391966999191,-67.3374300683074,12.));
#64961=CARTESIAN_POINT('Ctrl Pts',(26.2228539319526,-67.3191771848464,12.));
#64962=CARTESIAN_POINT('Ctrl Pts',(26.2065563198683,-67.3009393077652,12.));
#64963=CARTESIAN_POINT('Ctrl Pts',(26.1903038959589,-67.282716561383,12.));
#64964=CARTESIAN_POINT('Ctrl Pts',(26.1740966925528,-67.2645090705421,12.));
#64965=CARTESIAN_POINT('Ctrl Pts',(26.1579347420138,-67.2463169606115,12.));
#64966=CARTESIAN_POINT('Ctrl Pts',(26.1418180767489,-67.2281403574938,12.));
#64967=CARTESIAN_POINT('Ctrl Pts',(26.1257467292102,-67.2099793876297,12.));
#64968=CARTESIAN_POINT('Ctrl Pts',(26.1097207318949,-67.1918341780018,12.));
#64969=CARTESIAN_POINT('Ctrl Pts',(26.0937401173383,-67.173704856136,12.));
#64970=CARTESIAN_POINT('Ctrl Pts',(26.0778049181128,-67.1555915501049,12.));
#64971=CARTESIAN_POINT('Ctrl Pts',(26.061915166836,-67.1374943885354,12.));
#64972=CARTESIAN_POINT('Ctrl Pts',(26.0460708961725,-67.1194135006124,12.));
#64973=CARTESIAN_POINT('Ctrl Pts',(26.0302721388339,-67.101349016084,12.));
#64974=CARTESIAN_POINT('Ctrl Pts',(26.014518927573,-67.0833010652634,12.));
#64975=CARTESIAN_POINT('Ctrl Pts',(25.9988112951814,-67.0652697790325,12.));
#64976=CARTESIAN_POINT('Ctrl Pts',(25.9831492744983,-67.0472552888485,12.));
#64977=CARTESIAN_POINT('Ctrl Pts',(25.967532898412,-67.0292577267489,12.));
#64978=CARTESIAN_POINT('Ctrl Pts',(25.9519621998598,-67.0112772253556,12.));
#64979=CARTESIAN_POINT('Ctrl Pts',(25.9364372118222,-66.9933139178778,12.));
#64980=CARTESIAN_POINT('Ctrl Pts',(25.9209579673209,-66.975367938115,12.));
#64981=CARTESIAN_POINT('Ctrl Pts',(25.9055244994277,-66.9574394204663,12.));
#64982=CARTESIAN_POINT('Ctrl Pts',(25.890136841266,-66.939528499934,12.));
#64983=CARTESIAN_POINT('Ctrl Pts',(25.874795026011,-66.92163531213,12.));
#64984=CARTESIAN_POINT('Ctrl Pts',(25.8594990868833,-66.9037599932761,12.));
#64985=CARTESIAN_POINT('Ctrl Pts',(25.844249057147,-66.8859026802088,12.));
#64986=CARTESIAN_POINT('Ctrl Pts',(25.8290449701192,-66.8680635103876,12.));
#64987=CARTESIAN_POINT('Ctrl Pts',(25.8138868591709,-66.8502426219001,12.));
#64988=CARTESIAN_POINT('Ctrl Pts',(25.7987747577269,-66.8324401534668,12.));
#64989=CARTESIAN_POINT('Ctrl Pts',(25.7837086992594,-66.8146562444433,12.));
#64990=CARTESIAN_POINT('Ctrl Pts',(25.7686887172877,-66.7968910348245,12.));
#64991=CARTESIAN_POINT('Ctrl Pts',(25.7537148453863,-66.7791446652545,12.));
#64992=CARTESIAN_POINT('Ctrl Pts',(25.7387871171866,-66.7614172770316,12.));
#64993=CARTESIAN_POINT('Ctrl Pts',(25.7239055663772,-66.7437090121153,12.));
#64994=CARTESIAN_POINT('Ctrl Pts',(25.7090702266962,-66.7260200131266,12.));
#64995=CARTESIAN_POINT('Ctrl Pts',(25.6942811319322,-66.7083504233529,12.));
#64996=CARTESIAN_POINT('Ctrl Pts',(25.6795383159319,-66.6907003867572,12.));
#64997=CARTESIAN_POINT('Ctrl Pts',(25.6648418126013,-66.6730700479837,12.));
#64998=CARTESIAN_POINT('Ctrl Pts',(25.6501916559055,-66.6554595523624,12.));
#64999=CARTESIAN_POINT('Ctrl Pts',(25.6355878798613,-66.6378690459129,12.));
#65000=CARTESIAN_POINT('Ctrl Pts',(25.6210305185403,-66.6202986753507,12.));
#65001=CARTESIAN_POINT('Ctrl Pts',(25.6065196060755,-66.6027485880963,12.));
#65002=CARTESIAN_POINT('Ctrl Pts',(25.5920551766629,-66.5852189322813,12.));
#65003=CARTESIAN_POINT('Ctrl Pts',(25.5776372645601,-66.5677098567542,12.));
#65004=CARTESIAN_POINT('Ctrl Pts',(25.5632659040792,-66.5502215110829,12.));
#65005=CARTESIAN_POINT('Ctrl Pts',(25.5489411295911,-66.5327540455624,12.));
#65006=CARTESIAN_POINT('Ctrl Pts',(25.534662975532,-66.5153076112231,12.));
#65007=CARTESIAN_POINT('Ctrl Pts',(25.5204314764033,-66.4978823598354,12.));
#65008=CARTESIAN_POINT('Ctrl Pts',(25.5062466667702,-66.4804784439148,12.));
#65009=CARTESIAN_POINT('Ctrl Pts',(25.4921085812547,-66.4630960167252,12.));
#65010=CARTESIAN_POINT('Ctrl Pts',(25.4780172545417,-66.4457352322871,12.));
#65011=CARTESIAN_POINT('Ctrl Pts',(25.4639727213849,-66.4283962453899,12.));
#65012=CARTESIAN_POINT('Ctrl Pts',(25.4499750166078,-66.4110792116,12.));
#65013=CARTESIAN_POINT('Ctrl Pts',(25.4360241751017,-66.3937842872685,12.));
#65014=CARTESIAN_POINT('Ctrl Pts',(25.4221202318199,-66.3765116295365,12.));
#65015=CARTESIAN_POINT('Ctrl Pts',(25.4082632217847,-66.359261396341,12.));
#65016=CARTESIAN_POINT('Ctrl Pts',(25.3944531800901,-66.3420337464178,12.));
#65017=CARTESIAN_POINT('Ctrl Pts',(25.3806901419012,-66.3248288393046,12.));
#65018=CARTESIAN_POINT('Ctrl Pts',(25.3669741424488,-66.3076468353413,12.));
#65019=CARTESIAN_POINT('Ctrl Pts',(25.3533052170248,-66.290487895671,12.));
#65020=CARTESIAN_POINT('Ctrl Pts',(25.3396834009949,-66.2733521822662,12.));
#65021=CARTESIAN_POINT('Ctrl Pts',(25.3261087298026,-66.2562398579471,12.));
#65022=CARTESIAN_POINT('Ctrl Pts',(25.3125812389729,-66.2391510863998,12.));
#65023=CARTESIAN_POINT('Ctrl Pts',(25.2991009641094,-66.2220860321952,12.));
#65024=CARTESIAN_POINT('Ctrl Pts',(25.285667940893,-66.2050448607911,12.));
#65025=CARTESIAN_POINT('Ctrl Pts',(25.2722822050836,-66.1880277385136,12.));
#65026=CARTESIAN_POINT('Ctrl Pts',(25.2589437925146,-66.1710348325384,12.));
#65027=CARTESIAN_POINT('Ctrl Pts',(25.2456527390874,-66.1540663108754,12.));
#65028=CARTESIAN_POINT('Ctrl Pts',(25.2324090807549,-66.1371223423345,12.));
#65029=CARTESIAN_POINT('Ctrl Pts',(25.2192128535357,-66.1202030965759,12.));
#65030=CARTESIAN_POINT('Ctrl Pts',(25.2060640935365,-66.10330874419,12.));
#65031=CARTESIAN_POINT('Ctrl Pts',(25.1929628369684,-66.086439456768,12.));
#65032=CARTESIAN_POINT('Ctrl Pts',(25.1799091201599,-66.0695954069713,12.));
#65033=CARTESIAN_POINT('Ctrl Pts',(25.166902979566,-66.0527767686025,12.));
#65034=CARTESIAN_POINT('Ctrl Pts',(25.1539444517418,-66.0359837164734,12.));
#65035=CARTESIAN_POINT('Ctrl Pts',(25.1410335733098,-66.0192164262621,12.));
#65036=CARTESIAN_POINT('Ctrl Pts',(25.1281703809297,-66.0024750743897,12.));
#65037=CARTESIAN_POINT('Ctrl Pts',(25.1153549112503,-65.9857598378433,12.));
#65038=CARTESIAN_POINT('Ctrl Pts',(25.1025872009003,-65.9690708941558,12.));
#65039=CARTESIAN_POINT('Ctrl Pts',(25.0898672865915,-65.952408421814,12.));
#65040=CARTESIAN_POINT('Ctrl Pts',(25.0771952052028,-65.9357726006163,12.));
#65041=CARTESIAN_POINT('Ctrl Pts',(25.0645709938524,-65.919163611981,12.));
#65042=CARTESIAN_POINT('Ctrl Pts',(25.0519946900078,-65.9025816394424,12.));
#65043=CARTESIAN_POINT('Ctrl Pts',(25.0394663314055,-65.8860268683128,12.));
#65044=CARTESIAN_POINT('Ctrl Pts',(25.0269859558362,-65.8694994847617,12.));
#65045=CARTESIAN_POINT('Ctrl Pts',(25.0145536009604,-65.8529996750445,12.));
#65046=CARTESIAN_POINT('Ctrl Pts',(25.0021693041169,-65.8365276247128,12.));
#65047=CARTESIAN_POINT('Ctrl Pts',(24.9898331020983,-65.8200835177024,12.));
#65048=CARTESIAN_POINT('Ctrl Pts',(24.9775450315682,-65.8036675380718,12.));
#65049=CARTESIAN_POINT('Ctrl Pts',(24.965305129558,-65.7872798720823,12.));
#65050=CARTESIAN_POINT('Ctrl Pts',(24.9531134338696,-65.7709207098959,12.));
#65051=CARTESIAN_POINT('Ctrl Pts',(24.9409699836537,-65.7545902480323,12.));
#65052=CARTESIAN_POINT('Ctrl Pts',(24.928874819458,-65.7382886895888,12.));
#65053=CARTESIAN_POINT('Ctrl Pts',(24.9168279820106,-65.7220162391054,12.));
#65054=CARTESIAN_POINT('Ctrl Pts',(24.9048295111448,-65.7057730980483,12.));
#65055=CARTESIAN_POINT('Ctrl Pts',(24.8928794448607,-65.6895594608776,12.));
#65056=CARTESIAN_POINT('Ctrl Pts',(24.8809778178228,-65.6733755087669,12.));
#65057=CARTESIAN_POINT('Ctrl Pts',(24.8691246628056,-65.6572214156692,12.));
#65058=CARTESIAN_POINT('Ctrl Pts',(24.8573200135665,-65.6410973603661,12.));
#65059=CARTESIAN_POINT('Ctrl Pts',(24.8455639071516,-65.6250035361612,12.));
#65060=CARTESIAN_POINT('Ctrl Pts',(24.8338563866763,-65.6089401625628,12.));
#65061=CARTESIAN_POINT('Ctrl Pts',(24.8221975032103,-65.5929074932624,12.));
#65062=CARTESIAN_POINT('Ctrl Pts',(24.8105873098626,-65.5769057914333,12.));
#65063=CARTESIAN_POINT('Ctrl Pts',(24.7990258561259,-65.5609353062829,12.));
#65064=CARTESIAN_POINT('Ctrl Pts',(24.787513182749,-65.5449962514662,12.));
#65065=CARTESIAN_POINT('Ctrl Pts',(24.7760493148465,-65.5290887770232,12.));
#65066=CARTESIAN_POINT('Ctrl Pts',(24.7646342620841,-65.5132129675333,12.));
#65067=CARTESIAN_POINT('Ctrl Pts',(24.7555412724651,-65.5005376841101,12.));
#65068=CARTESIAN_POINT('Ctrl Pts',(24.7487434955981,-65.4910454936254,12.));
#65069=CARTESIAN_POINT('Ctrl Pts',(24.7442214063382,-65.4847237095443,12.));
#65070=CARTESIAN_POINT('Ctrl Pts',(24.7419628022041,-65.4815644032299,12.));
#65071=CARTESIAN_POINT('Ctrl Pts',(29.0944526440265,-68.2622612910179,-1.11022302462516E-15));
#65072=CARTESIAN_POINT('Ctrl Pts',(29.0944526440265,-68.2622612910179,4.));
#65073=CARTESIAN_POINT('Ctrl Pts',(29.0944526440265,-68.2622612910179,8.));
#65074=CARTESIAN_POINT('Ctrl Pts',(29.0944526440265,-68.2622612910179,12.));
#65075=CARTESIAN_POINT('Ctrl Pts',(29.0922231502662,-68.3721211369509,-1.11022302462516E-15));
#65076=CARTESIAN_POINT('Ctrl Pts',(29.0922231502662,-68.3721211369509,4.));
#65077=CARTESIAN_POINT('Ctrl Pts',(29.0922231502662,-68.3721211369509,8.));
#65078=CARTESIAN_POINT('Ctrl Pts',(29.0922231502662,-68.3721211369509,12.));
#65079=CARTESIAN_POINT('Ctrl Pts',(29.0225207419379,-68.5624216146674,-1.11022302462516E-15));
#65080=CARTESIAN_POINT('Ctrl Pts',(29.0225207419379,-68.5624216146674,4.00000000000001));
#65081=CARTESIAN_POINT('Ctrl Pts',(29.0225207419379,-68.5624216146674,7.99999999999999));
#65082=CARTESIAN_POINT('Ctrl Pts',(29.0225207419379,-68.5624216146674,12.));
#65083=CARTESIAN_POINT('Ctrl Pts',(28.8637726134454,-68.6814343344129,-1.11022302462516E-15));
#65084=CARTESIAN_POINT('Ctrl Pts',(28.8637726134454,-68.6814343344129,4.));
#65085=CARTESIAN_POINT('Ctrl Pts',(28.8637726134454,-68.6814343344129,8.00000000000001));
#65086=CARTESIAN_POINT('Ctrl Pts',(28.8637726134454,-68.6814343344129,12.));
#65087=CARTESIAN_POINT('Ctrl Pts',(28.7877620302417,-68.7132793373315,-1.11022302462516E-15));
#65088=CARTESIAN_POINT('Ctrl Pts',(28.7877620302417,-68.7132793373315,4.));
#65089=CARTESIAN_POINT('Ctrl Pts',(28.7877620302417,-68.7132793373315,8.));
#65090=CARTESIAN_POINT('Ctrl Pts',(28.7877620302417,-68.7132793373315,12.));
#65091=CARTESIAN_POINT('',(29.0944526440265,-68.2622612910179,0.));
#65092=CARTESIAN_POINT('',(28.7877620302418,-68.7132793373317,0.));
#65093=CARTESIAN_POINT('Ctrl Pts',(29.0944526440265,-68.2622612910179,0.));
#65094=CARTESIAN_POINT('Ctrl Pts',(29.0922231502662,-68.3721211369509,-7.70371977754894E-31));
#65095=CARTESIAN_POINT('Ctrl Pts',(29.05239320265,-68.4808642670746,6.16297582203915E-31));
#65096=CARTESIAN_POINT('Ctrl Pts',(28.9834871015109,-68.5663297619425,3.08148791101958E-31));
#65097=CARTESIAN_POINT('Ctrl Pts',(28.9318075256565,-68.6304288830934,-6.16297582203912E-32));
#65098=CARTESIAN_POINT('Ctrl Pts',(28.8637726134454,-68.6814343344129,-1.4482993181792E-30));
#65099=CARTESIAN_POINT('Ctrl Pts',(28.7877620302417,-68.7132793373315,-6.16297582203914E-32));
#65100=CARTESIAN_POINT('',(28.7877620302418,-68.7132793373317,12.));
#65101=CARTESIAN_POINT('Ctrl Pts',(28.7877620302417,-68.7132793373315,-1.11022302462516E-15));
#65102=CARTESIAN_POINT('Ctrl Pts',(28.7877620302417,-68.7132793373315,4.));
#65103=CARTESIAN_POINT('Ctrl Pts',(28.7877620302417,-68.7132793373315,8.));
#65104=CARTESIAN_POINT('Ctrl Pts',(28.7877620302417,-68.7132793373315,12.));
#65105=CARTESIAN_POINT('',(29.0944526440265,-68.2622612910179,12.));
#65106=CARTESIAN_POINT('Ctrl Pts',(28.7877620302417,-68.7132793373315,12.));
#65107=CARTESIAN_POINT('Ctrl Pts',(28.8637726134454,-68.6814343344129,12.));
#65108=CARTESIAN_POINT('Ctrl Pts',(28.9318075256565,-68.6304288830934,12.));
#65109=CARTESIAN_POINT('Ctrl Pts',(28.9834871015109,-68.5663297619425,12.));
#65110=CARTESIAN_POINT('Ctrl Pts',(29.05239320265,-68.4808642670746,12.));
#65111=CARTESIAN_POINT('Ctrl Pts',(29.0922231502662,-68.3721211369509,12.));
#65112=CARTESIAN_POINT('Ctrl Pts',(29.0944526440265,-68.2622612910179,12.));
#65113=CARTESIAN_POINT('Ctrl Pts',(29.0944526440265,-68.2622612910179,12.));
#65114=CARTESIAN_POINT('Ctrl Pts',(29.0944526440265,-68.2622612910179,8.));
#65115=CARTESIAN_POINT('Ctrl Pts',(29.0944526440265,-68.2622612910179,4.));
#65116=CARTESIAN_POINT('Ctrl Pts',(29.0944526440265,-68.2622612910179,-1.11022302462516E-15));
#65117=CARTESIAN_POINT('Origin',(1.43538201480493E-10,-3.46272497684358E-10,
0.));
#65118=CARTESIAN_POINT('Origin',(1.43538201480493E-10,-3.46272497684358E-10,
12.));
#65119=CARTESIAN_POINT('Origin',(1.43538201480493E-10,-3.46272497684358E-10,
0.));
#65120=CARTESIAN_POINT('Ctrl Pts',(22.1153394458716,-71.1418425484881,0.));
#65121=CARTESIAN_POINT('Ctrl Pts',(22.1153394458716,-71.1418425484881,4.));
#65122=CARTESIAN_POINT('Ctrl Pts',(22.1153394458716,-71.1418425484881,8.));
#65123=CARTESIAN_POINT('Ctrl Pts',(22.1153394458716,-71.1418425484881,12.));
#65124=CARTESIAN_POINT('Ctrl Pts',(22.0104100349462,-71.1744611799059,0.));
#65125=CARTESIAN_POINT('Ctrl Pts',(22.0104100349462,-71.1744611799059,4.));
#65126=CARTESIAN_POINT('Ctrl Pts',(22.0104100349461,-71.1744611799059,8.));
#65127=CARTESIAN_POINT('Ctrl Pts',(22.0104100349461,-71.1744611799059,12.));
#65128=CARTESIAN_POINT('Ctrl Pts',(21.807833456103,-71.168501135194,-7.30818592425997E-17));
#65129=CARTESIAN_POINT('Ctrl Pts',(21.807833456103,-71.168501135194,4.00000000000001));
#65130=CARTESIAN_POINT('Ctrl Pts',(21.807833456103,-71.168501135194,7.99999999999999));
#65131=CARTESIAN_POINT('Ctrl Pts',(21.807833456103,-71.168501135194,12.));
#65132=CARTESIAN_POINT('Ctrl Pts',(21.6447353227843,-71.0555229320376,-2.46611180232746E-16));
#65133=CARTESIAN_POINT('Ctrl Pts',(21.6447353227843,-71.0555229320376,3.99999999999999));
#65134=CARTESIAN_POINT('Ctrl Pts',(21.6447353227843,-71.0555229320376,8.00000000000001));
#65135=CARTESIAN_POINT('Ctrl Pts',(21.6447353227843,-71.0555229320376,12.));
#65136=CARTESIAN_POINT('Ctrl Pts',(21.5904919934803,-70.9934796068775,-3.30265160470244E-16));
#65137=CARTESIAN_POINT('Ctrl Pts',(21.5904919934803,-70.9934796068775,4.));
#65138=CARTESIAN_POINT('Ctrl Pts',(21.5904919934803,-70.9934796068775,8.));
#65139=CARTESIAN_POINT('Ctrl Pts',(21.5904919934803,-70.9934796068775,12.));
#65140=CARTESIAN_POINT('',(22.1153394458716,-71.1418425484881,0.));
#65141=CARTESIAN_POINT('',(21.59049199348,-70.9934796068777,0.));
#65142=CARTESIAN_POINT('Ctrl Pts',(22.1153394458716,-71.1418425484881,2.74425517504379E-17));
#65143=CARTESIAN_POINT('Ctrl Pts',(22.0104100349462,-71.1744611799059,2.74425517504379E-17));
#65144=CARTESIAN_POINT('Ctrl Pts',(21.8946519898929,-71.1710554400705,-1.43185106739048E-17));
#65145=CARTESIAN_POINT('Ctrl Pts',(21.7917848658273,-71.1327049954369,-8.88787442811197E-17));
#65146=CARTESIAN_POINT('Ctrl Pts',(21.7146345227781,-71.1039421619618,-1.44798919486531E-16));
#65147=CARTESIAN_POINT('Ctrl Pts',(21.6447353227843,-71.0555229320376,-2.19168628482308E-16));
#65148=CARTESIAN_POINT('Ctrl Pts',(21.5904919934803,-70.9934796068775,-3.02822608719806E-16));
#65149=CARTESIAN_POINT('',(21.59049199348,-70.9934796068777,12.));
#65150=CARTESIAN_POINT('Ctrl Pts',(21.5904919934803,-70.9934796068775,-3.30265160470244E-16));
#65151=CARTESIAN_POINT('Ctrl Pts',(21.5904919934803,-70.9934796068775,4.));
#65152=CARTESIAN_POINT('Ctrl Pts',(21.5904919934803,-70.9934796068775,8.));
#65153=CARTESIAN_POINT('Ctrl Pts',(21.5904919934803,-70.9934796068775,12.));
#65154=CARTESIAN_POINT('',(22.1153394458716,-71.1418425484881,12.));
#65155=CARTESIAN_POINT('Ctrl Pts',(21.5904919934803,-70.9934796068775,12.));
#65156=CARTESIAN_POINT('Ctrl Pts',(21.6447353227843,-71.0555229320376,12.));
#65157=CARTESIAN_POINT('Ctrl Pts',(21.714634522778,-71.1039421619618,12.));
#65158=CARTESIAN_POINT('Ctrl Pts',(21.7917848658272,-71.132704995437,12.));
#65159=CARTESIAN_POINT('Ctrl Pts',(21.8946519898929,-71.1710554400705,12.));
#65160=CARTESIAN_POINT('Ctrl Pts',(22.0104100349461,-71.1744611799059,12.));
#65161=CARTESIAN_POINT('Ctrl Pts',(22.1153394458716,-71.1418425484881,12.));
#65162=CARTESIAN_POINT('Ctrl Pts',(22.1153394458716,-71.1418425484881,12.));
#65163=CARTESIAN_POINT('Ctrl Pts',(22.1153394458716,-71.1418425484881,8.));
#65164=CARTESIAN_POINT('Ctrl Pts',(22.1153394458716,-71.1418425484881,4.));
#65165=CARTESIAN_POINT('Ctrl Pts',(22.1153394458716,-71.1418425484881,0.));
#65166=CARTESIAN_POINT('Ctrl Pts',(18.9407177820968,-67.3887914263118,0.));
#65167=CARTESIAN_POINT('Ctrl Pts',(18.9407177820968,-67.3887914263118,12.));
#65168=CARTESIAN_POINT('Ctrl Pts',(18.9426924398719,-67.3921355608328,0.));
#65169=CARTESIAN_POINT('Ctrl Pts',(18.9426924398719,-67.3921355608328,12.));
#65170=CARTESIAN_POINT('Ctrl Pts',(18.9466463414299,-67.3988274146651,0.));
#65171=CARTESIAN_POINT('Ctrl Pts',(18.9466463414299,-67.3988274146651,12.));
#65172=CARTESIAN_POINT('Ctrl Pts',(18.9525909517915,-67.4088759497911,0.));
#65173=CARTESIAN_POINT('Ctrl Pts',(18.9525909517915,-67.4088759497911,12.));
#65174=CARTESIAN_POINT('Ctrl Pts',(18.9605446160985,-67.4222955061981,0.));
#65175=CARTESIAN_POINT('Ctrl Pts',(18.9605446160985,-67.4222955061981,12.));
#65176=CARTESIAN_POINT('Ctrl Pts',(18.970532563171,-67.4391057908418,0.));
#65177=CARTESIAN_POINT('Ctrl Pts',(18.970532563171,-67.4391057908418,12.));
#65178=CARTESIAN_POINT('Ctrl Pts',(18.9805663798448,-67.4559518744638,0.));
#65179=CARTESIAN_POINT('Ctrl Pts',(18.9805663798448,-67.4559518744638,12.));
#65180=CARTESIAN_POINT('Ctrl Pts',(18.9906460638625,-67.472833671964,0.));
#65181=CARTESIAN_POINT('Ctrl Pts',(18.9906460638625,-67.472833671964,12.));
#65182=CARTESIAN_POINT('Ctrl Pts',(19.0007716032819,-67.4897510316844,0.));
#65183=CARTESIAN_POINT('Ctrl Pts',(19.0007716032819,-67.4897510316844,12.));
#65184=CARTESIAN_POINT('Ctrl Pts',(19.0109429761306,-67.5067037372317,0.));
#65185=CARTESIAN_POINT('Ctrl Pts',(19.0109429761306,-67.5067037372317,12.));
#65186=CARTESIAN_POINT('Ctrl Pts',(19.021160154824,-67.5236915360331,0.));
#65187=CARTESIAN_POINT('Ctrl Pts',(19.021160154824,-67.5236915360331,12.));
#65188=CARTESIAN_POINT('Ctrl Pts',(19.0314231093923,-67.540714161288,0.));
#65189=CARTESIAN_POINT('Ctrl Pts',(19.0314231093923,-67.540714161288,12.));
#65190=CARTESIAN_POINT('Ctrl Pts',(19.0417318110708,-67.5577713558194,0.));
#65191=CARTESIAN_POINT('Ctrl Pts',(19.0417318110708,-67.5577713558194,12.));
#65192=CARTESIAN_POINT('Ctrl Pts',(19.0520862360395,-67.5748628971964,0.));
#65193=CARTESIAN_POINT('Ctrl Pts',(19.0520862360395,-67.5748628971964,12.));
#65194=CARTESIAN_POINT('Ctrl Pts',(19.062486364241,-67.5919885896222,0.));
#65195=CARTESIAN_POINT('Ctrl Pts',(19.062486364241,-67.5919885896222,12.));
#65196=CARTESIAN_POINT('Ctrl Pts',(19.072932177628,-67.6091482520534,0.));
#65197=CARTESIAN_POINT('Ctrl Pts',(19.072932177628,-67.6091482520534,12.));
#65198=CARTESIAN_POINT('Ctrl Pts',(19.0834236587118,-67.6263417083426,0.));
#65199=CARTESIAN_POINT('Ctrl Pts',(19.0834236587118,-67.6263417083426,12.));
#65200=CARTESIAN_POINT('Ctrl Pts',(19.0939607887501,-67.6435687749841,0.));
#65201=CARTESIAN_POINT('Ctrl Pts',(19.0939607887501,-67.6435687749841,12.));
#65202=CARTESIAN_POINT('Ctrl Pts',(19.1045435468358,-67.6608292549462,0.));
#65203=CARTESIAN_POINT('Ctrl Pts',(19.1045435468358,-67.6608292549462,12.));
#65204=CARTESIAN_POINT('Ctrl Pts',(19.115171910846,-67.6781229440573,0.));
#65205=CARTESIAN_POINT('Ctrl Pts',(19.115171910846,-67.6781229440573,12.));
#65206=CARTESIAN_POINT('Ctrl Pts',(19.1258458580345,-67.6954496350063,0.));
#65207=CARTESIAN_POINT('Ctrl Pts',(19.1258458580345,-67.6954496350063,12.));
#65208=CARTESIAN_POINT('Ctrl Pts',(19.136565365709,-67.7128091219348,0.));
#65209=CARTESIAN_POINT('Ctrl Pts',(19.136565365709,-67.7128091219348,12.));
#65210=CARTESIAN_POINT('Ctrl Pts',(19.1473304119955,-67.7302012056584,0.));
#65211=CARTESIAN_POINT('Ctrl Pts',(19.1473304119955,-67.7302012056584,12.));
#65212=CARTESIAN_POINT('Ctrl Pts',(19.1581409758097,-67.7476256934444,0.));
#65213=CARTESIAN_POINT('Ctrl Pts',(19.1581409758097,-67.7476256934444,12.));
#65214=CARTESIAN_POINT('Ctrl Pts',(19.1689970364949,-67.7650823965127,0.));
#65215=CARTESIAN_POINT('Ctrl Pts',(19.1689970364949,-67.7650823965127,12.));
#65216=CARTESIAN_POINT('Ctrl Pts',(19.1798985735687,-67.7825711283096,0.));
#65217=CARTESIAN_POINT('Ctrl Pts',(19.1798985735687,-67.7825711283096,12.));
#65218=CARTESIAN_POINT('Ctrl Pts',(19.1908455664097,-67.8000917023926,0.));
#65219=CARTESIAN_POINT('Ctrl Pts',(19.1908455664097,-67.8000917023926,12.));
#65220=CARTESIAN_POINT('Ctrl Pts',(19.201837993993,-67.8176439306621,0.));
#65221=CARTESIAN_POINT('Ctrl Pts',(19.201837993993,-67.8176439306621,12.));
#65222=CARTESIAN_POINT('Ctrl Pts',(19.2128758350345,-67.835227624289,0.));
#65223=CARTESIAN_POINT('Ctrl Pts',(19.2128758350345,-67.835227624289,12.));
#65224=CARTESIAN_POINT('Ctrl Pts',(19.2239590681133,-67.8528425945184,0.));
#65225=CARTESIAN_POINT('Ctrl Pts',(19.2239590681133,-67.8528425945184,12.));
#65226=CARTESIAN_POINT('Ctrl Pts',(19.2350876717874,-67.8704886534544,0.));
#65227=CARTESIAN_POINT('Ctrl Pts',(19.2350876717874,-67.8704886534544,12.));
#65228=CARTESIAN_POINT('Ctrl Pts',(19.2462616247279,-67.8881656149955,0.));
#65229=CARTESIAN_POINT('Ctrl Pts',(19.2462616247279,-67.8881656149955,12.));
#65230=CARTESIAN_POINT('Ctrl Pts',(19.2574809057696,-67.9058732951788,0.));
#65231=CARTESIAN_POINT('Ctrl Pts',(19.2574809057696,-67.9058732951788,12.));
#65232=CARTESIAN_POINT('Ctrl Pts',(19.2687454938442,-67.9236115116758,0.));
#65233=CARTESIAN_POINT('Ctrl Pts',(19.2687454938442,-67.9236115116758,12.));
#65234=CARTESIAN_POINT('Ctrl Pts',(19.280055367936,-67.9413800834793,0.));
#65235=CARTESIAN_POINT('Ctrl Pts',(19.280055367936,-67.9413800834793,12.));
#65236=CARTESIAN_POINT('Ctrl Pts',(19.2914105070286,-67.9591788305394,0.));
#65237=CARTESIAN_POINT('Ctrl Pts',(19.2914105070286,-67.9591788305394,12.));
#65238=CARTESIAN_POINT('Ctrl Pts',(19.302810890038,-67.9770075733485,0.));
#65239=CARTESIAN_POINT('Ctrl Pts',(19.302810890038,-67.9770075733485,12.));
#65240=CARTESIAN_POINT('Ctrl Pts',(19.3142564958202,-67.9948661329617,0.));
#65241=CARTESIAN_POINT('Ctrl Pts',(19.3142564958202,-67.9948661329617,12.));
#65242=CARTESIAN_POINT('Ctrl Pts',(19.3257473032034,-68.0127543311776,0.));
#65243=CARTESIAN_POINT('Ctrl Pts',(19.3257473032034,-68.0127543311776,12.));
#65244=CARTESIAN_POINT('Ctrl Pts',(19.3372832910076,-68.0306719906636,0.));
#65245=CARTESIAN_POINT('Ctrl Pts',(19.3372832910076,-68.0306719906636,12.));
#65246=CARTESIAN_POINT('Ctrl Pts',(19.3488644380641,-68.0486189351011,0.));
#65247=CARTESIAN_POINT('Ctrl Pts',(19.3488644380641,-68.0486189351011,12.));
#65248=CARTESIAN_POINT('Ctrl Pts',(19.3604907232313,-68.0665949893195,0.));
#65249=CARTESIAN_POINT('Ctrl Pts',(19.3604907232313,-68.0665949893195,12.));
#65250=CARTESIAN_POINT('Ctrl Pts',(19.3721621253912,-68.0845999792247,0.));
#65251=CARTESIAN_POINT('Ctrl Pts',(19.3721621253912,-68.0845999792247,12.));
#65252=CARTESIAN_POINT('Ctrl Pts',(19.3838786234421,-68.1026337317285,0.));
#65253=CARTESIAN_POINT('Ctrl Pts',(19.3838786234421,-68.1026337317285,12.));
#65254=CARTESIAN_POINT('Ctrl Pts',(19.3956401962894,-68.1206960746769,0.));
#65255=CARTESIAN_POINT('Ctrl Pts',(19.3956401962894,-68.1206960746769,12.));
#65256=CARTESIAN_POINT('Ctrl Pts',(19.4074468228299,-68.1387868367691,0.));
#65257=CARTESIAN_POINT('Ctrl Pts',(19.4074468228299,-68.1387868367691,12.));
#65258=CARTESIAN_POINT('Ctrl Pts',(19.4192984819418,-68.1569058475054,0.));
#65259=CARTESIAN_POINT('Ctrl Pts',(19.4192984819418,-68.1569058475054,12.));
#65260=CARTESIAN_POINT('Ctrl Pts',(19.4311951524983,-68.1750529372232,0.));
#65261=CARTESIAN_POINT('Ctrl Pts',(19.4311951524983,-68.1750529372232,12.));
#65262=CARTESIAN_POINT('Ctrl Pts',(19.4431368133719,-68.1932279371127,0.));
#65263=CARTESIAN_POINT('Ctrl Pts',(19.4431368133719,-68.1932279371127,12.));
#65264=CARTESIAN_POINT('Ctrl Pts',(19.455123443438,-68.2114306792358,0.));
#65265=CARTESIAN_POINT('Ctrl Pts',(19.455123443438,-68.2114306792358,12.));
#65266=CARTESIAN_POINT('Ctrl Pts',(19.467155021572,-68.2296609965448,0.));
#65267=CARTESIAN_POINT('Ctrl Pts',(19.467155021572,-68.2296609965448,12.));
#65268=CARTESIAN_POINT('Ctrl Pts',(19.4792315266501,-68.2479187228803,0.));
#65269=CARTESIAN_POINT('Ctrl Pts',(19.4792315266501,-68.2479187228803,12.));
#65270=CARTESIAN_POINT('Ctrl Pts',(19.4913529375543,-68.2662036929526,0.));
#65271=CARTESIAN_POINT('Ctrl Pts',(19.4913529375543,-68.2662036929526,12.));
#65272=CARTESIAN_POINT('Ctrl Pts',(19.5035192331705,-68.2845157423233,0.));
#65273=CARTESIAN_POINT('Ctrl Pts',(19.5035192331705,-68.2845157423233,12.));
#65274=CARTESIAN_POINT('Ctrl Pts',(19.5157303923856,-68.3028547073865,0.));
#65275=CARTESIAN_POINT('Ctrl Pts',(19.5157303923856,-68.3028547073865,12.));
#65276=CARTESIAN_POINT('Ctrl Pts',(19.5279863940773,-68.3212204253417,0.));
#65277=CARTESIAN_POINT('Ctrl Pts',(19.5279863940773,-68.3212204253417,12.));
#65278=CARTESIAN_POINT('Ctrl Pts',(19.540287217119,-68.3396127341938,0.));
#65279=CARTESIAN_POINT('Ctrl Pts',(19.540287217119,-68.3396127341938,12.));
#65280=CARTESIAN_POINT('Ctrl Pts',(19.5526328403852,-68.3580314727523,0.));
#65281=CARTESIAN_POINT('Ctrl Pts',(19.5526328403852,-68.3580314727523,12.));
#65282=CARTESIAN_POINT('Ctrl Pts',(19.5650232427515,-68.3764764806287,0.));
#65283=CARTESIAN_POINT('Ctrl Pts',(19.5650232427515,-68.3764764806287,12.));
#65284=CARTESIAN_POINT('Ctrl Pts',(19.5774584030937,-68.3949475982335,0.));
#65285=CARTESIAN_POINT('Ctrl Pts',(19.5774584030937,-68.3949475982335,12.));
#65286=CARTESIAN_POINT('Ctrl Pts',(19.5899383002802,-68.4134446667696,0.));
#65287=CARTESIAN_POINT('Ctrl Pts',(19.5899383002802,-68.4134446667696,12.));
#65288=CARTESIAN_POINT('Ctrl Pts',(19.6024629131784,-68.4319675282275,0.));
#65289=CARTESIAN_POINT('Ctrl Pts',(19.6024629131784,-68.4319675282275,12.));
#65290=CARTESIAN_POINT('Ctrl Pts',(19.6150322206577,-68.4505160253778,0.));
#65291=CARTESIAN_POINT('Ctrl Pts',(19.6150322206577,-68.4505160253778,12.));
#65292=CARTESIAN_POINT('Ctrl Pts',(19.6276462015888,-68.4690900017632,0.));
#65293=CARTESIAN_POINT('Ctrl Pts',(19.6276462015888,-68.4690900017632,12.));
#65294=CARTESIAN_POINT('Ctrl Pts',(19.6403048348395,-68.4876893016856,0.));
#65295=CARTESIAN_POINT('Ctrl Pts',(19.6403048348395,-68.4876893016856,12.));
#65296=CARTESIAN_POINT('Ctrl Pts',(19.6530080992686,-68.5063137701971,0.));
#65297=CARTESIAN_POINT('Ctrl Pts',(19.6530080992686,-68.5063137701971,12.));
#65298=CARTESIAN_POINT('Ctrl Pts',(19.6657559737336,-68.5249632530979,0.));
#65299=CARTESIAN_POINT('Ctrl Pts',(19.6657559737336,-68.5249632530979,12.));
#65300=CARTESIAN_POINT('Ctrl Pts',(19.6785484370926,-68.5436375969311,0.));
#65301=CARTESIAN_POINT('Ctrl Pts',(19.6785484370926,-68.5436375969311,12.));
#65302=CARTESIAN_POINT('Ctrl Pts',(19.6913854682046,-68.5623366489779,0.));
#65303=CARTESIAN_POINT('Ctrl Pts',(19.6913854682046,-68.5623366489779,12.));
#65304=CARTESIAN_POINT('Ctrl Pts',(19.7042670459237,-68.581060257249,0.));
#65305=CARTESIAN_POINT('Ctrl Pts',(19.7042670459237,-68.581060257249,12.));
#65306=CARTESIAN_POINT('Ctrl Pts',(19.7171931490956,-68.5998082704766,0.));
#65307=CARTESIAN_POINT('Ctrl Pts',(19.7171931490956,-68.5998082704766,12.));
#65308=CARTESIAN_POINT('Ctrl Pts',(19.7301637565652,-68.6185805381126,0.));
#65309=CARTESIAN_POINT('Ctrl Pts',(19.7301637565652,-68.6185805381126,12.));
#65310=CARTESIAN_POINT('Ctrl Pts',(19.7431788471775,-68.6373769103224,0.));
#65311=CARTESIAN_POINT('Ctrl Pts',(19.7431788471775,-68.6373769103224,12.));
#65312=CARTESIAN_POINT('Ctrl Pts',(19.7562383997781,-68.6561972379793,0.));
#65313=CARTESIAN_POINT('Ctrl Pts',(19.7562383997781,-68.6561972379793,12.));
#65314=CARTESIAN_POINT('Ctrl Pts',(19.7693423932058,-68.6750413726547,0.));
#65315=CARTESIAN_POINT('Ctrl Pts',(19.7693423932058,-68.6750413726547,12.));
#65316=CARTESIAN_POINT('Ctrl Pts',(19.7824908062913,-68.6939091666111,0.));
#65317=CARTESIAN_POINT('Ctrl Pts',(19.7824908062913,-68.6939091666111,12.));
#65318=CARTESIAN_POINT('Ctrl Pts',(19.795683617864,-68.7128004727998,0.));
#65319=CARTESIAN_POINT('Ctrl Pts',(19.795683617864,-68.7128004727998,12.));
#65320=CARTESIAN_POINT('Ctrl Pts',(19.8089208067532,-68.7317151448557,0.));
#65321=CARTESIAN_POINT('Ctrl Pts',(19.8089208067532,-68.7317151448557,12.));
#65322=CARTESIAN_POINT('Ctrl Pts',(19.8222023517874,-68.7506530370918,0.));
#65323=CARTESIAN_POINT('Ctrl Pts',(19.8222023517874,-68.7506530370918,12.));
#65324=CARTESIAN_POINT('Ctrl Pts',(19.835528231787,-68.7696140044892,0.));
#65325=CARTESIAN_POINT('Ctrl Pts',(19.835528231787,-68.7696140044892,12.));
#65326=CARTESIAN_POINT('Ctrl Pts',(19.8488984255641,-68.7885979026927,0.));
#65327=CARTESIAN_POINT('Ctrl Pts',(19.8488984255641,-68.7885979026927,12.));
#65328=CARTESIAN_POINT('Ctrl Pts',(19.8623129119304,-68.8076045880102,0.));
#65329=CARTESIAN_POINT('Ctrl Pts',(19.8623129119304,-68.8076045880102,12.));
#65330=CARTESIAN_POINT('Ctrl Pts',(19.8757716696968,-68.8266339174068,0.));
#65331=CARTESIAN_POINT('Ctrl Pts',(19.8757716696968,-68.8266339174068,12.));
#65332=CARTESIAN_POINT('Ctrl Pts',(19.8892746776733,-68.8456857484988,0.));
#65333=CARTESIAN_POINT('Ctrl Pts',(19.8892746776733,-68.8456857484988,12.));
#65334=CARTESIAN_POINT('Ctrl Pts',(19.9028219146606,-68.8647599395437,0.));
#65335=CARTESIAN_POINT('Ctrl Pts',(19.9028219146606,-68.8647599395437,12.));
#65336=CARTESIAN_POINT('Ctrl Pts',(19.9164133594512,-68.8838563494356,0.));
#65337=CARTESIAN_POINT('Ctrl Pts',(19.9164133594512,-68.8838563494356,12.));
#65338=CARTESIAN_POINT('Ctrl Pts',(19.9300489908364,-68.902974837704,0.));
#65339=CARTESIAN_POINT('Ctrl Pts',(19.9300489908364,-68.902974837704,12.));
#65340=CARTESIAN_POINT('Ctrl Pts',(19.9437287876063,-68.9221152645086,0.));
#65341=CARTESIAN_POINT('Ctrl Pts',(19.9437287876063,-68.9221152645086,12.));
#65342=CARTESIAN_POINT('Ctrl Pts',(19.9574527285492,-68.9412774906346,0.));
#65343=CARTESIAN_POINT('Ctrl Pts',(19.9574527285492,-68.9412774906346,12.));
#65344=CARTESIAN_POINT('Ctrl Pts',(19.9712207924436,-68.960461377483,0.));
#65345=CARTESIAN_POINT('Ctrl Pts',(19.9712207924436,-68.960461377483,12.));
#65346=CARTESIAN_POINT('Ctrl Pts',(19.9850329580599,-68.9796667870667,0.));
#65347=CARTESIAN_POINT('Ctrl Pts',(19.9850329580599,-68.9796667870667,12.));
#65348=CARTESIAN_POINT('Ctrl Pts',(19.9988892041671,-68.9988935820101,0.));
#65349=CARTESIAN_POINT('Ctrl Pts',(19.9988892041671,-68.9988935820101,12.));
#65350=CARTESIAN_POINT('Ctrl Pts',(20.0127895095326,-69.0181416255433,0.));
#65351=CARTESIAN_POINT('Ctrl Pts',(20.0127895095326,-69.0181416255433,12.));
#65352=CARTESIAN_POINT('Ctrl Pts',(20.026733852922,-69.0374107814977,0.));
#65353=CARTESIAN_POINT('Ctrl Pts',(20.026733852922,-69.0374107814977,12.));
#65354=CARTESIAN_POINT('Ctrl Pts',(20.0407222130902,-69.0567009142968,0.));
#65355=CARTESIAN_POINT('Ctrl Pts',(20.0407222130902,-69.0567009142968,12.));
#65356=CARTESIAN_POINT('Ctrl Pts',(20.0547545687839,-69.0760118889525,0.));
#65357=CARTESIAN_POINT('Ctrl Pts',(20.0547545687839,-69.0760118889525,12.));
#65358=CARTESIAN_POINT('Ctrl Pts',(20.0688308987478,-69.0953435710634,0.));
#65359=CARTESIAN_POINT('Ctrl Pts',(20.0688308987478,-69.0953435710634,12.));
#65360=CARTESIAN_POINT('Ctrl Pts',(20.082951181725,-69.1146958268104,0.));
#65361=CARTESIAN_POINT('Ctrl Pts',(20.082951181725,-69.1146958268104,12.));
#65362=CARTESIAN_POINT('Ctrl Pts',(20.0971153964557,-69.1340685229516,0.));
#65363=CARTESIAN_POINT('Ctrl Pts',(20.0971153964557,-69.1340685229516,12.));
#65364=CARTESIAN_POINT('Ctrl Pts',(20.1113235216693,-69.1534615268153,0.));
#65365=CARTESIAN_POINT('Ctrl Pts',(20.1113235216693,-69.1534615268153,12.));
#65366=CARTESIAN_POINT('Ctrl Pts',(20.125575536087,-69.172874706296,0.));
#65367=CARTESIAN_POINT('Ctrl Pts',(20.125575536087,-69.172874706296,12.));
#65368=CARTESIAN_POINT('Ctrl Pts',(20.1398714184278,-69.1923079298534,0.));
#65369=CARTESIAN_POINT('Ctrl Pts',(20.1398714184278,-69.1923079298534,12.));
#65370=CARTESIAN_POINT('Ctrl Pts',(20.1542111474086,-69.2117610665073,0.));
#65371=CARTESIAN_POINT('Ctrl Pts',(20.1542111474086,-69.2117610665073,12.));
#65372=CARTESIAN_POINT('Ctrl Pts',(20.1685947017433,-69.2312339858337,0.));
#65373=CARTESIAN_POINT('Ctrl Pts',(20.1685947017433,-69.2312339858337,12.));
#65374=CARTESIAN_POINT('Ctrl Pts',(20.183022060135,-69.2507265579562,0.));
#65375=CARTESIAN_POINT('Ctrl Pts',(20.183022060135,-69.2507265579562,12.));
#65376=CARTESIAN_POINT('Ctrl Pts',(20.1974932012775,-69.2702386535432,0.));
#65377=CARTESIAN_POINT('Ctrl Pts',(20.1974932012775,-69.2702386535432,12.));
#65378=CARTESIAN_POINT('Ctrl Pts',(20.2120081038621,-69.2897701438066,0.));
#65379=CARTESIAN_POINT('Ctrl Pts',(20.2120081038621,-69.2897701438066,12.));
#65380=CARTESIAN_POINT('Ctrl Pts',(20.2265667465783,-69.3093209004986,0.));
#65381=CARTESIAN_POINT('Ctrl Pts',(20.2265667465783,-69.3093209004986,12.));
#65382=CARTESIAN_POINT('Ctrl Pts',(20.2411691081122,-69.3288907959065,0.));
#65383=CARTESIAN_POINT('Ctrl Pts',(20.2411691081122,-69.3288907959065,12.));
#65384=CARTESIAN_POINT('Ctrl Pts',(20.255815167139,-69.3484797028454,0.));
#65385=CARTESIAN_POINT('Ctrl Pts',(20.255815167139,-69.3484797028454,12.));
#65386=CARTESIAN_POINT('Ctrl Pts',(20.270504902324,-69.3680874946548,0.));
#65387=CARTESIAN_POINT('Ctrl Pts',(20.270504902324,-69.3680874946548,12.));
#65388=CARTESIAN_POINT('Ctrl Pts',(20.2852382923299,-69.3877140451975,0.));
#65389=CARTESIAN_POINT('Ctrl Pts',(20.2852382923299,-69.3877140451975,12.));
#65390=CARTESIAN_POINT('Ctrl Pts',(20.3000153158167,-69.4073592288562,0.));
#65391=CARTESIAN_POINT('Ctrl Pts',(20.3000153158167,-69.4073592288562,12.));
#65392=CARTESIAN_POINT('Ctrl Pts',(20.3148359514414,-69.4270229205296,0.));
#65393=CARTESIAN_POINT('Ctrl Pts',(20.3148359514414,-69.4270229205296,12.));
#65394=CARTESIAN_POINT('Ctrl Pts',(20.3297001778505,-69.4467049956257,0.));
#65395=CARTESIAN_POINT('Ctrl Pts',(20.3297001778505,-69.4467049956257,12.));
#65396=CARTESIAN_POINT('Ctrl Pts',(20.3446079736798,-69.4664053300579,0.));
#65397=CARTESIAN_POINT('Ctrl Pts',(20.3446079736798,-69.4664053300579,12.));
#65398=CARTESIAN_POINT('Ctrl Pts',(20.3595593175619,-69.4861238002433,0.));
#65399=CARTESIAN_POINT('Ctrl Pts',(20.3595593175619,-69.4861238002433,12.));
#65400=CARTESIAN_POINT('Ctrl Pts',(20.3745541881266,-69.5058602831004,0.));
#65401=CARTESIAN_POINT('Ctrl Pts',(20.3745541881266,-69.5058602831004,12.));
#65402=CARTESIAN_POINT('Ctrl Pts',(20.3895925640006,-69.5256146560444,0.));
#65403=CARTESIAN_POINT('Ctrl Pts',(20.3895925640006,-69.5256146560444,12.));
#65404=CARTESIAN_POINT('Ctrl Pts',(20.4046744238002,-69.5453867969815,0.));
#65405=CARTESIAN_POINT('Ctrl Pts',(20.4046744238002,-69.5453867969815,12.));
#65406=CARTESIAN_POINT('Ctrl Pts',(20.4197997461305,-69.565176584305,0.));
#65407=CARTESIAN_POINT('Ctrl Pts',(20.4197997461305,-69.565176584305,12.));
#65408=CARTESIAN_POINT('Ctrl Pts',(20.4349685095928,-69.5849838968944,0.));
#65409=CARTESIAN_POINT('Ctrl Pts',(20.4349685095928,-69.5849838968944,12.));
#65410=CARTESIAN_POINT('Ctrl Pts',(20.4501806927854,-69.6048086141122,0.));
#65411=CARTESIAN_POINT('Ctrl Pts',(20.4501806927854,-69.6048086141122,12.));
#65412=CARTESIAN_POINT('Ctrl Pts',(20.4654362743036,-69.6246506158009,0.));
#65413=CARTESIAN_POINT('Ctrl Pts',(20.4654362743036,-69.6246506158009,12.));
#65414=CARTESIAN_POINT('Ctrl Pts',(20.4807352327335,-69.6445097822778,0.));
#65415=CARTESIAN_POINT('Ctrl Pts',(20.4807352327335,-69.6445097822778,12.));
#65416=CARTESIAN_POINT('Ctrl Pts',(20.4960775466486,-69.6643859943291,0.));
#65417=CARTESIAN_POINT('Ctrl Pts',(20.4960775466486,-69.6643859943291,12.));
#65418=CARTESIAN_POINT('Ctrl Pts',(20.511463194618,-69.6842791332102,0.));
#65419=CARTESIAN_POINT('Ctrl Pts',(20.511463194618,-69.6842791332102,12.));
#65420=CARTESIAN_POINT('Ctrl Pts',(20.5268921552075,-69.7041890806421,0.));
#65421=CARTESIAN_POINT('Ctrl Pts',(20.5268921552075,-69.7041890806421,12.));
#65422=CARTESIAN_POINT('Ctrl Pts',(20.5423644069799,-69.7241157188086,0.));
#65423=CARTESIAN_POINT('Ctrl Pts',(20.5423644069799,-69.7241157188086,12.));
#65424=CARTESIAN_POINT('Ctrl Pts',(20.5578799284897,-69.7440589303511,0.));
#65425=CARTESIAN_POINT('Ctrl Pts',(20.5578799284897,-69.7440589303511,12.));
#65426=CARTESIAN_POINT('Ctrl Pts',(20.5734386982781,-69.7640185983641,0.));
#65427=CARTESIAN_POINT('Ctrl Pts',(20.5734386982781,-69.7640185983641,12.));
#65428=CARTESIAN_POINT('Ctrl Pts',(20.5890406948808,-69.7839946063942,0.));
#65429=CARTESIAN_POINT('Ctrl Pts',(20.5890406948808,-69.7839946063942,12.));
#65430=CARTESIAN_POINT('Ctrl Pts',(20.6046858968305,-69.8039868384382,0.));
#65431=CARTESIAN_POINT('Ctrl Pts',(20.6046858968305,-69.8039868384382,12.));
#65432=CARTESIAN_POINT('Ctrl Pts',(20.6203742826565,-69.8239951789402,0.));
#65433=CARTESIAN_POINT('Ctrl Pts',(20.6203742826565,-69.8239951789402,12.));
#65434=CARTESIAN_POINT('Ctrl Pts',(20.6361058308812,-69.8440195127874,0.));
#65435=CARTESIAN_POINT('Ctrl Pts',(20.6361058308812,-69.8440195127874,12.));
#65436=CARTESIAN_POINT('Ctrl Pts',(20.6518805200131,-69.8640597253058,0.));
#65437=CARTESIAN_POINT('Ctrl Pts',(20.6518805200131,-69.8640597253058,12.));
#65438=CARTESIAN_POINT('Ctrl Pts',(20.6676983285542,-69.884115702258,0.));
#65439=CARTESIAN_POINT('Ctrl Pts',(20.6676983285542,-69.884115702258,12.));
#65440=CARTESIAN_POINT('Ctrl Pts',(20.683559235003,-69.9041873298416,0.));
#65441=CARTESIAN_POINT('Ctrl Pts',(20.683559235003,-69.9041873298416,12.));
#65442=CARTESIAN_POINT('Ctrl Pts',(20.6994632178551,-69.9242744946854,0.));
#65443=CARTESIAN_POINT('Ctrl Pts',(20.6994632178551,-69.9242744946854,12.));
#65444=CARTESIAN_POINT('Ctrl Pts',(20.7154102555996,-69.9443770838444,0.));
#65445=CARTESIAN_POINT('Ctrl Pts',(20.7154102555996,-69.9443770838444,12.));
#65446=CARTESIAN_POINT('Ctrl Pts',(20.7314003267118,-69.9644949847929,0.));
#65447=CARTESIAN_POINT('Ctrl Pts',(20.7314003267118,-69.9644949847929,12.));
#65448=CARTESIAN_POINT('Ctrl Pts',(20.7474334096581,-69.9846280854254,0.));
#65449=CARTESIAN_POINT('Ctrl Pts',(20.7474334096581,-69.9846280854254,12.));
#65450=CARTESIAN_POINT('Ctrl Pts',(20.7635094829016,-70.0047762740569,0.));
#65451=CARTESIAN_POINT('Ctrl Pts',(20.7635094829016,-70.0047762740569,12.));
#65452=CARTESIAN_POINT('Ctrl Pts',(20.7796285249022,-70.0249394394221,0.));
#65453=CARTESIAN_POINT('Ctrl Pts',(20.7796285249022,-70.0249394394221,12.));
#65454=CARTESIAN_POINT('Ctrl Pts',(20.7957905141155,-70.0451174706739,0.));
#65455=CARTESIAN_POINT('Ctrl Pts',(20.7957905141155,-70.0451174706739,12.));
#65456=CARTESIAN_POINT('Ctrl Pts',(20.8119954289845,-70.0653102573798,0.));
#65457=CARTESIAN_POINT('Ctrl Pts',(20.8119954289845,-70.0653102573798,12.));
#65458=CARTESIAN_POINT('Ctrl Pts',(20.8282432479425,-70.0855176895185,0.));
#65459=CARTESIAN_POINT('Ctrl Pts',(20.8282432479425,-70.0855176895185,12.));
#65460=CARTESIAN_POINT('Ctrl Pts',(20.8445339494184,-70.1057396574741,0.));
#65461=CARTESIAN_POINT('Ctrl Pts',(20.8445339494184,-70.1057396574741,12.));
#65462=CARTESIAN_POINT('Ctrl Pts',(20.8608675118377,-70.1259760520306,0.));
#65463=CARTESIAN_POINT('Ctrl Pts',(20.8608675118377,-70.1259760520306,12.));
#65464=CARTESIAN_POINT('Ctrl Pts',(20.8772439136206,-70.1462267643649,0.));
#65465=CARTESIAN_POINT('Ctrl Pts',(20.8772439136206,-70.1462267643649,12.));
#65466=CARTESIAN_POINT('Ctrl Pts',(20.893663133175,-70.1664916860366,0.));
#65467=CARTESIAN_POINT('Ctrl Pts',(20.893663133175,-70.1664916860366,12.));
#65468=CARTESIAN_POINT('Ctrl Pts',(20.9101251488948,-70.1867707089866,0.));
#65469=CARTESIAN_POINT('Ctrl Pts',(20.9101251488948,-70.1867707089866,12.));
#65470=CARTESIAN_POINT('Ctrl Pts',(20.9266299391687,-70.2070637255469,0.));
#65471=CARTESIAN_POINT('Ctrl Pts',(20.9266299391687,-70.2070637255469,12.));
#65472=CARTESIAN_POINT('Ctrl Pts',(20.9431774823833,-70.2273706284479,0.));
#65473=CARTESIAN_POINT('Ctrl Pts',(20.9431774823833,-70.2273706284479,12.));
#65474=CARTESIAN_POINT('Ctrl Pts',(20.9597677569227,-70.2476913108242,0.));
#65475=CARTESIAN_POINT('Ctrl Pts',(20.9597677569227,-70.2476913108242,12.));
#65476=CARTESIAN_POINT('Ctrl Pts',(20.9764007411648,-70.2680256662215,0.));
#65477=CARTESIAN_POINT('Ctrl Pts',(20.9764007411648,-70.2680256662215,12.));
#65478=CARTESIAN_POINT('Ctrl Pts',(20.993076413477,-70.2883735885971,0.));
#65479=CARTESIAN_POINT('Ctrl Pts',(20.993076413477,-70.2883735885971,12.));
#65480=CARTESIAN_POINT('Ctrl Pts',(21.0097947522212,-70.3087349722959,0.));
#65481=CARTESIAN_POINT('Ctrl Pts',(21.0097947522212,-70.3087349722959,12.));
#65482=CARTESIAN_POINT('Ctrl Pts',(21.0265557357544,-70.3291097120293,0.));
#65483=CARTESIAN_POINT('Ctrl Pts',(21.0265557357544,-70.3291097120293,12.));
#65484=CARTESIAN_POINT('Ctrl Pts',(21.0433593424265,-70.3494977028497,0.));
#65485=CARTESIAN_POINT('Ctrl Pts',(21.0433593424265,-70.3494977028497,12.));
#65486=CARTESIAN_POINT('Ctrl Pts',(21.0602055505751,-70.3698988401291,0.));
#65487=CARTESIAN_POINT('Ctrl Pts',(21.0602055505751,-70.3698988401291,12.));
#65488=CARTESIAN_POINT('Ctrl Pts',(21.0770943385145,-70.3903130195279,0.));
#65489=CARTESIAN_POINT('Ctrl Pts',(21.0770943385145,-70.3903130195279,12.));
#65490=CARTESIAN_POINT('Ctrl Pts',(21.0940256845477,-70.4107401370403,0.));
#65491=CARTESIAN_POINT('Ctrl Pts',(21.0940256845477,-70.4107401370403,12.));
#65492=CARTESIAN_POINT('Ctrl Pts',(21.110999566975,-70.4311800890411,0.));
#65493=CARTESIAN_POINT('Ctrl Pts',(21.110999566975,-70.4311800890411,12.));
#65494=CARTESIAN_POINT('Ctrl Pts',(21.1280159641003,-70.4516327723349,0.));
#65495=CARTESIAN_POINT('Ctrl Pts',(21.1280159641003,-70.4516327723349,12.));
#65496=CARTESIAN_POINT('Ctrl Pts',(21.1450748542334,-70.4720980841934,0.));
#65497=CARTESIAN_POINT('Ctrl Pts',(21.1450748542334,-70.4720980841934,12.));
#65498=CARTESIAN_POINT('Ctrl Pts',(21.1621762156894,-70.4925759224208,0.));
#65499=CARTESIAN_POINT('Ctrl Pts',(21.1621762156894,-70.4925759224208,12.));
#65500=CARTESIAN_POINT('Ctrl Pts',(21.1793200267843,-70.5130661852946,0.));
#65501=CARTESIAN_POINT('Ctrl Pts',(21.1793200267843,-70.5130661852946,12.));
#65502=CARTESIAN_POINT('Ctrl Pts',(21.1965062658295,-70.5335687714422,0.));
#65503=CARTESIAN_POINT('Ctrl Pts',(21.1965062658295,-70.5335687714422,12.));
#65504=CARTESIAN_POINT('Ctrl Pts',(21.2137349111207,-70.5540835797281,0.));
#65505=CARTESIAN_POINT('Ctrl Pts',(21.2137349111207,-70.5540835797281,12.));
#65506=CARTESIAN_POINT('Ctrl Pts',(21.2310059409265,-70.5746105091503,0.));
#65507=CARTESIAN_POINT('Ctrl Pts',(21.2310059409265,-70.5746105091503,12.));
#65508=CARTESIAN_POINT('Ctrl Pts',(21.2483193334676,-70.5951494586961,0.));
#65509=CARTESIAN_POINT('Ctrl Pts',(21.2483193334676,-70.5951494586961,12.));
#65510=CARTESIAN_POINT('Ctrl Pts',(21.2656750669129,-70.6157003273326,0.));
#65511=CARTESIAN_POINT('Ctrl Pts',(21.2656750669129,-70.6157003273326,12.));
#65512=CARTESIAN_POINT('Ctrl Pts',(21.2830731194187,-70.6362630143062,0.));
#65513=CARTESIAN_POINT('Ctrl Pts',(21.2830731194187,-70.6362630143062,12.));
#65514=CARTESIAN_POINT('Ctrl Pts',(21.3005134691563,-70.6568374193786,0.));
#65515=CARTESIAN_POINT('Ctrl Pts',(21.3005134691563,-70.6568374193786,12.));
#65516=CARTESIAN_POINT('Ctrl Pts',(21.3179960943388,-70.6774234430899,0.));
#65517=CARTESIAN_POINT('Ctrl Pts',(21.3179960943388,-70.6774234430899,12.));
#65518=CARTESIAN_POINT('Ctrl Pts',(21.3355209732438,-70.6980209870032,0.));
#65519=CARTESIAN_POINT('Ctrl Pts',(21.3355209732438,-70.6980209870032,12.));
#65520=CARTESIAN_POINT('Ctrl Pts',(21.353088084234,-70.7186299539698,0.));
#65521=CARTESIAN_POINT('Ctrl Pts',(21.353088084234,-70.7186299539698,12.));
#65522=CARTESIAN_POINT('Ctrl Pts',(21.3706974057028,-70.7392502475438,0.));
#65523=CARTESIAN_POINT('Ctrl Pts',(21.3706974057028,-70.7392502475438,12.));
#65524=CARTESIAN_POINT('Ctrl Pts',(21.3883489160187,-70.7598817714078,0.));
#65525=CARTESIAN_POINT('Ctrl Pts',(21.3883489160187,-70.7598817714078,12.));
#65526=CARTESIAN_POINT('Ctrl Pts',(21.4060425934594,-70.780524428744,0.));
#65527=CARTESIAN_POINT('Ctrl Pts',(21.4060425934594,-70.780524428744,12.));
#65528=CARTESIAN_POINT('Ctrl Pts',(21.4237784161592,-70.8011781217409,0.));
#65529=CARTESIAN_POINT('Ctrl Pts',(21.4237784161592,-70.8011781217409,12.));
#65530=CARTESIAN_POINT('Ctrl Pts',(21.4415563620127,-70.8218427507545,0.));
#65531=CARTESIAN_POINT('Ctrl Pts',(21.4415563620127,-70.8218427507545,12.));
#65532=CARTESIAN_POINT('Ctrl Pts',(21.4593764087492,-70.84251821499,0.));
#65533=CARTESIAN_POINT('Ctrl Pts',(21.4593764087492,-70.84251821499,12.));
#65534=CARTESIAN_POINT('Ctrl Pts',(21.4772385340978,-70.8632044140166,0.));
#65535=CARTESIAN_POINT('Ctrl Pts',(21.4772385340978,-70.8632044140166,12.));
#65536=CARTESIAN_POINT('Ctrl Pts',(21.4951427159272,-70.8839012490903,0.));
#65537=CARTESIAN_POINT('Ctrl Pts',(21.4951427159272,-70.8839012490903,12.));
#65538=CARTESIAN_POINT('Ctrl Pts',(21.5130889323766,-70.9046086244123,0.));
#65539=CARTESIAN_POINT('Ctrl Pts',(21.5130889323766,-70.9046086244123,12.));
#65540=CARTESIAN_POINT('Ctrl Pts',(21.5310771620209,-70.9253264487576,0.));
#65541=CARTESIAN_POINT('Ctrl Pts',(21.5310771620209,-70.9253264487576,12.));
#65542=CARTESIAN_POINT('Ctrl Pts',(21.549107383907,-70.9460546358597,0.));
#65543=CARTESIAN_POINT('Ctrl Pts',(21.549107383907,-70.9460546358597,12.));
#65544=CARTESIAN_POINT('Ctrl Pts',(21.5671795771872,-70.9667931008097,0.));
#65545=CARTESIAN_POINT('Ctrl Pts',(21.5671795771872,-70.9667931008097,12.));
#65546=CARTESIAN_POINT('Ctrl Pts',(21.5852937208258,-70.9875417572138,0.));
#65547=CARTESIAN_POINT('Ctrl Pts',(21.5852937208258,-70.9875417572138,12.));
#65548=CARTESIAN_POINT('Ctrl Pts',(21.6034497932573,-71.0083005139086,0.));
#65549=CARTESIAN_POINT('Ctrl Pts',(21.6034497932573,-71.0083005139086,12.));
#65550=CARTESIAN_POINT('Ctrl Pts',(21.6216477720941,-71.0290692721932,0.));
#65551=CARTESIAN_POINT('Ctrl Pts',(21.6216477720941,-71.0290692721932,12.));
#65552=CARTESIAN_POINT('Ctrl Pts',(21.6398876337206,-71.0498479219659,0.));
#65553=CARTESIAN_POINT('Ctrl Pts',(21.6398876337206,-71.0498479219659,12.));
#65554=CARTESIAN_POINT('Ctrl Pts',(21.6581693538424,-71.0706363472965,0.));
#65555=CARTESIAN_POINT('Ctrl Pts',(21.6581693538424,-71.0706363472965,12.));
#65556=CARTESIAN_POINT('Ctrl Pts',(21.6764929081762,-71.0914344333048,0.));
#65557=CARTESIAN_POINT('Ctrl Pts',(21.6764929081762,-71.0914344333048,12.));
#65558=CARTESIAN_POINT('Ctrl Pts',(21.6948582730895,-71.1122420728349,0.));
#65559=CARTESIAN_POINT('Ctrl Pts',(21.6948582730895,-71.1122420728349,12.));
#65560=CARTESIAN_POINT('Ctrl Pts',(21.7132654262501,-71.133059172642,0.));
#65561=CARTESIAN_POINT('Ctrl Pts',(21.7132654262501,-71.133059172642,12.));
#65562=CARTESIAN_POINT('Ctrl Pts',(21.7317143472826,-71.1538856611899,0.));
#65563=CARTESIAN_POINT('Ctrl Pts',(21.7317143472826,-71.1538856611899,12.));
#65564=CARTESIAN_POINT('Ctrl Pts',(21.7502050183602,-71.1747214905981,0.));
#65565=CARTESIAN_POINT('Ctrl Pts',(21.7502050183602,-71.1747214905981,12.));
#65566=CARTESIAN_POINT('Ctrl Pts',(21.7687374247045,-71.1955666309591,0.));
#65567=CARTESIAN_POINT('Ctrl Pts',(21.7687374247045,-71.1955666309591,12.));
#65568=CARTESIAN_POINT('Ctrl Pts',(21.7835967290261,-71.212250179455,0.));
#65569=CARTESIAN_POINT('Ctrl Pts',(21.7835967290261,-71.212250179455,12.));
#65570=CARTESIAN_POINT('Ctrl Pts',(21.7947599798838,-71.2247670209821,0.));
#65571=CARTESIAN_POINT('Ctrl Pts',(21.7947599798838,-71.2247670209821,12.));
#65572=CARTESIAN_POINT('Ctrl Pts',(21.8022104901682,-71.2331134397743,0.));
#65573=CARTESIAN_POINT('Ctrl Pts',(21.8022104901682,-71.2331134397743,12.));
#65574=CARTESIAN_POINT('Ctrl Pts',(21.8059378310718,-71.2372871136137,0.));
#65575=CARTESIAN_POINT('Ctrl Pts',(21.8059378310718,-71.2372871136137,12.));
#65576=CARTESIAN_POINT('',(18.9407177820968,-67.3887914263118,0.));
#65577=CARTESIAN_POINT('Ctrl Pts',(18.9407177820968,-67.3887914263118,0.));
#65578=CARTESIAN_POINT('Ctrl Pts',(18.9426924398719,-67.3921355608328,0.));
#65579=CARTESIAN_POINT('Ctrl Pts',(18.9466463414299,-67.3988274146651,0.));
#65580=CARTESIAN_POINT('Ctrl Pts',(18.9525909517915,-67.4088759497911,0.));
#65581=CARTESIAN_POINT('Ctrl Pts',(18.9605446160985,-67.4222955061981,0.));
#65582=CARTESIAN_POINT('Ctrl Pts',(18.970532563171,-67.4391057908418,0.));
#65583=CARTESIAN_POINT('Ctrl Pts',(18.9805663798448,-67.4559518744638,0.));
#65584=CARTESIAN_POINT('Ctrl Pts',(18.9906460638625,-67.472833671964,0.));
#65585=CARTESIAN_POINT('Ctrl Pts',(19.0007716032819,-67.4897510316844,0.));
#65586=CARTESIAN_POINT('Ctrl Pts',(19.0109429761306,-67.5067037372317,0.));
#65587=CARTESIAN_POINT('Ctrl Pts',(19.021160154824,-67.5236915360331,0.));
#65588=CARTESIAN_POINT('Ctrl Pts',(19.0314231093923,-67.540714161288,0.));
#65589=CARTESIAN_POINT('Ctrl Pts',(19.0417318110708,-67.5577713558194,0.));
#65590=CARTESIAN_POINT('Ctrl Pts',(19.0520862360395,-67.5748628971964,0.));
#65591=CARTESIAN_POINT('Ctrl Pts',(19.062486364241,-67.5919885896222,0.));
#65592=CARTESIAN_POINT('Ctrl Pts',(19.072932177628,-67.6091482520534,0.));
#65593=CARTESIAN_POINT('Ctrl Pts',(19.0834236587118,-67.6263417083426,0.));
#65594=CARTESIAN_POINT('Ctrl Pts',(19.0939607887501,-67.6435687749841,0.));
#65595=CARTESIAN_POINT('Ctrl Pts',(19.1045435468358,-67.6608292549462,0.));
#65596=CARTESIAN_POINT('Ctrl Pts',(19.115171910846,-67.6781229440573,0.));
#65597=CARTESIAN_POINT('Ctrl Pts',(19.1258458580345,-67.6954496350063,0.));
#65598=CARTESIAN_POINT('Ctrl Pts',(19.136565365709,-67.7128091219348,0.));
#65599=CARTESIAN_POINT('Ctrl Pts',(19.1473304119955,-67.7302012056584,0.));
#65600=CARTESIAN_POINT('Ctrl Pts',(19.1581409758097,-67.7476256934444,0.));
#65601=CARTESIAN_POINT('Ctrl Pts',(19.1689970364949,-67.7650823965127,0.));
#65602=CARTESIAN_POINT('Ctrl Pts',(19.1798985735687,-67.7825711283096,0.));
#65603=CARTESIAN_POINT('Ctrl Pts',(19.1908455664097,-67.8000917023926,0.));
#65604=CARTESIAN_POINT('Ctrl Pts',(19.201837993993,-67.8176439306621,0.));
#65605=CARTESIAN_POINT('Ctrl Pts',(19.2128758350345,-67.835227624289,0.));
#65606=CARTESIAN_POINT('Ctrl Pts',(19.2239590681133,-67.8528425945184,0.));
#65607=CARTESIAN_POINT('Ctrl Pts',(19.2350876717874,-67.8704886534544,0.));
#65608=CARTESIAN_POINT('Ctrl Pts',(19.2462616247279,-67.8881656149955,0.));
#65609=CARTESIAN_POINT('Ctrl Pts',(19.2574809057696,-67.9058732951788,0.));
#65610=CARTESIAN_POINT('Ctrl Pts',(19.2687454938442,-67.9236115116758,0.));
#65611=CARTESIAN_POINT('Ctrl Pts',(19.280055367936,-67.9413800834793,0.));
#65612=CARTESIAN_POINT('Ctrl Pts',(19.2914105070286,-67.9591788305394,0.));
#65613=CARTESIAN_POINT('Ctrl Pts',(19.302810890038,-67.9770075733485,0.));
#65614=CARTESIAN_POINT('Ctrl Pts',(19.3142564958202,-67.9948661329617,0.));
#65615=CARTESIAN_POINT('Ctrl Pts',(19.3257473032034,-68.0127543311776,0.));
#65616=CARTESIAN_POINT('Ctrl Pts',(19.3372832910076,-68.0306719906636,0.));
#65617=CARTESIAN_POINT('Ctrl Pts',(19.3488644380641,-68.0486189351011,0.));
#65618=CARTESIAN_POINT('Ctrl Pts',(19.3604907232313,-68.0665949893195,0.));
#65619=CARTESIAN_POINT('Ctrl Pts',(19.3721621253912,-68.0845999792247,0.));
#65620=CARTESIAN_POINT('Ctrl Pts',(19.3838786234421,-68.1026337317285,0.));
#65621=CARTESIAN_POINT('Ctrl Pts',(19.3956401962894,-68.1206960746769,0.));
#65622=CARTESIAN_POINT('Ctrl Pts',(19.4074468228299,-68.1387868367691,0.));
#65623=CARTESIAN_POINT('Ctrl Pts',(19.4192984819418,-68.1569058475054,0.));
#65624=CARTESIAN_POINT('Ctrl Pts',(19.4311951524983,-68.1750529372232,0.));
#65625=CARTESIAN_POINT('Ctrl Pts',(19.4431368133719,-68.1932279371127,0.));
#65626=CARTESIAN_POINT('Ctrl Pts',(19.455123443438,-68.2114306792358,0.));
#65627=CARTESIAN_POINT('Ctrl Pts',(19.467155021572,-68.2296609965448,0.));
#65628=CARTESIAN_POINT('Ctrl Pts',(19.4792315266501,-68.2479187228803,0.));
#65629=CARTESIAN_POINT('Ctrl Pts',(19.4913529375543,-68.2662036929526,0.));
#65630=CARTESIAN_POINT('Ctrl Pts',(19.5035192331705,-68.2845157423233,0.));
#65631=CARTESIAN_POINT('Ctrl Pts',(19.5157303923856,-68.3028547073865,0.));
#65632=CARTESIAN_POINT('Ctrl Pts',(19.5279863940773,-68.3212204253417,0.));
#65633=CARTESIAN_POINT('Ctrl Pts',(19.540287217119,-68.3396127341938,0.));
#65634=CARTESIAN_POINT('Ctrl Pts',(19.5526328403852,-68.3580314727523,0.));
#65635=CARTESIAN_POINT('Ctrl Pts',(19.5650232427515,-68.3764764806287,0.));
#65636=CARTESIAN_POINT('Ctrl Pts',(19.5774584030937,-68.3949475982335,0.));
#65637=CARTESIAN_POINT('Ctrl Pts',(19.5899383002802,-68.4134446667696,0.));
#65638=CARTESIAN_POINT('Ctrl Pts',(19.6024629131784,-68.4319675282275,0.));
#65639=CARTESIAN_POINT('Ctrl Pts',(19.6150322206577,-68.4505160253778,0.));
#65640=CARTESIAN_POINT('Ctrl Pts',(19.6276462015888,-68.4690900017632,0.));
#65641=CARTESIAN_POINT('Ctrl Pts',(19.6403048348395,-68.4876893016856,0.));
#65642=CARTESIAN_POINT('Ctrl Pts',(19.6530080992686,-68.5063137701971,0.));
#65643=CARTESIAN_POINT('Ctrl Pts',(19.6657559737336,-68.5249632530979,0.));
#65644=CARTESIAN_POINT('Ctrl Pts',(19.6785484370926,-68.5436375969311,0.));
#65645=CARTESIAN_POINT('Ctrl Pts',(19.6913854682046,-68.5623366489779,0.));
#65646=CARTESIAN_POINT('Ctrl Pts',(19.7042670459237,-68.581060257249,0.));
#65647=CARTESIAN_POINT('Ctrl Pts',(19.7171931490956,-68.5998082704766,0.));
#65648=CARTESIAN_POINT('Ctrl Pts',(19.7301637565652,-68.6185805381126,0.));
#65649=CARTESIAN_POINT('Ctrl Pts',(19.7431788471775,-68.6373769103224,0.));
#65650=CARTESIAN_POINT('Ctrl Pts',(19.7562383997781,-68.6561972379793,0.));
#65651=CARTESIAN_POINT('Ctrl Pts',(19.7693423932058,-68.6750413726547,0.));
#65652=CARTESIAN_POINT('Ctrl Pts',(19.7824908062913,-68.6939091666111,0.));
#65653=CARTESIAN_POINT('Ctrl Pts',(19.795683617864,-68.7128004727998,0.));
#65654=CARTESIAN_POINT('Ctrl Pts',(19.8089208067532,-68.7317151448557,0.));
#65655=CARTESIAN_POINT('Ctrl Pts',(19.8222023517874,-68.7506530370918,0.));
#65656=CARTESIAN_POINT('Ctrl Pts',(19.835528231787,-68.7696140044892,0.));
#65657=CARTESIAN_POINT('Ctrl Pts',(19.8488984255641,-68.7885979026927,0.));
#65658=CARTESIAN_POINT('Ctrl Pts',(19.8623129119304,-68.8076045880102,0.));
#65659=CARTESIAN_POINT('Ctrl Pts',(19.8757716696968,-68.8266339174068,0.));
#65660=CARTESIAN_POINT('Ctrl Pts',(19.8892746776733,-68.8456857484988,0.));
#65661=CARTESIAN_POINT('Ctrl Pts',(19.9028219146606,-68.8647599395437,0.));
#65662=CARTESIAN_POINT('Ctrl Pts',(19.9164133594512,-68.8838563494356,0.));
#65663=CARTESIAN_POINT('Ctrl Pts',(19.9300489908364,-68.902974837704,0.));
#65664=CARTESIAN_POINT('Ctrl Pts',(19.9437287876063,-68.9221152645086,0.));
#65665=CARTESIAN_POINT('Ctrl Pts',(19.9574527285492,-68.9412774906346,0.));
#65666=CARTESIAN_POINT('Ctrl Pts',(19.9712207924436,-68.960461377483,0.));
#65667=CARTESIAN_POINT('Ctrl Pts',(19.9850329580599,-68.9796667870667,0.));
#65668=CARTESIAN_POINT('Ctrl Pts',(19.9988892041671,-68.9988935820101,0.));
#65669=CARTESIAN_POINT('Ctrl Pts',(20.0127895095326,-69.0181416255433,0.));
#65670=CARTESIAN_POINT('Ctrl Pts',(20.026733852922,-69.0374107814977,0.));
#65671=CARTESIAN_POINT('Ctrl Pts',(20.0407222130902,-69.0567009142968,0.));
#65672=CARTESIAN_POINT('Ctrl Pts',(20.0547545687839,-69.0760118889525,0.));
#65673=CARTESIAN_POINT('Ctrl Pts',(20.0688308987478,-69.0953435710634,0.));
#65674=CARTESIAN_POINT('Ctrl Pts',(20.082951181725,-69.1146958268104,0.));
#65675=CARTESIAN_POINT('Ctrl Pts',(20.0971153964557,-69.1340685229516,0.));
#65676=CARTESIAN_POINT('Ctrl Pts',(20.1113235216693,-69.1534615268153,0.));
#65677=CARTESIAN_POINT('Ctrl Pts',(20.125575536087,-69.172874706296,0.));
#65678=CARTESIAN_POINT('Ctrl Pts',(20.1398714184278,-69.1923079298534,0.));
#65679=CARTESIAN_POINT('Ctrl Pts',(20.1542111474086,-69.2117610665073,0.));
#65680=CARTESIAN_POINT('Ctrl Pts',(20.1685947017433,-69.2312339858337,0.));
#65681=CARTESIAN_POINT('Ctrl Pts',(20.183022060135,-69.2507265579562,0.));
#65682=CARTESIAN_POINT('Ctrl Pts',(20.1974932012775,-69.2702386535432,0.));
#65683=CARTESIAN_POINT('Ctrl Pts',(20.2120081038621,-69.2897701438066,0.));
#65684=CARTESIAN_POINT('Ctrl Pts',(20.2265667465783,-69.3093209004986,0.));
#65685=CARTESIAN_POINT('Ctrl Pts',(20.2411691081122,-69.3288907959065,0.));
#65686=CARTESIAN_POINT('Ctrl Pts',(20.255815167139,-69.3484797028454,0.));
#65687=CARTESIAN_POINT('Ctrl Pts',(20.270504902324,-69.3680874946548,0.));
#65688=CARTESIAN_POINT('Ctrl Pts',(20.2852382923299,-69.3877140451975,0.));
#65689=CARTESIAN_POINT('Ctrl Pts',(20.3000153158167,-69.4073592288562,0.));
#65690=CARTESIAN_POINT('Ctrl Pts',(20.3148359514414,-69.4270229205296,0.));
#65691=CARTESIAN_POINT('Ctrl Pts',(20.3297001778505,-69.4467049956257,0.));
#65692=CARTESIAN_POINT('Ctrl Pts',(20.3446079736798,-69.4664053300579,0.));
#65693=CARTESIAN_POINT('Ctrl Pts',(20.3595593175619,-69.4861238002433,0.));
#65694=CARTESIAN_POINT('Ctrl Pts',(20.3745541881266,-69.5058602831004,0.));
#65695=CARTESIAN_POINT('Ctrl Pts',(20.3895925640006,-69.5256146560444,0.));
#65696=CARTESIAN_POINT('Ctrl Pts',(20.4046744238002,-69.5453867969815,0.));
#65697=CARTESIAN_POINT('Ctrl Pts',(20.4197997461305,-69.565176584305,0.));
#65698=CARTESIAN_POINT('Ctrl Pts',(20.4349685095928,-69.5849838968944,0.));
#65699=CARTESIAN_POINT('Ctrl Pts',(20.4501806927854,-69.6048086141122,0.));
#65700=CARTESIAN_POINT('Ctrl Pts',(20.4654362743036,-69.6246506158009,0.));
#65701=CARTESIAN_POINT('Ctrl Pts',(20.4807352327335,-69.6445097822778,0.));
#65702=CARTESIAN_POINT('Ctrl Pts',(20.4960775466486,-69.6643859943291,0.));
#65703=CARTESIAN_POINT('Ctrl Pts',(20.511463194618,-69.6842791332102,0.));
#65704=CARTESIAN_POINT('Ctrl Pts',(20.5268921552075,-69.7041890806421,0.));
#65705=CARTESIAN_POINT('Ctrl Pts',(20.5423644069799,-69.7241157188086,0.));
#65706=CARTESIAN_POINT('Ctrl Pts',(20.5578799284897,-69.7440589303511,0.));
#65707=CARTESIAN_POINT('Ctrl Pts',(20.5734386982781,-69.7640185983641,0.));
#65708=CARTESIAN_POINT('Ctrl Pts',(20.5890406948808,-69.7839946063942,0.));
#65709=CARTESIAN_POINT('Ctrl Pts',(20.6046858968305,-69.8039868384382,0.));
#65710=CARTESIAN_POINT('Ctrl Pts',(20.6203742826565,-69.8239951789402,0.));
#65711=CARTESIAN_POINT('Ctrl Pts',(20.6361058308812,-69.8440195127874,0.));
#65712=CARTESIAN_POINT('Ctrl Pts',(20.6518805200131,-69.8640597253058,0.));
#65713=CARTESIAN_POINT('Ctrl Pts',(20.6676983285542,-69.884115702258,0.));
#65714=CARTESIAN_POINT('Ctrl Pts',(20.683559235003,-69.9041873298416,0.));
#65715=CARTESIAN_POINT('Ctrl Pts',(20.6994632178551,-69.9242744946854,0.));
#65716=CARTESIAN_POINT('Ctrl Pts',(20.7154102555996,-69.9443770838444,0.));
#65717=CARTESIAN_POINT('Ctrl Pts',(20.7314003267118,-69.9644949847929,0.));
#65718=CARTESIAN_POINT('Ctrl Pts',(20.7474334096581,-69.9846280854254,0.));
#65719=CARTESIAN_POINT('Ctrl Pts',(20.7635094829016,-70.0047762740569,0.));
#65720=CARTESIAN_POINT('Ctrl Pts',(20.7796285249022,-70.0249394394221,0.));
#65721=CARTESIAN_POINT('Ctrl Pts',(20.7957905141155,-70.0451174706739,0.));
#65722=CARTESIAN_POINT('Ctrl Pts',(20.8119954289845,-70.0653102573798,0.));
#65723=CARTESIAN_POINT('Ctrl Pts',(20.8282432479425,-70.0855176895185,0.));
#65724=CARTESIAN_POINT('Ctrl Pts',(20.8445339494184,-70.1057396574741,0.));
#65725=CARTESIAN_POINT('Ctrl Pts',(20.8608675118377,-70.1259760520306,0.));
#65726=CARTESIAN_POINT('Ctrl Pts',(20.8772439136206,-70.1462267643649,0.));
#65727=CARTESIAN_POINT('Ctrl Pts',(20.893663133175,-70.1664916860366,0.));
#65728=CARTESIAN_POINT('Ctrl Pts',(20.9101251488948,-70.1867707089866,0.));
#65729=CARTESIAN_POINT('Ctrl Pts',(20.9266299391687,-70.2070637255469,0.));
#65730=CARTESIAN_POINT('Ctrl Pts',(20.9431774823833,-70.2273706284479,0.));
#65731=CARTESIAN_POINT('Ctrl Pts',(20.9597677569227,-70.2476913108242,0.));
#65732=CARTESIAN_POINT('Ctrl Pts',(20.9764007411648,-70.2680256662215,0.));
#65733=CARTESIAN_POINT('Ctrl Pts',(20.993076413477,-70.2883735885971,0.));
#65734=CARTESIAN_POINT('Ctrl Pts',(21.0097947522212,-70.3087349722959,0.));
#65735=CARTESIAN_POINT('Ctrl Pts',(21.0265557357544,-70.3291097120293,0.));
#65736=CARTESIAN_POINT('Ctrl Pts',(21.0433593424265,-70.3494977028497,0.));
#65737=CARTESIAN_POINT('Ctrl Pts',(21.0602055505751,-70.3698988401291,0.));
#65738=CARTESIAN_POINT('Ctrl Pts',(21.0770943385145,-70.3903130195279,0.));
#65739=CARTESIAN_POINT('Ctrl Pts',(21.0940256845477,-70.4107401370403,0.));
#65740=CARTESIAN_POINT('Ctrl Pts',(21.110999566975,-70.4311800890411,0.));
#65741=CARTESIAN_POINT('Ctrl Pts',(21.1280159641003,-70.4516327723349,0.));
#65742=CARTESIAN_POINT('Ctrl Pts',(21.1450748542334,-70.4720980841934,0.));
#65743=CARTESIAN_POINT('Ctrl Pts',(21.1621762156894,-70.4925759224208,0.));
#65744=CARTESIAN_POINT('Ctrl Pts',(21.1793200267843,-70.5130661852946,0.));
#65745=CARTESIAN_POINT('Ctrl Pts',(21.1965062658295,-70.5335687714422,0.));
#65746=CARTESIAN_POINT('Ctrl Pts',(21.2137349111207,-70.5540835797281,0.));
#65747=CARTESIAN_POINT('Ctrl Pts',(21.2310059409265,-70.5746105091503,0.));
#65748=CARTESIAN_POINT('Ctrl Pts',(21.2483193334676,-70.5951494586961,0.));
#65749=CARTESIAN_POINT('Ctrl Pts',(21.2656750669129,-70.6157003273326,0.));
#65750=CARTESIAN_POINT('Ctrl Pts',(21.2830731194187,-70.6362630143062,0.));
#65751=CARTESIAN_POINT('Ctrl Pts',(21.3005134691563,-70.6568374193786,0.));
#65752=CARTESIAN_POINT('Ctrl Pts',(21.3179960943388,-70.6774234430899,0.));
#65753=CARTESIAN_POINT('Ctrl Pts',(21.3355209732438,-70.6980209870032,0.));
#65754=CARTESIAN_POINT('Ctrl Pts',(21.353088084234,-70.7186299539698,0.));
#65755=CARTESIAN_POINT('Ctrl Pts',(21.3706974057028,-70.7392502475438,0.));
#65756=CARTESIAN_POINT('Ctrl Pts',(21.3883489160187,-70.7598817714078,0.));
#65757=CARTESIAN_POINT('Ctrl Pts',(21.4060425934594,-70.780524428744,0.));
#65758=CARTESIAN_POINT('Ctrl Pts',(21.4237784161592,-70.8011781217409,0.));
#65759=CARTESIAN_POINT('Ctrl Pts',(21.4415563620127,-70.8218427507545,0.));
#65760=CARTESIAN_POINT('Ctrl Pts',(21.4593764087492,-70.84251821499,0.));
#65761=CARTESIAN_POINT('Ctrl Pts',(21.4772385340978,-70.8632044140166,0.));
#65762=CARTESIAN_POINT('Ctrl Pts',(21.4951427159272,-70.8839012490903,0.));
#65763=CARTESIAN_POINT('Ctrl Pts',(21.5130889323766,-70.9046086244123,0.));
#65764=CARTESIAN_POINT('Ctrl Pts',(21.5310771620209,-70.9253264487576,0.));
#65765=CARTESIAN_POINT('Ctrl Pts',(21.549107383907,-70.9460546358597,0.));
#65766=CARTESIAN_POINT('Ctrl Pts',(21.5645987555282,-70.9638315189647,0.));
#65767=CARTESIAN_POINT('Ctrl Pts',(21.576498336635,-70.9774662112376,0.));
#65768=CARTESIAN_POINT('Ctrl Pts',(21.584787543316,-70.9869541807808,0.));
#65769=CARTESIAN_POINT('Ctrl Pts',(21.5894540925368,-70.9922924595081,0.));
#65770=CARTESIAN_POINT('Ctrl Pts',(21.59049199348,-70.9934796068777,0.));
#65771=CARTESIAN_POINT('',(18.9407177820968,-67.3887914263118,12.));
#65772=CARTESIAN_POINT('',(18.9407177820968,-67.3887914263118,0.));
#65773=CARTESIAN_POINT('Ctrl Pts',(21.59049199348,-70.9934796068777,12.));
#65774=CARTESIAN_POINT('Ctrl Pts',(21.5894540925368,-70.9922924595081,12.));
#65775=CARTESIAN_POINT('Ctrl Pts',(21.584787543316,-70.9869541807808,12.));
#65776=CARTESIAN_POINT('Ctrl Pts',(21.576498336635,-70.9774662112376,12.));
#65777=CARTESIAN_POINT('Ctrl Pts',(21.5645987555282,-70.9638315189647,12.));
#65778=CARTESIAN_POINT('Ctrl Pts',(21.549107383907,-70.9460546358597,12.));
#65779=CARTESIAN_POINT('Ctrl Pts',(21.5310771620209,-70.9253264487576,12.));
#65780=CARTESIAN_POINT('Ctrl Pts',(21.5130889323766,-70.9046086244123,12.));
#65781=CARTESIAN_POINT('Ctrl Pts',(21.4951427159272,-70.8839012490903,12.));
#65782=CARTESIAN_POINT('Ctrl Pts',(21.4772385340978,-70.8632044140166,12.));
#65783=CARTESIAN_POINT('Ctrl Pts',(21.4593764087492,-70.84251821499,12.));
#65784=CARTESIAN_POINT('Ctrl Pts',(21.4415563620127,-70.8218427507545,12.));
#65785=CARTESIAN_POINT('Ctrl Pts',(21.4237784161592,-70.8011781217409,12.));
#65786=CARTESIAN_POINT('Ctrl Pts',(21.4060425934594,-70.780524428744,12.));
#65787=CARTESIAN_POINT('Ctrl Pts',(21.3883489160187,-70.7598817714078,12.));
#65788=CARTESIAN_POINT('Ctrl Pts',(21.3706974057028,-70.7392502475438,12.));
#65789=CARTESIAN_POINT('Ctrl Pts',(21.353088084234,-70.7186299539698,12.));
#65790=CARTESIAN_POINT('Ctrl Pts',(21.3355209732438,-70.6980209870032,12.));
#65791=CARTESIAN_POINT('Ctrl Pts',(21.3179960943388,-70.6774234430899,12.));
#65792=CARTESIAN_POINT('Ctrl Pts',(21.3005134691563,-70.6568374193786,12.));
#65793=CARTESIAN_POINT('Ctrl Pts',(21.2830731194187,-70.6362630143062,12.));
#65794=CARTESIAN_POINT('Ctrl Pts',(21.2656750669129,-70.6157003273326,12.));
#65795=CARTESIAN_POINT('Ctrl Pts',(21.2483193334676,-70.5951494586961,12.));
#65796=CARTESIAN_POINT('Ctrl Pts',(21.2310059409265,-70.5746105091503,12.));
#65797=CARTESIAN_POINT('Ctrl Pts',(21.2137349111207,-70.5540835797281,12.));
#65798=CARTESIAN_POINT('Ctrl Pts',(21.1965062658295,-70.5335687714422,12.));
#65799=CARTESIAN_POINT('Ctrl Pts',(21.1793200267843,-70.5130661852946,12.));
#65800=CARTESIAN_POINT('Ctrl Pts',(21.1621762156894,-70.4925759224208,12.));
#65801=CARTESIAN_POINT('Ctrl Pts',(21.1450748542334,-70.4720980841934,12.));
#65802=CARTESIAN_POINT('Ctrl Pts',(21.1280159641003,-70.4516327723349,12.));
#65803=CARTESIAN_POINT('Ctrl Pts',(21.110999566975,-70.4311800890411,12.));
#65804=CARTESIAN_POINT('Ctrl Pts',(21.0940256845477,-70.4107401370403,12.));
#65805=CARTESIAN_POINT('Ctrl Pts',(21.0770943385145,-70.3903130195279,12.));
#65806=CARTESIAN_POINT('Ctrl Pts',(21.0602055505751,-70.3698988401291,12.));
#65807=CARTESIAN_POINT('Ctrl Pts',(21.0433593424265,-70.3494977028497,12.));
#65808=CARTESIAN_POINT('Ctrl Pts',(21.0265557357544,-70.3291097120293,12.));
#65809=CARTESIAN_POINT('Ctrl Pts',(21.0097947522212,-70.3087349722959,12.));
#65810=CARTESIAN_POINT('Ctrl Pts',(20.993076413477,-70.2883735885971,12.));
#65811=CARTESIAN_POINT('Ctrl Pts',(20.9764007411648,-70.2680256662215,12.));
#65812=CARTESIAN_POINT('Ctrl Pts',(20.9597677569227,-70.2476913108242,12.));
#65813=CARTESIAN_POINT('Ctrl Pts',(20.9431774823833,-70.2273706284479,12.));
#65814=CARTESIAN_POINT('Ctrl Pts',(20.9266299391687,-70.2070637255469,12.));
#65815=CARTESIAN_POINT('Ctrl Pts',(20.9101251488948,-70.1867707089866,12.));
#65816=CARTESIAN_POINT('Ctrl Pts',(20.893663133175,-70.1664916860366,12.));
#65817=CARTESIAN_POINT('Ctrl Pts',(20.8772439136206,-70.1462267643649,12.));
#65818=CARTESIAN_POINT('Ctrl Pts',(20.8608675118377,-70.1259760520306,12.));
#65819=CARTESIAN_POINT('Ctrl Pts',(20.8445339494184,-70.1057396574741,12.));
#65820=CARTESIAN_POINT('Ctrl Pts',(20.8282432479425,-70.0855176895185,12.));
#65821=CARTESIAN_POINT('Ctrl Pts',(20.8119954289845,-70.0653102573798,12.));
#65822=CARTESIAN_POINT('Ctrl Pts',(20.7957905141155,-70.0451174706739,12.));
#65823=CARTESIAN_POINT('Ctrl Pts',(20.7796285249022,-70.0249394394221,12.));
#65824=CARTESIAN_POINT('Ctrl Pts',(20.7635094829016,-70.0047762740569,12.));
#65825=CARTESIAN_POINT('Ctrl Pts',(20.7474334096581,-69.9846280854254,12.));
#65826=CARTESIAN_POINT('Ctrl Pts',(20.7314003267118,-69.9644949847929,12.));
#65827=CARTESIAN_POINT('Ctrl Pts',(20.7154102555996,-69.9443770838444,12.));
#65828=CARTESIAN_POINT('Ctrl Pts',(20.6994632178551,-69.9242744946854,12.));
#65829=CARTESIAN_POINT('Ctrl Pts',(20.683559235003,-69.9041873298416,12.));
#65830=CARTESIAN_POINT('Ctrl Pts',(20.6676983285542,-69.884115702258,12.));
#65831=CARTESIAN_POINT('Ctrl Pts',(20.6518805200131,-69.8640597253058,12.));
#65832=CARTESIAN_POINT('Ctrl Pts',(20.6361058308812,-69.8440195127874,12.));
#65833=CARTESIAN_POINT('Ctrl Pts',(20.6203742826565,-69.8239951789402,12.));
#65834=CARTESIAN_POINT('Ctrl Pts',(20.6046858968305,-69.8039868384382,12.));
#65835=CARTESIAN_POINT('Ctrl Pts',(20.5890406948808,-69.7839946063942,12.));
#65836=CARTESIAN_POINT('Ctrl Pts',(20.5734386982781,-69.7640185983641,12.));
#65837=CARTESIAN_POINT('Ctrl Pts',(20.5578799284897,-69.7440589303511,12.));
#65838=CARTESIAN_POINT('Ctrl Pts',(20.5423644069799,-69.7241157188086,12.));
#65839=CARTESIAN_POINT('Ctrl Pts',(20.5268921552075,-69.7041890806421,12.));
#65840=CARTESIAN_POINT('Ctrl Pts',(20.511463194618,-69.6842791332102,12.));
#65841=CARTESIAN_POINT('Ctrl Pts',(20.4960775466486,-69.6643859943291,12.));
#65842=CARTESIAN_POINT('Ctrl Pts',(20.4807352327335,-69.6445097822778,12.));
#65843=CARTESIAN_POINT('Ctrl Pts',(20.4654362743036,-69.6246506158009,12.));
#65844=CARTESIAN_POINT('Ctrl Pts',(20.4501806927854,-69.6048086141122,12.));
#65845=CARTESIAN_POINT('Ctrl Pts',(20.4349685095928,-69.5849838968944,12.));
#65846=CARTESIAN_POINT('Ctrl Pts',(20.4197997461305,-69.565176584305,12.));
#65847=CARTESIAN_POINT('Ctrl Pts',(20.4046744238002,-69.5453867969815,12.));
#65848=CARTESIAN_POINT('Ctrl Pts',(20.3895925640006,-69.5256146560444,12.));
#65849=CARTESIAN_POINT('Ctrl Pts',(20.3745541881266,-69.5058602831004,12.));
#65850=CARTESIAN_POINT('Ctrl Pts',(20.3595593175619,-69.4861238002433,12.));
#65851=CARTESIAN_POINT('Ctrl Pts',(20.3446079736798,-69.4664053300579,12.));
#65852=CARTESIAN_POINT('Ctrl Pts',(20.3297001778505,-69.4467049956257,12.));
#65853=CARTESIAN_POINT('Ctrl Pts',(20.3148359514414,-69.4270229205296,12.));
#65854=CARTESIAN_POINT('Ctrl Pts',(20.3000153158167,-69.4073592288562,12.));
#65855=CARTESIAN_POINT('Ctrl Pts',(20.2852382923299,-69.3877140451975,12.));
#65856=CARTESIAN_POINT('Ctrl Pts',(20.270504902324,-69.3680874946548,12.));
#65857=CARTESIAN_POINT('Ctrl Pts',(20.255815167139,-69.3484797028454,12.));
#65858=CARTESIAN_POINT('Ctrl Pts',(20.2411691081122,-69.3288907959065,12.));
#65859=CARTESIAN_POINT('Ctrl Pts',(20.2265667465783,-69.3093209004986,12.));
#65860=CARTESIAN_POINT('Ctrl Pts',(20.2120081038621,-69.2897701438066,12.));
#65861=CARTESIAN_POINT('Ctrl Pts',(20.1974932012775,-69.2702386535432,12.));
#65862=CARTESIAN_POINT('Ctrl Pts',(20.183022060135,-69.2507265579562,12.));
#65863=CARTESIAN_POINT('Ctrl Pts',(20.1685947017433,-69.2312339858337,12.));
#65864=CARTESIAN_POINT('Ctrl Pts',(20.1542111474086,-69.2117610665073,12.));
#65865=CARTESIAN_POINT('Ctrl Pts',(20.1398714184278,-69.1923079298534,12.));
#65866=CARTESIAN_POINT('Ctrl Pts',(20.125575536087,-69.172874706296,12.));
#65867=CARTESIAN_POINT('Ctrl Pts',(20.1113235216693,-69.1534615268153,12.));
#65868=CARTESIAN_POINT('Ctrl Pts',(20.0971153964557,-69.1340685229516,12.));
#65869=CARTESIAN_POINT('Ctrl Pts',(20.082951181725,-69.1146958268104,12.));
#65870=CARTESIAN_POINT('Ctrl Pts',(20.0688308987478,-69.0953435710634,12.));
#65871=CARTESIAN_POINT('Ctrl Pts',(20.0547545687839,-69.0760118889525,12.));
#65872=CARTESIAN_POINT('Ctrl Pts',(20.0407222130902,-69.0567009142968,12.));
#65873=CARTESIAN_POINT('Ctrl Pts',(20.026733852922,-69.0374107814977,12.));
#65874=CARTESIAN_POINT('Ctrl Pts',(20.0127895095326,-69.0181416255433,12.));
#65875=CARTESIAN_POINT('Ctrl Pts',(19.9988892041671,-68.9988935820101,12.));
#65876=CARTESIAN_POINT('Ctrl Pts',(19.9850329580599,-68.9796667870667,12.));
#65877=CARTESIAN_POINT('Ctrl Pts',(19.9712207924436,-68.960461377483,12.));
#65878=CARTESIAN_POINT('Ctrl Pts',(19.9574527285492,-68.9412774906346,12.));
#65879=CARTESIAN_POINT('Ctrl Pts',(19.9437287876063,-68.9221152645086,12.));
#65880=CARTESIAN_POINT('Ctrl Pts',(19.9300489908364,-68.902974837704,12.));
#65881=CARTESIAN_POINT('Ctrl Pts',(19.9164133594512,-68.8838563494356,12.));
#65882=CARTESIAN_POINT('Ctrl Pts',(19.9028219146606,-68.8647599395437,12.));
#65883=CARTESIAN_POINT('Ctrl Pts',(19.8892746776733,-68.8456857484988,12.));
#65884=CARTESIAN_POINT('Ctrl Pts',(19.8757716696968,-68.8266339174068,12.));
#65885=CARTESIAN_POINT('Ctrl Pts',(19.8623129119304,-68.8076045880102,12.));
#65886=CARTESIAN_POINT('Ctrl Pts',(19.8488984255641,-68.7885979026927,12.));
#65887=CARTESIAN_POINT('Ctrl Pts',(19.835528231787,-68.7696140044892,12.));
#65888=CARTESIAN_POINT('Ctrl Pts',(19.8222023517874,-68.7506530370918,12.));
#65889=CARTESIAN_POINT('Ctrl Pts',(19.8089208067532,-68.7317151448557,12.));
#65890=CARTESIAN_POINT('Ctrl Pts',(19.795683617864,-68.7128004727998,12.));
#65891=CARTESIAN_POINT('Ctrl Pts',(19.7824908062913,-68.6939091666111,12.));
#65892=CARTESIAN_POINT('Ctrl Pts',(19.7693423932058,-68.6750413726547,12.));
#65893=CARTESIAN_POINT('Ctrl Pts',(19.7562383997781,-68.6561972379793,12.));
#65894=CARTESIAN_POINT('Ctrl Pts',(19.7431788471775,-68.6373769103224,12.));
#65895=CARTESIAN_POINT('Ctrl Pts',(19.7301637565652,-68.6185805381126,12.));
#65896=CARTESIAN_POINT('Ctrl Pts',(19.7171931490956,-68.5998082704766,12.));
#65897=CARTESIAN_POINT('Ctrl Pts',(19.7042670459237,-68.581060257249,12.));
#65898=CARTESIAN_POINT('Ctrl Pts',(19.6913854682046,-68.5623366489779,12.));
#65899=CARTESIAN_POINT('Ctrl Pts',(19.6785484370926,-68.5436375969311,12.));
#65900=CARTESIAN_POINT('Ctrl Pts',(19.6657559737336,-68.5249632530979,12.));
#65901=CARTESIAN_POINT('Ctrl Pts',(19.6530080992686,-68.5063137701971,12.));
#65902=CARTESIAN_POINT('Ctrl Pts',(19.6403048348395,-68.4876893016856,12.));
#65903=CARTESIAN_POINT('Ctrl Pts',(19.6276462015888,-68.4690900017632,12.));
#65904=CARTESIAN_POINT('Ctrl Pts',(19.6150322206577,-68.4505160253778,12.));
#65905=CARTESIAN_POINT('Ctrl Pts',(19.6024629131784,-68.4319675282275,12.));
#65906=CARTESIAN_POINT('Ctrl Pts',(19.5899383002802,-68.4134446667696,12.));
#65907=CARTESIAN_POINT('Ctrl Pts',(19.5774584030937,-68.3949475982335,12.));
#65908=CARTESIAN_POINT('Ctrl Pts',(19.5650232427515,-68.3764764806287,12.));
#65909=CARTESIAN_POINT('Ctrl Pts',(19.5526328403852,-68.3580314727523,12.));
#65910=CARTESIAN_POINT('Ctrl Pts',(19.540287217119,-68.3396127341938,12.));
#65911=CARTESIAN_POINT('Ctrl Pts',(19.5279863940773,-68.3212204253417,12.));
#65912=CARTESIAN_POINT('Ctrl Pts',(19.5157303923856,-68.3028547073865,12.));
#65913=CARTESIAN_POINT('Ctrl Pts',(19.5035192331705,-68.2845157423233,12.));
#65914=CARTESIAN_POINT('Ctrl Pts',(19.4913529375543,-68.2662036929526,12.));
#65915=CARTESIAN_POINT('Ctrl Pts',(19.4792315266501,-68.2479187228803,12.));
#65916=CARTESIAN_POINT('Ctrl Pts',(19.467155021572,-68.2296609965448,12.));
#65917=CARTESIAN_POINT('Ctrl Pts',(19.455123443438,-68.2114306792358,12.));
#65918=CARTESIAN_POINT('Ctrl Pts',(19.4431368133719,-68.1932279371127,12.));
#65919=CARTESIAN_POINT('Ctrl Pts',(19.4311951524983,-68.1750529372232,12.));
#65920=CARTESIAN_POINT('Ctrl Pts',(19.4192984819418,-68.1569058475054,12.));
#65921=CARTESIAN_POINT('Ctrl Pts',(19.4074468228299,-68.1387868367691,12.));
#65922=CARTESIAN_POINT('Ctrl Pts',(19.3956401962894,-68.1206960746769,12.));
#65923=CARTESIAN_POINT('Ctrl Pts',(19.3838786234421,-68.1026337317285,12.));
#65924=CARTESIAN_POINT('Ctrl Pts',(19.3721621253912,-68.0845999792247,12.));
#65925=CARTESIAN_POINT('Ctrl Pts',(19.3604907232313,-68.0665949893195,12.));
#65926=CARTESIAN_POINT('Ctrl Pts',(19.3488644380641,-68.0486189351011,12.));
#65927=CARTESIAN_POINT('Ctrl Pts',(19.3372832910076,-68.0306719906636,12.));
#65928=CARTESIAN_POINT('Ctrl Pts',(19.3257473032034,-68.0127543311776,12.));
#65929=CARTESIAN_POINT('Ctrl Pts',(19.3142564958202,-67.9948661329617,12.));
#65930=CARTESIAN_POINT('Ctrl Pts',(19.302810890038,-67.9770075733485,12.));
#65931=CARTESIAN_POINT('Ctrl Pts',(19.2914105070286,-67.9591788305394,12.));
#65932=CARTESIAN_POINT('Ctrl Pts',(19.280055367936,-67.9413800834793,12.));
#65933=CARTESIAN_POINT('Ctrl Pts',(19.2687454938442,-67.9236115116758,12.));
#65934=CARTESIAN_POINT('Ctrl Pts',(19.2574809057696,-67.9058732951788,12.));
#65935=CARTESIAN_POINT('Ctrl Pts',(19.2462616247279,-67.8881656149955,12.));
#65936=CARTESIAN_POINT('Ctrl Pts',(19.2350876717874,-67.8704886534544,12.));
#65937=CARTESIAN_POINT('Ctrl Pts',(19.2239590681133,-67.8528425945184,12.));
#65938=CARTESIAN_POINT('Ctrl Pts',(19.2128758350345,-67.835227624289,12.));
#65939=CARTESIAN_POINT('Ctrl Pts',(19.201837993993,-67.8176439306621,12.));
#65940=CARTESIAN_POINT('Ctrl Pts',(19.1908455664097,-67.8000917023926,12.));
#65941=CARTESIAN_POINT('Ctrl Pts',(19.1798985735687,-67.7825711283096,12.));
#65942=CARTESIAN_POINT('Ctrl Pts',(19.1689970364949,-67.7650823965127,12.));
#65943=CARTESIAN_POINT('Ctrl Pts',(19.1581409758097,-67.7476256934444,12.));
#65944=CARTESIAN_POINT('Ctrl Pts',(19.1473304119955,-67.7302012056584,12.));
#65945=CARTESIAN_POINT('Ctrl Pts',(19.136565365709,-67.7128091219348,12.));
#65946=CARTESIAN_POINT('Ctrl Pts',(19.1258458580345,-67.6954496350063,12.));
#65947=CARTESIAN_POINT('Ctrl Pts',(19.115171910846,-67.6781229440573,12.));
#65948=CARTESIAN_POINT('Ctrl Pts',(19.1045435468358,-67.6608292549462,12.));
#65949=CARTESIAN_POINT('Ctrl Pts',(19.0939607887501,-67.6435687749841,12.));
#65950=CARTESIAN_POINT('Ctrl Pts',(19.0834236587118,-67.6263417083426,12.));
#65951=CARTESIAN_POINT('Ctrl Pts',(19.072932177628,-67.6091482520534,12.));
#65952=CARTESIAN_POINT('Ctrl Pts',(19.062486364241,-67.5919885896222,12.));
#65953=CARTESIAN_POINT('Ctrl Pts',(19.0520862360395,-67.5748628971964,12.));
#65954=CARTESIAN_POINT('Ctrl Pts',(19.0417318110708,-67.5577713558194,12.));
#65955=CARTESIAN_POINT('Ctrl Pts',(19.0314231093923,-67.540714161288,12.));
#65956=CARTESIAN_POINT('Ctrl Pts',(19.021160154824,-67.5236915360331,12.));
#65957=CARTESIAN_POINT('Ctrl Pts',(19.0109429761306,-67.5067037372317,12.));
#65958=CARTESIAN_POINT('Ctrl Pts',(19.0007716032819,-67.4897510316844,12.));
#65959=CARTESIAN_POINT('Ctrl Pts',(18.9906460638625,-67.472833671964,12.));
#65960=CARTESIAN_POINT('Ctrl Pts',(18.9805663798448,-67.4559518744638,12.));
#65961=CARTESIAN_POINT('Ctrl Pts',(18.970532563171,-67.4391057908418,12.));
#65962=CARTESIAN_POINT('Ctrl Pts',(18.9605446160985,-67.4222955061981,12.));
#65963=CARTESIAN_POINT('Ctrl Pts',(18.9525909517915,-67.4088759497911,12.));
#65964=CARTESIAN_POINT('Ctrl Pts',(18.9466463414299,-67.3988274146651,12.));
#65965=CARTESIAN_POINT('Ctrl Pts',(18.9426924398719,-67.3921355608328,12.));
#65966=CARTESIAN_POINT('Ctrl Pts',(18.9407177820968,-67.3887914263118,12.));
#65967=CARTESIAN_POINT('Ctrl Pts',(23.0342913834072,-70.538251407892,-5.55111512312578E-16));
#65968=CARTESIAN_POINT('Ctrl Pts',(23.0342913834072,-70.538251407892,4.));
#65969=CARTESIAN_POINT('Ctrl Pts',(23.0342913834072,-70.538251407892,8.));
#65970=CARTESIAN_POINT('Ctrl Pts',(23.0342913834072,-70.538251407892,12.));
#65971=CARTESIAN_POINT('Ctrl Pts',(23.0224954570734,-70.6474988907591,-5.55111512312578E-16));
#65972=CARTESIAN_POINT('Ctrl Pts',(23.0224954570734,-70.6474988907591,4.));
#65973=CARTESIAN_POINT('Ctrl Pts',(23.0224954570734,-70.6474988907591,8.00000000000001));
#65974=CARTESIAN_POINT('Ctrl Pts',(23.0224954570734,-70.6474988907591,12.));
#65975=CARTESIAN_POINT('Ctrl Pts',(22.9364730048789,-70.83100071469,-5.55111512312578E-16));
#65976=CARTESIAN_POINT('Ctrl Pts',(22.9364730048789,-70.83100071469,4.));
#65977=CARTESIAN_POINT('Ctrl Pts',(22.9364730048789,-70.83100071469,7.99999999999999));
#65978=CARTESIAN_POINT('Ctrl Pts',(22.9364730048789,-70.83100071469,12.));
#65979=CARTESIAN_POINT('Ctrl Pts',(22.7679558220498,-70.9357242819029,-5.55111512312578E-16));
#65980=CARTESIAN_POINT('Ctrl Pts',(22.7679558220498,-70.9357242819029,4.));
#65981=CARTESIAN_POINT('Ctrl Pts',(22.7679558220498,-70.9357242819029,8.00000000000001));
#65982=CARTESIAN_POINT('Ctrl Pts',(22.7679558220498,-70.9357242819029,12.));
#65983=CARTESIAN_POINT('Ctrl Pts',(22.6894590071812,-70.9608233461354,-5.55111512312578E-16));
#65984=CARTESIAN_POINT('Ctrl Pts',(22.6894590071812,-70.9608233461354,4.));
#65985=CARTESIAN_POINT('Ctrl Pts',(22.6894590071812,-70.9608233461354,8.));
#65986=CARTESIAN_POINT('Ctrl Pts',(22.6894590071812,-70.9608233461354,12.));
#65987=CARTESIAN_POINT('',(23.0342913834072,-70.538251407892,2.77555756156289E-16));
#65988=CARTESIAN_POINT('',(22.6894590071812,-70.9608233461355,0.));
#65989=CARTESIAN_POINT('Ctrl Pts',(23.0342913834072,-70.538251407892,-1.38777878078145E-16));
#65990=CARTESIAN_POINT('Ctrl Pts',(23.0224954570734,-70.6474988907591,-1.38777878078145E-16));
#65991=CARTESIAN_POINT('Ctrl Pts',(22.9733397701051,-70.7523570758625,-1.38777878078144E-16));
#65992=CARTESIAN_POINT('Ctrl Pts',(22.8972470282357,-70.8314917485681,-1.38777878078145E-16));
#65993=CARTESIAN_POINT('Ctrl Pts',(22.8401774718337,-70.8908427530974,-1.38777878078145E-16));
#65994=CARTESIAN_POINT('Ctrl Pts',(22.7679558220498,-70.9357242819029,-1.38777878078145E-16));
#65995=CARTESIAN_POINT('Ctrl Pts',(22.6894590071812,-70.9608233461354,-1.38777878078145E-16));
#65996=CARTESIAN_POINT('',(22.6894590071812,-70.9608233461355,12.));
#65997=CARTESIAN_POINT('Ctrl Pts',(22.6894590071812,-70.9608233461354,-5.55111512312578E-16));
#65998=CARTESIAN_POINT('Ctrl Pts',(22.6894590071812,-70.9608233461354,4.));
#65999=CARTESIAN_POINT('Ctrl Pts',(22.6894590071812,-70.9608233461354,8.));
#66000=CARTESIAN_POINT('Ctrl Pts',(22.6894590071812,-70.9608233461354,12.));
#66001=CARTESIAN_POINT('',(23.0342913834072,-70.538251407892,12.));
#66002=CARTESIAN_POINT('Ctrl Pts',(22.6894590071812,-70.9608233461354,12.));
#66003=CARTESIAN_POINT('Ctrl Pts',(22.7679558220498,-70.9357242819029,12.));
#66004=CARTESIAN_POINT('Ctrl Pts',(22.8401774718337,-70.8908427530974,12.));
#66005=CARTESIAN_POINT('Ctrl Pts',(22.8972470282357,-70.8314917485681,12.));
#66006=CARTESIAN_POINT('Ctrl Pts',(22.9733397701051,-70.7523570758625,12.));
#66007=CARTESIAN_POINT('Ctrl Pts',(23.0224954570734,-70.6474988907591,12.));
#66008=CARTESIAN_POINT('Ctrl Pts',(23.0342913834072,-70.538251407892,12.));
#66009=CARTESIAN_POINT('Ctrl Pts',(23.0342913834072,-70.538251407892,12.));
#66010=CARTESIAN_POINT('Ctrl Pts',(23.0342913834072,-70.538251407892,8.));
#66011=CARTESIAN_POINT('Ctrl Pts',(23.0342913834072,-70.538251407892,4.));
#66012=CARTESIAN_POINT('Ctrl Pts',(23.0342913834072,-70.538251407892,-5.55111512312578E-16));
#66013=CARTESIAN_POINT('Origin',(1.12812358559725E-10,-3.57465004850839E-10,
0.));
#66014=CARTESIAN_POINT('Origin',(1.12812358559725E-10,-3.57465004850839E-10,
12.));
#66015=CARTESIAN_POINT('Origin',(1.12812358559725E-10,-3.57465004850839E-10,
0.));
#66016=CARTESIAN_POINT('Ctrl Pts',(15.8307637747259,-72.7986051948032,-5.55111512312578E-16));
#66017=CARTESIAN_POINT('Ctrl Pts',(15.8307637747259,-72.7986051948032,4.));
#66018=CARTESIAN_POINT('Ctrl Pts',(15.830763774726,-72.7986051948032,8.));
#66019=CARTESIAN_POINT('Ctrl Pts',(15.830763774726,-72.7986051948032,12.));
#66020=CARTESIAN_POINT('Ctrl Pts',(15.7233907508395,-72.8219545017353,-5.55111512312578E-16));
#66021=CARTESIAN_POINT('Ctrl Pts',(15.7233907508395,-72.8219545017353,4.));
#66022=CARTESIAN_POINT('Ctrl Pts',(15.7233907508395,-72.8219545017353,8.));
#66023=CARTESIAN_POINT('Ctrl Pts',(15.7233907508395,-72.8219545017353,12.));
#66024=CARTESIAN_POINT('Ctrl Pts',(15.522104120072,-72.7983622347336,-5.55111512312578E-16));
#66025=CARTESIAN_POINT('Ctrl Pts',(15.522104120072,-72.7983622347336,4.00000000000001));
#66026=CARTESIAN_POINT('Ctrl Pts',(15.522104120072,-72.7983622347336,7.99999999999999));
#66027=CARTESIAN_POINT('Ctrl Pts',(15.522104120072,-72.7983622347336,12.));
#66028=CARTESIAN_POINT('Ctrl Pts',(15.3694736926916,-72.6715981986661,-5.55111512312578E-16));
#66029=CARTESIAN_POINT('Ctrl Pts',(15.3694736926916,-72.6715981986661,4.));
#66030=CARTESIAN_POINT('Ctrl Pts',(15.3694736926916,-72.6715981986661,8.00000000000001));
#66031=CARTESIAN_POINT('Ctrl Pts',(15.3694736926916,-72.6715981986661,12.));
#66032=CARTESIAN_POINT('Ctrl Pts',(15.3208442077189,-72.6050633494351,-5.55111512312578E-16));
#66033=CARTESIAN_POINT('Ctrl Pts',(15.3208442077189,-72.6050633494351,4.));
#66034=CARTESIAN_POINT('Ctrl Pts',(15.3208442077189,-72.605063349435,8.));
#66035=CARTESIAN_POINT('Ctrl Pts',(15.3208442077189,-72.605063349435,12.));
#66036=CARTESIAN_POINT('',(15.8307637747259,-72.7986051948032,0.));
#66037=CARTESIAN_POINT('',(15.3208442077189,-72.6050633494351,2.77555756156289E-16));
#66038=CARTESIAN_POINT('Ctrl Pts',(15.8307637747259,-72.7986051948032,-2.77555756156289E-16));
#66039=CARTESIAN_POINT('Ctrl Pts',(15.7233907508395,-72.8219545017353,-2.77555756156289E-16));
#66040=CARTESIAN_POINT('Ctrl Pts',(15.6083698189723,-72.8084732063058,-2.77555756156289E-16));
#66041=CARTESIAN_POINT('Ctrl Pts',(15.5092366269867,-72.7613031699568,-2.77555756156289E-16));
#66042=CARTESIAN_POINT('Ctrl Pts',(15.4348867329975,-72.7259256426951,-2.77555756156289E-16));
#66043=CARTESIAN_POINT('Ctrl Pts',(15.3694736926916,-72.6715981986661,-2.7755575615629E-16));
#66044=CARTESIAN_POINT('Ctrl Pts',(15.3208442077189,-72.6050633494351,-2.77555756156289E-16));
#66045=CARTESIAN_POINT('',(15.3208442077188,-72.6050633494351,12.));
#66046=CARTESIAN_POINT('Ctrl Pts',(15.3208442077189,-72.6050633494351,-5.55111512312578E-16));
#66047=CARTESIAN_POINT('Ctrl Pts',(15.3208442077189,-72.6050633494351,4.));
#66048=CARTESIAN_POINT('Ctrl Pts',(15.3208442077189,-72.605063349435,8.));
#66049=CARTESIAN_POINT('Ctrl Pts',(15.3208442077189,-72.605063349435,12.));
#66050=CARTESIAN_POINT('',(15.830763774726,-72.7986051948032,12.));
#66051=CARTESIAN_POINT('Ctrl Pts',(15.3208442077189,-72.605063349435,12.));
#66052=CARTESIAN_POINT('Ctrl Pts',(15.3694736926916,-72.6715981986661,12.));
#66053=CARTESIAN_POINT('Ctrl Pts',(15.4348867329975,-72.725925642695,12.));
#66054=CARTESIAN_POINT('Ctrl Pts',(15.5092366269867,-72.7613031699568,12.));
#66055=CARTESIAN_POINT('Ctrl Pts',(15.6083698189723,-72.8084732063058,12.));
#66056=CARTESIAN_POINT('Ctrl Pts',(15.7233907508395,-72.8219545017353,12.));
#66057=CARTESIAN_POINT('Ctrl Pts',(15.830763774726,-72.7986051948032,12.));
#66058=CARTESIAN_POINT('Ctrl Pts',(15.830763774726,-72.7986051948032,12.));
#66059=CARTESIAN_POINT('Ctrl Pts',(15.830763774726,-72.7986051948032,8.));
#66060=CARTESIAN_POINT('Ctrl Pts',(15.8307637747259,-72.7986051948032,4.));
#66061=CARTESIAN_POINT('Ctrl Pts',(15.8307637747259,-72.7986051948032,-5.55111512312578E-16));
#66062=CARTESIAN_POINT('Ctrl Pts',(12.9953224629497,-68.7831490561748,0.));
#66063=CARTESIAN_POINT('Ctrl Pts',(12.9953224629497,-68.7831490561748,12.));
#66064=CARTESIAN_POINT('Ctrl Pts',(12.9969981460277,-68.7866525680193,0.));
#66065=CARTESIAN_POINT('Ctrl Pts',(12.9969981460277,-68.7866525680193,12.));
#66066=CARTESIAN_POINT('Ctrl Pts',(13.0003537683054,-68.7936635625545,0.));
#66067=CARTESIAN_POINT('Ctrl Pts',(13.0003537683054,-68.7936635625545,12.));
#66068=CARTESIAN_POINT('Ctrl Pts',(13.0053999700875,-68.804191966902,0.));
#66069=CARTESIAN_POINT('Ctrl Pts',(13.0053999700875,-68.804191966902,12.));
#66070=CARTESIAN_POINT('Ctrl Pts',(13.0121537768945,-68.8182536653656,0.));
#66071=CARTESIAN_POINT('Ctrl Pts',(13.0121537768945,-68.8182536653656,12.));
#66072=CARTESIAN_POINT('Ctrl Pts',(13.0206386039691,-68.8358704887468,0.));
#66073=CARTESIAN_POINT('Ctrl Pts',(13.0206386039691,-68.8358704887468,12.));
#66074=CARTESIAN_POINT('Ctrl Pts',(13.0291660060107,-68.8535269726793,0.));
#66075=CARTESIAN_POINT('Ctrl Pts',(13.0291660060107,-68.8535269726793,12.));
#66076=CARTESIAN_POINT('Ctrl Pts',(13.0377359881875,-68.8712230321906,0.));
#66077=CARTESIAN_POINT('Ctrl Pts',(13.0377359881875,-68.8712230321906,12.));
#66078=CARTESIAN_POINT('Ctrl Pts',(13.0463485518206,-68.8889585151585,0.));
#66079=CARTESIAN_POINT('Ctrl Pts',(13.0463485518206,-68.8889585151585,12.));
#66080=CARTESIAN_POINT('Ctrl Pts',(13.0550036938813,-68.9067332040985,0.));
#66081=CARTESIAN_POINT('Ctrl Pts',(13.0550036938813,-68.9067332040985,12.));
#66082=CARTESIAN_POINT('Ctrl Pts',(13.0637014089029,-68.9245468449945,0.));
#66083=CARTESIAN_POINT('Ctrl Pts',(13.0637014089029,-68.9245468449945,12.));
#66084=CARTESIAN_POINT('Ctrl Pts',(13.072441690283,-68.9423991694492,0.));
#66085=CARTESIAN_POINT('Ctrl Pts',(13.072441690283,-68.9423991694492,12.));
#66086=CARTESIAN_POINT('Ctrl Pts',(13.0812245317807,-68.9602899187573,0.));
#66087=CARTESIAN_POINT('Ctrl Pts',(13.0812245317807,-68.9602899187573,12.));
#66088=CARTESIAN_POINT('Ctrl Pts',(13.090049929053,-68.9782188692581,0.));
#66089=CARTESIAN_POINT('Ctrl Pts',(13.090049929053,-68.9782188692581,12.));
#66090=CARTESIAN_POINT('Ctrl Pts',(13.0989178791833,-68.9961858241519,0.));
#66091=CARTESIAN_POINT('Ctrl Pts',(13.0989178791833,-68.9961858241519,12.));
#66092=CARTESIAN_POINT('Ctrl Pts',(13.1078283799722,-69.0141906015113,0.));
#66093=CARTESIAN_POINT('Ctrl Pts',(13.1078283799722,-69.0141906015113,12.));
#66094=CARTESIAN_POINT('Ctrl Pts',(13.1167814293497,-69.0322330243348,0.));
#66095=CARTESIAN_POINT('Ctrl Pts',(13.1167814293497,-69.0322330243348,12.));
#66096=CARTESIAN_POINT('Ctrl Pts',(13.1257770246385,-69.0503129081817,0.));
#66097=CARTESIAN_POINT('Ctrl Pts',(13.1257770246385,-69.0503129081817,12.));
#66098=CARTESIAN_POINT('Ctrl Pts',(13.1348151621834,-69.0684300549477,0.));
#66099=CARTESIAN_POINT('Ctrl Pts',(13.1348151621834,-69.0684300549477,12.));
#66100=CARTESIAN_POINT('Ctrl Pts',(13.1438958377404,-69.0865842593102,0.));
#66101=CARTESIAN_POINT('Ctrl Pts',(13.1438958377404,-69.0865842593102,12.));
#66102=CARTESIAN_POINT('Ctrl Pts',(13.1530190467183,-69.1047753127643,0.));
#66103=CARTESIAN_POINT('Ctrl Pts',(13.1530190467183,-69.1047753127643,12.));
#66104=CARTESIAN_POINT('Ctrl Pts',(13.1621847844528,-69.1230030082573,0.));
#66105=CARTESIAN_POINT('Ctrl Pts',(13.1621847844528,-69.1230030082573,12.));
#66106=CARTESIAN_POINT('Ctrl Pts',(13.1713930465132,-69.1412671454564,0.));
#66107=CARTESIAN_POINT('Ctrl Pts',(13.1713930465132,-69.1412671454564,12.));
#66108=CARTESIAN_POINT('Ctrl Pts',(13.1806438286934,-69.1595675305245,0.));
#66109=CARTESIAN_POINT('Ctrl Pts',(13.1806438286934,-69.1595675305245,12.));
#66110=CARTESIAN_POINT('Ctrl Pts',(13.1899371268683,-69.1779039735996,0.));
#66111=CARTESIAN_POINT('Ctrl Pts',(13.1899371268683,-69.1779039735996,12.));
#66112=CARTESIAN_POINT('Ctrl Pts',(13.1992729368928,-69.1962762870527,0.));
#66113=CARTESIAN_POINT('Ctrl Pts',(13.1992729368928,-69.1962762870527,12.));
#66114=CARTESIAN_POINT('Ctrl Pts',(13.2086512544735,-69.2146842833537,0.));
#66115=CARTESIAN_POINT('Ctrl Pts',(13.2086512544735,-69.2146842833537,12.));
#66116=CARTESIAN_POINT('Ctrl Pts',(13.2180720750594,-69.2331277732861,0.));
#66117=CARTESIAN_POINT('Ctrl Pts',(13.2180720750594,-69.2331277732861,12.));
#66118=CARTESIAN_POINT('Ctrl Pts',(13.2275353939051,-69.2516065668844,0.));
#66119=CARTESIAN_POINT('Ctrl Pts',(13.2275353939051,-69.2516065668844,12.));
#66120=CARTESIAN_POINT('Ctrl Pts',(13.237041206122,-69.2701204742449,0.));
#66121=CARTESIAN_POINT('Ctrl Pts',(13.237041206122,-69.2701204742449,12.));
#66122=CARTESIAN_POINT('Ctrl Pts',(13.2465895067262,-69.2886693063182,0.));
#66123=CARTESIAN_POINT('Ctrl Pts',(13.2465895067262,-69.2886693063182,12.));
#66124=CARTESIAN_POINT('Ctrl Pts',(13.2561802906896,-69.3072528758518,0.));
#66125=CARTESIAN_POINT('Ctrl Pts',(13.2561802906896,-69.3072528758518,12.));
#66126=CARTESIAN_POINT('Ctrl Pts',(13.265813552961,-69.3258709977382,0.));
#66127=CARTESIAN_POINT('Ctrl Pts',(13.265813552961,-69.3258709977382,12.));
#66128=CARTESIAN_POINT('Ctrl Pts',(13.2754892884433,-69.3445234885065,0.));
#66129=CARTESIAN_POINT('Ctrl Pts',(13.2754892884433,-69.3445234885065,12.));
#66130=CARTESIAN_POINT('Ctrl Pts',(13.2852074919765,-69.3632101660066,0.));
#66131=CARTESIAN_POINT('Ctrl Pts',(13.2852074919765,-69.3632101660066,12.));
#66132=CARTESIAN_POINT('Ctrl Pts',(13.2949681583167,-69.3819308490422,0.));
#66133=CARTESIAN_POINT('Ctrl Pts',(13.2949681583167,-69.3819308490422,12.));
#66134=CARTESIAN_POINT('Ctrl Pts',(13.3047712821051,-69.4006853569511,0.));
#66135=CARTESIAN_POINT('Ctrl Pts',(13.3047712821051,-69.4006853569511,12.));
#66136=CARTESIAN_POINT('Ctrl Pts',(13.3146168578743,-69.4194735096265,0.));
#66137=CARTESIAN_POINT('Ctrl Pts',(13.3146168578743,-69.4194735096265,12.));
#66138=CARTESIAN_POINT('Ctrl Pts',(13.3245048800643,-69.4382951276998,0.));
#66139=CARTESIAN_POINT('Ctrl Pts',(13.3245048800643,-69.4382951276998,12.));
#66140=CARTESIAN_POINT('Ctrl Pts',(13.3344353430313,-69.4571500326673,0.));
#66141=CARTESIAN_POINT('Ctrl Pts',(13.3344353430313,-69.4571500326673,12.));
#66142=CARTESIAN_POINT('Ctrl Pts',(13.3444082410543,-69.4760380470365,0.));
#66143=CARTESIAN_POINT('Ctrl Pts',(13.3444082410543,-69.4760380470365,12.));
#66144=CARTESIAN_POINT('Ctrl Pts',(13.3544235683393,-69.4949589944606,0.));
#66145=CARTESIAN_POINT('Ctrl Pts',(13.3544235683393,-69.4949589944606,12.));
#66146=CARTESIAN_POINT('Ctrl Pts',(13.3644813190219,-69.5139126996675,0.));
#66147=CARTESIAN_POINT('Ctrl Pts',(13.3644813190219,-69.5139126996675,12.));
#66148=CARTESIAN_POINT('Ctrl Pts',(13.3745814871664,-69.5328989883885,0.));
#66149=CARTESIAN_POINT('Ctrl Pts',(13.3745814871664,-69.5328989883885,12.));
#66150=CARTESIAN_POINT('Ctrl Pts',(13.3847240667627,-69.5519176872862,0.));
#66151=CARTESIAN_POINT('Ctrl Pts',(13.3847240667627,-69.5519176872862,12.));
#66152=CARTESIAN_POINT('Ctrl Pts',(13.3949090517177,-69.5709686238724,0.));
#66153=CARTESIAN_POINT('Ctrl Pts',(13.3949090517177,-69.5709686238724,12.));
#66154=CARTESIAN_POINT('Ctrl Pts',(13.4051364358499,-69.5900516264553,0.));
#66155=CARTESIAN_POINT('Ctrl Pts',(13.4051364358499,-69.5900516264553,12.));
#66156=CARTESIAN_POINT('Ctrl Pts',(13.4154062129002,-69.6091665241765,0.));
#66157=CARTESIAN_POINT('Ctrl Pts',(13.4154062129002,-69.6091665241765,12.));
#66158=CARTESIAN_POINT('Ctrl Pts',(13.4257183765341,-69.6283131470273,0.));
#66159=CARTESIAN_POINT('Ctrl Pts',(13.4257183765341,-69.6283131470273,12.));
#66160=CARTESIAN_POINT('Ctrl Pts',(13.4360729203442,-69.6474913258675,0.));
#66161=CARTESIAN_POINT('Ctrl Pts',(13.4360729203442,-69.6474913258675,12.));
#66162=CARTESIAN_POINT('Ctrl Pts',(13.4464698378453,-69.666700892444,0.));
#66163=CARTESIAN_POINT('Ctrl Pts',(13.4464698378453,-69.666700892444,12.));
#66164=CARTESIAN_POINT('Ctrl Pts',(13.456909122476,-69.6859416793886,0.));
#66165=CARTESIAN_POINT('Ctrl Pts',(13.456909122476,-69.6859416793886,12.));
#66166=CARTESIAN_POINT('Ctrl Pts',(13.4673907676044,-69.7052135201998,0.));
#66167=CARTESIAN_POINT('Ctrl Pts',(13.4673907676044,-69.7052135201998,12.));
#66168=CARTESIAN_POINT('Ctrl Pts',(13.4779147665285,-69.724516249225,0.));
#66169=CARTESIAN_POINT('Ctrl Pts',(13.4779147665285,-69.724516249225,12.));
#66170=CARTESIAN_POINT('Ctrl Pts',(13.4884811124748,-69.7438497016406,0.));
#66171=CARTESIAN_POINT('Ctrl Pts',(13.4884811124748,-69.7438497016406,12.));
#66172=CARTESIAN_POINT('Ctrl Pts',(13.4990897985904,-69.7632137134249,0.));
#66173=CARTESIAN_POINT('Ctrl Pts',(13.4990897985904,-69.7632137134249,12.));
#66174=CARTESIAN_POINT('Ctrl Pts',(13.5097408179479,-69.7826081213576,0.));
#66175=CARTESIAN_POINT('Ctrl Pts',(13.5097408179479,-69.7826081213576,12.));
#66176=CARTESIAN_POINT('Ctrl Pts',(13.5204341635507,-69.8020327630205,0.));
#66177=CARTESIAN_POINT('Ctrl Pts',(13.5204341635507,-69.8020327630205,12.));
#66178=CARTESIAN_POINT('Ctrl Pts',(13.5311698283339,-69.8214874767944,0.));
#66179=CARTESIAN_POINT('Ctrl Pts',(13.5311698283339,-69.8214874767944,12.));
#66180=CARTESIAN_POINT('Ctrl Pts',(13.5419478051625,-69.840972101856,0.));
#66181=CARTESIAN_POINT('Ctrl Pts',(13.5419478051625,-69.840972101856,12.));
#66182=CARTESIAN_POINT('Ctrl Pts',(13.5527680868255,-69.8604864781706,0.));
#66183=CARTESIAN_POINT('Ctrl Pts',(13.5527680868255,-69.8604864781706,12.));
#66184=CARTESIAN_POINT('Ctrl Pts',(13.5636306660421,-69.8800304464882,0.));
#66185=CARTESIAN_POINT('Ctrl Pts',(13.5636306660421,-69.8800304464882,12.));
#66186=CARTESIAN_POINT('Ctrl Pts',(13.5745355354656,-69.8996038483361,0.));
#66187=CARTESIAN_POINT('Ctrl Pts',(13.5745355354656,-69.8996038483361,12.));
#66188=CARTESIAN_POINT('Ctrl Pts',(13.5854826876834,-69.9192065260108,0.));
#66189=CARTESIAN_POINT('Ctrl Pts',(13.5854826876834,-69.9192065260108,12.));
#66190=CARTESIAN_POINT('Ctrl Pts',(13.5964721152135,-69.9388383225648,0.));
#66191=CARTESIAN_POINT('Ctrl Pts',(13.5964721152135,-69.9388383225648,12.));
#66192=CARTESIAN_POINT('Ctrl Pts',(13.6075038104998,-69.9584990817974,0.));
#66193=CARTESIAN_POINT('Ctrl Pts',(13.6075038104998,-69.9584990817974,12.));
#66194=CARTESIAN_POINT('Ctrl Pts',(13.6185777659198,-69.9781886482527,0.));
#66195=CARTESIAN_POINT('Ctrl Pts',(13.6185777659198,-69.9781886482527,12.));
#66196=CARTESIAN_POINT('Ctrl Pts',(13.6296939737865,-69.9979068672153,0.));
#66197=CARTESIAN_POINT('Ctrl Pts',(13.6296939737865,-69.9979068672153,12.));
#66198=CARTESIAN_POINT('Ctrl Pts',(13.6408524263496,-70.0176535847049,0.));
#66199=CARTESIAN_POINT('Ctrl Pts',(13.6408524263496,-70.0176535847049,12.));
#66200=CARTESIAN_POINT('Ctrl Pts',(13.6520531157907,-70.0374286474677,0.));
#66201=CARTESIAN_POINT('Ctrl Pts',(13.6520531157907,-70.0374286474677,12.));
#66202=CARTESIAN_POINT('Ctrl Pts',(13.6632960342196,-70.0572319029676,0.));
#66203=CARTESIAN_POINT('Ctrl Pts',(13.6632960342196,-70.0572319029676,12.));
#66204=CARTESIAN_POINT('Ctrl Pts',(13.6745811736829,-70.0770631993856,0.));
#66205=CARTESIAN_POINT('Ctrl Pts',(13.6745811736829,-70.0770631993856,12.));
#66206=CARTESIAN_POINT('Ctrl Pts',(13.6859085261653,-70.0969223856136,0.));
#66207=CARTESIAN_POINT('Ctrl Pts',(13.6859085261653,-70.0969223856136,12.));
#66208=CARTESIAN_POINT('Ctrl Pts',(13.6972780835897,-70.1168093112486,0.));
#66209=CARTESIAN_POINT('Ctrl Pts',(13.6972780835897,-70.1168093112486,12.));
#66210=CARTESIAN_POINT('Ctrl Pts',(13.7086898378121,-70.1367238265825,0.));
#66211=CARTESIAN_POINT('Ctrl Pts',(13.7086898378121,-70.1367238265825,12.));
#66212=CARTESIAN_POINT('Ctrl Pts',(13.7201437806199,-70.156665782595,0.));
#66213=CARTESIAN_POINT('Ctrl Pts',(13.7201437806199,-70.156665782595,12.));
#66214=CARTESIAN_POINT('Ctrl Pts',(13.7316399037392,-70.1766350309518,0.));
#66215=CARTESIAN_POINT('Ctrl Pts',(13.7316399037392,-70.1766350309518,12.));
#66216=CARTESIAN_POINT('Ctrl Pts',(13.7431781988364,-70.1966314239995,0.));
#66217=CARTESIAN_POINT('Ctrl Pts',(13.7431781988364,-70.1966314239995,12.));
#66218=CARTESIAN_POINT('Ctrl Pts',(13.754758657518,-70.2166548147604,0.));
#66219=CARTESIAN_POINT('Ctrl Pts',(13.754758657518,-70.2166548147604,12.));
#66220=CARTESIAN_POINT('Ctrl Pts',(13.7663812713243,-70.2367050569215,0.));
#66221=CARTESIAN_POINT('Ctrl Pts',(13.7663812713243,-70.2367050569215,12.));
#66222=CARTESIAN_POINT('Ctrl Pts',(13.7780460317294,-70.2567820048303,0.));
#66223=CARTESIAN_POINT('Ctrl Pts',(13.7780460317294,-70.2567820048303,12.));
#66224=CARTESIAN_POINT('Ctrl Pts',(13.7897529301491,-70.2768855134947,0.));
#66225=CARTESIAN_POINT('Ctrl Pts',(13.7897529301491,-70.2768855134947,12.));
#66226=CARTESIAN_POINT('Ctrl Pts',(13.8015019579414,-70.2970154385774,0.));
#66227=CARTESIAN_POINT('Ctrl Pts',(13.8015019579414,-70.2970154385774,12.));
#66228=CARTESIAN_POINT('Ctrl Pts',(13.8132931064063,-70.3171716363897,0.));
#66229=CARTESIAN_POINT('Ctrl Pts',(13.8132931064063,-70.3171716363897,12.));
#66230=CARTESIAN_POINT('Ctrl Pts',(13.825126366779,-70.3373539638809,0.));
#66231=CARTESIAN_POINT('Ctrl Pts',(13.825126366779,-70.3373539638809,12.));
#66232=CARTESIAN_POINT('Ctrl Pts',(13.8370017302309,-70.3575622786335,0.));
#66233=CARTESIAN_POINT('Ctrl Pts',(13.8370017302309,-70.3575622786335,12.));
#66234=CARTESIAN_POINT('Ctrl Pts',(13.8489191878767,-70.3777964388632,0.));
#66235=CARTESIAN_POINT('Ctrl Pts',(13.8489191878767,-70.3777964388632,12.));
#66236=CARTESIAN_POINT('Ctrl Pts',(13.8608787307751,-70.3980563034133,0.));
#66237=CARTESIAN_POINT('Ctrl Pts',(13.8608787307751,-70.3980563034133,12.));
#66238=CARTESIAN_POINT('Ctrl Pts',(13.8728803499287,-70.4183417317499,0.));
#66239=CARTESIAN_POINT('Ctrl Pts',(13.8728803499287,-70.4183417317499,12.));
#66240=CARTESIAN_POINT('Ctrl Pts',(13.8849240362763,-70.4386525839521,0.));
#66241=CARTESIAN_POINT('Ctrl Pts',(13.8849240362763,-70.4386525839521,12.));
#66242=CARTESIAN_POINT('Ctrl Pts',(13.8970097806953,-70.4589887207073,0.));
#66243=CARTESIAN_POINT('Ctrl Pts',(13.8970097806953,-70.4589887207073,12.));
#66244=CARTESIAN_POINT('Ctrl Pts',(13.9091375740088,-70.4793500033124,0.));
#66245=CARTESIAN_POINT('Ctrl Pts',(13.9091375740088,-70.4793500033124,12.));
#66246=CARTESIAN_POINT('Ctrl Pts',(13.9213074069852,-70.4997362936673,0.));
#66247=CARTESIAN_POINT('Ctrl Pts',(13.9213074069852,-70.4997362936673,12.));
#66248=CARTESIAN_POINT('Ctrl Pts',(13.9335192703388,-70.520147454271,0.));
#66249=CARTESIAN_POINT('Ctrl Pts',(13.9335192703388,-70.520147454271,12.));
#66250=CARTESIAN_POINT('Ctrl Pts',(13.9457731547215,-70.5405833482112,0.));
#66251=CARTESIAN_POINT('Ctrl Pts',(13.9457731547215,-70.5405833482112,12.));
#66252=CARTESIAN_POINT('Ctrl Pts',(13.958069050726,-70.5610438391612,0.));
#66253=CARTESIAN_POINT('Ctrl Pts',(13.958069050726,-70.5610438391612,12.));
#66254=CARTESIAN_POINT('Ctrl Pts',(13.9704069488917,-70.5815287913784,0.));
#66255=CARTESIAN_POINT('Ctrl Pts',(13.9704069488917,-70.5815287913784,12.));
#66256=CARTESIAN_POINT('Ctrl Pts',(13.9827868397057,-70.6020380697004,0.));
#66257=CARTESIAN_POINT('Ctrl Pts',(13.9827868397057,-70.6020380697004,12.));
#66258=CARTESIAN_POINT('Ctrl Pts',(13.9952087136018,-70.6225715395394,0.));
#66259=CARTESIAN_POINT('Ctrl Pts',(13.9952087136018,-70.6225715395394,12.));
#66260=CARTESIAN_POINT('Ctrl Pts',(14.0076725609536,-70.6431290668745,0.));
#66261=CARTESIAN_POINT('Ctrl Pts',(14.0076725609536,-70.6431290668745,12.));
#66262=CARTESIAN_POINT('Ctrl Pts',(14.0201783720769,-70.6637105182484,0.));
#66263=CARTESIAN_POINT('Ctrl Pts',(14.0201783720769,-70.6637105182484,12.));
#66264=CARTESIAN_POINT('Ctrl Pts',(14.0327261372362,-70.6843157607668,0.));
#66265=CARTESIAN_POINT('Ctrl Pts',(14.0327261372362,-70.6843157607668,12.));
#66266=CARTESIAN_POINT('Ctrl Pts',(14.0453158466451,-70.7049446620928,0.));
#66267=CARTESIAN_POINT('Ctrl Pts',(14.0453158466451,-70.7049446620928,12.));
#66268=CARTESIAN_POINT('Ctrl Pts',(14.0579474904657,-70.7255970904436,0.));
#66269=CARTESIAN_POINT('Ctrl Pts',(14.0579474904657,-70.7255970904436,12.));
#66270=CARTESIAN_POINT('Ctrl Pts',(14.0706210588016,-70.7462729145807,0.));
#66271=CARTESIAN_POINT('Ctrl Pts',(14.0706210588016,-70.7462729145807,12.));
#66272=CARTESIAN_POINT('Ctrl Pts',(14.0833365416996,-70.7669720038077,0.));
#66273=CARTESIAN_POINT('Ctrl Pts',(14.0833365416996,-70.7669720038077,12.));
#66274=CARTESIAN_POINT('Ctrl Pts',(14.0960939291569,-70.7876942279697,0.));
#66275=CARTESIAN_POINT('Ctrl Pts',(14.0960939291569,-70.7876942279697,12.));
#66276=CARTESIAN_POINT('Ctrl Pts',(14.1088932111214,-70.8084394574493,0.));
#66277=CARTESIAN_POINT('Ctrl Pts',(14.1088932111214,-70.8084394574493,12.));
#66278=CARTESIAN_POINT('Ctrl Pts',(14.1217343774913,-70.8292075631621,0.));
#66279=CARTESIAN_POINT('Ctrl Pts',(14.1217343774913,-70.8292075631621,12.));
#66280=CARTESIAN_POINT('Ctrl Pts',(14.1346174181078,-70.8499984165489,0.));
#66281=CARTESIAN_POINT('Ctrl Pts',(14.1346174181078,-70.8499984165489,12.));
#66282=CARTESIAN_POINT('Ctrl Pts',(14.1475423227568,-70.8708118895715,0.));
#66283=CARTESIAN_POINT('Ctrl Pts',(14.1475423227568,-70.8708118895715,12.));
#66284=CARTESIAN_POINT('Ctrl Pts',(14.1605090811754,-70.8916478547132,0.));
#66285=CARTESIAN_POINT('Ctrl Pts',(14.1605090811754,-70.8916478547132,12.));
#66286=CARTESIAN_POINT('Ctrl Pts',(14.1735176830533,-70.9125061849745,0.));
#66287=CARTESIAN_POINT('Ctrl Pts',(14.1735176830533,-70.9125061849745,12.));
#66288=CARTESIAN_POINT('Ctrl Pts',(14.186568118032,-70.9333867538704,0.));
#66289=CARTESIAN_POINT('Ctrl Pts',(14.186568118032,-70.9333867538704,12.));
#66290=CARTESIAN_POINT('Ctrl Pts',(14.1996603756982,-70.9542894354216,0.));
#66291=CARTESIAN_POINT('Ctrl Pts',(14.1996603756982,-70.9542894354216,12.));
#66292=CARTESIAN_POINT('Ctrl Pts',(14.2127944455838,-70.9752141041518,0.));
#66293=CARTESIAN_POINT('Ctrl Pts',(14.2127944455838,-70.9752141041518,12.));
#66294=CARTESIAN_POINT('Ctrl Pts',(14.2259703171737,-70.9961606350861,0.));
#66295=CARTESIAN_POINT('Ctrl Pts',(14.2259703171737,-70.9961606350861,12.));
#66296=CARTESIAN_POINT('Ctrl Pts',(14.2391879799061,-71.0171289037488,0.));
#66297=CARTESIAN_POINT('Ctrl Pts',(14.2391879799061,-71.0171289037488,12.));
#66298=CARTESIAN_POINT('Ctrl Pts',(14.2524474231732,-71.0381187861588,0.));
#66299=CARTESIAN_POINT('Ctrl Pts',(14.2524474231732,-71.0381187861588,12.));
#66300=CARTESIAN_POINT('Ctrl Pts',(14.2657486363139,-71.0591301588231,0.));
#66301=CARTESIAN_POINT('Ctrl Pts',(14.2657486363139,-71.0591301588231,12.));
#66302=CARTESIAN_POINT('Ctrl Pts',(14.2790916086133,-71.0801628987332,0.));
#66303=CARTESIAN_POINT('Ctrl Pts',(14.2790916086133,-71.0801628987332,12.));
#66304=CARTESIAN_POINT('Ctrl Pts',(14.2924763293105,-71.1012168833643,0.));
#66305=CARTESIAN_POINT('Ctrl Pts',(14.2924763293105,-71.1012168833643,12.));
#66306=CARTESIAN_POINT('Ctrl Pts',(14.3059027875994,-71.1222919906727,0.));
#66307=CARTESIAN_POINT('Ctrl Pts',(14.3059027875994,-71.1222919906727,12.));
#66308=CARTESIAN_POINT('Ctrl Pts',(14.3193709726294,-71.1433880990929,0.));
#66309=CARTESIAN_POINT('Ctrl Pts',(14.3193709726294,-71.1433880990929,12.));
#66310=CARTESIAN_POINT('Ctrl Pts',(14.3328808734989,-71.1645050875308,0.));
#66311=CARTESIAN_POINT('Ctrl Pts',(14.3328808734989,-71.1645050875308,12.));
#66312=CARTESIAN_POINT('Ctrl Pts',(14.3464324792533,-71.1856428353593,0.));
#66313=CARTESIAN_POINT('Ctrl Pts',(14.3464324792533,-71.1856428353593,12.));
#66314=CARTESIAN_POINT('Ctrl Pts',(14.3600257788924,-71.2068012224174,0.));
#66315=CARTESIAN_POINT('Ctrl Pts',(14.3600257788924,-71.2068012224174,12.));
#66316=CARTESIAN_POINT('Ctrl Pts',(14.3736607613722,-71.2279801290084,0.));
#66317=CARTESIAN_POINT('Ctrl Pts',(14.3736607613722,-71.2279801290084,12.));
#66318=CARTESIAN_POINT('Ctrl Pts',(14.3873374156056,-71.2491794358958,0.));
#66319=CARTESIAN_POINT('Ctrl Pts',(14.3873374156056,-71.2491794358958,12.));
#66320=CARTESIAN_POINT('Ctrl Pts',(14.401055730457,-71.2703990242988,0.));
#66321=CARTESIAN_POINT('Ctrl Pts',(14.401055730457,-71.2703990242988,12.));
#66322=CARTESIAN_POINT('Ctrl Pts',(14.4148156947383,-71.2916387758861,0.));
#66323=CARTESIAN_POINT('Ctrl Pts',(14.4148156947383,-71.2916387758861,12.));
#66324=CARTESIAN_POINT('Ctrl Pts',(14.4286172972166,-71.312898572777,0.));
#66325=CARTESIAN_POINT('Ctrl Pts',(14.4286172972166,-71.312898572777,12.));
#66326=CARTESIAN_POINT('Ctrl Pts',(14.4424605266165,-71.3341782975386,0.));
#66327=CARTESIAN_POINT('Ctrl Pts',(14.4424605266165,-71.3341782975386,12.));
#66328=CARTESIAN_POINT('Ctrl Pts',(14.4563453716204,-71.3554778331835,0.));
#66329=CARTESIAN_POINT('Ctrl Pts',(14.4563453716204,-71.3554778331835,12.));
#66330=CARTESIAN_POINT('Ctrl Pts',(14.4702718208651,-71.376797063165,0.));
#66331=CARTESIAN_POINT('Ctrl Pts',(14.4702718208651,-71.376797063165,12.));
#66332=CARTESIAN_POINT('Ctrl Pts',(14.4842398629355,-71.3981358713723,0.));
#66333=CARTESIAN_POINT('Ctrl Pts',(14.4842398629355,-71.3981358713723,12.));
#66334=CARTESIAN_POINT('Ctrl Pts',(14.4982494863718,-71.4194941421292,0.));
#66335=CARTESIAN_POINT('Ctrl Pts',(14.4982494863718,-71.4194941421292,12.));
#66336=CARTESIAN_POINT('Ctrl Pts',(14.5123006796728,-71.4408717601923,0.));
#66337=CARTESIAN_POINT('Ctrl Pts',(14.5123006796728,-71.4408717601923,12.));
#66338=CARTESIAN_POINT('Ctrl Pts',(14.5263934312969,-71.4622686107475,0.));
#66339=CARTESIAN_POINT('Ctrl Pts',(14.5263934312969,-71.4622686107475,12.));
#66340=CARTESIAN_POINT('Ctrl Pts',(14.540527729659,-71.4836845794048,0.));
#66341=CARTESIAN_POINT('Ctrl Pts',(14.540527729659,-71.4836845794048,12.));
#66342=CARTESIAN_POINT('Ctrl Pts',(14.5547035631233,-71.5051195521909,0.));
#66343=CARTESIAN_POINT('Ctrl Pts',(14.5547035631233,-71.5051195521909,12.));
#66344=CARTESIAN_POINT('Ctrl Pts',(14.5689209200091,-71.5265734155498,0.));
#66345=CARTESIAN_POINT('Ctrl Pts',(14.5689209200091,-71.5265734155498,12.));
#66346=CARTESIAN_POINT('Ctrl Pts',(14.5831797885952,-71.5480460563447,0.));
#66347=CARTESIAN_POINT('Ctrl Pts',(14.5831797885952,-71.5480460563447,12.));
#66348=CARTESIAN_POINT('Ctrl Pts',(14.597480157121,-71.5695373618562,0.));
#66349=CARTESIAN_POINT('Ctrl Pts',(14.597480157121,-71.5695373618562,12.));
#66350=CARTESIAN_POINT('Ctrl Pts',(14.6118220137849,-71.5910472197813,0.));
#66351=CARTESIAN_POINT('Ctrl Pts',(14.6118220137849,-71.5910472197813,12.));
#66352=CARTESIAN_POINT('Ctrl Pts',(14.626205346737,-71.612575518229,0.));
#66353=CARTESIAN_POINT('Ctrl Pts',(14.626205346737,-71.612575518229,12.));
#66354=CARTESIAN_POINT('Ctrl Pts',(14.6406301440814,-71.6341221457169,0.));
#66355=CARTESIAN_POINT('Ctrl Pts',(14.6406301440814,-71.6341221457169,12.));
#66356=CARTESIAN_POINT('Ctrl Pts',(14.6550963938829,-71.6556869911662,0.));
#66357=CARTESIAN_POINT('Ctrl Pts',(14.6550963938829,-71.6556869911662,12.));
#66358=CARTESIAN_POINT('Ctrl Pts',(14.6696040841678,-71.6772699438963,0.));
#66359=CARTESIAN_POINT('Ctrl Pts',(14.6696040841678,-71.6772699438963,12.));
#66360=CARTESIAN_POINT('Ctrl Pts',(14.6841532029232,-71.6988708936172,0.));
#66361=CARTESIAN_POINT('Ctrl Pts',(14.6841532029232,-71.6988708936172,12.));
#66362=CARTESIAN_POINT('Ctrl Pts',(14.69874373809,-71.7204897304194,0.));
#66363=CARTESIAN_POINT('Ctrl Pts',(14.69874373809,-71.7204897304194,12.));
#66364=CARTESIAN_POINT('Ctrl Pts',(14.7133756775625,-71.7421263447719,0.));
#66365=CARTESIAN_POINT('Ctrl Pts',(14.7133756775625,-71.7421263447719,12.));
#66366=CARTESIAN_POINT('Ctrl Pts',(14.7280490091957,-71.7637806275328,0.));
#66367=CARTESIAN_POINT('Ctrl Pts',(14.7280490091957,-71.7637806275328,12.));
#66368=CARTESIAN_POINT('Ctrl Pts',(14.7427637208072,-71.7854524699569,0.));
#66369=CARTESIAN_POINT('Ctrl Pts',(14.7427637208072,-71.7854524699569,12.));
#66370=CARTESIAN_POINT('Ctrl Pts',(14.7575198001776,-71.8071417637017,0.));
#66371=CARTESIAN_POINT('Ctrl Pts',(14.7575198001776,-71.8071417637017,12.));
#66372=CARTESIAN_POINT('Ctrl Pts',(14.7723172350451,-71.8288484008333,0.));
#66373=CARTESIAN_POINT('Ctrl Pts',(14.7723172350451,-71.8288484008333,12.));
#66374=CARTESIAN_POINT('Ctrl Pts',(14.7871560131016,-71.8505722738272,0.));
#66375=CARTESIAN_POINT('Ctrl Pts',(14.7871560131016,-71.8505722738272,12.));
#66376=CARTESIAN_POINT('Ctrl Pts',(14.8020361219998,-71.8723132755446,0.));
#66377=CARTESIAN_POINT('Ctrl Pts',(14.8020361219998,-71.8723132755446,12.));
#66378=CARTESIAN_POINT('Ctrl Pts',(14.8169575493557,-71.8940712992109,0.));
#66379=CARTESIAN_POINT('Ctrl Pts',(14.8169575493557,-71.8940712992109,12.));
#66380=CARTESIAN_POINT('Ctrl Pts',(14.8319202827482,-71.9158462383914,0.));
#66381=CARTESIAN_POINT('Ctrl Pts',(14.8319202827482,-71.9158462383914,12.));
#66382=CARTESIAN_POINT('Ctrl Pts',(14.8469243097162,-71.9376379869678,0.));
#66383=CARTESIAN_POINT('Ctrl Pts',(14.8469243097162,-71.9376379869678,12.));
#66384=CARTESIAN_POINT('Ctrl Pts',(14.8619696177506,-71.9594464391078,0.));
#66385=CARTESIAN_POINT('Ctrl Pts',(14.8619696177506,-71.9594464391078,12.));
#66386=CARTESIAN_POINT('Ctrl Pts',(14.8770561943014,-71.9812714893102,0.));
#66387=CARTESIAN_POINT('Ctrl Pts',(14.8770561943014,-71.9812714893102,12.));
#66388=CARTESIAN_POINT('Ctrl Pts',(14.8921840267832,-72.0031130324529,0.));
#66389=CARTESIAN_POINT('Ctrl Pts',(14.8921840267832,-72.0031130324529,12.));
#66390=CARTESIAN_POINT('Ctrl Pts',(14.9073531025764,-72.0249709638422,0.));
#66391=CARTESIAN_POINT('Ctrl Pts',(14.9073531025764,-72.0249709638422,12.));
#66392=CARTESIAN_POINT('Ctrl Pts',(14.9225634090268,-72.0468451792505,0.));
#66393=CARTESIAN_POINT('Ctrl Pts',(14.9225634090268,-72.0468451792505,12.));
#66394=CARTESIAN_POINT('Ctrl Pts',(14.9378149334388,-72.0687355749806,0.));
#66395=CARTESIAN_POINT('Ctrl Pts',(14.9378149334388,-72.0687355749806,12.));
#66396=CARTESIAN_POINT('Ctrl Pts',(14.9531076630767,-72.0906420478076,0.));
#66397=CARTESIAN_POINT('Ctrl Pts',(14.9531076630767,-72.0906420478076,12.));
#66398=CARTESIAN_POINT('Ctrl Pts',(14.9684415851698,-72.112564494854,0.));
#66399=CARTESIAN_POINT('Ctrl Pts',(14.9684415851698,-72.112564494854,12.));
#66400=CARTESIAN_POINT('Ctrl Pts',(14.9838166869107,-72.1345028134777,0.));
#66401=CARTESIAN_POINT('Ctrl Pts',(14.9838166869107,-72.1345028134777,12.));
#66402=CARTESIAN_POINT('Ctrl Pts',(14.9992329554537,-72.1564569011669,0.));
#66403=CARTESIAN_POINT('Ctrl Pts',(14.9992329554537,-72.1564569011669,12.));
#66404=CARTESIAN_POINT('Ctrl Pts',(15.0146903779062,-72.1784266553953,0.));
#66405=CARTESIAN_POINT('Ctrl Pts',(15.0146903779062,-72.1784266553953,12.));
#66406=CARTESIAN_POINT('Ctrl Pts',(15.0301889413257,-72.2004119736115,0.));
#66407=CARTESIAN_POINT('Ctrl Pts',(15.0301889413257,-72.2004119736115,12.));
#66408=CARTESIAN_POINT('Ctrl Pts',(15.0457286327331,-72.2224127535415,0.));
#66409=CARTESIAN_POINT('Ctrl Pts',(15.0457286327331,-72.2224127535415,12.));
#66410=CARTESIAN_POINT('Ctrl Pts',(15.0613094391189,-72.2444288934262,0.));
#66411=CARTESIAN_POINT('Ctrl Pts',(15.0613094391189,-72.2444288934262,12.));
#66412=CARTESIAN_POINT('Ctrl Pts',(15.0769313474476,-72.2664602922852,0.));
#66413=CARTESIAN_POINT('Ctrl Pts',(15.0769313474476,-72.2664602922852,12.));
#66414=CARTESIAN_POINT('Ctrl Pts',(15.0925943446589,-72.2885068501628,0.));
#66415=CARTESIAN_POINT('Ctrl Pts',(15.0925943446589,-72.2885068501628,12.));
#66416=CARTESIAN_POINT('Ctrl Pts',(15.1082984176649,-72.3105684683944,0.));
#66417=CARTESIAN_POINT('Ctrl Pts',(15.1082984176649,-72.3105684683944,12.));
#66418=CARTESIAN_POINT('Ctrl Pts',(15.124043553347,-72.3326450490177,0.));
#66419=CARTESIAN_POINT('Ctrl Pts',(15.124043553347,-72.3326450490177,12.));
#66420=CARTESIAN_POINT('Ctrl Pts',(15.1398297385506,-72.3547364941969,0.));
#66421=CARTESIAN_POINT('Ctrl Pts',(15.1398297385506,-72.3547364941969,12.));
#66422=CARTESIAN_POINT('Ctrl Pts',(15.1556569600744,-72.376842705589,0.));
#66423=CARTESIAN_POINT('Ctrl Pts',(15.1556569600744,-72.376842705589,12.));
#66424=CARTESIAN_POINT('Ctrl Pts',(15.1715252046606,-72.3989635838492,0.));
#66425=CARTESIAN_POINT('Ctrl Pts',(15.1715252046606,-72.3989635838492,12.));
#66426=CARTESIAN_POINT('Ctrl Pts',(15.1874344589725,-72.421099027786,0.));
#66427=CARTESIAN_POINT('Ctrl Pts',(15.1874344589725,-72.421099027786,12.));
#66428=CARTESIAN_POINT('Ctrl Pts',(15.2033847096091,-72.4432489350471,0.));
#66429=CARTESIAN_POINT('Ctrl Pts',(15.2033847096091,-72.4432489350471,12.));
#66430=CARTESIAN_POINT('Ctrl Pts',(15.2193759431372,-72.4654132036428,0.));
#66431=CARTESIAN_POINT('Ctrl Pts',(15.2193759431372,-72.4654132036428,12.));
#66432=CARTESIAN_POINT('Ctrl Pts',(15.235408146116,-72.4875917332761,0.));
#66433=CARTESIAN_POINT('Ctrl Pts',(15.235408146116,-72.4875917332761,12.));
#66434=CARTESIAN_POINT('Ctrl Pts',(15.2514813051172,-72.5097844266075,0.));
#66435=CARTESIAN_POINT('Ctrl Pts',(15.2514813051172,-72.5097844266075,12.));
#66436=CARTESIAN_POINT('Ctrl Pts',(15.2675954067479,-72.5319911908917,0.));
#66437=CARTESIAN_POINT('Ctrl Pts',(15.2675954067479,-72.5319911908917,12.));
#66438=CARTESIAN_POINT('Ctrl Pts',(15.2837504376535,-72.5542119383642,0.));
#66439=CARTESIAN_POINT('Ctrl Pts',(15.2837504376535,-72.5542119383642,12.));
#66440=CARTESIAN_POINT('Ctrl Pts',(15.299946384466,-72.5764465826224,0.));
#66441=CARTESIAN_POINT('Ctrl Pts',(15.299946384466,-72.5764465826224,12.));
#66442=CARTESIAN_POINT('Ctrl Pts',(15.3161832337594,-72.5986950357677,0.));
#66443=CARTESIAN_POINT('Ctrl Pts',(15.3161832337594,-72.5986950357677,12.));
#66444=CARTESIAN_POINT('Ctrl Pts',(15.3324609719955,-72.6209572051042,0.));
#66445=CARTESIAN_POINT('Ctrl Pts',(15.3324609719955,-72.6209572051042,12.));
#66446=CARTESIAN_POINT('Ctrl Pts',(15.3487795854745,-72.6432329903553,0.));
#66447=CARTESIAN_POINT('Ctrl Pts',(15.3487795854745,-72.6432329903553,12.));
#66448=CARTESIAN_POINT('Ctrl Pts',(15.3651390602665,-72.6655222797801,0.));
#66449=CARTESIAN_POINT('Ctrl Pts',(15.3651390602665,-72.6655222797801,12.));
#66450=CARTESIAN_POINT('Ctrl Pts',(15.3815393822736,-72.687824955772,0.));
#66451=CARTESIAN_POINT('Ctrl Pts',(15.3815393822736,-72.687824955772,12.));
#66452=CARTESIAN_POINT('Ctrl Pts',(15.3979805373174,-72.7101409017716,0.));
#66453=CARTESIAN_POINT('Ctrl Pts',(15.3979805373174,-72.7101409017716,12.));
#66454=CARTESIAN_POINT('Ctrl Pts',(15.4144625111944,-72.7324700089712,0.));
#66455=CARTESIAN_POINT('Ctrl Pts',(15.4144625111944,-72.7324700089712,12.));
#66456=CARTESIAN_POINT('Ctrl Pts',(15.4309852897844,-72.7548121825342,0.));
#66457=CARTESIAN_POINT('Ctrl Pts',(15.4309852897844,-72.7548121825342,12.));
#66458=CARTESIAN_POINT('Ctrl Pts',(15.4475488590243,-72.777167349421,0.));
#66459=CARTESIAN_POINT('Ctrl Pts',(15.4475488590243,-72.777167349421,12.));
#66460=CARTESIAN_POINT('Ctrl Pts',(15.4641532053281,-72.7995354603795,0.));
#66461=CARTESIAN_POINT('Ctrl Pts',(15.4641532053281,-72.7995354603795,12.));
#66462=CARTESIAN_POINT('Ctrl Pts',(15.4807983165804,-72.8219164843279,0.));
#66463=CARTESIAN_POINT('Ctrl Pts',(15.4807983165804,-72.8219164843279,12.));
#66464=CARTESIAN_POINT('Ctrl Pts',(15.494147009702,-72.8398316205897,0.));
#66465=CARTESIAN_POINT('Ctrl Pts',(15.494147009702,-72.8398316205897,12.));
#66466=CARTESIAN_POINT('Ctrl Pts',(15.5041768663998,-72.8532737731759,0.));
#66467=CARTESIAN_POINT('Ctrl Pts',(15.5041768663998,-72.8532737731759,12.));
#66468=CARTESIAN_POINT('Ctrl Pts',(15.5108715869141,-72.8622377860824,0.));
#66469=CARTESIAN_POINT('Ctrl Pts',(15.5108715869141,-72.8622377860824,12.));
#66470=CARTESIAN_POINT('Ctrl Pts',(15.5142209845168,-72.8667204369977,0.));
#66471=CARTESIAN_POINT('Ctrl Pts',(15.5142209845168,-72.8667204369977,12.));
#66472=CARTESIAN_POINT('',(12.9953224629497,-68.7831490561748,0.));
#66473=CARTESIAN_POINT('Ctrl Pts',(12.9953224629497,-68.7831490561748,0.));
#66474=CARTESIAN_POINT('Ctrl Pts',(12.9969981460277,-68.7866525680193,0.));
#66475=CARTESIAN_POINT('Ctrl Pts',(13.0003537683054,-68.7936635625545,0.));
#66476=CARTESIAN_POINT('Ctrl Pts',(13.0053999700875,-68.804191966902,0.));
#66477=CARTESIAN_POINT('Ctrl Pts',(13.0121537768945,-68.8182536653656,0.));
#66478=CARTESIAN_POINT('Ctrl Pts',(13.0206386039691,-68.8358704887468,0.));
#66479=CARTESIAN_POINT('Ctrl Pts',(13.0291660060107,-68.8535269726793,0.));
#66480=CARTESIAN_POINT('Ctrl Pts',(13.0377359881875,-68.8712230321906,0.));
#66481=CARTESIAN_POINT('Ctrl Pts',(13.0463485518206,-68.8889585151585,0.));
#66482=CARTESIAN_POINT('Ctrl Pts',(13.0550036938813,-68.9067332040985,0.));
#66483=CARTESIAN_POINT('Ctrl Pts',(13.0637014089029,-68.9245468449945,0.));
#66484=CARTESIAN_POINT('Ctrl Pts',(13.072441690283,-68.9423991694492,0.));
#66485=CARTESIAN_POINT('Ctrl Pts',(13.0812245317807,-68.9602899187573,0.));
#66486=CARTESIAN_POINT('Ctrl Pts',(13.090049929053,-68.9782188692581,0.));
#66487=CARTESIAN_POINT('Ctrl Pts',(13.0989178791833,-68.9961858241519,0.));
#66488=CARTESIAN_POINT('Ctrl Pts',(13.1078283799722,-69.0141906015113,0.));
#66489=CARTESIAN_POINT('Ctrl Pts',(13.1167814293497,-69.0322330243348,0.));
#66490=CARTESIAN_POINT('Ctrl Pts',(13.1257770246385,-69.0503129081817,0.));
#66491=CARTESIAN_POINT('Ctrl Pts',(13.1348151621834,-69.0684300549477,0.));
#66492=CARTESIAN_POINT('Ctrl Pts',(13.1438958377404,-69.0865842593102,0.));
#66493=CARTESIAN_POINT('Ctrl Pts',(13.1530190467183,-69.1047753127643,0.));
#66494=CARTESIAN_POINT('Ctrl Pts',(13.1621847844528,-69.1230030082573,0.));
#66495=CARTESIAN_POINT('Ctrl Pts',(13.1713930465132,-69.1412671454564,0.));
#66496=CARTESIAN_POINT('Ctrl Pts',(13.1806438286934,-69.1595675305245,0.));
#66497=CARTESIAN_POINT('Ctrl Pts',(13.1899371268683,-69.1779039735996,0.));
#66498=CARTESIAN_POINT('Ctrl Pts',(13.1992729368928,-69.1962762870527,0.));
#66499=CARTESIAN_POINT('Ctrl Pts',(13.2086512544735,-69.2146842833537,0.));
#66500=CARTESIAN_POINT('Ctrl Pts',(13.2180720750594,-69.2331277732861,0.));
#66501=CARTESIAN_POINT('Ctrl Pts',(13.2275353939051,-69.2516065668844,0.));
#66502=CARTESIAN_POINT('Ctrl Pts',(13.237041206122,-69.2701204742449,0.));
#66503=CARTESIAN_POINT('Ctrl Pts',(13.2465895067262,-69.2886693063182,0.));
#66504=CARTESIAN_POINT('Ctrl Pts',(13.2561802906896,-69.3072528758518,0.));
#66505=CARTESIAN_POINT('Ctrl Pts',(13.265813552961,-69.3258709977382,0.));
#66506=CARTESIAN_POINT('Ctrl Pts',(13.2754892884433,-69.3445234885065,0.));
#66507=CARTESIAN_POINT('Ctrl Pts',(13.2852074919765,-69.3632101660066,0.));
#66508=CARTESIAN_POINT('Ctrl Pts',(13.2949681583167,-69.3819308490422,0.));
#66509=CARTESIAN_POINT('Ctrl Pts',(13.3047712821051,-69.4006853569511,0.));
#66510=CARTESIAN_POINT('Ctrl Pts',(13.3146168578743,-69.4194735096265,0.));
#66511=CARTESIAN_POINT('Ctrl Pts',(13.3245048800643,-69.4382951276998,0.));
#66512=CARTESIAN_POINT('Ctrl Pts',(13.3344353430313,-69.4571500326673,0.));
#66513=CARTESIAN_POINT('Ctrl Pts',(13.3444082410543,-69.4760380470365,0.));
#66514=CARTESIAN_POINT('Ctrl Pts',(13.3544235683393,-69.4949589944606,0.));
#66515=CARTESIAN_POINT('Ctrl Pts',(13.3644813190219,-69.5139126996675,0.));
#66516=CARTESIAN_POINT('Ctrl Pts',(13.3745814871664,-69.5328989883885,0.));
#66517=CARTESIAN_POINT('Ctrl Pts',(13.3847240667627,-69.5519176872862,0.));
#66518=CARTESIAN_POINT('Ctrl Pts',(13.3949090517177,-69.5709686238724,0.));
#66519=CARTESIAN_POINT('Ctrl Pts',(13.4051364358499,-69.5900516264553,0.));
#66520=CARTESIAN_POINT('Ctrl Pts',(13.4154062129002,-69.6091665241765,0.));
#66521=CARTESIAN_POINT('Ctrl Pts',(13.4257183765341,-69.6283131470273,0.));
#66522=CARTESIAN_POINT('Ctrl Pts',(13.4360729203442,-69.6474913258675,0.));
#66523=CARTESIAN_POINT('Ctrl Pts',(13.4464698378453,-69.666700892444,0.));
#66524=CARTESIAN_POINT('Ctrl Pts',(13.456909122476,-69.6859416793886,0.));
#66525=CARTESIAN_POINT('Ctrl Pts',(13.4673907676044,-69.7052135201998,0.));
#66526=CARTESIAN_POINT('Ctrl Pts',(13.4779147665285,-69.724516249225,0.));
#66527=CARTESIAN_POINT('Ctrl Pts',(13.4884811124748,-69.7438497016406,0.));
#66528=CARTESIAN_POINT('Ctrl Pts',(13.4990897985904,-69.7632137134249,0.));
#66529=CARTESIAN_POINT('Ctrl Pts',(13.5097408179479,-69.7826081213576,0.));
#66530=CARTESIAN_POINT('Ctrl Pts',(13.5204341635507,-69.8020327630205,0.));
#66531=CARTESIAN_POINT('Ctrl Pts',(13.5311698283339,-69.8214874767944,0.));
#66532=CARTESIAN_POINT('Ctrl Pts',(13.5419478051625,-69.840972101856,0.));
#66533=CARTESIAN_POINT('Ctrl Pts',(13.5527680868255,-69.8604864781706,0.));
#66534=CARTESIAN_POINT('Ctrl Pts',(13.5636306660421,-69.8800304464882,0.));
#66535=CARTESIAN_POINT('Ctrl Pts',(13.5745355354656,-69.8996038483361,0.));
#66536=CARTESIAN_POINT('Ctrl Pts',(13.5854826876834,-69.9192065260108,0.));
#66537=CARTESIAN_POINT('Ctrl Pts',(13.5964721152135,-69.9388383225648,0.));
#66538=CARTESIAN_POINT('Ctrl Pts',(13.6075038104998,-69.9584990817974,0.));
#66539=CARTESIAN_POINT('Ctrl Pts',(13.6185777659198,-69.9781886482527,0.));
#66540=CARTESIAN_POINT('Ctrl Pts',(13.6296939737865,-69.9979068672153,0.));
#66541=CARTESIAN_POINT('Ctrl Pts',(13.6408524263496,-70.0176535847049,0.));
#66542=CARTESIAN_POINT('Ctrl Pts',(13.6520531157907,-70.0374286474677,0.));
#66543=CARTESIAN_POINT('Ctrl Pts',(13.6632960342196,-70.0572319029676,0.));
#66544=CARTESIAN_POINT('Ctrl Pts',(13.6745811736829,-70.0770631993856,0.));
#66545=CARTESIAN_POINT('Ctrl Pts',(13.6859085261653,-70.0969223856136,0.));
#66546=CARTESIAN_POINT('Ctrl Pts',(13.6972780835897,-70.1168093112486,0.));
#66547=CARTESIAN_POINT('Ctrl Pts',(13.7086898378121,-70.1367238265825,0.));
#66548=CARTESIAN_POINT('Ctrl Pts',(13.7201437806199,-70.156665782595,0.));
#66549=CARTESIAN_POINT('Ctrl Pts',(13.7316399037392,-70.1766350309518,0.));
#66550=CARTESIAN_POINT('Ctrl Pts',(13.7431781988364,-70.1966314239995,0.));
#66551=CARTESIAN_POINT('Ctrl Pts',(13.754758657518,-70.2166548147604,0.));
#66552=CARTESIAN_POINT('Ctrl Pts',(13.7663812713243,-70.2367050569215,0.));
#66553=CARTESIAN_POINT('Ctrl Pts',(13.7780460317294,-70.2567820048303,0.));
#66554=CARTESIAN_POINT('Ctrl Pts',(13.7897529301491,-70.2768855134947,0.));
#66555=CARTESIAN_POINT('Ctrl Pts',(13.8015019579414,-70.2970154385774,0.));
#66556=CARTESIAN_POINT('Ctrl Pts',(13.8132931064063,-70.3171716363897,0.));
#66557=CARTESIAN_POINT('Ctrl Pts',(13.825126366779,-70.3373539638809,0.));
#66558=CARTESIAN_POINT('Ctrl Pts',(13.8370017302309,-70.3575622786335,0.));
#66559=CARTESIAN_POINT('Ctrl Pts',(13.8489191878767,-70.3777964388632,0.));
#66560=CARTESIAN_POINT('Ctrl Pts',(13.8608787307751,-70.3980563034133,0.));
#66561=CARTESIAN_POINT('Ctrl Pts',(13.8728803499287,-70.4183417317499,0.));
#66562=CARTESIAN_POINT('Ctrl Pts',(13.8849240362763,-70.4386525839521,0.));
#66563=CARTESIAN_POINT('Ctrl Pts',(13.8970097806953,-70.4589887207073,0.));
#66564=CARTESIAN_POINT('Ctrl Pts',(13.9091375740088,-70.4793500033124,0.));
#66565=CARTESIAN_POINT('Ctrl Pts',(13.9213074069852,-70.4997362936673,0.));
#66566=CARTESIAN_POINT('Ctrl Pts',(13.9335192703388,-70.520147454271,0.));
#66567=CARTESIAN_POINT('Ctrl Pts',(13.9457731547215,-70.5405833482112,0.));
#66568=CARTESIAN_POINT('Ctrl Pts',(13.958069050726,-70.5610438391612,0.));
#66569=CARTESIAN_POINT('Ctrl Pts',(13.9704069488917,-70.5815287913784,0.));
#66570=CARTESIAN_POINT('Ctrl Pts',(13.9827868397057,-70.6020380697004,0.));
#66571=CARTESIAN_POINT('Ctrl Pts',(13.9952087136018,-70.6225715395394,0.));
#66572=CARTESIAN_POINT('Ctrl Pts',(14.0076725609536,-70.6431290668745,0.));
#66573=CARTESIAN_POINT('Ctrl Pts',(14.0201783720769,-70.6637105182484,0.));
#66574=CARTESIAN_POINT('Ctrl Pts',(14.0327261372362,-70.6843157607668,0.));
#66575=CARTESIAN_POINT('Ctrl Pts',(14.0453158466451,-70.7049446620928,0.));
#66576=CARTESIAN_POINT('Ctrl Pts',(14.0579474904657,-70.7255970904436,0.));
#66577=CARTESIAN_POINT('Ctrl Pts',(14.0706210588016,-70.7462729145807,0.));
#66578=CARTESIAN_POINT('Ctrl Pts',(14.0833365416996,-70.7669720038077,0.));
#66579=CARTESIAN_POINT('Ctrl Pts',(14.0960939291569,-70.7876942279697,0.));
#66580=CARTESIAN_POINT('Ctrl Pts',(14.1088932111214,-70.8084394574493,0.));
#66581=CARTESIAN_POINT('Ctrl Pts',(14.1217343774913,-70.8292075631621,0.));
#66582=CARTESIAN_POINT('Ctrl Pts',(14.1346174181078,-70.8499984165489,0.));
#66583=CARTESIAN_POINT('Ctrl Pts',(14.1475423227568,-70.8708118895715,0.));
#66584=CARTESIAN_POINT('Ctrl Pts',(14.1605090811754,-70.8916478547132,0.));
#66585=CARTESIAN_POINT('Ctrl Pts',(14.1735176830533,-70.9125061849745,0.));
#66586=CARTESIAN_POINT('Ctrl Pts',(14.186568118032,-70.9333867538704,0.));
#66587=CARTESIAN_POINT('Ctrl Pts',(14.1996603756982,-70.9542894354216,0.));
#66588=CARTESIAN_POINT('Ctrl Pts',(14.2127944455838,-70.9752141041518,0.));
#66589=CARTESIAN_POINT('Ctrl Pts',(14.2259703171737,-70.9961606350861,0.));
#66590=CARTESIAN_POINT('Ctrl Pts',(14.2391879799061,-71.0171289037488,0.));
#66591=CARTESIAN_POINT('Ctrl Pts',(14.2524474231732,-71.0381187861588,0.));
#66592=CARTESIAN_POINT('Ctrl Pts',(14.2657486363139,-71.0591301588231,0.));
#66593=CARTESIAN_POINT('Ctrl Pts',(14.2790916086133,-71.0801628987332,0.));
#66594=CARTESIAN_POINT('Ctrl Pts',(14.2924763293105,-71.1012168833643,0.));
#66595=CARTESIAN_POINT('Ctrl Pts',(14.3059027875994,-71.1222919906727,0.));
#66596=CARTESIAN_POINT('Ctrl Pts',(14.3193709726294,-71.1433880990929,0.));
#66597=CARTESIAN_POINT('Ctrl Pts',(14.3328808734989,-71.1645050875308,0.));
#66598=CARTESIAN_POINT('Ctrl Pts',(14.3464324792533,-71.1856428353593,0.));
#66599=CARTESIAN_POINT('Ctrl Pts',(14.3600257788924,-71.2068012224174,0.));
#66600=CARTESIAN_POINT('Ctrl Pts',(14.3736607613722,-71.2279801290084,0.));
#66601=CARTESIAN_POINT('Ctrl Pts',(14.3873374156056,-71.2491794358958,0.));
#66602=CARTESIAN_POINT('Ctrl Pts',(14.401055730457,-71.2703990242988,0.));
#66603=CARTESIAN_POINT('Ctrl Pts',(14.4148156947383,-71.2916387758861,0.));
#66604=CARTESIAN_POINT('Ctrl Pts',(14.4286172972166,-71.312898572777,0.));
#66605=CARTESIAN_POINT('Ctrl Pts',(14.4424605266165,-71.3341782975386,0.));
#66606=CARTESIAN_POINT('Ctrl Pts',(14.4563453716204,-71.3554778331835,0.));
#66607=CARTESIAN_POINT('Ctrl Pts',(14.4702718208651,-71.376797063165,0.));
#66608=CARTESIAN_POINT('Ctrl Pts',(14.4842398629355,-71.3981358713723,0.));
#66609=CARTESIAN_POINT('Ctrl Pts',(14.4982494863718,-71.4194941421292,0.));
#66610=CARTESIAN_POINT('Ctrl Pts',(14.5123006796728,-71.4408717601923,0.));
#66611=CARTESIAN_POINT('Ctrl Pts',(14.5263934312969,-71.4622686107475,0.));
#66612=CARTESIAN_POINT('Ctrl Pts',(14.540527729659,-71.4836845794048,0.));
#66613=CARTESIAN_POINT('Ctrl Pts',(14.5547035631233,-71.5051195521909,0.));
#66614=CARTESIAN_POINT('Ctrl Pts',(14.5689209200091,-71.5265734155498,0.));
#66615=CARTESIAN_POINT('Ctrl Pts',(14.5831797885952,-71.5480460563447,0.));
#66616=CARTESIAN_POINT('Ctrl Pts',(14.597480157121,-71.5695373618562,0.));
#66617=CARTESIAN_POINT('Ctrl Pts',(14.6118220137849,-71.5910472197813,0.));
#66618=CARTESIAN_POINT('Ctrl Pts',(14.626205346737,-71.612575518229,0.));
#66619=CARTESIAN_POINT('Ctrl Pts',(14.6406301440814,-71.6341221457169,0.));
#66620=CARTESIAN_POINT('Ctrl Pts',(14.6550963938829,-71.6556869911662,0.));
#66621=CARTESIAN_POINT('Ctrl Pts',(14.6696040841678,-71.6772699438963,0.));
#66622=CARTESIAN_POINT('Ctrl Pts',(14.6841532029232,-71.6988708936172,0.));
#66623=CARTESIAN_POINT('Ctrl Pts',(14.69874373809,-71.7204897304194,0.));
#66624=CARTESIAN_POINT('Ctrl Pts',(14.7133756775625,-71.7421263447719,0.));
#66625=CARTESIAN_POINT('Ctrl Pts',(14.7280490091957,-71.7637806275328,0.));
#66626=CARTESIAN_POINT('Ctrl Pts',(14.7427637208072,-71.7854524699569,0.));
#66627=CARTESIAN_POINT('Ctrl Pts',(14.7575198001776,-71.8071417637017,0.));
#66628=CARTESIAN_POINT('Ctrl Pts',(14.7723172350451,-71.8288484008333,0.));
#66629=CARTESIAN_POINT('Ctrl Pts',(14.7871560131016,-71.8505722738272,0.));
#66630=CARTESIAN_POINT('Ctrl Pts',(14.8020361219998,-71.8723132755446,0.));
#66631=CARTESIAN_POINT('Ctrl Pts',(14.8169575493557,-71.8940712992109,0.));
#66632=CARTESIAN_POINT('Ctrl Pts',(14.8319202827482,-71.9158462383914,0.));
#66633=CARTESIAN_POINT('Ctrl Pts',(14.8469243097162,-71.9376379869678,0.));
#66634=CARTESIAN_POINT('Ctrl Pts',(14.8619696177506,-71.9594464391078,0.));
#66635=CARTESIAN_POINT('Ctrl Pts',(14.8770561943014,-71.9812714893102,0.));
#66636=CARTESIAN_POINT('Ctrl Pts',(14.8921840267832,-72.0031130324529,0.));
#66637=CARTESIAN_POINT('Ctrl Pts',(14.9073531025764,-72.0249709638422,0.));
#66638=CARTESIAN_POINT('Ctrl Pts',(14.9225634090268,-72.0468451792505,0.));
#66639=CARTESIAN_POINT('Ctrl Pts',(14.9378149334388,-72.0687355749806,0.));
#66640=CARTESIAN_POINT('Ctrl Pts',(14.9531076630767,-72.0906420478076,0.));
#66641=CARTESIAN_POINT('Ctrl Pts',(14.9684415851698,-72.112564494854,0.));
#66642=CARTESIAN_POINT('Ctrl Pts',(14.9838166869107,-72.1345028134777,0.));
#66643=CARTESIAN_POINT('Ctrl Pts',(14.9992329554537,-72.1564569011669,0.));
#66644=CARTESIAN_POINT('Ctrl Pts',(15.0146903779062,-72.1784266553953,0.));
#66645=CARTESIAN_POINT('Ctrl Pts',(15.0301889413257,-72.2004119736115,0.));
#66646=CARTESIAN_POINT('Ctrl Pts',(15.0457286327331,-72.2224127535415,0.));
#66647=CARTESIAN_POINT('Ctrl Pts',(15.0613094391189,-72.2444288934262,0.));
#66648=CARTESIAN_POINT('Ctrl Pts',(15.0769313474476,-72.2664602922852,0.));
#66649=CARTESIAN_POINT('Ctrl Pts',(15.0925943446589,-72.2885068501628,0.));
#66650=CARTESIAN_POINT('Ctrl Pts',(15.1082984176649,-72.3105684683944,0.));
#66651=CARTESIAN_POINT('Ctrl Pts',(15.124043553347,-72.3326450490177,0.));
#66652=CARTESIAN_POINT('Ctrl Pts',(15.1398297385506,-72.3547364941969,0.));
#66653=CARTESIAN_POINT('Ctrl Pts',(15.1556569600744,-72.376842705589,0.));
#66654=CARTESIAN_POINT('Ctrl Pts',(15.1715252046606,-72.3989635838492,0.));
#66655=CARTESIAN_POINT('Ctrl Pts',(15.1874344589725,-72.421099027786,0.));
#66656=CARTESIAN_POINT('Ctrl Pts',(15.2033847096091,-72.4432489350471,0.));
#66657=CARTESIAN_POINT('Ctrl Pts',(15.2193759431372,-72.4654132036428,0.));
#66658=CARTESIAN_POINT('Ctrl Pts',(15.235408146116,-72.4875917332761,0.));
#66659=CARTESIAN_POINT('Ctrl Pts',(15.2514813051172,-72.5097844266075,0.));
#66660=CARTESIAN_POINT('Ctrl Pts',(15.2675954067479,-72.5319911908917,0.));
#66661=CARTESIAN_POINT('Ctrl Pts',(15.2837504376535,-72.5542119383642,0.));
#66662=CARTESIAN_POINT('Ctrl Pts',(15.297633502478,-72.5732713370618,0.));
#66663=CARTESIAN_POINT('Ctrl Pts',(15.3082994603539,-72.5878912620439,0.));
#66664=CARTESIAN_POINT('Ctrl Pts',(15.3157301930682,-72.5980655789635,0.));
#66665=CARTESIAN_POINT('Ctrl Pts',(15.3199137230129,-72.6037902604921,0.));
#66666=CARTESIAN_POINT('Ctrl Pts',(15.3208442077189,-72.6050633494351,0.));
#66667=CARTESIAN_POINT('',(12.9953224629497,-68.7831490561748,12.));
#66668=CARTESIAN_POINT('',(12.9953224629497,-68.7831490561748,0.));
#66669=CARTESIAN_POINT('Ctrl Pts',(15.3208442077188,-72.6050633494351,12.));
#66670=CARTESIAN_POINT('Ctrl Pts',(15.3199137230129,-72.603790260492,12.));
#66671=CARTESIAN_POINT('Ctrl Pts',(15.3157301930681,-72.5980655789635,12.));
#66672=CARTESIAN_POINT('Ctrl Pts',(15.3082994603539,-72.5878912620439,12.));
#66673=CARTESIAN_POINT('Ctrl Pts',(15.297633502478,-72.5732713370618,12.));
#66674=CARTESIAN_POINT('Ctrl Pts',(15.2837504376535,-72.5542119383642,12.));
#66675=CARTESIAN_POINT('Ctrl Pts',(15.2675954067479,-72.5319911908917,12.));
#66676=CARTESIAN_POINT('Ctrl Pts',(15.2514813051172,-72.5097844266075,12.));
#66677=CARTESIAN_POINT('Ctrl Pts',(15.235408146116,-72.4875917332761,12.));
#66678=CARTESIAN_POINT('Ctrl Pts',(15.2193759431372,-72.4654132036428,12.));
#66679=CARTESIAN_POINT('Ctrl Pts',(15.2033847096091,-72.4432489350471,12.));
#66680=CARTESIAN_POINT('Ctrl Pts',(15.1874344589725,-72.421099027786,12.));
#66681=CARTESIAN_POINT('Ctrl Pts',(15.1715252046606,-72.3989635838492,12.));
#66682=CARTESIAN_POINT('Ctrl Pts',(15.1556569600744,-72.376842705589,12.));
#66683=CARTESIAN_POINT('Ctrl Pts',(15.1398297385506,-72.3547364941969,12.));
#66684=CARTESIAN_POINT('Ctrl Pts',(15.124043553347,-72.3326450490177,12.));
#66685=CARTESIAN_POINT('Ctrl Pts',(15.1082984176649,-72.3105684683944,12.));
#66686=CARTESIAN_POINT('Ctrl Pts',(15.0925943446589,-72.2885068501628,12.));
#66687=CARTESIAN_POINT('Ctrl Pts',(15.0769313474476,-72.2664602922852,12.));
#66688=CARTESIAN_POINT('Ctrl Pts',(15.0613094391189,-72.2444288934262,12.));
#66689=CARTESIAN_POINT('Ctrl Pts',(15.0457286327331,-72.2224127535415,12.));
#66690=CARTESIAN_POINT('Ctrl Pts',(15.0301889413257,-72.2004119736115,12.));
#66691=CARTESIAN_POINT('Ctrl Pts',(15.0146903779062,-72.1784266553953,12.));
#66692=CARTESIAN_POINT('Ctrl Pts',(14.9992329554537,-72.1564569011669,12.));
#66693=CARTESIAN_POINT('Ctrl Pts',(14.9838166869107,-72.1345028134777,12.));
#66694=CARTESIAN_POINT('Ctrl Pts',(14.9684415851698,-72.112564494854,12.));
#66695=CARTESIAN_POINT('Ctrl Pts',(14.9531076630767,-72.0906420478076,12.));
#66696=CARTESIAN_POINT('Ctrl Pts',(14.9378149334388,-72.0687355749806,12.));
#66697=CARTESIAN_POINT('Ctrl Pts',(14.9225634090268,-72.0468451792505,12.));
#66698=CARTESIAN_POINT('Ctrl Pts',(14.9073531025764,-72.0249709638422,12.));
#66699=CARTESIAN_POINT('Ctrl Pts',(14.8921840267832,-72.0031130324529,12.));
#66700=CARTESIAN_POINT('Ctrl Pts',(14.8770561943014,-71.9812714893102,12.));
#66701=CARTESIAN_POINT('Ctrl Pts',(14.8619696177506,-71.9594464391078,12.));
#66702=CARTESIAN_POINT('Ctrl Pts',(14.8469243097162,-71.9376379869678,12.));
#66703=CARTESIAN_POINT('Ctrl Pts',(14.8319202827482,-71.9158462383914,12.));
#66704=CARTESIAN_POINT('Ctrl Pts',(14.8169575493557,-71.8940712992109,12.));
#66705=CARTESIAN_POINT('Ctrl Pts',(14.8020361219998,-71.8723132755446,12.));
#66706=CARTESIAN_POINT('Ctrl Pts',(14.7871560131016,-71.8505722738272,12.));
#66707=CARTESIAN_POINT('Ctrl Pts',(14.7723172350451,-71.8288484008333,12.));
#66708=CARTESIAN_POINT('Ctrl Pts',(14.7575198001776,-71.8071417637017,12.));
#66709=CARTESIAN_POINT('Ctrl Pts',(14.7427637208072,-71.7854524699569,12.));
#66710=CARTESIAN_POINT('Ctrl Pts',(14.7280490091957,-71.7637806275328,12.));
#66711=CARTESIAN_POINT('Ctrl Pts',(14.7133756775625,-71.7421263447719,12.));
#66712=CARTESIAN_POINT('Ctrl Pts',(14.69874373809,-71.7204897304194,12.));
#66713=CARTESIAN_POINT('Ctrl Pts',(14.6841532029232,-71.6988708936172,12.));
#66714=CARTESIAN_POINT('Ctrl Pts',(14.6696040841678,-71.6772699438963,12.));
#66715=CARTESIAN_POINT('Ctrl Pts',(14.6550963938829,-71.6556869911662,12.));
#66716=CARTESIAN_POINT('Ctrl Pts',(14.6406301440814,-71.6341221457169,12.));
#66717=CARTESIAN_POINT('Ctrl Pts',(14.626205346737,-71.612575518229,12.));
#66718=CARTESIAN_POINT('Ctrl Pts',(14.6118220137849,-71.5910472197813,12.));
#66719=CARTESIAN_POINT('Ctrl Pts',(14.597480157121,-71.5695373618562,12.));
#66720=CARTESIAN_POINT('Ctrl Pts',(14.5831797885952,-71.5480460563447,12.));
#66721=CARTESIAN_POINT('Ctrl Pts',(14.5689209200091,-71.5265734155498,12.));
#66722=CARTESIAN_POINT('Ctrl Pts',(14.5547035631233,-71.5051195521909,12.));
#66723=CARTESIAN_POINT('Ctrl Pts',(14.540527729659,-71.4836845794048,12.));
#66724=CARTESIAN_POINT('Ctrl Pts',(14.5263934312969,-71.4622686107475,12.));
#66725=CARTESIAN_POINT('Ctrl Pts',(14.5123006796728,-71.4408717601923,12.));
#66726=CARTESIAN_POINT('Ctrl Pts',(14.4982494863718,-71.4194941421292,12.));
#66727=CARTESIAN_POINT('Ctrl Pts',(14.4842398629355,-71.3981358713723,12.));
#66728=CARTESIAN_POINT('Ctrl Pts',(14.4702718208651,-71.376797063165,12.));
#66729=CARTESIAN_POINT('Ctrl Pts',(14.4563453716204,-71.3554778331835,12.));
#66730=CARTESIAN_POINT('Ctrl Pts',(14.4424605266165,-71.3341782975386,12.));
#66731=CARTESIAN_POINT('Ctrl Pts',(14.4286172972166,-71.312898572777,12.));
#66732=CARTESIAN_POINT('Ctrl Pts',(14.4148156947383,-71.2916387758861,12.));
#66733=CARTESIAN_POINT('Ctrl Pts',(14.401055730457,-71.2703990242988,12.));
#66734=CARTESIAN_POINT('Ctrl Pts',(14.3873374156056,-71.2491794358958,12.));
#66735=CARTESIAN_POINT('Ctrl Pts',(14.3736607613722,-71.2279801290084,12.));
#66736=CARTESIAN_POINT('Ctrl Pts',(14.3600257788924,-71.2068012224174,12.));
#66737=CARTESIAN_POINT('Ctrl Pts',(14.3464324792533,-71.1856428353593,12.));
#66738=CARTESIAN_POINT('Ctrl Pts',(14.3328808734989,-71.1645050875308,12.));
#66739=CARTESIAN_POINT('Ctrl Pts',(14.3193709726294,-71.1433880990929,12.));
#66740=CARTESIAN_POINT('Ctrl Pts',(14.3059027875994,-71.1222919906727,12.));
#66741=CARTESIAN_POINT('Ctrl Pts',(14.2924763293105,-71.1012168833643,12.));
#66742=CARTESIAN_POINT('Ctrl Pts',(14.2790916086133,-71.0801628987332,12.));
#66743=CARTESIAN_POINT('Ctrl Pts',(14.2657486363139,-71.0591301588231,12.));
#66744=CARTESIAN_POINT('Ctrl Pts',(14.2524474231732,-71.0381187861588,12.));
#66745=CARTESIAN_POINT('Ctrl Pts',(14.2391879799061,-71.0171289037488,12.));
#66746=CARTESIAN_POINT('Ctrl Pts',(14.2259703171737,-70.9961606350861,12.));
#66747=CARTESIAN_POINT('Ctrl Pts',(14.2127944455838,-70.9752141041518,12.));
#66748=CARTESIAN_POINT('Ctrl Pts',(14.1996603756982,-70.9542894354216,12.));
#66749=CARTESIAN_POINT('Ctrl Pts',(14.186568118032,-70.9333867538704,12.));
#66750=CARTESIAN_POINT('Ctrl Pts',(14.1735176830533,-70.9125061849745,12.));
#66751=CARTESIAN_POINT('Ctrl Pts',(14.1605090811754,-70.8916478547132,12.));
#66752=CARTESIAN_POINT('Ctrl Pts',(14.1475423227568,-70.8708118895715,12.));
#66753=CARTESIAN_POINT('Ctrl Pts',(14.1346174181078,-70.8499984165489,12.));
#66754=CARTESIAN_POINT('Ctrl Pts',(14.1217343774913,-70.8292075631621,12.));
#66755=CARTESIAN_POINT('Ctrl Pts',(14.1088932111214,-70.8084394574493,12.));
#66756=CARTESIAN_POINT('Ctrl Pts',(14.0960939291569,-70.7876942279697,12.));
#66757=CARTESIAN_POINT('Ctrl Pts',(14.0833365416996,-70.7669720038077,12.));
#66758=CARTESIAN_POINT('Ctrl Pts',(14.0706210588016,-70.7462729145807,12.));
#66759=CARTESIAN_POINT('Ctrl Pts',(14.0579474904657,-70.7255970904436,12.));
#66760=CARTESIAN_POINT('Ctrl Pts',(14.0453158466451,-70.7049446620928,12.));
#66761=CARTESIAN_POINT('Ctrl Pts',(14.0327261372362,-70.6843157607668,12.));
#66762=CARTESIAN_POINT('Ctrl Pts',(14.0201783720769,-70.6637105182484,12.));
#66763=CARTESIAN_POINT('Ctrl Pts',(14.0076725609536,-70.6431290668745,12.));
#66764=CARTESIAN_POINT('Ctrl Pts',(13.9952087136018,-70.6225715395394,12.));
#66765=CARTESIAN_POINT('Ctrl Pts',(13.9827868397057,-70.6020380697004,12.));
#66766=CARTESIAN_POINT('Ctrl Pts',(13.9704069488917,-70.5815287913784,12.));
#66767=CARTESIAN_POINT('Ctrl Pts',(13.958069050726,-70.5610438391612,12.));
#66768=CARTESIAN_POINT('Ctrl Pts',(13.9457731547215,-70.5405833482112,12.));
#66769=CARTESIAN_POINT('Ctrl Pts',(13.9335192703388,-70.520147454271,12.));
#66770=CARTESIAN_POINT('Ctrl Pts',(13.9213074069852,-70.4997362936673,12.));
#66771=CARTESIAN_POINT('Ctrl Pts',(13.9091375740088,-70.4793500033124,12.));
#66772=CARTESIAN_POINT('Ctrl Pts',(13.8970097806953,-70.4589887207073,12.));
#66773=CARTESIAN_POINT('Ctrl Pts',(13.8849240362763,-70.4386525839521,12.));
#66774=CARTESIAN_POINT('Ctrl Pts',(13.8728803499287,-70.4183417317499,12.));
#66775=CARTESIAN_POINT('Ctrl Pts',(13.8608787307751,-70.3980563034133,12.));
#66776=CARTESIAN_POINT('Ctrl Pts',(13.8489191878767,-70.3777964388632,12.));
#66777=CARTESIAN_POINT('Ctrl Pts',(13.8370017302309,-70.3575622786335,12.));
#66778=CARTESIAN_POINT('Ctrl Pts',(13.825126366779,-70.3373539638809,12.));
#66779=CARTESIAN_POINT('Ctrl Pts',(13.8132931064063,-70.3171716363897,12.));
#66780=CARTESIAN_POINT('Ctrl Pts',(13.8015019579414,-70.2970154385774,12.));
#66781=CARTESIAN_POINT('Ctrl Pts',(13.7897529301491,-70.2768855134947,12.));
#66782=CARTESIAN_POINT('Ctrl Pts',(13.7780460317294,-70.2567820048303,12.));
#66783=CARTESIAN_POINT('Ctrl Pts',(13.7663812713243,-70.2367050569215,12.));
#66784=CARTESIAN_POINT('Ctrl Pts',(13.754758657518,-70.2166548147604,12.));
#66785=CARTESIAN_POINT('Ctrl Pts',(13.7431781988364,-70.1966314239995,12.));
#66786=CARTESIAN_POINT('Ctrl Pts',(13.7316399037392,-70.1766350309518,12.));
#66787=CARTESIAN_POINT('Ctrl Pts',(13.7201437806199,-70.156665782595,12.));
#66788=CARTESIAN_POINT('Ctrl Pts',(13.7086898378121,-70.1367238265825,12.));
#66789=CARTESIAN_POINT('Ctrl Pts',(13.6972780835897,-70.1168093112486,12.));
#66790=CARTESIAN_POINT('Ctrl Pts',(13.6859085261653,-70.0969223856136,12.));
#66791=CARTESIAN_POINT('Ctrl Pts',(13.6745811736829,-70.0770631993856,12.));
#66792=CARTESIAN_POINT('Ctrl Pts',(13.6632960342196,-70.0572319029676,12.));
#66793=CARTESIAN_POINT('Ctrl Pts',(13.6520531157907,-70.0374286474677,12.));
#66794=CARTESIAN_POINT('Ctrl Pts',(13.6408524263496,-70.0176535847049,12.));
#66795=CARTESIAN_POINT('Ctrl Pts',(13.6296939737865,-69.9979068672153,12.));
#66796=CARTESIAN_POINT('Ctrl Pts',(13.6185777659198,-69.9781886482527,12.));
#66797=CARTESIAN_POINT('Ctrl Pts',(13.6075038104998,-69.9584990817974,12.));
#66798=CARTESIAN_POINT('Ctrl Pts',(13.5964721152135,-69.9388383225648,12.));
#66799=CARTESIAN_POINT('Ctrl Pts',(13.5854826876834,-69.9192065260108,12.));
#66800=CARTESIAN_POINT('Ctrl Pts',(13.5745355354656,-69.8996038483361,12.));
#66801=CARTESIAN_POINT('Ctrl Pts',(13.5636306660421,-69.8800304464882,12.));
#66802=CARTESIAN_POINT('Ctrl Pts',(13.5527680868255,-69.8604864781706,12.));
#66803=CARTESIAN_POINT('Ctrl Pts',(13.5419478051625,-69.840972101856,12.));
#66804=CARTESIAN_POINT('Ctrl Pts',(13.5311698283339,-69.8214874767944,12.));
#66805=CARTESIAN_POINT('Ctrl Pts',(13.5204341635507,-69.8020327630205,12.));
#66806=CARTESIAN_POINT('Ctrl Pts',(13.5097408179479,-69.7826081213576,12.));
#66807=CARTESIAN_POINT('Ctrl Pts',(13.4990897985904,-69.7632137134249,12.));
#66808=CARTESIAN_POINT('Ctrl Pts',(13.4884811124748,-69.7438497016406,12.));
#66809=CARTESIAN_POINT('Ctrl Pts',(13.4779147665285,-69.724516249225,12.));
#66810=CARTESIAN_POINT('Ctrl Pts',(13.4673907676044,-69.7052135201998,12.));
#66811=CARTESIAN_POINT('Ctrl Pts',(13.456909122476,-69.6859416793886,12.));
#66812=CARTESIAN_POINT('Ctrl Pts',(13.4464698378453,-69.666700892444,12.));
#66813=CARTESIAN_POINT('Ctrl Pts',(13.4360729203442,-69.6474913258675,12.));
#66814=CARTESIAN_POINT('Ctrl Pts',(13.4257183765341,-69.6283131470273,12.));
#66815=CARTESIAN_POINT('Ctrl Pts',(13.4154062129002,-69.6091665241765,12.));
#66816=CARTESIAN_POINT('Ctrl Pts',(13.4051364358499,-69.5900516264553,12.));
#66817=CARTESIAN_POINT('Ctrl Pts',(13.3949090517177,-69.5709686238724,12.));
#66818=CARTESIAN_POINT('Ctrl Pts',(13.3847240667627,-69.5519176872862,12.));
#66819=CARTESIAN_POINT('Ctrl Pts',(13.3745814871664,-69.5328989883885,12.));
#66820=CARTESIAN_POINT('Ctrl Pts',(13.3644813190219,-69.5139126996675,12.));
#66821=CARTESIAN_POINT('Ctrl Pts',(13.3544235683393,-69.4949589944606,12.));
#66822=CARTESIAN_POINT('Ctrl Pts',(13.3444082410543,-69.4760380470365,12.));
#66823=CARTESIAN_POINT('Ctrl Pts',(13.3344353430313,-69.4571500326673,12.));
#66824=CARTESIAN_POINT('Ctrl Pts',(13.3245048800643,-69.4382951276998,12.));
#66825=CARTESIAN_POINT('Ctrl Pts',(13.3146168578743,-69.4194735096265,12.));
#66826=CARTESIAN_POINT('Ctrl Pts',(13.3047712821051,-69.4006853569511,12.));
#66827=CARTESIAN_POINT('Ctrl Pts',(13.2949681583167,-69.3819308490422,12.));
#66828=CARTESIAN_POINT('Ctrl Pts',(13.2852074919765,-69.3632101660066,12.));
#66829=CARTESIAN_POINT('Ctrl Pts',(13.2754892884433,-69.3445234885065,12.));
#66830=CARTESIAN_POINT('Ctrl Pts',(13.265813552961,-69.3258709977382,12.));
#66831=CARTESIAN_POINT('Ctrl Pts',(13.2561802906896,-69.3072528758518,12.));
#66832=CARTESIAN_POINT('Ctrl Pts',(13.2465895067262,-69.2886693063182,12.));
#66833=CARTESIAN_POINT('Ctrl Pts',(13.237041206122,-69.2701204742449,12.));
#66834=CARTESIAN_POINT('Ctrl Pts',(13.2275353939051,-69.2516065668844,12.));
#66835=CARTESIAN_POINT('Ctrl Pts',(13.2180720750594,-69.2331277732861,12.));
#66836=CARTESIAN_POINT('Ctrl Pts',(13.2086512544735,-69.2146842833537,12.));
#66837=CARTESIAN_POINT('Ctrl Pts',(13.1992729368928,-69.1962762870527,12.));
#66838=CARTESIAN_POINT('Ctrl Pts',(13.1899371268683,-69.1779039735996,12.));
#66839=CARTESIAN_POINT('Ctrl Pts',(13.1806438286934,-69.1595675305245,12.));
#66840=CARTESIAN_POINT('Ctrl Pts',(13.1713930465132,-69.1412671454564,12.));
#66841=CARTESIAN_POINT('Ctrl Pts',(13.1621847844528,-69.1230030082573,12.));
#66842=CARTESIAN_POINT('Ctrl Pts',(13.1530190467183,-69.1047753127643,12.));
#66843=CARTESIAN_POINT('Ctrl Pts',(13.1438958377404,-69.0865842593102,12.));
#66844=CARTESIAN_POINT('Ctrl Pts',(13.1348151621834,-69.0684300549477,12.));
#66845=CARTESIAN_POINT('Ctrl Pts',(13.1257770246385,-69.0503129081817,12.));
#66846=CARTESIAN_POINT('Ctrl Pts',(13.1167814293497,-69.0322330243348,12.));
#66847=CARTESIAN_POINT('Ctrl Pts',(13.1078283799722,-69.0141906015113,12.));
#66848=CARTESIAN_POINT('Ctrl Pts',(13.0989178791833,-68.9961858241519,12.));
#66849=CARTESIAN_POINT('Ctrl Pts',(13.090049929053,-68.9782188692581,12.));
#66850=CARTESIAN_POINT('Ctrl Pts',(13.0812245317807,-68.9602899187573,12.));
#66851=CARTESIAN_POINT('Ctrl Pts',(13.072441690283,-68.9423991694492,12.));
#66852=CARTESIAN_POINT('Ctrl Pts',(13.0637014089029,-68.9245468449945,12.));
#66853=CARTESIAN_POINT('Ctrl Pts',(13.0550036938813,-68.9067332040985,12.));
#66854=CARTESIAN_POINT('Ctrl Pts',(13.0463485518206,-68.8889585151585,12.));
#66855=CARTESIAN_POINT('Ctrl Pts',(13.0377359881875,-68.8712230321906,12.));
#66856=CARTESIAN_POINT('Ctrl Pts',(13.0291660060107,-68.8535269726793,12.));
#66857=CARTESIAN_POINT('Ctrl Pts',(13.0206386039691,-68.8358704887468,12.));
#66858=CARTESIAN_POINT('Ctrl Pts',(13.0121537768945,-68.8182536653656,12.));
#66859=CARTESIAN_POINT('Ctrl Pts',(13.0053999700875,-68.804191966902,12.));
#66860=CARTESIAN_POINT('Ctrl Pts',(13.0003537683054,-68.7936635625545,12.));
#66861=CARTESIAN_POINT('Ctrl Pts',(12.9969981460277,-68.7866525680193,12.));
#66862=CARTESIAN_POINT('Ctrl Pts',(12.9953224629497,-68.7831490561748,12.));
#66863=CARTESIAN_POINT('Ctrl Pts',(16.7988252568748,-72.2774028393915,0.));
#66864=CARTESIAN_POINT('Ctrl Pts',(16.7988252568748,-72.2774028393915,4.));
#66865=CARTESIAN_POINT('Ctrl Pts',(16.7988252568748,-72.2774028393915,8.));
#66866=CARTESIAN_POINT('Ctrl Pts',(16.7988252568748,-72.2774028393915,12.));
#66867=CARTESIAN_POINT('Ctrl Pts',(16.7775526720893,-72.3852065198826,0.));
#66868=CARTESIAN_POINT('Ctrl Pts',(16.7775526720893,-72.3852065198826,4.));
#66869=CARTESIAN_POINT('Ctrl Pts',(16.7775526720893,-72.3852065198826,8.));
#66870=CARTESIAN_POINT('Ctrl Pts',(16.7775526720893,-72.3852065198826,12.));
#66871=CARTESIAN_POINT('Ctrl Pts',(16.6758649025558,-72.5605133546291,0.));
#66872=CARTESIAN_POINT('Ctrl Pts',(16.6758649025558,-72.5605133546291,4.));
#66873=CARTESIAN_POINT('Ctrl Pts',(16.6758649025558,-72.5605133546291,7.99999999999999));
#66874=CARTESIAN_POINT('Ctrl Pts',(16.6758649025558,-72.5605133546291,12.));
#66875=CARTESIAN_POINT('Ctrl Pts',(16.4988611391808,-72.6501505354464,0.));
#66876=CARTESIAN_POINT('Ctrl Pts',(16.4988611391808,-72.6501505354464,4.));
#66877=CARTESIAN_POINT('Ctrl Pts',(16.4988611391808,-72.6501505354464,8.00000000000001));
#66878=CARTESIAN_POINT('Ctrl Pts',(16.4988611391808,-72.6501505354464,12.));
#66879=CARTESIAN_POINT('Ctrl Pts',(16.4184755008061,-72.6683126419587,0.));
#66880=CARTESIAN_POINT('Ctrl Pts',(16.4184755008061,-72.6683126419587,4.));
#66881=CARTESIAN_POINT('Ctrl Pts',(16.4184755008061,-72.6683126419587,8.));
#66882=CARTESIAN_POINT('Ctrl Pts',(16.4184755008061,-72.6683126419587,12.));
#66883=CARTESIAN_POINT('',(16.7988252568748,-72.2774028393915,0.));
#66884=CARTESIAN_POINT('',(16.4184755008061,-72.6683126419586,0.));
#66885=CARTESIAN_POINT('Ctrl Pts',(16.7988252568748,-72.2774028393915,2.77555756156289E-16));
#66886=CARTESIAN_POINT('Ctrl Pts',(16.7775526720893,-72.3852065198826,2.77555756156289E-16));
#66887=CARTESIAN_POINT('Ctrl Pts',(16.719445375213,-72.4853818540234,2.77555756156289E-16));
#66888=CARTESIAN_POINT('Ctrl Pts',(16.6367451007558,-72.557583423616,2.77555756156289E-16));
#66889=CARTESIAN_POINT('Ctrl Pts',(16.5747198949129,-72.6117346008104,2.77555756156289E-16));
#66890=CARTESIAN_POINT('Ctrl Pts',(16.4988611391808,-72.6501505354464,2.77555756156289E-16));
#66891=CARTESIAN_POINT('Ctrl Pts',(16.4184755008061,-72.6683126419587,2.77555756156289E-16));
#66892=CARTESIAN_POINT('',(16.4184755008061,-72.6683126419586,12.));
#66893=CARTESIAN_POINT('Ctrl Pts',(16.4184755008061,-72.6683126419587,0.));
#66894=CARTESIAN_POINT('Ctrl Pts',(16.4184755008061,-72.6683126419587,4.));
#66895=CARTESIAN_POINT('Ctrl Pts',(16.4184755008061,-72.6683126419587,8.));
#66896=CARTESIAN_POINT('Ctrl Pts',(16.4184755008061,-72.6683126419587,12.));
#66897=CARTESIAN_POINT('',(16.7988252568748,-72.2774028393915,12.));
#66898=CARTESIAN_POINT('Ctrl Pts',(16.4184755008061,-72.6683126419587,12.));
#66899=CARTESIAN_POINT('Ctrl Pts',(16.4988611391808,-72.6501505354464,12.));
#66900=CARTESIAN_POINT('Ctrl Pts',(16.5747198949129,-72.6117346008104,12.));
#66901=CARTESIAN_POINT('Ctrl Pts',(16.6367451007558,-72.557583423616,12.));
#66902=CARTESIAN_POINT('Ctrl Pts',(16.7194453752131,-72.4853818540234,12.));
#66903=CARTESIAN_POINT('Ctrl Pts',(16.7775526720893,-72.3852065198826,12.));
#66904=CARTESIAN_POINT('Ctrl Pts',(16.7988252568748,-72.2774028393915,12.));
#66905=CARTESIAN_POINT('Ctrl Pts',(16.7988252568748,-72.2774028393915,12.));
#66906=CARTESIAN_POINT('Ctrl Pts',(16.7988252568748,-72.2774028393915,8.));
#66907=CARTESIAN_POINT('Ctrl Pts',(16.7988252568748,-72.2774028393915,4.));
#66908=CARTESIAN_POINT('Ctrl Pts',(16.7988252568748,-72.2774028393915,0.));
#66909=CARTESIAN_POINT('Origin',(8.12279454723525E-11,-3.65936987487134E-10,
0.));
#66910=CARTESIAN_POINT('Origin',(8.12279454723525E-11,-3.65936987487134E-10,
12.));
#66911=CARTESIAN_POINT('Origin',(8.12279454723525E-11,-3.65936987487134E-10,
0.));
#66912=CARTESIAN_POINT('Ctrl Pts',(9.42570643237823,-73.9013264985861,-5.55111512312578E-16));
#66913=CARTESIAN_POINT('Ctrl Pts',(9.42570643237823,-73.9013264985861,4.));
#66914=CARTESIAN_POINT('Ctrl Pts',(9.42570643237823,-73.9013264985861,8.));
#66915=CARTESIAN_POINT('Ctrl Pts',(9.42570643237823,-73.9013264985861,12.));
#66916=CARTESIAN_POINT('Ctrl Pts',(9.31670696907615,-73.9152287787081,-5.55111512312578E-16));
#66917=CARTESIAN_POINT('Ctrl Pts',(9.31670696907615,-73.9152287787081,4.));
#66918=CARTESIAN_POINT('Ctrl Pts',(9.31670696907615,-73.9152287787081,8.00000000000001));
#66919=CARTESIAN_POINT('Ctrl Pts',(9.31670696907615,-73.9152287787081,12.));
#66920=CARTESIAN_POINT('Ctrl Pts',(9.11824194722557,-73.8741839722668,-5.55111512312578E-16));
#66921=CARTESIAN_POINT('Ctrl Pts',(9.11824194722557,-73.8741839722668,4.));
#66922=CARTESIAN_POINT('Ctrl Pts',(9.11824194722557,-73.8741839722668,7.99999999999999));
#66923=CARTESIAN_POINT('Ctrl Pts',(9.11824194722557,-73.8741839722668,12.));
#66924=CARTESIAN_POINT('Ctrl Pts',(8.97724108745579,-73.734598722692,-5.55111512312578E-16));
#66925=CARTESIAN_POINT('Ctrl Pts',(8.97724108745579,-73.734598722692,4.));
#66926=CARTESIAN_POINT('Ctrl Pts',(8.97724108745578,-73.734598722692,8.00000000000001));
#66927=CARTESIAN_POINT('Ctrl Pts',(8.97724108745578,-73.734598722692,12.));
#66928=CARTESIAN_POINT('Ctrl Pts',(8.93459554655837,-73.6640787197675,-5.55111512312578E-16));
#66929=CARTESIAN_POINT('Ctrl Pts',(8.93459554655837,-73.6640787197675,4.));
#66930=CARTESIAN_POINT('Ctrl Pts',(8.93459554655836,-73.6640787197675,8.));
#66931=CARTESIAN_POINT('Ctrl Pts',(8.93459554655836,-73.6640787197675,12.));
#66932=CARTESIAN_POINT('',(9.42570643237823,-73.9013264985861,0.));
#66933=CARTESIAN_POINT('',(8.93459554655838,-73.6640787197675,0.));
#66934=CARTESIAN_POINT('Ctrl Pts',(9.42570643237823,-73.9013264985861,4.16333634234434E-16));
#66935=CARTESIAN_POINT('Ctrl Pts',(9.31670696907615,-73.9152287787081,4.16333634234434E-16));
#66936=CARTESIAN_POINT('Ctrl Pts',(9.20329838516153,-73.8917746035988,4.16333634234434E-16));
#66937=CARTESIAN_POINT('Ctrl Pts',(9.1086536092733,-73.8361439572622,4.16333634234434E-16));
#66938=CARTESIAN_POINT('Ctrl Pts',(9.03767002735712,-73.7944209725098,4.16333634234434E-16));
#66939=CARTESIAN_POINT('Ctrl Pts',(8.97724108745579,-73.734598722692,4.16333634234433E-16));
#66940=CARTESIAN_POINT('Ctrl Pts',(8.93459554655837,-73.6640787197675,4.16333634234434E-16));
#66941=CARTESIAN_POINT('',(8.93459554655838,-73.6640787197675,12.));
#66942=CARTESIAN_POINT('Ctrl Pts',(8.93459554655837,-73.6640787197675,-5.55111512312578E-16));
#66943=CARTESIAN_POINT('Ctrl Pts',(8.93459554655837,-73.6640787197675,4.));
#66944=CARTESIAN_POINT('Ctrl Pts',(8.93459554655836,-73.6640787197675,8.));
#66945=CARTESIAN_POINT('Ctrl Pts',(8.93459554655836,-73.6640787197675,12.));
#66946=CARTESIAN_POINT('',(9.42570643237823,-73.9013264985861,12.));
#66947=CARTESIAN_POINT('Ctrl Pts',(8.93459554655836,-73.6640787197675,12.));
#66948=CARTESIAN_POINT('Ctrl Pts',(8.97724108745578,-73.734598722692,12.));
#66949=CARTESIAN_POINT('Ctrl Pts',(9.03767002735712,-73.7944209725098,12.));
#66950=CARTESIAN_POINT('Ctrl Pts',(9.10865360927329,-73.8361439572622,12.));
#66951=CARTESIAN_POINT('Ctrl Pts',(9.20329838516153,-73.8917746035988,12.));
#66952=CARTESIAN_POINT('Ctrl Pts',(9.31670696907615,-73.9152287787081,12.));
#66953=CARTESIAN_POINT('Ctrl Pts',(9.42570643237823,-73.9013264985861,12.));
#66954=CARTESIAN_POINT('Ctrl Pts',(9.42570643237823,-73.9013264985861,12.));
#66955=CARTESIAN_POINT('Ctrl Pts',(9.42570643237823,-73.9013264985861,8.));
#66956=CARTESIAN_POINT('Ctrl Pts',(9.42570643237823,-73.9013264985861,4.));
#66957=CARTESIAN_POINT('Ctrl Pts',(9.42570643237823,-73.9013264985861,-5.55111512312578E-16));
#66958=CARTESIAN_POINT('Ctrl Pts',(6.95102489306925,-69.6540253893192,0.));
#66959=CARTESIAN_POINT('Ctrl Pts',(6.95102489306925,-69.6540253893192,12.));
#66960=CARTESIAN_POINT('Ctrl Pts',(6.95238884849024,-69.6576616146467,0.));
#66961=CARTESIAN_POINT('Ctrl Pts',(6.95238884849024,-69.6576616146467,12.));
#66962=CARTESIAN_POINT('Ctrl Pts',(6.95512065317599,-69.664938391983,0.));
#66963=CARTESIAN_POINT('Ctrl Pts',(6.95512065317599,-69.664938391983,12.));
#66964=CARTESIAN_POINT('Ctrl Pts',(6.9592300417359,-69.6758665380378,0.));
#66965=CARTESIAN_POINT('Ctrl Pts',(6.9592300417359,-69.6758665380378,12.));
#66966=CARTESIAN_POINT('Ctrl Pts',(6.96473259049512,-69.6904633605421,0.));
#66967=CARTESIAN_POINT('Ctrl Pts',(6.96473259049512,-69.6904633605421,12.));
#66968=CARTESIAN_POINT('Ctrl Pts',(6.97164972291439,-69.7087526479973,0.));
#66969=CARTESIAN_POINT('Ctrl Pts',(6.97164972291439,-69.7087526479973,12.));
#66970=CARTESIAN_POINT('Ctrl Pts',(6.97860581164526,-69.7270851557366,0.));
#66971=CARTESIAN_POINT('Ctrl Pts',(6.97860581164526,-69.7270851557366,12.));
#66972=CARTESIAN_POINT('Ctrl Pts',(6.98560086924213,-69.7454607995607,0.));
#66973=CARTESIAN_POINT('Ctrl Pts',(6.98560086924213,-69.7454607995607,12.));
#66974=CARTESIAN_POINT('Ctrl Pts',(6.9926349102794,-69.7638794280419,0.));
#66975=CARTESIAN_POINT('Ctrl Pts',(6.9926349102794,-69.7638794280419,12.));
#66976=CARTESIAN_POINT('Ctrl Pts',(6.99970795069475,-69.782340824259,0.));
#66977=CARTESIAN_POINT('Ctrl Pts',(6.99970795069475,-69.782340824259,12.));
#66978=CARTESIAN_POINT('Ctrl Pts',(7.0068200071815,-69.8008447346863,0.));
#66979=CARTESIAN_POINT('Ctrl Pts',(7.0068200071815,-69.8008447346863,12.));
#66980=CARTESIAN_POINT('Ctrl Pts',(7.01397109655454,-69.8193908913722,0.));
#66981=CARTESIAN_POINT('Ctrl Pts',(7.01397109655454,-69.8193908913722,12.));
#66982=CARTESIAN_POINT('Ctrl Pts',(7.02116123514451,-69.8379790360518,0.));
#66983=CARTESIAN_POINT('Ctrl Pts',(7.02116123514451,-69.8379790360518,12.));
#66984=CARTESIAN_POINT('Ctrl Pts',(7.02839043811812,-69.8566089455375,0.));
#66985=CARTESIAN_POINT('Ctrl Pts',(7.02839043811812,-69.8566089455375,12.));
#66986=CARTESIAN_POINT('Ctrl Pts',(7.0356587197222,-69.8752804235238,0.));
#66987=CARTESIAN_POINT('Ctrl Pts',(7.0356587197222,-69.8752804235238,12.));
#66988=CARTESIAN_POINT('Ctrl Pts',(7.04296609362165,-69.8939932885841,0.));
#66989=CARTESIAN_POINT('Ctrl Pts',(7.04296609362165,-69.8939932885841,12.));
#66990=CARTESIAN_POINT('Ctrl Pts',(7.05031257318115,-69.9127473642099,0.));
#66991=CARTESIAN_POINT('Ctrl Pts',(7.05031257318115,-69.9127473642099,12.));
#66992=CARTESIAN_POINT('Ctrl Pts',(7.05769817180856,-69.9315424664291,0.));
#66993=CARTESIAN_POINT('Ctrl Pts',(7.05769817180856,-69.9315424664291,12.));
#66994=CARTESIAN_POINT('Ctrl Pts',(7.06512290312849,-69.9503783975727,0.));
#66995=CARTESIAN_POINT('Ctrl Pts',(7.06512290312849,-69.9503783975727,12.));
#66996=CARTESIAN_POINT('Ctrl Pts',(7.0725867808083,-69.9692549527296,0.));
#66997=CARTESIAN_POINT('Ctrl Pts',(7.0725867808083,-69.9692549527296,12.));
#66998=CARTESIAN_POINT('Ctrl Pts',(7.08008981844651,-69.988171923788,0.));
#66999=CARTESIAN_POINT('Ctrl Pts',(7.08008981844651,-69.988171923788,12.));
#67000=CARTESIAN_POINT('Ctrl Pts',(7.08763202944245,-70.0071291040766,0.));
#67001=CARTESIAN_POINT('Ctrl Pts',(7.08763202944245,-70.0071291040766,12.));
#67002=CARTESIAN_POINT('Ctrl Pts',(7.09521342684248,-70.0261262936388,0.));
#67003=CARTESIAN_POINT('Ctrl Pts',(7.09521342684248,-70.0261262936388,12.));
#67004=CARTESIAN_POINT('Ctrl Pts',(7.10283402335033,-70.0451632990086,0.));
#67005=CARTESIAN_POINT('Ctrl Pts',(7.10283402335033,-70.0451632990086,12.));
#67006=CARTESIAN_POINT('Ctrl Pts',(7.11049383140445,-70.0642399306869,0.));
#67007=CARTESIAN_POINT('Ctrl Pts',(7.11049383140445,-70.0642399306869,12.));
#67008=CARTESIAN_POINT('Ctrl Pts',(7.11819286322825,-70.0833560013975,0.));
#67009=CARTESIAN_POINT('Ctrl Pts',(7.11819286322825,-70.0833560013975,12.));
#67010=CARTESIAN_POINT('Ctrl Pts',(7.12593113088903,-70.1025113239495,0.));
#67011=CARTESIAN_POINT('Ctrl Pts',(7.12593113088903,-70.1025113239495,12.));
#67012=CARTESIAN_POINT('Ctrl Pts',(7.13370864634442,-70.1217057094499,0.));
#67013=CARTESIAN_POINT('Ctrl Pts',(7.13370864634442,-70.1217057094499,12.));
#67014=CARTESIAN_POINT('Ctrl Pts',(7.14152542142373,-70.1409389682424,0.));
#67015=CARTESIAN_POINT('Ctrl Pts',(7.14152542142373,-70.1409389682424,12.));
#67016=CARTESIAN_POINT('Ctrl Pts',(7.14938146780813,-70.1602109107202,0.));
#67017=CARTESIAN_POINT('Ctrl Pts',(7.14938146780813,-70.1602109107202,12.));
#67018=CARTESIAN_POINT('Ctrl Pts',(7.15727679700932,-70.1795213481185,0.));
#67019=CARTESIAN_POINT('Ctrl Pts',(7.15727679700932,-70.1795213481185,12.));
#67020=CARTESIAN_POINT('Ctrl Pts',(7.16521142033863,-70.1988700934593,0.));
#67021=CARTESIAN_POINT('Ctrl Pts',(7.16521142033863,-70.1988700934593,12.));
#67022=CARTESIAN_POINT('Ctrl Pts',(7.17318534889715,-70.2182569618994,0.));
#67023=CARTESIAN_POINT('Ctrl Pts',(7.17318534889715,-70.2182569618994,12.));
#67024=CARTESIAN_POINT('Ctrl Pts',(7.18119859359777,-70.2376817702215,0.));
#67025=CARTESIAN_POINT('Ctrl Pts',(7.18119859359777,-70.2376817702215,12.));
#67026=CARTESIAN_POINT('Ctrl Pts',(7.18925116517554,-70.2571443365192,0.));
#67027=CARTESIAN_POINT('Ctrl Pts',(7.18925116517554,-70.2571443365192,12.));
#67028=CARTESIAN_POINT('Ctrl Pts',(7.19734307419872,-70.2766444798285,0.));
#67029=CARTESIAN_POINT('Ctrl Pts',(7.19734307419872,-70.2766444798285,12.));
#67030=CARTESIAN_POINT('Ctrl Pts',(7.20547433107482,-70.2961820197077,0.));
#67031=CARTESIAN_POINT('Ctrl Pts',(7.20547433107482,-70.2961820197077,12.));
#67032=CARTESIAN_POINT('Ctrl Pts',(7.21364494605449,-70.3157567762588,0.));
#67033=CARTESIAN_POINT('Ctrl Pts',(7.21364494605449,-70.3157567762588,12.));
#67034=CARTESIAN_POINT('Ctrl Pts',(7.2218549292319,-70.3353685703112,0.));
#67035=CARTESIAN_POINT('Ctrl Pts',(7.2218549292319,-70.3353685703112,12.));
#67036=CARTESIAN_POINT('Ctrl Pts',(7.23010429054228,-70.3550172235486,0.));
#67037=CARTESIAN_POINT('Ctrl Pts',(7.23010429054228,-70.3550172235486,12.));
#67038=CARTESIAN_POINT('Ctrl Pts',(7.23839303975606,-70.3747025586552,0.));
#67039=CARTESIAN_POINT('Ctrl Pts',(7.23839303975606,-70.3747025586552,12.));
#67040=CARTESIAN_POINT('Ctrl Pts',(7.24672118647084,-70.3944243994504,0.));
#67041=CARTESIAN_POINT('Ctrl Pts',(7.24672118647084,-70.3944243994504,12.));
#67042=CARTESIAN_POINT('Ctrl Pts',(7.25508874012042,-70.4141825708178,0.));
#67043=CARTESIAN_POINT('Ctrl Pts',(7.25508874012042,-70.4141825708178,12.));
#67044=CARTESIAN_POINT('Ctrl Pts',(7.26349570998032,-70.4339768986346,0.));
#67045=CARTESIAN_POINT('Ctrl Pts',(7.26349570998032,-70.4339768986346,12.));
#67046=CARTESIAN_POINT('Ctrl Pts',(7.27194210517062,-70.4538072096992,0.));
#67047=CARTESIAN_POINT('Ctrl Pts',(7.27194210517062,-70.4538072096992,12.));
#67048=CARTESIAN_POINT('Ctrl Pts',(7.2804279346547,-70.4736733316487,0.));
#67049=CARTESIAN_POINT('Ctrl Pts',(7.2804279346547,-70.4736733316487,12.));
#67050=CARTESIAN_POINT('Ctrl Pts',(7.28895320723861,-70.4935750929058,0.));
#67051=CARTESIAN_POINT('Ctrl Pts',(7.28895320723861,-70.4935750929058,12.));
#67052=CARTESIAN_POINT('Ctrl Pts',(7.29751793157822,-70.5135123227169,0.));
#67053=CARTESIAN_POINT('Ctrl Pts',(7.29751793157822,-70.5135123227169,12.));
#67054=CARTESIAN_POINT('Ctrl Pts',(7.30612211618052,-70.5334848511681,0.));
#67055=CARTESIAN_POINT('Ctrl Pts',(7.30612211618052,-70.5334848511681,12.));
#67056=CARTESIAN_POINT('Ctrl Pts',(7.31476576940391,-70.5534925092043,0.));
#67057=CARTESIAN_POINT('Ctrl Pts',(7.31476576940391,-70.5534925092043,12.));
#67058=CARTESIAN_POINT('Ctrl Pts',(7.32344889945219,-70.5735351286476,0.));
#67059=CARTESIAN_POINT('Ctrl Pts',(7.32344889945219,-70.5735351286476,12.));
#67060=CARTESIAN_POINT('Ctrl Pts',(7.3321715143759,-70.5936125421946,0.));
#67061=CARTESIAN_POINT('Ctrl Pts',(7.3321715143759,-70.5936125421946,12.));
#67062=CARTESIAN_POINT('Ctrl Pts',(7.34093362208007,-70.6137245833996,0.));
#67063=CARTESIAN_POINT('Ctrl Pts',(7.34093362208007,-70.6137245833996,12.));
#67064=CARTESIAN_POINT('Ctrl Pts',(7.34973523032577,-70.6338710866562,0.));
#67065=CARTESIAN_POINT('Ctrl Pts',(7.34973523032577,-70.6338710866562,12.));
#67066=CARTESIAN_POINT('Ctrl Pts',(7.35857634673054,-70.6540518871775,0.));
#67067=CARTESIAN_POINT('Ctrl Pts',(7.35857634673054,-70.6540518871775,12.));
#67068=CARTESIAN_POINT('Ctrl Pts',(7.367456978763,-70.6742668209687,0.));
#67069=CARTESIAN_POINT('Ctrl Pts',(7.367456978763,-70.6742668209687,12.));
#67070=CARTESIAN_POINT('Ctrl Pts',(7.37637713374767,-70.694515724827,0.));
#67071=CARTESIAN_POINT('Ctrl Pts',(7.37637713374767,-70.694515724827,12.));
#67072=CARTESIAN_POINT('Ctrl Pts',(7.38533681887032,-70.7147984363424,0.));
#67073=CARTESIAN_POINT('Ctrl Pts',(7.38533681887032,-70.7147984363424,12.));
#67074=CARTESIAN_POINT('Ctrl Pts',(7.3943360411789,-70.735114793895,0.));
#67075=CARTESIAN_POINT('Ctrl Pts',(7.3943360411789,-70.735114793895,12.));
#67076=CARTESIAN_POINT('Ctrl Pts',(7.40337480758229,-70.7554646366514,0.));
#67077=CARTESIAN_POINT('Ctrl Pts',(7.40337480758229,-70.7554646366514,12.));
#67078=CARTESIAN_POINT('Ctrl Pts',(7.41245312484486,-70.7758478045576,0.));
#67079=CARTESIAN_POINT('Ctrl Pts',(7.41245312484486,-70.7758478045576,12.));
#67080=CARTESIAN_POINT('Ctrl Pts',(7.42157099959315,-70.7962641383351,0.));
#67081=CARTESIAN_POINT('Ctrl Pts',(7.42157099959315,-70.7962641383351,12.));
#67082=CARTESIAN_POINT('Ctrl Pts',(7.43072843832007,-70.8167134794738,0.));
#67083=CARTESIAN_POINT('Ctrl Pts',(7.43072843832007,-70.8167134794738,12.));
#67084=CARTESIAN_POINT('Ctrl Pts',(7.43992544738606,-70.8371956702242,0.));
#67085=CARTESIAN_POINT('Ctrl Pts',(7.43992544738606,-70.8371956702242,12.));
#67086=CARTESIAN_POINT('Ctrl Pts',(7.44916203301644,-70.8577105535841,0.));
#67087=CARTESIAN_POINT('Ctrl Pts',(7.44916203301644,-70.8577105535841,12.));
#67088=CARTESIAN_POINT('Ctrl Pts',(7.45843820129775,-70.8782579732885,0.));
#67089=CARTESIAN_POINT('Ctrl Pts',(7.45843820129775,-70.8782579732885,12.));
#67090=CARTESIAN_POINT('Ctrl Pts',(7.46775395818518,-70.8988377738088,0.));
#67091=CARTESIAN_POINT('Ctrl Pts',(7.46775395818518,-70.8988377738088,12.));
#67092=CARTESIAN_POINT('Ctrl Pts',(7.47710930950553,-70.9194498003483,0.));
#67093=CARTESIAN_POINT('Ctrl Pts',(7.47710930950553,-70.9194498003483,12.));
#67094=CARTESIAN_POINT('Ctrl Pts',(7.48650426095822,-70.9400938988373,0.));
#67095=CARTESIAN_POINT('Ctrl Pts',(7.48650426095822,-70.9400938988373,12.));
#67096=CARTESIAN_POINT('Ctrl Pts',(7.49593881811141,-70.9607699159234,0.));
#67097=CARTESIAN_POINT('Ctrl Pts',(7.49593881811141,-70.9607699159234,12.));
#67098=CARTESIAN_POINT('Ctrl Pts',(7.50541298639948,-70.9814776989637,0.));
#67099=CARTESIAN_POINT('Ctrl Pts',(7.50541298639948,-70.9814776989637,12.));
#67100=CARTESIAN_POINT('Ctrl Pts',(7.51492677113111,-71.0022170960235,0.));
#67101=CARTESIAN_POINT('Ctrl Pts',(7.51492677113111,-71.0022170960235,12.));
#67102=CARTESIAN_POINT('Ctrl Pts',(7.52448017749135,-71.0229879558713,0.));
#67103=CARTESIAN_POINT('Ctrl Pts',(7.52448017749135,-71.0229879558713,12.));
#67104=CARTESIAN_POINT('Ctrl Pts',(7.53407321054253,-71.0437901279722,0.));
#67105=CARTESIAN_POINT('Ctrl Pts',(7.53407321054253,-71.0437901279722,12.));
#67106=CARTESIAN_POINT('Ctrl Pts',(7.54370587521947,-71.0646234624783,0.));
#67107=CARTESIAN_POINT('Ctrl Pts',(7.54370587521947,-71.0646234624783,12.));
#67108=CARTESIAN_POINT('Ctrl Pts',(7.55337817632872,-71.0854878102203,0.));
#67109=CARTESIAN_POINT('Ctrl Pts',(7.55337817632872,-71.0854878102203,12.));
#67110=CARTESIAN_POINT('Ctrl Pts',(7.56309011855616,-71.1063830227074,0.));
#67111=CARTESIAN_POINT('Ctrl Pts',(7.56309011855616,-71.1063830227074,12.));
#67112=CARTESIAN_POINT('Ctrl Pts',(7.57284170646865,-71.1273089521218,0.));
#67113=CARTESIAN_POINT('Ctrl Pts',(7.57284170646865,-71.1273089521218,12.));
#67114=CARTESIAN_POINT('Ctrl Pts',(7.58263294451465,-71.1482654513133,0.));
#67115=CARTESIAN_POINT('Ctrl Pts',(7.58263294451465,-71.1482654513133,12.));
#67116=CARTESIAN_POINT('Ctrl Pts',(7.59246383701859,-71.1692523737887,0.));
#67117=CARTESIAN_POINT('Ctrl Pts',(7.59246383701859,-71.1692523737887,12.));
#67118=CARTESIAN_POINT('Ctrl Pts',(7.60233438818156,-71.1902695737063,0.));
#67119=CARTESIAN_POINT('Ctrl Pts',(7.60233438818156,-71.1902695737063,12.));
#67120=CARTESIAN_POINT('Ctrl Pts',(7.61224460208886,-71.2113169058778,0.));
#67121=CARTESIAN_POINT('Ctrl Pts',(7.61224460208886,-71.2113169058778,12.));
#67122=CARTESIAN_POINT('Ctrl Pts',(7.62219448271124,-71.232394225762,0.));
#67123=CARTESIAN_POINT('Ctrl Pts',(7.62219448271124,-71.232394225762,12.));
#67124=CARTESIAN_POINT('Ctrl Pts',(7.63218403390514,-71.2535013894587,0.));
#67125=CARTESIAN_POINT('Ctrl Pts',(7.63218403390514,-71.2535013894587,12.));
#67126=CARTESIAN_POINT('Ctrl Pts',(7.64221325940671,-71.2746382536974,0.));
#67127=CARTESIAN_POINT('Ctrl Pts',(7.64221325940671,-71.2746382536974,12.));
#67128=CARTESIAN_POINT('Ctrl Pts',(7.65228216283342,-71.2958046758334,0.));
#67129=CARTESIAN_POINT('Ctrl Pts',(7.65228216283342,-71.2958046758334,12.));
#67130=CARTESIAN_POINT('Ctrl Pts',(7.66239074769118,-71.3170005138474,0.));
#67131=CARTESIAN_POINT('Ctrl Pts',(7.66239074769118,-71.3170005138474,12.));
#67132=CARTESIAN_POINT('Ctrl Pts',(7.67253901737539,-71.3382256263405,0.));
#67133=CARTESIAN_POINT('Ctrl Pts',(7.67253901737539,-71.3382256263405,12.));
#67134=CARTESIAN_POINT('Ctrl Pts',(7.68272697517102,-71.3594798725294,0.));
#67135=CARTESIAN_POINT('Ctrl Pts',(7.68272697517102,-71.3594798725294,12.));
#67136=CARTESIAN_POINT('Ctrl Pts',(7.69295462424646,-71.380763112236,0.));
#67137=CARTESIAN_POINT('Ctrl Pts',(7.69295462424646,-71.380763112236,12.));
#67138=CARTESIAN_POINT('Ctrl Pts',(7.70322196765572,-71.4020752058827,0.));
#67139=CARTESIAN_POINT('Ctrl Pts',(7.70322196765572,-71.4020752058827,12.));
#67140=CARTESIAN_POINT('Ctrl Pts',(7.71352900834537,-71.4234160144943,0.));
#67141=CARTESIAN_POINT('Ctrl Pts',(7.71352900834537,-71.4234160144943,12.));
#67142=CARTESIAN_POINT('Ctrl Pts',(7.72387574915544,-71.4447853996919,0.));
#67143=CARTESIAN_POINT('Ctrl Pts',(7.72387574915544,-71.4447853996919,12.));
#67144=CARTESIAN_POINT('Ctrl Pts',(7.73426219281931,-71.4661832236881,0.));
#67145=CARTESIAN_POINT('Ctrl Pts',(7.73426219281931,-71.4661832236881,12.));
#67146=CARTESIAN_POINT('Ctrl Pts',(7.74468834195734,-71.487609349277,0.));
#67147=CARTESIAN_POINT('Ctrl Pts',(7.74468834195734,-71.487609349277,12.));
#67148=CARTESIAN_POINT('Ctrl Pts',(7.75515419907954,-71.5090636398307,0.));
#67149=CARTESIAN_POINT('Ctrl Pts',(7.75515419907954,-71.5090636398307,12.));
#67150=CARTESIAN_POINT('Ctrl Pts',(7.76565976659218,-71.5305459592987,0.));
#67151=CARTESIAN_POINT('Ctrl Pts',(7.76565976659218,-71.5305459592987,12.));
#67152=CARTESIAN_POINT('Ctrl Pts',(7.77620504679867,-71.5520561722039,0.));
#67153=CARTESIAN_POINT('Ctrl Pts',(7.77620504679867,-71.5520561722039,12.));
#67154=CARTESIAN_POINT('Ctrl Pts',(7.78679004189934,-71.5735941436366,0.));
#67155=CARTESIAN_POINT('Ctrl Pts',(7.78679004189934,-71.5735941436366,12.));
#67156=CARTESIAN_POINT('Ctrl Pts',(7.79741475398511,-71.5951597392471,0.));
#67157=CARTESIAN_POINT('Ctrl Pts',(7.79741475398511,-71.5951597392471,12.));
#67158=CARTESIAN_POINT('Ctrl Pts',(7.80807918504016,-71.616752825242,0.));
#67159=CARTESIAN_POINT('Ctrl Pts',(7.80807918504016,-71.616752825242,12.));
#67160=CARTESIAN_POINT('Ctrl Pts',(7.81878333694855,-71.638373268384,0.));
#67161=CARTESIAN_POINT('Ctrl Pts',(7.81878333694855,-71.638373268384,12.));
#67162=CARTESIAN_POINT('Ctrl Pts',(7.82952721149503,-71.6600209359869,0.));
#67163=CARTESIAN_POINT('Ctrl Pts',(7.82952721149503,-71.6600209359869,12.));
#67164=CARTESIAN_POINT('Ctrl Pts',(7.84031081036488,-71.681695695912,0.));
#67165=CARTESIAN_POINT('Ctrl Pts',(7.84031081036488,-71.681695695912,12.));
#67166=CARTESIAN_POINT('Ctrl Pts',(7.85113413513738,-71.7033974165576,0.));
#67167=CARTESIAN_POINT('Ctrl Pts',(7.85113413513738,-71.7033974165576,12.));
#67168=CARTESIAN_POINT('Ctrl Pts',(7.86199718728829,-71.7251259668573,0.));
#67169=CARTESIAN_POINT('Ctrl Pts',(7.86199718728829,-71.7251259668573,12.));
#67170=CARTESIAN_POINT('Ctrl Pts',(7.87289996819653,-71.7468812162795,0.));
#67171=CARTESIAN_POINT('Ctrl Pts',(7.87289996819653,-71.7468812162795,12.));
#67172=CARTESIAN_POINT('Ctrl Pts',(7.88384247914521,-71.768663034824,0.));
#67173=CARTESIAN_POINT('Ctrl Pts',(7.88384247914521,-71.768663034824,12.));
#67174=CARTESIAN_POINT('Ctrl Pts',(7.89482472132134,-71.7904712930172,0.));
#67175=CARTESIAN_POINT('Ctrl Pts',(7.89482472132134,-71.7904712930172,12.));
#67176=CARTESIAN_POINT('Ctrl Pts',(7.90584669580955,-71.8123058619038,0.));
#67177=CARTESIAN_POINT('Ctrl Pts',(7.90584669580955,-71.8123058619038,12.));
#67178=CARTESIAN_POINT('Ctrl Pts',(7.9169084035937,-71.8341666130424,0.));
#67179=CARTESIAN_POINT('Ctrl Pts',(7.9169084035937,-71.8341666130424,12.));
#67180=CARTESIAN_POINT('Ctrl Pts',(7.92800984556399,-71.8560534185071,0.));
#67181=CARTESIAN_POINT('Ctrl Pts',(7.92800984556399,-71.8560534185071,12.));
#67182=CARTESIAN_POINT('Ctrl Pts',(7.93915102251795,-71.8779661508833,0.));
#67183=CARTESIAN_POINT('Ctrl Pts',(7.93915102251795,-71.8779661508833,12.));
#67184=CARTESIAN_POINT('Ctrl Pts',(7.95033193516045,-71.8999046832642,0.));
#67185=CARTESIAN_POINT('Ctrl Pts',(7.95033193516045,-71.8999046832642,12.));
#67186=CARTESIAN_POINT('Ctrl Pts',(7.96155258409751,-71.9218688892426,0.));
#67187=CARTESIAN_POINT('Ctrl Pts',(7.96155258409751,-71.9218688892426,12.));
#67188=CARTESIAN_POINT('Ctrl Pts',(7.97281296983701,-71.9438586429072,0.));
#67189=CARTESIAN_POINT('Ctrl Pts',(7.97281296983701,-71.9438586429072,12.));
#67190=CARTESIAN_POINT('Ctrl Pts',(7.98411309279597,-71.9658738188421,0.));
#67191=CARTESIAN_POINT('Ctrl Pts',(7.98411309279597,-71.9658738188421,12.));
#67192=CARTESIAN_POINT('Ctrl Pts',(7.99545295330181,-71.9879142921248,0.));
#67193=CARTESIAN_POINT('Ctrl Pts',(7.99545295330181,-71.9879142921248,12.));
#67194=CARTESIAN_POINT('Ctrl Pts',(8.00683255159249,-72.0099799383216,0.));
#67195=CARTESIAN_POINT('Ctrl Pts',(8.00683255159249,-72.0099799383216,12.));
#67196=CARTESIAN_POINT('Ctrl Pts',(8.01825188781069,-72.0320706334802,0.));
#67197=CARTESIAN_POINT('Ctrl Pts',(8.01825188781069,-72.0320706334802,12.));
#67198=CARTESIAN_POINT('Ctrl Pts',(8.02971096200327,-72.0541862541262,0.));
#67199=CARTESIAN_POINT('Ctrl Pts',(8.02971096200327,-72.0541862541262,12.));
#67200=CARTESIAN_POINT('Ctrl Pts',(8.04120977412891,-72.0763266772632,0.));
#67201=CARTESIAN_POINT('Ctrl Pts',(8.04120977412891,-72.0763266772632,12.));
#67202=CARTESIAN_POINT('Ctrl Pts',(8.05274832405956,-72.0984917803702,0.));
#67203=CARTESIAN_POINT('Ctrl Pts',(8.05274832405956,-72.0984917803702,12.));
#67204=CARTESIAN_POINT('Ctrl Pts',(8.06432661158088,-72.1206814413985,0.));
#67205=CARTESIAN_POINT('Ctrl Pts',(8.06432661158088,-72.1206814413985,12.));
#67206=CARTESIAN_POINT('Ctrl Pts',(8.07594463638699,-72.1428955387648,0.));
#67207=CARTESIAN_POINT('Ctrl Pts',(8.07594463638699,-72.1428955387648,12.));
#67208=CARTESIAN_POINT('Ctrl Pts',(8.08760239807814,-72.165133951346,0.));
#67209=CARTESIAN_POINT('Ctrl Pts',(8.08760239807814,-72.165133951346,12.));
#67210=CARTESIAN_POINT('Ctrl Pts',(8.09929989616873,-72.18739655848,0.));
#67211=CARTESIAN_POINT('Ctrl Pts',(8.09929989616873,-72.18739655848,12.));
#67212=CARTESIAN_POINT('Ctrl Pts',(8.11103713008921,-72.2096832399626,0.));
#67213=CARTESIAN_POINT('Ctrl Pts',(8.11103713008921,-72.2096832399626,12.));
#67214=CARTESIAN_POINT('Ctrl Pts',(8.12281409918661,-72.2319938760451,0.));
#67215=CARTESIAN_POINT('Ctrl Pts',(8.12281409918661,-72.2319938760451,12.));
#67216=CARTESIAN_POINT('Ctrl Pts',(8.13463080272028,-72.2543283474279,0.));
#67217=CARTESIAN_POINT('Ctrl Pts',(8.13463080272028,-72.2543283474279,12.));
#67218=CARTESIAN_POINT('Ctrl Pts',(8.14648723985792,-72.2766865352552,0.));
#67219=CARTESIAN_POINT('Ctrl Pts',(8.14648723985792,-72.2766865352552,12.));
#67220=CARTESIAN_POINT('Ctrl Pts',(8.15838340968327,-72.2990683211155,0.));
#67221=CARTESIAN_POINT('Ctrl Pts',(8.15838340968327,-72.2990683211155,12.));
#67222=CARTESIAN_POINT('Ctrl Pts',(8.17031931119881,-72.3214735870402,0.));
#67223=CARTESIAN_POINT('Ctrl Pts',(8.17031931119881,-72.3214735870402,12.));
#67224=CARTESIAN_POINT('Ctrl Pts',(8.18229494332621,-72.3439022155007,0.));
#67225=CARTESIAN_POINT('Ctrl Pts',(8.18229494332621,-72.3439022155007,12.));
#67226=CARTESIAN_POINT('Ctrl Pts',(8.19431030490318,-72.3663540894034,0.));
#67227=CARTESIAN_POINT('Ctrl Pts',(8.19431030490318,-72.3663540894034,12.));
#67228=CARTESIAN_POINT('Ctrl Pts',(8.20636539467781,-72.3888290920845,0.));
#67229=CARTESIAN_POINT('Ctrl Pts',(8.20636539467781,-72.3888290920845,12.));
#67230=CARTESIAN_POINT('Ctrl Pts',(8.21846021131563,-72.4113271073091,0.));
#67231=CARTESIAN_POINT('Ctrl Pts',(8.21846021131563,-72.4113271073091,12.));
#67232=CARTESIAN_POINT('Ctrl Pts',(8.23059475340354,-72.4338480192701,0.));
#67233=CARTESIAN_POINT('Ctrl Pts',(8.23059475340354,-72.4338480192701,12.));
#67234=CARTESIAN_POINT('Ctrl Pts',(8.24276901945036,-72.4563917125842,0.));
#67235=CARTESIAN_POINT('Ctrl Pts',(8.24276901945036,-72.4563917125842,12.));
#67236=CARTESIAN_POINT('Ctrl Pts',(8.25498300788492,-72.4789580722871,0.));
#67237=CARTESIAN_POINT('Ctrl Pts',(8.25498300788492,-72.4789580722871,12.));
#67238=CARTESIAN_POINT('Ctrl Pts',(8.26723671704923,-72.501546983825,0.));
#67239=CARTESIAN_POINT('Ctrl Pts',(8.26723671704923,-72.501546983825,12.));
#67240=CARTESIAN_POINT('Ctrl Pts',(8.27953014520384,-72.524158333056,0.));
#67241=CARTESIAN_POINT('Ctrl Pts',(8.27953014520384,-72.524158333056,12.));
#67242=CARTESIAN_POINT('Ctrl Pts',(8.29186329053288,-72.5467920062522,0.));
#67243=CARTESIAN_POINT('Ctrl Pts',(8.29186329053288,-72.5467920062522,12.));
#67244=CARTESIAN_POINT('Ctrl Pts',(8.30423615114454,-72.5694478900983,0.));
#67245=CARTESIAN_POINT('Ctrl Pts',(8.30423615114454,-72.5694478900983,12.));
#67246=CARTESIAN_POINT('Ctrl Pts',(8.31664872507007,-72.5921258716899,0.));
#67247=CARTESIAN_POINT('Ctrl Pts',(8.31664872507007,-72.5921258716899,12.));
#67248=CARTESIAN_POINT('Ctrl Pts',(8.32910101025652,-72.614825838529,0.));
#67249=CARTESIAN_POINT('Ctrl Pts',(8.32910101025652,-72.614825838529,12.));
#67250=CARTESIAN_POINT('Ctrl Pts',(8.34159300456964,-72.6375476785208,0.));
#67251=CARTESIAN_POINT('Ctrl Pts',(8.34159300456964,-72.6375476785208,12.));
#67252=CARTESIAN_POINT('Ctrl Pts',(8.35412470580082,-72.6602912799689,0.));
#67253=CARTESIAN_POINT('Ctrl Pts',(8.35412470580082,-72.6602912799689,12.));
#67254=CARTESIAN_POINT('Ctrl Pts',(8.36669611166833,-72.68305653157,0.));
#67255=CARTESIAN_POINT('Ctrl Pts',(8.36669611166833,-72.68305653157,12.));
#67256=CARTESIAN_POINT('Ctrl Pts',(8.37930721981734,-72.7058433224072,0.));
#67257=CARTESIAN_POINT('Ctrl Pts',(8.37930721981734,-72.7058433224072,12.));
#67258=CARTESIAN_POINT('Ctrl Pts',(8.39195802781406,-72.728651541938,0.));
#67259=CARTESIAN_POINT('Ctrl Pts',(8.39195802781406,-72.728651541938,12.));
#67260=CARTESIAN_POINT('Ctrl Pts',(8.40464853314492,-72.7514810799932,0.));
#67261=CARTESIAN_POINT('Ctrl Pts',(8.40464853314492,-72.7514810799932,12.));
#67262=CARTESIAN_POINT('Ctrl Pts',(8.41737873322352,-72.7743318267876,0.));
#67263=CARTESIAN_POINT('Ctrl Pts',(8.41737873322352,-72.7743318267876,12.));
#67264=CARTESIAN_POINT('Ctrl Pts',(8.4301486253917,-72.7972036729283,0.));
#67265=CARTESIAN_POINT('Ctrl Pts',(8.4301486253917,-72.7972036729283,12.));
#67266=CARTESIAN_POINT('Ctrl Pts',(8.44295820691906,-72.8200965094197,0.));
#67267=CARTESIAN_POINT('Ctrl Pts',(8.44295820691906,-72.8200965094197,12.));
#67268=CARTESIAN_POINT('Ctrl Pts',(8.4558074749977,-72.8430102276703,0.));
#67269=CARTESIAN_POINT('Ctrl Pts',(8.4558074749977,-72.8430102276703,12.));
#67270=CARTESIAN_POINT('Ctrl Pts',(8.46869642673762,-72.8659447194918,0.));
#67271=CARTESIAN_POINT('Ctrl Pts',(8.46869642673762,-72.8659447194918,12.));
#67272=CARTESIAN_POINT('Ctrl Pts',(8.48162505917627,-72.888899877077,0.));
#67273=CARTESIAN_POINT('Ctrl Pts',(8.48162505917627,-72.888899877077,12.));
#67274=CARTESIAN_POINT('Ctrl Pts',(8.49459336928275,-72.9118755929785,0.));
#67275=CARTESIAN_POINT('Ctrl Pts',(8.49459336928275,-72.9118755929785,12.));
#67276=CARTESIAN_POINT('Ctrl Pts',(8.50760135395978,-72.9348717600837,0.));
#67277=CARTESIAN_POINT('Ctrl Pts',(8.50760135395978,-72.9348717600837,12.));
#67278=CARTESIAN_POINT('Ctrl Pts',(8.52064901004243,-72.9578882715923,0.));
#67279=CARTESIAN_POINT('Ctrl Pts',(8.52064901004243,-72.9578882715923,12.));
#67280=CARTESIAN_POINT('Ctrl Pts',(8.53373633429302,-72.9809250209843,0.));
#67281=CARTESIAN_POINT('Ctrl Pts',(8.53373633429302,-72.9809250209843,12.));
#67282=CARTESIAN_POINT('Ctrl Pts',(8.54686332340438,-73.0039819020663,0.));
#67283=CARTESIAN_POINT('Ctrl Pts',(8.54686332340438,-73.0039819020663,12.));
#67284=CARTESIAN_POINT('Ctrl Pts',(8.56002997400095,-73.0270588090193,0.));
#67285=CARTESIAN_POINT('Ctrl Pts',(8.56002997400095,-73.0270588090193,12.));
#67286=CARTESIAN_POINT('Ctrl Pts',(8.57323628263594,-73.0501556364482,0.));
#67287=CARTESIAN_POINT('Ctrl Pts',(8.57323628263594,-73.0501556364482,12.));
#67288=CARTESIAN_POINT('Ctrl Pts',(8.58648224578722,-73.073272279419,0.));
#67289=CARTESIAN_POINT('Ctrl Pts',(8.58648224578722,-73.073272279419,12.));
#67290=CARTESIAN_POINT('Ctrl Pts',(8.59976785984538,-73.0964086335226,0.));
#67291=CARTESIAN_POINT('Ctrl Pts',(8.59976785984538,-73.0964086335226,12.));
#67292=CARTESIAN_POINT('Ctrl Pts',(8.61309312111988,-73.1195645948169,0.));
#67293=CARTESIAN_POINT('Ctrl Pts',(8.61309312111988,-73.1195645948169,12.));
#67294=CARTESIAN_POINT('Ctrl Pts',(8.62645802585474,-73.142740059703,0.));
#67295=CARTESIAN_POINT('Ctrl Pts',(8.62645802585474,-73.142740059703,12.));
#67296=CARTESIAN_POINT('Ctrl Pts',(8.63986257023734,-73.165934924813,0.));
#67297=CARTESIAN_POINT('Ctrl Pts',(8.63986257023734,-73.165934924813,12.));
#67298=CARTESIAN_POINT('Ctrl Pts',(8.65330675040535,-73.1891490869057,0.));
#67299=CARTESIAN_POINT('Ctrl Pts',(8.65330675040535,-73.1891490869057,12.));
#67300=CARTESIAN_POINT('Ctrl Pts',(8.66679056245095,-73.2123824427212,0.));
#67301=CARTESIAN_POINT('Ctrl Pts',(8.66679056245095,-73.2123824427212,12.));
#67302=CARTESIAN_POINT('Ctrl Pts',(8.68031400241883,-73.2356348889704,0.));
#67303=CARTESIAN_POINT('Ctrl Pts',(8.68031400241883,-73.2356348889704,12.));
#67304=CARTESIAN_POINT('Ctrl Pts',(8.69387706629303,-73.2589063226373,0.));
#67305=CARTESIAN_POINT('Ctrl Pts',(8.69387706629303,-73.2589063226373,12.));
#67306=CARTESIAN_POINT('Ctrl Pts',(8.70747974998244,-73.282196641216,0.));
#67307=CARTESIAN_POINT('Ctrl Pts',(8.70747974998244,-73.282196641216,12.));
#67308=CARTESIAN_POINT('Ctrl Pts',(8.72112204930231,-73.3055057429744,0.));
#67309=CARTESIAN_POINT('Ctrl Pts',(8.72112204930231,-73.3055057429744,12.));
#67310=CARTESIAN_POINT('Ctrl Pts',(8.73480395995359,-73.3288335271989,0.));
#67311=CARTESIAN_POINT('Ctrl Pts',(8.73480395995359,-73.3288335271989,12.));
#67312=CARTESIAN_POINT('Ctrl Pts',(8.74852547749735,-73.3521798944595,0.));
#67313=CARTESIAN_POINT('Ctrl Pts',(8.74852547749735,-73.3521798944595,12.));
#67314=CARTESIAN_POINT('Ctrl Pts',(8.76228659740304,-73.3755447460235,0.));
#67315=CARTESIAN_POINT('Ctrl Pts',(8.76228659740304,-73.3755447460235,12.));
#67316=CARTESIAN_POINT('Ctrl Pts',(8.77608731509303,-73.3989279832808,0.));
#67317=CARTESIAN_POINT('Ctrl Pts',(8.77608731509303,-73.3989279832808,12.));
#67318=CARTESIAN_POINT('Ctrl Pts',(8.78992762598737,-73.422329507112,0.));
#67319=CARTESIAN_POINT('Ctrl Pts',(8.78992762598737,-73.422329507112,12.));
#67320=CARTESIAN_POINT('Ctrl Pts',(8.80380752553713,-73.4457492173949,0.));
#67321=CARTESIAN_POINT('Ctrl Pts',(8.80380752553713,-73.4457492173949,12.));
#67322=CARTESIAN_POINT('Ctrl Pts',(8.81772700927592,-73.4691870121608,0.));
#67323=CARTESIAN_POINT('Ctrl Pts',(8.81772700927592,-73.4691870121608,12.));
#67324=CARTESIAN_POINT('Ctrl Pts',(8.83168607277414,-73.4926427882787,0.));
#67325=CARTESIAN_POINT('Ctrl Pts',(8.83168607277414,-73.4926427882787,12.));
#67326=CARTESIAN_POINT('Ctrl Pts',(8.84568471153893,-73.5161164429765,0.));
#67327=CARTESIAN_POINT('Ctrl Pts',(8.84568471153893,-73.5161164429765,12.));
#67328=CARTESIAN_POINT('Ctrl Pts',(8.85972292092182,-73.5396078751672,0.));
#67329=CARTESIAN_POINT('Ctrl Pts',(8.85972292092182,-73.5396078751672,12.));
#67330=CARTESIAN_POINT('Ctrl Pts',(8.87380069602954,-73.5631169867113,0.));
#67331=CARTESIAN_POINT('Ctrl Pts',(8.87380069602954,-73.5631169867113,12.));
#67332=CARTESIAN_POINT('Ctrl Pts',(8.8879180316034,-73.5866436840493,0.));
#67333=CARTESIAN_POINT('Ctrl Pts',(8.8879180316034,-73.5866436840493,12.));
#67334=CARTESIAN_POINT('Ctrl Pts',(8.9020749219887,-73.6101878785868,0.));
#67335=CARTESIAN_POINT('Ctrl Pts',(8.9020749219887,-73.6101878785868,12.));
#67336=CARTESIAN_POINT('Ctrl Pts',(8.91627136139886,-73.6337494830846,0.));
#67337=CARTESIAN_POINT('Ctrl Pts',(8.91627136139886,-73.6337494830846,12.));
#67338=CARTESIAN_POINT('Ctrl Pts',(8.9305073441197,-73.6573284088088,0.));
#67339=CARTESIAN_POINT('Ctrl Pts',(8.9305073441197,-73.6573284088088,12.));
#67340=CARTESIAN_POINT('Ctrl Pts',(8.94478286474382,-73.6809245622361,0.));
#67341=CARTESIAN_POINT('Ctrl Pts',(8.94478286474382,-73.6809245622361,12.));
#67342=CARTESIAN_POINT('Ctrl Pts',(8.95909791836289,-73.7045378422775,0.));
#67343=CARTESIAN_POINT('Ctrl Pts',(8.95909791836289,-73.7045378422775,12.));
#67344=CARTESIAN_POINT('Ctrl Pts',(8.97345250083917,-73.7281681364031,0.));
#67345=CARTESIAN_POINT('Ctrl Pts',(8.97345250083917,-73.7281681364031,12.));
#67346=CARTESIAN_POINT('Ctrl Pts',(8.98784660837827,-73.7518153262253,0.));
#67347=CARTESIAN_POINT('Ctrl Pts',(8.98784660837827,-73.7518153262253,12.));
#67348=CARTESIAN_POINT('Ctrl Pts',(9.00228023701466,-73.7754792943925,0.));
#67349=CARTESIAN_POINT('Ctrl Pts',(9.00228023701466,-73.7754792943925,12.));
#67350=CARTESIAN_POINT('Ctrl Pts',(9.01675338208221,-73.7991599312731,0.));
#67351=CARTESIAN_POINT('Ctrl Pts',(9.01675338208221,-73.7991599312731,12.));
#67352=CARTESIAN_POINT('Ctrl Pts',(9.0312660377798,-73.8228571411607,0.));
#67353=CARTESIAN_POINT('Ctrl Pts',(9.0312660377798,-73.8228571411607,12.));
#67354=CARTESIAN_POINT('Ctrl Pts',(9.04581819646384,-73.8465708500679,0.));
#67355=CARTESIAN_POINT('Ctrl Pts',(9.04581819646384,-73.8465708500679,12.));
#67356=CARTESIAN_POINT('Ctrl Pts',(9.06040984889249,-73.870301007746,0.));
#67357=CARTESIAN_POINT('Ctrl Pts',(9.06040984889249,-73.870301007746,12.));
#67358=CARTESIAN_POINT('Ctrl Pts',(9.07504098570546,-73.8940475821756,0.));
#67359=CARTESIAN_POINT('Ctrl Pts',(9.07504098570546,-73.8940475821756,12.));
#67360=CARTESIAN_POINT('Ctrl Pts',(9.08677747601237,-73.9130579611989,0.));
#67361=CARTESIAN_POINT('Ctrl Pts',(9.08677747601237,-73.9130579611989,12.));
#67362=CARTESIAN_POINT('Ctrl Pts',(9.09559760528458,-73.9273231219464,0.));
#67363=CARTESIAN_POINT('Ctrl Pts',(9.09559760528458,-73.9273231219464,12.));
#67364=CARTESIAN_POINT('Ctrl Pts',(9.10148558516323,-73.9368365074164,0.));
#67365=CARTESIAN_POINT('Ctrl Pts',(9.10148558516323,-73.9368365074164,12.));
#67366=CARTESIAN_POINT('Ctrl Pts',(9.10443154852686,-73.9415940197274,0.));
#67367=CARTESIAN_POINT('Ctrl Pts',(9.10443154852686,-73.9415940197274,12.));
#67368=CARTESIAN_POINT('',(6.95102489306925,-69.6540253893192,0.));
#67369=CARTESIAN_POINT('Ctrl Pts',(6.95102489306925,-69.6540253893192,0.));
#67370=CARTESIAN_POINT('Ctrl Pts',(6.95238884849024,-69.6576616146467,0.));
#67371=CARTESIAN_POINT('Ctrl Pts',(6.95512065317599,-69.664938391983,0.));
#67372=CARTESIAN_POINT('Ctrl Pts',(6.9592300417359,-69.6758665380378,0.));
#67373=CARTESIAN_POINT('Ctrl Pts',(6.96473259049512,-69.6904633605421,0.));
#67374=CARTESIAN_POINT('Ctrl Pts',(6.97164972291439,-69.7087526479973,0.));
#67375=CARTESIAN_POINT('Ctrl Pts',(6.97860581164526,-69.7270851557366,0.));
#67376=CARTESIAN_POINT('Ctrl Pts',(6.98560086924213,-69.7454607995607,0.));
#67377=CARTESIAN_POINT('Ctrl Pts',(6.9926349102794,-69.7638794280419,0.));
#67378=CARTESIAN_POINT('Ctrl Pts',(6.99970795069475,-69.782340824259,0.));
#67379=CARTESIAN_POINT('Ctrl Pts',(7.0068200071815,-69.8008447346863,0.));
#67380=CARTESIAN_POINT('Ctrl Pts',(7.01397109655454,-69.8193908913722,0.));
#67381=CARTESIAN_POINT('Ctrl Pts',(7.02116123514451,-69.8379790360518,0.));
#67382=CARTESIAN_POINT('Ctrl Pts',(7.02839043811812,-69.8566089455375,0.));
#67383=CARTESIAN_POINT('Ctrl Pts',(7.0356587197222,-69.8752804235238,0.));
#67384=CARTESIAN_POINT('Ctrl Pts',(7.04296609362165,-69.8939932885841,0.));
#67385=CARTESIAN_POINT('Ctrl Pts',(7.05031257318115,-69.9127473642099,0.));
#67386=CARTESIAN_POINT('Ctrl Pts',(7.05769817180856,-69.9315424664291,0.));
#67387=CARTESIAN_POINT('Ctrl Pts',(7.06512290312849,-69.9503783975727,0.));
#67388=CARTESIAN_POINT('Ctrl Pts',(7.0725867808083,-69.9692549527296,0.));
#67389=CARTESIAN_POINT('Ctrl Pts',(7.08008981844651,-69.988171923788,0.));
#67390=CARTESIAN_POINT('Ctrl Pts',(7.08763202944245,-70.0071291040766,0.));
#67391=CARTESIAN_POINT('Ctrl Pts',(7.09521342684248,-70.0261262936388,0.));
#67392=CARTESIAN_POINT('Ctrl Pts',(7.10283402335033,-70.0451632990086,0.));
#67393=CARTESIAN_POINT('Ctrl Pts',(7.11049383140445,-70.0642399306869,0.));
#67394=CARTESIAN_POINT('Ctrl Pts',(7.11819286322825,-70.0833560013975,0.));
#67395=CARTESIAN_POINT('Ctrl Pts',(7.12593113088903,-70.1025113239495,0.));
#67396=CARTESIAN_POINT('Ctrl Pts',(7.13370864634442,-70.1217057094499,0.));
#67397=CARTESIAN_POINT('Ctrl Pts',(7.14152542142373,-70.1409389682424,0.));
#67398=CARTESIAN_POINT('Ctrl Pts',(7.14938146780813,-70.1602109107202,0.));
#67399=CARTESIAN_POINT('Ctrl Pts',(7.15727679700932,-70.1795213481185,0.));
#67400=CARTESIAN_POINT('Ctrl Pts',(7.16521142033863,-70.1988700934593,0.));
#67401=CARTESIAN_POINT('Ctrl Pts',(7.17318534889715,-70.2182569618994,0.));
#67402=CARTESIAN_POINT('Ctrl Pts',(7.18119859359777,-70.2376817702215,0.));
#67403=CARTESIAN_POINT('Ctrl Pts',(7.18925116517554,-70.2571443365192,0.));
#67404=CARTESIAN_POINT('Ctrl Pts',(7.19734307419872,-70.2766444798285,0.));
#67405=CARTESIAN_POINT('Ctrl Pts',(7.20547433107482,-70.2961820197077,0.));
#67406=CARTESIAN_POINT('Ctrl Pts',(7.21364494605449,-70.3157567762588,0.));
#67407=CARTESIAN_POINT('Ctrl Pts',(7.2218549292319,-70.3353685703112,0.));
#67408=CARTESIAN_POINT('Ctrl Pts',(7.23010429054228,-70.3550172235486,0.));
#67409=CARTESIAN_POINT('Ctrl Pts',(7.23839303975606,-70.3747025586552,0.));
#67410=CARTESIAN_POINT('Ctrl Pts',(7.24672118647084,-70.3944243994504,0.));
#67411=CARTESIAN_POINT('Ctrl Pts',(7.25508874012042,-70.4141825708178,0.));
#67412=CARTESIAN_POINT('Ctrl Pts',(7.26349570998032,-70.4339768986346,0.));
#67413=CARTESIAN_POINT('Ctrl Pts',(7.27194210517062,-70.4538072096992,0.));
#67414=CARTESIAN_POINT('Ctrl Pts',(7.2804279346547,-70.4736733316487,0.));
#67415=CARTESIAN_POINT('Ctrl Pts',(7.28895320723861,-70.4935750929058,0.));
#67416=CARTESIAN_POINT('Ctrl Pts',(7.29751793157822,-70.5135123227169,0.));
#67417=CARTESIAN_POINT('Ctrl Pts',(7.30612211618052,-70.5334848511681,0.));
#67418=CARTESIAN_POINT('Ctrl Pts',(7.31476576940391,-70.5534925092043,0.));
#67419=CARTESIAN_POINT('Ctrl Pts',(7.32344889945219,-70.5735351286476,0.));
#67420=CARTESIAN_POINT('Ctrl Pts',(7.3321715143759,-70.5936125421946,0.));
#67421=CARTESIAN_POINT('Ctrl Pts',(7.34093362208007,-70.6137245833996,0.));
#67422=CARTESIAN_POINT('Ctrl Pts',(7.34973523032577,-70.6338710866562,0.));
#67423=CARTESIAN_POINT('Ctrl Pts',(7.35857634673054,-70.6540518871775,0.));
#67424=CARTESIAN_POINT('Ctrl Pts',(7.367456978763,-70.6742668209687,0.));
#67425=CARTESIAN_POINT('Ctrl Pts',(7.37637713374767,-70.694515724827,0.));
#67426=CARTESIAN_POINT('Ctrl Pts',(7.38533681887032,-70.7147984363424,0.));
#67427=CARTESIAN_POINT('Ctrl Pts',(7.3943360411789,-70.735114793895,0.));
#67428=CARTESIAN_POINT('Ctrl Pts',(7.40337480758229,-70.7554646366514,0.));
#67429=CARTESIAN_POINT('Ctrl Pts',(7.41245312484486,-70.7758478045576,0.));
#67430=CARTESIAN_POINT('Ctrl Pts',(7.42157099959315,-70.7962641383351,0.));
#67431=CARTESIAN_POINT('Ctrl Pts',(7.43072843832007,-70.8167134794738,0.));
#67432=CARTESIAN_POINT('Ctrl Pts',(7.43992544738606,-70.8371956702242,0.));
#67433=CARTESIAN_POINT('Ctrl Pts',(7.44916203301644,-70.8577105535841,0.));
#67434=CARTESIAN_POINT('Ctrl Pts',(7.45843820129775,-70.8782579732885,0.));
#67435=CARTESIAN_POINT('Ctrl Pts',(7.46775395818518,-70.8988377738088,0.));
#67436=CARTESIAN_POINT('Ctrl Pts',(7.47710930950553,-70.9194498003483,0.));
#67437=CARTESIAN_POINT('Ctrl Pts',(7.48650426095822,-70.9400938988373,0.));
#67438=CARTESIAN_POINT('Ctrl Pts',(7.49593881811141,-70.9607699159234,0.));
#67439=CARTESIAN_POINT('Ctrl Pts',(7.50541298639948,-70.9814776989637,0.));
#67440=CARTESIAN_POINT('Ctrl Pts',(7.51492677113111,-71.0022170960235,0.));
#67441=CARTESIAN_POINT('Ctrl Pts',(7.52448017749135,-71.0229879558713,0.));
#67442=CARTESIAN_POINT('Ctrl Pts',(7.53407321054253,-71.0437901279722,0.));
#67443=CARTESIAN_POINT('Ctrl Pts',(7.54370587521947,-71.0646234624783,0.));
#67444=CARTESIAN_POINT('Ctrl Pts',(7.55337817632872,-71.0854878102203,0.));
#67445=CARTESIAN_POINT('Ctrl Pts',(7.56309011855616,-71.1063830227074,0.));
#67446=CARTESIAN_POINT('Ctrl Pts',(7.57284170646865,-71.1273089521218,0.));
#67447=CARTESIAN_POINT('Ctrl Pts',(7.58263294451465,-71.1482654513133,0.));
#67448=CARTESIAN_POINT('Ctrl Pts',(7.59246383701859,-71.1692523737887,0.));
#67449=CARTESIAN_POINT('Ctrl Pts',(7.60233438818156,-71.1902695737063,0.));
#67450=CARTESIAN_POINT('Ctrl Pts',(7.61224460208886,-71.2113169058778,0.));
#67451=CARTESIAN_POINT('Ctrl Pts',(7.62219448271124,-71.232394225762,0.));
#67452=CARTESIAN_POINT('Ctrl Pts',(7.63218403390514,-71.2535013894587,0.));
#67453=CARTESIAN_POINT('Ctrl Pts',(7.64221325940671,-71.2746382536974,0.));
#67454=CARTESIAN_POINT('Ctrl Pts',(7.65228216283342,-71.2958046758334,0.));
#67455=CARTESIAN_POINT('Ctrl Pts',(7.66239074769118,-71.3170005138474,0.));
#67456=CARTESIAN_POINT('Ctrl Pts',(7.67253901737539,-71.3382256263405,0.));
#67457=CARTESIAN_POINT('Ctrl Pts',(7.68272697517102,-71.3594798725294,0.));
#67458=CARTESIAN_POINT('Ctrl Pts',(7.69295462424646,-71.380763112236,0.));
#67459=CARTESIAN_POINT('Ctrl Pts',(7.70322196765572,-71.4020752058827,0.));
#67460=CARTESIAN_POINT('Ctrl Pts',(7.71352900834537,-71.4234160144943,0.));
#67461=CARTESIAN_POINT('Ctrl Pts',(7.72387574915544,-71.4447853996919,0.));
#67462=CARTESIAN_POINT('Ctrl Pts',(7.73426219281931,-71.4661832236881,0.));
#67463=CARTESIAN_POINT('Ctrl Pts',(7.74468834195734,-71.487609349277,0.));
#67464=CARTESIAN_POINT('Ctrl Pts',(7.75515419907954,-71.5090636398307,0.));
#67465=CARTESIAN_POINT('Ctrl Pts',(7.76565976659218,-71.5305459592987,0.));
#67466=CARTESIAN_POINT('Ctrl Pts',(7.77620504679867,-71.5520561722039,0.));
#67467=CARTESIAN_POINT('Ctrl Pts',(7.78679004189934,-71.5735941436366,0.));
#67468=CARTESIAN_POINT('Ctrl Pts',(7.79741475398511,-71.5951597392471,0.));
#67469=CARTESIAN_POINT('Ctrl Pts',(7.80807918504016,-71.616752825242,0.));
#67470=CARTESIAN_POINT('Ctrl Pts',(7.81878333694855,-71.638373268384,0.));
#67471=CARTESIAN_POINT('Ctrl Pts',(7.82952721149503,-71.6600209359869,0.));
#67472=CARTESIAN_POINT('Ctrl Pts',(7.84031081036488,-71.681695695912,0.));
#67473=CARTESIAN_POINT('Ctrl Pts',(7.85113413513738,-71.7033974165576,0.));
#67474=CARTESIAN_POINT('Ctrl Pts',(7.86199718728829,-71.7251259668573,0.));
#67475=CARTESIAN_POINT('Ctrl Pts',(7.87289996819653,-71.7468812162795,0.));
#67476=CARTESIAN_POINT('Ctrl Pts',(7.88384247914521,-71.768663034824,0.));
#67477=CARTESIAN_POINT('Ctrl Pts',(7.89482472132134,-71.7904712930172,0.));
#67478=CARTESIAN_POINT('Ctrl Pts',(7.90584669580955,-71.8123058619038,0.));
#67479=CARTESIAN_POINT('Ctrl Pts',(7.9169084035937,-71.8341666130424,0.));
#67480=CARTESIAN_POINT('Ctrl Pts',(7.92800984556399,-71.8560534185071,0.));
#67481=CARTESIAN_POINT('Ctrl Pts',(7.93915102251795,-71.8779661508833,0.));
#67482=CARTESIAN_POINT('Ctrl Pts',(7.95033193516045,-71.8999046832642,0.));
#67483=CARTESIAN_POINT('Ctrl Pts',(7.96155258409751,-71.9218688892426,0.));
#67484=CARTESIAN_POINT('Ctrl Pts',(7.97281296983701,-71.9438586429072,0.));
#67485=CARTESIAN_POINT('Ctrl Pts',(7.98411309279597,-71.9658738188421,0.));
#67486=CARTESIAN_POINT('Ctrl Pts',(7.99545295330181,-71.9879142921248,0.));
#67487=CARTESIAN_POINT('Ctrl Pts',(8.00683255159249,-72.0099799383216,0.));
#67488=CARTESIAN_POINT('Ctrl Pts',(8.01825188781069,-72.0320706334802,0.));
#67489=CARTESIAN_POINT('Ctrl Pts',(8.02971096200327,-72.0541862541262,0.));
#67490=CARTESIAN_POINT('Ctrl Pts',(8.04120977412891,-72.0763266772632,0.));
#67491=CARTESIAN_POINT('Ctrl Pts',(8.05274832405956,-72.0984917803702,0.));
#67492=CARTESIAN_POINT('Ctrl Pts',(8.06432661158088,-72.1206814413985,0.));
#67493=CARTESIAN_POINT('Ctrl Pts',(8.07594463638699,-72.1428955387648,0.));
#67494=CARTESIAN_POINT('Ctrl Pts',(8.08760239807814,-72.165133951346,0.));
#67495=CARTESIAN_POINT('Ctrl Pts',(8.09929989616873,-72.18739655848,0.));
#67496=CARTESIAN_POINT('Ctrl Pts',(8.11103713008921,-72.2096832399626,0.));
#67497=CARTESIAN_POINT('Ctrl Pts',(8.12281409918661,-72.2319938760451,0.));
#67498=CARTESIAN_POINT('Ctrl Pts',(8.13463080272028,-72.2543283474279,0.));
#67499=CARTESIAN_POINT('Ctrl Pts',(8.14648723985792,-72.2766865352552,0.));
#67500=CARTESIAN_POINT('Ctrl Pts',(8.15838340968327,-72.2990683211155,0.));
#67501=CARTESIAN_POINT('Ctrl Pts',(8.17031931119881,-72.3214735870402,0.));
#67502=CARTESIAN_POINT('Ctrl Pts',(8.18229494332621,-72.3439022155007,0.));
#67503=CARTESIAN_POINT('Ctrl Pts',(8.19431030490318,-72.3663540894034,0.));
#67504=CARTESIAN_POINT('Ctrl Pts',(8.20636539467781,-72.3888290920845,0.));
#67505=CARTESIAN_POINT('Ctrl Pts',(8.21846021131563,-72.4113271073091,0.));
#67506=CARTESIAN_POINT('Ctrl Pts',(8.23059475340354,-72.4338480192701,0.));
#67507=CARTESIAN_POINT('Ctrl Pts',(8.24276901945036,-72.4563917125842,0.));
#67508=CARTESIAN_POINT('Ctrl Pts',(8.25498300788492,-72.4789580722871,0.));
#67509=CARTESIAN_POINT('Ctrl Pts',(8.26723671704923,-72.501546983825,0.));
#67510=CARTESIAN_POINT('Ctrl Pts',(8.27953014520384,-72.524158333056,0.));
#67511=CARTESIAN_POINT('Ctrl Pts',(8.29186329053288,-72.5467920062522,0.));
#67512=CARTESIAN_POINT('Ctrl Pts',(8.30423615114454,-72.5694478900983,0.));
#67513=CARTESIAN_POINT('Ctrl Pts',(8.31664872507007,-72.5921258716899,0.));
#67514=CARTESIAN_POINT('Ctrl Pts',(8.32910101025652,-72.614825838529,0.));
#67515=CARTESIAN_POINT('Ctrl Pts',(8.34159300456964,-72.6375476785208,0.));
#67516=CARTESIAN_POINT('Ctrl Pts',(8.35412470580082,-72.6602912799689,0.));
#67517=CARTESIAN_POINT('Ctrl Pts',(8.36669611166833,-72.68305653157,0.));
#67518=CARTESIAN_POINT('Ctrl Pts',(8.37930721981734,-72.7058433224072,0.));
#67519=CARTESIAN_POINT('Ctrl Pts',(8.39195802781406,-72.728651541938,0.));
#67520=CARTESIAN_POINT('Ctrl Pts',(8.40464853314492,-72.7514810799932,0.));
#67521=CARTESIAN_POINT('Ctrl Pts',(8.41737873322352,-72.7743318267876,0.));
#67522=CARTESIAN_POINT('Ctrl Pts',(8.4301486253917,-72.7972036729283,0.));
#67523=CARTESIAN_POINT('Ctrl Pts',(8.44295820691906,-72.8200965094197,0.));
#67524=CARTESIAN_POINT('Ctrl Pts',(8.4558074749977,-72.8430102276703,0.));
#67525=CARTESIAN_POINT('Ctrl Pts',(8.46869642673762,-72.8659447194918,0.));
#67526=CARTESIAN_POINT('Ctrl Pts',(8.48162505917627,-72.888899877077,0.));
#67527=CARTESIAN_POINT('Ctrl Pts',(8.49459336928275,-72.9118755929785,0.));
#67528=CARTESIAN_POINT('Ctrl Pts',(8.50760135395978,-72.9348717600837,0.));
#67529=CARTESIAN_POINT('Ctrl Pts',(8.52064901004243,-72.9578882715923,0.));
#67530=CARTESIAN_POINT('Ctrl Pts',(8.53373633429302,-72.9809250209843,0.));
#67531=CARTESIAN_POINT('Ctrl Pts',(8.54686332340438,-73.0039819020663,0.));
#67532=CARTESIAN_POINT('Ctrl Pts',(8.56002997400095,-73.0270588090193,0.));
#67533=CARTESIAN_POINT('Ctrl Pts',(8.57323628263594,-73.0501556364482,0.));
#67534=CARTESIAN_POINT('Ctrl Pts',(8.58648224578722,-73.073272279419,0.));
#67535=CARTESIAN_POINT('Ctrl Pts',(8.59976785984538,-73.0964086335226,0.));
#67536=CARTESIAN_POINT('Ctrl Pts',(8.61309312111988,-73.1195645948169,0.));
#67537=CARTESIAN_POINT('Ctrl Pts',(8.62645802585474,-73.142740059703,0.));
#67538=CARTESIAN_POINT('Ctrl Pts',(8.63986257023734,-73.165934924813,0.));
#67539=CARTESIAN_POINT('Ctrl Pts',(8.65330675040535,-73.1891490869057,0.));
#67540=CARTESIAN_POINT('Ctrl Pts',(8.66679056245095,-73.2123824427212,0.));
#67541=CARTESIAN_POINT('Ctrl Pts',(8.68031400241883,-73.2356348889704,0.));
#67542=CARTESIAN_POINT('Ctrl Pts',(8.69387706629303,-73.2589063226373,0.));
#67543=CARTESIAN_POINT('Ctrl Pts',(8.70747974998244,-73.282196641216,0.));
#67544=CARTESIAN_POINT('Ctrl Pts',(8.72112204930231,-73.3055057429744,0.));
#67545=CARTESIAN_POINT('Ctrl Pts',(8.73480395995359,-73.3288335271989,0.));
#67546=CARTESIAN_POINT('Ctrl Pts',(8.74852547749735,-73.3521798944595,0.));
#67547=CARTESIAN_POINT('Ctrl Pts',(8.76228659740304,-73.3755447460235,0.));
#67548=CARTESIAN_POINT('Ctrl Pts',(8.77608731509303,-73.3989279832808,0.));
#67549=CARTESIAN_POINT('Ctrl Pts',(8.78992762598737,-73.422329507112,0.));
#67550=CARTESIAN_POINT('Ctrl Pts',(8.80380752553713,-73.4457492173949,0.));
#67551=CARTESIAN_POINT('Ctrl Pts',(8.81772700927592,-73.4691870121608,0.));
#67552=CARTESIAN_POINT('Ctrl Pts',(8.83168607277414,-73.4926427882787,0.));
#67553=CARTESIAN_POINT('Ctrl Pts',(8.84568471153893,-73.5161164429765,0.));
#67554=CARTESIAN_POINT('Ctrl Pts',(8.85972292092182,-73.5396078751672,0.));
#67555=CARTESIAN_POINT('Ctrl Pts',(8.87380069602954,-73.5631169867113,0.));
#67556=CARTESIAN_POINT('Ctrl Pts',(8.8879180316034,-73.5866436840493,0.));
#67557=CARTESIAN_POINT('Ctrl Pts',(8.9020749219887,-73.6101878785868,0.));
#67558=CARTESIAN_POINT('Ctrl Pts',(8.91424402151027,-73.6303847393445,0.));
#67559=CARTESIAN_POINT('Ctrl Pts',(8.92359518177562,-73.645878630579,0.));
#67560=CARTESIAN_POINT('Ctrl Pts',(8.9301108881604,-73.6566618621799,0.));
#67561=CARTESIAN_POINT('Ctrl Pts',(8.93377955964004,-73.6627293782266,0.));
#67562=CARTESIAN_POINT('Ctrl Pts',(8.93459554655838,-73.6640787197675,0.));
#67563=CARTESIAN_POINT('',(6.95102489306925,-69.6540253893192,12.));
#67564=CARTESIAN_POINT('',(6.95102489306925,-69.6540253893192,0.));
#67565=CARTESIAN_POINT('Ctrl Pts',(8.93459554655838,-73.6640787197675,12.));
#67566=CARTESIAN_POINT('Ctrl Pts',(8.93377955964004,-73.6627293782266,12.));
#67567=CARTESIAN_POINT('Ctrl Pts',(8.9301108881604,-73.6566618621799,12.));
#67568=CARTESIAN_POINT('Ctrl Pts',(8.92359518177562,-73.645878630579,12.));
#67569=CARTESIAN_POINT('Ctrl Pts',(8.91424402151027,-73.6303847393445,12.));
#67570=CARTESIAN_POINT('Ctrl Pts',(8.9020749219887,-73.6101878785868,12.));
#67571=CARTESIAN_POINT('Ctrl Pts',(8.8879180316034,-73.5866436840493,12.));
#67572=CARTESIAN_POINT('Ctrl Pts',(8.87380069602954,-73.5631169867113,12.));
#67573=CARTESIAN_POINT('Ctrl Pts',(8.85972292092182,-73.5396078751672,12.));
#67574=CARTESIAN_POINT('Ctrl Pts',(8.84568471153893,-73.5161164429765,12.));
#67575=CARTESIAN_POINT('Ctrl Pts',(8.83168607277414,-73.4926427882787,12.));
#67576=CARTESIAN_POINT('Ctrl Pts',(8.81772700927592,-73.4691870121608,12.));
#67577=CARTESIAN_POINT('Ctrl Pts',(8.80380752553713,-73.4457492173949,12.));
#67578=CARTESIAN_POINT('Ctrl Pts',(8.78992762598737,-73.422329507112,12.));
#67579=CARTESIAN_POINT('Ctrl Pts',(8.77608731509303,-73.3989279832808,12.));
#67580=CARTESIAN_POINT('Ctrl Pts',(8.76228659740304,-73.3755447460235,12.));
#67581=CARTESIAN_POINT('Ctrl Pts',(8.74852547749735,-73.3521798944595,12.));
#67582=CARTESIAN_POINT('Ctrl Pts',(8.73480395995359,-73.3288335271989,12.));
#67583=CARTESIAN_POINT('Ctrl Pts',(8.72112204930231,-73.3055057429744,12.));
#67584=CARTESIAN_POINT('Ctrl Pts',(8.70747974998244,-73.282196641216,12.));
#67585=CARTESIAN_POINT('Ctrl Pts',(8.69387706629303,-73.2589063226373,12.));
#67586=CARTESIAN_POINT('Ctrl Pts',(8.68031400241883,-73.2356348889704,12.));
#67587=CARTESIAN_POINT('Ctrl Pts',(8.66679056245095,-73.2123824427212,12.));
#67588=CARTESIAN_POINT('Ctrl Pts',(8.65330675040535,-73.1891490869057,12.));
#67589=CARTESIAN_POINT('Ctrl Pts',(8.63986257023734,-73.165934924813,12.));
#67590=CARTESIAN_POINT('Ctrl Pts',(8.62645802585474,-73.142740059703,12.));
#67591=CARTESIAN_POINT('Ctrl Pts',(8.61309312111988,-73.1195645948169,12.));
#67592=CARTESIAN_POINT('Ctrl Pts',(8.59976785984538,-73.0964086335226,12.));
#67593=CARTESIAN_POINT('Ctrl Pts',(8.58648224578722,-73.073272279419,12.));
#67594=CARTESIAN_POINT('Ctrl Pts',(8.57323628263594,-73.0501556364482,12.));
#67595=CARTESIAN_POINT('Ctrl Pts',(8.56002997400095,-73.0270588090193,12.));
#67596=CARTESIAN_POINT('Ctrl Pts',(8.54686332340438,-73.0039819020663,12.));
#67597=CARTESIAN_POINT('Ctrl Pts',(8.53373633429302,-72.9809250209843,12.));
#67598=CARTESIAN_POINT('Ctrl Pts',(8.52064901004243,-72.9578882715923,12.));
#67599=CARTESIAN_POINT('Ctrl Pts',(8.50760135395978,-72.9348717600837,12.));
#67600=CARTESIAN_POINT('Ctrl Pts',(8.49459336928275,-72.9118755929785,12.));
#67601=CARTESIAN_POINT('Ctrl Pts',(8.48162505917627,-72.888899877077,12.));
#67602=CARTESIAN_POINT('Ctrl Pts',(8.46869642673762,-72.8659447194918,12.));
#67603=CARTESIAN_POINT('Ctrl Pts',(8.4558074749977,-72.8430102276703,12.));
#67604=CARTESIAN_POINT('Ctrl Pts',(8.44295820691906,-72.8200965094197,12.));
#67605=CARTESIAN_POINT('Ctrl Pts',(8.4301486253917,-72.7972036729283,12.));
#67606=CARTESIAN_POINT('Ctrl Pts',(8.41737873322352,-72.7743318267876,12.));
#67607=CARTESIAN_POINT('Ctrl Pts',(8.40464853314492,-72.7514810799932,12.));
#67608=CARTESIAN_POINT('Ctrl Pts',(8.39195802781406,-72.728651541938,12.));
#67609=CARTESIAN_POINT('Ctrl Pts',(8.37930721981734,-72.7058433224072,12.));
#67610=CARTESIAN_POINT('Ctrl Pts',(8.36669611166833,-72.68305653157,12.));
#67611=CARTESIAN_POINT('Ctrl Pts',(8.35412470580082,-72.6602912799689,12.));
#67612=CARTESIAN_POINT('Ctrl Pts',(8.34159300456964,-72.6375476785208,12.));
#67613=CARTESIAN_POINT('Ctrl Pts',(8.32910101025652,-72.614825838529,12.));
#67614=CARTESIAN_POINT('Ctrl Pts',(8.31664872507007,-72.5921258716899,12.));
#67615=CARTESIAN_POINT('Ctrl Pts',(8.30423615114454,-72.5694478900983,12.));
#67616=CARTESIAN_POINT('Ctrl Pts',(8.29186329053288,-72.5467920062522,12.));
#67617=CARTESIAN_POINT('Ctrl Pts',(8.27953014520384,-72.524158333056,12.));
#67618=CARTESIAN_POINT('Ctrl Pts',(8.26723671704923,-72.501546983825,12.));
#67619=CARTESIAN_POINT('Ctrl Pts',(8.25498300788492,-72.4789580722871,12.));
#67620=CARTESIAN_POINT('Ctrl Pts',(8.24276901945036,-72.4563917125842,12.));
#67621=CARTESIAN_POINT('Ctrl Pts',(8.23059475340354,-72.4338480192701,12.));
#67622=CARTESIAN_POINT('Ctrl Pts',(8.21846021131563,-72.4113271073091,12.));
#67623=CARTESIAN_POINT('Ctrl Pts',(8.20636539467781,-72.3888290920845,12.));
#67624=CARTESIAN_POINT('Ctrl Pts',(8.19431030490318,-72.3663540894034,12.));
#67625=CARTESIAN_POINT('Ctrl Pts',(8.18229494332621,-72.3439022155007,12.));
#67626=CARTESIAN_POINT('Ctrl Pts',(8.17031931119881,-72.3214735870402,12.));
#67627=CARTESIAN_POINT('Ctrl Pts',(8.15838340968327,-72.2990683211155,12.));
#67628=CARTESIAN_POINT('Ctrl Pts',(8.14648723985792,-72.2766865352552,12.));
#67629=CARTESIAN_POINT('Ctrl Pts',(8.13463080272028,-72.2543283474279,12.));
#67630=CARTESIAN_POINT('Ctrl Pts',(8.12281409918661,-72.2319938760451,12.));
#67631=CARTESIAN_POINT('Ctrl Pts',(8.11103713008921,-72.2096832399626,12.));
#67632=CARTESIAN_POINT('Ctrl Pts',(8.09929989616873,-72.18739655848,12.));
#67633=CARTESIAN_POINT('Ctrl Pts',(8.08760239807814,-72.165133951346,12.));
#67634=CARTESIAN_POINT('Ctrl Pts',(8.07594463638699,-72.1428955387648,12.));
#67635=CARTESIAN_POINT('Ctrl Pts',(8.06432661158088,-72.1206814413985,12.));
#67636=CARTESIAN_POINT('Ctrl Pts',(8.05274832405956,-72.0984917803702,12.));
#67637=CARTESIAN_POINT('Ctrl Pts',(8.04120977412891,-72.0763266772632,12.));
#67638=CARTESIAN_POINT('Ctrl Pts',(8.02971096200327,-72.0541862541262,12.));
#67639=CARTESIAN_POINT('Ctrl Pts',(8.01825188781069,-72.0320706334802,12.));
#67640=CARTESIAN_POINT('Ctrl Pts',(8.00683255159249,-72.0099799383216,12.));
#67641=CARTESIAN_POINT('Ctrl Pts',(7.99545295330181,-71.9879142921248,12.));
#67642=CARTESIAN_POINT('Ctrl Pts',(7.98411309279597,-71.9658738188421,12.));
#67643=CARTESIAN_POINT('Ctrl Pts',(7.97281296983701,-71.9438586429072,12.));
#67644=CARTESIAN_POINT('Ctrl Pts',(7.96155258409751,-71.9218688892426,12.));
#67645=CARTESIAN_POINT('Ctrl Pts',(7.95033193516045,-71.8999046832642,12.));
#67646=CARTESIAN_POINT('Ctrl Pts',(7.93915102251795,-71.8779661508833,12.));
#67647=CARTESIAN_POINT('Ctrl Pts',(7.92800984556399,-71.8560534185071,12.));
#67648=CARTESIAN_POINT('Ctrl Pts',(7.9169084035937,-71.8341666130424,12.));
#67649=CARTESIAN_POINT('Ctrl Pts',(7.90584669580955,-71.8123058619038,12.));
#67650=CARTESIAN_POINT('Ctrl Pts',(7.89482472132134,-71.7904712930172,12.));
#67651=CARTESIAN_POINT('Ctrl Pts',(7.88384247914521,-71.768663034824,12.));
#67652=CARTESIAN_POINT('Ctrl Pts',(7.87289996819653,-71.7468812162795,12.));
#67653=CARTESIAN_POINT('Ctrl Pts',(7.86199718728829,-71.7251259668573,12.));
#67654=CARTESIAN_POINT('Ctrl Pts',(7.85113413513738,-71.7033974165576,12.));
#67655=CARTESIAN_POINT('Ctrl Pts',(7.84031081036488,-71.681695695912,12.));
#67656=CARTESIAN_POINT('Ctrl Pts',(7.82952721149503,-71.6600209359869,12.));
#67657=CARTESIAN_POINT('Ctrl Pts',(7.81878333694855,-71.638373268384,12.));
#67658=CARTESIAN_POINT('Ctrl Pts',(7.80807918504016,-71.616752825242,12.));
#67659=CARTESIAN_POINT('Ctrl Pts',(7.79741475398511,-71.5951597392471,12.));
#67660=CARTESIAN_POINT('Ctrl Pts',(7.78679004189934,-71.5735941436366,12.));
#67661=CARTESIAN_POINT('Ctrl Pts',(7.77620504679867,-71.5520561722039,12.));
#67662=CARTESIAN_POINT('Ctrl Pts',(7.76565976659218,-71.5305459592987,12.));
#67663=CARTESIAN_POINT('Ctrl Pts',(7.75515419907954,-71.5090636398307,12.));
#67664=CARTESIAN_POINT('Ctrl Pts',(7.74468834195734,-71.487609349277,12.));
#67665=CARTESIAN_POINT('Ctrl Pts',(7.73426219281931,-71.4661832236881,12.));
#67666=CARTESIAN_POINT('Ctrl Pts',(7.72387574915544,-71.4447853996919,12.));
#67667=CARTESIAN_POINT('Ctrl Pts',(7.71352900834537,-71.4234160144943,12.));
#67668=CARTESIAN_POINT('Ctrl Pts',(7.70322196765572,-71.4020752058827,12.));
#67669=CARTESIAN_POINT('Ctrl Pts',(7.69295462424646,-71.380763112236,12.));
#67670=CARTESIAN_POINT('Ctrl Pts',(7.68272697517102,-71.3594798725294,12.));
#67671=CARTESIAN_POINT('Ctrl Pts',(7.67253901737539,-71.3382256263405,12.));
#67672=CARTESIAN_POINT('Ctrl Pts',(7.66239074769118,-71.3170005138474,12.));
#67673=CARTESIAN_POINT('Ctrl Pts',(7.65228216283342,-71.2958046758334,12.));
#67674=CARTESIAN_POINT('Ctrl Pts',(7.64221325940671,-71.2746382536974,12.));
#67675=CARTESIAN_POINT('Ctrl Pts',(7.63218403390514,-71.2535013894587,12.));
#67676=CARTESIAN_POINT('Ctrl Pts',(7.62219448271124,-71.232394225762,12.));
#67677=CARTESIAN_POINT('Ctrl Pts',(7.61224460208886,-71.2113169058778,12.));
#67678=CARTESIAN_POINT('Ctrl Pts',(7.60233438818156,-71.1902695737063,12.));
#67679=CARTESIAN_POINT('Ctrl Pts',(7.59246383701859,-71.1692523737887,12.));
#67680=CARTESIAN_POINT('Ctrl Pts',(7.58263294451465,-71.1482654513133,12.));
#67681=CARTESIAN_POINT('Ctrl Pts',(7.57284170646865,-71.1273089521218,12.));
#67682=CARTESIAN_POINT('Ctrl Pts',(7.56309011855616,-71.1063830227074,12.));
#67683=CARTESIAN_POINT('Ctrl Pts',(7.55337817632872,-71.0854878102203,12.));
#67684=CARTESIAN_POINT('Ctrl Pts',(7.54370587521947,-71.0646234624783,12.));
#67685=CARTESIAN_POINT('Ctrl Pts',(7.53407321054253,-71.0437901279722,12.));
#67686=CARTESIAN_POINT('Ctrl Pts',(7.52448017749135,-71.0229879558713,12.));
#67687=CARTESIAN_POINT('Ctrl Pts',(7.51492677113111,-71.0022170960235,12.));
#67688=CARTESIAN_POINT('Ctrl Pts',(7.50541298639948,-70.9814776989637,12.));
#67689=CARTESIAN_POINT('Ctrl Pts',(7.49593881811141,-70.9607699159234,12.));
#67690=CARTESIAN_POINT('Ctrl Pts',(7.48650426095822,-70.9400938988373,12.));
#67691=CARTESIAN_POINT('Ctrl Pts',(7.47710930950553,-70.9194498003483,12.));
#67692=CARTESIAN_POINT('Ctrl Pts',(7.46775395818518,-70.8988377738088,12.));
#67693=CARTESIAN_POINT('Ctrl Pts',(7.45843820129775,-70.8782579732885,12.));
#67694=CARTESIAN_POINT('Ctrl Pts',(7.44916203301644,-70.8577105535841,12.));
#67695=CARTESIAN_POINT('Ctrl Pts',(7.43992544738606,-70.8371956702242,12.));
#67696=CARTESIAN_POINT('Ctrl Pts',(7.43072843832007,-70.8167134794738,12.));
#67697=CARTESIAN_POINT('Ctrl Pts',(7.42157099959315,-70.7962641383351,12.));
#67698=CARTESIAN_POINT('Ctrl Pts',(7.41245312484486,-70.7758478045576,12.));
#67699=CARTESIAN_POINT('Ctrl Pts',(7.40337480758229,-70.7554646366514,12.));
#67700=CARTESIAN_POINT('Ctrl Pts',(7.3943360411789,-70.735114793895,12.));
#67701=CARTESIAN_POINT('Ctrl Pts',(7.38533681887032,-70.7147984363424,12.));
#67702=CARTESIAN_POINT('Ctrl Pts',(7.37637713374767,-70.694515724827,12.));
#67703=CARTESIAN_POINT('Ctrl Pts',(7.367456978763,-70.6742668209687,12.));
#67704=CARTESIAN_POINT('Ctrl Pts',(7.35857634673054,-70.6540518871775,12.));
#67705=CARTESIAN_POINT('Ctrl Pts',(7.34973523032577,-70.6338710866562,12.));
#67706=CARTESIAN_POINT('Ctrl Pts',(7.34093362208007,-70.6137245833996,12.));
#67707=CARTESIAN_POINT('Ctrl Pts',(7.3321715143759,-70.5936125421946,12.));
#67708=CARTESIAN_POINT('Ctrl Pts',(7.32344889945219,-70.5735351286476,12.));
#67709=CARTESIAN_POINT('Ctrl Pts',(7.31476576940391,-70.5534925092043,12.));
#67710=CARTESIAN_POINT('Ctrl Pts',(7.30612211618052,-70.5334848511681,12.));
#67711=CARTESIAN_POINT('Ctrl Pts',(7.29751793157822,-70.5135123227169,12.));
#67712=CARTESIAN_POINT('Ctrl Pts',(7.28895320723861,-70.4935750929058,12.));
#67713=CARTESIAN_POINT('Ctrl Pts',(7.2804279346547,-70.4736733316487,12.));
#67714=CARTESIAN_POINT('Ctrl Pts',(7.27194210517062,-70.4538072096992,12.));
#67715=CARTESIAN_POINT('Ctrl Pts',(7.26349570998032,-70.4339768986346,12.));
#67716=CARTESIAN_POINT('Ctrl Pts',(7.25508874012042,-70.4141825708178,12.));
#67717=CARTESIAN_POINT('Ctrl Pts',(7.24672118647084,-70.3944243994504,12.));
#67718=CARTESIAN_POINT('Ctrl Pts',(7.23839303975606,-70.3747025586552,12.));
#67719=CARTESIAN_POINT('Ctrl Pts',(7.23010429054228,-70.3550172235486,12.));
#67720=CARTESIAN_POINT('Ctrl Pts',(7.2218549292319,-70.3353685703112,12.));
#67721=CARTESIAN_POINT('Ctrl Pts',(7.21364494605449,-70.3157567762588,12.));
#67722=CARTESIAN_POINT('Ctrl Pts',(7.20547433107482,-70.2961820197077,12.));
#67723=CARTESIAN_POINT('Ctrl Pts',(7.19734307419872,-70.2766444798285,12.));
#67724=CARTESIAN_POINT('Ctrl Pts',(7.18925116517554,-70.2571443365192,12.));
#67725=CARTESIAN_POINT('Ctrl Pts',(7.18119859359777,-70.2376817702215,12.));
#67726=CARTESIAN_POINT('Ctrl Pts',(7.17318534889715,-70.2182569618994,12.));
#67727=CARTESIAN_POINT('Ctrl Pts',(7.16521142033863,-70.1988700934593,12.));
#67728=CARTESIAN_POINT('Ctrl Pts',(7.15727679700932,-70.1795213481185,12.));
#67729=CARTESIAN_POINT('Ctrl Pts',(7.14938146780813,-70.1602109107202,12.));
#67730=CARTESIAN_POINT('Ctrl Pts',(7.14152542142373,-70.1409389682424,12.));
#67731=CARTESIAN_POINT('Ctrl Pts',(7.13370864634442,-70.1217057094499,12.));
#67732=CARTESIAN_POINT('Ctrl Pts',(7.12593113088903,-70.1025113239495,12.));
#67733=CARTESIAN_POINT('Ctrl Pts',(7.11819286322825,-70.0833560013975,12.));
#67734=CARTESIAN_POINT('Ctrl Pts',(7.11049383140445,-70.0642399306869,12.));
#67735=CARTESIAN_POINT('Ctrl Pts',(7.10283402335033,-70.0451632990086,12.));
#67736=CARTESIAN_POINT('Ctrl Pts',(7.09521342684248,-70.0261262936388,12.));
#67737=CARTESIAN_POINT('Ctrl Pts',(7.08763202944245,-70.0071291040766,12.));
#67738=CARTESIAN_POINT('Ctrl Pts',(7.08008981844651,-69.988171923788,12.));
#67739=CARTESIAN_POINT('Ctrl Pts',(7.0725867808083,-69.9692549527296,12.));
#67740=CARTESIAN_POINT('Ctrl Pts',(7.06512290312849,-69.9503783975727,12.));
#67741=CARTESIAN_POINT('Ctrl Pts',(7.05769817180856,-69.9315424664291,12.));
#67742=CARTESIAN_POINT('Ctrl Pts',(7.05031257318115,-69.9127473642099,12.));
#67743=CARTESIAN_POINT('Ctrl Pts',(7.04296609362165,-69.8939932885841,12.));
#67744=CARTESIAN_POINT('Ctrl Pts',(7.0356587197222,-69.8752804235238,12.));
#67745=CARTESIAN_POINT('Ctrl Pts',(7.02839043811812,-69.8566089455375,12.));
#67746=CARTESIAN_POINT('Ctrl Pts',(7.02116123514451,-69.8379790360518,12.));
#67747=CARTESIAN_POINT('Ctrl Pts',(7.01397109655454,-69.8193908913722,12.));
#67748=CARTESIAN_POINT('Ctrl Pts',(7.0068200071815,-69.8008447346863,12.));
#67749=CARTESIAN_POINT('Ctrl Pts',(6.99970795069475,-69.782340824259,12.));
#67750=CARTESIAN_POINT('Ctrl Pts',(6.9926349102794,-69.7638794280419,12.));
#67751=CARTESIAN_POINT('Ctrl Pts',(6.98560086924213,-69.7454607995607,12.));
#67752=CARTESIAN_POINT('Ctrl Pts',(6.97860581164526,-69.7270851557366,12.));
#67753=CARTESIAN_POINT('Ctrl Pts',(6.97164972291439,-69.7087526479973,12.));
#67754=CARTESIAN_POINT('Ctrl Pts',(6.96473259049512,-69.6904633605421,12.));
#67755=CARTESIAN_POINT('Ctrl Pts',(6.9592300417359,-69.6758665380378,12.));
#67756=CARTESIAN_POINT('Ctrl Pts',(6.95512065317599,-69.664938391983,12.));
#67757=CARTESIAN_POINT('Ctrl Pts',(6.95238884849024,-69.6576616146467,12.));
#67758=CARTESIAN_POINT('Ctrl Pts',(6.95102489306925,-69.6540253893192,12.));
#67759=CARTESIAN_POINT('Ctrl Pts',(10.4355099267296,-73.4664795929938,-5.55111512312578E-16));
#67760=CARTESIAN_POINT('Ctrl Pts',(10.4355099267296,-73.4664795929938,4.));
#67761=CARTESIAN_POINT('Ctrl Pts',(10.4355099267296,-73.4664795929938,8.));
#67762=CARTESIAN_POINT('Ctrl Pts',(10.4355099267296,-73.4664795929938,12.));
#67763=CARTESIAN_POINT('Ctrl Pts',(10.4049225807075,-73.5720190200067,-5.55111512312578E-16));
#67764=CARTESIAN_POINT('Ctrl Pts',(10.4049225807075,-73.5720190200067,3.99999999999999));
#67765=CARTESIAN_POINT('Ctrl Pts',(10.4049225807075,-73.5720190200067,8.00000000000001));
#67766=CARTESIAN_POINT('Ctrl Pts',(10.4049225807075,-73.5720190200067,12.));
#67767=CARTESIAN_POINT('Ctrl Pts',(10.2883434191783,-73.7377969500798,-5.55111512312578E-16));
#67768=CARTESIAN_POINT('Ctrl Pts',(10.2883434191783,-73.7377969500798,4.00000000000001));
#67769=CARTESIAN_POINT('Ctrl Pts',(10.2883434191783,-73.7377969500798,7.99999999999999));
#67770=CARTESIAN_POINT('Ctrl Pts',(10.2883434191783,-73.7377969500798,12.));
#67771=CARTESIAN_POINT('Ctrl Pts',(10.1042001607579,-73.8116652760545,-5.55111512312578E-16));
#67772=CARTESIAN_POINT('Ctrl Pts',(10.1042001607579,-73.8116652760545,3.99999999999999));
#67773=CARTESIAN_POINT('Ctrl Pts',(10.1042001607579,-73.8116652760546,8.00000000000001));
#67774=CARTESIAN_POINT('Ctrl Pts',(10.1042001607579,-73.8116652760546,12.));
#67775=CARTESIAN_POINT('Ctrl Pts',(10.0225374821233,-73.8227522002495,-5.55111512312578E-16));
#67776=CARTESIAN_POINT('Ctrl Pts',(10.0225374821233,-73.8227522002495,4.));
#67777=CARTESIAN_POINT('Ctrl Pts',(10.0225374821233,-73.8227522002495,8.));
#67778=CARTESIAN_POINT('Ctrl Pts',(10.0225374821233,-73.8227522002495,12.));
#67779=CARTESIAN_POINT('',(10.4355099267296,-73.4664795929938,0.));
#67780=CARTESIAN_POINT('',(10.0225374821233,-73.8227522002494,0.));
#67781=CARTESIAN_POINT('Ctrl Pts',(10.4355099267296,-73.4664795929938,0.));
#67782=CARTESIAN_POINT('Ctrl Pts',(10.4049225807075,-73.5720190200067,-6.93334779979405E-31));
#67783=CARTESIAN_POINT('Ctrl Pts',(10.3383059169766,-73.6667492657628,3.85185988877447E-31));
#67784=CARTESIAN_POINT('Ctrl Pts',(10.2496275073219,-73.7314682122214,1.54074395550979E-31));
#67785=CARTESIAN_POINT('Ctrl Pts',(10.1831187000809,-73.7800074220654,-3.08148791101957E-32));
#67786=CARTESIAN_POINT('Ctrl Pts',(10.1042001607579,-73.8116652760545,-9.55261252416069E-31));
#67787=CARTESIAN_POINT('Ctrl Pts',(10.0225374821233,-73.8227522002495,4.62223186652938E-32));
#67788=CARTESIAN_POINT('',(10.0225374821233,-73.8227522002494,12.));
#67789=CARTESIAN_POINT('Ctrl Pts',(10.0225374821233,-73.8227522002495,-5.55111512312578E-16));
#67790=CARTESIAN_POINT('Ctrl Pts',(10.0225374821233,-73.8227522002495,4.));
#67791=CARTESIAN_POINT('Ctrl Pts',(10.0225374821233,-73.8227522002495,8.));
#67792=CARTESIAN_POINT('Ctrl Pts',(10.0225374821233,-73.8227522002495,12.));
#67793=CARTESIAN_POINT('',(10.4355099267296,-73.4664795929938,12.));
#67794=CARTESIAN_POINT('Ctrl Pts',(10.0225374821233,-73.8227522002495,12.));
#67795=CARTESIAN_POINT('Ctrl Pts',(10.1042001607579,-73.8116652760546,12.));
#67796=CARTESIAN_POINT('Ctrl Pts',(10.1831187000809,-73.7800074220654,12.));
#67797=CARTESIAN_POINT('Ctrl Pts',(10.2496275073219,-73.7314682122214,12.));
#67798=CARTESIAN_POINT('Ctrl Pts',(10.3383059169765,-73.6667492657628,12.));
#67799=CARTESIAN_POINT('Ctrl Pts',(10.4049225807075,-73.5720190200067,12.));
#67800=CARTESIAN_POINT('Ctrl Pts',(10.4355099267296,-73.4664795929938,12.));
#67801=CARTESIAN_POINT('Ctrl Pts',(10.4355099267296,-73.4664795929938,12.));
#67802=CARTESIAN_POINT('Ctrl Pts',(10.4355099267296,-73.4664795929938,8.));
#67803=CARTESIAN_POINT('Ctrl Pts',(10.4355099267296,-73.4664795929938,4.));
#67804=CARTESIAN_POINT('Ctrl Pts',(10.4355099267296,-73.4664795929938,-5.55111512312578E-16));
#67805=CARTESIAN_POINT('Origin',(4.90253386731613E-11,-3.71623968689858E-10,
0.));
#67806=CARTESIAN_POINT('Origin',(4.90253386731613E-11,-3.71623968689858E-10,
12.));
#67807=CARTESIAN_POINT('Origin',(4.90253386731613E-11,-3.71623968689858E-10,
0.));
#67808=CARTESIAN_POINT('Ctrl Pts',(2.94891377268305,-74.4416140848738,0.));
#67809=CARTESIAN_POINT('Ctrl Pts',(2.94891377268305,-74.4416140848738,4.));
#67810=CARTESIAN_POINT('Ctrl Pts',(2.94891377268299,-74.4416140848738,8.));
#67811=CARTESIAN_POINT('Ctrl Pts',(2.94891377268299,-74.4416140848738,12.));
#67812=CARTESIAN_POINT('Ctrl Pts',(2.83911742169683,-74.4459635334396,0.));
#67813=CARTESIAN_POINT('Ctrl Pts',(2.83911742169683,-74.4459635334396,4.));
#67814=CARTESIAN_POINT('Ctrl Pts',(2.83911742169676,-74.4459635334396,8.));
#67815=CARTESIAN_POINT('Ctrl Pts',(2.83911742169676,-74.4459635334396,12.));
#67816=CARTESIAN_POINT('Ctrl Pts',(2.64498412359382,-74.3877786926473,0.));
#67817=CARTESIAN_POINT('Ctrl Pts',(2.64498412359382,-74.3877786926473,4.));
#67818=CARTESIAN_POINT('Ctrl Pts',(2.64498412359375,-74.3877786926473,7.99999999999999));
#67819=CARTESIAN_POINT('Ctrl Pts',(2.64498412359375,-74.3877786926473,12.));
#67820=CARTESIAN_POINT('Ctrl Pts',(2.51668625693838,-74.2364344282704,0.));
#67821=CARTESIAN_POINT('Ctrl Pts',(2.51668625693838,-74.2364344282704,4.));
#67822=CARTESIAN_POINT('Ctrl Pts',(2.51668625693828,-74.2364344282705,8.00000000000001));
#67823=CARTESIAN_POINT('Ctrl Pts',(2.51668625693828,-74.2364344282705,12.));
#67824=CARTESIAN_POINT('Ctrl Pts',(2.48034921843256,-74.1624659714558,0.));
#67825=CARTESIAN_POINT('Ctrl Pts',(2.48034921843256,-74.1624659714558,4.));
#67826=CARTESIAN_POINT('Ctrl Pts',(2.48034921843243,-74.1624659714559,8.));
#67827=CARTESIAN_POINT('Ctrl Pts',(2.48034921843243,-74.1624659714559,12.));
#67828=CARTESIAN_POINT('',(2.94891377268305,-74.4416140848738,0.));
#67829=CARTESIAN_POINT('',(2.48034921843246,-74.1624659714559,0.));
#67830=CARTESIAN_POINT('Ctrl Pts',(2.94891377268305,-74.4416140848738,0.));
#67831=CARTESIAN_POINT('Ctrl Pts',(2.83911742169683,-74.4459635334396,0.));
#67832=CARTESIAN_POINT('Ctrl Pts',(2.72818410849511,-74.4127150529868,0.));
#67833=CARTESIAN_POINT('Ctrl Pts',(2.63874807903137,-74.3490471689147,0.));
#67834=CARTESIAN_POINT('Ctrl Pts',(2.57167105693357,-74.3012962558605,0.));
#67835=CARTESIAN_POINT('Ctrl Pts',(2.51668625693838,-74.2364344282704,0.));
#67836=CARTESIAN_POINT('Ctrl Pts',(2.48034921843256,-74.1624659714558,0.));
#67837=CARTESIAN_POINT('',(2.48034921843246,-74.1624659714559,12.));
#67838=CARTESIAN_POINT('Ctrl Pts',(2.48034921843256,-74.1624659714558,0.));
#67839=CARTESIAN_POINT('Ctrl Pts',(2.48034921843256,-74.1624659714558,4.));
#67840=CARTESIAN_POINT('Ctrl Pts',(2.48034921843243,-74.1624659714559,8.));
#67841=CARTESIAN_POINT('Ctrl Pts',(2.48034921843243,-74.1624659714559,12.));
#67842=CARTESIAN_POINT('',(2.94891377268299,-74.4416140848738,12.));
#67843=CARTESIAN_POINT('Ctrl Pts',(2.48034921843243,-74.1624659714559,12.));
#67844=CARTESIAN_POINT('Ctrl Pts',(2.51668625693828,-74.2364344282705,12.));
#67845=CARTESIAN_POINT('Ctrl Pts',(2.57167105693348,-74.3012962558605,12.));
#67846=CARTESIAN_POINT('Ctrl Pts',(2.63874807903129,-74.3490471689147,12.));
#67847=CARTESIAN_POINT('Ctrl Pts',(2.72818410849504,-74.4127150529869,12.));
#67848=CARTESIAN_POINT('Ctrl Pts',(2.83911742169676,-74.4459635334396,12.));
#67849=CARTESIAN_POINT('Ctrl Pts',(2.94891377268299,-74.4416140848738,12.));
#67850=CARTESIAN_POINT('Ctrl Pts',(2.94891377268299,-74.4416140848738,12.));
#67851=CARTESIAN_POINT('Ctrl Pts',(2.94891377268299,-74.4416140848738,8.));
#67852=CARTESIAN_POINT('Ctrl Pts',(2.94891377268305,-74.4416140848738,4.));
#67853=CARTESIAN_POINT('Ctrl Pts',(2.94891377268305,-74.4416140848738,0.));
#67854=CARTESIAN_POINT('Ctrl Pts',(0.853825826608976,-69.9947925310006,
0.));
#67855=CARTESIAN_POINT('Ctrl Pts',(0.853825826608976,-69.9947925310006,
12.));
#67856=CARTESIAN_POINT('Ctrl Pts',(0.854867673848587,-69.9985337959407,
0.));
#67857=CARTESIAN_POINT('Ctrl Pts',(0.854867673848587,-69.9985337959407,
12.));
#67858=CARTESIAN_POINT('Ctrl Pts',(0.856954870259198,-70.0060209754087,
0.));
#67859=CARTESIAN_POINT('Ctrl Pts',(0.856954870259198,-70.0060209754087,
12.));
#67860=CARTESIAN_POINT('Ctrl Pts',(0.860096170668728,-70.0172656933806,
0.));
#67861=CARTESIAN_POINT('Ctrl Pts',(0.860096170668728,-70.0172656933806,
12.));
#67862=CARTESIAN_POINT('Ctrl Pts',(0.864305583661538,-70.0322865492925,
0.));
#67863=CARTESIAN_POINT('Ctrl Pts',(0.864305583661538,-70.0322865492925,
12.));
#67864=CARTESIAN_POINT('Ctrl Pts',(0.869602377871117,-70.051109108301,0.));
#67865=CARTESIAN_POINT('Ctrl Pts',(0.869602377871117,-70.051109108301,12.));
#67866=CARTESIAN_POINT('Ctrl Pts',(0.874934213255831,-70.0699781183935,
0.));
#67867=CARTESIAN_POINT('Ctrl Pts',(0.874934213255831,-70.0699781183935,
12.));
#67868=CARTESIAN_POINT('Ctrl Pts',(0.880301109660721,-70.0888934967855,
0.));
#67869=CARTESIAN_POINT('Ctrl Pts',(0.880301109660721,-70.0888934967855,
12.));
#67870=CARTESIAN_POINT('Ctrl Pts',(0.885703094802528,-70.1078550938958,
0.));
#67871=CARTESIAN_POINT('Ctrl Pts',(0.885703094802528,-70.1078550938958,
12.));
#67872=CARTESIAN_POINT('Ctrl Pts',(0.891140203464235,-70.1268626950175,
0.));
#67873=CARTESIAN_POINT('Ctrl Pts',(0.891140203464235,-70.1268626950175,
12.));
#67874=CARTESIAN_POINT('Ctrl Pts',(0.896612474371837,-70.1459160490446,
0.));
#67875=CARTESIAN_POINT('Ctrl Pts',(0.896612474371837,-70.1459160490446,
12.));
#67876=CARTESIAN_POINT('Ctrl Pts',(0.902119947629764,-70.1650148905109,
0.));
#67877=CARTESIAN_POINT('Ctrl Pts',(0.902119947629764,-70.1650148905109,
12.));
#67878=CARTESIAN_POINT('Ctrl Pts',(0.907662662015778,-70.1841589635574,
0.));
#67879=CARTESIAN_POINT('Ctrl Pts',(0.907662662015778,-70.1841589635574,
12.));
#67880=CARTESIAN_POINT('Ctrl Pts',(0.913240652090973,-70.2033480471676,
0.));
#67881=CARTESIAN_POINT('Ctrl Pts',(0.913240652090973,-70.2033480471676,
12.));
#67882=CARTESIAN_POINT('Ctrl Pts',(0.918853949157111,-70.2225819470248,
0.));
#67883=CARTESIAN_POINT('Ctrl Pts',(0.918853949157111,-70.2225819470248,
12.));
#67884=CARTESIAN_POINT('Ctrl Pts',(0.924502582639448,-70.2418604835837,
0.));
#67885=CARTESIAN_POINT('Ctrl Pts',(0.924502582639448,-70.2418604835837,
12.));
#67886=CARTESIAN_POINT('Ctrl Pts',(0.93018658123554,-70.2611834821724,0.));
#67887=CARTESIAN_POINT('Ctrl Pts',(0.93018658123554,-70.2611834821724,12.));
#67888=CARTESIAN_POINT('Ctrl Pts',(0.935905974336473,-70.2805507606872,
0.));
#67889=CARTESIAN_POINT('Ctrl Pts',(0.935905974336473,-70.2805507606872,
12.));
#67890=CARTESIAN_POINT('Ctrl Pts',(0.941660792742972,-70.299962123399,0.));
#67891=CARTESIAN_POINT('Ctrl Pts',(0.941660792742972,-70.299962123399,12.));
#67892=CARTESIAN_POINT('Ctrl Pts',(0.947451067929597,-70.3194173673674,
0.));
#67893=CARTESIAN_POINT('Ctrl Pts',(0.947451067929597,-70.3194173673674,
12.));
#67894=CARTESIAN_POINT('Ctrl Pts',(0.953276831581235,-70.338916286458,0.));
#67895=CARTESIAN_POINT('Ctrl Pts',(0.953276831581235,-70.338916286458,12.));
#67896=CARTESIAN_POINT('Ctrl Pts',(0.959138115058824,-70.3584586759536,
0.));
#67897=CARTESIAN_POINT('Ctrl Pts',(0.959138115058824,-70.3584586759536,
12.));
#67898=CARTESIAN_POINT('Ctrl Pts',(0.965034948786442,-70.3780443377956,
0.));
#67899=CARTESIAN_POINT('Ctrl Pts',(0.965034948786442,-70.3780443377956,
12.));
#67900=CARTESIAN_POINT('Ctrl Pts',(0.970967362281167,-70.3976730803614,
0.));
#67901=CARTESIAN_POINT('Ctrl Pts',(0.970967362281167,-70.3976730803614,
12.));
#67902=CARTESIAN_POINT('Ctrl Pts',(0.976935384450034,-70.417344715957,0.));
#67903=CARTESIAN_POINT('Ctrl Pts',(0.976935384450034,-70.417344715957,12.));
#67904=CARTESIAN_POINT('Ctrl Pts',(0.982939043792148,-70.4370590590842,
0.));
#67905=CARTESIAN_POINT('Ctrl Pts',(0.982939043792148,-70.4370590590842,
12.));
#67906=CARTESIAN_POINT('Ctrl Pts',(0.988978368643642,-70.4568159243163,
0.));
#67907=CARTESIAN_POINT('Ctrl Pts',(0.988978368643642,-70.4568159243163,
12.));
#67908=CARTESIAN_POINT('Ctrl Pts',(0.995053387379748,-70.4766151245212,
0.));
#67909=CARTESIAN_POINT('Ctrl Pts',(0.995053387379748,-70.4766151245212,
12.));
#67910=CARTESIAN_POINT('Ctrl Pts',(1.00116412831442,-70.4964564717953,0.));
#67911=CARTESIAN_POINT('Ctrl Pts',(1.00116412831442,-70.4964564717953,12.));
#67912=CARTESIAN_POINT('Ctrl Pts',(1.00731061960967,-70.5163397782713,0.));
#67913=CARTESIAN_POINT('Ctrl Pts',(1.00731061960967,-70.5163397782713,12.));
#67914=CARTESIAN_POINT('Ctrl Pts',(1.01349288918536,-70.5362648569061,0.));
#67915=CARTESIAN_POINT('Ctrl Pts',(1.01349288918536,-70.5362648569061,12.));
#67916=CARTESIAN_POINT('Ctrl Pts',(1.01971096460596,-70.556231522419,0.));
#67917=CARTESIAN_POINT('Ctrl Pts',(1.01971096460596,-70.556231522419,12.));
#67918=CARTESIAN_POINT('Ctrl Pts',(1.02596487304048,-70.5762395916377,0.));
#67919=CARTESIAN_POINT('Ctrl Pts',(1.02596487304048,-70.5762395916377,12.));
#67920=CARTESIAN_POINT('Ctrl Pts',(1.0322546413287,-70.5962888829934,0.));
#67921=CARTESIAN_POINT('Ctrl Pts',(1.0322546413287,-70.5962888829934,12.));
#67922=CARTESIAN_POINT('Ctrl Pts',(1.03858029601903,-70.6163792162073,0.));
#67923=CARTESIAN_POINT('Ctrl Pts',(1.03858029601903,-70.6163792162073,12.));
#67924=CARTESIAN_POINT('Ctrl Pts',(1.04494186341155,-70.6365104119252,0.));
#67925=CARTESIAN_POINT('Ctrl Pts',(1.04494186341155,-70.6365104119252,12.));
#67926=CARTESIAN_POINT('Ctrl Pts',(1.05133936960071,-70.6566822912991,0.));
#67927=CARTESIAN_POINT('Ctrl Pts',(1.05133936960071,-70.6566822912991,12.));
#67928=CARTESIAN_POINT('Ctrl Pts',(1.05777284047729,-70.676894676009,0.));
#67929=CARTESIAN_POINT('Ctrl Pts',(1.05777284047729,-70.676894676009,12.));
#67930=CARTESIAN_POINT('Ctrl Pts',(1.0642423017128,-70.6971473884459,0.));
#67931=CARTESIAN_POINT('Ctrl Pts',(1.0642423017128,-70.6971473884459,12.));
#67932=CARTESIAN_POINT('Ctrl Pts',(1.07074777874595,-70.7174402518378,0.));
#67933=CARTESIAN_POINT('Ctrl Pts',(1.07074777874595,-70.7174402518378,12.));
#67934=CARTESIAN_POINT('Ctrl Pts',(1.07728929676408,-70.7377730903953,0.));
#67935=CARTESIAN_POINT('Ctrl Pts',(1.07728929676408,-70.7377730903953,12.));
#67936=CARTESIAN_POINT('Ctrl Pts',(1.08386688068342,-70.7581457294447,0.));
#67937=CARTESIAN_POINT('Ctrl Pts',(1.08386688068342,-70.7581457294447,12.));
#67938=CARTESIAN_POINT('Ctrl Pts',(1.09048055516426,-70.7785579953583,0.));
#67939=CARTESIAN_POINT('Ctrl Pts',(1.09048055516426,-70.7785579953583,12.));
#67940=CARTESIAN_POINT('Ctrl Pts',(1.09713034462265,-70.799009715484,0.));
#67941=CARTESIAN_POINT('Ctrl Pts',(1.09713034462265,-70.799009715484,12.));
#67942=CARTESIAN_POINT('Ctrl Pts',(1.10381627323946,-70.8195007180745,0.));
#67943=CARTESIAN_POINT('Ctrl Pts',(1.10381627323946,-70.8195007180745,12.));
#67944=CARTESIAN_POINT('Ctrl Pts',(1.11053836496639,-70.8400308322037,0.));
#67945=CARTESIAN_POINT('Ctrl Pts',(1.11053836496639,-70.8400308322037,12.));
#67946=CARTESIAN_POINT('Ctrl Pts',(1.11729664352992,-70.8605998877149,0.));
#67947=CARTESIAN_POINT('Ctrl Pts',(1.11729664352992,-70.8605998877149,12.));
#67948=CARTESIAN_POINT('Ctrl Pts',(1.12409113243513,-70.8812077152586,0.));
#67949=CARTESIAN_POINT('Ctrl Pts',(1.12409113243513,-70.8812077152586,12.));
#67950=CARTESIAN_POINT('Ctrl Pts',(1.13092185496564,-70.9018541463089,0.));
#67951=CARTESIAN_POINT('Ctrl Pts',(1.13092185496564,-70.9018541463089,12.));
#67952=CARTESIAN_POINT('Ctrl Pts',(1.13778883418213,-70.9225390131826,0.));
#67953=CARTESIAN_POINT('Ctrl Pts',(1.13778883418213,-70.9225390131826,12.));
#67954=CARTESIAN_POINT('Ctrl Pts',(1.14469209291488,-70.9432621490566,0.));
#67955=CARTESIAN_POINT('Ctrl Pts',(1.14469209291488,-70.9432621490566,12.));
#67956=CARTESIAN_POINT('Ctrl Pts',(1.15163165376523,-70.9640233879659,0.));
#67957=CARTESIAN_POINT('Ctrl Pts',(1.15163165376523,-70.9640233879659,12.));
#67958=CARTESIAN_POINT('Ctrl Pts',(1.15860753911484,-70.9848225647871,0.));
#67959=CARTESIAN_POINT('Ctrl Pts',(1.15860753911484,-70.9848225647871,12.));
#67960=CARTESIAN_POINT('Ctrl Pts',(1.1656197711288,-71.0056595152204,0.));
#67961=CARTESIAN_POINT('Ctrl Pts',(1.1656197711288,-71.0056595152204,12.));
#67962=CARTESIAN_POINT('Ctrl Pts',(1.17266837175776,-71.0265340757699,0.));
#67963=CARTESIAN_POINT('Ctrl Pts',(1.17266837175776,-71.0265340757699,12.));
#67964=CARTESIAN_POINT('Ctrl Pts',(1.17975336273503,-71.0474460837159,0.));
#67965=CARTESIAN_POINT('Ctrl Pts',(1.17975336273503,-71.0474460837159,12.));
#67966=CARTESIAN_POINT('Ctrl Pts',(1.18687476558132,-71.0683953771149,0.));
#67967=CARTESIAN_POINT('Ctrl Pts',(1.18687476558132,-71.0683953771149,12.));
#67968=CARTESIAN_POINT('Ctrl Pts',(1.19403260161001,-71.089381794801,0.));
#67969=CARTESIAN_POINT('Ctrl Pts',(1.19403260161001,-71.089381794801,12.));
#67970=CARTESIAN_POINT('Ctrl Pts',(1.20122689192835,-71.1104051763839,0.));
#67971=CARTESIAN_POINT('Ctrl Pts',(1.20122689192835,-71.1104051763839,12.));
#67972=CARTESIAN_POINT('Ctrl Pts',(1.20845765743647,-71.1314653622442,0.));
#67973=CARTESIAN_POINT('Ctrl Pts',(1.20845765743647,-71.1314653622442,12.));
#67974=CARTESIAN_POINT('Ctrl Pts',(1.21572491882262,-71.1525621935267,0.));
#67975=CARTESIAN_POINT('Ctrl Pts',(1.21572491882262,-71.1525621935267,12.));
#67976=CARTESIAN_POINT('Ctrl Pts',(1.22302869657017,-71.1736955121362,0.));
#67977=CARTESIAN_POINT('Ctrl Pts',(1.22302869657017,-71.1736955121362,12.));
#67978=CARTESIAN_POINT('Ctrl Pts',(1.23036901096238,-71.194865160732,0.));
#67979=CARTESIAN_POINT('Ctrl Pts',(1.23036901096238,-71.194865160732,12.));
#67980=CARTESIAN_POINT('Ctrl Pts',(1.23774588208426,-71.2160709827191,0.));
#67981=CARTESIAN_POINT('Ctrl Pts',(1.23774588208426,-71.2160709827191,12.));
#67982=CARTESIAN_POINT('Ctrl Pts',(1.24515932982112,-71.2373128222352,0.));
#67983=CARTESIAN_POINT('Ctrl Pts',(1.24515932982112,-71.2373128222352,12.));
#67984=CARTESIAN_POINT('Ctrl Pts',(1.25260937385568,-71.2585905241406,0.));
#67985=CARTESIAN_POINT('Ctrl Pts',(1.25260937385568,-71.2585905241406,12.));
#67986=CARTESIAN_POINT('Ctrl Pts',(1.2600960336757,-71.2799039340175,0.));
#67987=CARTESIAN_POINT('Ctrl Pts',(1.2600960336757,-71.2799039340175,12.));
#67988=CARTESIAN_POINT('Ctrl Pts',(1.26761932857724,-71.3012528981661,0.));
#67989=CARTESIAN_POINT('Ctrl Pts',(1.26761932857724,-71.3012528981661,12.));
#67990=CARTESIAN_POINT('Ctrl Pts',(1.27517927766607,-71.3226372635996,0.));
#67991=CARTESIAN_POINT('Ctrl Pts',(1.27517927766607,-71.3226372635996,12.));
#67992=CARTESIAN_POINT('Ctrl Pts',(1.28277589985471,-71.3440568780347,0.));
#67993=CARTESIAN_POINT('Ctrl Pts',(1.28277589985471,-71.3440568780347,12.));
#67994=CARTESIAN_POINT('Ctrl Pts',(1.29040921386058,-71.3655115898827,0.));
#67995=CARTESIAN_POINT('Ctrl Pts',(1.29040921386058,-71.3655115898827,12.));
#67996=CARTESIAN_POINT('Ctrl Pts',(1.29807923821413,-71.3870012482499,0.));
#67997=CARTESIAN_POINT('Ctrl Pts',(1.29807923821413,-71.3870012482499,12.));
#67998=CARTESIAN_POINT('Ctrl Pts',(1.30578599126139,-71.4085257029322,0.));
#67999=CARTESIAN_POINT('Ctrl Pts',(1.30578599126139,-71.4085257029322,12.));
#68000=CARTESIAN_POINT('Ctrl Pts',(1.31352949116536,-71.4300848044087,0.));
#68001=CARTESIAN_POINT('Ctrl Pts',(1.31352949116536,-71.4300848044087,12.));
#68002=CARTESIAN_POINT('Ctrl Pts',(1.32130975590225,-71.4516784038317,0.));
#68003=CARTESIAN_POINT('Ctrl Pts',(1.32130975590225,-71.4516784038317,12.));
#68004=CARTESIAN_POINT('Ctrl Pts',(1.32912680326123,-71.4733063530187,0.));
#68005=CARTESIAN_POINT('Ctrl Pts',(1.32912680326123,-71.4733063530187,12.));
#68006=CARTESIAN_POINT('Ctrl Pts',(1.33698065085219,-71.4949685044522,0.));
#68007=CARTESIAN_POINT('Ctrl Pts',(1.33698065085219,-71.4949685044522,12.));
#68008=CARTESIAN_POINT('Ctrl Pts',(1.3448713161078,-71.516664711275,0.));
#68009=CARTESIAN_POINT('Ctrl Pts',(1.3448713161078,-71.516664711275,12.));
#68010=CARTESIAN_POINT('Ctrl Pts',(1.35279881628454,-71.5383948272845,0.));
#68011=CARTESIAN_POINT('Ctrl Pts',(1.35279881628454,-71.5383948272845,12.));
#68012=CARTESIAN_POINT('Ctrl Pts',(1.36076316845815,-71.5601587069217,0.));
#68013=CARTESIAN_POINT('Ctrl Pts',(1.36076316845815,-71.5601587069217,12.));
#68014=CARTESIAN_POINT('Ctrl Pts',(1.36876438952465,-71.5819562052663,0.));
#68015=CARTESIAN_POINT('Ctrl Pts',(1.36876438952465,-71.5819562052663,12.));
#68016=CARTESIAN_POINT('Ctrl Pts',(1.37680249620779,-71.6037871780385,0.));
#68017=CARTESIAN_POINT('Ctrl Pts',(1.37680249620779,-71.6037871780385,12.));
#68018=CARTESIAN_POINT('Ctrl Pts',(1.38487750506081,-71.625651481593,0.));
#68019=CARTESIAN_POINT('Ctrl Pts',(1.38487750506081,-71.625651481593,12.));
#68020=CARTESIAN_POINT('Ctrl Pts',(1.39298943246721,-71.6475489729134,0.));
#68021=CARTESIAN_POINT('Ctrl Pts',(1.39298943246721,-71.6475489729134,12.));
#68022=CARTESIAN_POINT('Ctrl Pts',(1.40113829463576,-71.6694795096001,0.));
#68023=CARTESIAN_POINT('Ctrl Pts',(1.40113829463576,-71.6694795096001,12.));
#68024=CARTESIAN_POINT('Ctrl Pts',(1.40932410760247,-71.6914429498663,0.));
#68025=CARTESIAN_POINT('Ctrl Pts',(1.40932410760247,-71.6914429498663,12.));
#68026=CARTESIAN_POINT('Ctrl Pts',(1.41754688723772,-71.7134391525389,0.));
#68027=CARTESIAN_POINT('Ctrl Pts',(1.41754688723772,-71.7134391525389,12.));
#68028=CARTESIAN_POINT('Ctrl Pts',(1.42580664924769,-71.7354679770528,0.));
#68029=CARTESIAN_POINT('Ctrl Pts',(1.42580664924769,-71.7354679770528,12.));
#68030=CARTESIAN_POINT('Ctrl Pts',(1.43410340917495,-71.7575292834469,0.));
#68031=CARTESIAN_POINT('Ctrl Pts',(1.43410340917495,-71.7575292834469,12.));
#68032=CARTESIAN_POINT('Ctrl Pts',(1.44243718239314,-71.7796229323526,0.));
#68033=CARTESIAN_POINT('Ctrl Pts',(1.44243718239314,-71.7796229323526,12.));
#68034=CARTESIAN_POINT('Ctrl Pts',(1.45080798410964,-71.8017487849895,0.));
#68035=CARTESIAN_POINT('Ctrl Pts',(1.45080798410964,-71.8017487849895,12.));
#68036=CARTESIAN_POINT('Ctrl Pts',(1.45921582937231,-71.8239067031683,0.));
#68037=CARTESIAN_POINT('Ctrl Pts',(1.45921582937231,-71.8239067031683,12.));
#68038=CARTESIAN_POINT('Ctrl Pts',(1.46766073307087,-71.8460965492839,0.));
#68039=CARTESIAN_POINT('Ctrl Pts',(1.46766073307087,-71.8460965492839,12.));
#68040=CARTESIAN_POINT('Ctrl Pts',(1.47614270993728,-71.8683181863116,0.));
#68041=CARTESIAN_POINT('Ctrl Pts',(1.47614270993728,-71.8683181863116,12.));
#68042=CARTESIAN_POINT('Ctrl Pts',(1.48466177454019,-71.8905714777961,0.));
#68043=CARTESIAN_POINT('Ctrl Pts',(1.48466177454019,-71.8905714777961,12.));
#68044=CARTESIAN_POINT('Ctrl Pts',(1.49321794128798,-71.912856287848,0.));
#68045=CARTESIAN_POINT('Ctrl Pts',(1.49321794128798,-71.912856287848,12.));
#68046=CARTESIAN_POINT('Ctrl Pts',(1.50181122443533,-71.9351724811443,0.));
#68047=CARTESIAN_POINT('Ctrl Pts',(1.50181122443533,-71.9351724811443,12.));
#68048=CARTESIAN_POINT('Ctrl Pts',(1.51044163808453,-71.9575199229241,0.));
#68049=CARTESIAN_POINT('Ctrl Pts',(1.51044163808453,-71.9575199229241,12.));
#68050=CARTESIAN_POINT('Ctrl Pts',(1.51910919618565,-71.979898478983,0.));
#68051=CARTESIAN_POINT('Ctrl Pts',(1.51910919618565,-71.979898478983,12.));
#68052=CARTESIAN_POINT('Ctrl Pts',(1.52781391253101,-72.0023080156647,0.));
#68053=CARTESIAN_POINT('Ctrl Pts',(1.52781391253101,-72.0023080156647,12.));
#68054=CARTESIAN_POINT('Ctrl Pts',(1.53655580075812,-72.0247483998579,0.));
#68055=CARTESIAN_POINT('Ctrl Pts',(1.53655580075812,-72.0247483998579,12.));
#68056=CARTESIAN_POINT('Ctrl Pts',(1.54533487435625,-72.0472194989963,0.));
#68057=CARTESIAN_POINT('Ctrl Pts',(1.54533487435625,-72.0472194989963,12.));
#68058=CARTESIAN_POINT('Ctrl Pts',(1.55415114666773,-72.0697211810545,0.));
#68059=CARTESIAN_POINT('Ctrl Pts',(1.55415114666773,-72.0697211810545,12.));
#68060=CARTESIAN_POINT('Ctrl Pts',(1.56300463088808,-72.0922533145433,0.));
#68061=CARTESIAN_POINT('Ctrl Pts',(1.56300463088808,-72.0922533145433,12.));
#68062=CARTESIAN_POINT('Ctrl Pts',(1.5718953400604,-72.1148157684995,0.));
#68063=CARTESIAN_POINT('Ctrl Pts',(1.5718953400604,-72.1148157684995,12.));
#68064=CARTESIAN_POINT('Ctrl Pts',(1.58082328707802,-72.1374084124839,0.));
#68065=CARTESIAN_POINT('Ctrl Pts',(1.58082328707802,-72.1374084124839,12.));
#68066=CARTESIAN_POINT('Ctrl Pts',(1.58978848469122,-72.1600311165821,0.));
#68067=CARTESIAN_POINT('Ctrl Pts',(1.58978848469122,-72.1600311165821,12.));
#68068=CARTESIAN_POINT('Ctrl Pts',(1.59879094550846,-72.1826837514001,0.));
#68069=CARTESIAN_POINT('Ctrl Pts',(1.59879094550846,-72.1826837514001,12.));
#68070=CARTESIAN_POINT('Ctrl Pts',(1.60783068199662,-72.2053661880608,0.));
#68071=CARTESIAN_POINT('Ctrl Pts',(1.60783068199662,-72.2053661880608,12.));
#68072=CARTESIAN_POINT('Ctrl Pts',(1.61690770647539,-72.2280782981937,0.));
#68073=CARTESIAN_POINT('Ctrl Pts',(1.61690770647539,-72.2280782981937,12.));
#68074=CARTESIAN_POINT('Ctrl Pts',(1.62602203111929,-72.2508199539323,0.));
#68075=CARTESIAN_POINT('Ctrl Pts',(1.62602203111929,-72.2508199539323,12.));
#68076=CARTESIAN_POINT('Ctrl Pts',(1.63517366796462,-72.2735910279149,0.));
#68077=CARTESIAN_POINT('Ctrl Pts',(1.63517366796462,-72.2735910279149,12.));
#68078=CARTESIAN_POINT('Ctrl Pts',(1.64436262891078,-72.2963913932813,0.));
#68079=CARTESIAN_POINT('Ctrl Pts',(1.64436262891078,-72.2963913932813,12.));
#68080=CARTESIAN_POINT('Ctrl Pts',(1.65358892572062,-72.319220923669,0.));
#68081=CARTESIAN_POINT('Ctrl Pts',(1.65358892572062,-72.319220923669,12.));
#68082=CARTESIAN_POINT('Ctrl Pts',(1.66285257001496,-72.3420794932047,0.));
#68083=CARTESIAN_POINT('Ctrl Pts',(1.66285257001496,-72.3420794932047,12.));
#68084=CARTESIAN_POINT('Ctrl Pts',(1.67215357327364,-72.3649669765004,0.));
#68085=CARTESIAN_POINT('Ctrl Pts',(1.67215357327364,-72.3649669765004,12.));
#68086=CARTESIAN_POINT('Ctrl Pts',(1.68149194684281,-72.387883248654,0.));
#68087=CARTESIAN_POINT('Ctrl Pts',(1.68149194684281,-72.387883248654,12.));
#68088=CARTESIAN_POINT('Ctrl Pts',(1.69086770193636,-72.4108281852467,0.));
#68089=CARTESIAN_POINT('Ctrl Pts',(1.69086770193636,-72.4108281852467,12.));
#68090=CARTESIAN_POINT('Ctrl Pts',(1.70028084963647,-72.4338016623391,0.));
#68091=CARTESIAN_POINT('Ctrl Pts',(1.70028084963647,-72.4338016623391,12.));
#68092=CARTESIAN_POINT('Ctrl Pts',(1.70973140088841,-72.456803556463,0.));
#68093=CARTESIAN_POINT('Ctrl Pts',(1.70973140088841,-72.456803556463,12.));
#68094=CARTESIAN_POINT('Ctrl Pts',(1.71921936650037,-72.479833744618,0.));
#68095=CARTESIAN_POINT('Ctrl Pts',(1.71921936650037,-72.479833744618,12.));
#68096=CARTESIAN_POINT('Ctrl Pts',(1.72874475715102,-72.5028921042721,0.));
#68097=CARTESIAN_POINT('Ctrl Pts',(1.72874475715102,-72.5028921042721,12.));
#68098=CARTESIAN_POINT('Ctrl Pts',(1.73830758339124,-72.5259785133595,0.));
#68099=CARTESIAN_POINT('Ctrl Pts',(1.73830758339124,-72.5259785133595,12.));
#68100=CARTESIAN_POINT('Ctrl Pts',(1.74790785564473,-72.5490928502769,0.));
#68101=CARTESIAN_POINT('Ctrl Pts',(1.74790785564473,-72.5490928502769,12.));
#68102=CARTESIAN_POINT('Ctrl Pts',(1.75754558420343,-72.5722349938774,0.));
#68103=CARTESIAN_POINT('Ctrl Pts',(1.75754558420343,-72.5722349938774,12.));
#68104=CARTESIAN_POINT('Ctrl Pts',(1.76722077922574,-72.5954048234638,0.));
#68105=CARTESIAN_POINT('Ctrl Pts',(1.76722077922574,-72.5954048234638,12.));
#68106=CARTESIAN_POINT('Ctrl Pts',(1.77693345074426,-72.6186022187907,0.));
#68107=CARTESIAN_POINT('Ctrl Pts',(1.77693345074426,-72.6186022187907,12.));
#68108=CARTESIAN_POINT('Ctrl Pts',(1.7866836086681,-72.6418270600619,0.));
#68109=CARTESIAN_POINT('Ctrl Pts',(1.7866836086681,-72.6418270600619,12.));
#68110=CARTESIAN_POINT('Ctrl Pts',(1.79647126278358,-72.6650792279274,0.));
#68111=CARTESIAN_POINT('Ctrl Pts',(1.79647126278358,-72.6650792279274,12.));
#68112=CARTESIAN_POINT('Ctrl Pts',(1.8062964227505,-72.6883586034769,0.));
#68113=CARTESIAN_POINT('Ctrl Pts',(1.8062964227505,-72.6883586034769,12.));
#68114=CARTESIAN_POINT('Ctrl Pts',(1.8161590980987,-72.7116650682344,0.));
#68115=CARTESIAN_POINT('Ctrl Pts',(1.8161590980987,-72.7116650682344,12.));
#68116=CARTESIAN_POINT('Ctrl Pts',(1.82605929823564,-72.7349985041592,0.));
#68117=CARTESIAN_POINT('Ctrl Pts',(1.82605929823564,-72.7349985041592,12.));
#68118=CARTESIAN_POINT('Ctrl Pts',(1.83599703244924,-72.7583587936447,0.));
#68119=CARTESIAN_POINT('Ctrl Pts',(1.83599703244924,-72.7583587936447,12.));
#68120=CARTESIAN_POINT('Ctrl Pts',(1.84597230990856,-72.7817458195155,0.));
#68121=CARTESIAN_POINT('Ctrl Pts',(1.84597230990856,-72.7817458195155,12.));
#68122=CARTESIAN_POINT('Ctrl Pts',(1.85598513966113,-72.8051594650222,0.));
#68123=CARTESIAN_POINT('Ctrl Pts',(1.85598513966113,-72.8051594650222,12.));
#68124=CARTESIAN_POINT('Ctrl Pts',(1.8660355306277,-72.8285996138359,0.));
#68125=CARTESIAN_POINT('Ctrl Pts',(1.8660355306277,-72.8285996138359,12.));
#68126=CARTESIAN_POINT('Ctrl Pts',(1.87612349160944,-72.8520661500477,0.));
#68127=CARTESIAN_POINT('Ctrl Pts',(1.87612349160944,-72.8520661500477,12.));
#68128=CARTESIAN_POINT('Ctrl Pts',(1.88624903129187,-72.875558958168,0.));
#68129=CARTESIAN_POINT('Ctrl Pts',(1.88624903129187,-72.875558958168,12.));
#68130=CARTESIAN_POINT('Ctrl Pts',(1.89641215824581,-72.8990779231226,0.));
#68131=CARTESIAN_POINT('Ctrl Pts',(1.89641215824581,-72.8990779231226,12.));
#68132=CARTESIAN_POINT('Ctrl Pts',(1.90661288092586,-72.9226229302478,0.));
#68133=CARTESIAN_POINT('Ctrl Pts',(1.90661288092586,-72.9226229302478,12.));
#68134=CARTESIAN_POINT('Ctrl Pts',(1.91685120766436,-72.9461938652811,0.));
#68135=CARTESIAN_POINT('Ctrl Pts',(1.91685120766436,-72.9461938652811,12.));
#68136=CARTESIAN_POINT('Ctrl Pts',(1.9271271466766,-72.9697906143636,0.));
#68137=CARTESIAN_POINT('Ctrl Pts',(1.9271271466766,-72.9697906143636,12.));
#68138=CARTESIAN_POINT('Ctrl Pts',(1.93744070606565,-72.9934130640415,0.));
#68139=CARTESIAN_POINT('Ctrl Pts',(1.93744070606565,-72.9934130640415,12.));
#68140=CARTESIAN_POINT('Ctrl Pts',(1.94779189382301,-73.0170611012661,0.));
#68141=CARTESIAN_POINT('Ctrl Pts',(1.94779189382301,-73.0170611012661,12.));
#68142=CARTESIAN_POINT('Ctrl Pts',(1.95818071782766,-73.040734613391,0.));
#68143=CARTESIAN_POINT('Ctrl Pts',(1.95818071782766,-73.040734613391,12.));
#68144=CARTESIAN_POINT('Ctrl Pts',(1.96860718583931,-73.0644334881673,0.));
#68145=CARTESIAN_POINT('Ctrl Pts',(1.96860718583931,-73.0644334881673,12.));
#68146=CARTESIAN_POINT('Ctrl Pts',(1.97907130550157,-73.0881576137407,0.));
#68147=CARTESIAN_POINT('Ctrl Pts',(1.97907130550157,-73.0881576137407,12.));
#68148=CARTESIAN_POINT('Ctrl Pts',(1.98957308434917,-73.1119068786475,0.));
#68149=CARTESIAN_POINT('Ctrl Pts',(1.98957308434917,-73.1119068786475,12.));
#68150=CARTESIAN_POINT('Ctrl Pts',(2.00011252980981,-73.1356811718091,0.));
#68151=CARTESIAN_POINT('Ctrl Pts',(2.00011252980981,-73.1356811718091,12.));
#68152=CARTESIAN_POINT('Ctrl Pts',(2.01068964920466,-73.1594803825252,0.));
#68153=CARTESIAN_POINT('Ctrl Pts',(2.01068964920466,-73.1594803825252,12.));
#68154=CARTESIAN_POINT('Ctrl Pts',(2.02130444974361,-73.183304400462,0.));
#68155=CARTESIAN_POINT('Ctrl Pts',(2.02130444974361,-73.183304400462,12.));
#68156=CARTESIAN_POINT('Ctrl Pts',(2.03195693852454,-73.2071531156504,0.));
#68157=CARTESIAN_POINT('Ctrl Pts',(2.03195693852454,-73.2071531156504,12.));
#68158=CARTESIAN_POINT('Ctrl Pts',(2.04264712253928,-73.2310264184976,0.));
#68159=CARTESIAN_POINT('Ctrl Pts',(2.04264712253928,-73.2310264184976,12.));
#68160=CARTESIAN_POINT('Ctrl Pts',(2.05337500867402,-73.2549241997953,0.));
#68161=CARTESIAN_POINT('Ctrl Pts',(2.05337500867402,-73.2549241997953,12.));
#68162=CARTESIAN_POINT('Ctrl Pts',(2.06414060370834,-73.2788463507246,0.));
#68163=CARTESIAN_POINT('Ctrl Pts',(2.06414060370834,-73.2788463507246,12.));
#68164=CARTESIAN_POINT('Ctrl Pts',(2.0749439143094,-73.3027927628626,0.));
#68165=CARTESIAN_POINT('Ctrl Pts',(2.0749439143094,-73.3027927628626,12.));
#68166=CARTESIAN_POINT('Ctrl Pts',(2.08578494702743,-73.3267633281807,0.));
#68167=CARTESIAN_POINT('Ctrl Pts',(2.08578494702743,-73.3267633281807,12.));
#68168=CARTESIAN_POINT('Ctrl Pts',(2.09666370830715,-73.3507579390239,0.));
#68169=CARTESIAN_POINT('Ctrl Pts',(2.09666370830715,-73.3507579390239,12.));
#68170=CARTESIAN_POINT('Ctrl Pts',(2.10758020449389,-73.3747764880893,0.));
#68171=CARTESIAN_POINT('Ctrl Pts',(2.10758020449389,-73.3747764880893,12.));
#68172=CARTESIAN_POINT('Ctrl Pts',(2.11853444183761,-73.3988188684021,0.));
#68173=CARTESIAN_POINT('Ctrl Pts',(2.11853444183761,-73.3988188684021,12.));
#68174=CARTESIAN_POINT('Ctrl Pts',(2.12952642649367,-73.4228849732925,0.));
#68175=CARTESIAN_POINT('Ctrl Pts',(2.12952642649367,-73.4228849732925,12.));
#68176=CARTESIAN_POINT('Ctrl Pts',(2.14055616452057,-73.4469746963637,0.));
#68177=CARTESIAN_POINT('Ctrl Pts',(2.14055616452057,-73.4469746963637,12.));
#68178=CARTESIAN_POINT('Ctrl Pts',(2.15162366187906,-73.4710879315382,0.));
#68179=CARTESIAN_POINT('Ctrl Pts',(2.15162366187906,-73.4710879315382,12.));
#68180=CARTESIAN_POINT('Ctrl Pts',(2.16272892442919,-73.4952245731054,0.));
#68181=CARTESIAN_POINT('Ctrl Pts',(2.16272892442919,-73.4952245731054,12.));
#68182=CARTESIAN_POINT('Ctrl Pts',(2.17387195792305,-73.5193845157708,0.));
#68183=CARTESIAN_POINT('Ctrl Pts',(2.17387195792305,-73.5193845157708,12.));
#68184=CARTESIAN_POINT('Ctrl Pts',(2.18505276799752,-73.5435676546929,0.));
#68185=CARTESIAN_POINT('Ctrl Pts',(2.18505276799752,-73.5435676546929,12.));
#68186=CARTESIAN_POINT('Ctrl Pts',(2.19627136015677,-73.5677738855452,0.));
#68187=CARTESIAN_POINT('Ctrl Pts',(2.19627136015677,-73.5677738855452,12.));
#68188=CARTESIAN_POINT('Ctrl Pts',(2.20752773978348,-73.5920031044595,0.));
#68189=CARTESIAN_POINT('Ctrl Pts',(2.20752773978348,-73.5920031044595,12.));
#68190=CARTESIAN_POINT('Ctrl Pts',(2.21882191216517,-73.6162552079038,0.));
#68191=CARTESIAN_POINT('Ctrl Pts',(2.21882191216517,-73.6162552079038,12.));
#68192=CARTESIAN_POINT('Ctrl Pts',(2.23015388251287,-73.6405300925712,0.));
#68193=CARTESIAN_POINT('Ctrl Pts',(2.23015388251287,-73.6405300925712,12.));
#68194=CARTESIAN_POINT('Ctrl Pts',(2.24152365597697,-73.6648276552767,0.));
#68195=CARTESIAN_POINT('Ctrl Pts',(2.24152365597697,-73.6648276552767,12.));
#68196=CARTESIAN_POINT('Ctrl Pts',(2.25293123766424,-73.6891477928129,0.));
#68197=CARTESIAN_POINT('Ctrl Pts',(2.25293123766424,-73.6891477928129,12.));
#68198=CARTESIAN_POINT('Ctrl Pts',(2.26437663263666,-73.7134904019389,0.));
#68199=CARTESIAN_POINT('Ctrl Pts',(2.26437663263666,-73.7134904019389,12.));
#68200=CARTESIAN_POINT('Ctrl Pts',(2.27585984587198,-73.7378553796807,0.));
#68201=CARTESIAN_POINT('Ctrl Pts',(2.27585984587198,-73.7378553796807,12.));
#68202=CARTESIAN_POINT('Ctrl Pts',(2.28738088222863,-73.762242623566,0.));
#68203=CARTESIAN_POINT('Ctrl Pts',(2.28738088222863,-73.762242623566,12.));
#68204=CARTESIAN_POINT('Ctrl Pts',(2.29893974640434,-73.786652031885,0.));
#68205=CARTESIAN_POINT('Ctrl Pts',(2.29893974640434,-73.786652031885,12.));
#68206=CARTESIAN_POINT('Ctrl Pts',(2.31053644289416,-73.8110835039327,0.));
#68207=CARTESIAN_POINT('Ctrl Pts',(2.31053644289416,-73.8110835039327,12.));
#68208=CARTESIAN_POINT('Ctrl Pts',(2.32217097594197,-73.8355369402706,0.));
#68209=CARTESIAN_POINT('Ctrl Pts',(2.32217097594197,-73.8355369402706,12.));
#68210=CARTESIAN_POINT('Ctrl Pts',(2.33384334963957,-73.8600122421468,0.));
#68211=CARTESIAN_POINT('Ctrl Pts',(2.33384334963957,-73.8600122421468,12.));
#68212=CARTESIAN_POINT('Ctrl Pts',(2.3455535680212,-73.8845093109274,0.));
#68213=CARTESIAN_POINT('Ctrl Pts',(2.3455535680212,-73.8845093109274,12.));
#68214=CARTESIAN_POINT('Ctrl Pts',(2.35730163516315,-73.9090280474712,0.));
#68215=CARTESIAN_POINT('Ctrl Pts',(2.35730163516315,-73.9090280474712,12.));
#68216=CARTESIAN_POINT('Ctrl Pts',(2.36908755526003,-73.9335683516404,0.));
#68217=CARTESIAN_POINT('Ctrl Pts',(2.36908755526003,-73.9335683516404,12.));
#68218=CARTESIAN_POINT('Ctrl Pts',(2.3809113327496,-73.958130121465,0.));
#68219=CARTESIAN_POINT('Ctrl Pts',(2.3809113327496,-73.958130121465,12.));
#68220=CARTESIAN_POINT('Ctrl Pts',(2.39277297220756,-73.9827132538206,0.));
#68221=CARTESIAN_POINT('Ctrl Pts',(2.39277297220756,-73.9827132538206,12.));
#68222=CARTESIAN_POINT('Ctrl Pts',(2.40467247811536,-74.0073176459344,0.));
#68223=CARTESIAN_POINT('Ctrl Pts',(2.40467247811536,-74.0073176459344,12.));
#68224=CARTESIAN_POINT('Ctrl Pts',(2.41660985465251,-74.0319431966989,0.));
#68225=CARTESIAN_POINT('Ctrl Pts',(2.41660985465251,-74.0319431966989,12.));
#68226=CARTESIAN_POINT('Ctrl Pts',(2.42858510549778,-74.0565898079218,0.));
#68227=CARTESIAN_POINT('Ctrl Pts',(2.42858510549778,-74.0565898079218,12.));
#68228=CARTESIAN_POINT('Ctrl Pts',(2.44059823356675,-74.0812573859411,0.));
#68229=CARTESIAN_POINT('Ctrl Pts',(2.44059823356675,-74.0812573859411,12.));
#68230=CARTESIAN_POINT('Ctrl Pts',(2.45264924094774,-74.1059458420067,0.));
#68231=CARTESIAN_POINT('Ctrl Pts',(2.45264924094774,-74.1059458420067,12.));
#68232=CARTESIAN_POINT('Ctrl Pts',(2.46473812947959,-74.1306550887071,0.));
#68233=CARTESIAN_POINT('Ctrl Pts',(2.46473812947959,-74.1306550887071,12.));
#68234=CARTESIAN_POINT('Ctrl Pts',(2.47686490120353,-74.155385037148,0.));
#68235=CARTESIAN_POINT('Ctrl Pts',(2.47686490120353,-74.155385037148,12.));
#68236=CARTESIAN_POINT('Ctrl Pts',(2.48902955888384,-74.1801355936907,0.));
#68237=CARTESIAN_POINT('Ctrl Pts',(2.48902955888384,-74.1801355936907,12.));
#68238=CARTESIAN_POINT('Ctrl Pts',(2.50123210644134,-74.2049066572031,0.));
#68239=CARTESIAN_POINT('Ctrl Pts',(2.50123210644134,-74.2049066572031,12.));
#68240=CARTESIAN_POINT('Ctrl Pts',(2.51347254956166,-74.229698115223,0.));
#68241=CARTESIAN_POINT('Ctrl Pts',(2.51347254956166,-74.229698115223,12.));
#68242=CARTESIAN_POINT('Ctrl Pts',(2.52575089478303,-74.2545098494824,0.));
#68243=CARTESIAN_POINT('Ctrl Pts',(2.52575089478303,-74.2545098494824,12.));
#68244=CARTESIAN_POINT('Ctrl Pts',(2.53806714838285,-74.2793417427308,0.));
#68245=CARTESIAN_POINT('Ctrl Pts',(2.53806714838285,-74.2793417427308,12.));
#68246=CARTESIAN_POINT('Ctrl Pts',(2.5504213152678,-74.3041936853468,0.));
#68247=CARTESIAN_POINT('Ctrl Pts',(2.5504213152678,-74.3041936853468,12.));
#68248=CARTESIAN_POINT('Ctrl Pts',(2.56281339800017,-74.3290655814831,0.));
#68249=CARTESIAN_POINT('Ctrl Pts',(2.56281339800017,-74.3290655814831,12.));
#68250=CARTESIAN_POINT('Ctrl Pts',(2.57524339541389,-74.3539573567672,0.));
#68251=CARTESIAN_POINT('Ctrl Pts',(2.57524339541389,-74.3539573567672,12.));
#68252=CARTESIAN_POINT('Ctrl Pts',(2.58771130268175,-74.3788689603363,0.));
#68253=CARTESIAN_POINT('Ctrl Pts',(2.58771130268175,-74.3788689603363,12.));
#68254=CARTESIAN_POINT('Ctrl Pts',(2.60021711326976,-74.4038003594771,0.));
#68255=CARTESIAN_POINT('Ctrl Pts',(2.60021711326976,-74.4038003594771,12.));
#68256=CARTESIAN_POINT('Ctrl Pts',(2.61025207898402,-74.4237613007988,0.));
#68257=CARTESIAN_POINT('Ctrl Pts',(2.61025207898402,-74.4237613007988,12.));
#68258=CARTESIAN_POINT('Ctrl Pts',(2.61779535432111,-74.4387409032207,0.));
#68259=CARTESIAN_POINT('Ctrl Pts',(2.61779535432111,-74.4387409032207,12.));
#68260=CARTESIAN_POINT('Ctrl Pts',(2.62283178248202,-74.4487312586464,0.));
#68261=CARTESIAN_POINT('Ctrl Pts',(2.62283178248202,-74.4487312586464,12.));
#68262=CARTESIAN_POINT('Ctrl Pts',(2.62535189104655,-74.4537274248118,0.));
#68263=CARTESIAN_POINT('Ctrl Pts',(2.62535189104655,-74.4537274248118,12.));
#68264=CARTESIAN_POINT('',(0.853825826608976,-69.9947925310006,0.));
#68265=CARTESIAN_POINT('Ctrl Pts',(0.853825826608976,-69.9947925310006,
0.));
#68266=CARTESIAN_POINT('Ctrl Pts',(0.854867673848587,-69.9985337959407,
0.));
#68267=CARTESIAN_POINT('Ctrl Pts',(0.856954870259198,-70.0060209754087,
0.));
#68268=CARTESIAN_POINT('Ctrl Pts',(0.860096170668728,-70.0172656933806,
0.));
#68269=CARTESIAN_POINT('Ctrl Pts',(0.864305583661538,-70.0322865492925,
0.));
#68270=CARTESIAN_POINT('Ctrl Pts',(0.869602377871117,-70.051109108301,0.));
#68271=CARTESIAN_POINT('Ctrl Pts',(0.874934213255831,-70.0699781183935,
0.));
#68272=CARTESIAN_POINT('Ctrl Pts',(0.880301109660721,-70.0888934967855,
0.));
#68273=CARTESIAN_POINT('Ctrl Pts',(0.885703094802528,-70.1078550938958,
0.));
#68274=CARTESIAN_POINT('Ctrl Pts',(0.891140203464235,-70.1268626950175,
0.));
#68275=CARTESIAN_POINT('Ctrl Pts',(0.896612474371837,-70.1459160490446,
0.));
#68276=CARTESIAN_POINT('Ctrl Pts',(0.902119947629764,-70.1650148905109,
0.));
#68277=CARTESIAN_POINT('Ctrl Pts',(0.907662662015778,-70.1841589635574,
0.));
#68278=CARTESIAN_POINT('Ctrl Pts',(0.913240652090973,-70.2033480471676,
0.));
#68279=CARTESIAN_POINT('Ctrl Pts',(0.918853949157111,-70.2225819470248,
0.));
#68280=CARTESIAN_POINT('Ctrl Pts',(0.924502582639448,-70.2418604835837,
0.));
#68281=CARTESIAN_POINT('Ctrl Pts',(0.93018658123554,-70.2611834821724,0.));
#68282=CARTESIAN_POINT('Ctrl Pts',(0.935905974336473,-70.2805507606872,
0.));
#68283=CARTESIAN_POINT('Ctrl Pts',(0.941660792742972,-70.299962123399,0.));
#68284=CARTESIAN_POINT('Ctrl Pts',(0.947451067929597,-70.3194173673674,
0.));
#68285=CARTESIAN_POINT('Ctrl Pts',(0.953276831581235,-70.338916286458,0.));
#68286=CARTESIAN_POINT('Ctrl Pts',(0.959138115058824,-70.3584586759536,
0.));
#68287=CARTESIAN_POINT('Ctrl Pts',(0.965034948786442,-70.3780443377956,
0.));
#68288=CARTESIAN_POINT('Ctrl Pts',(0.970967362281167,-70.3976730803614,
0.));
#68289=CARTESIAN_POINT('Ctrl Pts',(0.976935384450034,-70.417344715957,0.));
#68290=CARTESIAN_POINT('Ctrl Pts',(0.982939043792148,-70.4370590590842,
0.));
#68291=CARTESIAN_POINT('Ctrl Pts',(0.988978368643642,-70.4568159243163,
0.));
#68292=CARTESIAN_POINT('Ctrl Pts',(0.995053387379748,-70.4766151245212,
0.));
#68293=CARTESIAN_POINT('Ctrl Pts',(1.00116412831442,-70.4964564717953,0.));
#68294=CARTESIAN_POINT('Ctrl Pts',(1.00731061960967,-70.5163397782713,0.));
#68295=CARTESIAN_POINT('Ctrl Pts',(1.01349288918536,-70.5362648569061,0.));
#68296=CARTESIAN_POINT('Ctrl Pts',(1.01971096460596,-70.556231522419,0.));
#68297=CARTESIAN_POINT('Ctrl Pts',(1.02596487304048,-70.5762395916377,0.));
#68298=CARTESIAN_POINT('Ctrl Pts',(1.0322546413287,-70.5962888829934,0.));
#68299=CARTESIAN_POINT('Ctrl Pts',(1.03858029601903,-70.6163792162073,0.));
#68300=CARTESIAN_POINT('Ctrl Pts',(1.04494186341155,-70.6365104119252,0.));
#68301=CARTESIAN_POINT('Ctrl Pts',(1.05133936960071,-70.6566822912991,0.));
#68302=CARTESIAN_POINT('Ctrl Pts',(1.05777284047729,-70.676894676009,0.));
#68303=CARTESIAN_POINT('Ctrl Pts',(1.0642423017128,-70.6971473884459,0.));
#68304=CARTESIAN_POINT('Ctrl Pts',(1.07074777874595,-70.7174402518378,0.));
#68305=CARTESIAN_POINT('Ctrl Pts',(1.07728929676408,-70.7377730903953,0.));
#68306=CARTESIAN_POINT('Ctrl Pts',(1.08386688068342,-70.7581457294447,0.));
#68307=CARTESIAN_POINT('Ctrl Pts',(1.09048055516426,-70.7785579953583,0.));
#68308=CARTESIAN_POINT('Ctrl Pts',(1.09713034462265,-70.799009715484,0.));
#68309=CARTESIAN_POINT('Ctrl Pts',(1.10381627323946,-70.8195007180745,0.));
#68310=CARTESIAN_POINT('Ctrl Pts',(1.11053836496639,-70.8400308322037,0.));
#68311=CARTESIAN_POINT('Ctrl Pts',(1.11729664352992,-70.8605998877149,0.));
#68312=CARTESIAN_POINT('Ctrl Pts',(1.12409113243513,-70.8812077152586,0.));
#68313=CARTESIAN_POINT('Ctrl Pts',(1.13092185496564,-70.9018541463089,0.));
#68314=CARTESIAN_POINT('Ctrl Pts',(1.13778883418213,-70.9225390131826,0.));
#68315=CARTESIAN_POINT('Ctrl Pts',(1.14469209291488,-70.9432621490566,0.));
#68316=CARTESIAN_POINT('Ctrl Pts',(1.15163165376523,-70.9640233879659,0.));
#68317=CARTESIAN_POINT('Ctrl Pts',(1.15860753911484,-70.9848225647871,0.));
#68318=CARTESIAN_POINT('Ctrl Pts',(1.1656197711288,-71.0056595152204,0.));
#68319=CARTESIAN_POINT('Ctrl Pts',(1.17266837175776,-71.0265340757699,0.));
#68320=CARTESIAN_POINT('Ctrl Pts',(1.17975336273503,-71.0474460837159,0.));
#68321=CARTESIAN_POINT('Ctrl Pts',(1.18687476558132,-71.0683953771149,0.));
#68322=CARTESIAN_POINT('Ctrl Pts',(1.19403260161001,-71.089381794801,0.));
#68323=CARTESIAN_POINT('Ctrl Pts',(1.20122689192835,-71.1104051763839,0.));
#68324=CARTESIAN_POINT('Ctrl Pts',(1.20845765743647,-71.1314653622442,0.));
#68325=CARTESIAN_POINT('Ctrl Pts',(1.21572491882262,-71.1525621935267,0.));
#68326=CARTESIAN_POINT('Ctrl Pts',(1.22302869657017,-71.1736955121362,0.));
#68327=CARTESIAN_POINT('Ctrl Pts',(1.23036901096238,-71.194865160732,0.));
#68328=CARTESIAN_POINT('Ctrl Pts',(1.23774588208426,-71.2160709827191,0.));
#68329=CARTESIAN_POINT('Ctrl Pts',(1.24515932982112,-71.2373128222352,0.));
#68330=CARTESIAN_POINT('Ctrl Pts',(1.25260937385568,-71.2585905241406,0.));
#68331=CARTESIAN_POINT('Ctrl Pts',(1.2600960336757,-71.2799039340175,0.));
#68332=CARTESIAN_POINT('Ctrl Pts',(1.26761932857724,-71.3012528981661,0.));
#68333=CARTESIAN_POINT('Ctrl Pts',(1.27517927766607,-71.3226372635996,0.));
#68334=CARTESIAN_POINT('Ctrl Pts',(1.28277589985471,-71.3440568780347,0.));
#68335=CARTESIAN_POINT('Ctrl Pts',(1.29040921386058,-71.3655115898827,0.));
#68336=CARTESIAN_POINT('Ctrl Pts',(1.29807923821413,-71.3870012482499,0.));
#68337=CARTESIAN_POINT('Ctrl Pts',(1.30578599126139,-71.4085257029322,0.));
#68338=CARTESIAN_POINT('Ctrl Pts',(1.31352949116536,-71.4300848044087,0.));
#68339=CARTESIAN_POINT('Ctrl Pts',(1.32130975590225,-71.4516784038317,0.));
#68340=CARTESIAN_POINT('Ctrl Pts',(1.32912680326123,-71.4733063530187,0.));
#68341=CARTESIAN_POINT('Ctrl Pts',(1.33698065085219,-71.4949685044522,0.));
#68342=CARTESIAN_POINT('Ctrl Pts',(1.3448713161078,-71.516664711275,0.));
#68343=CARTESIAN_POINT('Ctrl Pts',(1.35279881628454,-71.5383948272845,0.));
#68344=CARTESIAN_POINT('Ctrl Pts',(1.36076316845815,-71.5601587069217,0.));
#68345=CARTESIAN_POINT('Ctrl Pts',(1.36876438952465,-71.5819562052663,0.));
#68346=CARTESIAN_POINT('Ctrl Pts',(1.37680249620779,-71.6037871780385,0.));
#68347=CARTESIAN_POINT('Ctrl Pts',(1.38487750506081,-71.625651481593,0.));
#68348=CARTESIAN_POINT('Ctrl Pts',(1.39298943246721,-71.6475489729134,0.));
#68349=CARTESIAN_POINT('Ctrl Pts',(1.40113829463576,-71.6694795096001,0.));
#68350=CARTESIAN_POINT('Ctrl Pts',(1.40932410760247,-71.6914429498663,0.));
#68351=CARTESIAN_POINT('Ctrl Pts',(1.41754688723772,-71.7134391525389,0.));
#68352=CARTESIAN_POINT('Ctrl Pts',(1.42580664924769,-71.7354679770528,0.));
#68353=CARTESIAN_POINT('Ctrl Pts',(1.43410340917495,-71.7575292834469,0.));
#68354=CARTESIAN_POINT('Ctrl Pts',(1.44243718239314,-71.7796229323526,0.));
#68355=CARTESIAN_POINT('Ctrl Pts',(1.45080798410964,-71.8017487849895,0.));
#68356=CARTESIAN_POINT('Ctrl Pts',(1.45921582937231,-71.8239067031683,0.));
#68357=CARTESIAN_POINT('Ctrl Pts',(1.46766073307087,-71.8460965492839,0.));
#68358=CARTESIAN_POINT('Ctrl Pts',(1.47614270993728,-71.8683181863116,0.));
#68359=CARTESIAN_POINT('Ctrl Pts',(1.48466177454019,-71.8905714777961,0.));
#68360=CARTESIAN_POINT('Ctrl Pts',(1.49321794128798,-71.912856287848,0.));
#68361=CARTESIAN_POINT('Ctrl Pts',(1.50181122443533,-71.9351724811443,0.));
#68362=CARTESIAN_POINT('Ctrl Pts',(1.51044163808453,-71.9575199229241,0.));
#68363=CARTESIAN_POINT('Ctrl Pts',(1.51910919618565,-71.979898478983,0.));
#68364=CARTESIAN_POINT('Ctrl Pts',(1.52781391253101,-72.0023080156647,0.));
#68365=CARTESIAN_POINT('Ctrl Pts',(1.53655580075812,-72.0247483998579,0.));
#68366=CARTESIAN_POINT('Ctrl Pts',(1.54533487435625,-72.0472194989963,0.));
#68367=CARTESIAN_POINT('Ctrl Pts',(1.55415114666773,-72.0697211810545,0.));
#68368=CARTESIAN_POINT('Ctrl Pts',(1.56300463088808,-72.0922533145433,0.));
#68369=CARTESIAN_POINT('Ctrl Pts',(1.5718953400604,-72.1148157684995,0.));
#68370=CARTESIAN_POINT('Ctrl Pts',(1.58082328707802,-72.1374084124839,0.));
#68371=CARTESIAN_POINT('Ctrl Pts',(1.58978848469122,-72.1600311165821,0.));
#68372=CARTESIAN_POINT('Ctrl Pts',(1.59879094550846,-72.1826837514001,0.));
#68373=CARTESIAN_POINT('Ctrl Pts',(1.60783068199662,-72.2053661880608,0.));
#68374=CARTESIAN_POINT('Ctrl Pts',(1.61690770647539,-72.2280782981937,0.));
#68375=CARTESIAN_POINT('Ctrl Pts',(1.62602203111929,-72.2508199539323,0.));
#68376=CARTESIAN_POINT('Ctrl Pts',(1.63517366796462,-72.2735910279149,0.));
#68377=CARTESIAN_POINT('Ctrl Pts',(1.64436262891078,-72.2963913932813,0.));
#68378=CARTESIAN_POINT('Ctrl Pts',(1.65358892572062,-72.319220923669,0.));
#68379=CARTESIAN_POINT('Ctrl Pts',(1.66285257001496,-72.3420794932047,0.));
#68380=CARTESIAN_POINT('Ctrl Pts',(1.67215357327364,-72.3649669765004,0.));
#68381=CARTESIAN_POINT('Ctrl Pts',(1.68149194684281,-72.387883248654,0.));
#68382=CARTESIAN_POINT('Ctrl Pts',(1.69086770193636,-72.4108281852467,0.));
#68383=CARTESIAN_POINT('Ctrl Pts',(1.70028084963647,-72.4338016623391,0.));
#68384=CARTESIAN_POINT('Ctrl Pts',(1.70973140088841,-72.456803556463,0.));
#68385=CARTESIAN_POINT('Ctrl Pts',(1.71921936650037,-72.479833744618,0.));
#68386=CARTESIAN_POINT('Ctrl Pts',(1.72874475715102,-72.5028921042721,0.));
#68387=CARTESIAN_POINT('Ctrl Pts',(1.73830758339124,-72.5259785133595,0.));
#68388=CARTESIAN_POINT('Ctrl Pts',(1.74790785564473,-72.5490928502769,0.));
#68389=CARTESIAN_POINT('Ctrl Pts',(1.75754558420343,-72.5722349938774,0.));
#68390=CARTESIAN_POINT('Ctrl Pts',(1.76722077922574,-72.5954048234638,0.));
#68391=CARTESIAN_POINT('Ctrl Pts',(1.77693345074426,-72.6186022187907,0.));
#68392=CARTESIAN_POINT('Ctrl Pts',(1.7866836086681,-72.6418270600619,0.));
#68393=CARTESIAN_POINT('Ctrl Pts',(1.79647126278358,-72.6650792279274,0.));
#68394=CARTESIAN_POINT('Ctrl Pts',(1.8062964227505,-72.6883586034769,0.));
#68395=CARTESIAN_POINT('Ctrl Pts',(1.8161590980987,-72.7116650682344,0.));
#68396=CARTESIAN_POINT('Ctrl Pts',(1.82605929823564,-72.7349985041592,0.));
#68397=CARTESIAN_POINT('Ctrl Pts',(1.83599703244924,-72.7583587936447,0.));
#68398=CARTESIAN_POINT('Ctrl Pts',(1.84597230990856,-72.7817458195155,0.));
#68399=CARTESIAN_POINT('Ctrl Pts',(1.85598513966113,-72.8051594650222,0.));
#68400=CARTESIAN_POINT('Ctrl Pts',(1.8660355306277,-72.8285996138359,0.));
#68401=CARTESIAN_POINT('Ctrl Pts',(1.87612349160944,-72.8520661500477,0.));
#68402=CARTESIAN_POINT('Ctrl Pts',(1.88624903129187,-72.875558958168,0.));
#68403=CARTESIAN_POINT('Ctrl Pts',(1.89641215824581,-72.8990779231226,0.));
#68404=CARTESIAN_POINT('Ctrl Pts',(1.90661288092586,-72.9226229302478,0.));
#68405=CARTESIAN_POINT('Ctrl Pts',(1.91685120766436,-72.9461938652811,0.));
#68406=CARTESIAN_POINT('Ctrl Pts',(1.9271271466766,-72.9697906143636,0.));
#68407=CARTESIAN_POINT('Ctrl Pts',(1.93744070606565,-72.9934130640415,0.));
#68408=CARTESIAN_POINT('Ctrl Pts',(1.94779189382301,-73.0170611012661,0.));
#68409=CARTESIAN_POINT('Ctrl Pts',(1.95818071782766,-73.040734613391,0.));
#68410=CARTESIAN_POINT('Ctrl Pts',(1.96860718583931,-73.0644334881673,0.));
#68411=CARTESIAN_POINT('Ctrl Pts',(1.97907130550157,-73.0881576137407,0.));
#68412=CARTESIAN_POINT('Ctrl Pts',(1.98957308434917,-73.1119068786475,0.));
#68413=CARTESIAN_POINT('Ctrl Pts',(2.00011252980981,-73.1356811718091,0.));
#68414=CARTESIAN_POINT('Ctrl Pts',(2.01068964920466,-73.1594803825252,0.));
#68415=CARTESIAN_POINT('Ctrl Pts',(2.02130444974361,-73.183304400462,0.));
#68416=CARTESIAN_POINT('Ctrl Pts',(2.03195693852454,-73.2071531156504,0.));
#68417=CARTESIAN_POINT('Ctrl Pts',(2.04264712253928,-73.2310264184976,0.));
#68418=CARTESIAN_POINT('Ctrl Pts',(2.05337500867402,-73.2549241997953,0.));
#68419=CARTESIAN_POINT('Ctrl Pts',(2.06414060370834,-73.2788463507246,0.));
#68420=CARTESIAN_POINT('Ctrl Pts',(2.0749439143094,-73.3027927628626,0.));
#68421=CARTESIAN_POINT('Ctrl Pts',(2.08578494702743,-73.3267633281807,0.));
#68422=CARTESIAN_POINT('Ctrl Pts',(2.09666370830715,-73.3507579390239,0.));
#68423=CARTESIAN_POINT('Ctrl Pts',(2.10758020449389,-73.3747764880893,0.));
#68424=CARTESIAN_POINT('Ctrl Pts',(2.11853444183761,-73.3988188684021,0.));
#68425=CARTESIAN_POINT('Ctrl Pts',(2.12952642649367,-73.4228849732925,0.));
#68426=CARTESIAN_POINT('Ctrl Pts',(2.14055616452057,-73.4469746963637,0.));
#68427=CARTESIAN_POINT('Ctrl Pts',(2.15162366187906,-73.4710879315382,0.));
#68428=CARTESIAN_POINT('Ctrl Pts',(2.16272892442919,-73.4952245731054,0.));
#68429=CARTESIAN_POINT('Ctrl Pts',(2.17387195792305,-73.5193845157708,0.));
#68430=CARTESIAN_POINT('Ctrl Pts',(2.18505276799752,-73.5435676546929,0.));
#68431=CARTESIAN_POINT('Ctrl Pts',(2.19627136015677,-73.5677738855452,0.));
#68432=CARTESIAN_POINT('Ctrl Pts',(2.20752773978348,-73.5920031044595,0.));
#68433=CARTESIAN_POINT('Ctrl Pts',(2.21882191216517,-73.6162552079038,0.));
#68434=CARTESIAN_POINT('Ctrl Pts',(2.23015388251287,-73.6405300925712,0.));
#68435=CARTESIAN_POINT('Ctrl Pts',(2.24152365597697,-73.6648276552767,0.));
#68436=CARTESIAN_POINT('Ctrl Pts',(2.25293123766424,-73.6891477928129,0.));
#68437=CARTESIAN_POINT('Ctrl Pts',(2.26437663263666,-73.7134904019389,0.));
#68438=CARTESIAN_POINT('Ctrl Pts',(2.27585984587198,-73.7378553796807,0.));
#68439=CARTESIAN_POINT('Ctrl Pts',(2.28738088222863,-73.762242623566,0.));
#68440=CARTESIAN_POINT('Ctrl Pts',(2.29893974640434,-73.786652031885,0.));
#68441=CARTESIAN_POINT('Ctrl Pts',(2.31053644289416,-73.8110835039327,0.));
#68442=CARTESIAN_POINT('Ctrl Pts',(2.32217097594197,-73.8355369402706,0.));
#68443=CARTESIAN_POINT('Ctrl Pts',(2.33384334963957,-73.8600122421468,0.));
#68444=CARTESIAN_POINT('Ctrl Pts',(2.3455535680212,-73.8845093109274,0.));
#68445=CARTESIAN_POINT('Ctrl Pts',(2.35730163516315,-73.9090280474712,0.));
#68446=CARTESIAN_POINT('Ctrl Pts',(2.36908755526003,-73.9335683516404,0.));
#68447=CARTESIAN_POINT('Ctrl Pts',(2.3809113327496,-73.958130121465,0.));
#68448=CARTESIAN_POINT('Ctrl Pts',(2.39277297220756,-73.9827132538206,0.));
#68449=CARTESIAN_POINT('Ctrl Pts',(2.40467247811536,-74.0073176459344,0.));
#68450=CARTESIAN_POINT('Ctrl Pts',(2.41660985465251,-74.0319431966989,0.));
#68451=CARTESIAN_POINT('Ctrl Pts',(2.42858510549778,-74.0565898079218,0.));
#68452=CARTESIAN_POINT('Ctrl Pts',(2.44059823356675,-74.0812573859411,0.));
#68453=CARTESIAN_POINT('Ctrl Pts',(2.45264924094774,-74.1059458420067,0.));
#68454=CARTESIAN_POINT('Ctrl Pts',(2.46301176097121,-74.127126454519,0.));
#68455=CARTESIAN_POINT('Ctrl Pts',(2.47097695564999,-74.1433763941382,0.));
#68456=CARTESIAN_POINT('Ctrl Pts',(2.47652804724548,-74.1546864735169,0.));
#68457=CARTESIAN_POINT('Ctrl Pts',(2.47965393945489,-74.1610506466209,0.));
#68458=CARTESIAN_POINT('Ctrl Pts',(2.48034921843246,-74.1624659714559,0.));
#68459=CARTESIAN_POINT('',(0.853825826608976,-69.9947925310006,12.));
#68460=CARTESIAN_POINT('',(0.853825826608976,-69.9947925310006,0.));
#68461=CARTESIAN_POINT('Ctrl Pts',(2.48034921843246,-74.1624659714559,12.));
#68462=CARTESIAN_POINT('Ctrl Pts',(2.47965393945489,-74.1610506466209,12.));
#68463=CARTESIAN_POINT('Ctrl Pts',(2.47652804724548,-74.1546864735169,12.));
#68464=CARTESIAN_POINT('Ctrl Pts',(2.47097695565,-74.1433763941382,12.));
#68465=CARTESIAN_POINT('Ctrl Pts',(2.46301176097121,-74.127126454519,12.));
#68466=CARTESIAN_POINT('Ctrl Pts',(2.45264924094774,-74.1059458420067,12.));
#68467=CARTESIAN_POINT('Ctrl Pts',(2.44059823356675,-74.0812573859411,12.));
#68468=CARTESIAN_POINT('Ctrl Pts',(2.42858510549778,-74.0565898079218,12.));
#68469=CARTESIAN_POINT('Ctrl Pts',(2.41660985465251,-74.0319431966989,12.));
#68470=CARTESIAN_POINT('Ctrl Pts',(2.40467247811536,-74.0073176459344,12.));
#68471=CARTESIAN_POINT('Ctrl Pts',(2.39277297220756,-73.9827132538206,12.));
#68472=CARTESIAN_POINT('Ctrl Pts',(2.3809113327496,-73.958130121465,12.));
#68473=CARTESIAN_POINT('Ctrl Pts',(2.36908755526003,-73.9335683516404,12.));
#68474=CARTESIAN_POINT('Ctrl Pts',(2.35730163516315,-73.9090280474712,12.));
#68475=CARTESIAN_POINT('Ctrl Pts',(2.3455535680212,-73.8845093109274,12.));
#68476=CARTESIAN_POINT('Ctrl Pts',(2.33384334963957,-73.8600122421468,12.));
#68477=CARTESIAN_POINT('Ctrl Pts',(2.32217097594197,-73.8355369402706,12.));
#68478=CARTESIAN_POINT('Ctrl Pts',(2.31053644289416,-73.8110835039327,12.));
#68479=CARTESIAN_POINT('Ctrl Pts',(2.29893974640434,-73.786652031885,12.));
#68480=CARTESIAN_POINT('Ctrl Pts',(2.28738088222863,-73.762242623566,12.));
#68481=CARTESIAN_POINT('Ctrl Pts',(2.27585984587198,-73.7378553796807,12.));
#68482=CARTESIAN_POINT('Ctrl Pts',(2.26437663263666,-73.7134904019389,12.));
#68483=CARTESIAN_POINT('Ctrl Pts',(2.25293123766424,-73.6891477928129,12.));
#68484=CARTESIAN_POINT('Ctrl Pts',(2.24152365597697,-73.6648276552767,12.));
#68485=CARTESIAN_POINT('Ctrl Pts',(2.23015388251287,-73.6405300925712,12.));
#68486=CARTESIAN_POINT('Ctrl Pts',(2.21882191216517,-73.6162552079038,12.));
#68487=CARTESIAN_POINT('Ctrl Pts',(2.20752773978348,-73.5920031044595,12.));
#68488=CARTESIAN_POINT('Ctrl Pts',(2.19627136015677,-73.5677738855452,12.));
#68489=CARTESIAN_POINT('Ctrl Pts',(2.18505276799752,-73.5435676546929,12.));
#68490=CARTESIAN_POINT('Ctrl Pts',(2.17387195792305,-73.5193845157708,12.));
#68491=CARTESIAN_POINT('Ctrl Pts',(2.16272892442919,-73.4952245731054,12.));
#68492=CARTESIAN_POINT('Ctrl Pts',(2.15162366187906,-73.4710879315382,12.));
#68493=CARTESIAN_POINT('Ctrl Pts',(2.14055616452057,-73.4469746963637,12.));
#68494=CARTESIAN_POINT('Ctrl Pts',(2.12952642649367,-73.4228849732925,12.));
#68495=CARTESIAN_POINT('Ctrl Pts',(2.11853444183761,-73.3988188684021,12.));
#68496=CARTESIAN_POINT('Ctrl Pts',(2.10758020449389,-73.3747764880893,12.));
#68497=CARTESIAN_POINT('Ctrl Pts',(2.09666370830715,-73.3507579390239,12.));
#68498=CARTESIAN_POINT('Ctrl Pts',(2.08578494702743,-73.3267633281807,12.));
#68499=CARTESIAN_POINT('Ctrl Pts',(2.0749439143094,-73.3027927628626,12.));
#68500=CARTESIAN_POINT('Ctrl Pts',(2.06414060370834,-73.2788463507246,12.));
#68501=CARTESIAN_POINT('Ctrl Pts',(2.05337500867402,-73.2549241997953,12.));
#68502=CARTESIAN_POINT('Ctrl Pts',(2.04264712253928,-73.2310264184976,12.));
#68503=CARTESIAN_POINT('Ctrl Pts',(2.03195693852454,-73.2071531156504,12.));
#68504=CARTESIAN_POINT('Ctrl Pts',(2.02130444974361,-73.183304400462,12.));
#68505=CARTESIAN_POINT('Ctrl Pts',(2.01068964920466,-73.1594803825252,12.));
#68506=CARTESIAN_POINT('Ctrl Pts',(2.00011252980981,-73.1356811718091,12.));
#68507=CARTESIAN_POINT('Ctrl Pts',(1.98957308434917,-73.1119068786475,12.));
#68508=CARTESIAN_POINT('Ctrl Pts',(1.97907130550157,-73.0881576137407,12.));
#68509=CARTESIAN_POINT('Ctrl Pts',(1.96860718583931,-73.0644334881673,12.));
#68510=CARTESIAN_POINT('Ctrl Pts',(1.95818071782766,-73.040734613391,12.));
#68511=CARTESIAN_POINT('Ctrl Pts',(1.94779189382301,-73.0170611012661,12.));
#68512=CARTESIAN_POINT('Ctrl Pts',(1.93744070606565,-72.9934130640415,12.));
#68513=CARTESIAN_POINT('Ctrl Pts',(1.9271271466766,-72.9697906143636,12.));
#68514=CARTESIAN_POINT('Ctrl Pts',(1.91685120766436,-72.9461938652811,12.));
#68515=CARTESIAN_POINT('Ctrl Pts',(1.90661288092586,-72.9226229302478,12.));
#68516=CARTESIAN_POINT('Ctrl Pts',(1.89641215824581,-72.8990779231226,12.));
#68517=CARTESIAN_POINT('Ctrl Pts',(1.88624903129187,-72.875558958168,12.));
#68518=CARTESIAN_POINT('Ctrl Pts',(1.87612349160944,-72.8520661500477,12.));
#68519=CARTESIAN_POINT('Ctrl Pts',(1.8660355306277,-72.8285996138359,12.));
#68520=CARTESIAN_POINT('Ctrl Pts',(1.85598513966113,-72.8051594650222,12.));
#68521=CARTESIAN_POINT('Ctrl Pts',(1.84597230990856,-72.7817458195155,12.));
#68522=CARTESIAN_POINT('Ctrl Pts',(1.83599703244924,-72.7583587936447,12.));
#68523=CARTESIAN_POINT('Ctrl Pts',(1.82605929823564,-72.7349985041592,12.));
#68524=CARTESIAN_POINT('Ctrl Pts',(1.8161590980987,-72.7116650682344,12.));
#68525=CARTESIAN_POINT('Ctrl Pts',(1.8062964227505,-72.6883586034769,12.));
#68526=CARTESIAN_POINT('Ctrl Pts',(1.79647126278358,-72.6650792279274,12.));
#68527=CARTESIAN_POINT('Ctrl Pts',(1.7866836086681,-72.6418270600619,12.));
#68528=CARTESIAN_POINT('Ctrl Pts',(1.77693345074426,-72.6186022187907,12.));
#68529=CARTESIAN_POINT('Ctrl Pts',(1.76722077922574,-72.5954048234638,12.));
#68530=CARTESIAN_POINT('Ctrl Pts',(1.75754558420343,-72.5722349938774,12.));
#68531=CARTESIAN_POINT('Ctrl Pts',(1.74790785564473,-72.5490928502769,12.));
#68532=CARTESIAN_POINT('Ctrl Pts',(1.73830758339124,-72.5259785133595,12.));
#68533=CARTESIAN_POINT('Ctrl Pts',(1.72874475715102,-72.5028921042721,12.));
#68534=CARTESIAN_POINT('Ctrl Pts',(1.71921936650037,-72.479833744618,12.));
#68535=CARTESIAN_POINT('Ctrl Pts',(1.70973140088841,-72.456803556463,12.));
#68536=CARTESIAN_POINT('Ctrl Pts',(1.70028084963647,-72.4338016623391,12.));
#68537=CARTESIAN_POINT('Ctrl Pts',(1.69086770193636,-72.4108281852467,12.));
#68538=CARTESIAN_POINT('Ctrl Pts',(1.68149194684281,-72.387883248654,12.));
#68539=CARTESIAN_POINT('Ctrl Pts',(1.67215357327364,-72.3649669765004,12.));
#68540=CARTESIAN_POINT('Ctrl Pts',(1.66285257001496,-72.3420794932047,12.));
#68541=CARTESIAN_POINT('Ctrl Pts',(1.65358892572062,-72.319220923669,12.));
#68542=CARTESIAN_POINT('Ctrl Pts',(1.64436262891078,-72.2963913932813,12.));
#68543=CARTESIAN_POINT('Ctrl Pts',(1.63517366796462,-72.2735910279149,12.));
#68544=CARTESIAN_POINT('Ctrl Pts',(1.62602203111929,-72.2508199539323,12.));
#68545=CARTESIAN_POINT('Ctrl Pts',(1.61690770647539,-72.2280782981937,12.));
#68546=CARTESIAN_POINT('Ctrl Pts',(1.60783068199662,-72.2053661880608,12.));
#68547=CARTESIAN_POINT('Ctrl Pts',(1.59879094550846,-72.1826837514001,12.));
#68548=CARTESIAN_POINT('Ctrl Pts',(1.58978848469122,-72.1600311165821,12.));
#68549=CARTESIAN_POINT('Ctrl Pts',(1.58082328707802,-72.1374084124839,12.));
#68550=CARTESIAN_POINT('Ctrl Pts',(1.5718953400604,-72.1148157684995,12.));
#68551=CARTESIAN_POINT('Ctrl Pts',(1.56300463088808,-72.0922533145433,12.));
#68552=CARTESIAN_POINT('Ctrl Pts',(1.55415114666773,-72.0697211810545,12.));
#68553=CARTESIAN_POINT('Ctrl Pts',(1.54533487435625,-72.0472194989963,12.));
#68554=CARTESIAN_POINT('Ctrl Pts',(1.53655580075812,-72.0247483998579,12.));
#68555=CARTESIAN_POINT('Ctrl Pts',(1.52781391253101,-72.0023080156647,12.));
#68556=CARTESIAN_POINT('Ctrl Pts',(1.51910919618565,-71.979898478983,12.));
#68557=CARTESIAN_POINT('Ctrl Pts',(1.51044163808453,-71.9575199229241,12.));
#68558=CARTESIAN_POINT('Ctrl Pts',(1.50181122443533,-71.9351724811443,12.));
#68559=CARTESIAN_POINT('Ctrl Pts',(1.49321794128798,-71.912856287848,12.));
#68560=CARTESIAN_POINT('Ctrl Pts',(1.48466177454019,-71.8905714777961,12.));
#68561=CARTESIAN_POINT('Ctrl Pts',(1.47614270993728,-71.8683181863116,12.));
#68562=CARTESIAN_POINT('Ctrl Pts',(1.46766073307087,-71.8460965492839,12.));
#68563=CARTESIAN_POINT('Ctrl Pts',(1.45921582937231,-71.8239067031683,12.));
#68564=CARTESIAN_POINT('Ctrl Pts',(1.45080798410964,-71.8017487849895,12.));
#68565=CARTESIAN_POINT('Ctrl Pts',(1.44243718239314,-71.7796229323526,12.));
#68566=CARTESIAN_POINT('Ctrl Pts',(1.43410340917495,-71.7575292834469,12.));
#68567=CARTESIAN_POINT('Ctrl Pts',(1.42580664924769,-71.7354679770528,12.));
#68568=CARTESIAN_POINT('Ctrl Pts',(1.41754688723772,-71.7134391525389,12.));
#68569=CARTESIAN_POINT('Ctrl Pts',(1.40932410760247,-71.6914429498663,12.));
#68570=CARTESIAN_POINT('Ctrl Pts',(1.40113829463576,-71.6694795096001,12.));
#68571=CARTESIAN_POINT('Ctrl Pts',(1.39298943246721,-71.6475489729134,12.));
#68572=CARTESIAN_POINT('Ctrl Pts',(1.38487750506081,-71.625651481593,12.));
#68573=CARTESIAN_POINT('Ctrl Pts',(1.37680249620779,-71.6037871780385,12.));
#68574=CARTESIAN_POINT('Ctrl Pts',(1.36876438952465,-71.5819562052663,12.));
#68575=CARTESIAN_POINT('Ctrl Pts',(1.36076316845815,-71.5601587069217,12.));
#68576=CARTESIAN_POINT('Ctrl Pts',(1.35279881628454,-71.5383948272845,12.));
#68577=CARTESIAN_POINT('Ctrl Pts',(1.3448713161078,-71.516664711275,12.));
#68578=CARTESIAN_POINT('Ctrl Pts',(1.33698065085219,-71.4949685044522,12.));
#68579=CARTESIAN_POINT('Ctrl Pts',(1.32912680326123,-71.4733063530187,12.));
#68580=CARTESIAN_POINT('Ctrl Pts',(1.32130975590225,-71.4516784038317,12.));
#68581=CARTESIAN_POINT('Ctrl Pts',(1.31352949116536,-71.4300848044087,12.));
#68582=CARTESIAN_POINT('Ctrl Pts',(1.30578599126139,-71.4085257029322,12.));
#68583=CARTESIAN_POINT('Ctrl Pts',(1.29807923821413,-71.3870012482499,12.));
#68584=CARTESIAN_POINT('Ctrl Pts',(1.29040921386058,-71.3655115898827,12.));
#68585=CARTESIAN_POINT('Ctrl Pts',(1.28277589985471,-71.3440568780347,12.));
#68586=CARTESIAN_POINT('Ctrl Pts',(1.27517927766607,-71.3226372635996,12.));
#68587=CARTESIAN_POINT('Ctrl Pts',(1.26761932857724,-71.3012528981661,12.));
#68588=CARTESIAN_POINT('Ctrl Pts',(1.2600960336757,-71.2799039340175,12.));
#68589=CARTESIAN_POINT('Ctrl Pts',(1.25260937385568,-71.2585905241406,12.));
#68590=CARTESIAN_POINT('Ctrl Pts',(1.24515932982112,-71.2373128222352,12.));
#68591=CARTESIAN_POINT('Ctrl Pts',(1.23774588208426,-71.2160709827191,12.));
#68592=CARTESIAN_POINT('Ctrl Pts',(1.23036901096238,-71.194865160732,12.));
#68593=CARTESIAN_POINT('Ctrl Pts',(1.22302869657017,-71.1736955121362,12.));
#68594=CARTESIAN_POINT('Ctrl Pts',(1.21572491882262,-71.1525621935267,12.));
#68595=CARTESIAN_POINT('Ctrl Pts',(1.20845765743647,-71.1314653622442,12.));
#68596=CARTESIAN_POINT('Ctrl Pts',(1.20122689192835,-71.1104051763839,12.));
#68597=CARTESIAN_POINT('Ctrl Pts',(1.19403260161001,-71.089381794801,12.));
#68598=CARTESIAN_POINT('Ctrl Pts',(1.18687476558132,-71.0683953771149,12.));
#68599=CARTESIAN_POINT('Ctrl Pts',(1.17975336273503,-71.0474460837159,12.));
#68600=CARTESIAN_POINT('Ctrl Pts',(1.17266837175776,-71.0265340757699,12.));
#68601=CARTESIAN_POINT('Ctrl Pts',(1.1656197711288,-71.0056595152204,12.));
#68602=CARTESIAN_POINT('Ctrl Pts',(1.15860753911484,-70.9848225647871,12.));
#68603=CARTESIAN_POINT('Ctrl Pts',(1.15163165376523,-70.9640233879659,12.));
#68604=CARTESIAN_POINT('Ctrl Pts',(1.14469209291488,-70.9432621490566,12.));
#68605=CARTESIAN_POINT('Ctrl Pts',(1.13778883418213,-70.9225390131826,12.));
#68606=CARTESIAN_POINT('Ctrl Pts',(1.13092185496564,-70.9018541463089,12.));
#68607=CARTESIAN_POINT('Ctrl Pts',(1.12409113243513,-70.8812077152586,12.));
#68608=CARTESIAN_POINT('Ctrl Pts',(1.11729664352992,-70.8605998877149,12.));
#68609=CARTESIAN_POINT('Ctrl Pts',(1.11053836496639,-70.8400308322037,12.));
#68610=CARTESIAN_POINT('Ctrl Pts',(1.10381627323946,-70.8195007180745,12.));
#68611=CARTESIAN_POINT('Ctrl Pts',(1.09713034462265,-70.799009715484,12.));
#68612=CARTESIAN_POINT('Ctrl Pts',(1.09048055516426,-70.7785579953583,12.));
#68613=CARTESIAN_POINT('Ctrl Pts',(1.08386688068342,-70.7581457294447,12.));
#68614=CARTESIAN_POINT('Ctrl Pts',(1.07728929676408,-70.7377730903953,12.));
#68615=CARTESIAN_POINT('Ctrl Pts',(1.07074777874595,-70.7174402518378,12.));
#68616=CARTESIAN_POINT('Ctrl Pts',(1.0642423017128,-70.6971473884459,12.));
#68617=CARTESIAN_POINT('Ctrl Pts',(1.05777284047729,-70.676894676009,12.));
#68618=CARTESIAN_POINT('Ctrl Pts',(1.05133936960071,-70.6566822912991,12.));
#68619=CARTESIAN_POINT('Ctrl Pts',(1.04494186341155,-70.6365104119252,12.));
#68620=CARTESIAN_POINT('Ctrl Pts',(1.03858029601903,-70.6163792162073,12.));
#68621=CARTESIAN_POINT('Ctrl Pts',(1.0322546413287,-70.5962888829934,12.));
#68622=CARTESIAN_POINT('Ctrl Pts',(1.02596487304048,-70.5762395916377,12.));
#68623=CARTESIAN_POINT('Ctrl Pts',(1.01971096460596,-70.556231522419,12.));
#68624=CARTESIAN_POINT('Ctrl Pts',(1.01349288918536,-70.5362648569061,12.));
#68625=CARTESIAN_POINT('Ctrl Pts',(1.00731061960967,-70.5163397782713,12.));
#68626=CARTESIAN_POINT('Ctrl Pts',(1.00116412831442,-70.4964564717953,12.));
#68627=CARTESIAN_POINT('Ctrl Pts',(0.995053387379748,-70.4766151245212,
12.));
#68628=CARTESIAN_POINT('Ctrl Pts',(0.988978368643642,-70.4568159243163,
12.));
#68629=CARTESIAN_POINT('Ctrl Pts',(0.982939043792148,-70.4370590590842,
12.));
#68630=CARTESIAN_POINT('Ctrl Pts',(0.976935384450034,-70.417344715957,12.));
#68631=CARTESIAN_POINT('Ctrl Pts',(0.970967362281167,-70.3976730803614,
12.));
#68632=CARTESIAN_POINT('Ctrl Pts',(0.965034948786442,-70.3780443377956,
12.));
#68633=CARTESIAN_POINT('Ctrl Pts',(0.959138115058824,-70.3584586759536,
12.));
#68634=CARTESIAN_POINT('Ctrl Pts',(0.953276831581235,-70.338916286458,12.));
#68635=CARTESIAN_POINT('Ctrl Pts',(0.947451067929597,-70.3194173673674,
12.));
#68636=CARTESIAN_POINT('Ctrl Pts',(0.941660792742972,-70.299962123399,12.));
#68637=CARTESIAN_POINT('Ctrl Pts',(0.935905974336473,-70.2805507606872,
12.));
#68638=CARTESIAN_POINT('Ctrl Pts',(0.93018658123554,-70.2611834821724,12.));
#68639=CARTESIAN_POINT('Ctrl Pts',(0.924502582639448,-70.2418604835837,
12.));
#68640=CARTESIAN_POINT('Ctrl Pts',(0.918853949157111,-70.2225819470248,
12.));
#68641=CARTESIAN_POINT('Ctrl Pts',(0.913240652090973,-70.2033480471676,
12.));
#68642=CARTESIAN_POINT('Ctrl Pts',(0.907662662015778,-70.1841589635574,
12.));
#68643=CARTESIAN_POINT('Ctrl Pts',(0.902119947629764,-70.1650148905109,
12.));
#68644=CARTESIAN_POINT('Ctrl Pts',(0.896612474371837,-70.1459160490446,
12.));
#68645=CARTESIAN_POINT('Ctrl Pts',(0.891140203464235,-70.1268626950175,
12.));
#68646=CARTESIAN_POINT('Ctrl Pts',(0.885703094802528,-70.1078550938958,
12.));
#68647=CARTESIAN_POINT('Ctrl Pts',(0.880301109660721,-70.0888934967855,
12.));
#68648=CARTESIAN_POINT('Ctrl Pts',(0.874934213255831,-70.0699781183935,
12.));
#68649=CARTESIAN_POINT('Ctrl Pts',(0.869602377871117,-70.051109108301,12.));
#68650=CARTESIAN_POINT('Ctrl Pts',(0.864305583661538,-70.0322865492925,
12.));
#68651=CARTESIAN_POINT('Ctrl Pts',(0.860096170668728,-70.0172656933806,
12.));
#68652=CARTESIAN_POINT('Ctrl Pts',(0.856954870259198,-70.0060209754087,
12.));
#68653=CARTESIAN_POINT('Ctrl Pts',(0.854867673848587,-69.9985337959407,
12.));
#68654=CARTESIAN_POINT('Ctrl Pts',(0.853825826608976,-69.9947925310006,
12.));
#68655=CARTESIAN_POINT('Ctrl Pts',(3.99277406490873,-74.0964320766207,-5.55111512312578E-16));
#68656=CARTESIAN_POINT('Ctrl Pts',(3.99277406490873,-74.0964320766207,4.));
#68657=CARTESIAN_POINT('Ctrl Pts',(3.99277406490871,-74.0964320766207,8.));
#68658=CARTESIAN_POINT('Ctrl Pts',(3.99277406490871,-74.0964320766207,12.));
#68659=CARTESIAN_POINT('Ctrl Pts',(3.95310474582233,-74.1989040313892,-5.55111512312578E-16));
#68660=CARTESIAN_POINT('Ctrl Pts',(3.95310474582233,-74.1989040313892,4.));
#68661=CARTESIAN_POINT('Ctrl Pts',(3.95310474582231,-74.1989040313893,8.));
#68662=CARTESIAN_POINT('Ctrl Pts',(3.95310474582231,-74.1989040313893,12.));
#68663=CARTESIAN_POINT('Ctrl Pts',(3.82252142018535,-74.3538917248566,-5.55111512312578E-16));
#68664=CARTESIAN_POINT('Ctrl Pts',(3.82252142018535,-74.3538917248566,4.00000000000001));
#68665=CARTESIAN_POINT('Ctrl Pts',(3.82252142018533,-74.3538917248566,8.));
#68666=CARTESIAN_POINT('Ctrl Pts',(3.82252142018533,-74.3538917248566,12.));
#68667=CARTESIAN_POINT('Ctrl Pts',(3.63264011802873,-74.4114286752098,-5.55111512312578E-16));
#68668=CARTESIAN_POINT('Ctrl Pts',(3.63264011802873,-74.4114286752098,4.));
#68669=CARTESIAN_POINT('Ctrl Pts',(3.63264011802872,-74.4114286752098,8.00000000000001));
#68670=CARTESIAN_POINT('Ctrl Pts',(3.63264011802872,-74.4114286752098,12.));
#68671=CARTESIAN_POINT('Ctrl Pts',(3.55032190142808,-74.4153560388998,-5.55111512312578E-16));
#68672=CARTESIAN_POINT('Ctrl Pts',(3.55032190142808,-74.4153560388998,4.));
#68673=CARTESIAN_POINT('Ctrl Pts',(3.55032190142807,-74.4153560388998,8.));
#68674=CARTESIAN_POINT('Ctrl Pts',(3.55032190142807,-74.4153560388998,12.));
#68675=CARTESIAN_POINT('',(3.99277406490873,-74.0964320766207,-2.77555756156289E-16));
#68676=CARTESIAN_POINT('',(3.55032190142809,-74.4153560388999,0.));
#68677=CARTESIAN_POINT('Ctrl Pts',(3.99277406490873,-74.0964320766207,-1.38777878078145E-16));
#68678=CARTESIAN_POINT('Ctrl Pts',(3.95310474582233,-74.1989040313892,-1.38777878078145E-16));
#68679=CARTESIAN_POINT('Ctrl Pts',(3.8784857026012,-74.2874684276563,-1.38777878078144E-16));
#68680=CARTESIAN_POINT('Ctrl Pts',(3.78450405480223,-74.3442121731105,-1.38777878078144E-16));
#68681=CARTESIAN_POINT('Ctrl Pts',(3.714017818953,-74.3867699822013,-1.38777878078144E-16));
#68682=CARTESIAN_POINT('Ctrl Pts',(3.63264011802873,-74.4114286752098,-1.38777878078145E-16));
#68683=CARTESIAN_POINT('Ctrl Pts',(3.55032190142808,-74.4153560388998,-1.38777878078144E-16));
#68684=CARTESIAN_POINT('',(3.55032190142808,-74.4153560388999,12.));
#68685=CARTESIAN_POINT('Ctrl Pts',(3.55032190142808,-74.4153560388998,-5.55111512312578E-16));
#68686=CARTESIAN_POINT('Ctrl Pts',(3.55032190142808,-74.4153560388998,4.));
#68687=CARTESIAN_POINT('Ctrl Pts',(3.55032190142807,-74.4153560388998,8.));
#68688=CARTESIAN_POINT('Ctrl Pts',(3.55032190142807,-74.4153560388998,12.));
#68689=CARTESIAN_POINT('',(3.99277406490871,-74.0964320766207,12.));
#68690=CARTESIAN_POINT('Ctrl Pts',(3.55032190142807,-74.4153560388998,12.));
#68691=CARTESIAN_POINT('Ctrl Pts',(3.63264011802872,-74.4114286752098,12.));
#68692=CARTESIAN_POINT('Ctrl Pts',(3.71401781895298,-74.3867699822013,12.));
#68693=CARTESIAN_POINT('Ctrl Pts',(3.78450405480221,-74.3442121731106,12.));
#68694=CARTESIAN_POINT('Ctrl Pts',(3.87848570260118,-74.2874684276563,12.));
#68695=CARTESIAN_POINT('Ctrl Pts',(3.95310474582231,-74.1989040313893,12.));
#68696=CARTESIAN_POINT('Ctrl Pts',(3.99277406490871,-74.0964320766207,12.));
#68697=CARTESIAN_POINT('Ctrl Pts',(3.99277406490871,-74.0964320766207,12.));
#68698=CARTESIAN_POINT('Ctrl Pts',(3.99277406490871,-74.0964320766207,8.));
#68699=CARTESIAN_POINT('Ctrl Pts',(3.99277406490873,-74.0964320766207,4.));
#68700=CARTESIAN_POINT('Ctrl Pts',(3.99277406490873,-74.0964320766207,-5.55111512312578E-16));
#68701=CARTESIAN_POINT('Origin',(1.64496194443586E-11,-3.74482667098164E-10,
0.));
#68702=CARTESIAN_POINT('Origin',(1.64496194443586E-11,-3.74482667098164E-10,
12.));
#68703=CARTESIAN_POINT('Origin',(1.64496194443586E-11,-3.74482667098164E-10,
0.));
#68704=CARTESIAN_POINT('Ctrl Pts',(-3.55032190142517,-74.4153560389001,
0.));
#68705=CARTESIAN_POINT('Ctrl Pts',(-3.55032190142517,-74.4153560389001,
4.));
#68706=CARTESIAN_POINT('Ctrl Pts',(-3.55032190142517,-74.4153560389001,
8.));
#68707=CARTESIAN_POINT('Ctrl Pts',(-3.55032190142517,-74.4153560389001,
12.));
#68708=CARTESIAN_POINT('Ctrl Pts',(-3.66007952356784,-74.4101195539797,
0.));
#68709=CARTESIAN_POINT('Ctrl Pts',(-3.66007952356784,-74.4101195539797,
4.));
#68710=CARTESIAN_POINT('Ctrl Pts',(-3.66007952356784,-74.4101195539797,
8.));
#68711=CARTESIAN_POINT('Ctrl Pts',(-3.66007952356784,-74.4101195539797,
12.));
#68712=CARTESIAN_POINT('Ctrl Pts',(-3.84840282419245,-74.3352361483147,
0.));
#68713=CARTESIAN_POINT('Ctrl Pts',(-3.84840282419245,-74.3352361483147,
4.));
#68714=CARTESIAN_POINT('Ctrl Pts',(-3.84840282419245,-74.3352361483147,
7.99999999999999));
#68715=CARTESIAN_POINT('Ctrl Pts',(-3.84840282419245,-74.3352361483147,
12.));
#68716=CARTESIAN_POINT('Ctrl Pts',(-3.96302207561163,-74.1732860426646,
0.));
#68717=CARTESIAN_POINT('Ctrl Pts',(-3.96302207561163,-74.1732860426646,
4.));
#68718=CARTESIAN_POINT('Ctrl Pts',(-3.96302207561163,-74.1732860426646,
8.00000000000001));
#68719=CARTESIAN_POINT('Ctrl Pts',(-3.96302207561163,-74.1732860426646,
12.));
#68720=CARTESIAN_POINT('Ctrl Pts',(-3.99277406492189,-74.0964320765795,
0.));
#68721=CARTESIAN_POINT('Ctrl Pts',(-3.99277406492189,-74.0964320765795,
4.));
#68722=CARTESIAN_POINT('Ctrl Pts',(-3.99277406492189,-74.0964320765795,
8.));
#68723=CARTESIAN_POINT('Ctrl Pts',(-3.99277406492189,-74.0964320765795,
12.));
#68724=CARTESIAN_POINT('',(-3.55032190142517,-74.4153560389001,0.));
#68725=CARTESIAN_POINT('',(-3.99277406492187,-74.0964320765795,0.));
#68726=CARTESIAN_POINT('Ctrl Pts',(-3.55032190142517,-74.4153560389001,
0.));
#68727=CARTESIAN_POINT('Ctrl Pts',(-3.66007952356784,-74.4101195539797,
0.));
#68728=CARTESIAN_POINT('Ctrl Pts',(-3.76769283821047,-74.3673290364569,
0.));
#68729=CARTESIAN_POINT('Ctrl Pts',(-3.85123952454113,-74.2961085760817,
0.));
#68730=CARTESIAN_POINT('Ctrl Pts',(-3.91389953928912,-74.2426932308003,
0.));
#68731=CARTESIAN_POINT('Ctrl Pts',(-3.96302207561163,-74.1732860426646,
0.));
#68732=CARTESIAN_POINT('Ctrl Pts',(-3.99277406492189,-74.0964320765795,
0.));
#68733=CARTESIAN_POINT('',(-3.99277406492187,-74.0964320765795,12.));
#68734=CARTESIAN_POINT('Ctrl Pts',(-3.99277406492189,-74.0964320765795,
0.));
#68735=CARTESIAN_POINT('Ctrl Pts',(-3.99277406492189,-74.0964320765795,
4.));
#68736=CARTESIAN_POINT('Ctrl Pts',(-3.99277406492189,-74.0964320765795,
8.));
#68737=CARTESIAN_POINT('Ctrl Pts',(-3.99277406492189,-74.0964320765795,
12.));
#68738=CARTESIAN_POINT('',(-3.55032190142517,-74.4153560389001,12.));
#68739=CARTESIAN_POINT('Ctrl Pts',(-3.99277406492189,-74.0964320765795,
12.));
#68740=CARTESIAN_POINT('Ctrl Pts',(-3.96302207561163,-74.1732860426646,
12.));
#68741=CARTESIAN_POINT('Ctrl Pts',(-3.91389953928912,-74.2426932308003,
12.));
#68742=CARTESIAN_POINT('Ctrl Pts',(-3.85123952454113,-74.2961085760817,
12.));
#68743=CARTESIAN_POINT('Ctrl Pts',(-3.76769283821047,-74.3673290364569,
12.));
#68744=CARTESIAN_POINT('Ctrl Pts',(-3.66007952356784,-74.4101195539797,
12.));
#68745=CARTESIAN_POINT('Ctrl Pts',(-3.55032190142517,-74.4153560389001,
12.));
#68746=CARTESIAN_POINT('Ctrl Pts',(-3.55032190142517,-74.4153560389001,
12.));
#68747=CARTESIAN_POINT('Ctrl Pts',(-3.55032190142517,-74.4153560389001,
8.));
#68748=CARTESIAN_POINT('Ctrl Pts',(-3.55032190142517,-74.4153560389001,
4.));
#68749=CARTESIAN_POINT('Ctrl Pts',(-3.55032190142517,-74.4153560389001,
0.));
#68750=CARTESIAN_POINT('Ctrl Pts',(-5.24987136994592,-69.8028570375097,
0.));
#68751=CARTESIAN_POINT('Ctrl Pts',(-5.24987136994592,-69.8028570375097,
12.));
#68752=CARTESIAN_POINT('Ctrl Pts',(-5.24915955997427,-69.8066748687772,
0.));
#68753=CARTESIAN_POINT('Ctrl Pts',(-5.24915955997427,-69.8066748687772,
12.));
#68754=CARTESIAN_POINT('Ctrl Pts',(-5.24773285666376,-69.8143154684204,
0.));
#68755=CARTESIAN_POINT('Ctrl Pts',(-5.24773285666376,-69.8143154684204,
12.));
#68756=CARTESIAN_POINT('Ctrl Pts',(-5.2455835515975,-69.8257911792159,0.));
#68757=CARTESIAN_POINT('Ctrl Pts',(-5.2455835515975,-69.8257911792159,12.));
#68758=CARTESIAN_POINT('Ctrl Pts',(-5.24269931054569,-69.841121750752,0.));
#68759=CARTESIAN_POINT('Ctrl Pts',(-5.24269931054569,-69.841121750752,12.));
#68760=CARTESIAN_POINT('Ctrl Pts',(-5.23906316634803,-69.8603343302743,
0.));
#68761=CARTESIAN_POINT('Ctrl Pts',(-5.23906316634803,-69.8603343302743,
12.));
#68762=CARTESIAN_POINT('Ctrl Pts',(-5.2353961627962,-69.8795962381599,0.));
#68763=CARTESIAN_POINT('Ctrl Pts',(-5.2353961627962,-69.8795962381599,12.));
#68764=CARTESIAN_POINT('Ctrl Pts',(-5.23169827290555,-69.8989073936688,
0.));
#68765=CARTESIAN_POINT('Ctrl Pts',(-5.23169827290555,-69.8989073936688,
12.));
#68766=CARTESIAN_POINT('Ctrl Pts',(-5.22796945602794,-69.9182676502048,
0.));
#68767=CARTESIAN_POINT('Ctrl Pts',(-5.22796945602794,-69.9182676502048,
12.));
#68768=CARTESIAN_POINT('Ctrl Pts',(-5.22420965879981,-69.9376767969095,
0.));
#68769=CARTESIAN_POINT('Ctrl Pts',(-5.22420965879981,-69.9376767969095,
12.));
#68770=CARTESIAN_POINT('Ctrl Pts',(-5.22041882075721,-69.9571345870076,
0.));
#68771=CARTESIAN_POINT('Ctrl Pts',(-5.22041882075721,-69.9571345870076,
12.));
#68772=CARTESIAN_POINT('Ctrl Pts',(-5.21659687881139,-69.9766407595385,
0.));
#68773=CARTESIAN_POINT('Ctrl Pts',(-5.21659687881139,-69.9766407595385,
12.));
#68774=CARTESIAN_POINT('Ctrl Pts',(-5.21274377203259,-69.9961950629965,
0.));
#68775=CARTESIAN_POINT('Ctrl Pts',(-5.21274377203259,-69.9961950629965,
12.));
#68776=CARTESIAN_POINT('Ctrl Pts',(-5.20885944672836,-70.0157972802182,
0.));
#68777=CARTESIAN_POINT('Ctrl Pts',(-5.20885944672836,-70.0157972802182,
12.));
#68778=CARTESIAN_POINT('Ctrl Pts',(-5.20494385478025,-70.0354472203546,
0.));
#68779=CARTESIAN_POINT('Ctrl Pts',(-5.20494385478025,-70.0354472203546,
12.));
#68780=CARTESIAN_POINT('Ctrl Pts',(-5.20099695122656,-70.0551447071082,
0.));
#68781=CARTESIAN_POINT('Ctrl Pts',(-5.20099695122656,-70.0551447071082,
12.));
#68782=CARTESIAN_POINT('Ctrl Pts',(-5.19701869225528,-70.0748895689729,
0.));
#68783=CARTESIAN_POINT('Ctrl Pts',(-5.19701869225528,-70.0748895689729,
12.));
#68784=CARTESIAN_POINT('Ctrl Pts',(-5.1930090327158,-70.0946816270997,0.));
#68785=CARTESIAN_POINT('Ctrl Pts',(-5.1930090327158,-70.0946816270997,12.));
#68786=CARTESIAN_POINT('Ctrl Pts',(-5.18896792486565,-70.1145206891885,
0.));
#68787=CARTESIAN_POINT('Ctrl Pts',(-5.18896792486565,-70.1145206891885,
12.));
#68788=CARTESIAN_POINT('Ctrl Pts',(-5.18489531966265,-70.1344065558145,
0.));
#68789=CARTESIAN_POINT('Ctrl Pts',(-5.18489531966265,-70.1344065558145,
12.));
#68790=CARTESIAN_POINT('Ctrl Pts',(-5.18079116757666,-70.1543390243892,
0.));
#68791=CARTESIAN_POINT('Ctrl Pts',(-5.18079116757666,-70.1543390243892,
12.));
#68792=CARTESIAN_POINT('Ctrl Pts',(-5.17665541952383,-70.1743178937077,
0.));
#68793=CARTESIAN_POINT('Ctrl Pts',(-5.17665541952383,-70.1743178937077,
12.));
#68794=CARTESIAN_POINT('Ctrl Pts',(-5.17248802793389,-70.1943429691167,
0.));
#68795=CARTESIAN_POINT('Ctrl Pts',(-5.17248802793389,-70.1943429691167,
12.));
#68796=CARTESIAN_POINT('Ctrl Pts',(-5.16828894670108,-70.2144140622953,
0.));
#68797=CARTESIAN_POINT('Ctrl Pts',(-5.16828894670108,-70.2144140622953,
12.));
#68798=CARTESIAN_POINT('Ctrl Pts',(-5.16405813066976,-70.2345309887833,
0.));
#68799=CARTESIAN_POINT('Ctrl Pts',(-5.16405813066976,-70.2345309887833,
12.));
#68800=CARTESIAN_POINT('Ctrl Pts',(-5.15979553528203,-70.2546935662722,
0.));
#68801=CARTESIAN_POINT('Ctrl Pts',(-5.15979553528203,-70.2546935662722,
12.));
#68802=CARTESIAN_POINT('Ctrl Pts',(-5.15550111614859,-70.2749016125105,
0.));
#68803=CARTESIAN_POINT('Ctrl Pts',(-5.15550111614859,-70.2749016125105,
12.));
#68804=CARTESIAN_POINT('Ctrl Pts',(-5.15117482869254,-70.2951549435512,
0.));
#68805=CARTESIAN_POINT('Ctrl Pts',(-5.15117482869254,-70.2951549435512,
12.));
#68806=CARTESIAN_POINT('Ctrl Pts',(-5.1468166283308,-70.3154533746736,0.));
#68807=CARTESIAN_POINT('Ctrl Pts',(-5.1468166283308,-70.3154533746736,12.));
#68808=CARTESIAN_POINT('Ctrl Pts',(-5.14242647063479,-70.3357967211796,
0.));
#68809=CARTESIAN_POINT('Ctrl Pts',(-5.14242647063479,-70.3357967211796,
12.));
#68810=CARTESIAN_POINT('Ctrl Pts',(-5.13800431148904,-70.3561847991714,
0.));
#68811=CARTESIAN_POINT('Ctrl Pts',(-5.13800431148904,-70.3561847991714,
12.));
#68812=CARTESIAN_POINT('Ctrl Pts',(-5.13355010728567,-70.3766174264757,
0.));
#68813=CARTESIAN_POINT('Ctrl Pts',(-5.13355010728567,-70.3766174264757,
12.));
#68814=CARTESIAN_POINT('Ctrl Pts',(-5.12906381499456,-70.3970944229851,
0.));
#68815=CARTESIAN_POINT('Ctrl Pts',(-5.12906381499456,-70.3970944229851,
12.));
#68816=CARTESIAN_POINT('Ctrl Pts',(-5.12454539205328,-70.417615610161,0.));
#68817=CARTESIAN_POINT('Ctrl Pts',(-5.12454539205328,-70.417615610161,12.));
#68818=CARTESIAN_POINT('Ctrl Pts',(-5.11999479630212,-70.4381808107245,
0.));
#68819=CARTESIAN_POINT('Ctrl Pts',(-5.11999479630212,-70.4381808107245,
12.));
#68820=CARTESIAN_POINT('Ctrl Pts',(-5.11541198590932,-70.458789848296,0.));
#68821=CARTESIAN_POINT('Ctrl Pts',(-5.11541198590932,-70.458789848296,12.));
#68822=CARTESIAN_POINT('Ctrl Pts',(-5.11079691929213,-70.4794425469825,
0.));
#68823=CARTESIAN_POINT('Ctrl Pts',(-5.11079691929213,-70.4794425469825,
12.));
#68824=CARTESIAN_POINT('Ctrl Pts',(-5.10614955511664,-70.500138731399,0.));
#68825=CARTESIAN_POINT('Ctrl Pts',(-5.10614955511664,-70.500138731399,12.));
#68826=CARTESIAN_POINT('Ctrl Pts',(-5.10146985232941,-70.5208782268497,
0.));
#68827=CARTESIAN_POINT('Ctrl Pts',(-5.10146985232941,-70.5208782268497,
12.));
#68828=CARTESIAN_POINT('Ctrl Pts',(-5.09675777018183,-70.5416608594526,
0.));
#68829=CARTESIAN_POINT('Ctrl Pts',(-5.09675777018183,-70.5416608594526,
12.));
#68830=CARTESIAN_POINT('Ctrl Pts',(-5.09201326826134,-70.5624864562824,
0.));
#68831=CARTESIAN_POINT('Ctrl Pts',(-5.09201326826134,-70.5624864562824,
12.));
#68832=CARTESIAN_POINT('Ctrl Pts',(-5.08723630652273,-70.5833548455014,
0.));
#68833=CARTESIAN_POINT('Ctrl Pts',(-5.08723630652273,-70.5833548455014,
12.));
#68834=CARTESIAN_POINT('Ctrl Pts',(-5.08242684526687,-70.6042658562923,
0.));
#68835=CARTESIAN_POINT('Ctrl Pts',(-5.08242684526687,-70.6042658562923,
12.));
#68836=CARTESIAN_POINT('Ctrl Pts',(-5.07758484512302,-70.6252193187878,
0.));
#68837=CARTESIAN_POINT('Ctrl Pts',(-5.07758484512302,-70.6252193187878,
12.));
#68838=CARTESIAN_POINT('Ctrl Pts',(-5.07271026703355,-70.6462150640015,
0.));
#68839=CARTESIAN_POINT('Ctrl Pts',(-5.07271026703355,-70.6462150640015,
12.));
#68840=CARTESIAN_POINT('Ctrl Pts',(-5.06780307224072,-70.6672529237455,
0.));
#68841=CARTESIAN_POINT('Ctrl Pts',(-5.06780307224072,-70.6672529237455,
12.));
#68842=CARTESIAN_POINT('Ctrl Pts',(-5.0628632222782,-70.6883327305784,0.));
#68843=CARTESIAN_POINT('Ctrl Pts',(-5.0628632222782,-70.6883327305784,12.));
#68844=CARTESIAN_POINT('Ctrl Pts',(-5.05789067897057,-70.7094543178438,
0.));
#68845=CARTESIAN_POINT('Ctrl Pts',(-5.05789067897057,-70.7094543178438,
12.));
#68846=CARTESIAN_POINT('Ctrl Pts',(-5.05288540443482,-70.7306175196863,
0.));
#68847=CARTESIAN_POINT('Ctrl Pts',(-5.05288540443482,-70.7306175196863,
12.));
#68848=CARTESIAN_POINT('Ctrl Pts',(-5.04784736108346,-70.7518221710706,
0.));
#68849=CARTESIAN_POINT('Ctrl Pts',(-5.04784736108346,-70.7518221710706,
12.));
#68850=CARTESIAN_POINT('Ctrl Pts',(-5.0427765116335,-70.7730681077983,0.));
#68851=CARTESIAN_POINT('Ctrl Pts',(-5.0427765116335,-70.7730681077983,12.));
#68852=CARTESIAN_POINT('Ctrl Pts',(-5.03767281910479,-70.7943551665059,
0.));
#68853=CARTESIAN_POINT('Ctrl Pts',(-5.03767281910479,-70.7943551665059,
12.));
#68854=CARTESIAN_POINT('Ctrl Pts',(-5.03253624680941,-70.8156831846488,
0.));
#68855=CARTESIAN_POINT('Ctrl Pts',(-5.03253624680941,-70.8156831846488,
12.));
#68856=CARTESIAN_POINT('Ctrl Pts',(-5.02736675834693,-70.8370520004843,
0.));
#68857=CARTESIAN_POINT('Ctrl Pts',(-5.02736675834693,-70.8370520004843,
12.));
#68858=CARTESIAN_POINT('Ctrl Pts',(-5.02216431760061,-70.8584614530519,
0.));
#68859=CARTESIAN_POINT('Ctrl Pts',(-5.02216431760061,-70.8584614530519,
12.));
#68860=CARTESIAN_POINT('Ctrl Pts',(-5.0169288887379,-70.8799113821452,0.));
#68861=CARTESIAN_POINT('Ctrl Pts',(-5.0169288887379,-70.8799113821452,12.));
#68862=CARTESIAN_POINT('Ctrl Pts',(-5.01166043620568,-70.9014016283124,
0.));
#68863=CARTESIAN_POINT('Ctrl Pts',(-5.01166043620568,-70.9014016283124,
12.));
#68864=CARTESIAN_POINT('Ctrl Pts',(-5.00635892472513,-70.9229320328589,
0.));
#68865=CARTESIAN_POINT('Ctrl Pts',(-5.00635892472513,-70.9229320328589,
12.));
#68866=CARTESIAN_POINT('Ctrl Pts',(-5.00102431929039,-70.9445024378439,
0.));
#68867=CARTESIAN_POINT('Ctrl Pts',(-5.00102431929039,-70.9445024378439,
12.));
#68868=CARTESIAN_POINT('Ctrl Pts',(-4.99565658516913,-70.9661126860773,
0.));
#68869=CARTESIAN_POINT('Ctrl Pts',(-4.99565658516913,-70.9661126860773,
12.));
#68870=CARTESIAN_POINT('Ctrl Pts',(-4.99025568790664,-70.9877626211113,
0.));
#68871=CARTESIAN_POINT('Ctrl Pts',(-4.99025568790664,-70.9877626211113,
12.));
#68872=CARTESIAN_POINT('Ctrl Pts',(-4.98482159331863,-71.0094520872377,
0.));
#68873=CARTESIAN_POINT('Ctrl Pts',(-4.98482159331863,-71.0094520872377,
12.));
#68874=CARTESIAN_POINT('Ctrl Pts',(-4.97935426748585,-71.0311809294821,
0.));
#68875=CARTESIAN_POINT('Ctrl Pts',(-4.97935426748585,-71.0311809294821,
12.));
#68876=CARTESIAN_POINT('Ctrl Pts',(-4.97385367675159,-71.0529489935961,
0.));
#68877=CARTESIAN_POINT('Ctrl Pts',(-4.97385367675159,-71.0529489935961,
12.));
#68878=CARTESIAN_POINT('Ctrl Pts',(-4.96831978772191,-71.0747561260436,
0.));
#68879=CARTESIAN_POINT('Ctrl Pts',(-4.96831978772191,-71.0747561260436,
12.));
#68880=CARTESIAN_POINT('Ctrl Pts',(-4.96275256726766,-71.0966021739907,
0.));
#68881=CARTESIAN_POINT('Ctrl Pts',(-4.96275256726766,-71.0966021739907,
12.));
#68882=CARTESIAN_POINT('Ctrl Pts',(-4.95715198251685,-71.1184869853056,
0.));
#68883=CARTESIAN_POINT('Ctrl Pts',(-4.95715198251685,-71.1184869853056,
12.));
#68884=CARTESIAN_POINT('Ctrl Pts',(-4.95151800085101,-71.1404104085552,
0.));
#68885=CARTESIAN_POINT('Ctrl Pts',(-4.95151800085101,-71.1404104085552,
12.));
#68886=CARTESIAN_POINT('Ctrl Pts',(-4.94585058990341,-71.1623722930001,
0.));
#68887=CARTESIAN_POINT('Ctrl Pts',(-4.94585058990341,-71.1623722930001,
12.));
#68888=CARTESIAN_POINT('Ctrl Pts',(-4.94014971756115,-71.1843724885847,
0.));
#68889=CARTESIAN_POINT('Ctrl Pts',(-4.94014971756115,-71.1843724885847,
12.));
#68890=CARTESIAN_POINT('Ctrl Pts',(-4.93441535196617,-71.2064108459286,
0.));
#68891=CARTESIAN_POINT('Ctrl Pts',(-4.93441535196617,-71.2064108459286,
12.));
#68892=CARTESIAN_POINT('Ctrl Pts',(-4.92864746150732,-71.2284872163273,
0.));
#68893=CARTESIAN_POINT('Ctrl Pts',(-4.92864746150732,-71.2284872163273,
12.));
#68894=CARTESIAN_POINT('Ctrl Pts',(-4.92284601481721,-71.250601451747,0.));
#68895=CARTESIAN_POINT('Ctrl Pts',(-4.92284601481721,-71.250601451747,12.));
#68896=CARTESIAN_POINT('Ctrl Pts',(-4.91701098077036,-71.2727534048192,
0.));
#68897=CARTESIAN_POINT('Ctrl Pts',(-4.91701098077036,-71.2727534048192,
12.));
#68898=CARTESIAN_POINT('Ctrl Pts',(-4.91114232848603,-71.294942928829,0.));
#68899=CARTESIAN_POINT('Ctrl Pts',(-4.91114232848603,-71.294942928829,12.));
#68900=CARTESIAN_POINT('Ctrl Pts',(-4.90524002732779,-71.3171698777084,
0.));
#68901=CARTESIAN_POINT('Ctrl Pts',(-4.90524002732779,-71.3171698777084,
12.));
#68902=CARTESIAN_POINT('Ctrl Pts',(-4.89930404689575,-71.3394341060359,
0.));
#68903=CARTESIAN_POINT('Ctrl Pts',(-4.89930404689575,-71.3394341060359,
12.));
#68904=CARTESIAN_POINT('Ctrl Pts',(-4.89333435702414,-71.3617354690325,
0.));
#68905=CARTESIAN_POINT('Ctrl Pts',(-4.89333435702414,-71.3617354690325,
12.));
#68906=CARTESIAN_POINT('Ctrl Pts',(-4.88733092777975,-71.3840738225562,
0.));
#68907=CARTESIAN_POINT('Ctrl Pts',(-4.88733092777975,-71.3840738225562,
12.));
#68908=CARTESIAN_POINT('Ctrl Pts',(-4.88129372946551,-71.4064490230899,
0.));
#68909=CARTESIAN_POINT('Ctrl Pts',(-4.88129372946551,-71.4064490230899,
12.));
#68910=CARTESIAN_POINT('Ctrl Pts',(-4.87522273261908,-71.4288609277374,
0.));
#68911=CARTESIAN_POINT('Ctrl Pts',(-4.87522273261908,-71.4288609277374,
12.));
#68912=CARTESIAN_POINT('Ctrl Pts',(-4.8691179080055,-71.4513093942255,0.));
#68913=CARTESIAN_POINT('Ctrl Pts',(-4.8691179080055,-71.4513093942255,12.));
#68914=CARTESIAN_POINT('Ctrl Pts',(-4.86297922661503,-71.4737942808982,
0.));
#68915=CARTESIAN_POINT('Ctrl Pts',(-4.86297922661503,-71.4737942808982,
12.));
#68916=CARTESIAN_POINT('Ctrl Pts',(-4.8568066596618,-71.4963154467113,0.));
#68917=CARTESIAN_POINT('Ctrl Pts',(-4.8568066596618,-71.4963154467113,12.));
#68918=CARTESIAN_POINT('Ctrl Pts',(-4.8506001785878,-71.5188727512197,0.));
#68919=CARTESIAN_POINT('Ctrl Pts',(-4.8506001785878,-71.5188727512197,12.));
#68920=CARTESIAN_POINT('Ctrl Pts',(-4.84435975506048,-71.5414660545739,
0.));
#68921=CARTESIAN_POINT('Ctrl Pts',(-4.84435975506048,-71.5414660545739,
12.));
#68922=CARTESIAN_POINT('Ctrl Pts',(-4.83808536096583,-71.564095217521,0.));
#68923=CARTESIAN_POINT('Ctrl Pts',(-4.83808536096583,-71.564095217521,12.));
#68924=CARTESIAN_POINT('Ctrl Pts',(-4.83177696840637,-71.5867601014,0.));
#68925=CARTESIAN_POINT('Ctrl Pts',(-4.83177696840637,-71.5867601014,12.));
#68926=CARTESIAN_POINT('Ctrl Pts',(-4.82543454970027,-71.6094605681366,
0.));
#68927=CARTESIAN_POINT('Ctrl Pts',(-4.82543454970027,-71.6094605681366,
12.));
#68928=CARTESIAN_POINT('Ctrl Pts',(-4.81905807738557,-71.6321964802326,
0.));
#68929=CARTESIAN_POINT('Ctrl Pts',(-4.81905807738557,-71.6321964802326,
12.));
#68930=CARTESIAN_POINT('Ctrl Pts',(-4.81264752421732,-71.6549677007613,
0.));
#68931=CARTESIAN_POINT('Ctrl Pts',(-4.81264752421732,-71.6549677007613,
12.));
#68932=CARTESIAN_POINT('Ctrl Pts',(-4.80620286316088,-71.6777740933705,
0.));
#68933=CARTESIAN_POINT('Ctrl Pts',(-4.80620286316088,-71.6777740933705,
12.));
#68934=CARTESIAN_POINT('Ctrl Pts',(-4.79972406739014,-71.7006155222766,
0.));
#68935=CARTESIAN_POINT('Ctrl Pts',(-4.79972406739014,-71.7006155222766,
12.));
#68936=CARTESIAN_POINT('Ctrl Pts',(-4.79321111028672,-71.7234918522604,
0.));
#68937=CARTESIAN_POINT('Ctrl Pts',(-4.79321111028672,-71.7234918522604,
12.));
#68938=CARTESIAN_POINT('Ctrl Pts',(-4.7866639654445,-71.7464029486552,0.));
#68939=CARTESIAN_POINT('Ctrl Pts',(-4.7866639654445,-71.7464029486552,12.));
#68940=CARTESIAN_POINT('Ctrl Pts',(-4.78008260666642,-71.7693486773449,
0.));
#68941=CARTESIAN_POINT('Ctrl Pts',(-4.78008260666642,-71.7693486773449,
12.));
#68942=CARTESIAN_POINT('Ctrl Pts',(-4.77346700795787,-71.7923289047636,
0.));
#68943=CARTESIAN_POINT('Ctrl Pts',(-4.77346700795787,-71.7923289047636,
12.));
#68944=CARTESIAN_POINT('Ctrl Pts',(-4.76681714352503,-71.8153434978924,
0.));
#68945=CARTESIAN_POINT('Ctrl Pts',(-4.76681714352503,-71.8153434978924,
12.));
#68946=CARTESIAN_POINT('Ctrl Pts',(-4.76013298777422,-71.8383923242533,
0.));
#68947=CARTESIAN_POINT('Ctrl Pts',(-4.76013298777422,-71.8383923242533,
12.));
#68948=CARTESIAN_POINT('Ctrl Pts',(-4.75341451531671,-71.8614752519008,
0.));
#68949=CARTESIAN_POINT('Ctrl Pts',(-4.75341451531671,-71.8614752519008,
12.));
#68950=CARTESIAN_POINT('Ctrl Pts',(-4.74666170096545,-71.8845921494186,
0.));
#68951=CARTESIAN_POINT('Ctrl Pts',(-4.74666170096545,-71.8845921494186,
12.));
#68952=CARTESIAN_POINT('Ctrl Pts',(-4.7398745197286,-71.9077428859207,0.));
#68953=CARTESIAN_POINT('Ctrl Pts',(-4.7398745197286,-71.9077428859207,12.));
#68954=CARTESIAN_POINT('Ctrl Pts',(-4.73305294680784,-71.9309273310469,
0.));
#68955=CARTESIAN_POINT('Ctrl Pts',(-4.73305294680784,-71.9309273310469,
12.));
#68956=CARTESIAN_POINT('Ctrl Pts',(-4.72619695759778,-71.9541453549582,
0.));
#68957=CARTESIAN_POINT('Ctrl Pts',(-4.72619695759778,-71.9541453549582,
12.));
#68958=CARTESIAN_POINT('Ctrl Pts',(-4.7193065276908,-71.9773968283267,0.));
#68959=CARTESIAN_POINT('Ctrl Pts',(-4.7193065276908,-71.9773968283267,12.));
#68960=CARTESIAN_POINT('Ctrl Pts',(-4.7123816328741,-72.0006816223335,0.));
#68961=CARTESIAN_POINT('Ctrl Pts',(-4.7123816328741,-72.0006816223335,12.));
#68962=CARTESIAN_POINT('Ctrl Pts',(-4.70542224912312,-72.0239996086694,
0.));
#68963=CARTESIAN_POINT('Ctrl Pts',(-4.70542224912312,-72.0239996086694,
12.));
#68964=CARTESIAN_POINT('Ctrl Pts',(-4.69842835259997,-72.047350659532,0.));
#68965=CARTESIAN_POINT('Ctrl Pts',(-4.69842835259997,-72.047350659532,12.));
#68966=CARTESIAN_POINT('Ctrl Pts',(-4.6913999196528,-72.070734647621,0.));
#68967=CARTESIAN_POINT('Ctrl Pts',(-4.6913999196528,-72.070734647621,12.));
#68968=CARTESIAN_POINT('Ctrl Pts',(-4.6843369268206,-72.0941514461283,0.));
#68969=CARTESIAN_POINT('Ctrl Pts',(-4.6843369268206,-72.0941514461283,12.));
#68970=CARTESIAN_POINT('Ctrl Pts',(-4.67723935083087,-72.1176009287349,
0.));
#68971=CARTESIAN_POINT('Ctrl Pts',(-4.67723935083087,-72.1176009287349,
12.));
#68972=CARTESIAN_POINT('Ctrl Pts',(-4.67010716859281,-72.1410829696129,
0.));
#68973=CARTESIAN_POINT('Ctrl Pts',(-4.67010716859281,-72.1410829696129,
12.));
#68974=CARTESIAN_POINT('Ctrl Pts',(-4.6629403571957,-72.1645974434218,0.));
#68975=CARTESIAN_POINT('Ctrl Pts',(-4.6629403571957,-72.1645974434218,12.));
#68976=CARTESIAN_POINT('Ctrl Pts',(-4.65573889390824,-72.1881442253052,
0.));
#68977=CARTESIAN_POINT('Ctrl Pts',(-4.65573889390824,-72.1881442253052,
12.));
#68978=CARTESIAN_POINT('Ctrl Pts',(-4.64850275618325,-72.2117231908816,
0.));
#68979=CARTESIAN_POINT('Ctrl Pts',(-4.64850275618325,-72.2117231908816,
12.));
#68980=CARTESIAN_POINT('Ctrl Pts',(-4.64123192165627,-72.2353342162408,
0.));
#68981=CARTESIAN_POINT('Ctrl Pts',(-4.64123192165627,-72.2353342162408,
12.));
#68982=CARTESIAN_POINT('Ctrl Pts',(-4.63392636813842,-72.2589771779447,
0.));
#68983=CARTESIAN_POINT('Ctrl Pts',(-4.63392636813842,-72.2589771779447,
12.));
#68984=CARTESIAN_POINT('Ctrl Pts',(-4.62658607361465,-72.2826519530254,
0.));
#68985=CARTESIAN_POINT('Ctrl Pts',(-4.62658607361465,-72.2826519530254,
12.));
#68986=CARTESIAN_POINT('Ctrl Pts',(-4.61921101624294,-72.306358418981,0.));
#68987=CARTESIAN_POINT('Ctrl Pts',(-4.61921101624294,-72.306358418981,12.));
#68988=CARTESIAN_POINT('Ctrl Pts',(-4.61180117435868,-72.330096453767,0.));
#68989=CARTESIAN_POINT('Ctrl Pts',(-4.61180117435868,-72.330096453767,12.));
#68990=CARTESIAN_POINT('Ctrl Pts',(-4.60435652647463,-72.3538659357932,
0.));
#68991=CARTESIAN_POINT('Ctrl Pts',(-4.60435652647463,-72.3538659357932,
12.));
#68992=CARTESIAN_POINT('Ctrl Pts',(-4.5968770512734,-72.3776667439244,0.));
#68993=CARTESIAN_POINT('Ctrl Pts',(-4.5968770512734,-72.3776667439244,12.));
#68994=CARTESIAN_POINT('Ctrl Pts',(-4.58936272760551,-72.4014987574789,
0.));
#68995=CARTESIAN_POINT('Ctrl Pts',(-4.58936272760551,-72.4014987574789,
12.));
#68996=CARTESIAN_POINT('Ctrl Pts',(-4.58181353448851,-72.4253618562249,
0.));
#68997=CARTESIAN_POINT('Ctrl Pts',(-4.58181353448851,-72.4253618562249,
12.));
#68998=CARTESIAN_POINT('Ctrl Pts',(-4.57422945111094,-72.449255920373,0.));
#68999=CARTESIAN_POINT('Ctrl Pts',(-4.57422945111094,-72.449255920373,12.));
#69000=CARTESIAN_POINT('Ctrl Pts',(-4.56661045683366,-72.473180830571,0.));
#69001=CARTESIAN_POINT('Ctrl Pts',(-4.56661045683366,-72.473180830571,12.));
#69002=CARTESIAN_POINT('Ctrl Pts',(-4.55895653118213,-72.4971364679055,
0.));
#69003=CARTESIAN_POINT('Ctrl Pts',(-4.55895653118213,-72.4971364679055,
12.));
#69004=CARTESIAN_POINT('Ctrl Pts',(-4.55126765384403,-72.5211227138997,
0.));
#69005=CARTESIAN_POINT('Ctrl Pts',(-4.55126765384403,-72.5211227138997,
12.));
#69006=CARTESIAN_POINT('Ctrl Pts',(-4.54354380466825,-72.5451394505106,
0.));
#69007=CARTESIAN_POINT('Ctrl Pts',(-4.54354380466825,-72.5451394505106,
12.));
#69008=CARTESIAN_POINT('Ctrl Pts',(-4.53578496366802,-72.5691865601225,
0.));
#69009=CARTESIAN_POINT('Ctrl Pts',(-4.53578496366802,-72.5691865601225,
12.));
#69010=CARTESIAN_POINT('Ctrl Pts',(-4.5279911110239,-72.5932639255406,0.));
#69011=CARTESIAN_POINT('Ctrl Pts',(-4.5279911110239,-72.5932639255406,12.));
#69012=CARTESIAN_POINT('Ctrl Pts',(-4.52016222707632,-72.6173714299935,
0.));
#69013=CARTESIAN_POINT('Ctrl Pts',(-4.52016222707632,-72.6173714299935,
12.));
#69014=CARTESIAN_POINT('Ctrl Pts',(-4.5122982923226,-72.6415089571314,0.));
#69015=CARTESIAN_POINT('Ctrl Pts',(-4.5122982923226,-72.6415089571314,12.));
#69016=CARTESIAN_POINT('Ctrl Pts',(-4.50439928741605,-72.6656763910241,
0.));
#69017=CARTESIAN_POINT('Ctrl Pts',(-4.50439928741605,-72.6656763910241,
12.));
#69018=CARTESIAN_POINT('Ctrl Pts',(-4.49646519316822,-72.689873616155,0.));
#69019=CARTESIAN_POINT('Ctrl Pts',(-4.49646519316822,-72.689873616155,12.));
#69020=CARTESIAN_POINT('Ctrl Pts',(-4.48849599055354,-72.7141005174153,
0.));
#69021=CARTESIAN_POINT('Ctrl Pts',(-4.48849599055354,-72.7141005174153,
12.));
#69022=CARTESIAN_POINT('Ctrl Pts',(-4.48049166070223,-72.7383569801042,
0.));
#69023=CARTESIAN_POINT('Ctrl Pts',(-4.48049166070223,-72.7383569801042,
12.));
#69024=CARTESIAN_POINT('Ctrl Pts',(-4.47245218489623,-72.7626428899287,
0.));
#69025=CARTESIAN_POINT('Ctrl Pts',(-4.47245218489623,-72.7626428899287,
12.));
#69026=CARTESIAN_POINT('Ctrl Pts',(-4.46437754456795,-72.7869581329994,
0.));
#69027=CARTESIAN_POINT('Ctrl Pts',(-4.46437754456795,-72.7869581329994,
12.));
#69028=CARTESIAN_POINT('Ctrl Pts',(-4.45626772130138,-72.8113025958258,
0.));
#69029=CARTESIAN_POINT('Ctrl Pts',(-4.45626772130138,-72.8113025958258,
12.));
#69030=CARTESIAN_POINT('Ctrl Pts',(-4.44812269683724,-72.8356761653064,
0.));
#69031=CARTESIAN_POINT('Ctrl Pts',(-4.44812269683724,-72.8356761653064,
12.));
#69032=CARTESIAN_POINT('Ctrl Pts',(-4.43994245306805,-72.8600787287316,
0.));
#69033=CARTESIAN_POINT('Ctrl Pts',(-4.43994245306805,-72.8600787287316,
12.));
#69034=CARTESIAN_POINT('Ctrl Pts',(-4.43172697203341,-72.8845101737856,
0.));
#69035=CARTESIAN_POINT('Ctrl Pts',(-4.43172697203341,-72.8845101737856,
12.));
#69036=CARTESIAN_POINT('Ctrl Pts',(-4.42347623591941,-72.9089703885463,
0.));
#69037=CARTESIAN_POINT('Ctrl Pts',(-4.42347623591941,-72.9089703885463,
12.));
#69038=CARTESIAN_POINT('Ctrl Pts',(-4.41519022705926,-72.9334592614828,
0.));
#69039=CARTESIAN_POINT('Ctrl Pts',(-4.41519022705926,-72.9334592614828,
12.));
#69040=CARTESIAN_POINT('Ctrl Pts',(-4.40686892793965,-72.9579766814495,
0.));
#69041=CARTESIAN_POINT('Ctrl Pts',(-4.40686892793965,-72.9579766814495,
12.));
#69042=CARTESIAN_POINT('Ctrl Pts',(-4.3985123211973,-72.9825225376839,0.));
#69043=CARTESIAN_POINT('Ctrl Pts',(-4.3985123211973,-72.9825225376839,12.));
#69044=CARTESIAN_POINT('Ctrl Pts',(-4.39012038961145,-73.0070967198033,
0.));
#69045=CARTESIAN_POINT('Ctrl Pts',(-4.39012038961145,-73.0070967198033,
12.));
#69046=CARTESIAN_POINT('Ctrl Pts',(-4.38169311610153,-73.031699117799,0.));
#69047=CARTESIAN_POINT('Ctrl Pts',(-4.38169311610153,-73.031699117799,12.));
#69048=CARTESIAN_POINT('Ctrl Pts',(-4.37323048372607,-73.0563296220301,
0.));
#69049=CARTESIAN_POINT('Ctrl Pts',(-4.37323048372607,-73.0563296220301,
12.));
#69050=CARTESIAN_POINT('Ctrl Pts',(-4.36473247568638,-73.0809881232111,
0.));
#69051=CARTESIAN_POINT('Ctrl Pts',(-4.36473247568638,-73.0809881232111,
12.));
#69052=CARTESIAN_POINT('Ctrl Pts',(-4.35619907532716,-73.1056745124099,
0.));
#69053=CARTESIAN_POINT('Ctrl Pts',(-4.35619907532716,-73.1056745124099,
12.));
#69054=CARTESIAN_POINT('Ctrl Pts',(-4.34763026613154,-73.1303886810602,
0.));
#69055=CARTESIAN_POINT('Ctrl Pts',(-4.34763026613154,-73.1303886810602,
12.));
#69056=CARTESIAN_POINT('Ctrl Pts',(-4.33902603172139,-73.1551305209692,
0.));
#69057=CARTESIAN_POINT('Ctrl Pts',(-4.33902603172139,-73.1551305209692,
12.));
#69058=CARTESIAN_POINT('Ctrl Pts',(-4.33038635585878,-73.1798999243234,
0.));
#69059=CARTESIAN_POINT('Ctrl Pts',(-4.33038635585878,-73.1798999243234,
12.));
#69060=CARTESIAN_POINT('Ctrl Pts',(-4.32171122245218,-73.204696783693,0.));
#69061=CARTESIAN_POINT('Ctrl Pts',(-4.32171122245218,-73.204696783693,12.));
#69062=CARTESIAN_POINT('Ctrl Pts',(-4.31300061556103,-73.2295209920319,
0.));
#69063=CARTESIAN_POINT('Ctrl Pts',(-4.31300061556103,-73.2295209920319,
12.));
#69064=CARTESIAN_POINT('Ctrl Pts',(-4.30425451938234,-73.2543724426562,
0.));
#69065=CARTESIAN_POINT('Ctrl Pts',(-4.30425451938234,-73.2543724426562,
12.));
#69066=CARTESIAN_POINT('Ctrl Pts',(-4.29547291824289,-73.2792510292243,
0.));
#69067=CARTESIAN_POINT('Ctrl Pts',(-4.29547291824289,-73.2792510292243,
12.));
#69068=CARTESIAN_POINT('Ctrl Pts',(-4.28665579659302,-73.3041566457134,
0.));
#69069=CARTESIAN_POINT('Ctrl Pts',(-4.28665579659302,-73.3041566457134,
12.));
#69070=CARTESIAN_POINT('Ctrl Pts',(-4.27780313900392,-73.3290891863959,
0.));
#69071=CARTESIAN_POINT('Ctrl Pts',(-4.27780313900392,-73.3290891863959,
12.));
#69072=CARTESIAN_POINT('Ctrl Pts',(-4.26891493016703,-73.354048545808,0.));
#69073=CARTESIAN_POINT('Ctrl Pts',(-4.26891493016703,-73.354048545808,12.));
#69074=CARTESIAN_POINT('Ctrl Pts',(-4.25999115489904,-73.3790346187953,
0.));
#69075=CARTESIAN_POINT('Ctrl Pts',(-4.25999115489904,-73.3790346187953,
12.));
#69076=CARTESIAN_POINT('Ctrl Pts',(-4.25103179814892,-73.4040473005603,
0.));
#69077=CARTESIAN_POINT('Ctrl Pts',(-4.25103179814892,-73.4040473005603,
12.));
#69078=CARTESIAN_POINT('Ctrl Pts',(-4.24203684500941,-73.4290864867103,
0.));
#69079=CARTESIAN_POINT('Ctrl Pts',(-4.24203684500941,-73.4290864867103,
12.));
#69080=CARTESIAN_POINT('Ctrl Pts',(-4.23300628072757,-73.4541520732943,
0.));
#69081=CARTESIAN_POINT('Ctrl Pts',(-4.23300628072757,-73.4541520732943,
12.));
#69082=CARTESIAN_POINT('Ctrl Pts',(-4.22394009072753,-73.4792439568624,
0.));
#69083=CARTESIAN_POINT('Ctrl Pts',(-4.22394009072753,-73.4792439568624,
12.));
#69084=CARTESIAN_POINT('Ctrl Pts',(-4.21483826059436,-73.5043620344107,
0.));
#69085=CARTESIAN_POINT('Ctrl Pts',(-4.21483826059436,-73.5043620344107,
12.));
#69086=CARTESIAN_POINT('Ctrl Pts',(-4.20570077603727,-73.5295062032621,
0.));
#69087=CARTESIAN_POINT('Ctrl Pts',(-4.20570077603727,-73.5295062032621,
12.));
#69088=CARTESIAN_POINT('Ctrl Pts',(-4.19652762286126,-73.554676360957,0.));
#69089=CARTESIAN_POINT('Ctrl Pts',(-4.19652762286126,-73.554676360957,12.));
#69090=CARTESIAN_POINT('Ctrl Pts',(-4.18731878694238,-73.5798724051519,
0.));
#69091=CARTESIAN_POINT('Ctrl Pts',(-4.18731878694238,-73.5798724051519,
12.));
#69092=CARTESIAN_POINT('Ctrl Pts',(-4.17807425419816,-73.6050942334773,
0.));
#69093=CARTESIAN_POINT('Ctrl Pts',(-4.17807425419816,-73.6050942334773,
12.));
#69094=CARTESIAN_POINT('Ctrl Pts',(-4.16879401058786,-73.6303417435262,
0.));
#69095=CARTESIAN_POINT('Ctrl Pts',(-4.16879401058786,-73.6303417435262,
12.));
#69096=CARTESIAN_POINT('Ctrl Pts',(-4.1594780421779,-73.6556148331504,0.));
#69097=CARTESIAN_POINT('Ctrl Pts',(-4.1594780421779,-73.6556148331504,12.));
#69098=CARTESIAN_POINT('Ctrl Pts',(-4.15012633519728,-73.6809134006909,
0.));
#69099=CARTESIAN_POINT('Ctrl Pts',(-4.15012633519728,-73.6809134006909,
12.));
#69100=CARTESIAN_POINT('Ctrl Pts',(-4.14073887610155,-73.7062373452344,
0.));
#69101=CARTESIAN_POINT('Ctrl Pts',(-4.14073887610155,-73.7062373452344,
12.));
#69102=CARTESIAN_POINT('Ctrl Pts',(-4.13131565163575,-73.7315865668508,
0.));
#69103=CARTESIAN_POINT('Ctrl Pts',(-4.13131565163575,-73.7315865668508,
12.));
#69104=CARTESIAN_POINT('Ctrl Pts',(-4.12185664890551,-73.7569609668501,
0.));
#69105=CARTESIAN_POINT('Ctrl Pts',(-4.12185664890551,-73.7569609668501,
12.));
#69106=CARTESIAN_POINT('Ctrl Pts',(-4.1123618552278,-73.7823604472126,0.));
#69107=CARTESIAN_POINT('Ctrl Pts',(-4.1123618552278,-73.7823604472126,12.));
#69108=CARTESIAN_POINT('Ctrl Pts',(-4.10283125798724,-73.8077849100314,
0.));
#69109=CARTESIAN_POINT('Ctrl Pts',(-4.10283125798724,-73.8077849100314,
12.));
#69110=CARTESIAN_POINT('Ctrl Pts',(-4.09326484448231,-73.8332342568978,
0.));
#69111=CARTESIAN_POINT('Ctrl Pts',(-4.09326484448231,-73.8332342568978,
12.));
#69112=CARTESIAN_POINT('Ctrl Pts',(-4.08366260180679,-73.8587083884208,
0.));
#69113=CARTESIAN_POINT('Ctrl Pts',(-4.08366260180679,-73.8587083884208,
12.));
#69114=CARTESIAN_POINT('Ctrl Pts',(-4.07402451665253,-73.884207203405,0.));
#69115=CARTESIAN_POINT('Ctrl Pts',(-4.07402451665253,-73.884207203405,12.));
#69116=CARTESIAN_POINT('Ctrl Pts',(-4.06435057547335,-73.9097305995173,
0.));
#69117=CARTESIAN_POINT('Ctrl Pts',(-4.06435057547335,-73.9097305995173,
12.));
#69118=CARTESIAN_POINT('Ctrl Pts',(-4.05464076484761,-73.9352784747665,
0.));
#69119=CARTESIAN_POINT('Ctrl Pts',(-4.05464076484761,-73.9352784747665,
12.));
#69120=CARTESIAN_POINT('Ctrl Pts',(-4.04489507179964,-73.9608507287943,
0.));
#69121=CARTESIAN_POINT('Ctrl Pts',(-4.04489507179964,-73.9608507287943,
12.));
#69122=CARTESIAN_POINT('Ctrl Pts',(-4.0351134841066,-73.9864472641025,0.));
#69123=CARTESIAN_POINT('Ctrl Pts',(-4.0351134841066,-73.9864472641025,12.));
#69124=CARTESIAN_POINT('Ctrl Pts',(-4.02529599070085,-74.0120679876396,
0.));
#69125=CARTESIAN_POINT('Ctrl Pts',(-4.02529599070085,-74.0120679876396,
12.));
#69126=CARTESIAN_POINT('Ctrl Pts',(-4.01544258176693,-74.0377128111754,
0.));
#69127=CARTESIAN_POINT('Ctrl Pts',(-4.01544258176693,-74.0377128111754,
12.));
#69128=CARTESIAN_POINT('Ctrl Pts',(-4.00555324785459,-74.0633816477912,
0.));
#69129=CARTESIAN_POINT('Ctrl Pts',(-4.00555324785459,-74.0633816477912,
12.));
#69130=CARTESIAN_POINT('Ctrl Pts',(-3.99562797918271,-74.0890744091088,
0.));
#69131=CARTESIAN_POINT('Ctrl Pts',(-3.99562797918271,-74.0890744091088,
12.));
#69132=CARTESIAN_POINT('Ctrl Pts',(-3.98566676483639,-74.1147910020869,
0.));
#69133=CARTESIAN_POINT('Ctrl Pts',(-3.98566676483639,-74.1147910020869,
12.));
#69134=CARTESIAN_POINT('Ctrl Pts',(-3.97566959209546,-74.1405313263198,
0.));
#69135=CARTESIAN_POINT('Ctrl Pts',(-3.97566959209546,-74.1405313263198,
12.));
#69136=CARTESIAN_POINT('Ctrl Pts',(-3.96563644549422,-74.1662952702689,
0.));
#69137=CARTESIAN_POINT('Ctrl Pts',(-3.96563644549422,-74.1662952702689,
12.));
#69138=CARTESIAN_POINT('Ctrl Pts',(-3.9555673082116,-74.1920827166861,0.));
#69139=CARTESIAN_POINT('Ctrl Pts',(-3.9555673082116,-74.1920827166861,12.));
#69140=CARTESIAN_POINT('Ctrl Pts',(-3.94546216377498,-74.217893549314,0.));
#69141=CARTESIAN_POINT('Ctrl Pts',(-3.94546216377498,-74.217893549314,12.));
#69142=CARTESIAN_POINT('Ctrl Pts',(-3.93532099774229,-74.2437276593763,
0.));
#69143=CARTESIAN_POINT('Ctrl Pts',(-3.93532099774229,-74.2437276593763,
12.));
#69144=CARTESIAN_POINT('Ctrl Pts',(-3.92514379920729,-74.2695849516134,
0.));
#69145=CARTESIAN_POINT('Ctrl Pts',(-3.92514379920729,-74.2695849516134,
12.));
#69146=CARTESIAN_POINT('Ctrl Pts',(-3.91493056284964,-74.2954653518345,
0.));
#69147=CARTESIAN_POINT('Ctrl Pts',(-3.91493056284964,-74.2954653518345,
12.));
#69148=CARTESIAN_POINT('Ctrl Pts',(-3.9046812890452,-74.3213688089495,0.));
#69149=CARTESIAN_POINT('Ctrl Pts',(-3.9046812890452,-74.3213688089495,12.));
#69150=CARTESIAN_POINT('Ctrl Pts',(-3.89439598145193,-74.3472952898,0.));
#69151=CARTESIAN_POINT('Ctrl Pts',(-3.89439598145193,-74.3472952898,12.));
#69152=CARTESIAN_POINT('Ctrl Pts',(-3.88613891247869,-74.3680548786039,
0.));
#69153=CARTESIAN_POINT('Ctrl Pts',(-3.88613891247869,-74.3680548786039,
12.));
#69154=CARTESIAN_POINT('Ctrl Pts',(-3.87992989995678,-74.3836349188809,
0.));
#69155=CARTESIAN_POINT('Ctrl Pts',(-3.87992989995678,-74.3836349188809,
12.));
#69156=CARTESIAN_POINT('Ctrl Pts',(-3.87578335377301,-74.3940262116251,
0.));
#69157=CARTESIAN_POINT('Ctrl Pts',(-3.87578335377301,-74.3940262116251,
12.));
#69158=CARTESIAN_POINT('Ctrl Pts',(-3.87370827955545,-74.3992230078037,
0.));
#69159=CARTESIAN_POINT('Ctrl Pts',(-3.87370827955545,-74.3992230078037,
12.));
#69160=CARTESIAN_POINT('',(-5.24987136994592,-69.8028570375097,0.));
#69161=CARTESIAN_POINT('Ctrl Pts',(-5.24987136994592,-69.8028570375097,
0.));
#69162=CARTESIAN_POINT('Ctrl Pts',(-5.24915955997427,-69.8066748687772,
0.));
#69163=CARTESIAN_POINT('Ctrl Pts',(-5.24773285666376,-69.8143154684204,
0.));
#69164=CARTESIAN_POINT('Ctrl Pts',(-5.2455835515975,-69.8257911792159,0.));
#69165=CARTESIAN_POINT('Ctrl Pts',(-5.24269931054569,-69.841121750752,0.));
#69166=CARTESIAN_POINT('Ctrl Pts',(-5.23906316634803,-69.8603343302743,
0.));
#69167=CARTESIAN_POINT('Ctrl Pts',(-5.2353961627962,-69.8795962381599,0.));
#69168=CARTESIAN_POINT('Ctrl Pts',(-5.23169827290555,-69.8989073936688,
0.));
#69169=CARTESIAN_POINT('Ctrl Pts',(-5.22796945602794,-69.9182676502048,
0.));
#69170=CARTESIAN_POINT('Ctrl Pts',(-5.22420965879981,-69.9376767969095,
0.));
#69171=CARTESIAN_POINT('Ctrl Pts',(-5.22041882075721,-69.9571345870076,
0.));
#69172=CARTESIAN_POINT('Ctrl Pts',(-5.21659687881139,-69.9766407595385,
0.));
#69173=CARTESIAN_POINT('Ctrl Pts',(-5.21274377203259,-69.9961950629965,
0.));
#69174=CARTESIAN_POINT('Ctrl Pts',(-5.20885944672836,-70.0157972802182,
0.));
#69175=CARTESIAN_POINT('Ctrl Pts',(-5.20494385478025,-70.0354472203546,
0.));
#69176=CARTESIAN_POINT('Ctrl Pts',(-5.20099695122656,-70.0551447071082,
0.));
#69177=CARTESIAN_POINT('Ctrl Pts',(-5.19701869225528,-70.0748895689729,
0.));
#69178=CARTESIAN_POINT('Ctrl Pts',(-5.1930090327158,-70.0946816270997,0.));
#69179=CARTESIAN_POINT('Ctrl Pts',(-5.18896792486565,-70.1145206891885,
0.));
#69180=CARTESIAN_POINT('Ctrl Pts',(-5.18489531966265,-70.1344065558145,
0.));
#69181=CARTESIAN_POINT('Ctrl Pts',(-5.18079116757666,-70.1543390243892,
0.));
#69182=CARTESIAN_POINT('Ctrl Pts',(-5.17665541952383,-70.1743178937077,
0.));
#69183=CARTESIAN_POINT('Ctrl Pts',(-5.17248802793389,-70.1943429691167,
0.));
#69184=CARTESIAN_POINT('Ctrl Pts',(-5.16828894670108,-70.2144140622953,
0.));
#69185=CARTESIAN_POINT('Ctrl Pts',(-5.16405813066976,-70.2345309887833,
0.));
#69186=CARTESIAN_POINT('Ctrl Pts',(-5.15979553528203,-70.2546935662722,
0.));
#69187=CARTESIAN_POINT('Ctrl Pts',(-5.15550111614859,-70.2749016125105,
0.));
#69188=CARTESIAN_POINT('Ctrl Pts',(-5.15117482869254,-70.2951549435512,
0.));
#69189=CARTESIAN_POINT('Ctrl Pts',(-5.1468166283308,-70.3154533746736,0.));
#69190=CARTESIAN_POINT('Ctrl Pts',(-5.14242647063479,-70.3357967211796,
0.));
#69191=CARTESIAN_POINT('Ctrl Pts',(-5.13800431148904,-70.3561847991714,
0.));
#69192=CARTESIAN_POINT('Ctrl Pts',(-5.13355010728567,-70.3766174264757,
0.));
#69193=CARTESIAN_POINT('Ctrl Pts',(-5.12906381499456,-70.3970944229851,
0.));
#69194=CARTESIAN_POINT('Ctrl Pts',(-5.12454539205328,-70.417615610161,0.));
#69195=CARTESIAN_POINT('Ctrl Pts',(-5.11999479630212,-70.4381808107245,
0.));
#69196=CARTESIAN_POINT('Ctrl Pts',(-5.11541198590932,-70.458789848296,0.));
#69197=CARTESIAN_POINT('Ctrl Pts',(-5.11079691929213,-70.4794425469825,
0.));
#69198=CARTESIAN_POINT('Ctrl Pts',(-5.10614955511664,-70.500138731399,0.));
#69199=CARTESIAN_POINT('Ctrl Pts',(-5.10146985232941,-70.5208782268497,
0.));
#69200=CARTESIAN_POINT('Ctrl Pts',(-5.09675777018183,-70.5416608594526,
0.));
#69201=CARTESIAN_POINT('Ctrl Pts',(-5.09201326826134,-70.5624864562824,
0.));
#69202=CARTESIAN_POINT('Ctrl Pts',(-5.08723630652273,-70.5833548455014,
0.));
#69203=CARTESIAN_POINT('Ctrl Pts',(-5.08242684526687,-70.6042658562923,
0.));
#69204=CARTESIAN_POINT('Ctrl Pts',(-5.07758484512302,-70.6252193187878,
0.));
#69205=CARTESIAN_POINT('Ctrl Pts',(-5.07271026703355,-70.6462150640015,
0.));
#69206=CARTESIAN_POINT('Ctrl Pts',(-5.06780307224072,-70.6672529237455,
0.));
#69207=CARTESIAN_POINT('Ctrl Pts',(-5.0628632222782,-70.6883327305784,0.));
#69208=CARTESIAN_POINT('Ctrl Pts',(-5.05789067897057,-70.7094543178438,
0.));
#69209=CARTESIAN_POINT('Ctrl Pts',(-5.05288540443482,-70.7306175196863,
0.));
#69210=CARTESIAN_POINT('Ctrl Pts',(-5.04784736108346,-70.7518221710706,
0.));
#69211=CARTESIAN_POINT('Ctrl Pts',(-5.0427765116335,-70.7730681077983,0.));
#69212=CARTESIAN_POINT('Ctrl Pts',(-5.03767281910479,-70.7943551665059,
0.));
#69213=CARTESIAN_POINT('Ctrl Pts',(-5.03253624680941,-70.8156831846488,
0.));
#69214=CARTESIAN_POINT('Ctrl Pts',(-5.02736675834693,-70.8370520004843,
0.));
#69215=CARTESIAN_POINT('Ctrl Pts',(-5.02216431760061,-70.8584614530519,
0.));
#69216=CARTESIAN_POINT('Ctrl Pts',(-5.0169288887379,-70.8799113821452,0.));
#69217=CARTESIAN_POINT('Ctrl Pts',(-5.01166043620568,-70.9014016283124,
0.));
#69218=CARTESIAN_POINT('Ctrl Pts',(-5.00635892472513,-70.9229320328589,
0.));
#69219=CARTESIAN_POINT('Ctrl Pts',(-5.00102431929039,-70.9445024378439,
0.));
#69220=CARTESIAN_POINT('Ctrl Pts',(-4.99565658516913,-70.9661126860773,
0.));
#69221=CARTESIAN_POINT('Ctrl Pts',(-4.99025568790664,-70.9877626211113,
0.));
#69222=CARTESIAN_POINT('Ctrl Pts',(-4.98482159331863,-71.0094520872377,
0.));
#69223=CARTESIAN_POINT('Ctrl Pts',(-4.97935426748585,-71.0311809294821,
0.));
#69224=CARTESIAN_POINT('Ctrl Pts',(-4.97385367675159,-71.0529489935961,
0.));
#69225=CARTESIAN_POINT('Ctrl Pts',(-4.96831978772191,-71.0747561260436,
0.));
#69226=CARTESIAN_POINT('Ctrl Pts',(-4.96275256726766,-71.0966021739907,
0.));
#69227=CARTESIAN_POINT('Ctrl Pts',(-4.95715198251685,-71.1184869853056,
0.));
#69228=CARTESIAN_POINT('Ctrl Pts',(-4.95151800085101,-71.1404104085552,
0.));
#69229=CARTESIAN_POINT('Ctrl Pts',(-4.94585058990341,-71.1623722930001,
0.));
#69230=CARTESIAN_POINT('Ctrl Pts',(-4.94014971756115,-71.1843724885847,
0.));
#69231=CARTESIAN_POINT('Ctrl Pts',(-4.93441535196617,-71.2064108459286,
0.));
#69232=CARTESIAN_POINT('Ctrl Pts',(-4.92864746150732,-71.2284872163273,
0.));
#69233=CARTESIAN_POINT('Ctrl Pts',(-4.92284601481721,-71.250601451747,0.));
#69234=CARTESIAN_POINT('Ctrl Pts',(-4.91701098077036,-71.2727534048192,
0.));
#69235=CARTESIAN_POINT('Ctrl Pts',(-4.91114232848603,-71.294942928829,0.));
#69236=CARTESIAN_POINT('Ctrl Pts',(-4.90524002732779,-71.3171698777084,
0.));
#69237=CARTESIAN_POINT('Ctrl Pts',(-4.89930404689575,-71.3394341060359,
0.));
#69238=CARTESIAN_POINT('Ctrl Pts',(-4.89333435702414,-71.3617354690325,
0.));
#69239=CARTESIAN_POINT('Ctrl Pts',(-4.88733092777975,-71.3840738225562,
0.));
#69240=CARTESIAN_POINT('Ctrl Pts',(-4.88129372946551,-71.4064490230899,
0.));
#69241=CARTESIAN_POINT('Ctrl Pts',(-4.87522273261908,-71.4288609277374,
0.));
#69242=CARTESIAN_POINT('Ctrl Pts',(-4.8691179080055,-71.4513093942255,0.));
#69243=CARTESIAN_POINT('Ctrl Pts',(-4.86297922661503,-71.4737942808982,
0.));
#69244=CARTESIAN_POINT('Ctrl Pts',(-4.8568066596618,-71.4963154467113,0.));
#69245=CARTESIAN_POINT('Ctrl Pts',(-4.8506001785878,-71.5188727512197,0.));
#69246=CARTESIAN_POINT('Ctrl Pts',(-4.84435975506048,-71.5414660545739,
0.));
#69247=CARTESIAN_POINT('Ctrl Pts',(-4.83808536096583,-71.564095217521,0.));
#69248=CARTESIAN_POINT('Ctrl Pts',(-4.83177696840637,-71.5867601014,0.));
#69249=CARTESIAN_POINT('Ctrl Pts',(-4.82543454970027,-71.6094605681366,
0.));
#69250=CARTESIAN_POINT('Ctrl Pts',(-4.81905807738557,-71.6321964802326,
0.));
#69251=CARTESIAN_POINT('Ctrl Pts',(-4.81264752421732,-71.6549677007613,
0.));
#69252=CARTESIAN_POINT('Ctrl Pts',(-4.80620286316088,-71.6777740933705,
0.));
#69253=CARTESIAN_POINT('Ctrl Pts',(-4.79972406739014,-71.7006155222766,
0.));
#69254=CARTESIAN_POINT('Ctrl Pts',(-4.79321111028672,-71.7234918522604,
0.));
#69255=CARTESIAN_POINT('Ctrl Pts',(-4.7866639654445,-71.7464029486552,0.));
#69256=CARTESIAN_POINT('Ctrl Pts',(-4.78008260666642,-71.7693486773449,
0.));
#69257=CARTESIAN_POINT('Ctrl Pts',(-4.77346700795787,-71.7923289047636,
0.));
#69258=CARTESIAN_POINT('Ctrl Pts',(-4.76681714352503,-71.8153434978924,
0.));
#69259=CARTESIAN_POINT('Ctrl Pts',(-4.76013298777422,-71.8383923242533,
0.));
#69260=CARTESIAN_POINT('Ctrl Pts',(-4.75341451531671,-71.8614752519008,
0.));
#69261=CARTESIAN_POINT('Ctrl Pts',(-4.74666170096545,-71.8845921494186,
0.));
#69262=CARTESIAN_POINT('Ctrl Pts',(-4.7398745197286,-71.9077428859207,0.));
#69263=CARTESIAN_POINT('Ctrl Pts',(-4.73305294680784,-71.9309273310469,
0.));
#69264=CARTESIAN_POINT('Ctrl Pts',(-4.72619695759778,-71.9541453549582,
0.));
#69265=CARTESIAN_POINT('Ctrl Pts',(-4.7193065276908,-71.9773968283267,0.));
#69266=CARTESIAN_POINT('Ctrl Pts',(-4.7123816328741,-72.0006816223335,0.));
#69267=CARTESIAN_POINT('Ctrl Pts',(-4.70542224912312,-72.0239996086694,
0.));
#69268=CARTESIAN_POINT('Ctrl Pts',(-4.69842835259997,-72.047350659532,0.));
#69269=CARTESIAN_POINT('Ctrl Pts',(-4.6913999196528,-72.070734647621,0.));
#69270=CARTESIAN_POINT('Ctrl Pts',(-4.6843369268206,-72.0941514461283,0.));
#69271=CARTESIAN_POINT('Ctrl Pts',(-4.67723935083087,-72.1176009287349,
0.));
#69272=CARTESIAN_POINT('Ctrl Pts',(-4.67010716859281,-72.1410829696129,
0.));
#69273=CARTESIAN_POINT('Ctrl Pts',(-4.6629403571957,-72.1645974434218,0.));
#69274=CARTESIAN_POINT('Ctrl Pts',(-4.65573889390824,-72.1881442253052,
0.));
#69275=CARTESIAN_POINT('Ctrl Pts',(-4.64850275618325,-72.2117231908816,
0.));
#69276=CARTESIAN_POINT('Ctrl Pts',(-4.64123192165627,-72.2353342162408,
0.));
#69277=CARTESIAN_POINT('Ctrl Pts',(-4.63392636813842,-72.2589771779447,
0.));
#69278=CARTESIAN_POINT('Ctrl Pts',(-4.62658607361465,-72.2826519530254,
0.));
#69279=CARTESIAN_POINT('Ctrl Pts',(-4.61921101624294,-72.306358418981,0.));
#69280=CARTESIAN_POINT('Ctrl Pts',(-4.61180117435868,-72.330096453767,0.));
#69281=CARTESIAN_POINT('Ctrl Pts',(-4.60435652647463,-72.3538659357932,
0.));
#69282=CARTESIAN_POINT('Ctrl Pts',(-4.5968770512734,-72.3776667439244,0.));
#69283=CARTESIAN_POINT('Ctrl Pts',(-4.58936272760551,-72.4014987574789,
0.));
#69284=CARTESIAN_POINT('Ctrl Pts',(-4.58181353448851,-72.4253618562249,
0.));
#69285=CARTESIAN_POINT('Ctrl Pts',(-4.57422945111094,-72.449255920373,0.));
#69286=CARTESIAN_POINT('Ctrl Pts',(-4.56661045683366,-72.473180830571,0.));
#69287=CARTESIAN_POINT('Ctrl Pts',(-4.55895653118213,-72.4971364679055,
0.));
#69288=CARTESIAN_POINT('Ctrl Pts',(-4.55126765384403,-72.5211227138997,
0.));
#69289=CARTESIAN_POINT('Ctrl Pts',(-4.54354380466825,-72.5451394505106,
0.));
#69290=CARTESIAN_POINT('Ctrl Pts',(-4.53578496366802,-72.5691865601225,
0.));
#69291=CARTESIAN_POINT('Ctrl Pts',(-4.5279911110239,-72.5932639255406,0.));
#69292=CARTESIAN_POINT('Ctrl Pts',(-4.52016222707632,-72.6173714299935,
0.));
#69293=CARTESIAN_POINT('Ctrl Pts',(-4.5122982923226,-72.6415089571314,0.));
#69294=CARTESIAN_POINT('Ctrl Pts',(-4.50439928741605,-72.6656763910241,
0.));
#69295=CARTESIAN_POINT('Ctrl Pts',(-4.49646519316822,-72.689873616155,0.));
#69296=CARTESIAN_POINT('Ctrl Pts',(-4.48849599055354,-72.7141005174153,
0.));
#69297=CARTESIAN_POINT('Ctrl Pts',(-4.48049166070223,-72.7383569801042,
0.));
#69298=CARTESIAN_POINT('Ctrl Pts',(-4.47245218489623,-72.7626428899287,
0.));
#69299=CARTESIAN_POINT('Ctrl Pts',(-4.46437754456795,-72.7869581329994,
0.));
#69300=CARTESIAN_POINT('Ctrl Pts',(-4.45626772130138,-72.8113025958258,
0.));
#69301=CARTESIAN_POINT('Ctrl Pts',(-4.44812269683724,-72.8356761653064,
0.));
#69302=CARTESIAN_POINT('Ctrl Pts',(-4.43994245306805,-72.8600787287316,
0.));
#69303=CARTESIAN_POINT('Ctrl Pts',(-4.43172697203341,-72.8845101737856,
0.));
#69304=CARTESIAN_POINT('Ctrl Pts',(-4.42347623591941,-72.9089703885463,
0.));
#69305=CARTESIAN_POINT('Ctrl Pts',(-4.41519022705926,-72.9334592614828,
0.));
#69306=CARTESIAN_POINT('Ctrl Pts',(-4.40686892793965,-72.9579766814495,
0.));
#69307=CARTESIAN_POINT('Ctrl Pts',(-4.3985123211973,-72.9825225376839,0.));
#69308=CARTESIAN_POINT('Ctrl Pts',(-4.39012038961145,-73.0070967198033,
0.));
#69309=CARTESIAN_POINT('Ctrl Pts',(-4.38169311610153,-73.031699117799,0.));
#69310=CARTESIAN_POINT('Ctrl Pts',(-4.37323048372607,-73.0563296220301,
0.));
#69311=CARTESIAN_POINT('Ctrl Pts',(-4.36473247568638,-73.0809881232111,
0.));
#69312=CARTESIAN_POINT('Ctrl Pts',(-4.35619907532716,-73.1056745124099,
0.));
#69313=CARTESIAN_POINT('Ctrl Pts',(-4.34763026613154,-73.1303886810602,
0.));
#69314=CARTESIAN_POINT('Ctrl Pts',(-4.33902603172139,-73.1551305209692,
0.));
#69315=CARTESIAN_POINT('Ctrl Pts',(-4.33038635585878,-73.1798999243234,
0.));
#69316=CARTESIAN_POINT('Ctrl Pts',(-4.32171122245218,-73.204696783693,0.));
#69317=CARTESIAN_POINT('Ctrl Pts',(-4.31300061556103,-73.2295209920319,
0.));
#69318=CARTESIAN_POINT('Ctrl Pts',(-4.30425451938234,-73.2543724426562,
0.));
#69319=CARTESIAN_POINT('Ctrl Pts',(-4.29547291824289,-73.2792510292243,
0.));
#69320=CARTESIAN_POINT('Ctrl Pts',(-4.28665579659302,-73.3041566457134,
0.));
#69321=CARTESIAN_POINT('Ctrl Pts',(-4.27780313900392,-73.3290891863959,
0.));
#69322=CARTESIAN_POINT('Ctrl Pts',(-4.26891493016703,-73.354048545808,0.));
#69323=CARTESIAN_POINT('Ctrl Pts',(-4.25999115489904,-73.3790346187953,
0.));
#69324=CARTESIAN_POINT('Ctrl Pts',(-4.25103179814892,-73.4040473005603,
0.));
#69325=CARTESIAN_POINT('Ctrl Pts',(-4.24203684500941,-73.4290864867103,
0.));
#69326=CARTESIAN_POINT('Ctrl Pts',(-4.23300628072757,-73.4541520732943,
0.));
#69327=CARTESIAN_POINT('Ctrl Pts',(-4.22394009072753,-73.4792439568624,
0.));
#69328=CARTESIAN_POINT('Ctrl Pts',(-4.21483826059436,-73.5043620344107,
0.));
#69329=CARTESIAN_POINT('Ctrl Pts',(-4.20570077603727,-73.5295062032621,
0.));
#69330=CARTESIAN_POINT('Ctrl Pts',(-4.19652762286126,-73.554676360957,0.));
#69331=CARTESIAN_POINT('Ctrl Pts',(-4.18731878694238,-73.5798724051519,
0.));
#69332=CARTESIAN_POINT('Ctrl Pts',(-4.17807425419816,-73.6050942334773,
0.));
#69333=CARTESIAN_POINT('Ctrl Pts',(-4.16879401058786,-73.6303417435262,
0.));
#69334=CARTESIAN_POINT('Ctrl Pts',(-4.1594780421779,-73.6556148331504,0.));
#69335=CARTESIAN_POINT('Ctrl Pts',(-4.15012633519728,-73.6809134006909,
0.));
#69336=CARTESIAN_POINT('Ctrl Pts',(-4.14073887610155,-73.7062373452344,
0.));
#69337=CARTESIAN_POINT('Ctrl Pts',(-4.13131565163575,-73.7315865668508,
0.));
#69338=CARTESIAN_POINT('Ctrl Pts',(-4.12185664890551,-73.7569609668501,
0.));
#69339=CARTESIAN_POINT('Ctrl Pts',(-4.1123618552278,-73.7823604472126,0.));
#69340=CARTESIAN_POINT('Ctrl Pts',(-4.10283125798724,-73.8077849100314,
0.));
#69341=CARTESIAN_POINT('Ctrl Pts',(-4.09326484448231,-73.8332342568978,
0.));
#69342=CARTESIAN_POINT('Ctrl Pts',(-4.08366260180679,-73.8587083884208,
0.));
#69343=CARTESIAN_POINT('Ctrl Pts',(-4.07402451665253,-73.884207203405,0.));
#69344=CARTESIAN_POINT('Ctrl Pts',(-4.06435057547335,-73.9097305995173,
0.));
#69345=CARTESIAN_POINT('Ctrl Pts',(-4.05464076484761,-73.9352784747665,
0.));
#69346=CARTESIAN_POINT('Ctrl Pts',(-4.04489507179964,-73.9608507287943,
0.));
#69347=CARTESIAN_POINT('Ctrl Pts',(-4.0351134841066,-73.9864472641025,0.));
#69348=CARTESIAN_POINT('Ctrl Pts',(-4.02529599070085,-74.0120679876396,
0.));
#69349=CARTESIAN_POINT('Ctrl Pts',(-4.01544258176693,-74.0377128111754,
0.));
#69350=CARTESIAN_POINT('Ctrl Pts',(-4.00696550627608,-74.0597159781918,
0.));
#69351=CARTESIAN_POINT('Ctrl Pts',(-4.00044689712494,-74.076598294343,0.));
#69352=CARTESIAN_POINT('Ctrl Pts',(-3.99590266747771,-74.0883491449661,
0.));
#69353=CARTESIAN_POINT('Ctrl Pts',(-3.99334334446578,-74.0949615399272,
0.));
#69354=CARTESIAN_POINT('Ctrl Pts',(-3.99277406492187,-74.0964320765795,
0.));
#69355=CARTESIAN_POINT('',(-5.24987136994592,-69.8028570375097,12.));
#69356=CARTESIAN_POINT('',(-5.24987136994592,-69.8028570375097,0.));
#69357=CARTESIAN_POINT('Ctrl Pts',(-3.99277406492187,-74.0964320765795,
12.));
#69358=CARTESIAN_POINT('Ctrl Pts',(-3.99334334446578,-74.0949615399272,
12.));
#69359=CARTESIAN_POINT('Ctrl Pts',(-3.99590266747771,-74.0883491449661,
12.));
#69360=CARTESIAN_POINT('Ctrl Pts',(-4.00044689712494,-74.076598294343,12.));
#69361=CARTESIAN_POINT('Ctrl Pts',(-4.00696550627608,-74.0597159781918,
12.));
#69362=CARTESIAN_POINT('Ctrl Pts',(-4.01544258176693,-74.0377128111754,
12.));
#69363=CARTESIAN_POINT('Ctrl Pts',(-4.02529599070085,-74.0120679876396,
12.));
#69364=CARTESIAN_POINT('Ctrl Pts',(-4.0351134841066,-73.9864472641025,12.));
#69365=CARTESIAN_POINT('Ctrl Pts',(-4.04489507179964,-73.9608507287943,
12.));
#69366=CARTESIAN_POINT('Ctrl Pts',(-4.05464076484761,-73.9352784747665,
12.));
#69367=CARTESIAN_POINT('Ctrl Pts',(-4.06435057547335,-73.9097305995173,
12.));
#69368=CARTESIAN_POINT('Ctrl Pts',(-4.07402451665253,-73.884207203405,12.));
#69369=CARTESIAN_POINT('Ctrl Pts',(-4.08366260180679,-73.8587083884208,
12.));
#69370=CARTESIAN_POINT('Ctrl Pts',(-4.09326484448231,-73.8332342568978,
12.));
#69371=CARTESIAN_POINT('Ctrl Pts',(-4.10283125798724,-73.8077849100314,
12.));
#69372=CARTESIAN_POINT('Ctrl Pts',(-4.1123618552278,-73.7823604472126,12.));
#69373=CARTESIAN_POINT('Ctrl Pts',(-4.12185664890551,-73.7569609668501,
12.));
#69374=CARTESIAN_POINT('Ctrl Pts',(-4.13131565163575,-73.7315865668508,
12.));
#69375=CARTESIAN_POINT('Ctrl Pts',(-4.14073887610155,-73.7062373452344,
12.));
#69376=CARTESIAN_POINT('Ctrl Pts',(-4.15012633519728,-73.6809134006909,
12.));
#69377=CARTESIAN_POINT('Ctrl Pts',(-4.1594780421779,-73.6556148331504,12.));
#69378=CARTESIAN_POINT('Ctrl Pts',(-4.16879401058786,-73.6303417435262,
12.));
#69379=CARTESIAN_POINT('Ctrl Pts',(-4.17807425419816,-73.6050942334773,
12.));
#69380=CARTESIAN_POINT('Ctrl Pts',(-4.18731878694238,-73.5798724051519,
12.));
#69381=CARTESIAN_POINT('Ctrl Pts',(-4.19652762286126,-73.554676360957,12.));
#69382=CARTESIAN_POINT('Ctrl Pts',(-4.20570077603727,-73.5295062032621,
12.));
#69383=CARTESIAN_POINT('Ctrl Pts',(-4.21483826059436,-73.5043620344107,
12.));
#69384=CARTESIAN_POINT('Ctrl Pts',(-4.22394009072753,-73.4792439568624,
12.));
#69385=CARTESIAN_POINT('Ctrl Pts',(-4.23300628072757,-73.4541520732943,
12.));
#69386=CARTESIAN_POINT('Ctrl Pts',(-4.24203684500941,-73.4290864867103,
12.));
#69387=CARTESIAN_POINT('Ctrl Pts',(-4.25103179814892,-73.4040473005603,
12.));
#69388=CARTESIAN_POINT('Ctrl Pts',(-4.25999115489904,-73.3790346187953,
12.));
#69389=CARTESIAN_POINT('Ctrl Pts',(-4.26891493016703,-73.354048545808,12.));
#69390=CARTESIAN_POINT('Ctrl Pts',(-4.27780313900392,-73.3290891863959,
12.));
#69391=CARTESIAN_POINT('Ctrl Pts',(-4.28665579659302,-73.3041566457134,
12.));
#69392=CARTESIAN_POINT('Ctrl Pts',(-4.29547291824289,-73.2792510292243,
12.));
#69393=CARTESIAN_POINT('Ctrl Pts',(-4.30425451938234,-73.2543724426562,
12.));
#69394=CARTESIAN_POINT('Ctrl Pts',(-4.31300061556103,-73.2295209920319,
12.));
#69395=CARTESIAN_POINT('Ctrl Pts',(-4.32171122245218,-73.204696783693,12.));
#69396=CARTESIAN_POINT('Ctrl Pts',(-4.33038635585878,-73.1798999243234,
12.));
#69397=CARTESIAN_POINT('Ctrl Pts',(-4.33902603172139,-73.1551305209692,
12.));
#69398=CARTESIAN_POINT('Ctrl Pts',(-4.34763026613154,-73.1303886810602,
12.));
#69399=CARTESIAN_POINT('Ctrl Pts',(-4.35619907532716,-73.1056745124099,
12.));
#69400=CARTESIAN_POINT('Ctrl Pts',(-4.36473247568638,-73.0809881232111,
12.));
#69401=CARTESIAN_POINT('Ctrl Pts',(-4.37323048372607,-73.0563296220301,
12.));
#69402=CARTESIAN_POINT('Ctrl Pts',(-4.38169311610153,-73.031699117799,12.));
#69403=CARTESIAN_POINT('Ctrl Pts',(-4.39012038961145,-73.0070967198033,
12.));
#69404=CARTESIAN_POINT('Ctrl Pts',(-4.3985123211973,-72.9825225376839,12.));
#69405=CARTESIAN_POINT('Ctrl Pts',(-4.40686892793965,-72.9579766814495,
12.));
#69406=CARTESIAN_POINT('Ctrl Pts',(-4.41519022705926,-72.9334592614828,
12.));
#69407=CARTESIAN_POINT('Ctrl Pts',(-4.42347623591941,-72.9089703885463,
12.));
#69408=CARTESIAN_POINT('Ctrl Pts',(-4.43172697203341,-72.8845101737856,
12.));
#69409=CARTESIAN_POINT('Ctrl Pts',(-4.43994245306805,-72.8600787287316,
12.));
#69410=CARTESIAN_POINT('Ctrl Pts',(-4.44812269683724,-72.8356761653064,
12.));
#69411=CARTESIAN_POINT('Ctrl Pts',(-4.45626772130138,-72.8113025958258,
12.));
#69412=CARTESIAN_POINT('Ctrl Pts',(-4.46437754456795,-72.7869581329994,
12.));
#69413=CARTESIAN_POINT('Ctrl Pts',(-4.47245218489623,-72.7626428899287,
12.));
#69414=CARTESIAN_POINT('Ctrl Pts',(-4.48049166070223,-72.7383569801042,
12.));
#69415=CARTESIAN_POINT('Ctrl Pts',(-4.48849599055354,-72.7141005174153,
12.));
#69416=CARTESIAN_POINT('Ctrl Pts',(-4.49646519316822,-72.689873616155,12.));
#69417=CARTESIAN_POINT('Ctrl Pts',(-4.50439928741605,-72.6656763910241,
12.));
#69418=CARTESIAN_POINT('Ctrl Pts',(-4.5122982923226,-72.6415089571314,12.));
#69419=CARTESIAN_POINT('Ctrl Pts',(-4.52016222707632,-72.6173714299935,
12.));
#69420=CARTESIAN_POINT('Ctrl Pts',(-4.5279911110239,-72.5932639255406,12.));
#69421=CARTESIAN_POINT('Ctrl Pts',(-4.53578496366802,-72.5691865601225,
12.));
#69422=CARTESIAN_POINT('Ctrl Pts',(-4.54354380466825,-72.5451394505106,
12.));
#69423=CARTESIAN_POINT('Ctrl Pts',(-4.55126765384403,-72.5211227138997,
12.));
#69424=CARTESIAN_POINT('Ctrl Pts',(-4.55895653118213,-72.4971364679055,
12.));
#69425=CARTESIAN_POINT('Ctrl Pts',(-4.56661045683366,-72.473180830571,12.));
#69426=CARTESIAN_POINT('Ctrl Pts',(-4.57422945111094,-72.449255920373,12.));
#69427=CARTESIAN_POINT('Ctrl Pts',(-4.58181353448851,-72.4253618562249,
12.));
#69428=CARTESIAN_POINT('Ctrl Pts',(-4.58936272760551,-72.4014987574789,
12.));
#69429=CARTESIAN_POINT('Ctrl Pts',(-4.5968770512734,-72.3776667439244,12.));
#69430=CARTESIAN_POINT('Ctrl Pts',(-4.60435652647463,-72.3538659357932,
12.));
#69431=CARTESIAN_POINT('Ctrl Pts',(-4.61180117435868,-72.330096453767,12.));
#69432=CARTESIAN_POINT('Ctrl Pts',(-4.61921101624294,-72.306358418981,12.));
#69433=CARTESIAN_POINT('Ctrl Pts',(-4.62658607361465,-72.2826519530254,
12.));
#69434=CARTESIAN_POINT('Ctrl Pts',(-4.63392636813842,-72.2589771779447,
12.));
#69435=CARTESIAN_POINT('Ctrl Pts',(-4.64123192165627,-72.2353342162408,
12.));
#69436=CARTESIAN_POINT('Ctrl Pts',(-4.64850275618325,-72.2117231908816,
12.));
#69437=CARTESIAN_POINT('Ctrl Pts',(-4.65573889390824,-72.1881442253052,
12.));
#69438=CARTESIAN_POINT('Ctrl Pts',(-4.6629403571957,-72.1645974434218,12.));
#69439=CARTESIAN_POINT('Ctrl Pts',(-4.67010716859281,-72.1410829696129,
12.));
#69440=CARTESIAN_POINT('Ctrl Pts',(-4.67723935083087,-72.1176009287349,
12.));
#69441=CARTESIAN_POINT('Ctrl Pts',(-4.6843369268206,-72.0941514461283,12.));
#69442=CARTESIAN_POINT('Ctrl Pts',(-4.6913999196528,-72.070734647621,12.));
#69443=CARTESIAN_POINT('Ctrl Pts',(-4.69842835259997,-72.047350659532,12.));
#69444=CARTESIAN_POINT('Ctrl Pts',(-4.70542224912312,-72.0239996086694,
12.));
#69445=CARTESIAN_POINT('Ctrl Pts',(-4.7123816328741,-72.0006816223335,12.));
#69446=CARTESIAN_POINT('Ctrl Pts',(-4.7193065276908,-71.9773968283267,12.));
#69447=CARTESIAN_POINT('Ctrl Pts',(-4.72619695759778,-71.9541453549582,
12.));
#69448=CARTESIAN_POINT('Ctrl Pts',(-4.73305294680784,-71.9309273310469,
12.));
#69449=CARTESIAN_POINT('Ctrl Pts',(-4.7398745197286,-71.9077428859207,12.));
#69450=CARTESIAN_POINT('Ctrl Pts',(-4.74666170096545,-71.8845921494186,
12.));
#69451=CARTESIAN_POINT('Ctrl Pts',(-4.75341451531671,-71.8614752519008,
12.));
#69452=CARTESIAN_POINT('Ctrl Pts',(-4.76013298777422,-71.8383923242533,
12.));
#69453=CARTESIAN_POINT('Ctrl Pts',(-4.76681714352503,-71.8153434978924,
12.));
#69454=CARTESIAN_POINT('Ctrl Pts',(-4.77346700795787,-71.7923289047636,
12.));
#69455=CARTESIAN_POINT('Ctrl Pts',(-4.78008260666642,-71.7693486773449,
12.));
#69456=CARTESIAN_POINT('Ctrl Pts',(-4.7866639654445,-71.7464029486552,12.));
#69457=CARTESIAN_POINT('Ctrl Pts',(-4.79321111028672,-71.7234918522604,
12.));
#69458=CARTESIAN_POINT('Ctrl Pts',(-4.79972406739014,-71.7006155222766,
12.));
#69459=CARTESIAN_POINT('Ctrl Pts',(-4.80620286316088,-71.6777740933705,
12.));
#69460=CARTESIAN_POINT('Ctrl Pts',(-4.81264752421732,-71.6549677007613,
12.));
#69461=CARTESIAN_POINT('Ctrl Pts',(-4.81905807738557,-71.6321964802326,
12.));
#69462=CARTESIAN_POINT('Ctrl Pts',(-4.82543454970027,-71.6094605681366,
12.));
#69463=CARTESIAN_POINT('Ctrl Pts',(-4.83177696840637,-71.5867601014,12.));
#69464=CARTESIAN_POINT('Ctrl Pts',(-4.83808536096583,-71.564095217521,12.));
#69465=CARTESIAN_POINT('Ctrl Pts',(-4.84435975506048,-71.5414660545739,
12.));
#69466=CARTESIAN_POINT('Ctrl Pts',(-4.8506001785878,-71.5188727512197,12.));
#69467=CARTESIAN_POINT('Ctrl Pts',(-4.8568066596618,-71.4963154467113,12.));
#69468=CARTESIAN_POINT('Ctrl Pts',(-4.86297922661503,-71.4737942808982,
12.));
#69469=CARTESIAN_POINT('Ctrl Pts',(-4.8691179080055,-71.4513093942255,12.));
#69470=CARTESIAN_POINT('Ctrl Pts',(-4.87522273261908,-71.4288609277374,
12.));
#69471=CARTESIAN_POINT('Ctrl Pts',(-4.88129372946551,-71.4064490230899,
12.));
#69472=CARTESIAN_POINT('Ctrl Pts',(-4.88733092777975,-71.3840738225562,
12.));
#69473=CARTESIAN_POINT('Ctrl Pts',(-4.89333435702414,-71.3617354690325,
12.));
#69474=CARTESIAN_POINT('Ctrl Pts',(-4.89930404689575,-71.3394341060359,
12.));
#69475=CARTESIAN_POINT('Ctrl Pts',(-4.90524002732779,-71.3171698777084,
12.));
#69476=CARTESIAN_POINT('Ctrl Pts',(-4.91114232848603,-71.294942928829,12.));
#69477=CARTESIAN_POINT('Ctrl Pts',(-4.91701098077036,-71.2727534048192,
12.));
#69478=CARTESIAN_POINT('Ctrl Pts',(-4.92284601481721,-71.250601451747,12.));
#69479=CARTESIAN_POINT('Ctrl Pts',(-4.92864746150732,-71.2284872163273,
12.));
#69480=CARTESIAN_POINT('Ctrl Pts',(-4.93441535196617,-71.2064108459286,
12.));
#69481=CARTESIAN_POINT('Ctrl Pts',(-4.94014971756115,-71.1843724885847,
12.));
#69482=CARTESIAN_POINT('Ctrl Pts',(-4.94585058990341,-71.1623722930001,
12.));
#69483=CARTESIAN_POINT('Ctrl Pts',(-4.95151800085101,-71.1404104085552,
12.));
#69484=CARTESIAN_POINT('Ctrl Pts',(-4.95715198251685,-71.1184869853056,
12.));
#69485=CARTESIAN_POINT('Ctrl Pts',(-4.96275256726766,-71.0966021739907,
12.));
#69486=CARTESIAN_POINT('Ctrl Pts',(-4.96831978772191,-71.0747561260436,
12.));
#69487=CARTESIAN_POINT('Ctrl Pts',(-4.97385367675159,-71.0529489935961,
12.));
#69488=CARTESIAN_POINT('Ctrl Pts',(-4.97935426748585,-71.0311809294821,
12.));
#69489=CARTESIAN_POINT('Ctrl Pts',(-4.98482159331863,-71.0094520872377,
12.));
#69490=CARTESIAN_POINT('Ctrl Pts',(-4.99025568790664,-70.9877626211113,
12.));
#69491=CARTESIAN_POINT('Ctrl Pts',(-4.99565658516913,-70.9661126860773,
12.));
#69492=CARTESIAN_POINT('Ctrl Pts',(-5.00102431929039,-70.9445024378439,
12.));
#69493=CARTESIAN_POINT('Ctrl Pts',(-5.00635892472513,-70.9229320328589,
12.));
#69494=CARTESIAN_POINT('Ctrl Pts',(-5.01166043620568,-70.9014016283124,
12.));
#69495=CARTESIAN_POINT('Ctrl Pts',(-5.0169288887379,-70.8799113821452,12.));
#69496=CARTESIAN_POINT('Ctrl Pts',(-5.02216431760061,-70.8584614530519,
12.));
#69497=CARTESIAN_POINT('Ctrl Pts',(-5.02736675834693,-70.8370520004843,
12.));
#69498=CARTESIAN_POINT('Ctrl Pts',(-5.03253624680941,-70.8156831846488,
12.));
#69499=CARTESIAN_POINT('Ctrl Pts',(-5.03767281910479,-70.7943551665059,
12.));
#69500=CARTESIAN_POINT('Ctrl Pts',(-5.0427765116335,-70.7730681077983,12.));
#69501=CARTESIAN_POINT('Ctrl Pts',(-5.04784736108346,-70.7518221710706,
12.));
#69502=CARTESIAN_POINT('Ctrl Pts',(-5.05288540443482,-70.7306175196863,
12.));
#69503=CARTESIAN_POINT('Ctrl Pts',(-5.05789067897057,-70.7094543178438,
12.));
#69504=CARTESIAN_POINT('Ctrl Pts',(-5.0628632222782,-70.6883327305784,12.));
#69505=CARTESIAN_POINT('Ctrl Pts',(-5.06780307224072,-70.6672529237455,
12.));
#69506=CARTESIAN_POINT('Ctrl Pts',(-5.07271026703355,-70.6462150640015,
12.));
#69507=CARTESIAN_POINT('Ctrl Pts',(-5.07758484512302,-70.6252193187878,
12.));
#69508=CARTESIAN_POINT('Ctrl Pts',(-5.08242684526687,-70.6042658562923,
12.));
#69509=CARTESIAN_POINT('Ctrl Pts',(-5.08723630652273,-70.5833548455014,
12.));
#69510=CARTESIAN_POINT('Ctrl Pts',(-5.09201326826134,-70.5624864562824,
12.));
#69511=CARTESIAN_POINT('Ctrl Pts',(-5.09675777018183,-70.5416608594526,
12.));
#69512=CARTESIAN_POINT('Ctrl Pts',(-5.10146985232941,-70.5208782268497,
12.));
#69513=CARTESIAN_POINT('Ctrl Pts',(-5.10614955511664,-70.500138731399,12.));
#69514=CARTESIAN_POINT('Ctrl Pts',(-5.11079691929213,-70.4794425469825,
12.));
#69515=CARTESIAN_POINT('Ctrl Pts',(-5.11541198590932,-70.458789848296,12.));
#69516=CARTESIAN_POINT('Ctrl Pts',(-5.11999479630212,-70.4381808107245,
12.));
#69517=CARTESIAN_POINT('Ctrl Pts',(-5.12454539205328,-70.417615610161,12.));
#69518=CARTESIAN_POINT('Ctrl Pts',(-5.12906381499456,-70.3970944229851,
12.));
#69519=CARTESIAN_POINT('Ctrl Pts',(-5.13355010728567,-70.3766174264757,
12.));
#69520=CARTESIAN_POINT('Ctrl Pts',(-5.13800431148904,-70.3561847991714,
12.));
#69521=CARTESIAN_POINT('Ctrl Pts',(-5.14242647063479,-70.3357967211796,
12.));
#69522=CARTESIAN_POINT('Ctrl Pts',(-5.1468166283308,-70.3154533746736,12.));
#69523=CARTESIAN_POINT('Ctrl Pts',(-5.15117482869254,-70.2951549435512,
12.));
#69524=CARTESIAN_POINT('Ctrl Pts',(-5.15550111614859,-70.2749016125105,
12.));
#69525=CARTESIAN_POINT('Ctrl Pts',(-5.15979553528203,-70.2546935662722,
12.));
#69526=CARTESIAN_POINT('Ctrl Pts',(-5.16405813066976,-70.2345309887833,
12.));
#69527=CARTESIAN_POINT('Ctrl Pts',(-5.16828894670108,-70.2144140622953,
12.));
#69528=CARTESIAN_POINT('Ctrl Pts',(-5.17248802793389,-70.1943429691167,
12.));
#69529=CARTESIAN_POINT('Ctrl Pts',(-5.17665541952383,-70.1743178937077,
12.));
#69530=CARTESIAN_POINT('Ctrl Pts',(-5.18079116757666,-70.1543390243892,
12.));
#69531=CARTESIAN_POINT('Ctrl Pts',(-5.18489531966265,-70.1344065558145,
12.));
#69532=CARTESIAN_POINT('Ctrl Pts',(-5.18896792486565,-70.1145206891885,
12.));
#69533=CARTESIAN_POINT('Ctrl Pts',(-5.1930090327158,-70.0946816270997,12.));
#69534=CARTESIAN_POINT('Ctrl Pts',(-5.19701869225528,-70.0748895689729,
12.));
#69535=CARTESIAN_POINT('Ctrl Pts',(-5.20099695122656,-70.0551447071082,
12.));
#69536=CARTESIAN_POINT('Ctrl Pts',(-5.20494385478025,-70.0354472203546,
12.));
#69537=CARTESIAN_POINT('Ctrl Pts',(-5.20885944672836,-70.0157972802182,
12.));
#69538=CARTESIAN_POINT('Ctrl Pts',(-5.21274377203259,-69.9961950629965,
12.));
#69539=CARTESIAN_POINT('Ctrl Pts',(-5.21659687881139,-69.9766407595385,
12.));
#69540=CARTESIAN_POINT('Ctrl Pts',(-5.22041882075721,-69.9571345870076,
12.));
#69541=CARTESIAN_POINT('Ctrl Pts',(-5.22420965879981,-69.9376767969095,
12.));
#69542=CARTESIAN_POINT('Ctrl Pts',(-5.22796945602794,-69.9182676502048,
12.));
#69543=CARTESIAN_POINT('Ctrl Pts',(-5.23169827290555,-69.8989073936688,
12.));
#69544=CARTESIAN_POINT('Ctrl Pts',(-5.2353961627962,-69.8795962381599,12.));
#69545=CARTESIAN_POINT('Ctrl Pts',(-5.23906316634803,-69.8603343302743,
12.));
#69546=CARTESIAN_POINT('Ctrl Pts',(-5.24269931054569,-69.841121750752,12.));
#69547=CARTESIAN_POINT('Ctrl Pts',(-5.2455835515975,-69.8257911792159,12.));
#69548=CARTESIAN_POINT('Ctrl Pts',(-5.24773285666376,-69.8143154684204,
12.));
#69549=CARTESIAN_POINT('Ctrl Pts',(-5.24915955997427,-69.8066748687772,
12.));
#69550=CARTESIAN_POINT('Ctrl Pts',(-5.24987136994592,-69.8028570375097,
12.));
#69551=CARTESIAN_POINT('Ctrl Pts',(-2.480349218449,-74.1624659714954,0.));
#69552=CARTESIAN_POINT('Ctrl Pts',(-2.480349218449,-74.1624659714954,4.));
#69553=CARTESIAN_POINT('Ctrl Pts',(-2.480349218449,-74.1624659714954,8.));
#69554=CARTESIAN_POINT('Ctrl Pts',(-2.480349218449,-74.1624659714954,12.));
#69555=CARTESIAN_POINT('Ctrl Pts',(-2.52879860312845,-74.2610905805697,
0.));
#69556=CARTESIAN_POINT('Ctrl Pts',(-2.52879860312845,-74.2610905805697,
4.));
#69557=CARTESIAN_POINT('Ctrl Pts',(-2.52879860312844,-74.2610905805697,
8.));
#69558=CARTESIAN_POINT('Ctrl Pts',(-2.52879860312844,-74.2610905805697,
12.));
#69559=CARTESIAN_POINT('Ctrl Pts',(-2.67239300265255,-74.4041075779818,
-7.30788408099537E-17));
#69560=CARTESIAN_POINT('Ctrl Pts',(-2.67239300265255,-74.4041075779818,
4.));
#69561=CARTESIAN_POINT('Ctrl Pts',(-2.67239300265254,-74.4041075779819,
7.99999999999999));
#69562=CARTESIAN_POINT('Ctrl Pts',(-2.67239300265254,-74.4041075779819,
12.));
#69563=CARTESIAN_POINT('Ctrl Pts',(-2.86656650944673,-74.4448761712979,
-2.46611180197105E-16));
#69564=CARTESIAN_POINT('Ctrl Pts',(-2.86656650944673,-74.4448761712979,
4.));
#69565=CARTESIAN_POINT('Ctrl Pts',(-2.86656650944675,-74.444876171298,8.00000000000001));
#69566=CARTESIAN_POINT('Ctrl Pts',(-2.86656650944675,-74.444876171298,12.));
#69567=CARTESIAN_POINT('Ctrl Pts',(-2.94891377268011,-74.4416140848738,
-3.30265160424791E-16));
#69568=CARTESIAN_POINT('Ctrl Pts',(-2.94891377268011,-74.4416140848738,
4.));
#69569=CARTESIAN_POINT('Ctrl Pts',(-2.94891377268014,-74.4416140848739,
8.));
#69570=CARTESIAN_POINT('Ctrl Pts',(-2.94891377268014,-74.4416140848739,
12.));
#69571=CARTESIAN_POINT('',(-2.480349218449,-74.1624659714954,0.));
#69572=CARTESIAN_POINT('',(-2.94891377268011,-74.4416140848739,0.));
#69573=CARTESIAN_POINT('Ctrl Pts',(-2.480349218449,-74.1624659714954,2.74425517504386E-17));
#69574=CARTESIAN_POINT('Ctrl Pts',(-2.52879860312845,-74.2610905805697,
2.74425517504386E-17));
#69575=CARTESIAN_POINT('Ctrl Pts',(-2.61085254571365,-74.3428145790909,
-1.43167858552492E-17));
#69576=CARTESIAN_POINT('Ctrl Pts',(-2.70942211516255,-74.3911513436216,
-8.88772658534914E-17));
#69577=CARTESIAN_POINT('Ctrl Pts',(-2.78334929224922,-74.4274039170196,
-1.44797625852173E-16));
#69578=CARTESIAN_POINT('Ctrl Pts',(-2.86656650944673,-74.4448761712979,
-2.19168628446667E-16));
#69579=CARTESIAN_POINT('Ctrl Pts',(-2.94891377268011,-74.4416140848738,
-3.02822608674353E-16));
#69580=CARTESIAN_POINT('',(-2.94891377268014,-74.4416140848739,12.));
#69581=CARTESIAN_POINT('Ctrl Pts',(-2.94891377268011,-74.4416140848738,
-3.30265160424791E-16));
#69582=CARTESIAN_POINT('Ctrl Pts',(-2.94891377268011,-74.4416140848738,
4.));
#69583=CARTESIAN_POINT('Ctrl Pts',(-2.94891377268014,-74.4416140848739,
8.));
#69584=CARTESIAN_POINT('Ctrl Pts',(-2.94891377268014,-74.4416140848739,
12.));
#69585=CARTESIAN_POINT('',(-2.480349218449,-74.1624659714954,12.));
#69586=CARTESIAN_POINT('Ctrl Pts',(-2.94891377268014,-74.4416140848739,
12.));
#69587=CARTESIAN_POINT('Ctrl Pts',(-2.86656650944675,-74.444876171298,12.));
#69588=CARTESIAN_POINT('Ctrl Pts',(-2.78334929224923,-74.4274039170196,
12.));
#69589=CARTESIAN_POINT('Ctrl Pts',(-2.70942211516255,-74.3911513436216,
12.));
#69590=CARTESIAN_POINT('Ctrl Pts',(-2.61085254571364,-74.342814579091,12.));
#69591=CARTESIAN_POINT('Ctrl Pts',(-2.52879860312844,-74.2610905805697,
12.));
#69592=CARTESIAN_POINT('Ctrl Pts',(-2.480349218449,-74.1624659714954,12.));
#69593=CARTESIAN_POINT('Ctrl Pts',(-2.480349218449,-74.1624659714954,12.));
#69594=CARTESIAN_POINT('Ctrl Pts',(-2.480349218449,-74.1624659714954,8.));
#69595=CARTESIAN_POINT('Ctrl Pts',(-2.480349218449,-74.1624659714954,4.));
#69596=CARTESIAN_POINT('Ctrl Pts',(-2.480349218449,-74.1624659714954,0.));
#69597=CARTESIAN_POINT('Origin',(-1.62512913209675E-11,-3.74491326291036E-10,
0.));
#69598=CARTESIAN_POINT('Origin',(-1.62512913209675E-11,-3.74491326291036E-10,
12.));
#69599=CARTESIAN_POINT('Origin',(-1.62512913209675E-11,-3.74491326291036E-10,
0.));
#69600=CARTESIAN_POINT('Ctrl Pts',(-10.0225374821204,-73.8227522002498,
-5.55111512312578E-16));
#69601=CARTESIAN_POINT('Ctrl Pts',(-10.0225374821204,-73.8227522002498,
4.));
#69602=CARTESIAN_POINT('Ctrl Pts',(-10.0225374821204,-73.8227522002498,
8.));
#69603=CARTESIAN_POINT('Ctrl Pts',(-10.0225374821204,-73.8227522002498,
12.));
#69604=CARTESIAN_POINT('Ctrl Pts',(-10.1314210536414,-73.8079696346555,
-5.55111512312578E-16));
#69605=CARTESIAN_POINT('Ctrl Pts',(-10.1314210536414,-73.8079696346555,
4.));
#69606=CARTESIAN_POINT('Ctrl Pts',(-10.1314210536414,-73.8079696346555,
8.00000000000001));
#69607=CARTESIAN_POINT('Ctrl Pts',(-10.1314210536414,-73.8079696346555,
12.));
#69608=CARTESIAN_POINT('Ctrl Pts',(-10.3125002643516,-73.7169567649192,
-6.28191717183155E-16));
#69609=CARTESIAN_POINT('Ctrl Pts',(-10.3125002643516,-73.7169567649192,
4.00000000000001));
#69610=CARTESIAN_POINT('Ctrl Pts',(-10.3125002643516,-73.7169567649192,
8.));
#69611=CARTESIAN_POINT('Ctrl Pts',(-10.3125002643516,-73.7169567649192,
12.));
#69612=CARTESIAN_POINT('Ctrl Pts',(-10.4125694172275,-73.5456341632196,
-8.01722692545273E-16));
#69613=CARTESIAN_POINT('Ctrl Pts',(-10.4125694172275,-73.5456341632196,
4.));
#69614=CARTESIAN_POINT('Ctrl Pts',(-10.4125694172275,-73.5456341632196,
8.00000000000001));
#69615=CARTESIAN_POINT('Ctrl Pts',(-10.4125694172275,-73.5456341632196,
12.));
#69616=CARTESIAN_POINT('Ctrl Pts',(-10.4355099267388,-73.4664795929518,
-8.85376672782757E-16));
#69617=CARTESIAN_POINT('Ctrl Pts',(-10.4355099267388,-73.4664795929518,
4.));
#69618=CARTESIAN_POINT('Ctrl Pts',(-10.4355099267388,-73.4664795929518,
8.));
#69619=CARTESIAN_POINT('Ctrl Pts',(-10.4355099267388,-73.4664795929518,
12.));
#69620=CARTESIAN_POINT('',(-10.0225374821204,-73.8227522002498,0.));
#69621=CARTESIAN_POINT('',(-10.4355099267391,-73.4664795929519,0.));
#69622=CARTESIAN_POINT('Ctrl Pts',(-10.0225374821204,-73.8227522002498,
-5.27668960562141E-16));
#69623=CARTESIAN_POINT('Ctrl Pts',(-10.1314210536414,-73.8079696346555,
-5.27668960562141E-16));
#69624=CARTESIAN_POINT('Ctrl Pts',(-10.234894888333,-73.7559622805204,-5.69429077631042E-16));
#69625=CARTESIAN_POINT('Ctrl Pts',(-10.3119164592419,-73.6777313404382,
-6.43989446289017E-16));
#69626=CARTESIAN_POINT('Ctrl Pts',(-10.3696826374235,-73.6190581353765,
-6.99909722782499E-16));
#69627=CARTESIAN_POINT('Ctrl Pts',(-10.4125694172275,-73.5456341632196,
-7.74280140794835E-16));
#69628=CARTESIAN_POINT('Ctrl Pts',(-10.4355099267388,-73.4664795929518,
-8.5793412103232E-16));
#69629=CARTESIAN_POINT('',(-10.4355099267391,-73.4664795929519,12.));
#69630=CARTESIAN_POINT('Ctrl Pts',(-10.4355099267388,-73.4664795929518,
-8.85376672782757E-16));
#69631=CARTESIAN_POINT('Ctrl Pts',(-10.4355099267388,-73.4664795929518,
4.));
#69632=CARTESIAN_POINT('Ctrl Pts',(-10.4355099267388,-73.4664795929518,
8.));
#69633=CARTESIAN_POINT('Ctrl Pts',(-10.4355099267388,-73.4664795929518,
12.));
#69634=CARTESIAN_POINT('',(-10.0225374821204,-73.8227522002498,12.));
#69635=CARTESIAN_POINT('Ctrl Pts',(-10.4355099267388,-73.4664795929518,
12.));
#69636=CARTESIAN_POINT('Ctrl Pts',(-10.4125694172275,-73.5456341632196,
12.));
#69637=CARTESIAN_POINT('Ctrl Pts',(-10.3696826374235,-73.6190581353765,
12.));
#69638=CARTESIAN_POINT('Ctrl Pts',(-10.3119164592419,-73.6777313404382,
12.));
#69639=CARTESIAN_POINT('Ctrl Pts',(-10.234894888333,-73.7559622805204,12.));
#69640=CARTESIAN_POINT('Ctrl Pts',(-10.1314210536414,-73.8079696346555,
12.));
#69641=CARTESIAN_POINT('Ctrl Pts',(-10.0225374821204,-73.8227522002498,
12.));
#69642=CARTESIAN_POINT('Ctrl Pts',(-10.0225374821204,-73.8227522002498,
12.));
#69643=CARTESIAN_POINT('Ctrl Pts',(-10.0225374821204,-73.8227522002498,
8.));
#69644=CARTESIAN_POINT('Ctrl Pts',(-10.0225374821204,-73.8227522002498,
4.));
#69645=CARTESIAN_POINT('Ctrl Pts',(-10.0225374821204,-73.8227522002498,
-5.55111512312578E-16));
#69646=CARTESIAN_POINT('Ctrl Pts',(-11.3136138754165,-69.079679653846,0.));
#69647=CARTESIAN_POINT('Ctrl Pts',(-11.3136138754165,-69.079679653846,12.));
#69648=CARTESIAN_POINT('Ctrl Pts',(-11.3132375200165,-69.0835449954396,
0.));
#69649=CARTESIAN_POINT('Ctrl Pts',(-11.3132375200165,-69.0835449954396,
12.));
#69650=CARTESIAN_POINT('Ctrl Pts',(-11.3124821678798,-69.0912808656811,
0.));
#69651=CARTESIAN_POINT('Ctrl Pts',(-11.3124821678798,-69.0912808656811,
12.));
#69652=CARTESIAN_POINT('Ctrl Pts',(-11.3113412156661,-69.1029002322118,
0.));
#69653=CARTESIAN_POINT('Ctrl Pts',(-11.3113412156661,-69.1029002322118,
12.));
#69654=CARTESIAN_POINT('Ctrl Pts',(-11.3098040973713,-69.118423844466,0.));
#69655=CARTESIAN_POINT('Ctrl Pts',(-11.3098040973713,-69.118423844466,12.));
#69656=CARTESIAN_POINT('Ctrl Pts',(-11.3078562764384,-69.1378802251711,
0.));
#69657=CARTESIAN_POINT('Ctrl Pts',(-11.3078562764384,-69.1378802251711,
12.));
#69658=CARTESIAN_POINT('Ctrl Pts',(-11.3058820128307,-69.1573884361,0.));
#69659=CARTESIAN_POINT('Ctrl Pts',(-11.3058820128307,-69.1573884361,12.));
#69660=CARTESIAN_POINT('Ctrl Pts',(-11.3038812726292,-69.1769483991721,
0.));
#69661=CARTESIAN_POINT('Ctrl Pts',(-11.3038812726292,-69.1769483991721,
12.));
#69662=CARTESIAN_POINT('Ctrl Pts',(-11.3018540025638,-69.1965599718914,
0.));
#69663=CARTESIAN_POINT('Ctrl Pts',(-11.3018540025638,-69.1965599718914,
12.));
#69664=CARTESIAN_POINT('Ctrl Pts',(-11.2998001310964,-69.2162229488531,
0.));
#69665=CARTESIAN_POINT('Ctrl Pts',(-11.2998001310964,-69.2162229488531,
12.));
#69666=CARTESIAN_POINT('Ctrl Pts',(-11.2977195764852,-69.2359370894907,
0.));
#69667=CARTESIAN_POINT('Ctrl Pts',(-11.2977195764852,-69.2359370894907,
12.));
#69668=CARTESIAN_POINT('Ctrl Pts',(-11.2956122531375,-69.255702139335,0.));
#69669=CARTESIAN_POINT('Ctrl Pts',(-11.2956122531375,-69.255702139335,12.));
#69670=CARTESIAN_POINT('Ctrl Pts',(-11.2934780784351,-69.275517853148,0.));
#69671=CARTESIAN_POINT('Ctrl Pts',(-11.2934780784351,-69.275517853148,12.));
#69672=CARTESIAN_POINT('Ctrl Pts',(-11.2913169799628,-69.295384019272,0.));
#69673=CARTESIAN_POINT('Ctrl Pts',(-11.2913169799628,-69.295384019272,12.));
#69674=CARTESIAN_POINT('Ctrl Pts',(-11.2891288931517,-69.3153004517783,
0.));
#69675=CARTESIAN_POINT('Ctrl Pts',(-11.2891288931517,-69.3153004517783,
12.));
#69676=CARTESIAN_POINT('Ctrl Pts',(-11.2869137578459,-69.3352669789587,
0.));
#69677=CARTESIAN_POINT('Ctrl Pts',(-11.2869137578459,-69.3352669789587,
12.));
#69678=CARTESIAN_POINT('Ctrl Pts',(-11.2846715154524,-69.3552834337784,
0.));
#69679=CARTESIAN_POINT('Ctrl Pts',(-11.2846715154524,-69.3552834337784,
12.));
#69680=CARTESIAN_POINT('Ctrl Pts',(-11.2824021054045,-69.3753496420039,
0.));
#69681=CARTESIAN_POINT('Ctrl Pts',(-11.2824021054045,-69.3753496420039,
12.));
#69682=CARTESIAN_POINT('Ctrl Pts',(-11.2801054633815,-69.3954654162281,
0.));
#69683=CARTESIAN_POINT('Ctrl Pts',(-11.2801054633815,-69.3954654162281,
12.));
#69684=CARTESIAN_POINT('Ctrl Pts',(-11.2777815231469,-69.4156305620593,
0.));
#69685=CARTESIAN_POINT('Ctrl Pts',(-11.2777815231469,-69.4156305620593,
12.));
#69686=CARTESIAN_POINT('Ctrl Pts',(-11.2754302177021,-69.4358448819967,
0.));
#69687=CARTESIAN_POINT('Ctrl Pts',(-11.2754302177021,-69.4358448819967,
12.));
#69688=CARTESIAN_POINT('Ctrl Pts',(-11.2730514806139,-69.456108179879,0.));
#69689=CARTESIAN_POINT('Ctrl Pts',(-11.2730514806139,-69.456108179879,12.));
#69690=CARTESIAN_POINT('Ctrl Pts',(-11.270645247528,-69.4764202659397,0.));
#69691=CARTESIAN_POINT('Ctrl Pts',(-11.270645247528,-69.4764202659397,12.));
#69692=CARTESIAN_POINT('Ctrl Pts',(-11.2682114561007,-69.4967809565929,
0.));
#69693=CARTESIAN_POINT('Ctrl Pts',(-11.2682114561007,-69.4967809565929,
12.));
#69694=CARTESIAN_POINT('Ctrl Pts',(-11.2657500452716,-69.5171900720158,
0.));
#69695=CARTESIAN_POINT('Ctrl Pts',(-11.2657500452716,-69.5171900720158,
12.));
#69696=CARTESIAN_POINT('Ctrl Pts',(-11.263260954763,-69.5376474344771,0.));
#69697=CARTESIAN_POINT('Ctrl Pts',(-11.263260954763,-69.5376474344771,12.));
#69698=CARTESIAN_POINT('Ctrl Pts',(-11.2607441244702,-69.5581528662877,
0.));
#69699=CARTESIAN_POINT('Ctrl Pts',(-11.2607441244702,-69.5581528662877,
12.));
#69700=CARTESIAN_POINT('Ctrl Pts',(-11.2581994939541,-69.5787061880857,
0.));
#69701=CARTESIAN_POINT('Ctrl Pts',(-11.2581994939541,-69.5787061880857,
12.));
#69702=CARTESIAN_POINT('Ctrl Pts',(-11.2556270027016,-69.599307219739,0.));
#69703=CARTESIAN_POINT('Ctrl Pts',(-11.2556270027016,-69.599307219739,12.));
#69704=CARTESIAN_POINT('Ctrl Pts',(-11.2530265903557,-69.6199557811245,
0.));
#69705=CARTESIAN_POINT('Ctrl Pts',(-11.2530265903557,-69.6199557811245,
12.));
#69706=CARTESIAN_POINT('Ctrl Pts',(-11.2503981969412,-69.6406516928891,
0.));
#69707=CARTESIAN_POINT('Ctrl Pts',(-11.2503981969412,-69.6406516928891,
12.));
#69708=CARTESIAN_POINT('Ctrl Pts',(-11.2477417631386,-69.6613947773534,
0.));
#69709=CARTESIAN_POINT('Ctrl Pts',(-11.2477417631386,-69.6613947773534,
12.));
#69710=CARTESIAN_POINT('Ctrl Pts',(-11.2450572303841,-69.6821848588457,
0.));
#69711=CARTESIAN_POINT('Ctrl Pts',(-11.2450572303841,-69.6821848588457,
12.));
#69712=CARTESIAN_POINT('Ctrl Pts',(-11.2423445407166,-69.7030217632164,
0.));
#69713=CARTESIAN_POINT('Ctrl Pts',(-11.2423445407166,-69.7030217632164,
12.));
#69714=CARTESIAN_POINT('Ctrl Pts',(-11.239603636686,-69.7239053175356,0.));
#69715=CARTESIAN_POINT('Ctrl Pts',(-11.239603636686,-69.7239053175356,12.));
#69716=CARTESIAN_POINT('Ctrl Pts',(-11.2368344612472,-69.7448353497408,
0.));
#69717=CARTESIAN_POINT('Ctrl Pts',(-11.2368344612472,-69.7448353497408,
12.));
#69718=CARTESIAN_POINT('Ctrl Pts',(-11.2340369576456,-69.7658116882324,
0.));
#69719=CARTESIAN_POINT('Ctrl Pts',(-11.2340369576456,-69.7658116882324,
12.));
#69720=CARTESIAN_POINT('Ctrl Pts',(-11.2312110694187,-69.7868341618954,
0.));
#69721=CARTESIAN_POINT('Ctrl Pts',(-11.2312110694187,-69.7868341618954,
12.));
#69722=CARTESIAN_POINT('Ctrl Pts',(-11.2283567404437,-69.8079026002768,
0.));
#69723=CARTESIAN_POINT('Ctrl Pts',(-11.2283567404437,-69.8079026002768,
12.));
#69724=CARTESIAN_POINT('Ctrl Pts',(-11.225473914972,-69.8290168337076,0.));
#69725=CARTESIAN_POINT('Ctrl Pts',(-11.225473914972,-69.8290168337076,12.));
#69726=CARTESIAN_POINT('Ctrl Pts',(-11.2225625376736,-69.8501766934428,
0.));
#69727=CARTESIAN_POINT('Ctrl Pts',(-11.2225625376736,-69.8501766934428,
12.));
#69728=CARTESIAN_POINT('Ctrl Pts',(-11.219622553679,-69.871382011789,0.));
#69729=CARTESIAN_POINT('Ctrl Pts',(-11.219622553679,-69.871382011789,12.));
#69730=CARTESIAN_POINT('Ctrl Pts',(-11.2166539085523,-69.8926326220385,
0.));
#69731=CARTESIAN_POINT('Ctrl Pts',(-11.2166539085523,-69.8926326220385,
12.));
#69732=CARTESIAN_POINT('Ctrl Pts',(-11.2136565482677,-69.9139283584022,
0.));
#69733=CARTESIAN_POINT('Ctrl Pts',(-11.2136565482677,-69.9139283584022,
12.));
#69734=CARTESIAN_POINT('Ctrl Pts',(-11.2106304191882,-69.9352690559405,
0.));
#69735=CARTESIAN_POINT('Ctrl Pts',(-11.2106304191882,-69.9352690559405,
12.));
#69736=CARTESIAN_POINT('Ctrl Pts',(-11.2075754680449,-69.9566545504837,
0.));
#69737=CARTESIAN_POINT('Ctrl Pts',(-11.2075754680449,-69.9566545504837,
12.));
#69738=CARTESIAN_POINT('Ctrl Pts',(-11.2044916419244,-69.97808467858,0.));
#69739=CARTESIAN_POINT('Ctrl Pts',(-11.2044916419244,-69.97808467858,12.));
#69740=CARTESIAN_POINT('Ctrl Pts',(-11.2013788882714,-69.9995592775343,
0.));
#69741=CARTESIAN_POINT('Ctrl Pts',(-11.2013788882714,-69.9995592775343,
12.));
#69742=CARTESIAN_POINT('Ctrl Pts',(-11.1982371548919,-70.0210781854243,
0.));
#69743=CARTESIAN_POINT('Ctrl Pts',(-11.1982371548919,-70.0210781854243,
12.));
#69744=CARTESIAN_POINT('Ctrl Pts',(-11.1950663899576,-70.0426412411185,
0.));
#69745=CARTESIAN_POINT('Ctrl Pts',(-11.1950663899576,-70.0426412411185,
12.));
#69746=CARTESIAN_POINT('Ctrl Pts',(-11.1918665420166,-70.0642482842928,
0.));
#69747=CARTESIAN_POINT('Ctrl Pts',(-11.1918665420166,-70.0642482842928,
12.));
#69748=CARTESIAN_POINT('Ctrl Pts',(-11.1886375599914,-70.0858991554283,
0.));
#69749=CARTESIAN_POINT('Ctrl Pts',(-11.1886375599914,-70.0858991554283,
12.));
#69750=CARTESIAN_POINT('Ctrl Pts',(-11.185379393167,-70.1075936957968,0.));
#69751=CARTESIAN_POINT('Ctrl Pts',(-11.185379393167,-70.1075936957968,12.));
#69752=CARTESIAN_POINT('Ctrl Pts',(-11.1820919911846,-70.1293317474432,
0.));
#69753=CARTESIAN_POINT('Ctrl Pts',(-11.1820919911846,-70.1293317474432,
12.));
#69754=CARTESIAN_POINT('Ctrl Pts',(-11.1787753040363,-70.1511131531674,
0.));
#69755=CARTESIAN_POINT('Ctrl Pts',(-11.1787753040363,-70.1511131531674,
12.));
#69756=CARTESIAN_POINT('Ctrl Pts',(-11.1754292820631,-70.1729377564956,
0.));
#69757=CARTESIAN_POINT('Ctrl Pts',(-11.1754292820631,-70.1729377564956,
12.));
#69758=CARTESIAN_POINT('Ctrl Pts',(-11.1720538759498,-70.1948054016817,
0.));
#69759=CARTESIAN_POINT('Ctrl Pts',(-11.1720538759498,-70.1948054016817,
12.));
#69760=CARTESIAN_POINT('Ctrl Pts',(-11.168649036721,-70.2167159337095,0.));
#69761=CARTESIAN_POINT('Ctrl Pts',(-11.168649036721,-70.2167159337095,12.));
#69762=CARTESIAN_POINT('Ctrl Pts',(-11.1652147157383,-70.2386691982902,
0.));
#69763=CARTESIAN_POINT('Ctrl Pts',(-11.1652147157383,-70.2386691982902,
12.));
#69764=CARTESIAN_POINT('Ctrl Pts',(-11.1617508647017,-70.2606650418589,
0.));
#69765=CARTESIAN_POINT('Ctrl Pts',(-11.1617508647017,-70.2606650418589,
12.));
#69766=CARTESIAN_POINT('Ctrl Pts',(-11.1582574356522,-70.2827033115662,
0.));
#69767=CARTESIAN_POINT('Ctrl Pts',(-11.1582574356522,-70.2827033115662,
12.));
#69768=CARTESIAN_POINT('Ctrl Pts',(-11.1547343809647,-70.3047838552758,
0.));
#69769=CARTESIAN_POINT('Ctrl Pts',(-11.1547343809647,-70.3047838552758,
12.));
#69770=CARTESIAN_POINT('Ctrl Pts',(-11.1511816533422,-70.3269065215591,
0.));
#69771=CARTESIAN_POINT('Ctrl Pts',(-11.1511816533422,-70.3269065215591,
12.));
#69772=CARTESIAN_POINT('Ctrl Pts',(-11.1475992058124,-70.3490711596882,
0.));
#69773=CARTESIAN_POINT('Ctrl Pts',(-11.1475992058124,-70.3490711596882,
12.));
#69774=CARTESIAN_POINT('Ctrl Pts',(-11.1439869917269,-70.3712776196216,
0.));
#69775=CARTESIAN_POINT('Ctrl Pts',(-11.1439869917269,-70.3712776196216,
12.));
#69776=CARTESIAN_POINT('Ctrl Pts',(-11.1403449647622,-70.3935257519945,
0.));
#69777=CARTESIAN_POINT('Ctrl Pts',(-11.1403449647622,-70.3935257519945,
12.));
#69778=CARTESIAN_POINT('Ctrl Pts',(-11.1366730789122,-70.415815408119,0.));
#69779=CARTESIAN_POINT('Ctrl Pts',(-11.1366730789122,-70.415815408119,12.));
#69780=CARTESIAN_POINT('Ctrl Pts',(-11.1329712884845,-70.438146439981,0.));
#69781=CARTESIAN_POINT('Ctrl Pts',(-11.1329712884845,-70.438146439981,12.));
#69782=CARTESIAN_POINT('Ctrl Pts',(-11.1292395480975,-70.4605187002356,
0.));
#69783=CARTESIAN_POINT('Ctrl Pts',(-11.1292395480975,-70.4605187002356,
12.));
#69784=CARTESIAN_POINT('Ctrl Pts',(-11.1254778126824,-70.4829320421973,
0.));
#69785=CARTESIAN_POINT('Ctrl Pts',(-11.1254778126824,-70.4829320421973,
12.));
#69786=CARTESIAN_POINT('Ctrl Pts',(-11.121686037483,-70.5053863198306,0.));
#69787=CARTESIAN_POINT('Ctrl Pts',(-11.121686037483,-70.5053863198306,12.));
#69788=CARTESIAN_POINT('Ctrl Pts',(-11.117864178048,-70.5278813877519,0.));
#69789=CARTESIAN_POINT('Ctrl Pts',(-11.117864178048,-70.5278813877519,12.));
#69790=CARTESIAN_POINT('Ctrl Pts',(-11.1140121902274,-70.5504171012247,
0.));
#69791=CARTESIAN_POINT('Ctrl Pts',(-11.1140121902274,-70.5504171012247,
12.));
#69792=CARTESIAN_POINT('Ctrl Pts',(-11.11013003017,-70.5729933161538,0.));
#69793=CARTESIAN_POINT('Ctrl Pts',(-11.11013003017,-70.5729933161538,12.));
#69794=CARTESIAN_POINT('Ctrl Pts',(-11.1062176543257,-70.5956098890744,
0.));
#69795=CARTESIAN_POINT('Ctrl Pts',(-11.1062176543257,-70.5956098890744,
12.));
#69796=CARTESIAN_POINT('Ctrl Pts',(-11.1022750194439,-70.6182666771441,
0.));
#69797=CARTESIAN_POINT('Ctrl Pts',(-11.1022750194439,-70.6182666771441,
12.));
#69798=CARTESIAN_POINT('Ctrl Pts',(-11.0983020825662,-70.6409635381446,
0.));
#69799=CARTESIAN_POINT('Ctrl Pts',(-11.0983020825662,-70.6409635381446,
12.));
#69800=CARTESIAN_POINT('Ctrl Pts',(-11.0942988010231,-70.6637003304768,
0.));
#69801=CARTESIAN_POINT('Ctrl Pts',(-11.0942988010231,-70.6637003304768,
12.));
#69802=CARTESIAN_POINT('Ctrl Pts',(-11.0902651324325,-70.686476913156,0.));
#69803=CARTESIAN_POINT('Ctrl Pts',(-11.0902651324325,-70.686476913156,12.));
#69804=CARTESIAN_POINT('Ctrl Pts',(-11.0862010347022,-70.7092931457996,
0.));
#69805=CARTESIAN_POINT('Ctrl Pts',(-11.0862010347022,-70.7092931457996,
12.));
#69806=CARTESIAN_POINT('Ctrl Pts',(-11.0821064660276,-70.7321488886229,
0.));
#69807=CARTESIAN_POINT('Ctrl Pts',(-11.0821064660276,-70.7321488886229,
12.));
#69808=CARTESIAN_POINT('Ctrl Pts',(-11.0779813848851,-70.7550440024422,
0.));
#69809=CARTESIAN_POINT('Ctrl Pts',(-11.0779813848851,-70.7550440024422,
12.));
#69810=CARTESIAN_POINT('Ctrl Pts',(-11.0738257500292,-70.7779783486689,
0.));
#69811=CARTESIAN_POINT('Ctrl Pts',(-11.0738257500292,-70.7779783486689,
12.));
#69812=CARTESIAN_POINT('Ctrl Pts',(-11.0696395204907,-70.8009517893042,
0.));
#69813=CARTESIAN_POINT('Ctrl Pts',(-11.0696395204907,-70.8009517893042,
12.));
#69814=CARTESIAN_POINT('Ctrl Pts',(-11.0654226555798,-70.8239641869266,
0.));
#69815=CARTESIAN_POINT('Ctrl Pts',(-11.0654226555798,-70.8239641869266,
12.));
#69816=CARTESIAN_POINT('Ctrl Pts',(-11.061175114883,-70.847015404688,0.));
#69817=CARTESIAN_POINT('Ctrl Pts',(-11.061175114883,-70.847015404688,12.));
#69818=CARTESIAN_POINT('Ctrl Pts',(-11.0568968582566,-70.8701053063158,
0.));
#69819=CARTESIAN_POINT('Ctrl Pts',(-11.0568968582566,-70.8701053063158,
12.));
#69820=CARTESIAN_POINT('Ctrl Pts',(-11.0525878458242,-70.8932337561078,
0.));
#69821=CARTESIAN_POINT('Ctrl Pts',(-11.0525878458242,-70.8932337561078,
12.));
#69822=CARTESIAN_POINT('Ctrl Pts',(-11.0482480379752,-70.9164006189283,
0.));
#69823=CARTESIAN_POINT('Ctrl Pts',(-11.0482480379752,-70.9164006189283,
12.));
#69824=CARTESIAN_POINT('Ctrl Pts',(-11.0438773953686,-70.9396057601953,
0.));
#69825=CARTESIAN_POINT('Ctrl Pts',(-11.0438773953686,-70.9396057601953,
12.));
#69826=CARTESIAN_POINT('Ctrl Pts',(-11.039475878929,-70.9628490458779,0.));
#69827=CARTESIAN_POINT('Ctrl Pts',(-11.039475878929,-70.9628490458779,12.));
#69828=CARTESIAN_POINT('Ctrl Pts',(-11.0350434498408,-70.9861303424989,
0.));
#69829=CARTESIAN_POINT('Ctrl Pts',(-11.0350434498408,-70.9861303424989,
12.));
#69830=CARTESIAN_POINT('Ctrl Pts',(-11.0305800695457,-71.0094495171295,
0.));
#69831=CARTESIAN_POINT('Ctrl Pts',(-11.0305800695457,-71.0094495171295,
12.));
#69832=CARTESIAN_POINT('Ctrl Pts',(-11.0260856997414,-71.0328064373849,
0.));
#69833=CARTESIAN_POINT('Ctrl Pts',(-11.0260856997414,-71.0328064373849,
12.));
#69834=CARTESIAN_POINT('Ctrl Pts',(-11.0215603023854,-71.0562009714125,
0.));
#69835=CARTESIAN_POINT('Ctrl Pts',(-11.0215603023854,-71.0562009714125,
12.));
#69836=CARTESIAN_POINT('Ctrl Pts',(-11.0170038396913,-71.0796329878896,
0.));
#69837=CARTESIAN_POINT('Ctrl Pts',(-11.0170038396913,-71.0796329878896,
12.));
#69838=CARTESIAN_POINT('Ctrl Pts',(-11.0124162741223,-71.1031023560243,
0.));
#69839=CARTESIAN_POINT('Ctrl Pts',(-11.0124162741223,-71.1031023560243,
12.));
#69840=CARTESIAN_POINT('Ctrl Pts',(-11.0077975683895,-71.1266089455517,
0.));
#69841=CARTESIAN_POINT('Ctrl Pts',(-11.0077975683895,-71.1266089455517,
12.));
#69842=CARTESIAN_POINT('Ctrl Pts',(-11.0031476854503,-71.1501526267288,
0.));
#69843=CARTESIAN_POINT('Ctrl Pts',(-11.0031476854503,-71.1501526267288,
12.));
#69844=CARTESIAN_POINT('Ctrl Pts',(-10.9984665885127,-71.1737332703248,
0.));
#69845=CARTESIAN_POINT('Ctrl Pts',(-10.9984665885127,-71.1737332703248,
12.));
#69846=CARTESIAN_POINT('Ctrl Pts',(-10.993754241032,-71.1973507476188,0.));
#69847=CARTESIAN_POINT('Ctrl Pts',(-10.993754241032,-71.1973507476188,12.));
#69848=CARTESIAN_POINT('Ctrl Pts',(-10.9890106067038,-71.221004930401,0.));
#69849=CARTESIAN_POINT('Ctrl Pts',(-10.9890106067038,-71.221004930401,12.));
#69850=CARTESIAN_POINT('Ctrl Pts',(-10.9842356494627,-71.2446956909685,
0.));
#69851=CARTESIAN_POINT('Ctrl Pts',(-10.9842356494627,-71.2446956909685,
12.));
#69852=CARTESIAN_POINT('Ctrl Pts',(-10.9794293334806,-71.2684229021209,
0.));
#69853=CARTESIAN_POINT('Ctrl Pts',(-10.9794293334806,-71.2684229021209,
12.));
#69854=CARTESIAN_POINT('Ctrl Pts',(-10.9745916231711,-71.2921864371499,
0.));
#69855=CARTESIAN_POINT('Ctrl Pts',(-10.9745916231711,-71.2921864371499,
12.));
#69856=CARTESIAN_POINT('Ctrl Pts',(-10.9697224831862,-71.3159861698368,
0.));
#69857=CARTESIAN_POINT('Ctrl Pts',(-10.9697224831862,-71.3159861698368,
12.));
#69858=CARTESIAN_POINT('Ctrl Pts',(-10.96482187841,-71.3398219744547,0.));
#69859=CARTESIAN_POINT('Ctrl Pts',(-10.96482187841,-71.3398219744547,12.));
#69860=CARTESIAN_POINT('Ctrl Pts',(-10.9598897739565,-71.3636937257651,
0.));
#69861=CARTESIAN_POINT('Ctrl Pts',(-10.9598897739565,-71.3636937257651,
12.));
#69862=CARTESIAN_POINT('Ctrl Pts',(-10.9549261351689,-71.3876012990135,
0.));
#69863=CARTESIAN_POINT('Ctrl Pts',(-10.9549261351689,-71.3876012990135,
12.));
#69864=CARTESIAN_POINT('Ctrl Pts',(-10.9499309276235,-71.411544569919,0.));
#69865=CARTESIAN_POINT('Ctrl Pts',(-10.9499309276235,-71.411544569919,12.));
#69866=CARTESIAN_POINT('Ctrl Pts',(-10.9449041171269,-71.4355234146718,
0.));
#69867=CARTESIAN_POINT('Ctrl Pts',(-10.9449041171269,-71.4355234146718,
12.));
#69868=CARTESIAN_POINT('Ctrl Pts',(-10.9398456697094,-71.4595377099352,
0.));
#69869=CARTESIAN_POINT('Ctrl Pts',(-10.9398456697094,-71.4595377099352,
12.));
#69870=CARTESIAN_POINT('Ctrl Pts',(-10.9347555516236,-71.4835873328425,
0.));
#69871=CARTESIAN_POINT('Ctrl Pts',(-10.9347555516236,-71.4835873328425,
12.));
#69872=CARTESIAN_POINT('Ctrl Pts',(-10.9296337293425,-71.5076721609936,
0.));
#69873=CARTESIAN_POINT('Ctrl Pts',(-10.9296337293425,-71.5076721609936,
12.));
#69874=CARTESIAN_POINT('Ctrl Pts',(-10.9244801695642,-71.5317920724453,
0.));
#69875=CARTESIAN_POINT('Ctrl Pts',(-10.9244801695642,-71.5317920724453,
12.));
#69876=CARTESIAN_POINT('Ctrl Pts',(-10.9192948392099,-71.5559469457082,
0.));
#69877=CARTESIAN_POINT('Ctrl Pts',(-10.9192948392099,-71.5559469457082,
12.));
#69878=CARTESIAN_POINT('Ctrl Pts',(-10.9140777054169,-71.5801366597479,
0.));
#69879=CARTESIAN_POINT('Ctrl Pts',(-10.9140777054169,-71.5801366597479,
12.));
#69880=CARTESIAN_POINT('Ctrl Pts',(-10.9088287355364,-71.604361093983,0.));
#69881=CARTESIAN_POINT('Ctrl Pts',(-10.9088287355364,-71.604361093983,12.));
#69882=CARTESIAN_POINT('Ctrl Pts',(-10.9035478971329,-71.6286201282815,
0.));
#69883=CARTESIAN_POINT('Ctrl Pts',(-10.9035478971329,-71.6286201282815,
12.));
#69884=CARTESIAN_POINT('Ctrl Pts',(-10.8982351579872,-71.6529136429515,
0.));
#69885=CARTESIAN_POINT('Ctrl Pts',(-10.8982351579872,-71.6529136429515,
12.));
#69886=CARTESIAN_POINT('Ctrl Pts',(-10.8928904860967,-71.6772415187382,
0.));
#69887=CARTESIAN_POINT('Ctrl Pts',(-10.8928904860967,-71.6772415187382,
12.));
#69888=CARTESIAN_POINT('Ctrl Pts',(-10.8875138496674,-71.7016036368254,
0.));
#69889=CARTESIAN_POINT('Ctrl Pts',(-10.8875138496674,-71.7016036368254,
12.));
#69890=CARTESIAN_POINT('Ctrl Pts',(-10.8821052171122,-71.7259998788337,
0.));
#69891=CARTESIAN_POINT('Ctrl Pts',(-10.8821052171122,-71.7259998788337,
12.));
#69892=CARTESIAN_POINT('Ctrl Pts',(-10.8766645570496,-71.7504301268177,
0.));
#69893=CARTESIAN_POINT('Ctrl Pts',(-10.8766645570496,-71.7504301268177,
12.));
#69894=CARTESIAN_POINT('Ctrl Pts',(-10.8711918383071,-71.7748942632578,
0.));
#69895=CARTESIAN_POINT('Ctrl Pts',(-10.8711918383071,-71.7748942632578,
12.));
#69896=CARTESIAN_POINT('Ctrl Pts',(-10.8656870299218,-71.7993921710546,
0.));
#69897=CARTESIAN_POINT('Ctrl Pts',(-10.8656870299218,-71.7993921710546,
12.));
#69898=CARTESIAN_POINT('Ctrl Pts',(-10.860150101133,-71.8239237335318,0.));
#69899=CARTESIAN_POINT('Ctrl Pts',(-10.860150101133,-71.8239237335318,12.));
#69900=CARTESIAN_POINT('Ctrl Pts',(-10.8545810213799,-71.8484888344335,
0.));
#69901=CARTESIAN_POINT('Ctrl Pts',(-10.8545810213799,-71.8484888344335,
12.));
#69902=CARTESIAN_POINT('Ctrl Pts',(-10.8489797602998,-71.8730873579226,
0.));
#69903=CARTESIAN_POINT('Ctrl Pts',(-10.8489797602998,-71.8730873579226,
12.));
#69904=CARTESIAN_POINT('Ctrl Pts',(-10.8433462877312,-71.8977191885726,
0.));
#69905=CARTESIAN_POINT('Ctrl Pts',(-10.8433462877312,-71.8977191885726,
12.));
#69906=CARTESIAN_POINT('Ctrl Pts',(-10.8376805737158,-71.9223842113622,
0.));
#69907=CARTESIAN_POINT('Ctrl Pts',(-10.8376805737158,-71.9223842113622,
12.));
#69908=CARTESIAN_POINT('Ctrl Pts',(-10.8319825884917,-71.9470823116777,
0.));
#69909=CARTESIAN_POINT('Ctrl Pts',(-10.8319825884917,-71.9470823116777,
12.));
#69910=CARTESIAN_POINT('Ctrl Pts',(-10.8262523024897,-71.971813375312,0.));
#69911=CARTESIAN_POINT('Ctrl Pts',(-10.8262523024897,-71.971813375312,12.));
#69912=CARTESIAN_POINT('Ctrl Pts',(-10.8204896863328,-71.9965772884619,
0.));
#69913=CARTESIAN_POINT('Ctrl Pts',(-10.8204896863328,-71.9965772884619,
12.));
#69914=CARTESIAN_POINT('Ctrl Pts',(-10.8146947108376,-72.0213739377231,
0.));
#69915=CARTESIAN_POINT('Ctrl Pts',(-10.8146947108376,-72.0213739377231,
12.));
#69916=CARTESIAN_POINT('Ctrl Pts',(-10.8088673470187,-72.0462032100828,
0.));
#69917=CARTESIAN_POINT('Ctrl Pts',(-10.8088673470187,-72.0462032100828,
12.));
#69918=CARTESIAN_POINT('Ctrl Pts',(-10.8030075660811,-72.0710649929214,
0.));
#69919=CARTESIAN_POINT('Ctrl Pts',(-10.8030075660811,-72.0710649929214,
12.));
#69920=CARTESIAN_POINT('Ctrl Pts',(-10.7971153394168,-72.095959174012,0.));
#69921=CARTESIAN_POINT('Ctrl Pts',(-10.7971153394168,-72.095959174012,12.));
#69922=CARTESIAN_POINT('Ctrl Pts',(-10.7911906386027,-72.1208856415171,
0.));
#69923=CARTESIAN_POINT('Ctrl Pts',(-10.7911906386027,-72.1208856415171,
12.));
#69924=CARTESIAN_POINT('Ctrl Pts',(-10.7852334354015,-72.145844283983,0.));
#69925=CARTESIAN_POINT('Ctrl Pts',(-10.7852334354015,-72.145844283983,12.));
#69926=CARTESIAN_POINT('Ctrl Pts',(-10.779243701766,-72.17083499033,0.));
#69927=CARTESIAN_POINT('Ctrl Pts',(-10.779243701766,-72.17083499033,12.));
#69928=CARTESIAN_POINT('Ctrl Pts',(-10.7732214098343,-72.1958576498556,
0.));
#69929=CARTESIAN_POINT('Ctrl Pts',(-10.7732214098343,-72.1958576498556,
12.));
#69930=CARTESIAN_POINT('Ctrl Pts',(-10.7671665319254,-72.2209121522367,
0.));
#69931=CARTESIAN_POINT('Ctrl Pts',(-10.7671665319254,-72.2209121522367,
12.));
#69932=CARTESIAN_POINT('Ctrl Pts',(-10.7610790405385,-72.2459983875298,
0.));
#69933=CARTESIAN_POINT('Ctrl Pts',(-10.7610790405385,-72.2459983875298,
12.));
#69934=CARTESIAN_POINT('Ctrl Pts',(-10.7549589083535,-72.2711162461679,
0.));
#69935=CARTESIAN_POINT('Ctrl Pts',(-10.7549589083535,-72.2711162461679,
12.));
#69936=CARTESIAN_POINT('Ctrl Pts',(-10.7488061082368,-72.296265618955,0.));
#69937=CARTESIAN_POINT('Ctrl Pts',(-10.7488061082368,-72.296265618955,12.));
#69938=CARTESIAN_POINT('Ctrl Pts',(-10.7426206132375,-72.3214463970634,
0.));
#69939=CARTESIAN_POINT('Ctrl Pts',(-10.7426206132375,-72.3214463970634,
12.));
#69940=CARTESIAN_POINT('Ctrl Pts',(-10.73640239658,-72.3466584720311,0.));
#69941=CARTESIAN_POINT('Ctrl Pts',(-10.73640239658,-72.3466584720311,12.));
#69942=CARTESIAN_POINT('Ctrl Pts',(-10.7301514316607,-72.3719017357568,
0.));
#69943=CARTESIAN_POINT('Ctrl Pts',(-10.7301514316607,-72.3719017357568,
12.));
#69944=CARTESIAN_POINT('Ctrl Pts',(-10.7238676920469,-72.3971760804935,
0.));
#69945=CARTESIAN_POINT('Ctrl Pts',(-10.7238676920469,-72.3971760804935,
12.));
#69946=CARTESIAN_POINT('Ctrl Pts',(-10.7175511514789,-72.4224813988355,
0.));
#69947=CARTESIAN_POINT('Ctrl Pts',(-10.7175511514789,-72.4224813988355,
12.));
#69948=CARTESIAN_POINT('Ctrl Pts',(-10.7112017838707,-72.4478175837168,
0.));
#69949=CARTESIAN_POINT('Ctrl Pts',(-10.7112017838707,-72.4478175837168,
12.));
#69950=CARTESIAN_POINT('Ctrl Pts',(-10.7048195633062,-72.4731845284238,
0.));
#69951=CARTESIAN_POINT('Ctrl Pts',(-10.7048195633062,-72.4731845284238,
12.));
#69952=CARTESIAN_POINT('Ctrl Pts',(-10.6984044640399,-72.4985821266031,
0.));
#69953=CARTESIAN_POINT('Ctrl Pts',(-10.6984044640399,-72.4985821266031,
12.));
#69954=CARTESIAN_POINT('Ctrl Pts',(-10.691956460499,-72.5240102722662,0.));
#69955=CARTESIAN_POINT('Ctrl Pts',(-10.691956460499,-72.5240102722662,12.));
#69956=CARTESIAN_POINT('Ctrl Pts',(-10.6854755272903,-72.5494688597951,
0.));
#69957=CARTESIAN_POINT('Ctrl Pts',(-10.6854755272903,-72.5494688597951,
12.));
#69958=CARTESIAN_POINT('Ctrl Pts',(-10.6789616392041,-72.57495778394,0.));
#69959=CARTESIAN_POINT('Ctrl Pts',(-10.6789616392041,-72.57495778394,12.));
#69960=CARTESIAN_POINT('Ctrl Pts',(-10.6724147711994,-72.6004769398004,
0.));
#69961=CARTESIAN_POINT('Ctrl Pts',(-10.6724147711994,-72.6004769398004,
12.));
#69962=CARTESIAN_POINT('Ctrl Pts',(-10.6658348983944,-72.6260262228055,
0.));
#69963=CARTESIAN_POINT('Ctrl Pts',(-10.6658348983944,-72.6260262228055,
12.));
#69964=CARTESIAN_POINT('Ctrl Pts',(-10.659221996058,-72.6516055286908,0.));
#69965=CARTESIAN_POINT('Ctrl Pts',(-10.659221996058,-72.6516055286908,12.));
#69966=CARTESIAN_POINT('Ctrl Pts',(-10.6525760396055,-72.6772147534762,
0.));
#69967=CARTESIAN_POINT('Ctrl Pts',(-10.6525760396055,-72.6772147534762,
12.));
#69968=CARTESIAN_POINT('Ctrl Pts',(-10.6458970045948,-72.7028537934332,
0.));
#69969=CARTESIAN_POINT('Ctrl Pts',(-10.6458970045948,-72.7028537934332,
12.));
#69970=CARTESIAN_POINT('Ctrl Pts',(-10.6391848667354,-72.7285225451309,
0.));
#69971=CARTESIAN_POINT('Ctrl Pts',(-10.6391848667354,-72.7285225451309,
12.));
#69972=CARTESIAN_POINT('Ctrl Pts',(-10.6324396018999,-72.7542209054823,
0.));
#69973=CARTESIAN_POINT('Ctrl Pts',(-10.6324396018999,-72.7542209054823,
12.));
#69974=CARTESIAN_POINT('Ctrl Pts',(-10.6256611861395,-72.7799487717914,
0.));
#69975=CARTESIAN_POINT('Ctrl Pts',(-10.6256611861395,-72.7799487717914,
12.));
#69976=CARTESIAN_POINT('Ctrl Pts',(-10.6188495956973,-72.8057060417882,
0.));
#69977=CARTESIAN_POINT('Ctrl Pts',(-10.6188495956973,-72.8057060417882,
12.));
#69978=CARTESIAN_POINT('Ctrl Pts',(-10.6120048070366,-72.8314926136872,
0.));
#69979=CARTESIAN_POINT('Ctrl Pts',(-10.6120048070366,-72.8314926136872,
12.));
#69980=CARTESIAN_POINT('Ctrl Pts',(-10.6051267968202,-72.8573083861328,
0.));
#69981=CARTESIAN_POINT('Ctrl Pts',(-10.6051267968202,-72.8573083861328,
12.));
#69982=CARTESIAN_POINT('Ctrl Pts',(-10.5982155418625,-72.8831532580839,
0.));
#69983=CARTESIAN_POINT('Ctrl Pts',(-10.5982155418625,-72.8831532580839,
12.));
#69984=CARTESIAN_POINT('Ctrl Pts',(-10.5912710190928,-72.9090271287081,
0.));
#69985=CARTESIAN_POINT('Ctrl Pts',(-10.5912710190928,-72.9090271287081,
12.));
#69986=CARTESIAN_POINT('Ctrl Pts',(-10.5842932055209,-72.9349298972823,
0.));
#69987=CARTESIAN_POINT('Ctrl Pts',(-10.5842932055209,-72.9349298972823,
12.));
#69988=CARTESIAN_POINT('Ctrl Pts',(-10.5772820781959,-72.9608614630539,
0.));
#69989=CARTESIAN_POINT('Ctrl Pts',(-10.5772820781959,-72.9608614630539,
12.));
#69990=CARTESIAN_POINT('Ctrl Pts',(-10.5702376142052,-72.9868217252293,
0.));
#69991=CARTESIAN_POINT('Ctrl Pts',(-10.5702376142052,-72.9868217252293,
12.));
#69992=CARTESIAN_POINT('Ctrl Pts',(-10.5631597907653,-73.0128105832635,
0.));
#69993=CARTESIAN_POINT('Ctrl Pts',(-10.5631597907653,-73.0128105832635,
12.));
#69994=CARTESIAN_POINT('Ctrl Pts',(-10.5560485852975,-73.0388279370845,
0.));
#69995=CARTESIAN_POINT('Ctrl Pts',(-10.5560485852975,-73.0388279370845,
12.));
#69996=CARTESIAN_POINT('Ctrl Pts',(-10.5489039755138,-73.0648736873435,
0.));
#69997=CARTESIAN_POINT('Ctrl Pts',(-10.5489039755138,-73.0648736873435,
12.));
#69998=CARTESIAN_POINT('Ctrl Pts',(-10.5417259395001,-73.090947735646,0.));
#69999=CARTESIAN_POINT('Ctrl Pts',(-10.5417259395001,-73.090947735646,12.));
#70000=CARTESIAN_POINT('Ctrl Pts',(-10.5345144558097,-73.1170499848012,
0.));
#70001=CARTESIAN_POINT('Ctrl Pts',(-10.5345144558097,-73.1170499848012,
12.));
#70002=CARTESIAN_POINT('Ctrl Pts',(-10.5272695032649,-73.1431803382677,
0.));
#70003=CARTESIAN_POINT('Ctrl Pts',(-10.5272695032649,-73.1431803382677,
12.));
#70004=CARTESIAN_POINT('Ctrl Pts',(-10.5199910607652,-73.169338699611,0.));
#70005=CARTESIAN_POINT('Ctrl Pts',(-10.5199910607652,-73.169338699611,12.));
#70006=CARTESIAN_POINT('Ctrl Pts',(-10.5126791070804,-73.1955249719037,
0.));
#70007=CARTESIAN_POINT('Ctrl Pts',(-10.5126791070804,-73.1955249719037,
12.));
#70008=CARTESIAN_POINT('Ctrl Pts',(-10.505333620691,-73.2217390572578,0.));
#70009=CARTESIAN_POINT('Ctrl Pts',(-10.505333620691,-73.2217390572578,12.));
#70010=CARTESIAN_POINT('Ctrl Pts',(-10.4979545795197,-73.247980856023,0.));
#70011=CARTESIAN_POINT('Ctrl Pts',(-10.4979545795197,-73.247980856023,12.));
#70012=CARTESIAN_POINT('Ctrl Pts',(-10.4905419611529,-73.2742502674361,
0.));
#70013=CARTESIAN_POINT('Ctrl Pts',(-10.4905419611529,-73.2742502674361,
12.));
#70014=CARTESIAN_POINT('Ctrl Pts',(-10.4830957433311,-73.3005471910639,
0.));
#70015=CARTESIAN_POINT('Ctrl Pts',(-10.4830957433311,-73.3005471910639,
12.));
#70016=CARTESIAN_POINT('Ctrl Pts',(-10.475615904381,-73.3268715280609,0.));
#70017=CARTESIAN_POINT('Ctrl Pts',(-10.475615904381,-73.3268715280609,12.));
#70018=CARTESIAN_POINT('Ctrl Pts',(-10.4681024236288,-73.353223182365,0.));
#70019=CARTESIAN_POINT('Ctrl Pts',(-10.4681024236288,-73.353223182365,12.));
#70020=CARTESIAN_POINT('Ctrl Pts',(-10.460555281939,-73.3796020622437,0.));
#70021=CARTESIAN_POINT('Ctrl Pts',(-10.460555281939,-73.3796020622437,12.));
#70022=CARTESIAN_POINT('Ctrl Pts',(-10.4529744618438,-73.4060080806577,
0.));
#70023=CARTESIAN_POINT('Ctrl Pts',(-10.4529744618438,-73.4060080806577,
12.));
#70024=CARTESIAN_POINT('Ctrl Pts',(-10.4453599463534,-73.432441151843,0.));
#70025=CARTESIAN_POINT('Ctrl Pts',(-10.4453599463534,-73.432441151843,12.));
#70026=CARTESIAN_POINT('Ctrl Pts',(-10.4377117180212,-73.45890118861,0.));
#70027=CARTESIAN_POINT('Ctrl Pts',(-10.4377117180212,-73.45890118861,12.));
#70028=CARTESIAN_POINT('Ctrl Pts',(-10.4300297578648,-73.4853880992228,
0.));
#70029=CARTESIAN_POINT('Ctrl Pts',(-10.4300297578648,-73.4853880992228,
12.));
#70030=CARTESIAN_POINT('Ctrl Pts',(-10.4223140444615,-73.5119017847664,
0.));
#70031=CARTESIAN_POINT('Ctrl Pts',(-10.4223140444615,-73.5119017847664,
12.));
#70032=CARTESIAN_POINT('Ctrl Pts',(-10.4145645526831,-73.5384421354746,
0.));
#70033=CARTESIAN_POINT('Ctrl Pts',(-10.4145645526831,-73.5384421354746,
12.));
#70034=CARTESIAN_POINT('Ctrl Pts',(-10.4067812555539,-73.5650090360114,
0.));
#70035=CARTESIAN_POINT('Ctrl Pts',(-10.4067812555539,-73.5650090360114,
12.));
#70036=CARTESIAN_POINT('Ctrl Pts',(-10.3989641265313,-73.5916023719976,
0.));
#70037=CARTESIAN_POINT('Ctrl Pts',(-10.3989641265313,-73.5916023719976,
12.));
#70038=CARTESIAN_POINT('Ctrl Pts',(-10.3911131417478,-73.6182220363295,
0.));
#70039=CARTESIAN_POINT('Ctrl Pts',(-10.3911131417478,-73.6182220363295,
12.));
#70040=CARTESIAN_POINT('Ctrl Pts',(-10.3832282820361,-73.6448679350605,
0.));
#70041=CARTESIAN_POINT('Ctrl Pts',(-10.3832282820361,-73.6448679350605,
12.));
#70042=CARTESIAN_POINT('Ctrl Pts',(-10.3753095356302,-73.6715399947459,
0.));
#70043=CARTESIAN_POINT('Ctrl Pts',(-10.3753095356302,-73.6715399947459,
12.));
#70044=CARTESIAN_POINT('Ctrl Pts',(-10.3673568984515,-73.6982381644571,
0.));
#70045=CARTESIAN_POINT('Ctrl Pts',(-10.3673568984515,-73.6982381644571,
12.));
#70046=CARTESIAN_POINT('Ctrl Pts',(-10.3593703712542,-73.7249624108433,
0.));
#70047=CARTESIAN_POINT('Ctrl Pts',(-10.3593703712542,-73.7249624108433,
12.));
#70048=CARTESIAN_POINT('Ctrl Pts',(-10.3529540403026,-73.7463626541235,
0.));
#70049=CARTESIAN_POINT('Ctrl Pts',(-10.3529540403026,-73.7463626541235,
12.));
#70050=CARTESIAN_POINT('Ctrl Pts',(-10.3481265449303,-73.7624245587416,
0.));
#70051=CARTESIAN_POINT('Ctrl Pts',(-10.3481265449303,-73.7624245587416,
12.));
#70052=CARTESIAN_POINT('Ctrl Pts',(-10.3449014384438,-73.7731377047922,
0.));
#70053=CARTESIAN_POINT('Ctrl Pts',(-10.3449014384438,-73.7731377047922,
12.));
#70054=CARTESIAN_POINT('Ctrl Pts',(-10.343287191141,-73.778495580227,0.));
#70055=CARTESIAN_POINT('Ctrl Pts',(-10.343287191141,-73.778495580227,12.));
#70056=CARTESIAN_POINT('',(-11.3136138754165,-69.079679653846,0.));
#70057=CARTESIAN_POINT('Ctrl Pts',(-11.3136138754165,-69.079679653846,0.));
#70058=CARTESIAN_POINT('Ctrl Pts',(-11.3132375200165,-69.0835449954396,
0.));
#70059=CARTESIAN_POINT('Ctrl Pts',(-11.3124821678798,-69.0912808656811,
0.));
#70060=CARTESIAN_POINT('Ctrl Pts',(-11.3113412156661,-69.1029002322118,
0.));
#70061=CARTESIAN_POINT('Ctrl Pts',(-11.3098040973713,-69.118423844466,0.));
#70062=CARTESIAN_POINT('Ctrl Pts',(-11.3078562764384,-69.1378802251711,
0.));
#70063=CARTESIAN_POINT('Ctrl Pts',(-11.3058820128307,-69.1573884361,0.));
#70064=CARTESIAN_POINT('Ctrl Pts',(-11.3038812726292,-69.1769483991721,
0.));
#70065=CARTESIAN_POINT('Ctrl Pts',(-11.3018540025638,-69.1965599718914,
0.));
#70066=CARTESIAN_POINT('Ctrl Pts',(-11.2998001310964,-69.2162229488531,
0.));
#70067=CARTESIAN_POINT('Ctrl Pts',(-11.2977195764852,-69.2359370894907,
0.));
#70068=CARTESIAN_POINT('Ctrl Pts',(-11.2956122531375,-69.255702139335,0.));
#70069=CARTESIAN_POINT('Ctrl Pts',(-11.2934780784351,-69.275517853148,0.));
#70070=CARTESIAN_POINT('Ctrl Pts',(-11.2913169799628,-69.295384019272,0.));
#70071=CARTESIAN_POINT('Ctrl Pts',(-11.2891288931517,-69.3153004517783,
0.));
#70072=CARTESIAN_POINT('Ctrl Pts',(-11.2869137578459,-69.3352669789587,
0.));
#70073=CARTESIAN_POINT('Ctrl Pts',(-11.2846715154524,-69.3552834337784,
0.));
#70074=CARTESIAN_POINT('Ctrl Pts',(-11.2824021054045,-69.3753496420039,
0.));
#70075=CARTESIAN_POINT('Ctrl Pts',(-11.2801054633815,-69.3954654162281,
0.));
#70076=CARTESIAN_POINT('Ctrl Pts',(-11.2777815231469,-69.4156305620593,
0.));
#70077=CARTESIAN_POINT('Ctrl Pts',(-11.2754302177021,-69.4358448819967,
0.));
#70078=CARTESIAN_POINT('Ctrl Pts',(-11.2730514806139,-69.456108179879,0.));
#70079=CARTESIAN_POINT('Ctrl Pts',(-11.270645247528,-69.4764202659397,0.));
#70080=CARTESIAN_POINT('Ctrl Pts',(-11.2682114561007,-69.4967809565929,
0.));
#70081=CARTESIAN_POINT('Ctrl Pts',(-11.2657500452716,-69.5171900720158,
0.));
#70082=CARTESIAN_POINT('Ctrl Pts',(-11.263260954763,-69.5376474344771,0.));
#70083=CARTESIAN_POINT('Ctrl Pts',(-11.2607441244702,-69.5581528662877,
0.));
#70084=CARTESIAN_POINT('Ctrl Pts',(-11.2581994939541,-69.5787061880857,
0.));
#70085=CARTESIAN_POINT('Ctrl Pts',(-11.2556270027016,-69.599307219739,0.));
#70086=CARTESIAN_POINT('Ctrl Pts',(-11.2530265903557,-69.6199557811245,
0.));
#70087=CARTESIAN_POINT('Ctrl Pts',(-11.2503981969412,-69.6406516928891,
0.));
#70088=CARTESIAN_POINT('Ctrl Pts',(-11.2477417631386,-69.6613947773534,
0.));
#70089=CARTESIAN_POINT('Ctrl Pts',(-11.2450572303841,-69.6821848588457,
0.));
#70090=CARTESIAN_POINT('Ctrl Pts',(-11.2423445407166,-69.7030217632164,
0.));
#70091=CARTESIAN_POINT('Ctrl Pts',(-11.239603636686,-69.7239053175356,0.));
#70092=CARTESIAN_POINT('Ctrl Pts',(-11.2368344612472,-69.7448353497408,
0.));
#70093=CARTESIAN_POINT('Ctrl Pts',(-11.2340369576456,-69.7658116882324,
0.));
#70094=CARTESIAN_POINT('Ctrl Pts',(-11.2312110694187,-69.7868341618954,
0.));
#70095=CARTESIAN_POINT('Ctrl Pts',(-11.2283567404437,-69.8079026002768,
0.));
#70096=CARTESIAN_POINT('Ctrl Pts',(-11.225473914972,-69.8290168337076,0.));
#70097=CARTESIAN_POINT('Ctrl Pts',(-11.2225625376736,-69.8501766934428,
0.));
#70098=CARTESIAN_POINT('Ctrl Pts',(-11.219622553679,-69.871382011789,0.));
#70099=CARTESIAN_POINT('Ctrl Pts',(-11.2166539085523,-69.8926326220385,
0.));
#70100=CARTESIAN_POINT('Ctrl Pts',(-11.2136565482677,-69.9139283584022,
0.));
#70101=CARTESIAN_POINT('Ctrl Pts',(-11.2106304191882,-69.9352690559405,
0.));
#70102=CARTESIAN_POINT('Ctrl Pts',(-11.2075754680449,-69.9566545504837,
0.));
#70103=CARTESIAN_POINT('Ctrl Pts',(-11.2044916419244,-69.97808467858,0.));
#70104=CARTESIAN_POINT('Ctrl Pts',(-11.2013788882714,-69.9995592775343,
0.));
#70105=CARTESIAN_POINT('Ctrl Pts',(-11.1982371548919,-70.0210781854243,
0.));
#70106=CARTESIAN_POINT('Ctrl Pts',(-11.1950663899576,-70.0426412411185,
0.));
#70107=CARTESIAN_POINT('Ctrl Pts',(-11.1918665420166,-70.0642482842928,
0.));
#70108=CARTESIAN_POINT('Ctrl Pts',(-11.1886375599914,-70.0858991554283,
0.));
#70109=CARTESIAN_POINT('Ctrl Pts',(-11.185379393167,-70.1075936957968,0.));
#70110=CARTESIAN_POINT('Ctrl Pts',(-11.1820919911846,-70.1293317474432,
0.));
#70111=CARTESIAN_POINT('Ctrl Pts',(-11.1787753040363,-70.1511131531674,
0.));
#70112=CARTESIAN_POINT('Ctrl Pts',(-11.1754292820631,-70.1729377564956,
0.));
#70113=CARTESIAN_POINT('Ctrl Pts',(-11.1720538759498,-70.1948054016817,
0.));
#70114=CARTESIAN_POINT('Ctrl Pts',(-11.168649036721,-70.2167159337095,0.));
#70115=CARTESIAN_POINT('Ctrl Pts',(-11.1652147157383,-70.2386691982902,
0.));
#70116=CARTESIAN_POINT('Ctrl Pts',(-11.1617508647017,-70.2606650418589,
0.));
#70117=CARTESIAN_POINT('Ctrl Pts',(-11.1582574356522,-70.2827033115662,
0.));
#70118=CARTESIAN_POINT('Ctrl Pts',(-11.1547343809647,-70.3047838552758,
0.));
#70119=CARTESIAN_POINT('Ctrl Pts',(-11.1511816533422,-70.3269065215591,
0.));
#70120=CARTESIAN_POINT('Ctrl Pts',(-11.1475992058124,-70.3490711596882,
0.));
#70121=CARTESIAN_POINT('Ctrl Pts',(-11.1439869917269,-70.3712776196216,
0.));
#70122=CARTESIAN_POINT('Ctrl Pts',(-11.1403449647622,-70.3935257519945,
0.));
#70123=CARTESIAN_POINT('Ctrl Pts',(-11.1366730789122,-70.415815408119,0.));
#70124=CARTESIAN_POINT('Ctrl Pts',(-11.1329712884845,-70.438146439981,0.));
#70125=CARTESIAN_POINT('Ctrl Pts',(-11.1292395480975,-70.4605187002356,
0.));
#70126=CARTESIAN_POINT('Ctrl Pts',(-11.1254778126824,-70.4829320421973,
0.));
#70127=CARTESIAN_POINT('Ctrl Pts',(-11.121686037483,-70.5053863198306,0.));
#70128=CARTESIAN_POINT('Ctrl Pts',(-11.117864178048,-70.5278813877519,0.));
#70129=CARTESIAN_POINT('Ctrl Pts',(-11.1140121902274,-70.5504171012247,
0.));
#70130=CARTESIAN_POINT('Ctrl Pts',(-11.11013003017,-70.5729933161538,0.));
#70131=CARTESIAN_POINT('Ctrl Pts',(-11.1062176543257,-70.5956098890744,
0.));
#70132=CARTESIAN_POINT('Ctrl Pts',(-11.1022750194439,-70.6182666771441,
0.));
#70133=CARTESIAN_POINT('Ctrl Pts',(-11.0983020825662,-70.6409635381446,
0.));
#70134=CARTESIAN_POINT('Ctrl Pts',(-11.0942988010231,-70.6637003304768,
0.));
#70135=CARTESIAN_POINT('Ctrl Pts',(-11.0902651324325,-70.686476913156,0.));
#70136=CARTESIAN_POINT('Ctrl Pts',(-11.0862010347022,-70.7092931457996,
0.));
#70137=CARTESIAN_POINT('Ctrl Pts',(-11.0821064660276,-70.7321488886229,
0.));
#70138=CARTESIAN_POINT('Ctrl Pts',(-11.0779813848851,-70.7550440024422,
0.));
#70139=CARTESIAN_POINT('Ctrl Pts',(-11.0738257500292,-70.7779783486689,
0.));
#70140=CARTESIAN_POINT('Ctrl Pts',(-11.0696395204907,-70.8009517893042,
0.));
#70141=CARTESIAN_POINT('Ctrl Pts',(-11.0654226555798,-70.8239641869266,
0.));
#70142=CARTESIAN_POINT('Ctrl Pts',(-11.061175114883,-70.847015404688,0.));
#70143=CARTESIAN_POINT('Ctrl Pts',(-11.0568968582566,-70.8701053063158,
0.));
#70144=CARTESIAN_POINT('Ctrl Pts',(-11.0525878458242,-70.8932337561078,
0.));
#70145=CARTESIAN_POINT('Ctrl Pts',(-11.0482480379752,-70.9164006189283,
0.));
#70146=CARTESIAN_POINT('Ctrl Pts',(-11.0438773953686,-70.9396057601953,
0.));
#70147=CARTESIAN_POINT('Ctrl Pts',(-11.039475878929,-70.9628490458779,0.));
#70148=CARTESIAN_POINT('Ctrl Pts',(-11.0350434498408,-70.9861303424989,
0.));
#70149=CARTESIAN_POINT('Ctrl Pts',(-11.0305800695457,-71.0094495171295,
0.));
#70150=CARTESIAN_POINT('Ctrl Pts',(-11.0260856997414,-71.0328064373849,
0.));
#70151=CARTESIAN_POINT('Ctrl Pts',(-11.0215603023854,-71.0562009714125,
0.));
#70152=CARTESIAN_POINT('Ctrl Pts',(-11.0170038396913,-71.0796329878896,
0.));
#70153=CARTESIAN_POINT('Ctrl Pts',(-11.0124162741223,-71.1031023560243,
0.));
#70154=CARTESIAN_POINT('Ctrl Pts',(-11.0077975683895,-71.1266089455517,
0.));
#70155=CARTESIAN_POINT('Ctrl Pts',(-11.0031476854503,-71.1501526267288,
0.));
#70156=CARTESIAN_POINT('Ctrl Pts',(-10.9984665885127,-71.1737332703248,
0.));
#70157=CARTESIAN_POINT('Ctrl Pts',(-10.993754241032,-71.1973507476188,0.));
#70158=CARTESIAN_POINT('Ctrl Pts',(-10.9890106067038,-71.221004930401,0.));
#70159=CARTESIAN_POINT('Ctrl Pts',(-10.9842356494627,-71.2446956909685,
0.));
#70160=CARTESIAN_POINT('Ctrl Pts',(-10.9794293334806,-71.2684229021209,
0.));
#70161=CARTESIAN_POINT('Ctrl Pts',(-10.9745916231711,-71.2921864371499,
0.));
#70162=CARTESIAN_POINT('Ctrl Pts',(-10.9697224831862,-71.3159861698368,
0.));
#70163=CARTESIAN_POINT('Ctrl Pts',(-10.96482187841,-71.3398219744547,0.));
#70164=CARTESIAN_POINT('Ctrl Pts',(-10.9598897739565,-71.3636937257651,
0.));
#70165=CARTESIAN_POINT('Ctrl Pts',(-10.9549261351689,-71.3876012990135,
0.));
#70166=CARTESIAN_POINT('Ctrl Pts',(-10.9499309276235,-71.411544569919,0.));
#70167=CARTESIAN_POINT('Ctrl Pts',(-10.9449041171269,-71.4355234146718,
0.));
#70168=CARTESIAN_POINT('Ctrl Pts',(-10.9398456697094,-71.4595377099352,
0.));
#70169=CARTESIAN_POINT('Ctrl Pts',(-10.9347555516236,-71.4835873328425,
0.));
#70170=CARTESIAN_POINT('Ctrl Pts',(-10.9296337293425,-71.5076721609936,
0.));
#70171=CARTESIAN_POINT('Ctrl Pts',(-10.9244801695642,-71.5317920724453,
0.));
#70172=CARTESIAN_POINT('Ctrl Pts',(-10.9192948392099,-71.5559469457082,
0.));
#70173=CARTESIAN_POINT('Ctrl Pts',(-10.9140777054169,-71.5801366597479,
0.));
#70174=CARTESIAN_POINT('Ctrl Pts',(-10.9088287355364,-71.604361093983,0.));
#70175=CARTESIAN_POINT('Ctrl Pts',(-10.9035478971329,-71.6286201282815,
0.));
#70176=CARTESIAN_POINT('Ctrl Pts',(-10.8982351579872,-71.6529136429515,
0.));
#70177=CARTESIAN_POINT('Ctrl Pts',(-10.8928904860967,-71.6772415187382,
0.));
#70178=CARTESIAN_POINT('Ctrl Pts',(-10.8875138496674,-71.7016036368254,
0.));
#70179=CARTESIAN_POINT('Ctrl Pts',(-10.8821052171122,-71.7259998788337,
0.));
#70180=CARTESIAN_POINT('Ctrl Pts',(-10.8766645570496,-71.7504301268177,
0.));
#70181=CARTESIAN_POINT('Ctrl Pts',(-10.8711918383071,-71.7748942632578,
0.));
#70182=CARTESIAN_POINT('Ctrl Pts',(-10.8656870299218,-71.7993921710546,
0.));
#70183=CARTESIAN_POINT('Ctrl Pts',(-10.860150101133,-71.8239237335318,0.));
#70184=CARTESIAN_POINT('Ctrl Pts',(-10.8545810213799,-71.8484888344335,
0.));
#70185=CARTESIAN_POINT('Ctrl Pts',(-10.8489797602998,-71.8730873579226,
0.));
#70186=CARTESIAN_POINT('Ctrl Pts',(-10.8433462877312,-71.8977191885726,
0.));
#70187=CARTESIAN_POINT('Ctrl Pts',(-10.8376805737158,-71.9223842113622,
0.));
#70188=CARTESIAN_POINT('Ctrl Pts',(-10.8319825884917,-71.9470823116777,
0.));
#70189=CARTESIAN_POINT('Ctrl Pts',(-10.8262523024897,-71.971813375312,0.));
#70190=CARTESIAN_POINT('Ctrl Pts',(-10.8204896863328,-71.9965772884619,
0.));
#70191=CARTESIAN_POINT('Ctrl Pts',(-10.8146947108376,-72.0213739377231,
0.));
#70192=CARTESIAN_POINT('Ctrl Pts',(-10.8088673470187,-72.0462032100828,
0.));
#70193=CARTESIAN_POINT('Ctrl Pts',(-10.8030075660811,-72.0710649929214,
0.));
#70194=CARTESIAN_POINT('Ctrl Pts',(-10.7971153394168,-72.095959174012,0.));
#70195=CARTESIAN_POINT('Ctrl Pts',(-10.7911906386027,-72.1208856415171,
0.));
#70196=CARTESIAN_POINT('Ctrl Pts',(-10.7852334354015,-72.145844283983,0.));
#70197=CARTESIAN_POINT('Ctrl Pts',(-10.779243701766,-72.17083499033,0.));
#70198=CARTESIAN_POINT('Ctrl Pts',(-10.7732214098343,-72.1958576498556,
0.));
#70199=CARTESIAN_POINT('Ctrl Pts',(-10.7671665319254,-72.2209121522367,
0.));
#70200=CARTESIAN_POINT('Ctrl Pts',(-10.7610790405385,-72.2459983875298,
0.));
#70201=CARTESIAN_POINT('Ctrl Pts',(-10.7549589083535,-72.2711162461679,
0.));
#70202=CARTESIAN_POINT('Ctrl Pts',(-10.7488061082368,-72.296265618955,0.));
#70203=CARTESIAN_POINT('Ctrl Pts',(-10.7426206132375,-72.3214463970634,
0.));
#70204=CARTESIAN_POINT('Ctrl Pts',(-10.73640239658,-72.3466584720311,0.));
#70205=CARTESIAN_POINT('Ctrl Pts',(-10.7301514316607,-72.3719017357568,
0.));
#70206=CARTESIAN_POINT('Ctrl Pts',(-10.7238676920469,-72.3971760804935,
0.));
#70207=CARTESIAN_POINT('Ctrl Pts',(-10.7175511514789,-72.4224813988355,
0.));
#70208=CARTESIAN_POINT('Ctrl Pts',(-10.7112017838707,-72.4478175837168,
0.));
#70209=CARTESIAN_POINT('Ctrl Pts',(-10.7048195633062,-72.4731845284238,
0.));
#70210=CARTESIAN_POINT('Ctrl Pts',(-10.6984044640399,-72.4985821266031,
0.));
#70211=CARTESIAN_POINT('Ctrl Pts',(-10.691956460499,-72.5240102722662,0.));
#70212=CARTESIAN_POINT('Ctrl Pts',(-10.6854755272903,-72.5494688597951,
0.));
#70213=CARTESIAN_POINT('Ctrl Pts',(-10.6789616392041,-72.57495778394,0.));
#70214=CARTESIAN_POINT('Ctrl Pts',(-10.6724147711994,-72.6004769398004,
0.));
#70215=CARTESIAN_POINT('Ctrl Pts',(-10.6658348983944,-72.6260262228055,
0.));
#70216=CARTESIAN_POINT('Ctrl Pts',(-10.659221996058,-72.6516055286908,0.));
#70217=CARTESIAN_POINT('Ctrl Pts',(-10.6525760396055,-72.6772147534762,
0.));
#70218=CARTESIAN_POINT('Ctrl Pts',(-10.6458970045948,-72.7028537934332,
0.));
#70219=CARTESIAN_POINT('Ctrl Pts',(-10.6391848667354,-72.7285225451309,
0.));
#70220=CARTESIAN_POINT('Ctrl Pts',(-10.6324396018999,-72.7542209054823,
0.));
#70221=CARTESIAN_POINT('Ctrl Pts',(-10.6256611861395,-72.7799487717914,
0.));
#70222=CARTESIAN_POINT('Ctrl Pts',(-10.6188495956973,-72.8057060417882,
0.));
#70223=CARTESIAN_POINT('Ctrl Pts',(-10.6120048070366,-72.8314926136872,
0.));
#70224=CARTESIAN_POINT('Ctrl Pts',(-10.6051267968202,-72.8573083861328,
0.));
#70225=CARTESIAN_POINT('Ctrl Pts',(-10.5982155418625,-72.8831532580839,
0.));
#70226=CARTESIAN_POINT('Ctrl Pts',(-10.5912710190928,-72.9090271287081,
0.));
#70227=CARTESIAN_POINT('Ctrl Pts',(-10.5842932055209,-72.9349298972823,
0.));
#70228=CARTESIAN_POINT('Ctrl Pts',(-10.5772820781959,-72.9608614630539,
0.));
#70229=CARTESIAN_POINT('Ctrl Pts',(-10.5702376142052,-72.9868217252293,
0.));
#70230=CARTESIAN_POINT('Ctrl Pts',(-10.5631597907653,-73.0128105832635,
0.));
#70231=CARTESIAN_POINT('Ctrl Pts',(-10.5560485852975,-73.0388279370845,
0.));
#70232=CARTESIAN_POINT('Ctrl Pts',(-10.5489039755138,-73.0648736873435,
0.));
#70233=CARTESIAN_POINT('Ctrl Pts',(-10.5417259395001,-73.090947735646,0.));
#70234=CARTESIAN_POINT('Ctrl Pts',(-10.5345144558097,-73.1170499848012,
0.));
#70235=CARTESIAN_POINT('Ctrl Pts',(-10.5272695032649,-73.1431803382677,
0.));
#70236=CARTESIAN_POINT('Ctrl Pts',(-10.5199910607652,-73.169338699611,0.));
#70237=CARTESIAN_POINT('Ctrl Pts',(-10.5126791070804,-73.1955249719037,
0.));
#70238=CARTESIAN_POINT('Ctrl Pts',(-10.505333620691,-73.2217390572578,0.));
#70239=CARTESIAN_POINT('Ctrl Pts',(-10.4979545795197,-73.247980856023,0.));
#70240=CARTESIAN_POINT('Ctrl Pts',(-10.4905419611529,-73.2742502674361,
0.));
#70241=CARTESIAN_POINT('Ctrl Pts',(-10.4830957433311,-73.3005471910639,
0.));
#70242=CARTESIAN_POINT('Ctrl Pts',(-10.475615904381,-73.3268715280609,0.));
#70243=CARTESIAN_POINT('Ctrl Pts',(-10.4681024236288,-73.353223182365,0.));
#70244=CARTESIAN_POINT('Ctrl Pts',(-10.460555281939,-73.3796020622437,0.));
#70245=CARTESIAN_POINT('Ctrl Pts',(-10.4529744618438,-73.4060080806577,
0.));
#70246=CARTESIAN_POINT('Ctrl Pts',(-10.4464473465486,-73.4286663447915,
0.));
#70247=CARTESIAN_POINT('Ctrl Pts',(-10.4414249334768,-73.4460525528551,
0.));
#70248=CARTESIAN_POINT('Ctrl Pts',(-10.4379221501093,-73.458154743654,0.));
#70249=CARTESIAN_POINT('Ctrl Pts',(-10.4359488742883,-73.464965036154,0.));
#70250=CARTESIAN_POINT('Ctrl Pts',(-10.4355099267391,-73.4664795929519,
0.));
#70251=CARTESIAN_POINT('',(-11.3136138754165,-69.079679653846,12.));
#70252=CARTESIAN_POINT('',(-11.3136138754165,-69.079679653846,0.));
#70253=CARTESIAN_POINT('Ctrl Pts',(-10.4355099267391,-73.4664795929519,
12.));
#70254=CARTESIAN_POINT('Ctrl Pts',(-10.4359488742883,-73.464965036154,12.));
#70255=CARTESIAN_POINT('Ctrl Pts',(-10.4379221501093,-73.458154743654,12.));
#70256=CARTESIAN_POINT('Ctrl Pts',(-10.4414249334768,-73.4460525528551,
12.));
#70257=CARTESIAN_POINT('Ctrl Pts',(-10.4464473465486,-73.4286663447915,
12.));
#70258=CARTESIAN_POINT('Ctrl Pts',(-10.4529744618438,-73.4060080806577,
12.));
#70259=CARTESIAN_POINT('Ctrl Pts',(-10.460555281939,-73.3796020622437,12.));
#70260=CARTESIAN_POINT('Ctrl Pts',(-10.4681024236288,-73.353223182365,12.));
#70261=CARTESIAN_POINT('Ctrl Pts',(-10.475615904381,-73.3268715280609,12.));
#70262=CARTESIAN_POINT('Ctrl Pts',(-10.4830957433311,-73.3005471910639,
12.));
#70263=CARTESIAN_POINT('Ctrl Pts',(-10.4905419611529,-73.2742502674361,
12.));
#70264=CARTESIAN_POINT('Ctrl Pts',(-10.4979545795197,-73.247980856023,12.));
#70265=CARTESIAN_POINT('Ctrl Pts',(-10.505333620691,-73.2217390572578,12.));
#70266=CARTESIAN_POINT('Ctrl Pts',(-10.5126791070804,-73.1955249719037,
12.));
#70267=CARTESIAN_POINT('Ctrl Pts',(-10.5199910607652,-73.169338699611,12.));
#70268=CARTESIAN_POINT('Ctrl Pts',(-10.5272695032649,-73.1431803382677,
12.));
#70269=CARTESIAN_POINT('Ctrl Pts',(-10.5345144558097,-73.1170499848012,
12.));
#70270=CARTESIAN_POINT('Ctrl Pts',(-10.5417259395001,-73.090947735646,12.));
#70271=CARTESIAN_POINT('Ctrl Pts',(-10.5489039755138,-73.0648736873435,
12.));
#70272=CARTESIAN_POINT('Ctrl Pts',(-10.5560485852975,-73.0388279370845,
12.));
#70273=CARTESIAN_POINT('Ctrl Pts',(-10.5631597907653,-73.0128105832635,
12.));
#70274=CARTESIAN_POINT('Ctrl Pts',(-10.5702376142052,-72.9868217252293,
12.));
#70275=CARTESIAN_POINT('Ctrl Pts',(-10.5772820781959,-72.9608614630539,
12.));
#70276=CARTESIAN_POINT('Ctrl Pts',(-10.5842932055209,-72.9349298972823,
12.));
#70277=CARTESIAN_POINT('Ctrl Pts',(-10.5912710190928,-72.9090271287081,
12.));
#70278=CARTESIAN_POINT('Ctrl Pts',(-10.5982155418625,-72.8831532580839,
12.));
#70279=CARTESIAN_POINT('Ctrl Pts',(-10.6051267968202,-72.8573083861328,
12.));
#70280=CARTESIAN_POINT('Ctrl Pts',(-10.6120048070366,-72.8314926136872,
12.));
#70281=CARTESIAN_POINT('Ctrl Pts',(-10.6188495956973,-72.8057060417882,
12.));
#70282=CARTESIAN_POINT('Ctrl Pts',(-10.6256611861395,-72.7799487717914,
12.));
#70283=CARTESIAN_POINT('Ctrl Pts',(-10.6324396018999,-72.7542209054823,
12.));
#70284=CARTESIAN_POINT('Ctrl Pts',(-10.6391848667354,-72.7285225451309,
12.));
#70285=CARTESIAN_POINT('Ctrl Pts',(-10.6458970045948,-72.7028537934332,
12.));
#70286=CARTESIAN_POINT('Ctrl Pts',(-10.6525760396055,-72.6772147534762,
12.));
#70287=CARTESIAN_POINT('Ctrl Pts',(-10.659221996058,-72.6516055286908,12.));
#70288=CARTESIAN_POINT('Ctrl Pts',(-10.6658348983944,-72.6260262228055,
12.));
#70289=CARTESIAN_POINT('Ctrl Pts',(-10.6724147711994,-72.6004769398004,
12.));
#70290=CARTESIAN_POINT('Ctrl Pts',(-10.6789616392041,-72.57495778394,12.));
#70291=CARTESIAN_POINT('Ctrl Pts',(-10.6854755272903,-72.5494688597951,
12.));
#70292=CARTESIAN_POINT('Ctrl Pts',(-10.691956460499,-72.5240102722662,12.));
#70293=CARTESIAN_POINT('Ctrl Pts',(-10.6984044640399,-72.4985821266031,
12.));
#70294=CARTESIAN_POINT('Ctrl Pts',(-10.7048195633062,-72.4731845284238,
12.));
#70295=CARTESIAN_POINT('Ctrl Pts',(-10.7112017838707,-72.4478175837168,
12.));
#70296=CARTESIAN_POINT('Ctrl Pts',(-10.7175511514789,-72.4224813988355,
12.));
#70297=CARTESIAN_POINT('Ctrl Pts',(-10.7238676920469,-72.3971760804935,
12.));
#70298=CARTESIAN_POINT('Ctrl Pts',(-10.7301514316607,-72.3719017357568,
12.));
#70299=CARTESIAN_POINT('Ctrl Pts',(-10.73640239658,-72.3466584720311,12.));
#70300=CARTESIAN_POINT('Ctrl Pts',(-10.7426206132375,-72.3214463970634,
12.));
#70301=CARTESIAN_POINT('Ctrl Pts',(-10.7488061082368,-72.296265618955,12.));
#70302=CARTESIAN_POINT('Ctrl Pts',(-10.7549589083535,-72.2711162461679,
12.));
#70303=CARTESIAN_POINT('Ctrl Pts',(-10.7610790405385,-72.2459983875298,
12.));
#70304=CARTESIAN_POINT('Ctrl Pts',(-10.7671665319254,-72.2209121522367,
12.));
#70305=CARTESIAN_POINT('Ctrl Pts',(-10.7732214098343,-72.1958576498556,
12.));
#70306=CARTESIAN_POINT('Ctrl Pts',(-10.779243701766,-72.17083499033,12.));
#70307=CARTESIAN_POINT('Ctrl Pts',(-10.7852334354015,-72.145844283983,12.));
#70308=CARTESIAN_POINT('Ctrl Pts',(-10.7911906386027,-72.1208856415171,
12.));
#70309=CARTESIAN_POINT('Ctrl Pts',(-10.7971153394168,-72.095959174012,12.));
#70310=CARTESIAN_POINT('Ctrl Pts',(-10.8030075660811,-72.0710649929214,
12.));
#70311=CARTESIAN_POINT('Ctrl Pts',(-10.8088673470187,-72.0462032100828,
12.));
#70312=CARTESIAN_POINT('Ctrl Pts',(-10.8146947108376,-72.0213739377231,
12.));
#70313=CARTESIAN_POINT('Ctrl Pts',(-10.8204896863328,-71.9965772884619,
12.));
#70314=CARTESIAN_POINT('Ctrl Pts',(-10.8262523024897,-71.971813375312,12.));
#70315=CARTESIAN_POINT('Ctrl Pts',(-10.8319825884917,-71.9470823116777,
12.));
#70316=CARTESIAN_POINT('Ctrl Pts',(-10.8376805737158,-71.9223842113622,
12.));
#70317=CARTESIAN_POINT('Ctrl Pts',(-10.8433462877312,-71.8977191885726,
12.));
#70318=CARTESIAN_POINT('Ctrl Pts',(-10.8489797602998,-71.8730873579226,
12.));
#70319=CARTESIAN_POINT('Ctrl Pts',(-10.8545810213799,-71.8484888344335,
12.));
#70320=CARTESIAN_POINT('Ctrl Pts',(-10.860150101133,-71.8239237335318,12.));
#70321=CARTESIAN_POINT('Ctrl Pts',(-10.8656870299218,-71.7993921710546,
12.));
#70322=CARTESIAN_POINT('Ctrl Pts',(-10.8711918383071,-71.7748942632578,
12.));
#70323=CARTESIAN_POINT('Ctrl Pts',(-10.8766645570496,-71.7504301268177,
12.));
#70324=CARTESIAN_POINT('Ctrl Pts',(-10.8821052171122,-71.7259998788337,
12.));
#70325=CARTESIAN_POINT('Ctrl Pts',(-10.8875138496674,-71.7016036368254,
12.));
#70326=CARTESIAN_POINT('Ctrl Pts',(-10.8928904860967,-71.6772415187382,
12.));
#70327=CARTESIAN_POINT('Ctrl Pts',(-10.8982351579872,-71.6529136429515,
12.));
#70328=CARTESIAN_POINT('Ctrl Pts',(-10.9035478971329,-71.6286201282815,
12.));
#70329=CARTESIAN_POINT('Ctrl Pts',(-10.9088287355364,-71.604361093983,12.));
#70330=CARTESIAN_POINT('Ctrl Pts',(-10.9140777054169,-71.5801366597479,
12.));
#70331=CARTESIAN_POINT('Ctrl Pts',(-10.9192948392099,-71.5559469457082,
12.));
#70332=CARTESIAN_POINT('Ctrl Pts',(-10.9244801695642,-71.5317920724453,
12.));
#70333=CARTESIAN_POINT('Ctrl Pts',(-10.9296337293425,-71.5076721609936,
12.));
#70334=CARTESIAN_POINT('Ctrl Pts',(-10.9347555516236,-71.4835873328425,
12.));
#70335=CARTESIAN_POINT('Ctrl Pts',(-10.9398456697094,-71.4595377099352,
12.));
#70336=CARTESIAN_POINT('Ctrl Pts',(-10.9449041171269,-71.4355234146718,
12.));
#70337=CARTESIAN_POINT('Ctrl Pts',(-10.9499309276235,-71.411544569919,12.));
#70338=CARTESIAN_POINT('Ctrl Pts',(-10.9549261351689,-71.3876012990135,
12.));
#70339=CARTESIAN_POINT('Ctrl Pts',(-10.9598897739565,-71.3636937257651,
12.));
#70340=CARTESIAN_POINT('Ctrl Pts',(-10.96482187841,-71.3398219744547,12.));
#70341=CARTESIAN_POINT('Ctrl Pts',(-10.9697224831862,-71.3159861698368,
12.));
#70342=CARTESIAN_POINT('Ctrl Pts',(-10.9745916231711,-71.2921864371499,
12.));
#70343=CARTESIAN_POINT('Ctrl Pts',(-10.9794293334806,-71.2684229021209,
12.));
#70344=CARTESIAN_POINT('Ctrl Pts',(-10.9842356494627,-71.2446956909685,
12.));
#70345=CARTESIAN_POINT('Ctrl Pts',(-10.9890106067038,-71.221004930401,12.));
#70346=CARTESIAN_POINT('Ctrl Pts',(-10.993754241032,-71.1973507476188,12.));
#70347=CARTESIAN_POINT('Ctrl Pts',(-10.9984665885127,-71.1737332703248,
12.));
#70348=CARTESIAN_POINT('Ctrl Pts',(-11.0031476854503,-71.1501526267288,
12.));
#70349=CARTESIAN_POINT('Ctrl Pts',(-11.0077975683895,-71.1266089455517,
12.));
#70350=CARTESIAN_POINT('Ctrl Pts',(-11.0124162741223,-71.1031023560243,
12.));
#70351=CARTESIAN_POINT('Ctrl Pts',(-11.0170038396913,-71.0796329878896,
12.));
#70352=CARTESIAN_POINT('Ctrl Pts',(-11.0215603023854,-71.0562009714125,
12.));
#70353=CARTESIAN_POINT('Ctrl Pts',(-11.0260856997414,-71.0328064373849,
12.));
#70354=CARTESIAN_POINT('Ctrl Pts',(-11.0305800695457,-71.0094495171295,
12.));
#70355=CARTESIAN_POINT('Ctrl Pts',(-11.0350434498408,-70.9861303424989,
12.));
#70356=CARTESIAN_POINT('Ctrl Pts',(-11.039475878929,-70.9628490458779,12.));
#70357=CARTESIAN_POINT('Ctrl Pts',(-11.0438773953686,-70.9396057601953,
12.));
#70358=CARTESIAN_POINT('Ctrl Pts',(-11.0482480379752,-70.9164006189283,
12.));
#70359=CARTESIAN_POINT('Ctrl Pts',(-11.0525878458242,-70.8932337561078,
12.));
#70360=CARTESIAN_POINT('Ctrl Pts',(-11.0568968582566,-70.8701053063158,
12.));
#70361=CARTESIAN_POINT('Ctrl Pts',(-11.061175114883,-70.847015404688,12.));
#70362=CARTESIAN_POINT('Ctrl Pts',(-11.0654226555798,-70.8239641869266,
12.));
#70363=CARTESIAN_POINT('Ctrl Pts',(-11.0696395204907,-70.8009517893042,
12.));
#70364=CARTESIAN_POINT('Ctrl Pts',(-11.0738257500292,-70.7779783486689,
12.));
#70365=CARTESIAN_POINT('Ctrl Pts',(-11.0779813848851,-70.7550440024422,
12.));
#70366=CARTESIAN_POINT('Ctrl Pts',(-11.0821064660276,-70.7321488886229,
12.));
#70367=CARTESIAN_POINT('Ctrl Pts',(-11.0862010347022,-70.7092931457996,
12.));
#70368=CARTESIAN_POINT('Ctrl Pts',(-11.0902651324325,-70.686476913156,12.));
#70369=CARTESIAN_POINT('Ctrl Pts',(-11.0942988010231,-70.6637003304768,
12.));
#70370=CARTESIAN_POINT('Ctrl Pts',(-11.0983020825662,-70.6409635381446,
12.));
#70371=CARTESIAN_POINT('Ctrl Pts',(-11.1022750194439,-70.6182666771441,
12.));
#70372=CARTESIAN_POINT('Ctrl Pts',(-11.1062176543257,-70.5956098890744,
12.));
#70373=CARTESIAN_POINT('Ctrl Pts',(-11.11013003017,-70.5729933161538,12.));
#70374=CARTESIAN_POINT('Ctrl Pts',(-11.1140121902274,-70.5504171012247,
12.));
#70375=CARTESIAN_POINT('Ctrl Pts',(-11.117864178048,-70.5278813877519,12.));
#70376=CARTESIAN_POINT('Ctrl Pts',(-11.121686037483,-70.5053863198306,12.));
#70377=CARTESIAN_POINT('Ctrl Pts',(-11.1254778126824,-70.4829320421973,
12.));
#70378=CARTESIAN_POINT('Ctrl Pts',(-11.1292395480975,-70.4605187002356,
12.));
#70379=CARTESIAN_POINT('Ctrl Pts',(-11.1329712884845,-70.438146439981,12.));
#70380=CARTESIAN_POINT('Ctrl Pts',(-11.1366730789122,-70.415815408119,12.));
#70381=CARTESIAN_POINT('Ctrl Pts',(-11.1403449647622,-70.3935257519945,
12.));
#70382=CARTESIAN_POINT('Ctrl Pts',(-11.1439869917269,-70.3712776196216,
12.));
#70383=CARTESIAN_POINT('Ctrl Pts',(-11.1475992058124,-70.3490711596882,
12.));
#70384=CARTESIAN_POINT('Ctrl Pts',(-11.1511816533422,-70.3269065215591,
12.));
#70385=CARTESIAN_POINT('Ctrl Pts',(-11.1547343809647,-70.3047838552758,
12.));
#70386=CARTESIAN_POINT('Ctrl Pts',(-11.1582574356522,-70.2827033115662,
12.));
#70387=CARTESIAN_POINT('Ctrl Pts',(-11.1617508647017,-70.2606650418589,
12.));
#70388=CARTESIAN_POINT('Ctrl Pts',(-11.1652147157383,-70.2386691982902,
12.));
#70389=CARTESIAN_POINT('Ctrl Pts',(-11.168649036721,-70.2167159337095,12.));
#70390=CARTESIAN_POINT('Ctrl Pts',(-11.1720538759498,-70.1948054016817,
12.));
#70391=CARTESIAN_POINT('Ctrl Pts',(-11.1754292820631,-70.1729377564956,
12.));
#70392=CARTESIAN_POINT('Ctrl Pts',(-11.1787753040363,-70.1511131531674,
12.));
#70393=CARTESIAN_POINT('Ctrl Pts',(-11.1820919911846,-70.1293317474432,
12.));
#70394=CARTESIAN_POINT('Ctrl Pts',(-11.185379393167,-70.1075936957968,12.));
#70395=CARTESIAN_POINT('Ctrl Pts',(-11.1886375599914,-70.0858991554283,
12.));
#70396=CARTESIAN_POINT('Ctrl Pts',(-11.1918665420166,-70.0642482842928,
12.));
#70397=CARTESIAN_POINT('Ctrl Pts',(-11.1950663899576,-70.0426412411185,
12.));
#70398=CARTESIAN_POINT('Ctrl Pts',(-11.1982371548919,-70.0210781854243,
12.));
#70399=CARTESIAN_POINT('Ctrl Pts',(-11.2013788882714,-69.9995592775343,
12.));
#70400=CARTESIAN_POINT('Ctrl Pts',(-11.2044916419244,-69.97808467858,12.));
#70401=CARTESIAN_POINT('Ctrl Pts',(-11.2075754680449,-69.9566545504837,
12.));
#70402=CARTESIAN_POINT('Ctrl Pts',(-11.2106304191882,-69.9352690559405,
12.));
#70403=CARTESIAN_POINT('Ctrl Pts',(-11.2136565482677,-69.9139283584022,
12.));
#70404=CARTESIAN_POINT('Ctrl Pts',(-11.2166539085523,-69.8926326220385,
12.));
#70405=CARTESIAN_POINT('Ctrl Pts',(-11.219622553679,-69.871382011789,12.));
#70406=CARTESIAN_POINT('Ctrl Pts',(-11.2225625376736,-69.8501766934428,
12.));
#70407=CARTESIAN_POINT('Ctrl Pts',(-11.225473914972,-69.8290168337076,12.));
#70408=CARTESIAN_POINT('Ctrl Pts',(-11.2283567404437,-69.8079026002768,
12.));
#70409=CARTESIAN_POINT('Ctrl Pts',(-11.2312110694187,-69.7868341618954,
12.));
#70410=CARTESIAN_POINT('Ctrl Pts',(-11.2340369576456,-69.7658116882324,
12.));
#70411=CARTESIAN_POINT('Ctrl Pts',(-11.2368344612472,-69.7448353497408,
12.));
#70412=CARTESIAN_POINT('Ctrl Pts',(-11.239603636686,-69.7239053175356,12.));
#70413=CARTESIAN_POINT('Ctrl Pts',(-11.2423445407166,-69.7030217632164,
12.));
#70414=CARTESIAN_POINT('Ctrl Pts',(-11.2450572303841,-69.6821848588457,
12.));
#70415=CARTESIAN_POINT('Ctrl Pts',(-11.2477417631386,-69.6613947773534,
12.));
#70416=CARTESIAN_POINT('Ctrl Pts',(-11.2503981969412,-69.6406516928891,
12.));
#70417=CARTESIAN_POINT('Ctrl Pts',(-11.2530265903557,-69.6199557811245,
12.));
#70418=CARTESIAN_POINT('Ctrl Pts',(-11.2556270027016,-69.599307219739,12.));
#70419=CARTESIAN_POINT('Ctrl Pts',(-11.2581994939541,-69.5787061880857,
12.));
#70420=CARTESIAN_POINT('Ctrl Pts',(-11.2607441244702,-69.5581528662877,
12.));
#70421=CARTESIAN_POINT('Ctrl Pts',(-11.263260954763,-69.5376474344771,12.));
#70422=CARTESIAN_POINT('Ctrl Pts',(-11.2657500452716,-69.5171900720158,
12.));
#70423=CARTESIAN_POINT('Ctrl Pts',(-11.2682114561007,-69.4967809565929,
12.));
#70424=CARTESIAN_POINT('Ctrl Pts',(-11.270645247528,-69.4764202659397,12.));
#70425=CARTESIAN_POINT('Ctrl Pts',(-11.2730514806139,-69.456108179879,12.));
#70426=CARTESIAN_POINT('Ctrl Pts',(-11.2754302177021,-69.4358448819967,
12.));
#70427=CARTESIAN_POINT('Ctrl Pts',(-11.2777815231469,-69.4156305620593,
12.));
#70428=CARTESIAN_POINT('Ctrl Pts',(-11.2801054633815,-69.3954654162281,
12.));
#70429=CARTESIAN_POINT('Ctrl Pts',(-11.2824021054045,-69.3753496420039,
12.));
#70430=CARTESIAN_POINT('Ctrl Pts',(-11.2846715154524,-69.3552834337784,
12.));
#70431=CARTESIAN_POINT('Ctrl Pts',(-11.2869137578459,-69.3352669789587,
12.));
#70432=CARTESIAN_POINT('Ctrl Pts',(-11.2891288931517,-69.3153004517783,
12.));
#70433=CARTESIAN_POINT('Ctrl Pts',(-11.2913169799628,-69.295384019272,12.));
#70434=CARTESIAN_POINT('Ctrl Pts',(-11.2934780784351,-69.275517853148,12.));
#70435=CARTESIAN_POINT('Ctrl Pts',(-11.2956122531375,-69.255702139335,12.));
#70436=CARTESIAN_POINT('Ctrl Pts',(-11.2977195764852,-69.2359370894907,
12.));
#70437=CARTESIAN_POINT('Ctrl Pts',(-11.2998001310964,-69.2162229488531,
12.));
#70438=CARTESIAN_POINT('Ctrl Pts',(-11.3018540025638,-69.1965599718914,
12.));
#70439=CARTESIAN_POINT('Ctrl Pts',(-11.3038812726292,-69.1769483991721,
12.));
#70440=CARTESIAN_POINT('Ctrl Pts',(-11.3058820128307,-69.1573884361,12.));
#70441=CARTESIAN_POINT('Ctrl Pts',(-11.3078562764384,-69.1378802251711,
12.));
#70442=CARTESIAN_POINT('Ctrl Pts',(-11.3098040973713,-69.118423844466,12.));
#70443=CARTESIAN_POINT('Ctrl Pts',(-11.3113412156661,-69.1029002322118,
12.));
#70444=CARTESIAN_POINT('Ctrl Pts',(-11.3124821678798,-69.0912808656811,
12.));
#70445=CARTESIAN_POINT('Ctrl Pts',(-11.3132375200165,-69.0835449954396,
12.));
#70446=CARTESIAN_POINT('Ctrl Pts',(-11.3136138754165,-69.079679653846,12.));
#70447=CARTESIAN_POINT('Ctrl Pts',(-8.93459554657871,-73.6640787198061,
-5.55111512312578E-16));
#70448=CARTESIAN_POINT('Ctrl Pts',(-8.93459554657871,-73.6640787198061,
4.));
#70449=CARTESIAN_POINT('Ctrl Pts',(-8.93459554657871,-73.6640787198061,
8.));
#70450=CARTESIAN_POINT('Ctrl Pts',(-8.93459554657871,-73.6640787198061,
12.));
#70451=CARTESIAN_POINT('Ctrl Pts',(-8.9914562677793,-73.7581053903597,-5.55111512312578E-16));
#70452=CARTESIAN_POINT('Ctrl Pts',(-8.9914562677793,-73.7581053903597,4.));
#70453=CARTESIAN_POINT('Ctrl Pts',(-8.9914562677793,-73.7581053903597,8.));
#70454=CARTESIAN_POINT('Ctrl Pts',(-8.9914562677793,-73.7581053903597,12.));
#70455=CARTESIAN_POINT('Ctrl Pts',(-9.14696952162315,-73.8880618019207,
-5.55111512312578E-16));
#70456=CARTESIAN_POINT('Ctrl Pts',(-9.14696952162315,-73.8880618019207,
4.00000000000001));
#70457=CARTESIAN_POINT('Ctrl Pts',(-9.14696952162315,-73.8880618019207,
7.99999999999999));
#70458=CARTESIAN_POINT('Ctrl Pts',(-9.14696952162315,-73.8880618019207,
12.));
#70459=CARTESIAN_POINT('Ctrl Pts',(-9.3439568349051,-73.911753208677,-5.55111512312578E-16));
#70460=CARTESIAN_POINT('Ctrl Pts',(-9.3439568349051,-73.911753208677,4.));
#70461=CARTESIAN_POINT('Ctrl Pts',(-9.3439568349051,-73.911753208677,8.00000000000001));
#70462=CARTESIAN_POINT('Ctrl Pts',(-9.3439568349051,-73.911753208677,12.));
#70463=CARTESIAN_POINT('Ctrl Pts',(-9.42570643237529,-73.9013264985863,
-5.55111512312578E-16));
#70464=CARTESIAN_POINT('Ctrl Pts',(-9.42570643237529,-73.9013264985863,
4.));
#70465=CARTESIAN_POINT('Ctrl Pts',(-9.42570643237529,-73.9013264985863,
8.));
#70466=CARTESIAN_POINT('Ctrl Pts',(-9.42570643237529,-73.9013264985863,
12.));
#70467=CARTESIAN_POINT('',(-8.93459554657871,-73.6640787198061,-2.77555756156289E-16));
#70468=CARTESIAN_POINT('',(-9.42570643237531,-73.9013264985865,2.77555756156289E-16));
#70469=CARTESIAN_POINT('Ctrl Pts',(-8.93459554657871,-73.6640787198061,
1.23259516440783E-31));
#70470=CARTESIAN_POINT('Ctrl Pts',(-8.9914562677793,-73.7581053903597,-2.61926472436664E-31));
#70471=CARTESIAN_POINT('Ctrl Pts',(-9.0803209842615,-73.832366196966,4.93038065763132E-31));
#70472=CARTESIAN_POINT('Ctrl Pts',(-9.1827282507643,-73.8719282264932,3.23556230657056E-31));
#70473=CARTESIAN_POINT('Ctrl Pts',(-9.25953370064141,-73.9015997486385,
1.54074395550979E-31));
#70474=CARTESIAN_POINT('Ctrl Pts',(-9.3439568349051,-73.911753208677,-5.23852944873328E-31));
#70475=CARTESIAN_POINT('Ctrl Pts',(-9.42570643237529,-73.9013264985863,
1.69481835106077E-31));
#70476=CARTESIAN_POINT('',(-9.42570643237531,-73.9013264985865,12.));
#70477=CARTESIAN_POINT('Ctrl Pts',(-9.42570643237529,-73.9013264985863,
-5.55111512312578E-16));
#70478=CARTESIAN_POINT('Ctrl Pts',(-9.42570643237529,-73.9013264985863,
4.));
#70479=CARTESIAN_POINT('Ctrl Pts',(-9.42570643237529,-73.9013264985863,
8.));
#70480=CARTESIAN_POINT('Ctrl Pts',(-9.42570643237529,-73.9013264985863,
12.));
#70481=CARTESIAN_POINT('',(-8.93459554657871,-73.6640787198061,12.));
#70482=CARTESIAN_POINT('Ctrl Pts',(-9.42570643237529,-73.9013264985863,
12.));
#70483=CARTESIAN_POINT('Ctrl Pts',(-9.3439568349051,-73.911753208677,12.));
#70484=CARTESIAN_POINT('Ctrl Pts',(-9.25953370064141,-73.9015997486385,
12.));
#70485=CARTESIAN_POINT('Ctrl Pts',(-9.1827282507643,-73.8719282264932,12.));
#70486=CARTESIAN_POINT('Ctrl Pts',(-9.0803209842615,-73.832366196966,12.));
#70487=CARTESIAN_POINT('Ctrl Pts',(-8.9914562677793,-73.7581053903597,12.));
#70488=CARTESIAN_POINT('Ctrl Pts',(-8.93459554657871,-73.6640787198061,
12.));
#70489=CARTESIAN_POINT('Ctrl Pts',(-8.93459554657871,-73.6640787198061,
12.));
#70490=CARTESIAN_POINT('Ctrl Pts',(-8.93459554657871,-73.6640787198061,
8.));
#70491=CARTESIAN_POINT('Ctrl Pts',(-8.93459554657871,-73.6640787198061,
4.));
#70492=CARTESIAN_POINT('Ctrl Pts',(-8.93459554657871,-73.6640787198061,
-5.55111512312578E-16));
#70493=CARTESIAN_POINT('Origin',(-4.88285199465431E-11,-3.71649880366789E-10,
0.));
#70494=CARTESIAN_POINT('Origin',(-4.88285199465431E-11,-3.71649880366789E-10,
12.));
#70495=CARTESIAN_POINT('Origin',(-4.88285199465431E-11,-3.71649880366789E-10,
0.));
#70496=CARTESIAN_POINT('Ctrl Pts',(-16.4184755008033,-72.6683126419592,
-5.55111512312578E-16));
#70497=CARTESIAN_POINT('Ctrl Pts',(-16.4184755008033,-72.6683126419592,
4.));
#70498=CARTESIAN_POINT('Ctrl Pts',(-16.4184755008033,-72.6683126419592,
8.));
#70499=CARTESIAN_POINT('Ctrl Pts',(-16.4184755008033,-72.6683126419592,
12.));
#70500=CARTESIAN_POINT('Ctrl Pts',(-16.5256563519778,-72.6440964999409,
-5.55111512312578E-16));
#70501=CARTESIAN_POINT('Ctrl Pts',(-16.5256563519778,-72.6440964999409,
4.));
#70502=CARTESIAN_POINT('Ctrl Pts',(-16.5256563519778,-72.6440964999409,
8.00000000000001));
#70503=CARTESIAN_POINT('Ctrl Pts',(-16.5256563519778,-72.6440964999409,
12.));
#70504=CARTESIAN_POINT('Ctrl Pts',(-16.6981133841326,-72.5376471652844,
-5.55111512312578E-16));
#70505=CARTESIAN_POINT('Ctrl Pts',(-16.6981133841326,-72.5376471652844,
4.));
#70506=CARTESIAN_POINT('Ctrl Pts',(-16.6981133841326,-72.5376471652844,
7.99999999999999));
#70507=CARTESIAN_POINT('Ctrl Pts',(-16.6981133841326,-72.5376471652844,
12.));
#70508=CARTESIAN_POINT('Ctrl Pts',(-16.7828708182974,-72.3582555997246,
-5.55111512312578E-16));
#70509=CARTESIAN_POINT('Ctrl Pts',(-16.7828708182974,-72.3582555997246,
4.));
#70510=CARTESIAN_POINT('Ctrl Pts',(-16.7828708182974,-72.3582555997246,
8.00000000000001));
#70511=CARTESIAN_POINT('Ctrl Pts',(-16.7828708182974,-72.3582555997246,
12.));
#70512=CARTESIAN_POINT('Ctrl Pts',(-16.7988252568806,-72.2774028393486,
-5.55111512312578E-16));
#70513=CARTESIAN_POINT('Ctrl Pts',(-16.7988252568806,-72.2774028393486,
4.));
#70514=CARTESIAN_POINT('Ctrl Pts',(-16.7988252568806,-72.2774028393486,
8.));
#70515=CARTESIAN_POINT('Ctrl Pts',(-16.7988252568806,-72.2774028393486,
12.));
#70516=CARTESIAN_POINT('',(-16.4184755008033,-72.6683126419592,0.));
#70517=CARTESIAN_POINT('',(-16.7988252568806,-72.2774028393486,0.));
#70518=CARTESIAN_POINT('Ctrl Pts',(-16.4184755008033,-72.6683126419592,
4.16333634234434E-16));
#70519=CARTESIAN_POINT('Ctrl Pts',(-16.5256563519778,-72.6440964999409,
4.16333634234433E-16));
#70520=CARTESIAN_POINT('Ctrl Pts',(-16.6242032274948,-72.5832683087087,
4.16333634234434E-16));
#70521=CARTESIAN_POINT('Ctrl Pts',(-16.6941134995865,-72.498622246161,4.16333634234434E-16));
#70522=CARTESIAN_POINT('Ctrl Pts',(-16.7465462036553,-72.4351376992502,
4.16333634234434E-16));
#70523=CARTESIAN_POINT('Ctrl Pts',(-16.7828708182974,-72.3582555997246,
4.16333634234433E-16));
#70524=CARTESIAN_POINT('Ctrl Pts',(-16.7988252568806,-72.2774028393486,
4.16333634234434E-16));
#70525=CARTESIAN_POINT('',(-16.7988252568806,-72.2774028393486,12.));
#70526=CARTESIAN_POINT('Ctrl Pts',(-16.7988252568806,-72.2774028393486,
-5.55111512312578E-16));
#70527=CARTESIAN_POINT('Ctrl Pts',(-16.7988252568806,-72.2774028393486,
4.));
#70528=CARTESIAN_POINT('Ctrl Pts',(-16.7988252568806,-72.2774028393486,
8.));
#70529=CARTESIAN_POINT('Ctrl Pts',(-16.7988252568806,-72.2774028393486,
12.));
#70530=CARTESIAN_POINT('',(-16.4184755008033,-72.6683126419592,12.));
#70531=CARTESIAN_POINT('Ctrl Pts',(-16.7988252568806,-72.2774028393486,
12.));
#70532=CARTESIAN_POINT('Ctrl Pts',(-16.7828708182974,-72.3582555997246,
12.));
#70533=CARTESIAN_POINT('Ctrl Pts',(-16.7465462036554,-72.4351376992502,
12.));
#70534=CARTESIAN_POINT('Ctrl Pts',(-16.6941134995865,-72.498622246161,12.));
#70535=CARTESIAN_POINT('Ctrl Pts',(-16.6242032274948,-72.5832683087087,
12.));
#70536=CARTESIAN_POINT('Ctrl Pts',(-16.5256563519778,-72.6440964999409,
12.));
#70537=CARTESIAN_POINT('Ctrl Pts',(-16.4184755008033,-72.6683126419592,
12.));
#70538=CARTESIAN_POINT('Ctrl Pts',(-16.4184755008033,-72.6683126419592,
12.));
#70539=CARTESIAN_POINT('Ctrl Pts',(-16.4184755008033,-72.6683126419592,
8.));
#70540=CARTESIAN_POINT('Ctrl Pts',(-16.4184755008033,-72.6683126419592,
4.));
#70541=CARTESIAN_POINT('Ctrl Pts',(-16.4184755008033,-72.6683126419592,
-5.55111512312578E-16));
#70542=CARTESIAN_POINT('Ctrl Pts',(-17.2912529479484,-67.8307641965655,
0.));
#70543=CARTESIAN_POINT('Ctrl Pts',(-17.2912529479484,-67.8307641965655,
12.));
#70544=CARTESIAN_POINT('Ctrl Pts',(-17.2912149114119,-67.8346476309018,
0.));
#70545=CARTESIAN_POINT('Ctrl Pts',(-17.2912149114119,-67.8346476309018,
12.));
#70546=CARTESIAN_POINT('Ctrl Pts',(-17.2911366591347,-67.842419897098,0.));
#70547=CARTESIAN_POINT('Ctrl Pts',(-17.2911366591347,-67.842419897098,12.));
#70548=CARTESIAN_POINT('Ctrl Pts',(-17.291012743109,-67.8540944889687,0.));
#70549=CARTESIAN_POINT('Ctrl Pts',(-17.291012743109,-67.8540944889687,12.));
#70550=CARTESIAN_POINT('Ctrl Pts',(-17.2908344459694,-67.8696929978782,
0.));
#70551=CARTESIAN_POINT('Ctrl Pts',(-17.2908344459694,-67.8696929978782,
12.));
#70552=CARTESIAN_POINT('Ctrl Pts',(-17.2905897723948,-67.8892451049608,
0.));
#70553=CARTESIAN_POINT('Ctrl Pts',(-17.2905897723948,-67.8892451049608,
12.));
#70554=CARTESIAN_POINT('Ctrl Pts',(-17.2903232740694,-67.9088511496686,
0.));
#70555=CARTESIAN_POINT('Ctrl Pts',(-17.2903232740694,-67.9088511496686,
12.));
#70556=CARTESIAN_POINT('Ctrl Pts',(-17.2900349103981,-67.9285110571741,
0.));
#70557=CARTESIAN_POINT('Ctrl Pts',(-17.2900349103981,-67.9285110571741,
12.));
#70558=CARTESIAN_POINT('Ctrl Pts',(-17.2897246158941,-67.9482246901667,
0.));
#70559=CARTESIAN_POINT('Ctrl Pts',(-17.2897246158941,-67.9482246901667,
12.));
#70560=CARTESIAN_POINT('Ctrl Pts',(-17.2893923013894,-67.9679918502579,
0.));
#70561=CARTESIAN_POINT('Ctrl Pts',(-17.2893923013894,-67.9679918502579,
12.));
#70562=CARTESIAN_POINT('Ctrl Pts',(-17.2890378644866,-67.987812304921,0.));
#70563=CARTESIAN_POINT('Ctrl Pts',(-17.2890378644866,-67.987812304921,12.));
#70564=CARTESIAN_POINT('Ctrl Pts',(-17.28866119774,-68.007685808115,0.));
#70565=CARTESIAN_POINT('Ctrl Pts',(-17.28866119774,-68.007685808115,12.));
#70566=CARTESIAN_POINT('Ctrl Pts',(-17.2882621974721,-68.0276121227356,
0.));
#70567=CARTESIAN_POINT('Ctrl Pts',(-17.2882621974721,-68.0276121227356,
12.));
#70568=CARTESIAN_POINT('Ctrl Pts',(-17.2878407730961,-68.0475910442424,
0.));
#70569=CARTESIAN_POINT('Ctrl Pts',(-17.2878407730961,-68.0475910442424,
12.));
#70570=CARTESIAN_POINT('Ctrl Pts',(-17.2873968440839,-68.0676223930412,
0.));
#70571=CARTESIAN_POINT('Ctrl Pts',(-17.2873968440839,-68.0676223930412,
12.));
#70572=CARTESIAN_POINT('Ctrl Pts',(-17.2869303355432,-68.0877060033205,
0.));
#70573=CARTESIAN_POINT('Ctrl Pts',(-17.2869303355432,-68.0877060033205,
12.));
#70574=CARTESIAN_POINT('Ctrl Pts',(-17.2864411745459,-68.1078417137877,
0.));
#70575=CARTESIAN_POINT('Ctrl Pts',(-17.2864411745459,-68.1078417137877,
12.));
#70576=CARTESIAN_POINT('Ctrl Pts',(-17.2859292855705,-68.1280293561511,
0.));
#70577=CARTESIAN_POINT('Ctrl Pts',(-17.2859292855705,-68.1280293561511,
12.));
#70578=CARTESIAN_POINT('Ctrl Pts',(-17.2853945882072,-68.1482687493226,
0.));
#70579=CARTESIAN_POINT('Ctrl Pts',(-17.2853945882072,-68.1482687493226,
12.));
#70580=CARTESIAN_POINT('Ctrl Pts',(-17.2848369995293,-68.1685597054232,
0.));
#70581=CARTESIAN_POINT('Ctrl Pts',(-17.2848369995293,-68.1685597054232,
12.));
#70582=CARTESIAN_POINT('Ctrl Pts',(-17.2842564355799,-68.1889020335427,
0.));
#70583=CARTESIAN_POINT('Ctrl Pts',(-17.2842564355799,-68.1889020335427,
12.));
#70584=CARTESIAN_POINT('Ctrl Pts',(-17.2836528130819,-68.2092955440567,
0.));
#70585=CARTESIAN_POINT('Ctrl Pts',(-17.2836528130819,-68.2092955440567,
12.));
#70586=CARTESIAN_POINT('Ctrl Pts',(-17.2830260513867,-68.2297400535294,
0.));
#70587=CARTESIAN_POINT('Ctrl Pts',(-17.2830260513867,-68.2297400535294,
12.));
#70588=CARTESIAN_POINT('Ctrl Pts',(-17.2823760723874,-68.2502353845071,
0.));
#70589=CARTESIAN_POINT('Ctrl Pts',(-17.2823760723874,-68.2502353845071,
12.));
#70590=CARTESIAN_POINT('Ctrl Pts',(-17.2817027995831,-68.2707813631731,
0.));
#70591=CARTESIAN_POINT('Ctrl Pts',(-17.2817027995831,-68.2707813631731,
12.));
#70592=CARTESIAN_POINT('Ctrl Pts',(-17.2810061574353,-68.2913778177261,
0.));
#70593=CARTESIAN_POINT('Ctrl Pts',(-17.2810061574353,-68.2913778177261,
12.));
#70594=CARTESIAN_POINT('Ctrl Pts',(-17.2802860705815,-68.3120245763914,
0.));
#70595=CARTESIAN_POINT('Ctrl Pts',(-17.2802860705815,-68.3120245763914,
12.));
#70596=CARTESIAN_POINT('Ctrl Pts',(-17.2795424631799,-68.3327214657575,
0.));
#70597=CARTESIAN_POINT('Ctrl Pts',(-17.2795424631799,-68.3327214657575,
12.));
#70598=CARTESIAN_POINT('Ctrl Pts',(-17.2787752592484,-68.3534683116515,
0.));
#70599=CARTESIAN_POINT('Ctrl Pts',(-17.2787752592484,-68.3534683116515,
12.));
#70600=CARTESIAN_POINT('Ctrl Pts',(-17.2779843829608,-68.3742649398964,
0.));
#70601=CARTESIAN_POINT('Ctrl Pts',(-17.2779843829608,-68.3742649398964,
12.));
#70602=CARTESIAN_POINT('Ctrl Pts',(-17.2771697589384,-68.3951111770487,
0.));
#70603=CARTESIAN_POINT('Ctrl Pts',(-17.2771697589384,-68.3951111770487,
12.));
#70604=CARTESIAN_POINT('Ctrl Pts',(-17.2763313126018,-68.4160068512753,
0.));
#70605=CARTESIAN_POINT('Ctrl Pts',(-17.2763313126018,-68.4160068512753,
12.));
#70606=CARTESIAN_POINT('Ctrl Pts',(-17.2754689702992,-68.436951792677,0.));
#70607=CARTESIAN_POINT('Ctrl Pts',(-17.2754689702992,-68.436951792677,12.));
#70608=CARTESIAN_POINT('Ctrl Pts',(-17.2745826591119,-68.4579458328185,
0.));
#70609=CARTESIAN_POINT('Ctrl Pts',(-17.2745826591119,-68.4579458328185,
12.));
#70610=CARTESIAN_POINT('Ctrl Pts',(-17.2736723067365,-68.4789888044351,
0.));
#70611=CARTESIAN_POINT('Ctrl Pts',(-17.2736723067365,-68.4789888044351,
12.));
#70612=CARTESIAN_POINT('Ctrl Pts',(-17.2727378413489,-68.5000805410911,
0.));
#70613=CARTESIAN_POINT('Ctrl Pts',(-17.2727378413489,-68.5000805410911,
12.));
#70614=CARTESIAN_POINT('Ctrl Pts',(-17.2717791914544,-68.521220876786,0.));
#70615=CARTESIAN_POINT('Ctrl Pts',(-17.2717791914544,-68.521220876786,12.));
#70616=CARTESIAN_POINT('Ctrl Pts',(-17.2707962858919,-68.5424096459772,
0.));
#70617=CARTESIAN_POINT('Ctrl Pts',(-17.2707962858919,-68.5424096459772,
12.));
#70618=CARTESIAN_POINT('Ctrl Pts',(-17.269789053896,-68.5636466837517,0.));
#70619=CARTESIAN_POINT('Ctrl Pts',(-17.269789053896,-68.5636466837517,12.));
#70620=CARTESIAN_POINT('Ctrl Pts',(-17.2687574251428,-68.5849318259449,
0.));
#70621=CARTESIAN_POINT('Ctrl Pts',(-17.2687574251428,-68.5849318259449,
12.));
#70622=CARTESIAN_POINT('Ctrl Pts',(-17.2677013298057,-68.6062649092764,
0.));
#70623=CARTESIAN_POINT('Ctrl Pts',(-17.2677013298057,-68.6062649092764,
12.));
#70624=CARTESIAN_POINT('Ctrl Pts',(-17.2666206986084,-68.6276457714729,
0.));
#70625=CARTESIAN_POINT('Ctrl Pts',(-17.2666206986084,-68.6276457714729,
12.));
#70626=CARTESIAN_POINT('Ctrl Pts',(-17.2655154627928,-68.6490742512057,
0.));
#70627=CARTESIAN_POINT('Ctrl Pts',(-17.2655154627928,-68.6490742512057,
12.));
#70628=CARTESIAN_POINT('Ctrl Pts',(-17.2643855540892,-68.6705501880249,
0.));
#70629=CARTESIAN_POINT('Ctrl Pts',(-17.2643855540892,-68.6705501880249,
12.));
#70630=CARTESIAN_POINT('Ctrl Pts',(-17.2632309046892,-68.6920734222938,
0.));
#70631=CARTESIAN_POINT('Ctrl Pts',(-17.2632309046892,-68.6920734222938,
12.));
#70632=CARTESIAN_POINT('Ctrl Pts',(-17.2620514472182,-68.7136437951097,
0.));
#70633=CARTESIAN_POINT('Ctrl Pts',(-17.2620514472182,-68.7136437951097,
12.));
#70634=CARTESIAN_POINT('Ctrl Pts',(-17.2608471147185,-68.7352611482547,
0.));
#70635=CARTESIAN_POINT('Ctrl Pts',(-17.2608471147185,-68.7352611482547,
12.));
#70636=CARTESIAN_POINT('Ctrl Pts',(-17.259617840655,-68.7569253242333,0.));
#70637=CARTESIAN_POINT('Ctrl Pts',(-17.259617840655,-68.7569253242333,12.));
#70638=CARTESIAN_POINT('Ctrl Pts',(-17.2583635589198,-68.7786361662882,
0.));
#70639=CARTESIAN_POINT('Ctrl Pts',(-17.2583635589198,-68.7786361662882,
12.));
#70640=CARTESIAN_POINT('Ctrl Pts',(-17.2570842038383,-68.8003935184184,
0.));
#70641=CARTESIAN_POINT('Ctrl Pts',(-17.2570842038383,-68.8003935184184,
12.));
#70642=CARTESIAN_POINT('Ctrl Pts',(-17.2557797101812,-68.8221972253941,
0.));
#70643=CARTESIAN_POINT('Ctrl Pts',(-17.2557797101812,-68.8221972253941,
12.));
#70644=CARTESIAN_POINT('Ctrl Pts',(-17.2544500131624,-68.844047132755,0.));
#70645=CARTESIAN_POINT('Ctrl Pts',(-17.2544500131624,-68.844047132755,12.));
#70646=CARTESIAN_POINT('Ctrl Pts',(-17.2530950484258,-68.8659430867972,
0.));
#70647=CARTESIAN_POINT('Ctrl Pts',(-17.2530950484258,-68.8659430867972,
12.));
#70648=CARTESIAN_POINT('Ctrl Pts',(-17.2517147520376,-68.8878849345557,
0.));
#70649=CARTESIAN_POINT('Ctrl Pts',(-17.2517147520376,-68.8878849345557,
12.));
#70650=CARTESIAN_POINT('Ctrl Pts',(-17.2503090604792,-68.909872523787,0.));
#70651=CARTESIAN_POINT('Ctrl Pts',(-17.2503090604792,-68.909872523787,12.));
#70652=CARTESIAN_POINT('Ctrl Pts',(-17.248877910643,-68.9319057029409,0.));
#70653=CARTESIAN_POINT('Ctrl Pts',(-17.248877910643,-68.9319057029409,12.));
#70654=CARTESIAN_POINT('Ctrl Pts',(-17.2474212398275,-68.9539843211619,
0.));
#70655=CARTESIAN_POINT('Ctrl Pts',(-17.2474212398275,-68.9539843211619,
12.));
#70656=CARTESIAN_POINT('Ctrl Pts',(-17.2459389857327,-68.9761082282922,
0.));
#70657=CARTESIAN_POINT('Ctrl Pts',(-17.2459389857327,-68.9761082282922,
12.));
#70658=CARTESIAN_POINT('Ctrl Pts',(-17.2444310864585,-68.9982772748694,
0.));
#70659=CARTESIAN_POINT('Ctrl Pts',(-17.2444310864585,-68.9982772748694,
12.));
#70660=CARTESIAN_POINT('Ctrl Pts',(-17.2428974805044,-69.0204913121225,
0.));
#70661=CARTESIAN_POINT('Ctrl Pts',(-17.2428974805044,-69.0204913121225,
12.));
#70662=CARTESIAN_POINT('Ctrl Pts',(-17.2413381067723,-69.0427501919636,
0.));
#70663=CARTESIAN_POINT('Ctrl Pts',(-17.2413381067723,-69.0427501919636,
12.));
#70664=CARTESIAN_POINT('Ctrl Pts',(-17.2397529045589,-69.065053766986,0.));
#70665=CARTESIAN_POINT('Ctrl Pts',(-17.2397529045589,-69.065053766986,12.));
#70666=CARTESIAN_POINT('Ctrl Pts',(-17.238141813549,-69.0874018904599,0.));
#70667=CARTESIAN_POINT('Ctrl Pts',(-17.238141813549,-69.0874018904599,12.));
#70668=CARTESIAN_POINT('Ctrl Pts',(-17.2365047738125,-69.1097944163245,
0.));
#70669=CARTESIAN_POINT('Ctrl Pts',(-17.2365047738125,-69.1097944163245,
12.));
#70670=CARTESIAN_POINT('Ctrl Pts',(-17.2348417258015,-69.1322311991752,
0.));
#70671=CARTESIAN_POINT('Ctrl Pts',(-17.2348417258015,-69.1322311991752,
12.));
#70672=CARTESIAN_POINT('Ctrl Pts',(-17.2331526103506,-69.1547120942527,
0.));
#70673=CARTESIAN_POINT('Ctrl Pts',(-17.2331526103506,-69.1547120942527,
12.));
#70674=CARTESIAN_POINT('Ctrl Pts',(-17.23143736867,-69.1772369574447,0.));
#70675=CARTESIAN_POINT('Ctrl Pts',(-17.23143736867,-69.1772369574447,12.));
#70676=CARTESIAN_POINT('Ctrl Pts',(-17.2296959423407,-69.1998056452828,
0.));
#70677=CARTESIAN_POINT('Ctrl Pts',(-17.2296959423407,-69.1998056452828,
12.));
#70678=CARTESIAN_POINT('Ctrl Pts',(-17.227928273312,-69.222418014938,0.));
#70679=CARTESIAN_POINT('Ctrl Pts',(-17.227928273312,-69.222418014938,12.));
#70680=CARTESIAN_POINT('Ctrl Pts',(-17.226134303902,-69.2450739242109,0.));
#70681=CARTESIAN_POINT('Ctrl Pts',(-17.226134303902,-69.2450739242109,12.));
#70682=CARTESIAN_POINT('Ctrl Pts',(-17.224313976797,-69.2677732315224,0.));
#70683=CARTESIAN_POINT('Ctrl Pts',(-17.224313976797,-69.2677732315224,12.));
#70684=CARTESIAN_POINT('Ctrl Pts',(-17.2224672350438,-69.2905157959166,
0.));
#70685=CARTESIAN_POINT('Ctrl Pts',(-17.2224672350438,-69.2905157959166,
12.));
#70686=CARTESIAN_POINT('Ctrl Pts',(-17.2205940220459,-69.3133014770555,
0.));
#70687=CARTESIAN_POINT('Ctrl Pts',(-17.2205940220459,-69.3133014770555,
12.));
#70688=CARTESIAN_POINT('Ctrl Pts',(-17.2186942815602,-69.3361301352141,
0.));
#70689=CARTESIAN_POINT('Ctrl Pts',(-17.2186942815602,-69.3361301352141,
12.));
#70690=CARTESIAN_POINT('Ctrl Pts',(-17.2167679576984,-69.3590016312692,
0.));
#70691=CARTESIAN_POINT('Ctrl Pts',(-17.2167679576984,-69.3590016312692,
12.));
#70692=CARTESIAN_POINT('Ctrl Pts',(-17.2148149949252,-69.3819158266916,
0.));
#70693=CARTESIAN_POINT('Ctrl Pts',(-17.2148149949252,-69.3819158266916,
12.));
#70694=CARTESIAN_POINT('Ctrl Pts',(-17.2128353380502,-69.404872583548,0.));
#70695=CARTESIAN_POINT('Ctrl Pts',(-17.2128353380502,-69.404872583548,12.));
#70696=CARTESIAN_POINT('Ctrl Pts',(-17.2108289322254,-69.4278717644973,
0.));
#70697=CARTESIAN_POINT('Ctrl Pts',(-17.2108289322254,-69.4278717644973,
12.));
#70698=CARTESIAN_POINT('Ctrl Pts',(-17.2087957229423,-69.450913232785,0.));
#70699=CARTESIAN_POINT('Ctrl Pts',(-17.2087957229423,-69.450913232785,12.));
#70700=CARTESIAN_POINT('Ctrl Pts',(-17.2067356560336,-69.4739968522313,
0.));
#70701=CARTESIAN_POINT('Ctrl Pts',(-17.2067356560336,-69.4739968522313,
12.));
#70702=CARTESIAN_POINT('Ctrl Pts',(-17.2046486776708,-69.4971224872269,
0.));
#70703=CARTESIAN_POINT('Ctrl Pts',(-17.2046486776708,-69.4971224872269,
12.));
#70704=CARTESIAN_POINT('Ctrl Pts',(-17.2025347343577,-69.5202900027367,
0.));
#70705=CARTESIAN_POINT('Ctrl Pts',(-17.2025347343577,-69.5202900027367,
12.));
#70706=CARTESIAN_POINT('Ctrl Pts',(-17.2003937729268,-69.5434992642944,
0.));
#70707=CARTESIAN_POINT('Ctrl Pts',(-17.2003937729268,-69.5434992642944,
12.));
#70708=CARTESIAN_POINT('Ctrl Pts',(-17.1982257405377,-69.5667501379969,
0.));
#70709=CARTESIAN_POINT('Ctrl Pts',(-17.1982257405377,-69.5667501379969,
12.));
#70710=CARTESIAN_POINT('Ctrl Pts',(-17.196030584678,-69.5900424904921,0.));
#70711=CARTESIAN_POINT('Ctrl Pts',(-17.196030584678,-69.5900424904921,12.));
#70712=CARTESIAN_POINT('Ctrl Pts',(-17.1938082531612,-69.6133761889748,
0.));
#70713=CARTESIAN_POINT('Ctrl Pts',(-17.1938082531612,-69.6133761889748,
12.));
#70714=CARTESIAN_POINT('Ctrl Pts',(-17.1915586941192,-69.6367511011898,
0.));
#70715=CARTESIAN_POINT('Ctrl Pts',(-17.1915586941192,-69.6367511011898,
12.));
#70716=CARTESIAN_POINT('Ctrl Pts',(-17.1892818560002,-69.6601670954269,
0.));
#70717=CARTESIAN_POINT('Ctrl Pts',(-17.1892818560002,-69.6601670954269,
12.));
#70718=CARTESIAN_POINT('Ctrl Pts',(-17.1869776875666,-69.6836240405164,
0.));
#70719=CARTESIAN_POINT('Ctrl Pts',(-17.1869776875666,-69.6836240405164,
12.));
#70720=CARTESIAN_POINT('Ctrl Pts',(-17.1846461378973,-69.7071218058178,
0.));
#70721=CARTESIAN_POINT('Ctrl Pts',(-17.1846461378973,-69.7071218058178,
12.));
#70722=CARTESIAN_POINT('Ctrl Pts',(-17.1822871563842,-69.7306602612155,
0.));
#70723=CARTESIAN_POINT('Ctrl Pts',(-17.1822871563842,-69.7306602612155,
12.));
#70724=CARTESIAN_POINT('Ctrl Pts',(-17.179900692726,-69.7542392771234,0.));
#70725=CARTESIAN_POINT('Ctrl Pts',(-17.179900692726,-69.7542392771234,12.));
#70726=CARTESIAN_POINT('Ctrl Pts',(-17.1774866969256,-69.777858724479,0.));
#70727=CARTESIAN_POINT('Ctrl Pts',(-17.1774866969256,-69.777858724479,12.));
#70728=CARTESIAN_POINT('Ctrl Pts',(-17.1750451192885,-69.8015184747398,
0.));
#70729=CARTESIAN_POINT('Ctrl Pts',(-17.1750451192885,-69.8015184747398,
12.));
#70730=CARTESIAN_POINT('Ctrl Pts',(-17.1725759104251,-69.8252183998702,
0.));
#70731=CARTESIAN_POINT('Ctrl Pts',(-17.1725759104251,-69.8252183998702,
12.));
#70732=CARTESIAN_POINT('Ctrl Pts',(-17.1700790212473,-69.8489583723407,
0.));
#70733=CARTESIAN_POINT('Ctrl Pts',(-17.1700790212473,-69.8489583723407,
12.));
#70734=CARTESIAN_POINT('Ctrl Pts',(-17.167554402962,-69.8727382651286,0.));
#70735=CARTESIAN_POINT('Ctrl Pts',(-17.167554402962,-69.8727382651286,12.));
#70736=CARTESIAN_POINT('Ctrl Pts',(-17.1650020070686,-69.8965579517147,
0.));
#70737=CARTESIAN_POINT('Ctrl Pts',(-17.1650020070686,-69.8965579517147,
12.));
#70738=CARTESIAN_POINT('Ctrl Pts',(-17.1624217853578,-69.9204173060781,
0.));
#70739=CARTESIAN_POINT('Ctrl Pts',(-17.1624217853578,-69.9204173060781,
12.));
#70740=CARTESIAN_POINT('Ctrl Pts',(-17.1598136899144,-69.9443162026865,
0.));
#70741=CARTESIAN_POINT('Ctrl Pts',(-17.1598136899144,-69.9443162026865,
12.));
#70742=CARTESIAN_POINT('Ctrl Pts',(-17.1571776731139,-69.9682545164939,
0.));
#70743=CARTESIAN_POINT('Ctrl Pts',(-17.1571776731139,-69.9682545164939,
12.));
#70744=CARTESIAN_POINT('Ctrl Pts',(-17.154513687616,-69.9922321229424,0.));
#70745=CARTESIAN_POINT('Ctrl Pts',(-17.154513687616,-69.9922321229424,12.));
#70746=CARTESIAN_POINT('Ctrl Pts',(-17.1518216863623,-70.0162488979584,
0.));
#70747=CARTESIAN_POINT('Ctrl Pts',(-17.1518216863623,-70.0162488979584,
12.));
#70748=CARTESIAN_POINT('Ctrl Pts',(-17.1491016225749,-70.0403047179483,
0.));
#70749=CARTESIAN_POINT('Ctrl Pts',(-17.1491016225749,-70.0403047179483,
12.));
#70750=CARTESIAN_POINT('Ctrl Pts',(-17.1463534497594,-70.0643994597873,
0.));
#70751=CARTESIAN_POINT('Ctrl Pts',(-17.1463534497594,-70.0643994597873,
12.));
#70752=CARTESIAN_POINT('Ctrl Pts',(-17.1435771217018,-70.0885330008179,
0.));
#70753=CARTESIAN_POINT('Ctrl Pts',(-17.1435771217018,-70.0885330008179,
12.));
#70754=CARTESIAN_POINT('Ctrl Pts',(-17.1407725924617,-70.1127052188522,
0.));
#70755=CARTESIAN_POINT('Ctrl Pts',(-17.1407725924617,-70.1127052188522,
12.));
#70756=CARTESIAN_POINT('Ctrl Pts',(-17.1379398163709,-70.1369159921687,
0.));
#70757=CARTESIAN_POINT('Ctrl Pts',(-17.1379398163709,-70.1369159921687,
12.));
#70758=CARTESIAN_POINT('Ctrl Pts',(-17.1350787480312,-70.1611651995083,
0.));
#70759=CARTESIAN_POINT('Ctrl Pts',(-17.1350787480312,-70.1611651995083,
12.));
#70760=CARTESIAN_POINT('Ctrl Pts',(-17.1321893423182,-70.1854527200631,
0.));
#70761=CARTESIAN_POINT('Ctrl Pts',(-17.1321893423182,-70.1854527200631,
12.));
#70762=CARTESIAN_POINT('Ctrl Pts',(-17.1292715543778,-70.2097784334747,
0.));
#70763=CARTESIAN_POINT('Ctrl Pts',(-17.1292715543778,-70.2097784334747,
12.));
#70764=CARTESIAN_POINT('Ctrl Pts',(-17.1263253396202,-70.2341422198363,
0.));
#70765=CARTESIAN_POINT('Ctrl Pts',(-17.1263253396202,-70.2341422198363,
12.));
#70766=CARTESIAN_POINT('Ctrl Pts',(-17.1233506537176,-70.2585439596901,
0.));
#70767=CARTESIAN_POINT('Ctrl Pts',(-17.1233506537176,-70.2585439596901,
12.));
#70768=CARTESIAN_POINT('Ctrl Pts',(-17.1203474526031,-70.2829835340238,
0.));
#70769=CARTESIAN_POINT('Ctrl Pts',(-17.1203474526031,-70.2829835340238,
12.));
#70770=CARTESIAN_POINT('Ctrl Pts',(-17.1173156924733,-70.3074608242608,
0.));
#70771=CARTESIAN_POINT('Ctrl Pts',(-17.1173156924733,-70.3074608242608,
12.));
#70772=CARTESIAN_POINT('Ctrl Pts',(-17.1142553297867,-70.3319757122568,
0.));
#70773=CARTESIAN_POINT('Ctrl Pts',(-17.1142553297867,-70.3319757122568,
12.));
#70774=CARTESIAN_POINT('Ctrl Pts',(-17.1111663212568,-70.3565280803022,
0.));
#70775=CARTESIAN_POINT('Ctrl Pts',(-17.1111663212568,-70.3565280803022,
12.));
#70776=CARTESIAN_POINT('Ctrl Pts',(-17.1080486238499,-70.3811178111201,
0.));
#70777=CARTESIAN_POINT('Ctrl Pts',(-17.1080486238499,-70.3811178111201,
12.));
#70778=CARTESIAN_POINT('Ctrl Pts',(-17.1049021947834,-70.4057447878624,
0.));
#70779=CARTESIAN_POINT('Ctrl Pts',(-17.1049021947834,-70.4057447878624,
12.));
#70780=CARTESIAN_POINT('Ctrl Pts',(-17.1017269915292,-70.430408894101,0.));
#70781=CARTESIAN_POINT('Ctrl Pts',(-17.1017269915292,-70.430408894101,12.));
#70782=CARTESIAN_POINT('Ctrl Pts',(-17.0985229718124,-70.4551100138238,
0.));
#70783=CARTESIAN_POINT('Ctrl Pts',(-17.0985229718124,-70.4551100138238,
12.));
#70784=CARTESIAN_POINT('Ctrl Pts',(-17.0952900936048,-70.4798480314381,
0.));
#70785=CARTESIAN_POINT('Ctrl Pts',(-17.0952900936048,-70.4798480314381,
12.));
#70786=CARTESIAN_POINT('Ctrl Pts',(-17.0920283151219,-70.5046228317677,
0.));
#70787=CARTESIAN_POINT('Ctrl Pts',(-17.0920283151219,-70.5046228317677,
12.));
#70788=CARTESIAN_POINT('Ctrl Pts',(-17.088737594822,-70.5294343000513,0.));
#70789=CARTESIAN_POINT('Ctrl Pts',(-17.088737594822,-70.5294343000513,12.));
#70790=CARTESIAN_POINT('Ctrl Pts',(-17.0854178914087,-70.5542823219331,
0.));
#70791=CARTESIAN_POINT('Ctrl Pts',(-17.0854178914087,-70.5542823219331,
12.));
#70792=CARTESIAN_POINT('Ctrl Pts',(-17.082069163831,-70.5791667834582,0.));
#70793=CARTESIAN_POINT('Ctrl Pts',(-17.082069163831,-70.5791667834582,12.));
#70794=CARTESIAN_POINT('Ctrl Pts',(-17.0786913712763,-70.6040875710749,
0.));
#70795=CARTESIAN_POINT('Ctrl Pts',(-17.0786913712763,-70.6040875710749,
12.));
#70796=CARTESIAN_POINT('Ctrl Pts',(-17.0752844731678,-70.6290445716337,
0.));
#70797=CARTESIAN_POINT('Ctrl Pts',(-17.0752844731678,-70.6290445716337,
12.));
#70798=CARTESIAN_POINT('Ctrl Pts',(-17.0718484291624,-70.6540376723841,
0.));
#70799=CARTESIAN_POINT('Ctrl Pts',(-17.0718484291624,-70.6540376723841,
12.));
#70800=CARTESIAN_POINT('Ctrl Pts',(-17.0683831991532,-70.6790667609679,
0.));
#70801=CARTESIAN_POINT('Ctrl Pts',(-17.0683831991532,-70.6790667609679,
12.));
#70802=CARTESIAN_POINT('Ctrl Pts',(-17.0648887432713,-70.7041317254125,
0.));
#70803=CARTESIAN_POINT('Ctrl Pts',(-17.0648887432713,-70.7041317254125,
12.));
#70804=CARTESIAN_POINT('Ctrl Pts',(-17.0613650218787,-70.7292324541341,
0.));
#70805=CARTESIAN_POINT('Ctrl Pts',(-17.0613650218787,-70.7292324541341,
12.));
#70806=CARTESIAN_POINT('Ctrl Pts',(-17.0578119955649,-70.7543688359374,
0.));
#70807=CARTESIAN_POINT('Ctrl Pts',(-17.0578119955649,-70.7543688359374,
12.));
#70808=CARTESIAN_POINT('Ctrl Pts',(-17.0542296251462,-70.7795407600127,
0.));
#70809=CARTESIAN_POINT('Ctrl Pts',(-17.0542296251462,-70.7795407600127,
12.));
#70810=CARTESIAN_POINT('Ctrl Pts',(-17.0506178716664,-70.8047481159306,
0.));
#70811=CARTESIAN_POINT('Ctrl Pts',(-17.0506178716664,-70.8047481159306,
12.));
#70812=CARTESIAN_POINT('Ctrl Pts',(-17.0469766964005,-70.8299907936346,
0.));
#70813=CARTESIAN_POINT('Ctrl Pts',(-17.0469766964005,-70.8299907936346,
12.));
#70814=CARTESIAN_POINT('Ctrl Pts',(-17.0433060608478,-70.8552686834435,
0.));
#70815=CARTESIAN_POINT('Ctrl Pts',(-17.0433060608478,-70.8552686834435,
12.));
#70816=CARTESIAN_POINT('Ctrl Pts',(-17.0396059267279,-70.8805816760507,
0.));
#70817=CARTESIAN_POINT('Ctrl Pts',(-17.0396059267279,-70.8805816760507,
12.));
#70818=CARTESIAN_POINT('Ctrl Pts',(-17.0358762559786,-70.9059296625214,
0.));
#70819=CARTESIAN_POINT('Ctrl Pts',(-17.0358762559786,-70.9059296625214,
12.));
#70820=CARTESIAN_POINT('Ctrl Pts',(-17.0321170107562,-70.9313125342872,
0.));
#70821=CARTESIAN_POINT('Ctrl Pts',(-17.0321170107562,-70.9313125342872,
12.));
#70822=CARTESIAN_POINT('Ctrl Pts',(-17.028328153439,-70.9567301831355,0.));
#70823=CARTESIAN_POINT('Ctrl Pts',(-17.028328153439,-70.9567301831355,12.));
#70824=CARTESIAN_POINT('Ctrl Pts',(-17.0245096466228,-70.9821825012134,
0.));
#70825=CARTESIAN_POINT('Ctrl Pts',(-17.0245096466228,-70.9821825012134,
12.));
#70826=CARTESIAN_POINT('Ctrl Pts',(-17.0206614531165,-71.0076693810303,
0.));
#70827=CARTESIAN_POINT('Ctrl Pts',(-17.0206614531165,-71.0076693810303,
12.));
#70828=CARTESIAN_POINT('Ctrl Pts',(-17.0167835359419,-71.0331907154575,
0.));
#70829=CARTESIAN_POINT('Ctrl Pts',(-17.0167835359419,-71.0331907154575,
12.));
#70830=CARTESIAN_POINT('Ctrl Pts',(-17.0128758583335,-71.0587463977266,
0.));
#70831=CARTESIAN_POINT('Ctrl Pts',(-17.0128758583335,-71.0587463977266,
12.));
#70832=CARTESIAN_POINT('Ctrl Pts',(-17.0089383837436,-71.0843363214216,
0.));
#70833=CARTESIAN_POINT('Ctrl Pts',(-17.0089383837436,-71.0843363214216,
12.));
#70834=CARTESIAN_POINT('Ctrl Pts',(-17.0049710758393,-71.1099603804779,
0.));
#70835=CARTESIAN_POINT('Ctrl Pts',(-17.0049710758393,-71.1099603804779,
12.));
#70836=CARTESIAN_POINT('Ctrl Pts',(-17.0009738984935,-71.1356184691799,
0.));
#70837=CARTESIAN_POINT('Ctrl Pts',(-17.0009738984935,-71.1356184691799,
12.));
#70838=CARTESIAN_POINT('Ctrl Pts',(-16.9969468157824,-71.1613104821565,
0.));
#70839=CARTESIAN_POINT('Ctrl Pts',(-16.9969468157824,-71.1613104821565,
12.));
#70840=CARTESIAN_POINT('Ctrl Pts',(-16.9928897919829,-71.1870363143742,
0.));
#70841=CARTESIAN_POINT('Ctrl Pts',(-16.9928897919829,-71.1870363143742,
12.));
#70842=CARTESIAN_POINT('Ctrl Pts',(-16.9888027915743,-71.2127958611248,
0.));
#70843=CARTESIAN_POINT('Ctrl Pts',(-16.9888027915743,-71.2127958611248,
12.));
#70844=CARTESIAN_POINT('Ctrl Pts',(-16.9846857792385,-71.2385890180233,
0.));
#70845=CARTESIAN_POINT('Ctrl Pts',(-16.9846857792385,-71.2385890180233,
12.));
#70846=CARTESIAN_POINT('Ctrl Pts',(-16.9805387198573,-71.2644156810209,
0.));
#70847=CARTESIAN_POINT('Ctrl Pts',(-16.9805387198573,-71.2644156810209,
12.));
#70848=CARTESIAN_POINT('Ctrl Pts',(-16.9763615785137,-71.2902757464127,
0.));
#70849=CARTESIAN_POINT('Ctrl Pts',(-16.9763615785137,-71.2902757464127,
12.));
#70850=CARTESIAN_POINT('Ctrl Pts',(-16.9721543204951,-71.3161691108425,
0.));
#70851=CARTESIAN_POINT('Ctrl Pts',(-16.9721543204951,-71.3161691108425,
12.));
#70852=CARTESIAN_POINT('Ctrl Pts',(-16.9679169112993,-71.3420956713072,
0.));
#70853=CARTESIAN_POINT('Ctrl Pts',(-16.9679169112993,-71.3420956713072,
12.));
#70854=CARTESIAN_POINT('Ctrl Pts',(-16.9636493166395,-71.3680553251548,
0.));
#70855=CARTESIAN_POINT('Ctrl Pts',(-16.9636493166395,-71.3680553251548,
12.));
#70856=CARTESIAN_POINT('Ctrl Pts',(-16.9593515024274,-71.3940479700663,
0.));
#70857=CARTESIAN_POINT('Ctrl Pts',(-16.9593515024274,-71.3940479700663,
12.));
#70858=CARTESIAN_POINT('Ctrl Pts',(-16.9550234347619,-71.4200735040374,
0.));
#70859=CARTESIAN_POINT('Ctrl Pts',(-16.9550234347619,-71.4200735040374,
12.));
#70860=CARTESIAN_POINT('Ctrl Pts',(-16.9506650799188,-71.4461318253561,
0.));
#70861=CARTESIAN_POINT('Ctrl Pts',(-16.9506650799188,-71.4461318253561,
12.));
#70862=CARTESIAN_POINT('Ctrl Pts',(-16.9462764043445,-71.4722228325805,
0.));
#70863=CARTESIAN_POINT('Ctrl Pts',(-16.9462764043445,-71.4722228325805,
12.));
#70864=CARTESIAN_POINT('Ctrl Pts',(-16.9418573746492,-71.498346424507,0.));
#70865=CARTESIAN_POINT('Ctrl Pts',(-16.9418573746492,-71.498346424507,12.));
#70866=CARTESIAN_POINT('Ctrl Pts',(-16.9374079576204,-71.5245025002154,
0.));
#70867=CARTESIAN_POINT('Ctrl Pts',(-16.9374079576204,-71.5245025002154,
12.));
#70868=CARTESIAN_POINT('Ctrl Pts',(-16.9329281202379,-71.5506909591139,
0.));
#70869=CARTESIAN_POINT('Ctrl Pts',(-16.9329281202379,-71.5506909591139,
12.));
#70870=CARTESIAN_POINT('Ctrl Pts',(-16.9284178296934,-71.5769117009844,
0.));
#70871=CARTESIAN_POINT('Ctrl Pts',(-16.9284178296934,-71.5769117009844,
12.));
#70872=CARTESIAN_POINT('Ctrl Pts',(-16.923877053407,-71.6031646260169,0.));
#70873=CARTESIAN_POINT('Ctrl Pts',(-16.923877053407,-71.6031646260169,12.));
#70874=CARTESIAN_POINT('Ctrl Pts',(-16.9193057590605,-71.6294496348644,
0.));
#70875=CARTESIAN_POINT('Ctrl Pts',(-16.9193057590605,-71.6294496348644,
12.));
#70876=CARTESIAN_POINT('Ctrl Pts',(-16.9147039145715,-71.6557666285908,
0.));
#70877=CARTESIAN_POINT('Ctrl Pts',(-16.9147039145715,-71.6557666285908,
12.));
#70878=CARTESIAN_POINT('Ctrl Pts',(-16.9100714880367,-71.6821155085605,
0.));
#70879=CARTESIAN_POINT('Ctrl Pts',(-16.9100714880367,-71.6821155085605,
12.));
#70880=CARTESIAN_POINT('Ctrl Pts',(-16.9054084476847,-71.7084961763355,
0.));
#70881=CARTESIAN_POINT('Ctrl Pts',(-16.9054084476847,-71.7084961763355,
12.));
#70882=CARTESIAN_POINT('Ctrl Pts',(-16.9007147618344,-71.7349085335796,
0.));
#70883=CARTESIAN_POINT('Ctrl Pts',(-16.9007147618344,-71.7349085335796,
12.));
#70884=CARTESIAN_POINT('Ctrl Pts',(-16.895990398841,-71.761352481924,0.));
#70885=CARTESIAN_POINT('Ctrl Pts',(-16.895990398841,-71.761352481924,12.));
#70886=CARTESIAN_POINT('Ctrl Pts',(-16.8912353270944,-71.7878279229556,
0.));
#70887=CARTESIAN_POINT('Ctrl Pts',(-16.8912353270944,-71.7878279229556,
12.));
#70888=CARTESIAN_POINT('Ctrl Pts',(-16.8864495151347,-71.8143347584977,
0.));
#70889=CARTESIAN_POINT('Ctrl Pts',(-16.8864495151347,-71.8143347584977,
12.));
#70890=CARTESIAN_POINT('Ctrl Pts',(-16.8816329317473,-71.8408728908269,
0.));
#70891=CARTESIAN_POINT('Ctrl Pts',(-16.8816329317473,-71.8408728908269,
12.));
#70892=CARTESIAN_POINT('Ctrl Pts',(-16.87678554607,-71.8674422229151,0.));
#70893=CARTESIAN_POINT('Ctrl Pts',(-16.87678554607,-71.8674422229151,12.));
#70894=CARTESIAN_POINT('Ctrl Pts',(-16.8719073276967,-71.8940426586521,
0.));
#70895=CARTESIAN_POINT('Ctrl Pts',(-16.8719073276967,-71.8940426586521,
12.));
#70896=CARTESIAN_POINT('Ctrl Pts',(-16.8669982467915,-71.920674103086,0.));
#70897=CARTESIAN_POINT('Ctrl Pts',(-16.8669982467915,-71.920674103086,12.));
#70898=CARTESIAN_POINT('Ctrl Pts',(-16.862058273843,-71.9473364618889,0.));
#70899=CARTESIAN_POINT('Ctrl Pts',(-16.862058273843,-71.9473364618889,12.));
#70900=CARTESIAN_POINT('Ctrl Pts',(-16.8570873794264,-71.9740296408319,
0.));
#70901=CARTESIAN_POINT('Ctrl Pts',(-16.8570873794264,-71.9740296408319,
12.));
#70902=CARTESIAN_POINT('Ctrl Pts',(-16.8520855339444,-72.0007535452071,
0.));
#70903=CARTESIAN_POINT('Ctrl Pts',(-16.8520855339444,-72.0007535452071,
12.));
#70904=CARTESIAN_POINT('Ctrl Pts',(-16.8470527074278,-72.0275080793742,
0.));
#70905=CARTESIAN_POINT('Ctrl Pts',(-16.8470527074278,-72.0275080793742,
12.));
#70906=CARTESIAN_POINT('Ctrl Pts',(-16.8419888691984,-72.0542931459865,
0.));
#70907=CARTESIAN_POINT('Ctrl Pts',(-16.8419888691984,-72.0542931459865,
12.));
#70908=CARTESIAN_POINT('Ctrl Pts',(-16.8368939881457,-72.0811086466177,
0.));
#70909=CARTESIAN_POINT('Ctrl Pts',(-16.8368939881457,-72.0811086466177,
12.));
#70910=CARTESIAN_POINT('Ctrl Pts',(-16.8317680333415,-72.1079544831568,
0.));
#70911=CARTESIAN_POINT('Ctrl Pts',(-16.8317680333415,-72.1079544831568,
12.));
#70912=CARTESIAN_POINT('Ctrl Pts',(-16.8266109745801,-72.1348305590233,
0.));
#70913=CARTESIAN_POINT('Ctrl Pts',(-16.8266109745801,-72.1348305590233,
12.));
#70914=CARTESIAN_POINT('Ctrl Pts',(-16.8214227828941,-72.1617367803226,
0.));
#70915=CARTESIAN_POINT('Ctrl Pts',(-16.8214227828941,-72.1617367803226,
12.));
#70916=CARTESIAN_POINT('Ctrl Pts',(-16.8162034312257,-72.1886730573389,
0.));
#70917=CARTESIAN_POINT('Ctrl Pts',(-16.8162034312257,-72.1886730573389,
12.));
#70918=CARTESIAN_POINT('Ctrl Pts',(-16.8109528945876,-72.2156393048868,
0.));
#70919=CARTESIAN_POINT('Ctrl Pts',(-16.8109528945876,-72.2156393048868,
12.));
#70920=CARTESIAN_POINT('Ctrl Pts',(-16.8056711485797,-72.242635439009,0.));
#70921=CARTESIAN_POINT('Ctrl Pts',(-16.8056711485797,-72.242635439009,12.));
#70922=CARTESIAN_POINT('Ctrl Pts',(-16.800358168223,-72.2696613743687,0.));
#70923=CARTESIAN_POINT('Ctrl Pts',(-16.800358168223,-72.2696613743687,12.));
#70924=CARTESIAN_POINT('Ctrl Pts',(-16.7950139266117,-72.2967170212331,
0.));
#70925=CARTESIAN_POINT('Ctrl Pts',(-16.7950139266117,-72.2967170212331,
12.));
#70926=CARTESIAN_POINT('Ctrl Pts',(-16.7896383937839,-72.323802282931,0.));
#70927=CARTESIAN_POINT('Ctrl Pts',(-16.7896383937839,-72.323802282931,12.));
#70928=CARTESIAN_POINT('Ctrl Pts',(-16.7842315351401,-72.3509170523038,
0.));
#70929=CARTESIAN_POINT('Ctrl Pts',(-16.7842315351401,-72.3509170523038,
12.));
#70930=CARTESIAN_POINT('Ctrl Pts',(-16.7787933137551,-72.3780612168057,
0.));
#70931=CARTESIAN_POINT('Ctrl Pts',(-16.7787933137551,-72.3780612168057,
12.));
#70932=CARTESIAN_POINT('Ctrl Pts',(-16.7733236932185,-72.4052346648058,
0.));
#70933=CARTESIAN_POINT('Ctrl Pts',(-16.7733236932185,-72.4052346648058,
12.));
#70934=CARTESIAN_POINT('Ctrl Pts',(-16.7678226404189,-72.4324372916884,
0.));
#70935=CARTESIAN_POINT('Ctrl Pts',(-16.7678226404189,-72.4324372916884,
12.));
#70936=CARTESIAN_POINT('Ctrl Pts',(-16.7622901280741,-72.4596690055347,
0.));
#70937=CARTESIAN_POINT('Ctrl Pts',(-16.7622901280741,-72.4596690055347,
12.));
#70938=CARTESIAN_POINT('Ctrl Pts',(-16.7567261380614,-72.4869297342051,
0.));
#70939=CARTESIAN_POINT('Ctrl Pts',(-16.7567261380614,-72.4869297342051,
12.));
#70940=CARTESIAN_POINT('Ctrl Pts',(-16.7511306618793,-72.5142194273203,
0.));
#70941=CARTESIAN_POINT('Ctrl Pts',(-16.7511306618793,-72.5142194273203,
12.));
#70942=CARTESIAN_POINT('Ctrl Pts',(-16.7455036973724,-72.5415380515905,
0.));
#70943=CARTESIAN_POINT('Ctrl Pts',(-16.7455036973724,-72.5415380515905,
12.));
#70944=CARTESIAN_POINT('Ctrl Pts',(-16.7409769365953,-72.563416080574,0.));
#70945=CARTESIAN_POINT('Ctrl Pts',(-16.7409769365953,-72.563416080574,12.));
#70946=CARTESIAN_POINT('Ctrl Pts',(-16.7375676985272,-72.5798376087406,
0.));
#70947=CARTESIAN_POINT('Ctrl Pts',(-16.7375676985272,-72.5798376087406,
12.));
#70948=CARTESIAN_POINT('Ctrl Pts',(-16.7352885767459,-72.5907910745874,
0.));
#70949=CARTESIAN_POINT('Ctrl Pts',(-16.7352885767459,-72.5907910745874,
12.));
#70950=CARTESIAN_POINT('Ctrl Pts',(-16.7341474417544,-72.5962692526112,
0.));
#70951=CARTESIAN_POINT('Ctrl Pts',(-16.7341474417544,-72.5962692526112,
12.));
#70952=CARTESIAN_POINT('',(-17.2912529479484,-67.8307641965655,0.));
#70953=CARTESIAN_POINT('Ctrl Pts',(-17.2912529479484,-67.8307641965655,
0.));
#70954=CARTESIAN_POINT('Ctrl Pts',(-17.2912149114119,-67.8346476309018,
0.));
#70955=CARTESIAN_POINT('Ctrl Pts',(-17.2911366591347,-67.842419897098,0.));
#70956=CARTESIAN_POINT('Ctrl Pts',(-17.291012743109,-67.8540944889687,0.));
#70957=CARTESIAN_POINT('Ctrl Pts',(-17.2908344459694,-67.8696929978782,
0.));
#70958=CARTESIAN_POINT('Ctrl Pts',(-17.2905897723948,-67.8892451049608,
0.));
#70959=CARTESIAN_POINT('Ctrl Pts',(-17.2903232740694,-67.9088511496686,
0.));
#70960=CARTESIAN_POINT('Ctrl Pts',(-17.2900349103981,-67.9285110571741,
0.));
#70961=CARTESIAN_POINT('Ctrl Pts',(-17.2897246158941,-67.9482246901667,
0.));
#70962=CARTESIAN_POINT('Ctrl Pts',(-17.2893923013894,-67.9679918502579,
0.));
#70963=CARTESIAN_POINT('Ctrl Pts',(-17.2890378644866,-67.987812304921,0.));
#70964=CARTESIAN_POINT('Ctrl Pts',(-17.28866119774,-68.007685808115,0.));
#70965=CARTESIAN_POINT('Ctrl Pts',(-17.2882621974721,-68.0276121227356,
0.));
#70966=CARTESIAN_POINT('Ctrl Pts',(-17.2878407730961,-68.0475910442424,
0.));
#70967=CARTESIAN_POINT('Ctrl Pts',(-17.2873968440839,-68.0676223930412,
0.));
#70968=CARTESIAN_POINT('Ctrl Pts',(-17.2869303355432,-68.0877060033205,
0.));
#70969=CARTESIAN_POINT('Ctrl Pts',(-17.2864411745459,-68.1078417137877,
0.));
#70970=CARTESIAN_POINT('Ctrl Pts',(-17.2859292855705,-68.1280293561511,
0.));
#70971=CARTESIAN_POINT('Ctrl Pts',(-17.2853945882072,-68.1482687493226,
0.));
#70972=CARTESIAN_POINT('Ctrl Pts',(-17.2848369995293,-68.1685597054232,
0.));
#70973=CARTESIAN_POINT('Ctrl Pts',(-17.2842564355799,-68.1889020335427,
0.));
#70974=CARTESIAN_POINT('Ctrl Pts',(-17.2836528130819,-68.2092955440567,
0.));
#70975=CARTESIAN_POINT('Ctrl Pts',(-17.2830260513867,-68.2297400535294,
0.));
#70976=CARTESIAN_POINT('Ctrl Pts',(-17.2823760723874,-68.2502353845071,
0.));
#70977=CARTESIAN_POINT('Ctrl Pts',(-17.2817027995831,-68.2707813631731,
0.));
#70978=CARTESIAN_POINT('Ctrl Pts',(-17.2810061574353,-68.2913778177261,
0.));
#70979=CARTESIAN_POINT('Ctrl Pts',(-17.2802860705815,-68.3120245763914,
0.));
#70980=CARTESIAN_POINT('Ctrl Pts',(-17.2795424631799,-68.3327214657575,
0.));
#70981=CARTESIAN_POINT('Ctrl Pts',(-17.2787752592484,-68.3534683116515,
0.));
#70982=CARTESIAN_POINT('Ctrl Pts',(-17.2779843829608,-68.3742649398964,
0.));
#70983=CARTESIAN_POINT('Ctrl Pts',(-17.2771697589384,-68.3951111770487,
0.));
#70984=CARTESIAN_POINT('Ctrl Pts',(-17.2763313126018,-68.4160068512753,
0.));
#70985=CARTESIAN_POINT('Ctrl Pts',(-17.2754689702992,-68.436951792677,0.));
#70986=CARTESIAN_POINT('Ctrl Pts',(-17.2745826591119,-68.4579458328185,
0.));
#70987=CARTESIAN_POINT('Ctrl Pts',(-17.2736723067365,-68.4789888044351,
0.));
#70988=CARTESIAN_POINT('Ctrl Pts',(-17.2727378413489,-68.5000805410911,
0.));
#70989=CARTESIAN_POINT('Ctrl Pts',(-17.2717791914544,-68.521220876786,0.));
#70990=CARTESIAN_POINT('Ctrl Pts',(-17.2707962858919,-68.5424096459772,
0.));
#70991=CARTESIAN_POINT('Ctrl Pts',(-17.269789053896,-68.5636466837517,0.));
#70992=CARTESIAN_POINT('Ctrl Pts',(-17.2687574251428,-68.5849318259449,
0.));
#70993=CARTESIAN_POINT('Ctrl Pts',(-17.2677013298057,-68.6062649092764,
0.));
#70994=CARTESIAN_POINT('Ctrl Pts',(-17.2666206986084,-68.6276457714729,
0.));
#70995=CARTESIAN_POINT('Ctrl Pts',(-17.2655154627928,-68.6490742512057,
0.));
#70996=CARTESIAN_POINT('Ctrl Pts',(-17.2643855540892,-68.6705501880249,
0.));
#70997=CARTESIAN_POINT('Ctrl Pts',(-17.2632309046892,-68.6920734222938,
0.));
#70998=CARTESIAN_POINT('Ctrl Pts',(-17.2620514472182,-68.7136437951097,
0.));
#70999=CARTESIAN_POINT('Ctrl Pts',(-17.2608471147185,-68.7352611482547,
0.));
#71000=CARTESIAN_POINT('Ctrl Pts',(-17.259617840655,-68.7569253242333,0.));
#71001=CARTESIAN_POINT('Ctrl Pts',(-17.2583635589198,-68.7786361662882,
0.));
#71002=CARTESIAN_POINT('Ctrl Pts',(-17.2570842038383,-68.8003935184184,
0.));
#71003=CARTESIAN_POINT('Ctrl Pts',(-17.2557797101812,-68.8221972253941,
0.));
#71004=CARTESIAN_POINT('Ctrl Pts',(-17.2544500131624,-68.844047132755,0.));
#71005=CARTESIAN_POINT('Ctrl Pts',(-17.2530950484258,-68.8659430867972,
0.));
#71006=CARTESIAN_POINT('Ctrl Pts',(-17.2517147520376,-68.8878849345557,
0.));
#71007=CARTESIAN_POINT('Ctrl Pts',(-17.2503090604792,-68.909872523787,0.));
#71008=CARTESIAN_POINT('Ctrl Pts',(-17.248877910643,-68.9319057029409,0.));
#71009=CARTESIAN_POINT('Ctrl Pts',(-17.2474212398275,-68.9539843211619,
0.));
#71010=CARTESIAN_POINT('Ctrl Pts',(-17.2459389857327,-68.9761082282922,
0.));
#71011=CARTESIAN_POINT('Ctrl Pts',(-17.2444310864585,-68.9982772748694,
0.));
#71012=CARTESIAN_POINT('Ctrl Pts',(-17.2428974805044,-69.0204913121225,
0.));
#71013=CARTESIAN_POINT('Ctrl Pts',(-17.2413381067723,-69.0427501919636,
0.));
#71014=CARTESIAN_POINT('Ctrl Pts',(-17.2397529045589,-69.065053766986,0.));
#71015=CARTESIAN_POINT('Ctrl Pts',(-17.238141813549,-69.0874018904599,0.));
#71016=CARTESIAN_POINT('Ctrl Pts',(-17.2365047738125,-69.1097944163245,
0.));
#71017=CARTESIAN_POINT('Ctrl Pts',(-17.2348417258015,-69.1322311991752,
0.));
#71018=CARTESIAN_POINT('Ctrl Pts',(-17.2331526103506,-69.1547120942527,
0.));
#71019=CARTESIAN_POINT('Ctrl Pts',(-17.23143736867,-69.1772369574447,0.));
#71020=CARTESIAN_POINT('Ctrl Pts',(-17.2296959423407,-69.1998056452828,
0.));
#71021=CARTESIAN_POINT('Ctrl Pts',(-17.227928273312,-69.222418014938,0.));
#71022=CARTESIAN_POINT('Ctrl Pts',(-17.226134303902,-69.2450739242109,0.));
#71023=CARTESIAN_POINT('Ctrl Pts',(-17.224313976797,-69.2677732315224,0.));
#71024=CARTESIAN_POINT('Ctrl Pts',(-17.2224672350438,-69.2905157959166,
0.));
#71025=CARTESIAN_POINT('Ctrl Pts',(-17.2205940220459,-69.3133014770555,
0.));
#71026=CARTESIAN_POINT('Ctrl Pts',(-17.2186942815602,-69.3361301352141,
0.));
#71027=CARTESIAN_POINT('Ctrl Pts',(-17.2167679576984,-69.3590016312692,
0.));
#71028=CARTESIAN_POINT('Ctrl Pts',(-17.2148149949252,-69.3819158266916,
0.));
#71029=CARTESIAN_POINT('Ctrl Pts',(-17.2128353380502,-69.404872583548,0.));
#71030=CARTESIAN_POINT('Ctrl Pts',(-17.2108289322254,-69.4278717644973,
0.));
#71031=CARTESIAN_POINT('Ctrl Pts',(-17.2087957229423,-69.450913232785,0.));
#71032=CARTESIAN_POINT('Ctrl Pts',(-17.2067356560336,-69.4739968522313,
0.));
#71033=CARTESIAN_POINT('Ctrl Pts',(-17.2046486776708,-69.4971224872269,
0.));
#71034=CARTESIAN_POINT('Ctrl Pts',(-17.2025347343577,-69.5202900027367,
0.));
#71035=CARTESIAN_POINT('Ctrl Pts',(-17.2003937729268,-69.5434992642944,
0.));
#71036=CARTESIAN_POINT('Ctrl Pts',(-17.1982257405377,-69.5667501379969,
0.));
#71037=CARTESIAN_POINT('Ctrl Pts',(-17.196030584678,-69.5900424904921,0.));
#71038=CARTESIAN_POINT('Ctrl Pts',(-17.1938082531612,-69.6133761889748,
0.));
#71039=CARTESIAN_POINT('Ctrl Pts',(-17.1915586941192,-69.6367511011898,
0.));
#71040=CARTESIAN_POINT('Ctrl Pts',(-17.1892818560002,-69.6601670954269,
0.));
#71041=CARTESIAN_POINT('Ctrl Pts',(-17.1869776875666,-69.6836240405164,
0.));
#71042=CARTESIAN_POINT('Ctrl Pts',(-17.1846461378973,-69.7071218058178,
0.));
#71043=CARTESIAN_POINT('Ctrl Pts',(-17.1822871563842,-69.7306602612155,
0.));
#71044=CARTESIAN_POINT('Ctrl Pts',(-17.179900692726,-69.7542392771234,0.));
#71045=CARTESIAN_POINT('Ctrl Pts',(-17.1774866969256,-69.777858724479,0.));
#71046=CARTESIAN_POINT('Ctrl Pts',(-17.1750451192885,-69.8015184747398,
0.));
#71047=CARTESIAN_POINT('Ctrl Pts',(-17.1725759104251,-69.8252183998702,
0.));
#71048=CARTESIAN_POINT('Ctrl Pts',(-17.1700790212473,-69.8489583723407,
0.));
#71049=CARTESIAN_POINT('Ctrl Pts',(-17.167554402962,-69.8727382651286,0.));
#71050=CARTESIAN_POINT('Ctrl Pts',(-17.1650020070686,-69.8965579517147,
0.));
#71051=CARTESIAN_POINT('Ctrl Pts',(-17.1624217853578,-69.9204173060781,
0.));
#71052=CARTESIAN_POINT('Ctrl Pts',(-17.1598136899144,-69.9443162026865,
0.));
#71053=CARTESIAN_POINT('Ctrl Pts',(-17.1571776731139,-69.9682545164939,
0.));
#71054=CARTESIAN_POINT('Ctrl Pts',(-17.154513687616,-69.9922321229424,0.));
#71055=CARTESIAN_POINT('Ctrl Pts',(-17.1518216863623,-70.0162488979584,
0.));
#71056=CARTESIAN_POINT('Ctrl Pts',(-17.1491016225749,-70.0403047179483,
0.));
#71057=CARTESIAN_POINT('Ctrl Pts',(-17.1463534497594,-70.0643994597873,
0.));
#71058=CARTESIAN_POINT('Ctrl Pts',(-17.1435771217018,-70.0885330008179,
0.));
#71059=CARTESIAN_POINT('Ctrl Pts',(-17.1407725924617,-70.1127052188522,
0.));
#71060=CARTESIAN_POINT('Ctrl Pts',(-17.1379398163709,-70.1369159921687,
0.));
#71061=CARTESIAN_POINT('Ctrl Pts',(-17.1350787480312,-70.1611651995083,
0.));
#71062=CARTESIAN_POINT('Ctrl Pts',(-17.1321893423182,-70.1854527200631,
0.));
#71063=CARTESIAN_POINT('Ctrl Pts',(-17.1292715543778,-70.2097784334747,
0.));
#71064=CARTESIAN_POINT('Ctrl Pts',(-17.1263253396202,-70.2341422198363,
0.));
#71065=CARTESIAN_POINT('Ctrl Pts',(-17.1233506537176,-70.2585439596901,
0.));
#71066=CARTESIAN_POINT('Ctrl Pts',(-17.1203474526031,-70.2829835340238,
0.));
#71067=CARTESIAN_POINT('Ctrl Pts',(-17.1173156924733,-70.3074608242608,
0.));
#71068=CARTESIAN_POINT('Ctrl Pts',(-17.1142553297867,-70.3319757122568,
0.));
#71069=CARTESIAN_POINT('Ctrl Pts',(-17.1111663212568,-70.3565280803022,
0.));
#71070=CARTESIAN_POINT('Ctrl Pts',(-17.1080486238499,-70.3811178111201,
0.));
#71071=CARTESIAN_POINT('Ctrl Pts',(-17.1049021947834,-70.4057447878624,
0.));
#71072=CARTESIAN_POINT('Ctrl Pts',(-17.1017269915292,-70.430408894101,0.));
#71073=CARTESIAN_POINT('Ctrl Pts',(-17.0985229718124,-70.4551100138238,
0.));
#71074=CARTESIAN_POINT('Ctrl Pts',(-17.0952900936048,-70.4798480314381,
0.));
#71075=CARTESIAN_POINT('Ctrl Pts',(-17.0920283151219,-70.5046228317677,
0.));
#71076=CARTESIAN_POINT('Ctrl Pts',(-17.088737594822,-70.5294343000513,0.));
#71077=CARTESIAN_POINT('Ctrl Pts',(-17.0854178914087,-70.5542823219331,
0.));
#71078=CARTESIAN_POINT('Ctrl Pts',(-17.082069163831,-70.5791667834582,0.));
#71079=CARTESIAN_POINT('Ctrl Pts',(-17.0786913712763,-70.6040875710749,
0.));
#71080=CARTESIAN_POINT('Ctrl Pts',(-17.0752844731678,-70.6290445716337,
0.));
#71081=CARTESIAN_POINT('Ctrl Pts',(-17.0718484291624,-70.6540376723841,
0.));
#71082=CARTESIAN_POINT('Ctrl Pts',(-17.0683831991532,-70.6790667609679,
0.));
#71083=CARTESIAN_POINT('Ctrl Pts',(-17.0648887432713,-70.7041317254125,
0.));
#71084=CARTESIAN_POINT('Ctrl Pts',(-17.0613650218787,-70.7292324541341,
0.));
#71085=CARTESIAN_POINT('Ctrl Pts',(-17.0578119955649,-70.7543688359374,
0.));
#71086=CARTESIAN_POINT('Ctrl Pts',(-17.0542296251462,-70.7795407600127,
0.));
#71087=CARTESIAN_POINT('Ctrl Pts',(-17.0506178716664,-70.8047481159306,
0.));
#71088=CARTESIAN_POINT('Ctrl Pts',(-17.0469766964005,-70.8299907936346,
0.));
#71089=CARTESIAN_POINT('Ctrl Pts',(-17.0433060608478,-70.8552686834435,
0.));
#71090=CARTESIAN_POINT('Ctrl Pts',(-17.0396059267279,-70.8805816760507,
0.));
#71091=CARTESIAN_POINT('Ctrl Pts',(-17.0358762559786,-70.9059296625214,
0.));
#71092=CARTESIAN_POINT('Ctrl Pts',(-17.0321170107562,-70.9313125342872,
0.));
#71093=CARTESIAN_POINT('Ctrl Pts',(-17.028328153439,-70.9567301831355,0.));
#71094=CARTESIAN_POINT('Ctrl Pts',(-17.0245096466228,-70.9821825012134,
0.));
#71095=CARTESIAN_POINT('Ctrl Pts',(-17.0206614531165,-71.0076693810303,
0.));
#71096=CARTESIAN_POINT('Ctrl Pts',(-17.0167835359419,-71.0331907154575,
0.));
#71097=CARTESIAN_POINT('Ctrl Pts',(-17.0128758583335,-71.0587463977266,
0.));
#71098=CARTESIAN_POINT('Ctrl Pts',(-17.0089383837436,-71.0843363214216,
0.));
#71099=CARTESIAN_POINT('Ctrl Pts',(-17.0049710758393,-71.1099603804779,
0.));
#71100=CARTESIAN_POINT('Ctrl Pts',(-17.0009738984935,-71.1356184691799,
0.));
#71101=CARTESIAN_POINT('Ctrl Pts',(-16.9969468157824,-71.1613104821565,
0.));
#71102=CARTESIAN_POINT('Ctrl Pts',(-16.9928897919829,-71.1870363143742,
0.));
#71103=CARTESIAN_POINT('Ctrl Pts',(-16.9888027915743,-71.2127958611248,
0.));
#71104=CARTESIAN_POINT('Ctrl Pts',(-16.9846857792385,-71.2385890180233,
0.));
#71105=CARTESIAN_POINT('Ctrl Pts',(-16.9805387198573,-71.2644156810209,
0.));
#71106=CARTESIAN_POINT('Ctrl Pts',(-16.9763615785137,-71.2902757464127,
0.));
#71107=CARTESIAN_POINT('Ctrl Pts',(-16.9721543204951,-71.3161691108425,
0.));
#71108=CARTESIAN_POINT('Ctrl Pts',(-16.9679169112993,-71.3420956713072,
0.));
#71109=CARTESIAN_POINT('Ctrl Pts',(-16.9636493166395,-71.3680553251548,
0.));
#71110=CARTESIAN_POINT('Ctrl Pts',(-16.9593515024274,-71.3940479700663,
0.));
#71111=CARTESIAN_POINT('Ctrl Pts',(-16.9550234347619,-71.4200735040374,
0.));
#71112=CARTESIAN_POINT('Ctrl Pts',(-16.9506650799188,-71.4461318253561,
0.));
#71113=CARTESIAN_POINT('Ctrl Pts',(-16.9462764043445,-71.4722228325805,
0.));
#71114=CARTESIAN_POINT('Ctrl Pts',(-16.9418573746492,-71.498346424507,0.));
#71115=CARTESIAN_POINT('Ctrl Pts',(-16.9374079576204,-71.5245025002154,
0.));
#71116=CARTESIAN_POINT('Ctrl Pts',(-16.9329281202379,-71.5506909591139,
0.));
#71117=CARTESIAN_POINT('Ctrl Pts',(-16.9284178296934,-71.5769117009844,
0.));
#71118=CARTESIAN_POINT('Ctrl Pts',(-16.923877053407,-71.6031646260169,0.));
#71119=CARTESIAN_POINT('Ctrl Pts',(-16.9193057590605,-71.6294496348644,
0.));
#71120=CARTESIAN_POINT('Ctrl Pts',(-16.9147039145715,-71.6557666285908,
0.));
#71121=CARTESIAN_POINT('Ctrl Pts',(-16.9100714880367,-71.6821155085605,
0.));
#71122=CARTESIAN_POINT('Ctrl Pts',(-16.9054084476847,-71.7084961763355,
0.));
#71123=CARTESIAN_POINT('Ctrl Pts',(-16.9007147618344,-71.7349085335796,
0.));
#71124=CARTESIAN_POINT('Ctrl Pts',(-16.895990398841,-71.761352481924,0.));
#71125=CARTESIAN_POINT('Ctrl Pts',(-16.8912353270944,-71.7878279229556,
0.));
#71126=CARTESIAN_POINT('Ctrl Pts',(-16.8864495151347,-71.8143347584977,
0.));
#71127=CARTESIAN_POINT('Ctrl Pts',(-16.8816329317473,-71.8408728908269,
0.));
#71128=CARTESIAN_POINT('Ctrl Pts',(-16.87678554607,-71.8674422229151,0.));
#71129=CARTESIAN_POINT('Ctrl Pts',(-16.8719073276967,-71.8940426586521,
0.));
#71130=CARTESIAN_POINT('Ctrl Pts',(-16.8669982467915,-71.920674103086,0.));
#71131=CARTESIAN_POINT('Ctrl Pts',(-16.862058273843,-71.9473364618889,0.));
#71132=CARTESIAN_POINT('Ctrl Pts',(-16.8570873794264,-71.9740296408319,
0.));
#71133=CARTESIAN_POINT('Ctrl Pts',(-16.8520855339444,-72.0007535452071,
0.));
#71134=CARTESIAN_POINT('Ctrl Pts',(-16.8470527074278,-72.0275080793742,
0.));
#71135=CARTESIAN_POINT('Ctrl Pts',(-16.8419888691984,-72.0542931459865,
0.));
#71136=CARTESIAN_POINT('Ctrl Pts',(-16.8368939881457,-72.0811086466177,
0.));
#71137=CARTESIAN_POINT('Ctrl Pts',(-16.8317680333415,-72.1079544831568,
0.));
#71138=CARTESIAN_POINT('Ctrl Pts',(-16.8266109745801,-72.1348305590233,
0.));
#71139=CARTESIAN_POINT('Ctrl Pts',(-16.8214227828941,-72.1617367803226,
0.));
#71140=CARTESIAN_POINT('Ctrl Pts',(-16.8162034312257,-72.1886730573389,
0.));
#71141=CARTESIAN_POINT('Ctrl Pts',(-16.8109528945876,-72.2156393048868,
0.));
#71142=CARTESIAN_POINT('Ctrl Pts',(-16.8064254147766,-72.2387802230663,
0.));
#71143=CARTESIAN_POINT('Ctrl Pts',(-16.8029374213802,-72.2565380035009,
0.));
#71144=CARTESIAN_POINT('Ctrl Pts',(-16.8005027425888,-72.2688994294961,
0.));
#71145=CARTESIAN_POINT('Ctrl Pts',(-16.7991305317792,-72.275855789097,0.));
#71146=CARTESIAN_POINT('Ctrl Pts',(-16.7988252568806,-72.2774028393486,
0.));
#71147=CARTESIAN_POINT('',(-17.2912529479484,-67.8307641965655,12.));
#71148=CARTESIAN_POINT('',(-17.2912529479484,-67.8307641965655,0.));
#71149=CARTESIAN_POINT('Ctrl Pts',(-16.7988252568806,-72.2774028393486,
12.));
#71150=CARTESIAN_POINT('Ctrl Pts',(-16.7991305317792,-72.275855789097,12.));
#71151=CARTESIAN_POINT('Ctrl Pts',(-16.8005027425888,-72.2688994294961,
12.));
#71152=CARTESIAN_POINT('Ctrl Pts',(-16.8029374213802,-72.2565380035009,
12.));
#71153=CARTESIAN_POINT('Ctrl Pts',(-16.8064254147766,-72.2387802230663,
12.));
#71154=CARTESIAN_POINT('Ctrl Pts',(-16.8109528945876,-72.2156393048868,
12.));
#71155=CARTESIAN_POINT('Ctrl Pts',(-16.8162034312257,-72.1886730573389,
12.));
#71156=CARTESIAN_POINT('Ctrl Pts',(-16.8214227828941,-72.1617367803226,
12.));
#71157=CARTESIAN_POINT('Ctrl Pts',(-16.8266109745801,-72.1348305590233,
12.));
#71158=CARTESIAN_POINT('Ctrl Pts',(-16.8317680333415,-72.1079544831568,
12.));
#71159=CARTESIAN_POINT('Ctrl Pts',(-16.8368939881457,-72.0811086466177,
12.));
#71160=CARTESIAN_POINT('Ctrl Pts',(-16.8419888691984,-72.0542931459865,
12.));
#71161=CARTESIAN_POINT('Ctrl Pts',(-16.8470527074278,-72.0275080793742,
12.));
#71162=CARTESIAN_POINT('Ctrl Pts',(-16.8520855339444,-72.0007535452071,
12.));
#71163=CARTESIAN_POINT('Ctrl Pts',(-16.8570873794264,-71.9740296408319,
12.));
#71164=CARTESIAN_POINT('Ctrl Pts',(-16.862058273843,-71.9473364618889,12.));
#71165=CARTESIAN_POINT('Ctrl Pts',(-16.8669982467915,-71.920674103086,12.));
#71166=CARTESIAN_POINT('Ctrl Pts',(-16.8719073276967,-71.8940426586521,
12.));
#71167=CARTESIAN_POINT('Ctrl Pts',(-16.87678554607,-71.8674422229151,12.));
#71168=CARTESIAN_POINT('Ctrl Pts',(-16.8816329317473,-71.8408728908269,
12.));
#71169=CARTESIAN_POINT('Ctrl Pts',(-16.8864495151347,-71.8143347584977,
12.));
#71170=CARTESIAN_POINT('Ctrl Pts',(-16.8912353270944,-71.7878279229556,
12.));
#71171=CARTESIAN_POINT('Ctrl Pts',(-16.895990398841,-71.761352481924,12.));
#71172=CARTESIAN_POINT('Ctrl Pts',(-16.9007147618344,-71.7349085335796,
12.));
#71173=CARTESIAN_POINT('Ctrl Pts',(-16.9054084476847,-71.7084961763355,
12.));
#71174=CARTESIAN_POINT('Ctrl Pts',(-16.9100714880367,-71.6821155085605,
12.));
#71175=CARTESIAN_POINT('Ctrl Pts',(-16.9147039145715,-71.6557666285908,
12.));
#71176=CARTESIAN_POINT('Ctrl Pts',(-16.9193057590605,-71.6294496348644,
12.));
#71177=CARTESIAN_POINT('Ctrl Pts',(-16.923877053407,-71.6031646260169,12.));
#71178=CARTESIAN_POINT('Ctrl Pts',(-16.9284178296934,-71.5769117009844,
12.));
#71179=CARTESIAN_POINT('Ctrl Pts',(-16.9329281202379,-71.5506909591139,
12.));
#71180=CARTESIAN_POINT('Ctrl Pts',(-16.9374079576204,-71.5245025002154,
12.));
#71181=CARTESIAN_POINT('Ctrl Pts',(-16.9418573746492,-71.498346424507,12.));
#71182=CARTESIAN_POINT('Ctrl Pts',(-16.9462764043445,-71.4722228325805,
12.));
#71183=CARTESIAN_POINT('Ctrl Pts',(-16.9506650799188,-71.4461318253561,
12.));
#71184=CARTESIAN_POINT('Ctrl Pts',(-16.9550234347619,-71.4200735040374,
12.));
#71185=CARTESIAN_POINT('Ctrl Pts',(-16.9593515024274,-71.3940479700663,
12.));
#71186=CARTESIAN_POINT('Ctrl Pts',(-16.9636493166395,-71.3680553251548,
12.));
#71187=CARTESIAN_POINT('Ctrl Pts',(-16.9679169112993,-71.3420956713072,
12.));
#71188=CARTESIAN_POINT('Ctrl Pts',(-16.9721543204951,-71.3161691108425,
12.));
#71189=CARTESIAN_POINT('Ctrl Pts',(-16.9763615785137,-71.2902757464127,
12.));
#71190=CARTESIAN_POINT('Ctrl Pts',(-16.9805387198573,-71.2644156810209,
12.));
#71191=CARTESIAN_POINT('Ctrl Pts',(-16.9846857792385,-71.2385890180233,
12.));
#71192=CARTESIAN_POINT('Ctrl Pts',(-16.9888027915743,-71.2127958611248,
12.));
#71193=CARTESIAN_POINT('Ctrl Pts',(-16.9928897919829,-71.1870363143742,
12.));
#71194=CARTESIAN_POINT('Ctrl Pts',(-16.9969468157824,-71.1613104821565,
12.));
#71195=CARTESIAN_POINT('Ctrl Pts',(-17.0009738984935,-71.1356184691799,
12.));
#71196=CARTESIAN_POINT('Ctrl Pts',(-17.0049710758393,-71.1099603804779,
12.));
#71197=CARTESIAN_POINT('Ctrl Pts',(-17.0089383837436,-71.0843363214216,
12.));
#71198=CARTESIAN_POINT('Ctrl Pts',(-17.0128758583335,-71.0587463977266,
12.));
#71199=CARTESIAN_POINT('Ctrl Pts',(-17.0167835359419,-71.0331907154575,
12.));
#71200=CARTESIAN_POINT('Ctrl Pts',(-17.0206614531165,-71.0076693810303,
12.));
#71201=CARTESIAN_POINT('Ctrl Pts',(-17.0245096466228,-70.9821825012134,
12.));
#71202=CARTESIAN_POINT('Ctrl Pts',(-17.028328153439,-70.9567301831355,12.));
#71203=CARTESIAN_POINT('Ctrl Pts',(-17.0321170107562,-70.9313125342872,
12.));
#71204=CARTESIAN_POINT('Ctrl Pts',(-17.0358762559786,-70.9059296625214,
12.));
#71205=CARTESIAN_POINT('Ctrl Pts',(-17.0396059267279,-70.8805816760507,
12.));
#71206=CARTESIAN_POINT('Ctrl Pts',(-17.0433060608478,-70.8552686834435,
12.));
#71207=CARTESIAN_POINT('Ctrl Pts',(-17.0469766964005,-70.8299907936346,
12.));
#71208=CARTESIAN_POINT('Ctrl Pts',(-17.0506178716664,-70.8047481159306,
12.));
#71209=CARTESIAN_POINT('Ctrl Pts',(-17.0542296251462,-70.7795407600127,
12.));
#71210=CARTESIAN_POINT('Ctrl Pts',(-17.0578119955649,-70.7543688359374,
12.));
#71211=CARTESIAN_POINT('Ctrl Pts',(-17.0613650218787,-70.7292324541341,
12.));
#71212=CARTESIAN_POINT('Ctrl Pts',(-17.0648887432713,-70.7041317254125,
12.));
#71213=CARTESIAN_POINT('Ctrl Pts',(-17.0683831991532,-70.6790667609679,
12.));
#71214=CARTESIAN_POINT('Ctrl Pts',(-17.0718484291624,-70.6540376723841,
12.));
#71215=CARTESIAN_POINT('Ctrl Pts',(-17.0752844731678,-70.6290445716337,
12.));
#71216=CARTESIAN_POINT('Ctrl Pts',(-17.0786913712763,-70.6040875710749,
12.));
#71217=CARTESIAN_POINT('Ctrl Pts',(-17.082069163831,-70.5791667834582,12.));
#71218=CARTESIAN_POINT('Ctrl Pts',(-17.0854178914087,-70.5542823219331,
12.));
#71219=CARTESIAN_POINT('Ctrl Pts',(-17.088737594822,-70.5294343000513,12.));
#71220=CARTESIAN_POINT('Ctrl Pts',(-17.0920283151219,-70.5046228317677,
12.));
#71221=CARTESIAN_POINT('Ctrl Pts',(-17.0952900936048,-70.4798480314381,
12.));
#71222=CARTESIAN_POINT('Ctrl Pts',(-17.0985229718124,-70.4551100138238,
12.));
#71223=CARTESIAN_POINT('Ctrl Pts',(-17.1017269915292,-70.430408894101,12.));
#71224=CARTESIAN_POINT('Ctrl Pts',(-17.1049021947834,-70.4057447878624,
12.));
#71225=CARTESIAN_POINT('Ctrl Pts',(-17.1080486238499,-70.3811178111201,
12.));
#71226=CARTESIAN_POINT('Ctrl Pts',(-17.1111663212568,-70.3565280803022,
12.));
#71227=CARTESIAN_POINT('Ctrl Pts',(-17.1142553297867,-70.3319757122568,
12.));
#71228=CARTESIAN_POINT('Ctrl Pts',(-17.1173156924733,-70.3074608242608,
12.));
#71229=CARTESIAN_POINT('Ctrl Pts',(-17.1203474526031,-70.2829835340238,
12.));
#71230=CARTESIAN_POINT('Ctrl Pts',(-17.1233506537176,-70.2585439596901,
12.));
#71231=CARTESIAN_POINT('Ctrl Pts',(-17.1263253396202,-70.2341422198363,
12.));
#71232=CARTESIAN_POINT('Ctrl Pts',(-17.1292715543778,-70.2097784334747,
12.));
#71233=CARTESIAN_POINT('Ctrl Pts',(-17.1321893423182,-70.1854527200631,
12.));
#71234=CARTESIAN_POINT('Ctrl Pts',(-17.1350787480312,-70.1611651995083,
12.));
#71235=CARTESIAN_POINT('Ctrl Pts',(-17.1379398163709,-70.1369159921687,
12.));
#71236=CARTESIAN_POINT('Ctrl Pts',(-17.1407725924617,-70.1127052188522,
12.));
#71237=CARTESIAN_POINT('Ctrl Pts',(-17.1435771217018,-70.0885330008179,
12.));
#71238=CARTESIAN_POINT('Ctrl Pts',(-17.1463534497594,-70.0643994597873,
12.));
#71239=CARTESIAN_POINT('Ctrl Pts',(-17.1491016225749,-70.0403047179483,
12.));
#71240=CARTESIAN_POINT('Ctrl Pts',(-17.1518216863623,-70.0162488979584,
12.));
#71241=CARTESIAN_POINT('Ctrl Pts',(-17.154513687616,-69.9922321229424,12.));
#71242=CARTESIAN_POINT('Ctrl Pts',(-17.1571776731139,-69.9682545164939,
12.));
#71243=CARTESIAN_POINT('Ctrl Pts',(-17.1598136899144,-69.9443162026865,
12.));
#71244=CARTESIAN_POINT('Ctrl Pts',(-17.1624217853578,-69.9204173060781,
12.));
#71245=CARTESIAN_POINT('Ctrl Pts',(-17.1650020070686,-69.8965579517147,
12.));
#71246=CARTESIAN_POINT('Ctrl Pts',(-17.167554402962,-69.8727382651286,12.));
#71247=CARTESIAN_POINT('Ctrl Pts',(-17.1700790212473,-69.8489583723407,
12.));
#71248=CARTESIAN_POINT('Ctrl Pts',(-17.1725759104251,-69.8252183998702,
12.));
#71249=CARTESIAN_POINT('Ctrl Pts',(-17.1750451192885,-69.8015184747398,
12.));
#71250=CARTESIAN_POINT('Ctrl Pts',(-17.1774866969256,-69.777858724479,12.));
#71251=CARTESIAN_POINT('Ctrl Pts',(-17.179900692726,-69.7542392771234,12.));
#71252=CARTESIAN_POINT('Ctrl Pts',(-17.1822871563842,-69.7306602612155,
12.));
#71253=CARTESIAN_POINT('Ctrl Pts',(-17.1846461378973,-69.7071218058178,
12.));
#71254=CARTESIAN_POINT('Ctrl Pts',(-17.1869776875666,-69.6836240405164,
12.));
#71255=CARTESIAN_POINT('Ctrl Pts',(-17.1892818560002,-69.6601670954269,
12.));
#71256=CARTESIAN_POINT('Ctrl Pts',(-17.1915586941192,-69.6367511011898,
12.));
#71257=CARTESIAN_POINT('Ctrl Pts',(-17.1938082531612,-69.6133761889748,
12.));
#71258=CARTESIAN_POINT('Ctrl Pts',(-17.196030584678,-69.5900424904921,12.));
#71259=CARTESIAN_POINT('Ctrl Pts',(-17.1982257405377,-69.5667501379969,
12.));
#71260=CARTESIAN_POINT('Ctrl Pts',(-17.2003937729268,-69.5434992642944,
12.));
#71261=CARTESIAN_POINT('Ctrl Pts',(-17.2025347343577,-69.5202900027367,
12.));
#71262=CARTESIAN_POINT('Ctrl Pts',(-17.2046486776708,-69.4971224872269,
12.));
#71263=CARTESIAN_POINT('Ctrl Pts',(-17.2067356560336,-69.4739968522313,
12.));
#71264=CARTESIAN_POINT('Ctrl Pts',(-17.2087957229423,-69.450913232785,12.));
#71265=CARTESIAN_POINT('Ctrl Pts',(-17.2108289322254,-69.4278717644973,
12.));
#71266=CARTESIAN_POINT('Ctrl Pts',(-17.2128353380502,-69.404872583548,12.));
#71267=CARTESIAN_POINT('Ctrl Pts',(-17.2148149949252,-69.3819158266916,
12.));
#71268=CARTESIAN_POINT('Ctrl Pts',(-17.2167679576984,-69.3590016312692,
12.));
#71269=CARTESIAN_POINT('Ctrl Pts',(-17.2186942815602,-69.3361301352141,
12.));
#71270=CARTESIAN_POINT('Ctrl Pts',(-17.2205940220459,-69.3133014770555,
12.));
#71271=CARTESIAN_POINT('Ctrl Pts',(-17.2224672350438,-69.2905157959166,
12.));
#71272=CARTESIAN_POINT('Ctrl Pts',(-17.224313976797,-69.2677732315224,12.));
#71273=CARTESIAN_POINT('Ctrl Pts',(-17.226134303902,-69.2450739242109,12.));
#71274=CARTESIAN_POINT('Ctrl Pts',(-17.227928273312,-69.222418014938,12.));
#71275=CARTESIAN_POINT('Ctrl Pts',(-17.2296959423407,-69.1998056452828,
12.));
#71276=CARTESIAN_POINT('Ctrl Pts',(-17.23143736867,-69.1772369574447,12.));
#71277=CARTESIAN_POINT('Ctrl Pts',(-17.2331526103506,-69.1547120942527,
12.));
#71278=CARTESIAN_POINT('Ctrl Pts',(-17.2348417258015,-69.1322311991752,
12.));
#71279=CARTESIAN_POINT('Ctrl Pts',(-17.2365047738125,-69.1097944163245,
12.));
#71280=CARTESIAN_POINT('Ctrl Pts',(-17.238141813549,-69.0874018904599,12.));
#71281=CARTESIAN_POINT('Ctrl Pts',(-17.2397529045589,-69.065053766986,12.));
#71282=CARTESIAN_POINT('Ctrl Pts',(-17.2413381067723,-69.0427501919636,
12.));
#71283=CARTESIAN_POINT('Ctrl Pts',(-17.2428974805044,-69.0204913121225,
12.));
#71284=CARTESIAN_POINT('Ctrl Pts',(-17.2444310864585,-68.9982772748694,
12.));
#71285=CARTESIAN_POINT('Ctrl Pts',(-17.2459389857327,-68.9761082282922,
12.));
#71286=CARTESIAN_POINT('Ctrl Pts',(-17.2474212398275,-68.9539843211619,
12.));
#71287=CARTESIAN_POINT('Ctrl Pts',(-17.248877910643,-68.9319057029409,12.));
#71288=CARTESIAN_POINT('Ctrl Pts',(-17.2503090604792,-68.909872523787,12.));
#71289=CARTESIAN_POINT('Ctrl Pts',(-17.2517147520376,-68.8878849345557,
12.));
#71290=CARTESIAN_POINT('Ctrl Pts',(-17.2530950484258,-68.8659430867972,
12.));
#71291=CARTESIAN_POINT('Ctrl Pts',(-17.2544500131624,-68.844047132755,12.));
#71292=CARTESIAN_POINT('Ctrl Pts',(-17.2557797101812,-68.8221972253941,
12.));
#71293=CARTESIAN_POINT('Ctrl Pts',(-17.2570842038383,-68.8003935184184,
12.));
#71294=CARTESIAN_POINT('Ctrl Pts',(-17.2583635589198,-68.7786361662882,
12.));
#71295=CARTESIAN_POINT('Ctrl Pts',(-17.259617840655,-68.7569253242333,12.));
#71296=CARTESIAN_POINT('Ctrl Pts',(-17.2608471147185,-68.7352611482547,
12.));
#71297=CARTESIAN_POINT('Ctrl Pts',(-17.2620514472182,-68.7136437951097,
12.));
#71298=CARTESIAN_POINT('Ctrl Pts',(-17.2632309046892,-68.6920734222938,
12.));
#71299=CARTESIAN_POINT('Ctrl Pts',(-17.2643855540892,-68.6705501880249,
12.));
#71300=CARTESIAN_POINT('Ctrl Pts',(-17.2655154627928,-68.6490742512057,
12.));
#71301=CARTESIAN_POINT('Ctrl Pts',(-17.2666206986084,-68.6276457714729,
12.));
#71302=CARTESIAN_POINT('Ctrl Pts',(-17.2677013298057,-68.6062649092764,
12.));
#71303=CARTESIAN_POINT('Ctrl Pts',(-17.2687574251428,-68.5849318259449,
12.));
#71304=CARTESIAN_POINT('Ctrl Pts',(-17.269789053896,-68.5636466837517,12.));
#71305=CARTESIAN_POINT('Ctrl Pts',(-17.2707962858919,-68.5424096459772,
12.));
#71306=CARTESIAN_POINT('Ctrl Pts',(-17.2717791914544,-68.521220876786,12.));
#71307=CARTESIAN_POINT('Ctrl Pts',(-17.2727378413489,-68.5000805410911,
12.));
#71308=CARTESIAN_POINT('Ctrl Pts',(-17.2736723067365,-68.4789888044351,
12.));
#71309=CARTESIAN_POINT('Ctrl Pts',(-17.2745826591119,-68.4579458328185,
12.));
#71310=CARTESIAN_POINT('Ctrl Pts',(-17.2754689702992,-68.436951792677,12.));
#71311=CARTESIAN_POINT('Ctrl Pts',(-17.2763313126018,-68.4160068512753,
12.));
#71312=CARTESIAN_POINT('Ctrl Pts',(-17.2771697589384,-68.3951111770487,
12.));
#71313=CARTESIAN_POINT('Ctrl Pts',(-17.2779843829608,-68.3742649398964,
12.));
#71314=CARTESIAN_POINT('Ctrl Pts',(-17.2787752592484,-68.3534683116515,
12.));
#71315=CARTESIAN_POINT('Ctrl Pts',(-17.2795424631799,-68.3327214657575,
12.));
#71316=CARTESIAN_POINT('Ctrl Pts',(-17.2802860705815,-68.3120245763914,
12.));
#71317=CARTESIAN_POINT('Ctrl Pts',(-17.2810061574353,-68.2913778177261,
12.));
#71318=CARTESIAN_POINT('Ctrl Pts',(-17.2817027995831,-68.2707813631731,
12.));
#71319=CARTESIAN_POINT('Ctrl Pts',(-17.2823760723874,-68.2502353845071,
12.));
#71320=CARTESIAN_POINT('Ctrl Pts',(-17.2830260513867,-68.2297400535294,
12.));
#71321=CARTESIAN_POINT('Ctrl Pts',(-17.2836528130819,-68.2092955440567,
12.));
#71322=CARTESIAN_POINT('Ctrl Pts',(-17.2842564355799,-68.1889020335427,
12.));
#71323=CARTESIAN_POINT('Ctrl Pts',(-17.2848369995293,-68.1685597054232,
12.));
#71324=CARTESIAN_POINT('Ctrl Pts',(-17.2853945882072,-68.1482687493226,
12.));
#71325=CARTESIAN_POINT('Ctrl Pts',(-17.2859292855705,-68.1280293561511,
12.));
#71326=CARTESIAN_POINT('Ctrl Pts',(-17.2864411745459,-68.1078417137877,
12.));
#71327=CARTESIAN_POINT('Ctrl Pts',(-17.2869303355432,-68.0877060033205,
12.));
#71328=CARTESIAN_POINT('Ctrl Pts',(-17.2873968440839,-68.0676223930412,
12.));
#71329=CARTESIAN_POINT('Ctrl Pts',(-17.2878407730961,-68.0475910442424,
12.));
#71330=CARTESIAN_POINT('Ctrl Pts',(-17.2882621974721,-68.0276121227356,
12.));
#71331=CARTESIAN_POINT('Ctrl Pts',(-17.28866119774,-68.007685808115,12.));
#71332=CARTESIAN_POINT('Ctrl Pts',(-17.2890378644866,-67.987812304921,12.));
#71333=CARTESIAN_POINT('Ctrl Pts',(-17.2893923013894,-67.9679918502579,
12.));
#71334=CARTESIAN_POINT('Ctrl Pts',(-17.2897246158941,-67.9482246901667,
12.));
#71335=CARTESIAN_POINT('Ctrl Pts',(-17.2900349103981,-67.9285110571741,
12.));
#71336=CARTESIAN_POINT('Ctrl Pts',(-17.2903232740694,-67.9088511496686,
12.));
#71337=CARTESIAN_POINT('Ctrl Pts',(-17.2905897723948,-67.8892451049608,
12.));
#71338=CARTESIAN_POINT('Ctrl Pts',(-17.2908344459694,-67.8696929978782,
12.));
#71339=CARTESIAN_POINT('Ctrl Pts',(-17.291012743109,-67.8540944889687,12.));
#71340=CARTESIAN_POINT('Ctrl Pts',(-17.2911366591347,-67.842419897098,12.));
#71341=CARTESIAN_POINT('Ctrl Pts',(-17.2912149114119,-67.8346476309018,
12.));
#71342=CARTESIAN_POINT('Ctrl Pts',(-17.2912529479484,-67.8307641965655,
12.));
#71343=CARTESIAN_POINT('Ctrl Pts',(-15.3208442077421,-72.6050633494713,
0.));
#71344=CARTESIAN_POINT('Ctrl Pts',(-15.3208442077421,-72.6050633494713,
4.));
#71345=CARTESIAN_POINT('Ctrl Pts',(-15.3208442077421,-72.6050633494713,
8.));
#71346=CARTESIAN_POINT('Ctrl Pts',(-15.3208442077421,-72.6050633494713,
12.));
#71347=CARTESIAN_POINT('Ctrl Pts',(-15.385683521042,-72.6937764817669,0.));
#71348=CARTESIAN_POINT('Ctrl Pts',(-15.385683521042,-72.6937764817669,4.));
#71349=CARTESIAN_POINT('Ctrl Pts',(-15.385683521042,-72.6937764817669,8.));
#71350=CARTESIAN_POINT('Ctrl Pts',(-15.385683521042,-72.6937764817669,12.));
#71351=CARTESIAN_POINT('Ctrl Pts',(-15.5519317750287,-72.809683430771,0.));
#71352=CARTESIAN_POINT('Ctrl Pts',(-15.5519317750287,-72.809683430771,4.00000000000001));
#71353=CARTESIAN_POINT('Ctrl Pts',(-15.5519317750287,-72.809683430771,7.99999999999999));
#71354=CARTESIAN_POINT('Ctrl Pts',(-15.5519317750287,-72.809683430771,12.));
#71355=CARTESIAN_POINT('Ctrl Pts',(-15.7502340068145,-72.8161171750016,
0.));
#71356=CARTESIAN_POINT('Ctrl Pts',(-15.7502340068145,-72.8161171750016,
4.));
#71357=CARTESIAN_POINT('Ctrl Pts',(-15.7502340068145,-72.8161171750016,
8.00000000000001));
#71358=CARTESIAN_POINT('Ctrl Pts',(-15.7502340068145,-72.8161171750016,
12.));
#71359=CARTESIAN_POINT('Ctrl Pts',(-15.8307637747231,-72.7986051948038,
0.));
#71360=CARTESIAN_POINT('Ctrl Pts',(-15.8307637747231,-72.7986051948038,
4.));
#71361=CARTESIAN_POINT('Ctrl Pts',(-15.8307637747231,-72.7986051948038,
8.));
#71362=CARTESIAN_POINT('Ctrl Pts',(-15.8307637747231,-72.7986051948038,
12.));
#71363=CARTESIAN_POINT('',(-15.3208442077421,-72.6050633494713,0.));
#71364=CARTESIAN_POINT('',(-15.8307637747231,-72.7986051948038,0.));
#71365=CARTESIAN_POINT('Ctrl Pts',(-15.3208442077421,-72.6050633494713,
2.77555756156289E-16));
#71366=CARTESIAN_POINT('Ctrl Pts',(-15.385683521042,-72.6937764817669,2.77555756156289E-16));
#71367=CARTESIAN_POINT('Ctrl Pts',(-15.4806825233201,-72.760009024055,2.77555756156289E-16));
#71368=CARTESIAN_POINT('Ctrl Pts',(-15.5861481305938,-72.7904952137639,
2.77555756156289E-16));
#71369=CARTESIAN_POINT('Ctrl Pts',(-15.6652473360491,-72.8133598560456,
2.77555756156289E-16));
#71370=CARTESIAN_POINT('Ctrl Pts',(-15.7502340068145,-72.8161171750016,
2.77555756156289E-16));
#71371=CARTESIAN_POINT('Ctrl Pts',(-15.8307637747231,-72.7986051948038,
2.77555756156289E-16));
#71372=CARTESIAN_POINT('',(-15.8307637747231,-72.7986051948038,12.));
#71373=CARTESIAN_POINT('Ctrl Pts',(-15.8307637747231,-72.7986051948038,
0.));
#71374=CARTESIAN_POINT('Ctrl Pts',(-15.8307637747231,-72.7986051948038,
4.));
#71375=CARTESIAN_POINT('Ctrl Pts',(-15.8307637747231,-72.7986051948038,
8.));
#71376=CARTESIAN_POINT('Ctrl Pts',(-15.8307637747231,-72.7986051948038,
12.));
#71377=CARTESIAN_POINT('',(-15.3208442077421,-72.6050633494713,12.));
#71378=CARTESIAN_POINT('Ctrl Pts',(-15.8307637747231,-72.7986051948038,
12.));
#71379=CARTESIAN_POINT('Ctrl Pts',(-15.7502340068145,-72.8161171750016,
12.));
#71380=CARTESIAN_POINT('Ctrl Pts',(-15.6652473360491,-72.8133598560456,
12.));
#71381=CARTESIAN_POINT('Ctrl Pts',(-15.5861481305938,-72.7904952137639,
12.));
#71382=CARTESIAN_POINT('Ctrl Pts',(-15.4806825233201,-72.760009024055,12.));
#71383=CARTESIAN_POINT('Ctrl Pts',(-15.385683521042,-72.6937764817669,12.));
#71384=CARTESIAN_POINT('Ctrl Pts',(-15.3208442077421,-72.6050633494713,
12.));
#71385=CARTESIAN_POINT('Ctrl Pts',(-15.3208442077421,-72.6050633494713,
12.));
#71386=CARTESIAN_POINT('Ctrl Pts',(-15.3208442077421,-72.6050633494713,
8.));
#71387=CARTESIAN_POINT('Ctrl Pts',(-15.3208442077421,-72.6050633494713,
4.));
#71388=CARTESIAN_POINT('Ctrl Pts',(-15.3208442077421,-72.6050633494713,
0.));
#71389=CARTESIAN_POINT('Origin',(-8.1034134051859E-11,-3.65979954444617E-10,
0.));
#71390=CARTESIAN_POINT('Origin',(-8.1034134051859E-11,-3.65979954444617E-10,
12.));
#71391=CARTESIAN_POINT('Origin',(-8.1034134051859E-11,-3.65979954444617E-10,
0.));
#71392=CARTESIAN_POINT('Ctrl Pts',(-22.6894590071785,-70.9608233461364,
0.));
#71393=CARTESIAN_POINT('Ctrl Pts',(-22.6894590071785,-70.9608233461364,
4.));
#71394=CARTESIAN_POINT('Ctrl Pts',(-22.6894590071785,-70.9608233461363,
8.));
#71395=CARTESIAN_POINT('Ctrl Pts',(-22.6894590071785,-70.9608233461363,
12.));
#71396=CARTESIAN_POINT('Ctrl Pts',(-22.7941214270114,-70.9273579271571,
0.));
#71397=CARTESIAN_POINT('Ctrl Pts',(-22.7941214270114,-70.9273579271571,
4.));
#71398=CARTESIAN_POINT('Ctrl Pts',(-22.7941214270114,-70.9273579271571,
8.00000000000001));
#71399=CARTESIAN_POINT('Ctrl Pts',(-22.7941214270114,-70.9273579271571,
12.));
#71400=CARTESIAN_POINT('Ctrl Pts',(-22.9566438338674,-70.8062825417802,
0.));
#71401=CARTESIAN_POINT('Ctrl Pts',(-22.9566438338674,-70.8062825417802,
4.));
#71402=CARTESIAN_POINT('Ctrl Pts',(-22.9566438338675,-70.8062825417802,
8.));
#71403=CARTESIAN_POINT('Ctrl Pts',(-22.9566438338675,-70.8062825417802,
12.));
#71404=CARTESIAN_POINT('Ctrl Pts',(-23.0254444386655,-70.6201870200063,
0.));
#71405=CARTESIAN_POINT('Ctrl Pts',(-23.0254444386655,-70.6201870200063,
4.));
#71406=CARTESIAN_POINT('Ctrl Pts',(-23.0254444386655,-70.6201870200063,
8.00000000000001));
#71407=CARTESIAN_POINT('Ctrl Pts',(-23.0254444386655,-70.6201870200063,
12.));
#71408=CARTESIAN_POINT('Ctrl Pts',(-23.0342913834093,-70.5382514078489,
0.));
#71409=CARTESIAN_POINT('Ctrl Pts',(-23.0342913834093,-70.5382514078489,
4.));
#71410=CARTESIAN_POINT('Ctrl Pts',(-23.0342913834093,-70.5382514078489,
8.));
#71411=CARTESIAN_POINT('Ctrl Pts',(-23.0342913834093,-70.5382514078489,
12.));
#71412=CARTESIAN_POINT('',(-22.6894590071785,-70.9608233461364,0.));
#71413=CARTESIAN_POINT('',(-23.0342913834093,-70.5382514078489,0.));
#71414=CARTESIAN_POINT('Ctrl Pts',(-22.6894590071785,-70.9608233461364,
1.38777878078145E-16));
#71415=CARTESIAN_POINT('Ctrl Pts',(-22.7941214270114,-70.9273579271571,
1.38777878078145E-16));
#71416=CARTESIAN_POINT('Ctrl Pts',(-22.8869913737863,-70.858171992656,1.38777878078145E-16));
#71417=CARTESIAN_POINT('Ctrl Pts',(-22.9492582831545,-70.767754993209,1.38777878078145E-16));
#71418=CARTESIAN_POINT('Ctrl Pts',(-22.9959584651806,-70.6999422436237,
1.38777878078145E-16));
#71419=CARTESIAN_POINT('Ctrl Pts',(-23.0254444386655,-70.6201870200063,
1.38777878078144E-16));
#71420=CARTESIAN_POINT('Ctrl Pts',(-23.0342913834093,-70.5382514078489,
1.38777878078145E-16));
#71421=CARTESIAN_POINT('',(-23.0342913834093,-70.5382514078489,12.));
#71422=CARTESIAN_POINT('Ctrl Pts',(-23.0342913834093,-70.5382514078489,
0.));
#71423=CARTESIAN_POINT('Ctrl Pts',(-23.0342913834093,-70.5382514078489,
4.));
#71424=CARTESIAN_POINT('Ctrl Pts',(-23.0342913834093,-70.5382514078489,
8.));
#71425=CARTESIAN_POINT('Ctrl Pts',(-23.0342913834093,-70.5382514078489,
12.));
#71426=CARTESIAN_POINT('',(-22.6894590071785,-70.9608233461363,12.));
#71427=CARTESIAN_POINT('Ctrl Pts',(-23.0342913834093,-70.5382514078489,
12.));
#71428=CARTESIAN_POINT('Ctrl Pts',(-23.0254444386655,-70.6201870200063,
12.));
#71429=CARTESIAN_POINT('Ctrl Pts',(-22.9959584651806,-70.6999422436237,
12.));
#71430=CARTESIAN_POINT('Ctrl Pts',(-22.9492582831545,-70.767754993209,12.));
#71431=CARTESIAN_POINT('Ctrl Pts',(-22.8869913737863,-70.858171992656,12.));
#71432=CARTESIAN_POINT('Ctrl Pts',(-22.7941214270114,-70.9273579271571,
12.));
#71433=CARTESIAN_POINT('Ctrl Pts',(-22.6894590071785,-70.9608233461363,
12.));
#71434=CARTESIAN_POINT('Ctrl Pts',(-22.6894590071785,-70.9608233461363,
12.));
#71435=CARTESIAN_POINT('Ctrl Pts',(-22.6894590071785,-70.9608233461363,
8.));
#71436=CARTESIAN_POINT('Ctrl Pts',(-22.6894590071785,-70.9608233461364,
4.));
#71437=CARTESIAN_POINT('Ctrl Pts',(-22.6894590071785,-70.9608233461364,
0.));
#71438=CARTESIAN_POINT('Ctrl Pts',(-23.1372951448024,-66.0656156664138,
0.));
#71439=CARTESIAN_POINT('Ctrl Pts',(-23.1372951448024,-66.0656156664138,
12.));
#71440=CARTESIAN_POINT('Ctrl Pts',(-23.1375957166104,-66.0694876382127,
0.));
#71441=CARTESIAN_POINT('Ctrl Pts',(-23.1375957166104,-66.0694876382127,
12.));
#71442=CARTESIAN_POINT('Ctrl Pts',(-23.13819515974,-66.0772371487248,0.));
#71443=CARTESIAN_POINT('Ctrl Pts',(-23.13819515974,-66.0772371487248,12.));
#71444=CARTESIAN_POINT('Ctrl Pts',(-23.1390892229779,-66.088878115242,0.));
#71445=CARTESIAN_POINT('Ctrl Pts',(-23.1390892229779,-66.088878115242,12.));
#71446=CARTESIAN_POINT('Ctrl Pts',(-23.1402711039425,-66.1044328067355,
0.));
#71447=CARTESIAN_POINT('Ctrl Pts',(-23.1402711039425,-66.1044328067355,
12.));
#71448=CARTESIAN_POINT('Ctrl Pts',(-23.1417314398398,-66.1239318368548,
0.));
#71449=CARTESIAN_POINT('Ctrl Pts',(-23.1417314398398,-66.1239318368548,
12.));
#71450=CARTESIAN_POINT('Ctrl Pts',(-23.1431747350098,-66.1434865015027,
0.));
#71451=CARTESIAN_POINT('Ctrl Pts',(-23.1431747350098,-66.1434865015027,
12.));
#71452=CARTESIAN_POINT('Ctrl Pts',(-23.1446009424903,-66.1630967296747,
0.));
#71453=CARTESIAN_POINT('Ctrl Pts',(-23.1446009424903,-66.1630967296747,
12.));
#71454=CARTESIAN_POINT('Ctrl Pts',(-23.1460099850763,-66.18276239029,0.));
#71455=CARTESIAN_POINT('Ctrl Pts',(-23.1460099850763,-66.18276239029,12.));
#71456=CARTESIAN_POINT('Ctrl Pts',(-23.1474017566484,-66.2024832934866,
0.));
#71457=CARTESIAN_POINT('Ctrl Pts',(-23.1474017566484,-66.2024832934866,
12.));
#71458=CARTESIAN_POINT('Ctrl Pts',(-23.1487761349328,-66.2222592165473,
0.));
#71459=CARTESIAN_POINT('Ctrl Pts',(-23.1487761349328,-66.2222592165473,
12.));
#71460=CARTESIAN_POINT('Ctrl Pts',(-23.1501329914488,-66.2420899237317,
0.));
#71461=CARTESIAN_POINT('Ctrl Pts',(-23.1501329914488,-66.2420899237317,
12.));
#71462=CARTESIAN_POINT('Ctrl Pts',(-23.1514722022483,-66.2619751878741,
0.));
#71463=CARTESIAN_POINT('Ctrl Pts',(-23.1514722022483,-66.2619751878741,
12.));
#71464=CARTESIAN_POINT('Ctrl Pts',(-23.1527936592625,-66.2819148131072,
0.));
#71465=CARTESIAN_POINT('Ctrl Pts',(-23.1527936592625,-66.2819148131072,
12.));
#71466=CARTESIAN_POINT('Ctrl Pts',(-23.154097266617,-66.301908627539,0.));
#71467=CARTESIAN_POINT('Ctrl Pts',(-23.154097266617,-66.301908627539,12.));
#71468=CARTESIAN_POINT('Ctrl Pts',(-23.1553829352531,-66.3219564725161,
0.));
#71469=CARTESIAN_POINT('Ctrl Pts',(-23.1553829352531,-66.3219564725161,
12.));
#71470=CARTESIAN_POINT('Ctrl Pts',(-23.1566505784626,-66.3420581937159,
0.));
#71471=CARTESIAN_POINT('Ctrl Pts',(-23.1566505784626,-66.3420581937159,
12.));
#71472=CARTESIAN_POINT('Ctrl Pts',(-23.1579001063438,-66.3622136300692,
0.));
#71473=CARTESIAN_POINT('Ctrl Pts',(-23.1579001063438,-66.3622136300692,
12.));
#71474=CARTESIAN_POINT('Ctrl Pts',(-23.1591314230101,-66.382422608185,0.));
#71475=CARTESIAN_POINT('Ctrl Pts',(-23.1591314230101,-66.382422608185,12.));
#71476=CARTESIAN_POINT('Ctrl Pts',(-23.1603444294754,-66.402684948127,0.));
#71477=CARTESIAN_POINT('Ctrl Pts',(-23.1603444294754,-66.402684948127,12.));
#71478=CARTESIAN_POINT('Ctrl Pts',(-23.1615390254635,-66.4230004670288,
0.));
#71479=CARTESIAN_POINT('Ctrl Pts',(-23.1615390254635,-66.4230004670288,
12.));
#71480=CARTESIAN_POINT('Ctrl Pts',(-23.1627151114875,-66.4433689832454,
0.));
#71481=CARTESIAN_POINT('Ctrl Pts',(-23.1627151114875,-66.4433689832454,
12.));
#71482=CARTESIAN_POINT('Ctrl Pts',(-23.163872591218,-66.4637903210682,0.));
#71483=CARTESIAN_POINT('Ctrl Pts',(-23.163872591218,-66.4637903210682,12.));
#71484=CARTESIAN_POINT('Ctrl Pts',(-23.1650113713792,-66.4842643105263,
0.));
#71485=CARTESIAN_POINT('Ctrl Pts',(-23.1650113713792,-66.4842643105263,
12.));
#71486=CARTESIAN_POINT('Ctrl Pts',(-23.1661313606123,-66.5047907851319,
0.));
#71487=CARTESIAN_POINT('Ctrl Pts',(-23.1661313606123,-66.5047907851319,
12.));
#71488=CARTESIAN_POINT('Ctrl Pts',(-23.1672324686928,-66.5253695803209,
0.));
#71489=CARTESIAN_POINT('Ctrl Pts',(-23.1672324686928,-66.5253695803209,
12.));
#71490=CARTESIAN_POINT('Ctrl Pts',(-23.1683146055736,-66.5460005315406,
0.));
#71491=CARTESIAN_POINT('Ctrl Pts',(-23.1683146055736,-66.5460005315406,
12.));
#71492=CARTESIAN_POINT('Ctrl Pts',(-23.169377680588,-66.5666834726494,0.));
#71493=CARTESIAN_POINT('Ctrl Pts',(-23.169377680588,-66.5666834726494,12.));
#71494=CARTESIAN_POINT('Ctrl Pts',(-23.1704216028626,-66.5874182367596,
0.));
#71495=CARTESIAN_POINT('Ctrl Pts',(-23.1704216028626,-66.5874182367596,
12.));
#71496=CARTESIAN_POINT('Ctrl Pts',(-23.1714462816794,-66.6082046569657,
0.));
#71497=CARTESIAN_POINT('Ctrl Pts',(-23.1714462816794,-66.6082046569657,
12.));
#71498=CARTESIAN_POINT('Ctrl Pts',(-23.1724516268299,-66.6290425670538,
0.));
#71499=CARTESIAN_POINT('Ctrl Pts',(-23.1724516268299,-66.6290425670538,
12.));
#71500=CARTESIAN_POINT('Ctrl Pts',(-23.1734375490421,-66.6499318023445,
0.));
#71501=CARTESIAN_POINT('Ctrl Pts',(-23.1734375490421,-66.6499318023445,
12.));
#71502=CARTESIAN_POINT('Ctrl Pts',(-23.174403960137,-66.6708722000046,0.));
#71503=CARTESIAN_POINT('Ctrl Pts',(-23.174403960137,-66.6708722000046,12.));
#71504=CARTESIAN_POINT('Ctrl Pts',(-23.1753507727932,-66.691863598595,0.));
#71505=CARTESIAN_POINT('Ctrl Pts',(-23.1753507727932,-66.691863598595,12.));
#71506=CARTESIAN_POINT('Ctrl Pts',(-23.1762779004043,-66.712905837789,0.));
#71507=CARTESIAN_POINT('Ctrl Pts',(-23.1762779004043,-66.712905837789,12.));
#71508=CARTESIAN_POINT('Ctrl Pts',(-23.1771852569137,-66.7339987580441,
0.));
#71509=CARTESIAN_POINT('Ctrl Pts',(-23.1771852569137,-66.7339987580441,
12.));
#71510=CARTESIAN_POINT('Ctrl Pts',(-23.1780727566309,-66.7551422002229,
0.));
#71511=CARTESIAN_POINT('Ctrl Pts',(-23.1780727566309,-66.7551422002229,
12.));
#71512=CARTESIAN_POINT('Ctrl Pts',(-23.1789403142376,-66.7763360056146,
0.));
#71513=CARTESIAN_POINT('Ctrl Pts',(-23.1789403142376,-66.7763360056146,
12.));
#71514=CARTESIAN_POINT('Ctrl Pts',(-23.1797878448645,-66.7975800161014,
0.));
#71515=CARTESIAN_POINT('Ctrl Pts',(-23.1797878448645,-66.7975800161014,
12.));
#71516=CARTESIAN_POINT('Ctrl Pts',(-23.1806152641475,-66.8188740742727,
0.));
#71517=CARTESIAN_POINT('Ctrl Pts',(-23.1806152641475,-66.8188740742727,
12.));
#71518=CARTESIAN_POINT('Ctrl Pts',(-23.1814224882948,-66.8402180235549,
0.));
#71519=CARTESIAN_POINT('Ctrl Pts',(-23.1814224882948,-66.8402180235549,
12.));
#71520=CARTESIAN_POINT('Ctrl Pts',(-23.1822094341508,-66.8616117083304,
0.));
#71521=CARTESIAN_POINT('Ctrl Pts',(-23.1822094341508,-66.8616117083304,
12.));
#71522=CARTESIAN_POINT('Ctrl Pts',(-23.1829760191583,-66.8830549738768,
0.));
#71523=CARTESIAN_POINT('Ctrl Pts',(-23.1829760191583,-66.8830549738768,
12.));
#71524=CARTESIAN_POINT('Ctrl Pts',(-23.1837221613231,-66.904547666305,0.));
#71525=CARTESIAN_POINT('Ctrl Pts',(-23.1837221613231,-66.904547666305,12.));
#71526=CARTESIAN_POINT('Ctrl Pts',(-23.1844477791816,-66.9260896324955,
0.));
#71527=CARTESIAN_POINT('Ctrl Pts',(-23.1844477791816,-66.9260896324955,
12.));
#71528=CARTESIAN_POINT('Ctrl Pts',(-23.1851527917666,-66.9476807200225,
0.));
#71529=CARTESIAN_POINT('Ctrl Pts',(-23.1851527917666,-66.9476807200225,
12.));
#71530=CARTESIAN_POINT('Ctrl Pts',(-23.1858371185852,-66.9693207771058,
0.));
#71531=CARTESIAN_POINT('Ctrl Pts',(-23.1858371185852,-66.9693207771058,
12.));
#71532=CARTESIAN_POINT('Ctrl Pts',(-23.1865006796291,-66.9910096526483,
0.));
#71533=CARTESIAN_POINT('Ctrl Pts',(-23.1865006796291,-66.9910096526483,
12.));
#71534=CARTESIAN_POINT('Ctrl Pts',(-23.1871433953795,-67.0127471962507,
0.));
#71535=CARTESIAN_POINT('Ctrl Pts',(-23.1871433953795,-67.0127471962507,
12.));
#71536=CARTESIAN_POINT('Ctrl Pts',(-23.1877651868155,-67.0345332582297,
0.));
#71537=CARTESIAN_POINT('Ctrl Pts',(-23.1877651868155,-67.0345332582297,
12.));
#71538=CARTESIAN_POINT('Ctrl Pts',(-23.1883659754268,-67.0563676896312,
0.));
#71539=CARTESIAN_POINT('Ctrl Pts',(-23.1883659754268,-67.0563676896312,
12.));
#71540=CARTESIAN_POINT('Ctrl Pts',(-23.1889456832116,-67.0782503422293,
0.));
#71541=CARTESIAN_POINT('Ctrl Pts',(-23.1889456832116,-67.0782503422293,
12.));
#71542=CARTESIAN_POINT('Ctrl Pts',(-23.1895042326626,-67.1001810685138,
0.));
#71543=CARTESIAN_POINT('Ctrl Pts',(-23.1895042326626,-67.1001810685138,
12.));
#71544=CARTESIAN_POINT('Ctrl Pts',(-23.1900415467575,-67.122159721674,0.));
#71545=CARTESIAN_POINT('Ctrl Pts',(-23.1900415467575,-67.122159721674,12.));
#71546=CARTESIAN_POINT('Ctrl Pts',(-23.1905575489506,-67.1441861555819,
0.));
#71547=CARTESIAN_POINT('Ctrl Pts',(-23.1905575489506,-67.1441861555819,
12.));
#71548=CARTESIAN_POINT('Ctrl Pts',(-23.1910521631658,-67.1662602247641,
0.));
#71549=CARTESIAN_POINT('Ctrl Pts',(-23.1910521631658,-67.1662602247641,
12.));
#71550=CARTESIAN_POINT('Ctrl Pts',(-23.1915253137924,-67.1883817844039,
0.));
#71551=CARTESIAN_POINT('Ctrl Pts',(-23.1915253137924,-67.1883817844039,
12.));
#71552=CARTESIAN_POINT('Ctrl Pts',(-23.1919769256803,-67.2105506903448,
0.));
#71553=CARTESIAN_POINT('Ctrl Pts',(-23.1919769256803,-67.2105506903448,
12.));
#71554=CARTESIAN_POINT('Ctrl Pts',(-23.1924069241386,-67.232766799088,0.));
#71555=CARTESIAN_POINT('Ctrl Pts',(-23.1924069241386,-67.232766799088,12.));
#71556=CARTESIAN_POINT('Ctrl Pts',(-23.1928152349344,-67.2550299677888,
0.));
#71557=CARTESIAN_POINT('Ctrl Pts',(-23.1928152349344,-67.2550299677888,
12.));
#71558=CARTESIAN_POINT('Ctrl Pts',(-23.1932017842954,-67.2773400542477,
0.));
#71559=CARTESIAN_POINT('Ctrl Pts',(-23.1932017842954,-67.2773400542477,
12.));
#71560=CARTESIAN_POINT('Ctrl Pts',(-23.193566498902,-67.2996969169099,0.));
#71561=CARTESIAN_POINT('Ctrl Pts',(-23.193566498902,-67.2996969169099,12.));
#71562=CARTESIAN_POINT('Ctrl Pts',(-23.1939093058802,-67.3221004148604,
0.));
#71563=CARTESIAN_POINT('Ctrl Pts',(-23.1939093058802,-67.3221004148604,
12.));
#71564=CARTESIAN_POINT('Ctrl Pts',(-23.1942301327979,-67.3445504078178,
0.));
#71565=CARTESIAN_POINT('Ctrl Pts',(-23.1942301327979,-67.3445504078178,
12.));
#71566=CARTESIAN_POINT('Ctrl Pts',(-23.1945289076608,-67.3670467561205,
0.));
#71567=CARTESIAN_POINT('Ctrl Pts',(-23.1945289076608,-67.3670467561205,
12.));
#71568=CARTESIAN_POINT('Ctrl Pts',(-23.1948055589123,-67.3895893207168,
0.));
#71569=CARTESIAN_POINT('Ctrl Pts',(-23.1948055589123,-67.3895893207168,
12.));
#71570=CARTESIAN_POINT('Ctrl Pts',(-23.195060015426,-67.4121779631666,0.));
#71571=CARTESIAN_POINT('Ctrl Pts',(-23.195060015426,-67.4121779631666,12.));
#71572=CARTESIAN_POINT('Ctrl Pts',(-23.1952922065009,-67.4348125456389,
0.));
#71573=CARTESIAN_POINT('Ctrl Pts',(-23.1952922065009,-67.4348125456389,
12.));
#71574=CARTESIAN_POINT('Ctrl Pts',(-23.1955020618591,-67.4574929309078,
0.));
#71575=CARTESIAN_POINT('Ctrl Pts',(-23.1955020618591,-67.4574929309078,
12.));
#71576=CARTESIAN_POINT('Ctrl Pts',(-23.1956895116446,-67.4802189823423,
0.));
#71577=CARTESIAN_POINT('Ctrl Pts',(-23.1956895116446,-67.4802189823423,
12.));
#71578=CARTESIAN_POINT('Ctrl Pts',(-23.1958544864224,-67.5029905638973,
0.));
#71579=CARTESIAN_POINT('Ctrl Pts',(-23.1958544864224,-67.5029905638973,
12.));
#71580=CARTESIAN_POINT('Ctrl Pts',(-23.195996917171,-67.525807540117,0.));
#71581=CARTESIAN_POINT('Ctrl Pts',(-23.195996917171,-67.525807540117,12.));
#71582=CARTESIAN_POINT('Ctrl Pts',(-23.1961167352777,-67.5486697761301,
0.));
#71583=CARTESIAN_POINT('Ctrl Pts',(-23.1961167352777,-67.5486697761301,
12.));
#71584=CARTESIAN_POINT('Ctrl Pts',(-23.1962138725358,-67.5715771376454,
0.));
#71585=CARTESIAN_POINT('Ctrl Pts',(-23.1962138725358,-67.5715771376454,
12.));
#71586=CARTESIAN_POINT('Ctrl Pts',(-23.1962882611444,-67.5945294909398,
0.));
#71587=CARTESIAN_POINT('Ctrl Pts',(-23.1962882611444,-67.5945294909398,
12.));
#71588=CARTESIAN_POINT('Ctrl Pts',(-23.1963398337056,-67.6175267028516,
0.));
#71589=CARTESIAN_POINT('Ctrl Pts',(-23.1963398337056,-67.6175267028516,
12.));
#71590=CARTESIAN_POINT('Ctrl Pts',(-23.1963685232176,-67.6405686407828,
0.));
#71591=CARTESIAN_POINT('Ctrl Pts',(-23.1963685232176,-67.6405686407828,
12.));
#71592=CARTESIAN_POINT('Ctrl Pts',(-23.196374263071,-67.6636551726948,0.));
#71593=CARTESIAN_POINT('Ctrl Pts',(-23.196374263071,-67.6636551726948,12.));
#71594=CARTESIAN_POINT('Ctrl Pts',(-23.1963569870457,-67.6867861671044,
0.));
#71595=CARTESIAN_POINT('Ctrl Pts',(-23.1963569870457,-67.6867861671044,
12.));
#71596=CARTESIAN_POINT('Ctrl Pts',(-23.1963166293116,-67.7099614930712,
0.));
#71597=CARTESIAN_POINT('Ctrl Pts',(-23.1963166293116,-67.7099614930712,
12.));
#71598=CARTESIAN_POINT('Ctrl Pts',(-23.1962531244261,-67.7331810201931,
0.));
#71599=CARTESIAN_POINT('Ctrl Pts',(-23.1962531244261,-67.7331810201931,
12.));
#71600=CARTESIAN_POINT('Ctrl Pts',(-23.1961664073274,-67.7564446186115,
0.));
#71601=CARTESIAN_POINT('Ctrl Pts',(-23.1961664073274,-67.7564446186115,
12.));
#71602=CARTESIAN_POINT('Ctrl Pts',(-23.1960564133308,-67.7797521590056,
0.));
#71603=CARTESIAN_POINT('Ctrl Pts',(-23.1960564133308,-67.7797521590056,
12.));
#71604=CARTESIAN_POINT('Ctrl Pts',(-23.1959230781265,-67.8031035125873,
0.));
#71605=CARTESIAN_POINT('Ctrl Pts',(-23.1959230781265,-67.8031035125873,
12.));
#71606=CARTESIAN_POINT('Ctrl Pts',(-23.1957663377798,-67.8264985510884,
0.));
#71607=CARTESIAN_POINT('Ctrl Pts',(-23.1957663377798,-67.8264985510884,
12.));
#71608=CARTESIAN_POINT('Ctrl Pts',(-23.1955861287276,-67.8499371467578,
0.));
#71609=CARTESIAN_POINT('Ctrl Pts',(-23.1955861287276,-67.8499371467578,
12.));
#71610=CARTESIAN_POINT('Ctrl Pts',(-23.1953823877727,-67.8734191723639,
0.));
#71611=CARTESIAN_POINT('Ctrl Pts',(-23.1953823877727,-67.8734191723639,
12.));
#71612=CARTESIAN_POINT('Ctrl Pts',(-23.19515505208,-67.8969445011908,0.));
#71613=CARTESIAN_POINT('Ctrl Pts',(-23.19515505208,-67.8969445011908,12.));
#71614=CARTESIAN_POINT('Ctrl Pts',(-23.1949040591748,-67.9205130070337,
0.));
#71615=CARTESIAN_POINT('Ctrl Pts',(-23.1949040591748,-67.9205130070337,
12.));
#71616=CARTESIAN_POINT('Ctrl Pts',(-23.1946293469437,-67.944124564187,0.));
#71617=CARTESIAN_POINT('Ctrl Pts',(-23.1946293469437,-67.944124564187,12.));
#71618=CARTESIAN_POINT('Ctrl Pts',(-23.1943308536307,-67.9677790474414,
0.));
#71619=CARTESIAN_POINT('Ctrl Pts',(-23.1943308536307,-67.9677790474414,
12.));
#71620=CARTESIAN_POINT('Ctrl Pts',(-23.194008517832,-67.9914763320878,0.));
#71621=CARTESIAN_POINT('Ctrl Pts',(-23.194008517832,-67.9914763320878,12.));
#71622=CARTESIAN_POINT('Ctrl Pts',(-23.193662278492,-68.0152162939123,0.));
#71623=CARTESIAN_POINT('Ctrl Pts',(-23.193662278492,-68.0152162939123,12.));
#71624=CARTESIAN_POINT('Ctrl Pts',(-23.1932920749021,-68.0389988091926,
0.));
#71625=CARTESIAN_POINT('Ctrl Pts',(-23.1932920749021,-68.0389988091926,
12.));
#71626=CARTESIAN_POINT('Ctrl Pts',(-23.1928978467018,-68.0628237546852,
0.));
#71627=CARTESIAN_POINT('Ctrl Pts',(-23.1928978467018,-68.0628237546852,
12.));
#71628=CARTESIAN_POINT('Ctrl Pts',(-23.1924795338746,-68.086691007624,0.));
#71629=CARTESIAN_POINT('Ctrl Pts',(-23.1924795338746,-68.086691007624,12.));
#71630=CARTESIAN_POINT('Ctrl Pts',(-23.1920370767424,-68.1106004457223,
0.));
#71631=CARTESIAN_POINT('Ctrl Pts',(-23.1920370767424,-68.1106004457223,
12.));
#71632=CARTESIAN_POINT('Ctrl Pts',(-23.1915704159624,-68.1345519471695,
0.));
#71633=CARTESIAN_POINT('Ctrl Pts',(-23.1915704159624,-68.1345519471695,
12.));
#71634=CARTESIAN_POINT('Ctrl Pts',(-23.1910794925252,-68.1585453906259,
0.));
#71635=CARTESIAN_POINT('Ctrl Pts',(-23.1910794925252,-68.1585453906259,
12.));
#71636=CARTESIAN_POINT('Ctrl Pts',(-23.1905642477572,-68.182580655213,0.));
#71637=CARTESIAN_POINT('Ctrl Pts',(-23.1905642477572,-68.182580655213,12.));
#71638=CARTESIAN_POINT('Ctrl Pts',(-23.1900246233165,-68.2066576205113,
0.));
#71639=CARTESIAN_POINT('Ctrl Pts',(-23.1900246233165,-68.2066576205113,
12.));
#71640=CARTESIAN_POINT('Ctrl Pts',(-23.189460561187,-68.2307761665629,0.));
#71641=CARTESIAN_POINT('Ctrl Pts',(-23.189460561187,-68.2307761665629,12.));
#71642=CARTESIAN_POINT('Ctrl Pts',(-23.1888720036757,-68.2549361738679,
0.));
#71643=CARTESIAN_POINT('Ctrl Pts',(-23.1888720036757,-68.2549361738679,
12.));
#71644=CARTESIAN_POINT('Ctrl Pts',(-23.1882588934108,-68.2791375233798,
0.));
#71645=CARTESIAN_POINT('Ctrl Pts',(-23.1882588934108,-68.2791375233798,
12.));
#71646=CARTESIAN_POINT('Ctrl Pts',(-23.1876211733439,-68.3033800964946,
0.));
#71647=CARTESIAN_POINT('Ctrl Pts',(-23.1876211733439,-68.3033800964946,
12.));
#71648=CARTESIAN_POINT('Ctrl Pts',(-23.1869587867463,-68.3276637750494,
0.));
#71649=CARTESIAN_POINT('Ctrl Pts',(-23.1869587867463,-68.3276637750494,
12.));
#71650=CARTESIAN_POINT('Ctrl Pts',(-23.1862716772034,-68.3519884413253,
0.));
#71651=CARTESIAN_POINT('Ctrl Pts',(-23.1862716772034,-68.3519884413253,
12.));
#71652=CARTESIAN_POINT('Ctrl Pts',(-23.1855597886117,-68.3763539780442,
0.));
#71653=CARTESIAN_POINT('Ctrl Pts',(-23.1855597886117,-68.3763539780442,
12.));
#71654=CARTESIAN_POINT('Ctrl Pts',(-23.1848230651776,-68.4007602683649,
0.));
#71655=CARTESIAN_POINT('Ctrl Pts',(-23.1848230651776,-68.4007602683649,
12.));
#71656=CARTESIAN_POINT('Ctrl Pts',(-23.1840614514191,-68.4252071958725,
0.));
#71657=CARTESIAN_POINT('Ctrl Pts',(-23.1840614514191,-68.4252071958725,
12.));
#71658=CARTESIAN_POINT('Ctrl Pts',(-23.1832748921629,-68.4496946445756,
0.));
#71659=CARTESIAN_POINT('Ctrl Pts',(-23.1832748921629,-68.4496946445756,
12.));
#71660=CARTESIAN_POINT('Ctrl Pts',(-23.1824633325385,-68.4742224989099,
0.));
#71661=CARTESIAN_POINT('Ctrl Pts',(-23.1824633325385,-68.4742224989099,
12.));
#71662=CARTESIAN_POINT('Ctrl Pts',(-23.1816267179752,-68.4987906437357,
0.));
#71663=CARTESIAN_POINT('Ctrl Pts',(-23.1816267179752,-68.4987906437357,
12.));
#71664=CARTESIAN_POINT('Ctrl Pts',(-23.1807649942011,-68.5233989643344,
0.));
#71665=CARTESIAN_POINT('Ctrl Pts',(-23.1807649942011,-68.5233989643344,
12.));
#71666=CARTESIAN_POINT('Ctrl Pts',(-23.1798781072449,-68.548047346398,0.));
#71667=CARTESIAN_POINT('Ctrl Pts',(-23.1798781072449,-68.548047346398,12.));
#71668=CARTESIAN_POINT('Ctrl Pts',(-23.178966003434,-68.572735676027,0.));
#71669=CARTESIAN_POINT('Ctrl Pts',(-23.178966003434,-68.572735676027,12.));
#71670=CARTESIAN_POINT('Ctrl Pts',(-23.1780286293873,-68.5974638397322,
0.));
#71671=CARTESIAN_POINT('Ctrl Pts',(-23.1780286293873,-68.5974638397322,
12.));
#71672=CARTESIAN_POINT('Ctrl Pts',(-23.1770659320137,-68.6222317244336,
0.));
#71673=CARTESIAN_POINT('Ctrl Pts',(-23.1770659320137,-68.6222317244336,
12.));
#71674=CARTESIAN_POINT('Ctrl Pts',(-23.1760778585094,-68.6470392174567,
0.));
#71675=CARTESIAN_POINT('Ctrl Pts',(-23.1760778585094,-68.6470392174567,
12.));
#71676=CARTESIAN_POINT('Ctrl Pts',(-23.1750643563606,-68.6718862065227,
0.));
#71677=CARTESIAN_POINT('Ctrl Pts',(-23.1750643563606,-68.6718862065227,
12.));
#71678=CARTESIAN_POINT('Ctrl Pts',(-23.1740253733423,-68.6967725797457,
0.));
#71679=CARTESIAN_POINT('Ctrl Pts',(-23.1740253733423,-68.6967725797457,
12.));
#71680=CARTESIAN_POINT('Ctrl Pts',(-23.1729608575115,-68.7216982256357,
0.));
#71681=CARTESIAN_POINT('Ctrl Pts',(-23.1729608575115,-68.7216982256357,
12.));
#71682=CARTESIAN_POINT('Ctrl Pts',(-23.1718707572047,-68.7466630330968,
0.));
#71683=CARTESIAN_POINT('Ctrl Pts',(-23.1718707572047,-68.7466630330968,
12.));
#71684=CARTESIAN_POINT('Ctrl Pts',(-23.1707550210359,-68.7716668914246,
0.));
#71685=CARTESIAN_POINT('Ctrl Pts',(-23.1707550210359,-68.7716668914246,
12.));
#71686=CARTESIAN_POINT('Ctrl Pts',(-23.1696135978993,-68.7967096902981,
0.));
#71687=CARTESIAN_POINT('Ctrl Pts',(-23.1696135978993,-68.7967096902981,
12.));
#71688=CARTESIAN_POINT('Ctrl Pts',(-23.1684464369681,-68.8217913197735,
0.));
#71689=CARTESIAN_POINT('Ctrl Pts',(-23.1684464369681,-68.8217913197735,
12.));
#71690=CARTESIAN_POINT('Ctrl Pts',(-23.1672534876885,-68.8469116702885,
0.));
#71691=CARTESIAN_POINT('Ctrl Pts',(-23.1672534876885,-68.8469116702885,
12.));
#71692=CARTESIAN_POINT('Ctrl Pts',(-23.1660346997763,-68.8720706326606,
0.));
#71693=CARTESIAN_POINT('Ctrl Pts',(-23.1660346997763,-68.8720706326606,
12.));
#71694=CARTESIAN_POINT('Ctrl Pts',(-23.1647900232152,-68.8972680980844,
0.));
#71695=CARTESIAN_POINT('Ctrl Pts',(-23.1647900232152,-68.8972680980844,
12.));
#71696=CARTESIAN_POINT('Ctrl Pts',(-23.1635194082582,-68.9225039581249,
0.));
#71697=CARTESIAN_POINT('Ctrl Pts',(-23.1635194082582,-68.9225039581249,
12.));
#71698=CARTESIAN_POINT('Ctrl Pts',(-23.162222805429,-68.9477781047103,0.));
#71699=CARTESIAN_POINT('Ctrl Pts',(-23.162222805429,-68.9477781047103,12.));
#71700=CARTESIAN_POINT('Ctrl Pts',(-23.1609001655154,-68.9730904301362,
0.));
#71701=CARTESIAN_POINT('Ctrl Pts',(-23.1609001655154,-68.9730904301362,
12.));
#71702=CARTESIAN_POINT('Ctrl Pts',(-23.1595514395655,-68.9984408270652,
0.));
#71703=CARTESIAN_POINT('Ctrl Pts',(-23.1595514395655,-68.9984408270652,
12.));
#71704=CARTESIAN_POINT('Ctrl Pts',(-23.1581765788869,-69.0238291885245,
0.));
#71705=CARTESIAN_POINT('Ctrl Pts',(-23.1581765788869,-69.0238291885245,
12.));
#71706=CARTESIAN_POINT('Ctrl Pts',(-23.1567755350472,-69.0492554078999,
0.));
#71707=CARTESIAN_POINT('Ctrl Pts',(-23.1567755350472,-69.0492554078999,
12.));
#71708=CARTESIAN_POINT('Ctrl Pts',(-23.1553482598768,-69.0747193789291,
0.));
#71709=CARTESIAN_POINT('Ctrl Pts',(-23.1553482598768,-69.0747193789291,
12.));
#71710=CARTESIAN_POINT('Ctrl Pts',(-23.153894705462,-69.1002209957036,0.));
#71711=CARTESIAN_POINT('Ctrl Pts',(-23.153894705462,-69.1002209957036,12.));
#71712=CARTESIAN_POINT('Ctrl Pts',(-23.1524148241413,-69.1257601526692,
0.));
#71713=CARTESIAN_POINT('Ctrl Pts',(-23.1524148241413,-69.1257601526692,
12.));
#71714=CARTESIAN_POINT('Ctrl Pts',(-23.1509085685033,-69.1513367446231,
0.));
#71715=CARTESIAN_POINT('Ctrl Pts',(-23.1509085685033,-69.1513367446231,
12.));
#71716=CARTESIAN_POINT('Ctrl Pts',(-23.1493758913857,-69.176950666708,0.));
#71717=CARTESIAN_POINT('Ctrl Pts',(-23.1493758913857,-69.176950666708,12.));
#71718=CARTESIAN_POINT('Ctrl Pts',(-23.1478167458787,-69.2026018144023,
0.));
#71719=CARTESIAN_POINT('Ctrl Pts',(-23.1478167458787,-69.2026018144023,
12.));
#71720=CARTESIAN_POINT('Ctrl Pts',(-23.1462310853205,-69.2282900835234,
0.));
#71721=CARTESIAN_POINT('Ctrl Pts',(-23.1462310853205,-69.2282900835234,
12.));
#71722=CARTESIAN_POINT('Ctrl Pts',(-23.1446188632931,-69.2540153702311,
0.));
#71723=CARTESIAN_POINT('Ctrl Pts',(-23.1446188632931,-69.2540153702311,
12.));
#71724=CARTESIAN_POINT('Ctrl Pts',(-23.1429800336221,-69.2797775710275,
0.));
#71725=CARTESIAN_POINT('Ctrl Pts',(-23.1429800336221,-69.2797775710275,
12.));
#71726=CARTESIAN_POINT('Ctrl Pts',(-23.1413145503762,-69.3055765827544,
0.));
#71727=CARTESIAN_POINT('Ctrl Pts',(-23.1413145503762,-69.3055765827544,
12.));
#71728=CARTESIAN_POINT('Ctrl Pts',(-23.1396223678725,-69.3314123025863,
0.));
#71729=CARTESIAN_POINT('Ctrl Pts',(-23.1396223678725,-69.3314123025863,
12.));
#71730=CARTESIAN_POINT('Ctrl Pts',(-23.1379034406718,-69.3572846280289,
0.));
#71731=CARTESIAN_POINT('Ctrl Pts',(-23.1379034406718,-69.3572846280289,
12.));
#71732=CARTESIAN_POINT('Ctrl Pts',(-23.1361577235708,-69.3831934569176,
0.));
#71733=CARTESIAN_POINT('Ctrl Pts',(-23.1361577235708,-69.3831934569176,
12.));
#71734=CARTESIAN_POINT('Ctrl Pts',(-23.1343851715989,-69.4091386874129,
0.));
#71735=CARTESIAN_POINT('Ctrl Pts',(-23.1343851715989,-69.4091386874129,
12.));
#71736=CARTESIAN_POINT('Ctrl Pts',(-23.1325857400145,-69.4351202179948,
0.));
#71737=CARTESIAN_POINT('Ctrl Pts',(-23.1325857400145,-69.4351202179948,
12.));
#71738=CARTESIAN_POINT('Ctrl Pts',(-23.1307593843063,-69.4611379474492,
0.));
#71739=CARTESIAN_POINT('Ctrl Pts',(-23.1307593843063,-69.4611379474492,
12.));
#71740=CARTESIAN_POINT('Ctrl Pts',(-23.1289060601927,-69.4871917748665,
0.));
#71741=CARTESIAN_POINT('Ctrl Pts',(-23.1289060601927,-69.4871917748665,
12.));
#71742=CARTESIAN_POINT('Ctrl Pts',(-23.1270257236207,-69.5132815996548,
0.));
#71743=CARTESIAN_POINT('Ctrl Pts',(-23.1270257236207,-69.5132815996548,
12.));
#71744=CARTESIAN_POINT('Ctrl Pts',(-23.1251183307678,-69.5394073215467,
0.));
#71745=CARTESIAN_POINT('Ctrl Pts',(-23.1251183307678,-69.5394073215467,
12.));
#71746=CARTESIAN_POINT('Ctrl Pts',(-23.1231838380452,-69.565568840605,0.));
#71747=CARTESIAN_POINT('Ctrl Pts',(-23.1231838380452,-69.565568840605,12.));
#71748=CARTESIAN_POINT('Ctrl Pts',(-23.1212222021049,-69.5917660572255,
0.));
#71749=CARTESIAN_POINT('Ctrl Pts',(-23.1212222021049,-69.5917660572255,
12.));
#71750=CARTESIAN_POINT('Ctrl Pts',(-23.1192333798438,-69.617998872135,0.));
#71751=CARTESIAN_POINT('Ctrl Pts',(-23.1192333798438,-69.617998872135,12.));
#71752=CARTESIAN_POINT('Ctrl Pts',(-23.1172173283856,-69.6442671863751,
0.));
#71753=CARTESIAN_POINT('Ctrl Pts',(-23.1172173283856,-69.6442671863751,
12.));
#71754=CARTESIAN_POINT('Ctrl Pts',(-23.1151740050679,-69.6705709012842,
0.));
#71755=CARTESIAN_POINT('Ctrl Pts',(-23.1151740050679,-69.6705709012842,
12.));
#71756=CARTESIAN_POINT('Ctrl Pts',(-23.1131033674301,-69.6969099184766,
0.));
#71757=CARTESIAN_POINT('Ctrl Pts',(-23.1131033674301,-69.6969099184766,
12.));
#71758=CARTESIAN_POINT('Ctrl Pts',(-23.111005373205,-69.7232841398207,0.));
#71759=CARTESIAN_POINT('Ctrl Pts',(-23.111005373205,-69.7232841398207,12.));
#71760=CARTESIAN_POINT('Ctrl Pts',(-23.1088799803094,-69.7496934674083,
0.));
#71761=CARTESIAN_POINT('Ctrl Pts',(-23.1088799803094,-69.7496934674083,
12.));
#71762=CARTESIAN_POINT('Ctrl Pts',(-23.1067271468614,-69.7761378035979,
0.));
#71763=CARTESIAN_POINT('Ctrl Pts',(-23.1067271468614,-69.7761378035979,
12.));
#71764=CARTESIAN_POINT('Ctrl Pts',(-23.1045468311994,-69.8026170510582,
0.));
#71765=CARTESIAN_POINT('Ctrl Pts',(-23.1045468311994,-69.8026170510582,
12.));
#71766=CARTESIAN_POINT('Ctrl Pts',(-23.1023389919052,-69.8291311128121,
0.));
#71767=CARTESIAN_POINT('Ctrl Pts',(-23.1023389919052,-69.8291311128121,
12.));
#71768=CARTESIAN_POINT('Ctrl Pts',(-23.100103587824,-69.8556798922688,0.));
#71769=CARTESIAN_POINT('Ctrl Pts',(-23.100103587824,-69.8556798922688,12.));
#71770=CARTESIAN_POINT('Ctrl Pts',(-23.0978405781018,-69.8822632932759,
0.));
#71771=CARTESIAN_POINT('Ctrl Pts',(-23.0978405781018,-69.8822632932759,
12.));
#71772=CARTESIAN_POINT('Ctrl Pts',(-23.0955499221556,-69.9088812200703,
0.));
#71773=CARTESIAN_POINT('Ctrl Pts',(-23.0955499221556,-69.9088812200703,
12.));
#71774=CARTESIAN_POINT('Ctrl Pts',(-23.0932315796066,-69.9355335771722,
0.));
#71775=CARTESIAN_POINT('Ctrl Pts',(-23.0932315796066,-69.9355335771722,
12.));
#71776=CARTESIAN_POINT('Ctrl Pts',(-23.0908855102251,-69.9622202692871,
0.));
#71777=CARTESIAN_POINT('Ctrl Pts',(-23.0908855102251,-69.9622202692871,
12.));
#71778=CARTESIAN_POINT('Ctrl Pts',(-23.0885116738798,-69.9889412012143,
0.));
#71779=CARTESIAN_POINT('Ctrl Pts',(-23.0885116738798,-69.9889412012143,
12.));
#71780=CARTESIAN_POINT('Ctrl Pts',(-23.0861100304731,-70.0156962777173,
0.));
#71781=CARTESIAN_POINT('Ctrl Pts',(-23.0861100304731,-70.0156962777173,
12.));
#71782=CARTESIAN_POINT('Ctrl Pts',(-23.0836805399378,-70.0424854035125,
0.));
#71783=CARTESIAN_POINT('Ctrl Pts',(-23.0836805399378,-70.0424854035125,
12.));
#71784=CARTESIAN_POINT('Ctrl Pts',(-23.081223162377,-70.0693084835387,0.));
#71785=CARTESIAN_POINT('Ctrl Pts',(-23.081223162377,-70.0693084835387,12.));
#71786=CARTESIAN_POINT('Ctrl Pts',(-23.0787378581778,-70.096165423165,0.));
#71787=CARTESIAN_POINT('Ctrl Pts',(-23.0787378581778,-70.096165423165,12.));
#71788=CARTESIAN_POINT('Ctrl Pts',(-23.076224588139,-70.1230561284222,0.));
#71789=CARTESIAN_POINT('Ctrl Pts',(-23.076224588139,-70.1230561284222,12.));
#71790=CARTESIAN_POINT('Ctrl Pts',(-23.0736833135934,-70.1499805062159,
0.));
#71791=CARTESIAN_POINT('Ctrl Pts',(-23.0736833135934,-70.1499805062159,
12.));
#71792=CARTESIAN_POINT('Ctrl Pts',(-23.0711139965432,-70.176938464556,0.));
#71793=CARTESIAN_POINT('Ctrl Pts',(-23.0711139965432,-70.176938464556,12.));
#71794=CARTESIAN_POINT('Ctrl Pts',(-23.0685165993681,-70.2039299120456,
0.));
#71795=CARTESIAN_POINT('Ctrl Pts',(-23.0685165993681,-70.2039299120456,
12.));
#71796=CARTESIAN_POINT('Ctrl Pts',(-23.0658910845425,-70.2309547573788,
0.));
#71797=CARTESIAN_POINT('Ctrl Pts',(-23.0658910845425,-70.2309547573788,
12.));
#71798=CARTESIAN_POINT('Ctrl Pts',(-23.0632374143276,-70.2580129087877,
0.));
#71799=CARTESIAN_POINT('Ctrl Pts',(-23.0632374143276,-70.2580129087877,
12.));
#71800=CARTESIAN_POINT('Ctrl Pts',(-23.0605555505326,-70.2851042736081,
0.));
#71801=CARTESIAN_POINT('Ctrl Pts',(-23.0605555505326,-70.2851042736081,
12.));
#71802=CARTESIAN_POINT('Ctrl Pts',(-23.0578454541116,-70.3122287575374,
0.));
#71803=CARTESIAN_POINT('Ctrl Pts',(-23.0578454541116,-70.3122287575374,
12.));
#71804=CARTESIAN_POINT('Ctrl Pts',(-23.0551070854942,-70.3393862652353,
0.));
#71805=CARTESIAN_POINT('Ctrl Pts',(-23.0551070854942,-70.3393862652353,
12.));
#71806=CARTESIAN_POINT('Ctrl Pts',(-23.0523404053188,-70.3665767016596,
0.));
#71807=CARTESIAN_POINT('Ctrl Pts',(-23.0523404053188,-70.3665767016596,
12.));
#71808=CARTESIAN_POINT('Ctrl Pts',(-23.0495453750773,-70.39379997323,0.));
#71809=CARTESIAN_POINT('Ctrl Pts',(-23.0495453750773,-70.39379997323,12.));
#71810=CARTESIAN_POINT('Ctrl Pts',(-23.0467219577289,-70.421055988934,0.));
#71811=CARTESIAN_POINT('Ctrl Pts',(-23.0467219577289,-70.421055988934,12.));
#71812=CARTESIAN_POINT('Ctrl Pts',(-23.0438701184995,-70.4483446617553,
0.));
#71813=CARTESIAN_POINT('Ctrl Pts',(-23.0438701184995,-70.4483446617553,
12.));
#71814=CARTESIAN_POINT('Ctrl Pts',(-23.0409898250726,-70.4756659090104,
0.));
#71815=CARTESIAN_POINT('Ctrl Pts',(-23.0409898250726,-70.4756659090104,
12.));
#71816=CARTESIAN_POINT('Ctrl Pts',(-23.0380810458237,-70.5030196491883,
0.));
#71817=CARTESIAN_POINT('Ctrl Pts',(-23.0380810458237,-70.5030196491883,
12.));
#71818=CARTESIAN_POINT('Ctrl Pts',(-23.035143748431,-70.5304057994537,0.));
#71819=CARTESIAN_POINT('Ctrl Pts',(-23.035143748431,-70.5304057994537,12.));
#71820=CARTESIAN_POINT('Ctrl Pts',(-23.0321778982705,-70.5578242727606,
0.));
#71821=CARTESIAN_POINT('Ctrl Pts',(-23.0321778982705,-70.5578242727606,
12.));
#71822=CARTESIAN_POINT('Ctrl Pts',(-23.0291834570688,-70.5852749754167,
0.));
#71823=CARTESIAN_POINT('Ctrl Pts',(-23.0291834570688,-70.5852749754167,
12.));
#71824=CARTESIAN_POINT('Ctrl Pts',(-23.0261603810187,-70.6127578036869,
0.));
#71825=CARTESIAN_POINT('Ctrl Pts',(-23.0261603810187,-70.6127578036869,
12.));
#71826=CARTESIAN_POINT('Ctrl Pts',(-23.0231086235263,-70.6402726486718,
0.));
#71827=CARTESIAN_POINT('Ctrl Pts',(-23.0231086235263,-70.6402726486718,
12.));
#71828=CARTESIAN_POINT('Ctrl Pts',(-23.0200281385906,-70.6678194023389,
0.));
#71829=CARTESIAN_POINT('Ctrl Pts',(-23.0200281385906,-70.6678194023389,
12.));
#71830=CARTESIAN_POINT('Ctrl Pts',(-23.0169188841084,-70.6953979633561,
0.));
#71831=CARTESIAN_POINT('Ctrl Pts',(-23.0169188841084,-70.6953979633561,
12.));
#71832=CARTESIAN_POINT('Ctrl Pts',(-23.0137808248899,-70.7230082425324,
0.));
#71833=CARTESIAN_POINT('Ctrl Pts',(-23.0137808248899,-70.7230082425324,
12.));
#71834=CARTESIAN_POINT('Ctrl Pts',(-23.0106139365941,-70.7506501695822,
0.));
#71835=CARTESIAN_POINT('Ctrl Pts',(-23.0106139365941,-70.7506501695822,
12.));
#71836=CARTESIAN_POINT('Ctrl Pts',(-23.0074182063611,-70.7783236950588,
0.));
#71837=CARTESIAN_POINT('Ctrl Pts',(-23.0074182063611,-70.7783236950588,
12.));
#71838=CARTESIAN_POINT('Ctrl Pts',(-23.004193629142,-70.806028785987,0.));
#71839=CARTESIAN_POINT('Ctrl Pts',(-23.004193629142,-70.806028785987,12.));
#71840=CARTESIAN_POINT('Ctrl Pts',(-23.0015908899222,-70.8282180956627,
0.));
#71841=CARTESIAN_POINT('Ctrl Pts',(-23.0015908899222,-70.8282180956627,
12.));
#71842=CARTESIAN_POINT('Ctrl Pts',(-22.9996258555187,-70.8448742696329,
0.));
#71843=CARTESIAN_POINT('Ctrl Pts',(-22.9996258555187,-70.8448742696329,
12.));
#71844=CARTESIAN_POINT('Ctrl Pts',(-22.9983100639354,-70.8559846927868,
0.));
#71845=CARTESIAN_POINT('Ctrl Pts',(-22.9983100639354,-70.8559846927868,
12.));
#71846=CARTESIAN_POINT('Ctrl Pts',(-22.9976507259817,-70.8615414811571,
0.));
#71847=CARTESIAN_POINT('Ctrl Pts',(-22.9976507259817,-70.8615414811571,
12.));
#71848=CARTESIAN_POINT('',(-23.1372951448024,-66.0656156664138,0.));
#71849=CARTESIAN_POINT('Ctrl Pts',(-23.1372951448024,-66.0656156664138,
0.));
#71850=CARTESIAN_POINT('Ctrl Pts',(-23.1375957166104,-66.0694876382127,
0.));
#71851=CARTESIAN_POINT('Ctrl Pts',(-23.13819515974,-66.0772371487248,0.));
#71852=CARTESIAN_POINT('Ctrl Pts',(-23.1390892229779,-66.088878115242,0.));
#71853=CARTESIAN_POINT('Ctrl Pts',(-23.1402711039425,-66.1044328067355,
0.));
#71854=CARTESIAN_POINT('Ctrl Pts',(-23.1417314398398,-66.1239318368548,
0.));
#71855=CARTESIAN_POINT('Ctrl Pts',(-23.1431747350098,-66.1434865015027,
0.));
#71856=CARTESIAN_POINT('Ctrl Pts',(-23.1446009424903,-66.1630967296747,
0.));
#71857=CARTESIAN_POINT('Ctrl Pts',(-23.1460099850763,-66.18276239029,0.));
#71858=CARTESIAN_POINT('Ctrl Pts',(-23.1474017566484,-66.2024832934866,
0.));
#71859=CARTESIAN_POINT('Ctrl Pts',(-23.1487761349328,-66.2222592165473,
0.));
#71860=CARTESIAN_POINT('Ctrl Pts',(-23.1501329914488,-66.2420899237317,
0.));
#71861=CARTESIAN_POINT('Ctrl Pts',(-23.1514722022483,-66.2619751878741,
0.));
#71862=CARTESIAN_POINT('Ctrl Pts',(-23.1527936592625,-66.2819148131072,
0.));
#71863=CARTESIAN_POINT('Ctrl Pts',(-23.154097266617,-66.301908627539,0.));
#71864=CARTESIAN_POINT('Ctrl Pts',(-23.1553829352531,-66.3219564725161,
0.));
#71865=CARTESIAN_POINT('Ctrl Pts',(-23.1566505784626,-66.3420581937159,
0.));
#71866=CARTESIAN_POINT('Ctrl Pts',(-23.1579001063438,-66.3622136300692,
0.));
#71867=CARTESIAN_POINT('Ctrl Pts',(-23.1591314230101,-66.382422608185,0.));
#71868=CARTESIAN_POINT('Ctrl Pts',(-23.1603444294754,-66.402684948127,0.));
#71869=CARTESIAN_POINT('Ctrl Pts',(-23.1615390254635,-66.4230004670288,
0.));
#71870=CARTESIAN_POINT('Ctrl Pts',(-23.1627151114875,-66.4433689832454,
0.));
#71871=CARTESIAN_POINT('Ctrl Pts',(-23.163872591218,-66.4637903210682,0.));
#71872=CARTESIAN_POINT('Ctrl Pts',(-23.1650113713792,-66.4842643105263,
0.));
#71873=CARTESIAN_POINT('Ctrl Pts',(-23.1661313606123,-66.5047907851319,
0.));
#71874=CARTESIAN_POINT('Ctrl Pts',(-23.1672324686928,-66.5253695803209,
0.));
#71875=CARTESIAN_POINT('Ctrl Pts',(-23.1683146055736,-66.5460005315406,
0.));
#71876=CARTESIAN_POINT('Ctrl Pts',(-23.169377680588,-66.5666834726494,0.));
#71877=CARTESIAN_POINT('Ctrl Pts',(-23.1704216028626,-66.5874182367596,
0.));
#71878=CARTESIAN_POINT('Ctrl Pts',(-23.1714462816794,-66.6082046569657,
0.));
#71879=CARTESIAN_POINT('Ctrl Pts',(-23.1724516268299,-66.6290425670538,
0.));
#71880=CARTESIAN_POINT('Ctrl Pts',(-23.1734375490421,-66.6499318023445,
0.));
#71881=CARTESIAN_POINT('Ctrl Pts',(-23.174403960137,-66.6708722000046,0.));
#71882=CARTESIAN_POINT('Ctrl Pts',(-23.1753507727932,-66.691863598595,0.));
#71883=CARTESIAN_POINT('Ctrl Pts',(-23.1762779004043,-66.712905837789,0.));
#71884=CARTESIAN_POINT('Ctrl Pts',(-23.1771852569137,-66.7339987580441,
0.));
#71885=CARTESIAN_POINT('Ctrl Pts',(-23.1780727566309,-66.7551422002229,
0.));
#71886=CARTESIAN_POINT('Ctrl Pts',(-23.1789403142376,-66.7763360056146,
0.));
#71887=CARTESIAN_POINT('Ctrl Pts',(-23.1797878448645,-66.7975800161014,
0.));
#71888=CARTESIAN_POINT('Ctrl Pts',(-23.1806152641475,-66.8188740742727,
0.));
#71889=CARTESIAN_POINT('Ctrl Pts',(-23.1814224882948,-66.8402180235549,
0.));
#71890=CARTESIAN_POINT('Ctrl Pts',(-23.1822094341508,-66.8616117083304,
0.));
#71891=CARTESIAN_POINT('Ctrl Pts',(-23.1829760191583,-66.8830549738768,
0.));
#71892=CARTESIAN_POINT('Ctrl Pts',(-23.1837221613231,-66.904547666305,0.));
#71893=CARTESIAN_POINT('Ctrl Pts',(-23.1844477791816,-66.9260896324955,
0.));
#71894=CARTESIAN_POINT('Ctrl Pts',(-23.1851527917666,-66.9476807200225,
0.));
#71895=CARTESIAN_POINT('Ctrl Pts',(-23.1858371185852,-66.9693207771058,
0.));
#71896=CARTESIAN_POINT('Ctrl Pts',(-23.1865006796291,-66.9910096526483,
0.));
#71897=CARTESIAN_POINT('Ctrl Pts',(-23.1871433953795,-67.0127471962507,
0.));
#71898=CARTESIAN_POINT('Ctrl Pts',(-23.1877651868155,-67.0345332582297,
0.));
#71899=CARTESIAN_POINT('Ctrl Pts',(-23.1883659754268,-67.0563676896312,
0.));
#71900=CARTESIAN_POINT('Ctrl Pts',(-23.1889456832116,-67.0782503422293,
0.));
#71901=CARTESIAN_POINT('Ctrl Pts',(-23.1895042326626,-67.1001810685138,
0.));
#71902=CARTESIAN_POINT('Ctrl Pts',(-23.1900415467575,-67.122159721674,0.));
#71903=CARTESIAN_POINT('Ctrl Pts',(-23.1905575489506,-67.1441861555819,
0.));
#71904=CARTESIAN_POINT('Ctrl Pts',(-23.1910521631658,-67.1662602247641,
0.));
#71905=CARTESIAN_POINT('Ctrl Pts',(-23.1915253137924,-67.1883817844039,
0.));
#71906=CARTESIAN_POINT('Ctrl Pts',(-23.1919769256803,-67.2105506903448,
0.));
#71907=CARTESIAN_POINT('Ctrl Pts',(-23.1924069241386,-67.232766799088,0.));
#71908=CARTESIAN_POINT('Ctrl Pts',(-23.1928152349344,-67.2550299677888,
0.));
#71909=CARTESIAN_POINT('Ctrl Pts',(-23.1932017842954,-67.2773400542477,
0.));
#71910=CARTESIAN_POINT('Ctrl Pts',(-23.193566498902,-67.2996969169099,0.));
#71911=CARTESIAN_POINT('Ctrl Pts',(-23.1939093058802,-67.3221004148604,
0.));
#71912=CARTESIAN_POINT('Ctrl Pts',(-23.1942301327979,-67.3445504078178,
0.));
#71913=CARTESIAN_POINT('Ctrl Pts',(-23.1945289076608,-67.3670467561205,
0.));
#71914=CARTESIAN_POINT('Ctrl Pts',(-23.1948055589123,-67.3895893207168,
0.));
#71915=CARTESIAN_POINT('Ctrl Pts',(-23.195060015426,-67.4121779631666,0.));
#71916=CARTESIAN_POINT('Ctrl Pts',(-23.1952922065009,-67.4348125456389,
0.));
#71917=CARTESIAN_POINT('Ctrl Pts',(-23.1955020618591,-67.4574929309078,
0.));
#71918=CARTESIAN_POINT('Ctrl Pts',(-23.1956895116446,-67.4802189823423,
0.));
#71919=CARTESIAN_POINT('Ctrl Pts',(-23.1958544864224,-67.5029905638973,
0.));
#71920=CARTESIAN_POINT('Ctrl Pts',(-23.195996917171,-67.525807540117,0.));
#71921=CARTESIAN_POINT('Ctrl Pts',(-23.1961167352777,-67.5486697761301,
0.));
#71922=CARTESIAN_POINT('Ctrl Pts',(-23.1962138725358,-67.5715771376454,
0.));
#71923=CARTESIAN_POINT('Ctrl Pts',(-23.1962882611444,-67.5945294909398,
0.));
#71924=CARTESIAN_POINT('Ctrl Pts',(-23.1963398337056,-67.6175267028516,
0.));
#71925=CARTESIAN_POINT('Ctrl Pts',(-23.1963685232176,-67.6405686407828,
0.));
#71926=CARTESIAN_POINT('Ctrl Pts',(-23.196374263071,-67.6636551726948,0.));
#71927=CARTESIAN_POINT('Ctrl Pts',(-23.1963569870457,-67.6867861671044,
0.));
#71928=CARTESIAN_POINT('Ctrl Pts',(-23.1963166293116,-67.7099614930712,
0.));
#71929=CARTESIAN_POINT('Ctrl Pts',(-23.1962531244261,-67.7331810201931,
0.));
#71930=CARTESIAN_POINT('Ctrl Pts',(-23.1961664073274,-67.7564446186115,
0.));
#71931=CARTESIAN_POINT('Ctrl Pts',(-23.1960564133308,-67.7797521590056,
0.));
#71932=CARTESIAN_POINT('Ctrl Pts',(-23.1959230781265,-67.8031035125873,
0.));
#71933=CARTESIAN_POINT('Ctrl Pts',(-23.1957663377798,-67.8264985510884,
0.));
#71934=CARTESIAN_POINT('Ctrl Pts',(-23.1955861287276,-67.8499371467578,
0.));
#71935=CARTESIAN_POINT('Ctrl Pts',(-23.1953823877727,-67.8734191723639,
0.));
#71936=CARTESIAN_POINT('Ctrl Pts',(-23.19515505208,-67.8969445011908,0.));
#71937=CARTESIAN_POINT('Ctrl Pts',(-23.1949040591748,-67.9205130070337,
0.));
#71938=CARTESIAN_POINT('Ctrl Pts',(-23.1946293469437,-67.944124564187,0.));
#71939=CARTESIAN_POINT('Ctrl Pts',(-23.1943308536307,-67.9677790474414,
0.));
#71940=CARTESIAN_POINT('Ctrl Pts',(-23.194008517832,-67.9914763320878,0.));
#71941=CARTESIAN_POINT('Ctrl Pts',(-23.193662278492,-68.0152162939123,0.));
#71942=CARTESIAN_POINT('Ctrl Pts',(-23.1932920749021,-68.0389988091926,
0.));
#71943=CARTESIAN_POINT('Ctrl Pts',(-23.1928978467018,-68.0628237546852,
0.));
#71944=CARTESIAN_POINT('Ctrl Pts',(-23.1924795338746,-68.086691007624,0.));
#71945=CARTESIAN_POINT('Ctrl Pts',(-23.1920370767424,-68.1106004457223,
0.));
#71946=CARTESIAN_POINT('Ctrl Pts',(-23.1915704159624,-68.1345519471695,
0.));
#71947=CARTESIAN_POINT('Ctrl Pts',(-23.1910794925252,-68.1585453906259,
0.));
#71948=CARTESIAN_POINT('Ctrl Pts',(-23.1905642477572,-68.182580655213,0.));
#71949=CARTESIAN_POINT('Ctrl Pts',(-23.1900246233165,-68.2066576205113,
0.));
#71950=CARTESIAN_POINT('Ctrl Pts',(-23.189460561187,-68.2307761665629,0.));
#71951=CARTESIAN_POINT('Ctrl Pts',(-23.1888720036757,-68.2549361738679,
0.));
#71952=CARTESIAN_POINT('Ctrl Pts',(-23.1882588934108,-68.2791375233798,
0.));
#71953=CARTESIAN_POINT('Ctrl Pts',(-23.1876211733439,-68.3033800964946,
0.));
#71954=CARTESIAN_POINT('Ctrl Pts',(-23.1869587867463,-68.3276637750494,
0.));
#71955=CARTESIAN_POINT('Ctrl Pts',(-23.1862716772034,-68.3519884413253,
0.));
#71956=CARTESIAN_POINT('Ctrl Pts',(-23.1855597886117,-68.3763539780442,
0.));
#71957=CARTESIAN_POINT('Ctrl Pts',(-23.1848230651776,-68.4007602683649,
0.));
#71958=CARTESIAN_POINT('Ctrl Pts',(-23.1840614514191,-68.4252071958725,
0.));
#71959=CARTESIAN_POINT('Ctrl Pts',(-23.1832748921629,-68.4496946445756,
0.));
#71960=CARTESIAN_POINT('Ctrl Pts',(-23.1824633325385,-68.4742224989099,
0.));
#71961=CARTESIAN_POINT('Ctrl Pts',(-23.1816267179752,-68.4987906437357,
0.));
#71962=CARTESIAN_POINT('Ctrl Pts',(-23.1807649942011,-68.5233989643344,
0.));
#71963=CARTESIAN_POINT('Ctrl Pts',(-23.1798781072449,-68.548047346398,0.));
#71964=CARTESIAN_POINT('Ctrl Pts',(-23.178966003434,-68.572735676027,0.));
#71965=CARTESIAN_POINT('Ctrl Pts',(-23.1780286293873,-68.5974638397322,
0.));
#71966=CARTESIAN_POINT('Ctrl Pts',(-23.1770659320137,-68.6222317244336,
0.));
#71967=CARTESIAN_POINT('Ctrl Pts',(-23.1760778585094,-68.6470392174567,
0.));
#71968=CARTESIAN_POINT('Ctrl Pts',(-23.1750643563606,-68.6718862065227,
0.));
#71969=CARTESIAN_POINT('Ctrl Pts',(-23.1740253733423,-68.6967725797457,
0.));
#71970=CARTESIAN_POINT('Ctrl Pts',(-23.1729608575115,-68.7216982256357,
0.));
#71971=CARTESIAN_POINT('Ctrl Pts',(-23.1718707572047,-68.7466630330968,
0.));
#71972=CARTESIAN_POINT('Ctrl Pts',(-23.1707550210359,-68.7716668914246,
0.));
#71973=CARTESIAN_POINT('Ctrl Pts',(-23.1696135978993,-68.7967096902981,
0.));
#71974=CARTESIAN_POINT('Ctrl Pts',(-23.1684464369681,-68.8217913197735,
0.));
#71975=CARTESIAN_POINT('Ctrl Pts',(-23.1672534876885,-68.8469116702885,
0.));
#71976=CARTESIAN_POINT('Ctrl Pts',(-23.1660346997763,-68.8720706326606,
0.));
#71977=CARTESIAN_POINT('Ctrl Pts',(-23.1647900232152,-68.8972680980844,
0.));
#71978=CARTESIAN_POINT('Ctrl Pts',(-23.1635194082582,-68.9225039581249,
0.));
#71979=CARTESIAN_POINT('Ctrl Pts',(-23.162222805429,-68.9477781047103,0.));
#71980=CARTESIAN_POINT('Ctrl Pts',(-23.1609001655154,-68.9730904301362,
0.));
#71981=CARTESIAN_POINT('Ctrl Pts',(-23.1595514395655,-68.9984408270652,
0.));
#71982=CARTESIAN_POINT('Ctrl Pts',(-23.1581765788869,-69.0238291885245,
0.));
#71983=CARTESIAN_POINT('Ctrl Pts',(-23.1567755350472,-69.0492554078999,
0.));
#71984=CARTESIAN_POINT('Ctrl Pts',(-23.1553482598768,-69.0747193789291,
0.));
#71985=CARTESIAN_POINT('Ctrl Pts',(-23.153894705462,-69.1002209957036,0.));
#71986=CARTESIAN_POINT('Ctrl Pts',(-23.1524148241413,-69.1257601526692,
0.));
#71987=CARTESIAN_POINT('Ctrl Pts',(-23.1509085685033,-69.1513367446231,
0.));
#71988=CARTESIAN_POINT('Ctrl Pts',(-23.1493758913857,-69.176950666708,0.));
#71989=CARTESIAN_POINT('Ctrl Pts',(-23.1478167458787,-69.2026018144023,
0.));
#71990=CARTESIAN_POINT('Ctrl Pts',(-23.1462310853205,-69.2282900835234,
0.));
#71991=CARTESIAN_POINT('Ctrl Pts',(-23.1446188632931,-69.2540153702311,
0.));
#71992=CARTESIAN_POINT('Ctrl Pts',(-23.1429800336221,-69.2797775710275,
0.));
#71993=CARTESIAN_POINT('Ctrl Pts',(-23.1413145503762,-69.3055765827544,
0.));
#71994=CARTESIAN_POINT('Ctrl Pts',(-23.1396223678725,-69.3314123025863,
0.));
#71995=CARTESIAN_POINT('Ctrl Pts',(-23.1379034406718,-69.3572846280289,
0.));
#71996=CARTESIAN_POINT('Ctrl Pts',(-23.1361577235708,-69.3831934569176,
0.));
#71997=CARTESIAN_POINT('Ctrl Pts',(-23.1343851715989,-69.4091386874129,
0.));
#71998=CARTESIAN_POINT('Ctrl Pts',(-23.1325857400145,-69.4351202179948,
0.));
#71999=CARTESIAN_POINT('Ctrl Pts',(-23.1307593843063,-69.4611379474492,
0.));
#72000=CARTESIAN_POINT('Ctrl Pts',(-23.1289060601927,-69.4871917748665,
0.));
#72001=CARTESIAN_POINT('Ctrl Pts',(-23.1270257236207,-69.5132815996548,
0.));
#72002=CARTESIAN_POINT('Ctrl Pts',(-23.1251183307678,-69.5394073215467,
0.));
#72003=CARTESIAN_POINT('Ctrl Pts',(-23.1231838380452,-69.565568840605,0.));
#72004=CARTESIAN_POINT('Ctrl Pts',(-23.1212222021049,-69.5917660572255,
0.));
#72005=CARTESIAN_POINT('Ctrl Pts',(-23.1192333798438,-69.617998872135,0.));
#72006=CARTESIAN_POINT('Ctrl Pts',(-23.1172173283856,-69.6442671863751,
0.));
#72007=CARTESIAN_POINT('Ctrl Pts',(-23.1151740050679,-69.6705709012842,
0.));
#72008=CARTESIAN_POINT('Ctrl Pts',(-23.1131033674301,-69.6969099184766,
0.));
#72009=CARTESIAN_POINT('Ctrl Pts',(-23.111005373205,-69.7232841398207,0.));
#72010=CARTESIAN_POINT('Ctrl Pts',(-23.1088799803094,-69.7496934674083,
0.));
#72011=CARTESIAN_POINT('Ctrl Pts',(-23.1067271468614,-69.7761378035979,
0.));
#72012=CARTESIAN_POINT('Ctrl Pts',(-23.1045468311994,-69.8026170510582,
0.));
#72013=CARTESIAN_POINT('Ctrl Pts',(-23.1023389919052,-69.8291311128121,
0.));
#72014=CARTESIAN_POINT('Ctrl Pts',(-23.100103587824,-69.8556798922688,0.));
#72015=CARTESIAN_POINT('Ctrl Pts',(-23.0978405781018,-69.8822632932759,
0.));
#72016=CARTESIAN_POINT('Ctrl Pts',(-23.0955499221556,-69.9088812200703,
0.));
#72017=CARTESIAN_POINT('Ctrl Pts',(-23.0932315796066,-69.9355335771722,
0.));
#72018=CARTESIAN_POINT('Ctrl Pts',(-23.0908855102251,-69.9622202692871,
0.));
#72019=CARTESIAN_POINT('Ctrl Pts',(-23.0885116738798,-69.9889412012143,
0.));
#72020=CARTESIAN_POINT('Ctrl Pts',(-23.0861100304731,-70.0156962777173,
0.));
#72021=CARTESIAN_POINT('Ctrl Pts',(-23.0836805399378,-70.0424854035125,
0.));
#72022=CARTESIAN_POINT('Ctrl Pts',(-23.081223162377,-70.0693084835387,0.));
#72023=CARTESIAN_POINT('Ctrl Pts',(-23.0787378581778,-70.096165423165,0.));
#72024=CARTESIAN_POINT('Ctrl Pts',(-23.076224588139,-70.1230561284222,0.));
#72025=CARTESIAN_POINT('Ctrl Pts',(-23.0736833135934,-70.1499805062159,
0.));
#72026=CARTESIAN_POINT('Ctrl Pts',(-23.0711139965432,-70.176938464556,0.));
#72027=CARTESIAN_POINT('Ctrl Pts',(-23.0685165993681,-70.2039299120456,
0.));
#72028=CARTESIAN_POINT('Ctrl Pts',(-23.0658910845425,-70.2309547573788,
0.));
#72029=CARTESIAN_POINT('Ctrl Pts',(-23.0632374143276,-70.2580129087877,
0.));
#72030=CARTESIAN_POINT('Ctrl Pts',(-23.0605555505326,-70.2851042736081,
0.));
#72031=CARTESIAN_POINT('Ctrl Pts',(-23.0578454541116,-70.3122287575374,
0.));
#72032=CARTESIAN_POINT('Ctrl Pts',(-23.0551070854942,-70.3393862652353,
0.));
#72033=CARTESIAN_POINT('Ctrl Pts',(-23.0523404053188,-70.3665767016596,
0.));
#72034=CARTESIAN_POINT('Ctrl Pts',(-23.0495453750773,-70.39379997323,0.));
#72035=CARTESIAN_POINT('Ctrl Pts',(-23.0467219577289,-70.421055988934,0.));
#72036=CARTESIAN_POINT('Ctrl Pts',(-23.0438701184995,-70.4483446617553,
0.));
#72037=CARTESIAN_POINT('Ctrl Pts',(-23.0409898250726,-70.4756659090104,
0.));
#72038=CARTESIAN_POINT('Ctrl Pts',(-23.0384964376011,-70.4991133648756,
0.));
#72039=CARTESIAN_POINT('Ctrl Pts',(-23.0365694096158,-70.5171075702495,
0.));
#72040=CARTESIAN_POINT('Ctrl Pts',(-23.0352213647764,-70.5296341535252,
0.));
#72041=CARTESIAN_POINT('Ctrl Pts',(-23.034460662331,-70.5366836381299,0.));
#72042=CARTESIAN_POINT('Ctrl Pts',(-23.0342913834093,-70.5382514078489,
0.));
#72043=CARTESIAN_POINT('',(-23.1372951448024,-66.0656156664138,12.));
#72044=CARTESIAN_POINT('',(-23.1372951448024,-66.0656156664138,0.));
#72045=CARTESIAN_POINT('Ctrl Pts',(-23.0342913834093,-70.5382514078489,
12.));
#72046=CARTESIAN_POINT('Ctrl Pts',(-23.034460662331,-70.5366836381299,12.));
#72047=CARTESIAN_POINT('Ctrl Pts',(-23.0352213647764,-70.5296341535252,
12.));
#72048=CARTESIAN_POINT('Ctrl Pts',(-23.0365694096158,-70.5171075702495,
12.));
#72049=CARTESIAN_POINT('Ctrl Pts',(-23.0384964376011,-70.4991133648756,
12.));
#72050=CARTESIAN_POINT('Ctrl Pts',(-23.0409898250726,-70.4756659090104,
12.));
#72051=CARTESIAN_POINT('Ctrl Pts',(-23.0438701184995,-70.4483446617553,
12.));
#72052=CARTESIAN_POINT('Ctrl Pts',(-23.0467219577289,-70.421055988934,12.));
#72053=CARTESIAN_POINT('Ctrl Pts',(-23.0495453750773,-70.39379997323,12.));
#72054=CARTESIAN_POINT('Ctrl Pts',(-23.0523404053188,-70.3665767016596,
12.));
#72055=CARTESIAN_POINT('Ctrl Pts',(-23.0551070854942,-70.3393862652353,
12.));
#72056=CARTESIAN_POINT('Ctrl Pts',(-23.0578454541116,-70.3122287575374,
12.));
#72057=CARTESIAN_POINT('Ctrl Pts',(-23.0605555505326,-70.2851042736081,
12.));
#72058=CARTESIAN_POINT('Ctrl Pts',(-23.0632374143276,-70.2580129087877,
12.));
#72059=CARTESIAN_POINT('Ctrl Pts',(-23.0658910845425,-70.2309547573788,
12.));
#72060=CARTESIAN_POINT('Ctrl Pts',(-23.0685165993681,-70.2039299120456,
12.));
#72061=CARTESIAN_POINT('Ctrl Pts',(-23.0711139965432,-70.176938464556,12.));
#72062=CARTESIAN_POINT('Ctrl Pts',(-23.0736833135934,-70.1499805062159,
12.));
#72063=CARTESIAN_POINT('Ctrl Pts',(-23.076224588139,-70.1230561284222,12.));
#72064=CARTESIAN_POINT('Ctrl Pts',(-23.0787378581778,-70.096165423165,12.));
#72065=CARTESIAN_POINT('Ctrl Pts',(-23.081223162377,-70.0693084835387,12.));
#72066=CARTESIAN_POINT('Ctrl Pts',(-23.0836805399378,-70.0424854035125,
12.));
#72067=CARTESIAN_POINT('Ctrl Pts',(-23.0861100304731,-70.0156962777173,
12.));
#72068=CARTESIAN_POINT('Ctrl Pts',(-23.0885116738798,-69.9889412012143,
12.));
#72069=CARTESIAN_POINT('Ctrl Pts',(-23.0908855102251,-69.9622202692871,
12.));
#72070=CARTESIAN_POINT('Ctrl Pts',(-23.0932315796066,-69.9355335771722,
12.));
#72071=CARTESIAN_POINT('Ctrl Pts',(-23.0955499221556,-69.9088812200703,
12.));
#72072=CARTESIAN_POINT('Ctrl Pts',(-23.0978405781018,-69.8822632932759,
12.));
#72073=CARTESIAN_POINT('Ctrl Pts',(-23.100103587824,-69.8556798922688,12.));
#72074=CARTESIAN_POINT('Ctrl Pts',(-23.1023389919052,-69.8291311128121,
12.));
#72075=CARTESIAN_POINT('Ctrl Pts',(-23.1045468311994,-69.8026170510582,
12.));
#72076=CARTESIAN_POINT('Ctrl Pts',(-23.1067271468614,-69.7761378035979,
12.));
#72077=CARTESIAN_POINT('Ctrl Pts',(-23.1088799803094,-69.7496934674083,
12.));
#72078=CARTESIAN_POINT('Ctrl Pts',(-23.111005373205,-69.7232841398207,12.));
#72079=CARTESIAN_POINT('Ctrl Pts',(-23.1131033674301,-69.6969099184766,
12.));
#72080=CARTESIAN_POINT('Ctrl Pts',(-23.1151740050679,-69.6705709012842,
12.));
#72081=CARTESIAN_POINT('Ctrl Pts',(-23.1172173283856,-69.6442671863751,
12.));
#72082=CARTESIAN_POINT('Ctrl Pts',(-23.1192333798438,-69.617998872135,12.));
#72083=CARTESIAN_POINT('Ctrl Pts',(-23.1212222021049,-69.5917660572255,
12.));
#72084=CARTESIAN_POINT('Ctrl Pts',(-23.1231838380452,-69.565568840605,12.));
#72085=CARTESIAN_POINT('Ctrl Pts',(-23.1251183307678,-69.5394073215467,
12.));
#72086=CARTESIAN_POINT('Ctrl Pts',(-23.1270257236207,-69.5132815996548,
12.));
#72087=CARTESIAN_POINT('Ctrl Pts',(-23.1289060601927,-69.4871917748665,
12.));
#72088=CARTESIAN_POINT('Ctrl Pts',(-23.1307593843063,-69.4611379474492,
12.));
#72089=CARTESIAN_POINT('Ctrl Pts',(-23.1325857400145,-69.4351202179948,
12.));
#72090=CARTESIAN_POINT('Ctrl Pts',(-23.1343851715989,-69.4091386874129,
12.));
#72091=CARTESIAN_POINT('Ctrl Pts',(-23.1361577235708,-69.3831934569176,
12.));
#72092=CARTESIAN_POINT('Ctrl Pts',(-23.1379034406718,-69.3572846280289,
12.));
#72093=CARTESIAN_POINT('Ctrl Pts',(-23.1396223678725,-69.3314123025863,
12.));
#72094=CARTESIAN_POINT('Ctrl Pts',(-23.1413145503762,-69.3055765827544,
12.));
#72095=CARTESIAN_POINT('Ctrl Pts',(-23.1429800336221,-69.2797775710275,
12.));
#72096=CARTESIAN_POINT('Ctrl Pts',(-23.1446188632931,-69.2540153702311,
12.));
#72097=CARTESIAN_POINT('Ctrl Pts',(-23.1462310853205,-69.2282900835234,
12.));
#72098=CARTESIAN_POINT('Ctrl Pts',(-23.1478167458787,-69.2026018144023,
12.));
#72099=CARTESIAN_POINT('Ctrl Pts',(-23.1493758913857,-69.176950666708,12.));
#72100=CARTESIAN_POINT('Ctrl Pts',(-23.1509085685033,-69.1513367446231,
12.));
#72101=CARTESIAN_POINT('Ctrl Pts',(-23.1524148241413,-69.1257601526692,
12.));
#72102=CARTESIAN_POINT('Ctrl Pts',(-23.153894705462,-69.1002209957036,12.));
#72103=CARTESIAN_POINT('Ctrl Pts',(-23.1553482598768,-69.0747193789291,
12.));
#72104=CARTESIAN_POINT('Ctrl Pts',(-23.1567755350472,-69.0492554078999,
12.));
#72105=CARTESIAN_POINT('Ctrl Pts',(-23.1581765788869,-69.0238291885245,
12.));
#72106=CARTESIAN_POINT('Ctrl Pts',(-23.1595514395655,-68.9984408270652,
12.));
#72107=CARTESIAN_POINT('Ctrl Pts',(-23.1609001655154,-68.9730904301362,
12.));
#72108=CARTESIAN_POINT('Ctrl Pts',(-23.162222805429,-68.9477781047103,12.));
#72109=CARTESIAN_POINT('Ctrl Pts',(-23.1635194082582,-68.9225039581249,
12.));
#72110=CARTESIAN_POINT('Ctrl Pts',(-23.1647900232152,-68.8972680980844,
12.));
#72111=CARTESIAN_POINT('Ctrl Pts',(-23.1660346997763,-68.8720706326606,
12.));
#72112=CARTESIAN_POINT('Ctrl Pts',(-23.1672534876885,-68.8469116702885,
12.));
#72113=CARTESIAN_POINT('Ctrl Pts',(-23.1684464369681,-68.8217913197735,
12.));
#72114=CARTESIAN_POINT('Ctrl Pts',(-23.1696135978993,-68.7967096902981,
12.));
#72115=CARTESIAN_POINT('Ctrl Pts',(-23.1707550210359,-68.7716668914246,
12.));
#72116=CARTESIAN_POINT('Ctrl Pts',(-23.1718707572047,-68.7466630330968,
12.));
#72117=CARTESIAN_POINT('Ctrl Pts',(-23.1729608575115,-68.7216982256357,
12.));
#72118=CARTESIAN_POINT('Ctrl Pts',(-23.1740253733423,-68.6967725797457,
12.));
#72119=CARTESIAN_POINT('Ctrl Pts',(-23.1750643563606,-68.6718862065227,
12.));
#72120=CARTESIAN_POINT('Ctrl Pts',(-23.1760778585094,-68.6470392174567,
12.));
#72121=CARTESIAN_POINT('Ctrl Pts',(-23.1770659320137,-68.6222317244336,
12.));
#72122=CARTESIAN_POINT('Ctrl Pts',(-23.1780286293873,-68.5974638397322,
12.));
#72123=CARTESIAN_POINT('Ctrl Pts',(-23.178966003434,-68.572735676027,12.));
#72124=CARTESIAN_POINT('Ctrl Pts',(-23.1798781072449,-68.548047346398,12.));
#72125=CARTESIAN_POINT('Ctrl Pts',(-23.1807649942011,-68.5233989643344,
12.));
#72126=CARTESIAN_POINT('Ctrl Pts',(-23.1816267179752,-68.4987906437357,
12.));
#72127=CARTESIAN_POINT('Ctrl Pts',(-23.1824633325385,-68.4742224989099,
12.));
#72128=CARTESIAN_POINT('Ctrl Pts',(-23.1832748921629,-68.4496946445756,
12.));
#72129=CARTESIAN_POINT('Ctrl Pts',(-23.1840614514191,-68.4252071958725,
12.));
#72130=CARTESIAN_POINT('Ctrl Pts',(-23.1848230651776,-68.4007602683649,
12.));
#72131=CARTESIAN_POINT('Ctrl Pts',(-23.1855597886117,-68.3763539780442,
12.));
#72132=CARTESIAN_POINT('Ctrl Pts',(-23.1862716772034,-68.3519884413253,
12.));
#72133=CARTESIAN_POINT('Ctrl Pts',(-23.1869587867463,-68.3276637750494,
12.));
#72134=CARTESIAN_POINT('Ctrl Pts',(-23.1876211733439,-68.3033800964946,
12.));
#72135=CARTESIAN_POINT('Ctrl Pts',(-23.1882588934108,-68.2791375233798,
12.));
#72136=CARTESIAN_POINT('Ctrl Pts',(-23.1888720036757,-68.2549361738679,
12.));
#72137=CARTESIAN_POINT('Ctrl Pts',(-23.189460561187,-68.2307761665629,12.));
#72138=CARTESIAN_POINT('Ctrl Pts',(-23.1900246233165,-68.2066576205113,
12.));
#72139=CARTESIAN_POINT('Ctrl Pts',(-23.1905642477572,-68.182580655213,12.));
#72140=CARTESIAN_POINT('Ctrl Pts',(-23.1910794925252,-68.1585453906259,
12.));
#72141=CARTESIAN_POINT('Ctrl Pts',(-23.1915704159624,-68.1345519471695,
12.));
#72142=CARTESIAN_POINT('Ctrl Pts',(-23.1920370767424,-68.1106004457223,
12.));
#72143=CARTESIAN_POINT('Ctrl Pts',(-23.1924795338746,-68.086691007624,12.));
#72144=CARTESIAN_POINT('Ctrl Pts',(-23.1928978467018,-68.0628237546852,
12.));
#72145=CARTESIAN_POINT('Ctrl Pts',(-23.1932920749021,-68.0389988091926,
12.));
#72146=CARTESIAN_POINT('Ctrl Pts',(-23.193662278492,-68.0152162939123,12.));
#72147=CARTESIAN_POINT('Ctrl Pts',(-23.194008517832,-67.9914763320878,12.));
#72148=CARTESIAN_POINT('Ctrl Pts',(-23.1943308536307,-67.9677790474414,
12.));
#72149=CARTESIAN_POINT('Ctrl Pts',(-23.1946293469437,-67.944124564187,12.));
#72150=CARTESIAN_POINT('Ctrl Pts',(-23.1949040591748,-67.9205130070337,
12.));
#72151=CARTESIAN_POINT('Ctrl Pts',(-23.19515505208,-67.8969445011908,12.));
#72152=CARTESIAN_POINT('Ctrl Pts',(-23.1953823877727,-67.8734191723639,
12.));
#72153=CARTESIAN_POINT('Ctrl Pts',(-23.1955861287276,-67.8499371467578,
12.));
#72154=CARTESIAN_POINT('Ctrl Pts',(-23.1957663377798,-67.8264985510884,
12.));
#72155=CARTESIAN_POINT('Ctrl Pts',(-23.1959230781265,-67.8031035125873,
12.));
#72156=CARTESIAN_POINT('Ctrl Pts',(-23.1960564133308,-67.7797521590056,
12.));
#72157=CARTESIAN_POINT('Ctrl Pts',(-23.1961664073274,-67.7564446186115,
12.));
#72158=CARTESIAN_POINT('Ctrl Pts',(-23.1962531244261,-67.7331810201931,
12.));
#72159=CARTESIAN_POINT('Ctrl Pts',(-23.1963166293116,-67.7099614930712,
12.));
#72160=CARTESIAN_POINT('Ctrl Pts',(-23.1963569870457,-67.6867861671044,
12.));
#72161=CARTESIAN_POINT('Ctrl Pts',(-23.196374263071,-67.6636551726948,12.));
#72162=CARTESIAN_POINT('Ctrl Pts',(-23.1963685232176,-67.6405686407828,
12.));
#72163=CARTESIAN_POINT('Ctrl Pts',(-23.1963398337056,-67.6175267028516,
12.));
#72164=CARTESIAN_POINT('Ctrl Pts',(-23.1962882611444,-67.5945294909398,
12.));
#72165=CARTESIAN_POINT('Ctrl Pts',(-23.1962138725358,-67.5715771376454,
12.));
#72166=CARTESIAN_POINT('Ctrl Pts',(-23.1961167352777,-67.5486697761301,
12.));
#72167=CARTESIAN_POINT('Ctrl Pts',(-23.195996917171,-67.525807540117,12.));
#72168=CARTESIAN_POINT('Ctrl Pts',(-23.1958544864224,-67.5029905638973,
12.));
#72169=CARTESIAN_POINT('Ctrl Pts',(-23.1956895116446,-67.4802189823423,
12.));
#72170=CARTESIAN_POINT('Ctrl Pts',(-23.1955020618591,-67.4574929309078,
12.));
#72171=CARTESIAN_POINT('Ctrl Pts',(-23.1952922065009,-67.4348125456389,
12.));
#72172=CARTESIAN_POINT('Ctrl Pts',(-23.195060015426,-67.4121779631666,12.));
#72173=CARTESIAN_POINT('Ctrl Pts',(-23.1948055589123,-67.3895893207168,
12.));
#72174=CARTESIAN_POINT('Ctrl Pts',(-23.1945289076608,-67.3670467561205,
12.));
#72175=CARTESIAN_POINT('Ctrl Pts',(-23.1942301327979,-67.3445504078178,
12.));
#72176=CARTESIAN_POINT('Ctrl Pts',(-23.1939093058802,-67.3221004148604,
12.));
#72177=CARTESIAN_POINT('Ctrl Pts',(-23.193566498902,-67.2996969169099,12.));
#72178=CARTESIAN_POINT('Ctrl Pts',(-23.1932017842954,-67.2773400542477,
12.));
#72179=CARTESIAN_POINT('Ctrl Pts',(-23.1928152349344,-67.2550299677888,
12.));
#72180=CARTESIAN_POINT('Ctrl Pts',(-23.1924069241386,-67.232766799088,12.));
#72181=CARTESIAN_POINT('Ctrl Pts',(-23.1919769256803,-67.2105506903448,
12.));
#72182=CARTESIAN_POINT('Ctrl Pts',(-23.1915253137924,-67.1883817844039,
12.));
#72183=CARTESIAN_POINT('Ctrl Pts',(-23.1910521631658,-67.1662602247641,
12.));
#72184=CARTESIAN_POINT('Ctrl Pts',(-23.1905575489506,-67.1441861555819,
12.));
#72185=CARTESIAN_POINT('Ctrl Pts',(-23.1900415467575,-67.122159721674,12.));
#72186=CARTESIAN_POINT('Ctrl Pts',(-23.1895042326626,-67.1001810685138,
12.));
#72187=CARTESIAN_POINT('Ctrl Pts',(-23.1889456832116,-67.0782503422293,
12.));
#72188=CARTESIAN_POINT('Ctrl Pts',(-23.1883659754268,-67.0563676896312,
12.));
#72189=CARTESIAN_POINT('Ctrl Pts',(-23.1877651868155,-67.0345332582297,
12.));
#72190=CARTESIAN_POINT('Ctrl Pts',(-23.1871433953795,-67.0127471962507,
12.));
#72191=CARTESIAN_POINT('Ctrl Pts',(-23.1865006796291,-66.9910096526483,
12.));
#72192=CARTESIAN_POINT('Ctrl Pts',(-23.1858371185852,-66.9693207771058,
12.));
#72193=CARTESIAN_POINT('Ctrl Pts',(-23.1851527917666,-66.9476807200225,
12.));
#72194=CARTESIAN_POINT('Ctrl Pts',(-23.1844477791816,-66.9260896324955,
12.));
#72195=CARTESIAN_POINT('Ctrl Pts',(-23.1837221613231,-66.904547666305,12.));
#72196=CARTESIAN_POINT('Ctrl Pts',(-23.1829760191583,-66.8830549738768,
12.));
#72197=CARTESIAN_POINT('Ctrl Pts',(-23.1822094341508,-66.8616117083304,
12.));
#72198=CARTESIAN_POINT('Ctrl Pts',(-23.1814224882948,-66.8402180235549,
12.));
#72199=CARTESIAN_POINT('Ctrl Pts',(-23.1806152641475,-66.8188740742727,
12.));
#72200=CARTESIAN_POINT('Ctrl Pts',(-23.1797878448645,-66.7975800161014,
12.));
#72201=CARTESIAN_POINT('Ctrl Pts',(-23.1789403142376,-66.7763360056146,
12.));
#72202=CARTESIAN_POINT('Ctrl Pts',(-23.1780727566309,-66.7551422002229,
12.));
#72203=CARTESIAN_POINT('Ctrl Pts',(-23.1771852569137,-66.7339987580441,
12.));
#72204=CARTESIAN_POINT('Ctrl Pts',(-23.1762779004043,-66.712905837789,12.));
#72205=CARTESIAN_POINT('Ctrl Pts',(-23.1753507727932,-66.691863598595,12.));
#72206=CARTESIAN_POINT('Ctrl Pts',(-23.174403960137,-66.6708722000046,12.));
#72207=CARTESIAN_POINT('Ctrl Pts',(-23.1734375490421,-66.6499318023445,
12.));
#72208=CARTESIAN_POINT('Ctrl Pts',(-23.1724516268299,-66.6290425670538,
12.));
#72209=CARTESIAN_POINT('Ctrl Pts',(-23.1714462816794,-66.6082046569657,
12.));
#72210=CARTESIAN_POINT('Ctrl Pts',(-23.1704216028626,-66.5874182367596,
12.));
#72211=CARTESIAN_POINT('Ctrl Pts',(-23.169377680588,-66.5666834726494,12.));
#72212=CARTESIAN_POINT('Ctrl Pts',(-23.1683146055736,-66.5460005315406,
12.));
#72213=CARTESIAN_POINT('Ctrl Pts',(-23.1672324686928,-66.5253695803209,
12.));
#72214=CARTESIAN_POINT('Ctrl Pts',(-23.1661313606123,-66.5047907851319,
12.));
#72215=CARTESIAN_POINT('Ctrl Pts',(-23.1650113713792,-66.4842643105263,
12.));
#72216=CARTESIAN_POINT('Ctrl Pts',(-23.163872591218,-66.4637903210682,12.));
#72217=CARTESIAN_POINT('Ctrl Pts',(-23.1627151114875,-66.4433689832454,
12.));
#72218=CARTESIAN_POINT('Ctrl Pts',(-23.1615390254635,-66.4230004670288,
12.));
#72219=CARTESIAN_POINT('Ctrl Pts',(-23.1603444294754,-66.402684948127,12.));
#72220=CARTESIAN_POINT('Ctrl Pts',(-23.1591314230101,-66.382422608185,12.));
#72221=CARTESIAN_POINT('Ctrl Pts',(-23.1579001063438,-66.3622136300692,
12.));
#72222=CARTESIAN_POINT('Ctrl Pts',(-23.1566505784626,-66.3420581937159,
12.));
#72223=CARTESIAN_POINT('Ctrl Pts',(-23.1553829352531,-66.3219564725161,
12.));
#72224=CARTESIAN_POINT('Ctrl Pts',(-23.154097266617,-66.301908627539,12.));
#72225=CARTESIAN_POINT('Ctrl Pts',(-23.1527936592625,-66.2819148131072,
12.));
#72226=CARTESIAN_POINT('Ctrl Pts',(-23.1514722022483,-66.2619751878741,
12.));
#72227=CARTESIAN_POINT('Ctrl Pts',(-23.1501329914488,-66.2420899237317,
12.));
#72228=CARTESIAN_POINT('Ctrl Pts',(-23.1487761349328,-66.2222592165473,
12.));
#72229=CARTESIAN_POINT('Ctrl Pts',(-23.1474017566484,-66.2024832934866,
12.));
#72230=CARTESIAN_POINT('Ctrl Pts',(-23.1460099850763,-66.18276239029,12.));
#72231=CARTESIAN_POINT('Ctrl Pts',(-23.1446009424903,-66.1630967296747,
12.));
#72232=CARTESIAN_POINT('Ctrl Pts',(-23.1431747350098,-66.1434865015027,
12.));
#72233=CARTESIAN_POINT('Ctrl Pts',(-23.1417314398398,-66.1239318368548,
12.));
#72234=CARTESIAN_POINT('Ctrl Pts',(-23.1402711039425,-66.1044328067355,
12.));
#72235=CARTESIAN_POINT('Ctrl Pts',(-23.1390892229779,-66.088878115242,12.));
#72236=CARTESIAN_POINT('Ctrl Pts',(-23.13819515974,-66.0772371487248,12.));
#72237=CARTESIAN_POINT('Ctrl Pts',(-23.1375957166104,-66.0694876382127,
12.));
#72238=CARTESIAN_POINT('Ctrl Pts',(-23.1372951448024,-66.0656156664138,
12.));
#72239=CARTESIAN_POINT('Ctrl Pts',(-21.5904919935066,-70.993479606912,-5.55111512312578E-16));
#72240=CARTESIAN_POINT('Ctrl Pts',(-21.5904919935066,-70.993479606912,4.));
#72241=CARTESIAN_POINT('Ctrl Pts',(-21.5904919935066,-70.993479606912,8.));
#72242=CARTESIAN_POINT('Ctrl Pts',(-21.5904919935066,-70.993479606912,12.));
#72243=CARTESIAN_POINT('Ctrl Pts',(-21.6628164325805,-71.0762040404459,
-5.55111512312578E-16));
#72244=CARTESIAN_POINT('Ctrl Pts',(-21.6628164325805,-71.0762040404459,
4.));
#72245=CARTESIAN_POINT('Ctrl Pts',(-21.6628164325805,-71.076204040446,8.));
#72246=CARTESIAN_POINT('Ctrl Pts',(-21.6628164325805,-71.076204040446,12.));
#72247=CARTESIAN_POINT('Ctrl Pts',(-21.8385342042359,-71.1771795679079,
-5.55111512312578E-16));
#72248=CARTESIAN_POINT('Ctrl Pts',(-21.8385342042359,-71.1771795679079,
4.00000000000001));
#72249=CARTESIAN_POINT('Ctrl Pts',(-21.8385342042359,-71.177179567908,7.99999999999999));
#72250=CARTESIAN_POINT('Ctrl Pts',(-21.8385342042359,-71.177179567908,12.));
#72251=CARTESIAN_POINT('Ctrl Pts',(-22.0366423876806,-71.1663065220503,
-5.55111512312578E-16));
#72252=CARTESIAN_POINT('Ctrl Pts',(-22.0366423876806,-71.1663065220503,
3.99999999999999));
#72253=CARTESIAN_POINT('Ctrl Pts',(-22.0366423876807,-71.1663065220504,
8.00000000000001));
#72254=CARTESIAN_POINT('Ctrl Pts',(-22.0366423876807,-71.1663065220504,
12.));
#72255=CARTESIAN_POINT('Ctrl Pts',(-22.1153394458686,-71.1418425484889,
-5.55111512312578E-16));
#72256=CARTESIAN_POINT('Ctrl Pts',(-22.1153394458686,-71.1418425484889,
4.));
#72257=CARTESIAN_POINT('Ctrl Pts',(-22.1153394458687,-71.141842548489,8.));
#72258=CARTESIAN_POINT('Ctrl Pts',(-22.1153394458687,-71.141842548489,12.));
#72259=CARTESIAN_POINT('',(-21.5904919935066,-70.993479606912,-2.77555756156289E-16));
#72260=CARTESIAN_POINT('',(-22.1153394458687,-71.1418425484891,2.77555756156289E-16));
#72261=CARTESIAN_POINT('Ctrl Pts',(-21.5904919935066,-70.993479606912,0.));
#72262=CARTESIAN_POINT('Ctrl Pts',(-21.6628164325805,-71.0762040404459,
-6.93334779979405E-31));
#72263=CARTESIAN_POINT('Ctrl Pts',(-21.7632265878122,-71.1339043418528,
5.23852944873328E-31));
#72264=CARTESIAN_POINT('Ctrl Pts',(-21.8709478979138,-71.1550826601349,
1.54074395550979E-31));
#72265=CARTESIAN_POINT('Ctrl Pts',(-21.95173888049,-71.1709663988464,9.24446373305873E-32));
#72266=CARTESIAN_POINT('Ctrl Pts',(-22.0366423876806,-71.1663065220503,
-8.32001735975286E-31));
#72267=CARTESIAN_POINT('Ctrl Pts',(-22.1153394458686,-71.1418425484889,
1.69481835106077E-31));
#72268=CARTESIAN_POINT('',(-22.1153394458687,-71.1418425484891,12.));
#72269=CARTESIAN_POINT('Ctrl Pts',(-22.1153394458686,-71.1418425484889,
-5.55111512312578E-16));
#72270=CARTESIAN_POINT('Ctrl Pts',(-22.1153394458686,-71.1418425484889,
4.));
#72271=CARTESIAN_POINT('Ctrl Pts',(-22.1153394458687,-71.141842548489,8.));
#72272=CARTESIAN_POINT('Ctrl Pts',(-22.1153394458687,-71.141842548489,12.));
#72273=CARTESIAN_POINT('',(-21.5904919935066,-70.993479606912,12.));
#72274=CARTESIAN_POINT('Ctrl Pts',(-22.1153394458687,-71.141842548489,12.));
#72275=CARTESIAN_POINT('Ctrl Pts',(-22.0366423876807,-71.1663065220504,
12.));
#72276=CARTESIAN_POINT('Ctrl Pts',(-21.9517388804901,-71.1709663988466,
12.));
#72277=CARTESIAN_POINT('Ctrl Pts',(-21.8709478979138,-71.155082660135,12.));
#72278=CARTESIAN_POINT('Ctrl Pts',(-21.7632265878122,-71.1339043418528,
12.));
#72279=CARTESIAN_POINT('Ctrl Pts',(-21.6628164325805,-71.076204040446,12.));
#72280=CARTESIAN_POINT('Ctrl Pts',(-21.5904919935066,-70.993479606912,12.));
#72281=CARTESIAN_POINT('Ctrl Pts',(-21.5904919935066,-70.993479606912,12.));
#72282=CARTESIAN_POINT('Ctrl Pts',(-21.5904919935066,-70.993479606912,8.));
#72283=CARTESIAN_POINT('Ctrl Pts',(-21.5904919935066,-70.993479606912,4.));
#72284=CARTESIAN_POINT('Ctrl Pts',(-21.5904919935066,-70.993479606912,-5.55111512312578E-16));
#72285=CARTESIAN_POINT('Origin',(-1.12623029467293E-10,-3.57524700084383E-10,
0.));
#72286=CARTESIAN_POINT('Origin',(-1.12623029467293E-10,-3.57524700084383E-10,
12.));
#72287=CARTESIAN_POINT('Origin',(-1.12623029467293E-10,-3.57524700084383E-10,
0.));
#72288=CARTESIAN_POINT('Ctrl Pts',(-28.7877620302392,-68.7132793373328,
0.));
#72289=CARTESIAN_POINT('Ctrl Pts',(-28.7877620302392,-68.7132793373328,
4.));
#72290=CARTESIAN_POINT('Ctrl Pts',(-28.7877620302391,-68.7132793373328,
8.));
#72291=CARTESIAN_POINT('Ctrl Pts',(-28.7877620302391,-68.7132793373328,
12.));
#72292=CARTESIAN_POINT('Ctrl Pts',(-28.8891094745187,-68.6708193334379,
0.));
#72293=CARTESIAN_POINT('Ctrl Pts',(-28.8891094745187,-68.6708193334379,
4.));
#72294=CARTESIAN_POINT('Ctrl Pts',(-28.8891094745187,-68.6708193334379,
8.));
#72295=CARTESIAN_POINT('Ctrl Pts',(-28.8891094745187,-68.6708193334379,
12.));
#72296=CARTESIAN_POINT('Ctrl Pts',(-29.0404604348958,-68.5360395709811,
0.));
#72297=CARTESIAN_POINT('Ctrl Pts',(-29.0404604348958,-68.5360395709811,
4.));
#72298=CARTESIAN_POINT('Ctrl Pts',(-29.0404604348958,-68.5360395709811,
8.));
#72299=CARTESIAN_POINT('Ctrl Pts',(-29.0404604348958,-68.5360395709811,
12.));
#72300=CARTESIAN_POINT('Ctrl Pts',(-29.092780523712,-68.3446561754307,0.));
#72301=CARTESIAN_POINT('Ctrl Pts',(-29.092780523712,-68.3446561754307,4.));
#72302=CARTESIAN_POINT('Ctrl Pts',(-29.0927805237119,-68.3446561754307,
8.));
#72303=CARTESIAN_POINT('Ctrl Pts',(-29.0927805237119,-68.3446561754307,
12.));
#72304=CARTESIAN_POINT('Ctrl Pts',(-29.094452644025,-68.2622612909743,0.));
#72305=CARTESIAN_POINT('Ctrl Pts',(-29.094452644025,-68.2622612909743,4.));
#72306=CARTESIAN_POINT('Ctrl Pts',(-29.0944526440249,-68.2622612909743,
8.));
#72307=CARTESIAN_POINT('Ctrl Pts',(-29.0944526440249,-68.2622612909743,
12.));
#72308=CARTESIAN_POINT('',(-28.7877620302392,-68.7132793373328,0.));
#72309=CARTESIAN_POINT('',(-29.0944526440249,-68.2622612909743,2.77555756156289E-16));
#72310=CARTESIAN_POINT('Ctrl Pts',(-28.7877620302392,-68.7132793373328,
2.08166817117217E-16));
#72311=CARTESIAN_POINT('Ctrl Pts',(-28.8891094745187,-68.6708193334379,
2.08166817117217E-16));
#72312=CARTESIAN_POINT('Ctrl Pts',(-28.9755957375913,-68.5938023263197,
2.08166817117217E-16));
#72313=CARTESIAN_POINT('Ctrl Pts',(-29.029745389542,-68.4983025002322,2.08166817117217E-16));
#72314=CARTESIAN_POINT('Ctrl Pts',(-29.070357628505,-68.4266776306666,2.08166817117217E-16));
#72315=CARTESIAN_POINT('Ctrl Pts',(-29.092780523712,-68.3446561754307,2.08166817117217E-16));
#72316=CARTESIAN_POINT('Ctrl Pts',(-29.094452644025,-68.2622612909743,2.08166817117217E-16));
#72317=CARTESIAN_POINT('',(-29.0944526440249,-68.2622612909743,12.));
#72318=CARTESIAN_POINT('Ctrl Pts',(-29.094452644025,-68.2622612909743,0.));
#72319=CARTESIAN_POINT('Ctrl Pts',(-29.094452644025,-68.2622612909743,4.));
#72320=CARTESIAN_POINT('Ctrl Pts',(-29.0944526440249,-68.2622612909743,
8.));
#72321=CARTESIAN_POINT('Ctrl Pts',(-29.0944526440249,-68.2622612909743,
12.));
#72322=CARTESIAN_POINT('',(-28.7877620302391,-68.7132793373328,12.));
#72323=CARTESIAN_POINT('Ctrl Pts',(-29.0944526440249,-68.2622612909743,
12.));
#72324=CARTESIAN_POINT('Ctrl Pts',(-29.0927805237119,-68.3446561754307,
12.));
#72325=CARTESIAN_POINT('Ctrl Pts',(-29.070357628505,-68.4266776306666,12.));
#72326=CARTESIAN_POINT('Ctrl Pts',(-29.029745389542,-68.4983025002322,12.));
#72327=CARTESIAN_POINT('Ctrl Pts',(-28.9755957375913,-68.5938023263197,
12.));
#72328=CARTESIAN_POINT('Ctrl Pts',(-28.8891094745187,-68.6708193334379,
12.));
#72329=CARTESIAN_POINT('Ctrl Pts',(-28.7877620302391,-68.7132793373328,
12.));
#72330=CARTESIAN_POINT('Ctrl Pts',(-28.7877620302391,-68.7132793373328,
12.));
#72331=CARTESIAN_POINT('Ctrl Pts',(-28.7877620302391,-68.7132793373328,
8.));
#72332=CARTESIAN_POINT('Ctrl Pts',(-28.7877620302392,-68.7132793373328,
4.));
#72333=CARTESIAN_POINT('Ctrl Pts',(-28.7877620302392,-68.7132793373328,
0.));
#72334=CARTESIAN_POINT('Ctrl Pts',(-28.8072485549237,-63.7976679095314,
0.));
#72335=CARTESIAN_POINT('Ctrl Pts',(-28.8072485549237,-63.7976679095314,
12.));
#72336=CARTESIAN_POINT('Ctrl Pts',(-28.8078854475432,-63.8014989507494,
0.));
#72337=CARTESIAN_POINT('Ctrl Pts',(-28.8078854475432,-63.8014989507494,
12.));
#72338=CARTESIAN_POINT('Ctrl Pts',(-28.8091580239553,-63.8091667271231,
0.));
#72339=CARTESIAN_POINT('Ctrl Pts',(-28.8091580239553,-63.8091667271231,
12.));
#72340=CARTESIAN_POINT('Ctrl Pts',(-28.8110632620958,-63.8206854735027,
0.));
#72341=CARTESIAN_POINT('Ctrl Pts',(-28.8110632620958,-63.8206854735027,
12.));
#72342=CARTESIAN_POINT('Ctrl Pts',(-28.8135963263369,-63.8360779669856,
0.));
#72343=CARTESIAN_POINT('Ctrl Pts',(-28.8135963263369,-63.8360779669856,
12.));
#72344=CARTESIAN_POINT('Ctrl Pts',(-28.8167505576681,-63.8553755207486,
0.));
#72345=CARTESIAN_POINT('Ctrl Pts',(-28.8167505576681,-63.8553755207486,
12.));
#72346=CARTESIAN_POINT('Ctrl Pts',(-28.8198926619858,-63.8747299825313,
0.));
#72347=CARTESIAN_POINT('Ctrl Pts',(-28.8198926619858,-63.8747299825313,
12.));
#72348=CARTESIAN_POINT('Ctrl Pts',(-28.823022586318,-63.8941412856923,0.));
#72349=CARTESIAN_POINT('Ctrl Pts',(-28.823022586318,-63.8941412856923,12.));
#72350=CARTESIAN_POINT('Ctrl Pts',(-28.8261402423291,-63.9136093063786,
0.));
#72351=CARTESIAN_POINT('Ctrl Pts',(-28.8261402423291,-63.9136093063786,
12.));
#72352=CARTESIAN_POINT('Ctrl Pts',(-28.8292455077559,-63.9331338646996,
0.));
#72353=CARTESIAN_POINT('Ctrl Pts',(-28.8292455077559,-63.9331338646996,
12.));
#72354=CARTESIAN_POINT('Ctrl Pts',(-28.8323382413789,-63.9527147494423,
0.));
#72355=CARTESIAN_POINT('Ctrl Pts',(-28.8323382413789,-63.9527147494423,
12.));
#72356=CARTESIAN_POINT('Ctrl Pts',(-28.8354182946601,-63.9723517369614,
0.));
#72357=CARTESIAN_POINT('Ctrl Pts',(-28.8354182946601,-63.9723517369614,
12.));
#72358=CARTESIAN_POINT('Ctrl Pts',(-28.8384855243243,-63.9920446117582,
0.));
#72359=CARTESIAN_POINT('Ctrl Pts',(-28.8384855243243,-63.9920446117582,
12.));
#72360=CARTESIAN_POINT('Ctrl Pts',(-28.8415398056428,-64.0117931881298,
0.));
#72361=CARTESIAN_POINT('Ctrl Pts',(-28.8415398056428,-64.0117931881298,
12.));
#72362=CARTESIAN_POINT('Ctrl Pts',(-28.844581028125,-64.0315973031942,0.));
#72363=CARTESIAN_POINT('Ctrl Pts',(-28.844581028125,-64.0315973031942,12.));
#72364=CARTESIAN_POINT('Ctrl Pts',(-28.8476090892232,-64.0514568066637,
0.));
#72365=CARTESIAN_POINT('Ctrl Pts',(-28.8476090892232,-64.0514568066637,
12.));
#72366=CARTESIAN_POINT('Ctrl Pts',(-28.8506238891093,-64.0713715523599,
0.));
#72367=CARTESIAN_POINT('Ctrl Pts',(-28.8506238891093,-64.0713715523599,
12.));
#72368=CARTESIAN_POINT('Ctrl Pts',(-28.8536253241854,-64.0913413876622,
0.));
#72369=CARTESIAN_POINT('Ctrl Pts',(-28.8536253241854,-64.0913413876622,
12.));
#72370=CARTESIAN_POINT('Ctrl Pts',(-28.8566132838179,-64.1113661481965,
0.));
#72371=CARTESIAN_POINT('Ctrl Pts',(-28.8566132838179,-64.1113661481965,
12.));
#72372=CARTESIAN_POINT('Ctrl Pts',(-28.8595876537148,-64.1314456633381,
0.));
#72373=CARTESIAN_POINT('Ctrl Pts',(-28.8595876537148,-64.1314456633381,
12.));
#72374=CARTESIAN_POINT('Ctrl Pts',(-28.8625483180438,-64.1515797596564,
0.));
#72375=CARTESIAN_POINT('Ctrl Pts',(-28.8625483180438,-64.1515797596564,
12.));
#72376=CARTESIAN_POINT('Ctrl Pts',(-28.8654951618649,-64.1717682648685,
0.));
#72377=CARTESIAN_POINT('Ctrl Pts',(-28.8654951618649,-64.1717682648685,
12.));
#72378=CARTESIAN_POINT('Ctrl Pts',(-28.8684280739014,-64.1920110123299,
0.));
#72379=CARTESIAN_POINT('Ctrl Pts',(-28.8684280739014,-64.1920110123299,
12.));
#72380=CARTESIAN_POINT('Ctrl Pts',(-28.8713469464185,-64.2123078408461,
0.));
#72381=CARTESIAN_POINT('Ctrl Pts',(-28.8713469464185,-64.2123078408461,
12.));
#72382=CARTESIAN_POINT('Ctrl Pts',(-28.8742516738947,-64.2326585925252,
0.));
#72383=CARTESIAN_POINT('Ctrl Pts',(-28.8742516738947,-64.2326585925252,
12.));
#72384=CARTESIAN_POINT('Ctrl Pts',(-28.877142152106,-64.2530631112929,0.));
#72385=CARTESIAN_POINT('Ctrl Pts',(-28.877142152106,-64.2530631112929,12.));
#72386=CARTESIAN_POINT('Ctrl Pts',(-28.8800182770065,-64.273521241071,0.));
#72387=CARTESIAN_POINT('Ctrl Pts',(-28.8800182770065,-64.273521241071,12.));
#72388=CARTESIAN_POINT('Ctrl Pts',(-28.882879943794,-64.2940328242521,0.));
#72389=CARTESIAN_POINT('Ctrl Pts',(-28.882879943794,-64.2940328242521,12.));
#72390=CARTESIAN_POINT('Ctrl Pts',(-28.8857270473959,-64.3145977025037,
0.));
#72391=CARTESIAN_POINT('Ctrl Pts',(-28.8857270473959,-64.3145977025037,
12.));
#72392=CARTESIAN_POINT('Ctrl Pts',(-28.8885594828926,-64.3352157174619,
0.));
#72393=CARTESIAN_POINT('Ctrl Pts',(-28.8885594828926,-64.3352157174619,
12.));
#72394=CARTESIAN_POINT('Ctrl Pts',(-28.8913771459323,-64.3558867114076,
0.));
#72395=CARTESIAN_POINT('Ctrl Pts',(-28.8913771459323,-64.3558867114076,
12.));
#72396=CARTESIAN_POINT('Ctrl Pts',(-28.89417993323,-64.3766105280688,0.));
#72397=CARTESIAN_POINT('Ctrl Pts',(-28.89417993323,-64.3766105280688,12.));
#72398=CARTESIAN_POINT('Ctrl Pts',(-28.8969677427504,-64.3973870129169,
0.));
#72399=CARTESIAN_POINT('Ctrl Pts',(-28.8969677427504,-64.3973870129169,
12.));
#72400=CARTESIAN_POINT('Ctrl Pts',(-28.899740473434,-64.4182160127379,0.));
#72401=CARTESIAN_POINT('Ctrl Pts',(-28.899740473434,-64.4182160127379,12.));
#72402=CARTESIAN_POINT('Ctrl Pts',(-28.9024980250307,-64.4390973753634,
0.));
#72403=CARTESIAN_POINT('Ctrl Pts',(-28.9024980250307,-64.4390973753634,
12.));
#72404=CARTESIAN_POINT('Ctrl Pts',(-28.9052402979062,-64.4600309493583,
0.));
#72405=CARTESIAN_POINT('Ctrl Pts',(-28.9052402979062,-64.4600309493583,
12.));
#72406=CARTESIAN_POINT('Ctrl Pts',(-28.9079671928264,-64.4810165836592,
0.));
#72407=CARTESIAN_POINT('Ctrl Pts',(-28.9079671928264,-64.4810165836592,
12.));
#72408=CARTESIAN_POINT('Ctrl Pts',(-28.910678610965,-64.5020541275951,0.));
#72409=CARTESIAN_POINT('Ctrl Pts',(-28.910678610965,-64.5020541275951,12.));
#72410=CARTESIAN_POINT('Ctrl Pts',(-28.9133744539949,-64.523143431047,0.));
#72411=CARTESIAN_POINT('Ctrl Pts',(-28.9133744539949,-64.523143431047,12.));
#72412=CARTESIAN_POINT('Ctrl Pts',(-28.9160546241538,-64.5442843445559,
0.));
#72413=CARTESIAN_POINT('Ctrl Pts',(-28.9160546241538,-64.5442843445559,
12.));
#72414=CARTESIAN_POINT('Ctrl Pts',(-28.9187190243224,-64.5654767194471,
0.));
#72415=CARTESIAN_POINT('Ctrl Pts',(-28.9187190243224,-64.5654767194471,
12.));
#72416=CARTESIAN_POINT('Ctrl Pts',(-28.9213675580985,-64.5867204079426,
0.));
#72417=CARTESIAN_POINT('Ctrl Pts',(-28.9213675580985,-64.5867204079426,
12.));
#72418=CARTESIAN_POINT('Ctrl Pts',(-28.9240001297542,-64.6080152631039,
0.));
#72419=CARTESIAN_POINT('Ctrl Pts',(-28.9240001297542,-64.6080152631039,
12.));
#72420=CARTESIAN_POINT('Ctrl Pts',(-28.9266166441951,-64.629361138774,0.));
#72421=CARTESIAN_POINT('Ctrl Pts',(-28.9266166441951,-64.629361138774,12.));
#72422=CARTESIAN_POINT('Ctrl Pts',(-28.9292170069222,-64.6507578895161,
0.));
#72423=CARTESIAN_POINT('Ctrl Pts',(-28.9292170069222,-64.6507578895161,
12.));
#72424=CARTESIAN_POINT('Ctrl Pts',(-28.9318011239915,-64.672205370541,0.));
#72425=CARTESIAN_POINT('Ctrl Pts',(-28.9318011239915,-64.672205370541,12.));
#72426=CARTESIAN_POINT('Ctrl Pts',(-28.9343689019882,-64.6937034376617,
0.));
#72427=CARTESIAN_POINT('Ctrl Pts',(-28.9343689019882,-64.6937034376617,
12.));
#72428=CARTESIAN_POINT('Ctrl Pts',(-28.9369202480393,-64.715251947329,0.));
#72429=CARTESIAN_POINT('Ctrl Pts',(-28.9369202480393,-64.715251947329,12.));
#72430=CARTESIAN_POINT('Ctrl Pts',(-28.9394550698204,-64.7368507566467,
0.));
#72431=CARTESIAN_POINT('Ctrl Pts',(-28.9394550698204,-64.7368507566467,
12.));
#72432=CARTESIAN_POINT('Ctrl Pts',(-28.9419732755656,-64.758499723388,0.));
#72433=CARTESIAN_POINT('Ctrl Pts',(-28.9419732755656,-64.758499723388,12.));
#72434=CARTESIAN_POINT('Ctrl Pts',(-28.944474774081,-64.7801987060084,0.));
#72435=CARTESIAN_POINT('Ctrl Pts',(-28.944474774081,-64.7801987060084,12.));
#72436=CARTESIAN_POINT('Ctrl Pts',(-28.9469594747432,-64.8019475636442,
0.));
#72437=CARTESIAN_POINT('Ctrl Pts',(-28.9469594747432,-64.8019475636442,
12.));
#72438=CARTESIAN_POINT('Ctrl Pts',(-28.9494272874832,-64.8237461561018,
0.));
#72439=CARTESIAN_POINT('Ctrl Pts',(-28.9494272874832,-64.8237461561018,
12.));
#72440=CARTESIAN_POINT('Ctrl Pts',(-28.9518781227765,-64.8455943438423,
0.));
#72441=CARTESIAN_POINT('Ctrl Pts',(-28.9518781227765,-64.8455943438423,
12.));
#72442=CARTESIAN_POINT('Ctrl Pts',(-28.9543118916328,-64.8674919879648,
0.));
#72443=CARTESIAN_POINT('Ctrl Pts',(-28.9543118916328,-64.8674919879648,
12.));
#72444=CARTESIAN_POINT('Ctrl Pts',(-28.9567285055867,-64.8894389501801,
0.));
#72445=CARTESIAN_POINT('Ctrl Pts',(-28.9567285055867,-64.8894389501801,
12.));
#72446=CARTESIAN_POINT('Ctrl Pts',(-28.9591278766934,-64.9114350928125,
0.));
#72447=CARTESIAN_POINT('Ctrl Pts',(-28.9591278766934,-64.9114350928125,
12.));
#72448=CARTESIAN_POINT('Ctrl Pts',(-28.961509917525,-64.9334802788038,0.));
#72449=CARTESIAN_POINT('Ctrl Pts',(-28.961509917525,-64.9334802788038,12.));
#72450=CARTESIAN_POINT('Ctrl Pts',(-28.9638745411677,-64.9555743717109,
0.));
#72451=CARTESIAN_POINT('Ctrl Pts',(-28.9638745411677,-64.9555743717109,
12.));
#72452=CARTESIAN_POINT('Ctrl Pts',(-28.9662216612217,-64.9777172357027,
0.));
#72453=CARTESIAN_POINT('Ctrl Pts',(-28.9662216612217,-64.9777172357027,
12.));
#72454=CARTESIAN_POINT('Ctrl Pts',(-28.9685511918018,-64.9999087355504,
0.));
#72455=CARTESIAN_POINT('Ctrl Pts',(-28.9685511918018,-64.9999087355504,
12.));
#72456=CARTESIAN_POINT('Ctrl Pts',(-28.97086304753,-65.022148736628,0.));
#72457=CARTESIAN_POINT('Ctrl Pts',(-28.97086304753,-65.022148736628,12.));
#72458=CARTESIAN_POINT('Ctrl Pts',(-28.9731571435283,-65.0444371049082,
0.));
#72459=CARTESIAN_POINT('Ctrl Pts',(-28.9731571435283,-65.0444371049082,
12.));
#72460=CARTESIAN_POINT('Ctrl Pts',(-28.9754333954135,-65.0667737069563,
0.));
#72461=CARTESIAN_POINT('Ctrl Pts',(-28.9754333954135,-65.0667737069563,
12.));
#72462=CARTESIAN_POINT('Ctrl Pts',(-28.9776917192933,-65.0891584099168,
0.));
#72463=CARTESIAN_POINT('Ctrl Pts',(-28.9776917192933,-65.0891584099168,
12.));
#72464=CARTESIAN_POINT('Ctrl Pts',(-28.9799320317641,-65.1115910815037,
0.));
#72465=CARTESIAN_POINT('Ctrl Pts',(-28.9799320317641,-65.1115910815037,
12.));
#72466=CARTESIAN_POINT('Ctrl Pts',(-28.9821542499043,-65.1340715900028,
0.));
#72467=CARTESIAN_POINT('Ctrl Pts',(-28.9821542499043,-65.1340715900028,
12.));
#72468=CARTESIAN_POINT('Ctrl Pts',(-28.9843582912693,-65.1565998042697,
0.));
#72469=CARTESIAN_POINT('Ctrl Pts',(-28.9843582912693,-65.1565998042697,
12.));
#72470=CARTESIAN_POINT('Ctrl Pts',(-28.9865440738884,-65.1791755937256,
0.));
#72471=CARTESIAN_POINT('Ctrl Pts',(-28.9865440738884,-65.1791755937256,
12.));
#72472=CARTESIAN_POINT('Ctrl Pts',(-28.9887115162634,-65.2017988283479,
0.));
#72473=CARTESIAN_POINT('Ctrl Pts',(-28.9887115162634,-65.2017988283479,
12.));
#72474=CARTESIAN_POINT('Ctrl Pts',(-28.9908605373663,-65.2244693786609,
0.));
#72475=CARTESIAN_POINT('Ctrl Pts',(-28.9908605373663,-65.2244693786609,
12.));
#72476=CARTESIAN_POINT('Ctrl Pts',(-28.9929910566325,-65.2471871157397,
0.));
#72477=CARTESIAN_POINT('Ctrl Pts',(-28.9929910566325,-65.2471871157397,
12.));
#72478=CARTESIAN_POINT('Ctrl Pts',(-28.9951029939557,-65.2699519112064,
0.));
#72479=CARTESIAN_POINT('Ctrl Pts',(-28.9951029939557,-65.2699519112064,
12.));
#72480=CARTESIAN_POINT('Ctrl Pts',(-28.9971962696845,-65.2927636372253,
0.));
#72481=CARTESIAN_POINT('Ctrl Pts',(-28.9971962696845,-65.2927636372253,
12.));
#72482=CARTESIAN_POINT('Ctrl Pts',(-28.9992708046212,-65.3156221664916,
0.));
#72483=CARTESIAN_POINT('Ctrl Pts',(-28.9992708046212,-65.3156221664916,
12.));
#72484=CARTESIAN_POINT('Ctrl Pts',(-29.0013265200185,-65.3385273722241,
0.));
#72485=CARTESIAN_POINT('Ctrl Pts',(-29.0013265200185,-65.3385273722241,
12.));
#72486=CARTESIAN_POINT('Ctrl Pts',(-29.003363337573,-65.3614791281692,0.));
#72487=CARTESIAN_POINT('Ctrl Pts',(-29.003363337573,-65.3614791281692,12.));
#72488=CARTESIAN_POINT('Ctrl Pts',(-29.0053811794207,-65.3844773085961,
0.));
#72489=CARTESIAN_POINT('Ctrl Pts',(-29.0053811794207,-65.3844773085961,
12.));
#72490=CARTESIAN_POINT('Ctrl Pts',(-29.0073799681342,-65.4075217882934,
0.));
#72491=CARTESIAN_POINT('Ctrl Pts',(-29.0073799681342,-65.4075217882934,
12.));
#72492=CARTESIAN_POINT('Ctrl Pts',(-29.0093596267216,-65.4306124425562,
0.));
#72493=CARTESIAN_POINT('Ctrl Pts',(-29.0093596267216,-65.4306124425562,
12.));
#72494=CARTESIAN_POINT('Ctrl Pts',(-29.0113200786239,-65.4537491471828,
0.));
#72495=CARTESIAN_POINT('Ctrl Pts',(-29.0113200786239,-65.4537491471828,
12.));
#72496=CARTESIAN_POINT('Ctrl Pts',(-29.013261247709,-65.4769317784789,0.));
#72497=CARTESIAN_POINT('Ctrl Pts',(-29.013261247709,-65.4769317784789,12.));
#72498=CARTESIAN_POINT('Ctrl Pts',(-29.0151830582675,-65.5001602132535,
0.));
#72499=CARTESIAN_POINT('Ctrl Pts',(-29.0151830582675,-65.5001602132535,
12.));
#72500=CARTESIAN_POINT('Ctrl Pts',(-29.0170854350095,-65.5234343288136,
0.));
#72501=CARTESIAN_POINT('Ctrl Pts',(-29.0170854350095,-65.5234343288136,
12.));
#72502=CARTESIAN_POINT('Ctrl Pts',(-29.0189683030642,-65.5467540029514,
0.));
#72503=CARTESIAN_POINT('Ctrl Pts',(-29.0189683030642,-65.5467540029514,
12.));
#72504=CARTESIAN_POINT('Ctrl Pts',(-29.0208315879764,-65.5701191139418,
0.));
#72505=CARTESIAN_POINT('Ctrl Pts',(-29.0208315879764,-65.5701191139418,
12.));
#72506=CARTESIAN_POINT('Ctrl Pts',(-29.0226752157003,-65.5935295405453,
0.));
#72507=CARTESIAN_POINT('Ctrl Pts',(-29.0226752157003,-65.5935295405453,
12.));
#72508=CARTESIAN_POINT('Ctrl Pts',(-29.0244991125959,-65.6169851620046,
0.));
#72509=CARTESIAN_POINT('Ctrl Pts',(-29.0244991125959,-65.6169851620046,
12.));
#72510=CARTESIAN_POINT('Ctrl Pts',(-29.0263032054266,-65.6404858580403,
0.));
#72511=CARTESIAN_POINT('Ctrl Pts',(-29.0263032054266,-65.6404858580403,
12.));
#72512=CARTESIAN_POINT('Ctrl Pts',(-29.0280874213596,-65.6640315088388,
0.));
#72513=CARTESIAN_POINT('Ctrl Pts',(-29.0280874213596,-65.6640315088388,
12.));
#72514=CARTESIAN_POINT('Ctrl Pts',(-29.0298516879612,-65.6876219950493,
0.));
#72515=CARTESIAN_POINT('Ctrl Pts',(-29.0298516879612,-65.6876219950493,
12.));
#72516=CARTESIAN_POINT('Ctrl Pts',(-29.0315959331919,-65.7112571977891,
0.));
#72517=CARTESIAN_POINT('Ctrl Pts',(-29.0315959331919,-65.7112571977891,
12.));
#72518=CARTESIAN_POINT('Ctrl Pts',(-29.0333200854028,-65.7349369986384,
0.));
#72519=CARTESIAN_POINT('Ctrl Pts',(-29.0333200854028,-65.7349369986384,
12.));
#72520=CARTESIAN_POINT('Ctrl Pts',(-29.035024073333,-65.7586612796368,0.));
#72521=CARTESIAN_POINT('Ctrl Pts',(-29.035024073333,-65.7586612796368,12.));
#72522=CARTESIAN_POINT('Ctrl Pts',(-29.0367078261103,-65.7824299232705,
0.));
#72523=CARTESIAN_POINT('Ctrl Pts',(-29.0367078261103,-65.7824299232705,
12.));
#72524=CARTESIAN_POINT('Ctrl Pts',(-29.0383712732469,-65.8062428124713,
0.));
#72525=CARTESIAN_POINT('Ctrl Pts',(-29.0383712732469,-65.8062428124713,
12.));
#72526=CARTESIAN_POINT('Ctrl Pts',(-29.0400143446338,-65.8300998306191,
0.));
#72527=CARTESIAN_POINT('Ctrl Pts',(-29.0400143446338,-65.8300998306191,
12.));
#72528=CARTESIAN_POINT('Ctrl Pts',(-29.0416369705375,-65.854000861539,0.));
#72529=CARTESIAN_POINT('Ctrl Pts',(-29.0416369705375,-65.854000861539,12.));
#72530=CARTESIAN_POINT('Ctrl Pts',(-29.0432390815978,-65.8779457894961,
0.));
#72531=CARTESIAN_POINT('Ctrl Pts',(-29.0432390815978,-65.8779457894961,
12.));
#72532=CARTESIAN_POINT('Ctrl Pts',(-29.0448206088289,-65.9019344991854,
0.));
#72533=CARTESIAN_POINT('Ctrl Pts',(-29.0448206088289,-65.9019344991854,
12.));
#72534=CARTESIAN_POINT('Ctrl Pts',(-29.0463814836157,-65.9259668757306,
0.));
#72535=CARTESIAN_POINT('Ctrl Pts',(-29.0463814836157,-65.9259668757306,
12.));
#72536=CARTESIAN_POINT('Ctrl Pts',(-29.0479216377081,-65.9500428046868,
0.));
#72537=CARTESIAN_POINT('Ctrl Pts',(-29.0479216377081,-65.9500428046868,
12.));
#72538=CARTESIAN_POINT('Ctrl Pts',(-29.0494410032173,-65.9741621720369,
0.));
#72539=CARTESIAN_POINT('Ctrl Pts',(-29.0494410032173,-65.9741621720369,
12.));
#72540=CARTESIAN_POINT('Ctrl Pts',(-29.0509395126143,-65.9983248641879,
0.));
#72541=CARTESIAN_POINT('Ctrl Pts',(-29.0509395126143,-65.9983248641879,
12.));
#72542=CARTESIAN_POINT('Ctrl Pts',(-29.0524170987307,-66.0225307679591,
0.));
#72543=CARTESIAN_POINT('Ctrl Pts',(-29.0524170987307,-66.0225307679591,
12.));
#72544=CARTESIAN_POINT('Ctrl Pts',(-29.0538736947552,-66.0467797705815,
0.));
#72545=CARTESIAN_POINT('Ctrl Pts',(-29.0538736947552,-66.0467797705815,
12.));
#72546=CARTESIAN_POINT('Ctrl Pts',(-29.0553092342279,-66.0710717597009,
0.));
#72547=CARTESIAN_POINT('Ctrl Pts',(-29.0553092342279,-66.0710717597009,
12.));
#72548=CARTESIAN_POINT('Ctrl Pts',(-29.0567236510374,-66.0954066233754,
0.));
#72549=CARTESIAN_POINT('Ctrl Pts',(-29.0567236510374,-66.0954066233754,
12.));
#72550=CARTESIAN_POINT('Ctrl Pts',(-29.058116879419,-66.1197842500711,0.));
#72551=CARTESIAN_POINT('Ctrl Pts',(-29.058116879419,-66.1197842500711,12.));
#72552=CARTESIAN_POINT('Ctrl Pts',(-29.0594888539556,-66.1442045286516,
0.));
#72553=CARTESIAN_POINT('Ctrl Pts',(-29.0594888539556,-66.1442045286516,
12.));
#72554=CARTESIAN_POINT('Ctrl Pts',(-29.0608395095746,-66.1686673483755,
0.));
#72555=CARTESIAN_POINT('Ctrl Pts',(-29.0608395095746,-66.1686673483755,
12.));
#72556=CARTESIAN_POINT('Ctrl Pts',(-29.062168781542,-66.1931725989008,0.));
#72557=CARTESIAN_POINT('Ctrl Pts',(-29.062168781542,-66.1931725989008,12.));
#72558=CARTESIAN_POINT('Ctrl Pts',(-29.0634766054599,-66.2177201702819,
0.));
#72559=CARTESIAN_POINT('Ctrl Pts',(-29.0634766054599,-66.2177201702819,
12.));
#72560=CARTESIAN_POINT('Ctrl Pts',(-29.0647629172645,-66.2423099529668,
0.));
#72561=CARTESIAN_POINT('Ctrl Pts',(-29.0647629172645,-66.2423099529668,
12.));
#72562=CARTESIAN_POINT('Ctrl Pts',(-29.0660276532272,-66.2669418377865,
0.));
#72563=CARTESIAN_POINT('Ctrl Pts',(-29.0660276532272,-66.2669418377865,
12.));
#72564=CARTESIAN_POINT('Ctrl Pts',(-29.0672707499527,-66.2916157159527,
0.));
#72565=CARTESIAN_POINT('Ctrl Pts',(-29.0672707499527,-66.2916157159527,
12.));
#72566=CARTESIAN_POINT('Ctrl Pts',(-29.0684921443718,-66.3163314790607,
0.));
#72567=CARTESIAN_POINT('Ctrl Pts',(-29.0684921443718,-66.3163314790607,
12.));
#72568=CARTESIAN_POINT('Ctrl Pts',(-29.0696917737398,-66.3410890190879,
0.));
#72569=CARTESIAN_POINT('Ctrl Pts',(-29.0696917737398,-66.3410890190879,
12.));
#72570=CARTESIAN_POINT('Ctrl Pts',(-29.0708695756336,-66.3658882283906,
0.));
#72571=CARTESIAN_POINT('Ctrl Pts',(-29.0708695756336,-66.3658882283906,
12.));
#72572=CARTESIAN_POINT('Ctrl Pts',(-29.0720254879535,-66.3907289996942,
0.));
#72573=CARTESIAN_POINT('Ctrl Pts',(-29.0720254879535,-66.3907289996942,
12.));
#72574=CARTESIAN_POINT('Ctrl Pts',(-29.0731594489219,-66.4156112260904,
0.));
#72575=CARTESIAN_POINT('Ctrl Pts',(-29.0731594489219,-66.4156112260904,
12.));
#72576=CARTESIAN_POINT('Ctrl Pts',(-29.0742713970762,-66.4405348010404,
0.));
#72577=CARTESIAN_POINT('Ctrl Pts',(-29.0742713970762,-66.4405348010404,
12.));
#72578=CARTESIAN_POINT('Ctrl Pts',(-29.075361271267,-66.4654996183739,0.));
#72579=CARTESIAN_POINT('Ctrl Pts',(-29.075361271267,-66.4654996183739,12.));
#72580=CARTESIAN_POINT('Ctrl Pts',(-29.0764290106553,-66.4905055722864,
0.));
#72581=CARTESIAN_POINT('Ctrl Pts',(-29.0764290106553,-66.4905055722864,
12.));
#72582=CARTESIAN_POINT('Ctrl Pts',(-29.0774745547146,-66.5155525573308,
0.));
#72583=CARTESIAN_POINT('Ctrl Pts',(-29.0774745547146,-66.5155525573308,
12.));
#72584=CARTESIAN_POINT('Ctrl Pts',(-29.0784978432294,-66.5406404684116,
0.));
#72585=CARTESIAN_POINT('Ctrl Pts',(-29.0784978432294,-66.5406404684116,
12.));
#72586=CARTESIAN_POINT('Ctrl Pts',(-29.0794988162892,-66.5657692007894,
0.));
#72587=CARTESIAN_POINT('Ctrl Pts',(-29.0794988162892,-66.5657692007894,
12.));
#72588=CARTESIAN_POINT('Ctrl Pts',(-29.0804774142852,-66.5909386500796,
0.));
#72589=CARTESIAN_POINT('Ctrl Pts',(-29.0804774142852,-66.5909386500796,
12.));
#72590=CARTESIAN_POINT('Ctrl Pts',(-29.0814335779086,-66.6161487122504,
0.));
#72591=CARTESIAN_POINT('Ctrl Pts',(-29.0814335779086,-66.6161487122504,
12.));
#72592=CARTESIAN_POINT('Ctrl Pts',(-29.0823672481508,-66.6413992836148,
0.));
#72593=CARTESIAN_POINT('Ctrl Pts',(-29.0823672481508,-66.6413992836148,
12.));
#72594=CARTESIAN_POINT('Ctrl Pts',(-29.0832783663049,-66.6666902608246,
0.));
#72595=CARTESIAN_POINT('Ctrl Pts',(-29.0832783663049,-66.6666902608246,
12.));
#72596=CARTESIAN_POINT('Ctrl Pts',(-29.0841668739585,-66.6920215408744,
0.));
#72597=CARTESIAN_POINT('Ctrl Pts',(-29.0841668739585,-66.6920215408744,
12.));
#72598=CARTESIAN_POINT('Ctrl Pts',(-29.0850327129914,-66.7173930211015,
0.));
#72599=CARTESIAN_POINT('Ctrl Pts',(-29.0850327129914,-66.7173930211015,
12.));
#72600=CARTESIAN_POINT('Ctrl Pts',(-29.0858758255729,-66.742804599184,0.));
#72601=CARTESIAN_POINT('Ctrl Pts',(-29.0858758255729,-66.742804599184,12.));
#72602=CARTESIAN_POINT('Ctrl Pts',(-29.086696154163,-66.7682561731348,0.));
#72603=CARTESIAN_POINT('Ctrl Pts',(-29.086696154163,-66.7682561731348,12.));
#72604=CARTESIAN_POINT('Ctrl Pts',(-29.0874936415138,-66.7937476412941,
0.));
#72605=CARTESIAN_POINT('Ctrl Pts',(-29.0874936415138,-66.7937476412941,
12.));
#72606=CARTESIAN_POINT('Ctrl Pts',(-29.0882682306636,-66.8192789023323,
0.));
#72607=CARTESIAN_POINT('Ctrl Pts',(-29.0882682306636,-66.8192789023323,
12.));
#72608=CARTESIAN_POINT('Ctrl Pts',(-29.0890198649327,-66.8448498552508,
0.));
#72609=CARTESIAN_POINT('Ctrl Pts',(-29.0890198649327,-66.8448498552508,
12.));
#72610=CARTESIAN_POINT('Ctrl Pts',(-29.0897484879208,-66.8704603993794,
0.));
#72611=CARTESIAN_POINT('Ctrl Pts',(-29.0897484879208,-66.8704603993794,
12.));
#72612=CARTESIAN_POINT('Ctrl Pts',(-29.0904540435063,-66.8961104343703,
0.));
#72613=CARTESIAN_POINT('Ctrl Pts',(-29.0904540435063,-66.8961104343703,
12.));
#72614=CARTESIAN_POINT('Ctrl Pts',(-29.0911364758484,-66.9217998601881,
0.));
#72615=CARTESIAN_POINT('Ctrl Pts',(-29.0911364758484,-66.9217998601881,
12.));
#72616=CARTESIAN_POINT('Ctrl Pts',(-29.0917957293824,-66.9475285771133,
0.));
#72617=CARTESIAN_POINT('Ctrl Pts',(-29.0917957293824,-66.9475285771133,
12.));
#72618=CARTESIAN_POINT('Ctrl Pts',(-29.092431748817,-66.9732964857467,0.));
#72619=CARTESIAN_POINT('Ctrl Pts',(-29.092431748817,-66.9732964857467,12.));
#72620=CARTESIAN_POINT('Ctrl Pts',(-29.0930444791329,-66.9991034870084,
0.));
#72621=CARTESIAN_POINT('Ctrl Pts',(-29.0930444791329,-66.9991034870084,
12.));
#72622=CARTESIAN_POINT('Ctrl Pts',(-29.0936338655828,-67.0249494821361,
0.));
#72623=CARTESIAN_POINT('Ctrl Pts',(-29.0936338655828,-67.0249494821361,
12.));
#72624=CARTESIAN_POINT('Ctrl Pts',(-29.0941998536958,-67.0508343726771,
0.));
#72625=CARTESIAN_POINT('Ctrl Pts',(-29.0941998536958,-67.0508343726771,
12.));
#72626=CARTESIAN_POINT('Ctrl Pts',(-29.0947423892725,-67.0767580604872,
0.));
#72627=CARTESIAN_POINT('Ctrl Pts',(-29.0947423892725,-67.0767580604872,
12.));
#72628=CARTESIAN_POINT('Ctrl Pts',(-29.0952614183777,-67.1027204477304,
0.));
#72629=CARTESIAN_POINT('Ctrl Pts',(-29.0952614183777,-67.1027204477304,
12.));
#72630=CARTESIAN_POINT('Ctrl Pts',(-29.0957568873358,-67.1287214368743,
0.));
#72631=CARTESIAN_POINT('Ctrl Pts',(-29.0957568873358,-67.1287214368743,
12.));
#72632=CARTESIAN_POINT('Ctrl Pts',(-29.0962287427274,-67.1547609306845,
0.));
#72633=CARTESIAN_POINT('Ctrl Pts',(-29.0962287427274,-67.1547609306845,
12.));
#72634=CARTESIAN_POINT('Ctrl Pts',(-29.0966769313893,-67.1808388322116,
0.));
#72635=CARTESIAN_POINT('Ctrl Pts',(-29.0966769313893,-67.1808388322116,
12.));
#72636=CARTESIAN_POINT('Ctrl Pts',(-29.0971014004135,-67.2069550447895,
0.));
#72637=CARTESIAN_POINT('Ctrl Pts',(-29.0971014004135,-67.2069550447895,
12.));
#72638=CARTESIAN_POINT('Ctrl Pts',(-29.0975020971474,-67.2331094720482,
0.));
#72639=CARTESIAN_POINT('Ctrl Pts',(-29.0975020971474,-67.2331094720482,
12.));
#72640=CARTESIAN_POINT('Ctrl Pts',(-29.0978789691965,-67.2593020179216,
0.));
#72641=CARTESIAN_POINT('Ctrl Pts',(-29.0978789691965,-67.2593020179216,
12.));
#72642=CARTESIAN_POINT('Ctrl Pts',(-29.0982319644277,-67.2855325866516,
0.));
#72643=CARTESIAN_POINT('Ctrl Pts',(-29.0982319644277,-67.2855325866516,
12.));
#72644=CARTESIAN_POINT('Ctrl Pts',(-29.0985610309768,-67.311801082791,0.));
#72645=CARTESIAN_POINT('Ctrl Pts',(-29.0985610309768,-67.311801082791,12.));
#72646=CARTESIAN_POINT('Ctrl Pts',(-29.0988661172526,-67.3381074112013,
0.));
#72647=CARTESIAN_POINT('Ctrl Pts',(-29.0988661172526,-67.3381074112013,
12.));
#72648=CARTESIAN_POINT('Ctrl Pts',(-29.0991471719172,-67.3644514770373,
0.));
#72649=CARTESIAN_POINT('Ctrl Pts',(-29.0991471719172,-67.3644514770373,
12.));
#72650=CARTESIAN_POINT('Ctrl Pts',(-29.0994041438715,-67.3908331857313,
0.));
#72651=CARTESIAN_POINT('Ctrl Pts',(-29.0994041438715,-67.3908331857313,
12.));
#72652=CARTESIAN_POINT('Ctrl Pts',(-29.0996369822418,-67.4172524429726,
0.));
#72653=CARTESIAN_POINT('Ctrl Pts',(-29.0996369822418,-67.4172524429726,
12.));
#72654=CARTESIAN_POINT('Ctrl Pts',(-29.0998456363687,-67.4437091546869,
0.));
#72655=CARTESIAN_POINT('Ctrl Pts',(-29.0998456363687,-67.4437091546869,
12.));
#72656=CARTESIAN_POINT('Ctrl Pts',(-29.1000300557961,-67.4702032270062,
0.));
#72657=CARTESIAN_POINT('Ctrl Pts',(-29.1000300557961,-67.4702032270062,
12.));
#72658=CARTESIAN_POINT('Ctrl Pts',(-29.1001901902915,-67.496734566311,0.));
#72659=CARTESIAN_POINT('Ctrl Pts',(-29.1001901902915,-67.496734566311,12.));
#72660=CARTESIAN_POINT('Ctrl Pts',(-29.1003259898686,-67.5233030792714,
0.));
#72661=CARTESIAN_POINT('Ctrl Pts',(-29.1003259898686,-67.5233030792714,
12.));
#72662=CARTESIAN_POINT('Ctrl Pts',(-29.1004374048149,-67.5499086728891,
0.));
#72663=CARTESIAN_POINT('Ctrl Pts',(-29.1004374048149,-67.5499086728891,
12.));
#72664=CARTESIAN_POINT('Ctrl Pts',(-29.1005243857137,-67.5765512545276,
0.));
#72665=CARTESIAN_POINT('Ctrl Pts',(-29.1005243857137,-67.5765512545276,
12.));
#72666=CARTESIAN_POINT('Ctrl Pts',(-29.1005868834863,-67.6032307319614,
0.));
#72667=CARTESIAN_POINT('Ctrl Pts',(-29.1005868834863,-67.6032307319614,
12.));
#72668=CARTESIAN_POINT('Ctrl Pts',(-29.1006248493577,-67.6299470133286,
0.));
#72669=CARTESIAN_POINT('Ctrl Pts',(-29.1006248493577,-67.6299470133286,
12.));
#72670=CARTESIAN_POINT('Ctrl Pts',(-29.1006382347812,-67.6567000070319,
0.));
#72671=CARTESIAN_POINT('Ctrl Pts',(-29.1006382347812,-67.6567000070319,
12.));
#72672=CARTESIAN_POINT('Ctrl Pts',(-29.1006269913747,-67.6834896216458,
0.));
#72673=CARTESIAN_POINT('Ctrl Pts',(-29.1006269913747,-67.6834896216458,
12.));
#72674=CARTESIAN_POINT('Ctrl Pts',(-29.1005910708625,-67.7103157658296,
0.));
#72675=CARTESIAN_POINT('Ctrl Pts',(-29.1005910708625,-67.7103157658296,
12.));
#72676=CARTESIAN_POINT('Ctrl Pts',(-29.1005304249989,-67.7371783482038,
0.));
#72677=CARTESIAN_POINT('Ctrl Pts',(-29.1005304249989,-67.7371783482038,
12.));
#72678=CARTESIAN_POINT('Ctrl Pts',(-29.1004450055647,-67.7640772773397,
0.));
#72679=CARTESIAN_POINT('Ctrl Pts',(-29.1004450055647,-67.7640772773397,
12.));
#72680=CARTESIAN_POINT('Ctrl Pts',(-29.10033476453,-67.7910124620148,0.));
#72681=CARTESIAN_POINT('Ctrl Pts',(-29.10033476453,-67.7910124620148,12.));
#72682=CARTESIAN_POINT('Ctrl Pts',(-29.1001996541847,-67.8179838114109,
0.));
#72683=CARTESIAN_POINT('Ctrl Pts',(-29.1001996541847,-67.8179838114109,
12.));
#72684=CARTESIAN_POINT('Ctrl Pts',(-29.1000396272868,-67.844991235333,0.));
#72685=CARTESIAN_POINT('Ctrl Pts',(-29.1000396272868,-67.844991235333,12.));
#72686=CARTESIAN_POINT('Ctrl Pts',(-29.0998546372027,-67.8720346444111,
0.));
#72687=CARTESIAN_POINT('Ctrl Pts',(-29.0998546372027,-67.8720346444111,
12.));
#72688=CARTESIAN_POINT('Ctrl Pts',(-29.0996446380617,-67.8991139503168,
0.));
#72689=CARTESIAN_POINT('Ctrl Pts',(-29.0996446380617,-67.8991139503168,
12.));
#72690=CARTESIAN_POINT('Ctrl Pts',(-29.0994095844208,-67.9262290652797,
0.));
#72691=CARTESIAN_POINT('Ctrl Pts',(-29.0994095844208,-67.9262290652797,
12.));
#72692=CARTESIAN_POINT('Ctrl Pts',(-29.0991494309395,-67.9533799016122,
0.));
#72693=CARTESIAN_POINT('Ctrl Pts',(-29.0991494309395,-67.9533799016122,
12.));
#72694=CARTESIAN_POINT('Ctrl Pts',(-29.0988641320243,-67.9805663711845,
0.));
#72695=CARTESIAN_POINT('Ctrl Pts',(-29.0988641320243,-67.9805663711845,
12.));
#72696=CARTESIAN_POINT('Ctrl Pts',(-29.0985536415537,-68.0077883850136,
0.));
#72697=CARTESIAN_POINT('Ctrl Pts',(-29.0985536415537,-68.0077883850136,
12.));
#72698=CARTESIAN_POINT('Ctrl Pts',(-29.0982179124113,-68.0350458525589,
0.));
#72699=CARTESIAN_POINT('Ctrl Pts',(-29.0982179124113,-68.0350458525589,
12.));
#72700=CARTESIAN_POINT('Ctrl Pts',(-29.0978568968678,-68.0623386822917,
0.));
#72701=CARTESIAN_POINT('Ctrl Pts',(-29.0978568968678,-68.0623386822917,
12.));
#72702=CARTESIAN_POINT('Ctrl Pts',(-29.0974705474279,-68.089666782962,0.));
#72703=CARTESIAN_POINT('Ctrl Pts',(-29.0974705474279,-68.089666782962,12.));
#72704=CARTESIAN_POINT('Ctrl Pts',(-29.0970588175741,-68.1170300647019,
0.));
#72705=CARTESIAN_POINT('Ctrl Pts',(-29.0970588175741,-68.1170300647019,
12.));
#72706=CARTESIAN_POINT('Ctrl Pts',(-29.0966216624741,-68.1444284400734,
0.));
#72707=CARTESIAN_POINT('Ctrl Pts',(-29.0966216624741,-68.1444284400734,
12.));
#72708=CARTESIAN_POINT('Ctrl Pts',(-29.0961590399023,-68.1718618254221,
0.));
#72709=CARTESIAN_POINT('Ctrl Pts',(-29.0961590399023,-68.1718618254221,
12.));
#72710=CARTESIAN_POINT('Ctrl Pts',(-29.0956709104588,-68.1993301411959,
0.));
#72711=CARTESIAN_POINT('Ctrl Pts',(-29.0956709104588,-68.1993301411959,
12.));
#72712=CARTESIAN_POINT('Ctrl Pts',(-29.0951572355353,-68.22683330895,0.));
#72713=CARTESIAN_POINT('Ctrl Pts',(-29.0951572355353,-68.22683330895,12.));
#72714=CARTESIAN_POINT('Ctrl Pts',(-29.0946179757133,-68.2543712489815,
0.));
#72715=CARTESIAN_POINT('Ctrl Pts',(-29.0946179757133,-68.2543712489815,
12.));
#72716=CARTESIAN_POINT('Ctrl Pts',(-29.0940530889142,-68.2819438775932,
0.));
#72717=CARTESIAN_POINT('Ctrl Pts',(-29.0940530889142,-68.2819438775932,
12.));
#72718=CARTESIAN_POINT('Ctrl Pts',(-29.0934625288442,-68.3095511047852,
0.));
#72719=CARTESIAN_POINT('Ctrl Pts',(-29.0934625288442,-68.3095511047852,
12.));
#72720=CARTESIAN_POINT('Ctrl Pts',(-29.0928462428218,-68.3371928310351,
0.));
#72721=CARTESIAN_POINT('Ctrl Pts',(-29.0928462428218,-68.3371928310351,
12.));
#72722=CARTESIAN_POINT('Ctrl Pts',(-29.0922041749393,-68.3648689519188,
0.));
#72723=CARTESIAN_POINT('Ctrl Pts',(-29.0922041749393,-68.3648689519188,
12.));
#72724=CARTESIAN_POINT('Ctrl Pts',(-29.091536269955,-68.3925793638241,0.));
#72725=CARTESIAN_POINT('Ctrl Pts',(-29.091536269955,-68.3925793638241,12.));
#72726=CARTESIAN_POINT('Ctrl Pts',(-29.0908424770941,-68.4203239694742,
0.));
#72727=CARTESIAN_POINT('Ctrl Pts',(-29.0908424770941,-68.4203239694742,
12.));
#72728=CARTESIAN_POINT('Ctrl Pts',(-29.0901227535274,-68.4481026830845,
0.));
#72729=CARTESIAN_POINT('Ctrl Pts',(-29.0901227535274,-68.4481026830845,
12.));
#72730=CARTESIAN_POINT('Ctrl Pts',(-29.0893770688808,-68.4759154367582,
0.));
#72731=CARTESIAN_POINT('Ctrl Pts',(-29.0893770688808,-68.4759154367582,
12.));
#72732=CARTESIAN_POINT('Ctrl Pts',(-29.0886054060334,-68.5037621823575,
0.));
#72733=CARTESIAN_POINT('Ctrl Pts',(-29.0886054060334,-68.5037621823575,
12.));
#72734=CARTESIAN_POINT('Ctrl Pts',(-29.0878077570819,-68.5316428874729,
0.));
#72735=CARTESIAN_POINT('Ctrl Pts',(-29.0878077570819,-68.5316428874729,
12.));
#72736=CARTESIAN_POINT('Ctrl Pts',(-29.0871488478365,-68.5539746037961,
0.));
#72737=CARTESIAN_POINT('Ctrl Pts',(-29.0871488478365,-68.5539746037961,
12.));
#72738=CARTESIAN_POINT('Ctrl Pts',(-29.0866429721959,-68.5707386600286,
0.));
#72739=CARTESIAN_POINT('Ctrl Pts',(-29.0866429721959,-68.5707386600286,
12.));
#72740=CARTESIAN_POINT('Ctrl Pts',(-29.086300524779,-68.5819214834609,0.));
#72741=CARTESIAN_POINT('Ctrl Pts',(-29.086300524779,-68.5819214834609,12.));
#72742=CARTESIAN_POINT('Ctrl Pts',(-29.086128001823,-68.5875145916629,0.));
#72743=CARTESIAN_POINT('Ctrl Pts',(-29.086128001823,-68.5875145916629,12.));
#72744=CARTESIAN_POINT('',(-28.8072485549237,-63.7976679095314,0.));
#72745=CARTESIAN_POINT('Ctrl Pts',(-28.8072485549237,-63.7976679095314,
0.));
#72746=CARTESIAN_POINT('Ctrl Pts',(-28.8078854475432,-63.8014989507494,
0.));
#72747=CARTESIAN_POINT('Ctrl Pts',(-28.8091580239553,-63.8091667271231,
0.));
#72748=CARTESIAN_POINT('Ctrl Pts',(-28.8110632620958,-63.8206854735027,
0.));
#72749=CARTESIAN_POINT('Ctrl Pts',(-28.8135963263369,-63.8360779669856,
0.));
#72750=CARTESIAN_POINT('Ctrl Pts',(-28.8167505576681,-63.8553755207486,
0.));
#72751=CARTESIAN_POINT('Ctrl Pts',(-28.8198926619858,-63.8747299825313,
0.));
#72752=CARTESIAN_POINT('Ctrl Pts',(-28.823022586318,-63.8941412856923,0.));
#72753=CARTESIAN_POINT('Ctrl Pts',(-28.8261402423291,-63.9136093063786,
0.));
#72754=CARTESIAN_POINT('Ctrl Pts',(-28.8292455077559,-63.9331338646996,
0.));
#72755=CARTESIAN_POINT('Ctrl Pts',(-28.8323382413789,-63.9527147494423,
0.));
#72756=CARTESIAN_POINT('Ctrl Pts',(-28.8354182946601,-63.9723517369614,
0.));
#72757=CARTESIAN_POINT('Ctrl Pts',(-28.8384855243243,-63.9920446117582,
0.));
#72758=CARTESIAN_POINT('Ctrl Pts',(-28.8415398056428,-64.0117931881298,
0.));
#72759=CARTESIAN_POINT('Ctrl Pts',(-28.844581028125,-64.0315973031942,0.));
#72760=CARTESIAN_POINT('Ctrl Pts',(-28.8476090892232,-64.0514568066637,
0.));
#72761=CARTESIAN_POINT('Ctrl Pts',(-28.8506238891093,-64.0713715523599,
0.));
#72762=CARTESIAN_POINT('Ctrl Pts',(-28.8536253241854,-64.0913413876622,
0.));
#72763=CARTESIAN_POINT('Ctrl Pts',(-28.8566132838179,-64.1113661481965,
0.));
#72764=CARTESIAN_POINT('Ctrl Pts',(-28.8595876537148,-64.1314456633381,
0.));
#72765=CARTESIAN_POINT('Ctrl Pts',(-28.8625483180438,-64.1515797596564,
0.));
#72766=CARTESIAN_POINT('Ctrl Pts',(-28.8654951618649,-64.1717682648685,
0.));
#72767=CARTESIAN_POINT('Ctrl Pts',(-28.8684280739014,-64.1920110123299,
0.));
#72768=CARTESIAN_POINT('Ctrl Pts',(-28.8713469464185,-64.2123078408461,
0.));
#72769=CARTESIAN_POINT('Ctrl Pts',(-28.8742516738947,-64.2326585925252,
0.));
#72770=CARTESIAN_POINT('Ctrl Pts',(-28.877142152106,-64.2530631112929,0.));
#72771=CARTESIAN_POINT('Ctrl Pts',(-28.8800182770065,-64.273521241071,0.));
#72772=CARTESIAN_POINT('Ctrl Pts',(-28.882879943794,-64.2940328242521,0.));
#72773=CARTESIAN_POINT('Ctrl Pts',(-28.8857270473959,-64.3145977025037,
0.));
#72774=CARTESIAN_POINT('Ctrl Pts',(-28.8885594828926,-64.3352157174619,
0.));
#72775=CARTESIAN_POINT('Ctrl Pts',(-28.8913771459323,-64.3558867114076,
0.));
#72776=CARTESIAN_POINT('Ctrl Pts',(-28.89417993323,-64.3766105280688,0.));
#72777=CARTESIAN_POINT('Ctrl Pts',(-28.8969677427504,-64.3973870129169,
0.));
#72778=CARTESIAN_POINT('Ctrl Pts',(-28.899740473434,-64.4182160127379,0.));
#72779=CARTESIAN_POINT('Ctrl Pts',(-28.9024980250307,-64.4390973753634,
0.));
#72780=CARTESIAN_POINT('Ctrl Pts',(-28.9052402979062,-64.4600309493583,
0.));
#72781=CARTESIAN_POINT('Ctrl Pts',(-28.9079671928264,-64.4810165836592,
0.));
#72782=CARTESIAN_POINT('Ctrl Pts',(-28.910678610965,-64.5020541275951,0.));
#72783=CARTESIAN_POINT('Ctrl Pts',(-28.9133744539949,-64.523143431047,0.));
#72784=CARTESIAN_POINT('Ctrl Pts',(-28.9160546241538,-64.5442843445559,
0.));
#72785=CARTESIAN_POINT('Ctrl Pts',(-28.9187190243224,-64.5654767194471,
0.));
#72786=CARTESIAN_POINT('Ctrl Pts',(-28.9213675580985,-64.5867204079426,
0.));
#72787=CARTESIAN_POINT('Ctrl Pts',(-28.9240001297542,-64.6080152631039,
0.));
#72788=CARTESIAN_POINT('Ctrl Pts',(-28.9266166441951,-64.629361138774,0.));
#72789=CARTESIAN_POINT('Ctrl Pts',(-28.9292170069222,-64.6507578895161,
0.));
#72790=CARTESIAN_POINT('Ctrl Pts',(-28.9318011239915,-64.672205370541,0.));
#72791=CARTESIAN_POINT('Ctrl Pts',(-28.9343689019882,-64.6937034376617,
0.));
#72792=CARTESIAN_POINT('Ctrl Pts',(-28.9369202480393,-64.715251947329,0.));
#72793=CARTESIAN_POINT('Ctrl Pts',(-28.9394550698204,-64.7368507566467,
0.));
#72794=CARTESIAN_POINT('Ctrl Pts',(-28.9419732755656,-64.758499723388,0.));
#72795=CARTESIAN_POINT('Ctrl Pts',(-28.944474774081,-64.7801987060084,0.));
#72796=CARTESIAN_POINT('Ctrl Pts',(-28.9469594747432,-64.8019475636442,
0.));
#72797=CARTESIAN_POINT('Ctrl Pts',(-28.9494272874832,-64.8237461561018,
0.));
#72798=CARTESIAN_POINT('Ctrl Pts',(-28.9518781227765,-64.8455943438423,
0.));
#72799=CARTESIAN_POINT('Ctrl Pts',(-28.9543118916328,-64.8674919879648,
0.));
#72800=CARTESIAN_POINT('Ctrl Pts',(-28.9567285055867,-64.8894389501801,
0.));
#72801=CARTESIAN_POINT('Ctrl Pts',(-28.9591278766934,-64.9114350928125,
0.));
#72802=CARTESIAN_POINT('Ctrl Pts',(-28.961509917525,-64.9334802788038,0.));
#72803=CARTESIAN_POINT('Ctrl Pts',(-28.9638745411677,-64.9555743717109,
0.));
#72804=CARTESIAN_POINT('Ctrl Pts',(-28.9662216612217,-64.9777172357027,
0.));
#72805=CARTESIAN_POINT('Ctrl Pts',(-28.9685511918018,-64.9999087355504,
0.));
#72806=CARTESIAN_POINT('Ctrl Pts',(-28.97086304753,-65.022148736628,0.));
#72807=CARTESIAN_POINT('Ctrl Pts',(-28.9731571435283,-65.0444371049082,
0.));
#72808=CARTESIAN_POINT('Ctrl Pts',(-28.9754333954135,-65.0667737069563,
0.));
#72809=CARTESIAN_POINT('Ctrl Pts',(-28.9776917192933,-65.0891584099168,
0.));
#72810=CARTESIAN_POINT('Ctrl Pts',(-28.9799320317641,-65.1115910815037,
0.));
#72811=CARTESIAN_POINT('Ctrl Pts',(-28.9821542499043,-65.1340715900028,
0.));
#72812=CARTESIAN_POINT('Ctrl Pts',(-28.9843582912693,-65.1565998042697,
0.));
#72813=CARTESIAN_POINT('Ctrl Pts',(-28.9865440738884,-65.1791755937256,
0.));
#72814=CARTESIAN_POINT('Ctrl Pts',(-28.9887115162634,-65.2017988283479,
0.));
#72815=CARTESIAN_POINT('Ctrl Pts',(-28.9908605373663,-65.2244693786609,
0.));
#72816=CARTESIAN_POINT('Ctrl Pts',(-28.9929910566325,-65.2471871157397,
0.));
#72817=CARTESIAN_POINT('Ctrl Pts',(-28.9951029939557,-65.2699519112064,
0.));
#72818=CARTESIAN_POINT('Ctrl Pts',(-28.9971962696845,-65.2927636372253,
0.));
#72819=CARTESIAN_POINT('Ctrl Pts',(-28.9992708046212,-65.3156221664916,
0.));
#72820=CARTESIAN_POINT('Ctrl Pts',(-29.0013265200185,-65.3385273722241,
0.));
#72821=CARTESIAN_POINT('Ctrl Pts',(-29.003363337573,-65.3614791281692,0.));
#72822=CARTESIAN_POINT('Ctrl Pts',(-29.0053811794207,-65.3844773085961,
0.));
#72823=CARTESIAN_POINT('Ctrl Pts',(-29.0073799681342,-65.4075217882934,
0.));
#72824=CARTESIAN_POINT('Ctrl Pts',(-29.0093596267216,-65.4306124425562,
0.));
#72825=CARTESIAN_POINT('Ctrl Pts',(-29.0113200786239,-65.4537491471828,
0.));
#72826=CARTESIAN_POINT('Ctrl Pts',(-29.013261247709,-65.4769317784789,0.));
#72827=CARTESIAN_POINT('Ctrl Pts',(-29.0151830582675,-65.5001602132535,
0.));
#72828=CARTESIAN_POINT('Ctrl Pts',(-29.0170854350095,-65.5234343288136,
0.));
#72829=CARTESIAN_POINT('Ctrl Pts',(-29.0189683030642,-65.5467540029514,
0.));
#72830=CARTESIAN_POINT('Ctrl Pts',(-29.0208315879764,-65.5701191139418,
0.));
#72831=CARTESIAN_POINT('Ctrl Pts',(-29.0226752157003,-65.5935295405453,
0.));
#72832=CARTESIAN_POINT('Ctrl Pts',(-29.0244991125959,-65.6169851620046,
0.));
#72833=CARTESIAN_POINT('Ctrl Pts',(-29.0263032054266,-65.6404858580403,
0.));
#72834=CARTESIAN_POINT('Ctrl Pts',(-29.0280874213596,-65.6640315088388,
0.));
#72835=CARTESIAN_POINT('Ctrl Pts',(-29.0298516879612,-65.6876219950493,
0.));
#72836=CARTESIAN_POINT('Ctrl Pts',(-29.0315959331919,-65.7112571977891,
0.));
#72837=CARTESIAN_POINT('Ctrl Pts',(-29.0333200854028,-65.7349369986384,
0.));
#72838=CARTESIAN_POINT('Ctrl Pts',(-29.035024073333,-65.7586612796368,0.));
#72839=CARTESIAN_POINT('Ctrl Pts',(-29.0367078261103,-65.7824299232705,
0.));
#72840=CARTESIAN_POINT('Ctrl Pts',(-29.0383712732469,-65.8062428124713,
0.));
#72841=CARTESIAN_POINT('Ctrl Pts',(-29.0400143446338,-65.8300998306191,
0.));
#72842=CARTESIAN_POINT('Ctrl Pts',(-29.0416369705375,-65.854000861539,0.));
#72843=CARTESIAN_POINT('Ctrl Pts',(-29.0432390815978,-65.8779457894961,
0.));
#72844=CARTESIAN_POINT('Ctrl Pts',(-29.0448206088289,-65.9019344991854,
0.));
#72845=CARTESIAN_POINT('Ctrl Pts',(-29.0463814836157,-65.9259668757306,
0.));
#72846=CARTESIAN_POINT('Ctrl Pts',(-29.0479216377081,-65.9500428046868,
0.));
#72847=CARTESIAN_POINT('Ctrl Pts',(-29.0494410032173,-65.9741621720369,
0.));
#72848=CARTESIAN_POINT('Ctrl Pts',(-29.0509395126143,-65.9983248641879,
0.));
#72849=CARTESIAN_POINT('Ctrl Pts',(-29.0524170987307,-66.0225307679591,
0.));
#72850=CARTESIAN_POINT('Ctrl Pts',(-29.0538736947552,-66.0467797705815,
0.));
#72851=CARTESIAN_POINT('Ctrl Pts',(-29.0553092342279,-66.0710717597009,
0.));
#72852=CARTESIAN_POINT('Ctrl Pts',(-29.0567236510374,-66.0954066233754,
0.));
#72853=CARTESIAN_POINT('Ctrl Pts',(-29.058116879419,-66.1197842500711,0.));
#72854=CARTESIAN_POINT('Ctrl Pts',(-29.0594888539556,-66.1442045286516,
0.));
#72855=CARTESIAN_POINT('Ctrl Pts',(-29.0608395095746,-66.1686673483755,
0.));
#72856=CARTESIAN_POINT('Ctrl Pts',(-29.062168781542,-66.1931725989008,0.));
#72857=CARTESIAN_POINT('Ctrl Pts',(-29.0634766054599,-66.2177201702819,
0.));
#72858=CARTESIAN_POINT('Ctrl Pts',(-29.0647629172645,-66.2423099529668,
0.));
#72859=CARTESIAN_POINT('Ctrl Pts',(-29.0660276532272,-66.2669418377865,
0.));
#72860=CARTESIAN_POINT('Ctrl Pts',(-29.0672707499527,-66.2916157159527,
0.));
#72861=CARTESIAN_POINT('Ctrl Pts',(-29.0684921443718,-66.3163314790607,
0.));
#72862=CARTESIAN_POINT('Ctrl Pts',(-29.0696917737398,-66.3410890190879,
0.));
#72863=CARTESIAN_POINT('Ctrl Pts',(-29.0708695756336,-66.3658882283906,
0.));
#72864=CARTESIAN_POINT('Ctrl Pts',(-29.0720254879535,-66.3907289996942,
0.));
#72865=CARTESIAN_POINT('Ctrl Pts',(-29.0731594489219,-66.4156112260904,
0.));
#72866=CARTESIAN_POINT('Ctrl Pts',(-29.0742713970762,-66.4405348010404,
0.));
#72867=CARTESIAN_POINT('Ctrl Pts',(-29.075361271267,-66.4654996183739,0.));
#72868=CARTESIAN_POINT('Ctrl Pts',(-29.0764290106553,-66.4905055722864,
0.));
#72869=CARTESIAN_POINT('Ctrl Pts',(-29.0774745547146,-66.5155525573308,
0.));
#72870=CARTESIAN_POINT('Ctrl Pts',(-29.0784978432294,-66.5406404684116,
0.));
#72871=CARTESIAN_POINT('Ctrl Pts',(-29.0794988162892,-66.5657692007894,
0.));
#72872=CARTESIAN_POINT('Ctrl Pts',(-29.0804774142852,-66.5909386500796,
0.));
#72873=CARTESIAN_POINT('Ctrl Pts',(-29.0814335779086,-66.6161487122504,
0.));
#72874=CARTESIAN_POINT('Ctrl Pts',(-29.0823672481508,-66.6413992836148,
0.));
#72875=CARTESIAN_POINT('Ctrl Pts',(-29.0832783663049,-66.6666902608246,
0.));
#72876=CARTESIAN_POINT('Ctrl Pts',(-29.0841668739585,-66.6920215408744,
0.));
#72877=CARTESIAN_POINT('Ctrl Pts',(-29.0850327129914,-66.7173930211015,
0.));
#72878=CARTESIAN_POINT('Ctrl Pts',(-29.0858758255729,-66.742804599184,0.));
#72879=CARTESIAN_POINT('Ctrl Pts',(-29.086696154163,-66.7682561731348,0.));
#72880=CARTESIAN_POINT('Ctrl Pts',(-29.0874936415138,-66.7937476412941,
0.));
#72881=CARTESIAN_POINT('Ctrl Pts',(-29.0882682306636,-66.8192789023323,
0.));
#72882=CARTESIAN_POINT('Ctrl Pts',(-29.0890198649327,-66.8448498552508,
0.));
#72883=CARTESIAN_POINT('Ctrl Pts',(-29.0897484879208,-66.8704603993794,
0.));
#72884=CARTESIAN_POINT('Ctrl Pts',(-29.0904540435063,-66.8961104343703,
0.));
#72885=CARTESIAN_POINT('Ctrl Pts',(-29.0911364758484,-66.9217998601881,
0.));
#72886=CARTESIAN_POINT('Ctrl Pts',(-29.0917957293824,-66.9475285771133,
0.));
#72887=CARTESIAN_POINT('Ctrl Pts',(-29.092431748817,-66.9732964857467,0.));
#72888=CARTESIAN_POINT('Ctrl Pts',(-29.0930444791329,-66.9991034870084,
0.));
#72889=CARTESIAN_POINT('Ctrl Pts',(-29.0936338655828,-67.0249494821361,
0.));
#72890=CARTESIAN_POINT('Ctrl Pts',(-29.0941998536958,-67.0508343726771,
0.));
#72891=CARTESIAN_POINT('Ctrl Pts',(-29.0947423892725,-67.0767580604872,
0.));
#72892=CARTESIAN_POINT('Ctrl Pts',(-29.0952614183777,-67.1027204477304,
0.));
#72893=CARTESIAN_POINT('Ctrl Pts',(-29.0957568873358,-67.1287214368743,
0.));
#72894=CARTESIAN_POINT('Ctrl Pts',(-29.0962287427274,-67.1547609306845,
0.));
#72895=CARTESIAN_POINT('Ctrl Pts',(-29.0966769313893,-67.1808388322116,
0.));
#72896=CARTESIAN_POINT('Ctrl Pts',(-29.0971014004135,-67.2069550447895,
0.));
#72897=CARTESIAN_POINT('Ctrl Pts',(-29.0975020971474,-67.2331094720482,
0.));
#72898=CARTESIAN_POINT('Ctrl Pts',(-29.0978789691965,-67.2593020179216,
0.));
#72899=CARTESIAN_POINT('Ctrl Pts',(-29.0982319644277,-67.2855325866516,
0.));
#72900=CARTESIAN_POINT('Ctrl Pts',(-29.0985610309768,-67.311801082791,0.));
#72901=CARTESIAN_POINT('Ctrl Pts',(-29.0988661172526,-67.3381074112013,
0.));
#72902=CARTESIAN_POINT('Ctrl Pts',(-29.0991471719172,-67.3644514770373,
0.));
#72903=CARTESIAN_POINT('Ctrl Pts',(-29.0994041438715,-67.3908331857313,
0.));
#72904=CARTESIAN_POINT('Ctrl Pts',(-29.0996369822418,-67.4172524429726,
0.));
#72905=CARTESIAN_POINT('Ctrl Pts',(-29.0998456363687,-67.4437091546869,
0.));
#72906=CARTESIAN_POINT('Ctrl Pts',(-29.1000300557961,-67.4702032270062,
0.));
#72907=CARTESIAN_POINT('Ctrl Pts',(-29.1001901902915,-67.496734566311,0.));
#72908=CARTESIAN_POINT('Ctrl Pts',(-29.1003259898686,-67.5233030792714,
0.));
#72909=CARTESIAN_POINT('Ctrl Pts',(-29.1004374048149,-67.5499086728891,
0.));
#72910=CARTESIAN_POINT('Ctrl Pts',(-29.1005243857137,-67.5765512545276,
0.));
#72911=CARTESIAN_POINT('Ctrl Pts',(-29.1005868834863,-67.6032307319614,
0.));
#72912=CARTESIAN_POINT('Ctrl Pts',(-29.1006248493577,-67.6299470133286,
0.));
#72913=CARTESIAN_POINT('Ctrl Pts',(-29.1006382347812,-67.6567000070319,
0.));
#72914=CARTESIAN_POINT('Ctrl Pts',(-29.1006269913747,-67.6834896216458,
0.));
#72915=CARTESIAN_POINT('Ctrl Pts',(-29.1005910708625,-67.7103157658296,
0.));
#72916=CARTESIAN_POINT('Ctrl Pts',(-29.1005304249989,-67.7371783482038,
0.));
#72917=CARTESIAN_POINT('Ctrl Pts',(-29.1004450055647,-67.7640772773397,
0.));
#72918=CARTESIAN_POINT('Ctrl Pts',(-29.10033476453,-67.7910124620148,0.));
#72919=CARTESIAN_POINT('Ctrl Pts',(-29.1001996541847,-67.8179838114109,
0.));
#72920=CARTESIAN_POINT('Ctrl Pts',(-29.1000396272868,-67.844991235333,0.));
#72921=CARTESIAN_POINT('Ctrl Pts',(-29.0998546372027,-67.8720346444111,
0.));
#72922=CARTESIAN_POINT('Ctrl Pts',(-29.0996446380617,-67.8991139503168,
0.));
#72923=CARTESIAN_POINT('Ctrl Pts',(-29.0994095844208,-67.9262290652797,
0.));
#72924=CARTESIAN_POINT('Ctrl Pts',(-29.0991494309395,-67.9533799016122,
0.));
#72925=CARTESIAN_POINT('Ctrl Pts',(-29.0988641320243,-67.9805663711845,
0.));
#72926=CARTESIAN_POINT('Ctrl Pts',(-29.0985536415537,-68.0077883850136,
0.));
#72927=CARTESIAN_POINT('Ctrl Pts',(-29.0982179124113,-68.0350458525589,
0.));
#72928=CARTESIAN_POINT('Ctrl Pts',(-29.0978568968678,-68.0623386822917,
0.));
#72929=CARTESIAN_POINT('Ctrl Pts',(-29.0974705474279,-68.089666782962,0.));
#72930=CARTESIAN_POINT('Ctrl Pts',(-29.0970588175741,-68.1170300647019,
0.));
#72931=CARTESIAN_POINT('Ctrl Pts',(-29.0966216624741,-68.1444284400734,
0.));
#72932=CARTESIAN_POINT('Ctrl Pts',(-29.0961590399023,-68.1718618254221,
0.));
#72933=CARTESIAN_POINT('Ctrl Pts',(-29.0956709104588,-68.1993301411959,
0.));
#72934=CARTESIAN_POINT('Ctrl Pts',(-29.0952305915108,-68.2229056854495,
0.));
#72935=CARTESIAN_POINT('Ctrl Pts',(-29.0948791947834,-68.2409993689947,
0.));
#72936=CARTESIAN_POINT('Ctrl Pts',(-29.094628043331,-68.2535957746883,0.));
#72937=CARTESIAN_POINT('Ctrl Pts',(-29.0944846386549,-68.2606847334624,
0.));
#72938=CARTESIAN_POINT('Ctrl Pts',(-29.0944526440249,-68.2622612909743,
0.));
#72939=CARTESIAN_POINT('',(-28.8072485549237,-63.7976679095314,12.));
#72940=CARTESIAN_POINT('',(-28.8072485549237,-63.7976679095314,0.));
#72941=CARTESIAN_POINT('Ctrl Pts',(-29.0944526440249,-68.2622612909743,
12.));
#72942=CARTESIAN_POINT('Ctrl Pts',(-29.0944846386549,-68.2606847334624,
12.));
#72943=CARTESIAN_POINT('Ctrl Pts',(-29.094628043331,-68.2535957746883,12.));
#72944=CARTESIAN_POINT('Ctrl Pts',(-29.0948791947834,-68.2409993689947,
12.));
#72945=CARTESIAN_POINT('Ctrl Pts',(-29.0952305915108,-68.2229056854495,
12.));
#72946=CARTESIAN_POINT('Ctrl Pts',(-29.0956709104588,-68.1993301411959,
12.));
#72947=CARTESIAN_POINT('Ctrl Pts',(-29.0961590399023,-68.1718618254221,
12.));
#72948=CARTESIAN_POINT('Ctrl Pts',(-29.0966216624741,-68.1444284400734,
12.));
#72949=CARTESIAN_POINT('Ctrl Pts',(-29.0970588175741,-68.1170300647019,
12.));
#72950=CARTESIAN_POINT('Ctrl Pts',(-29.0974705474279,-68.089666782962,12.));
#72951=CARTESIAN_POINT('Ctrl Pts',(-29.0978568968678,-68.0623386822917,
12.));
#72952=CARTESIAN_POINT('Ctrl Pts',(-29.0982179124113,-68.0350458525589,
12.));
#72953=CARTESIAN_POINT('Ctrl Pts',(-29.0985536415537,-68.0077883850136,
12.));
#72954=CARTESIAN_POINT('Ctrl Pts',(-29.0988641320243,-67.9805663711845,
12.));
#72955=CARTESIAN_POINT('Ctrl Pts',(-29.0991494309395,-67.9533799016122,
12.));
#72956=CARTESIAN_POINT('Ctrl Pts',(-29.0994095844208,-67.9262290652797,
12.));
#72957=CARTESIAN_POINT('Ctrl Pts',(-29.0996446380617,-67.8991139503168,
12.));
#72958=CARTESIAN_POINT('Ctrl Pts',(-29.0998546372027,-67.8720346444111,
12.));
#72959=CARTESIAN_POINT('Ctrl Pts',(-29.1000396272868,-67.844991235333,12.));
#72960=CARTESIAN_POINT('Ctrl Pts',(-29.1001996541847,-67.8179838114109,
12.));
#72961=CARTESIAN_POINT('Ctrl Pts',(-29.10033476453,-67.7910124620148,12.));
#72962=CARTESIAN_POINT('Ctrl Pts',(-29.1004450055647,-67.7640772773397,
12.));
#72963=CARTESIAN_POINT('Ctrl Pts',(-29.1005304249989,-67.7371783482038,
12.));
#72964=CARTESIAN_POINT('Ctrl Pts',(-29.1005910708625,-67.7103157658296,
12.));
#72965=CARTESIAN_POINT('Ctrl Pts',(-29.1006269913747,-67.6834896216458,
12.));
#72966=CARTESIAN_POINT('Ctrl Pts',(-29.1006382347812,-67.6567000070319,
12.));
#72967=CARTESIAN_POINT('Ctrl Pts',(-29.1006248493577,-67.6299470133286,
12.));
#72968=CARTESIAN_POINT('Ctrl Pts',(-29.1005868834863,-67.6032307319614,
12.));
#72969=CARTESIAN_POINT('Ctrl Pts',(-29.1005243857137,-67.5765512545276,
12.));
#72970=CARTESIAN_POINT('Ctrl Pts',(-29.1004374048149,-67.5499086728891,
12.));
#72971=CARTESIAN_POINT('Ctrl Pts',(-29.1003259898686,-67.5233030792714,
12.));
#72972=CARTESIAN_POINT('Ctrl Pts',(-29.1001901902915,-67.496734566311,12.));
#72973=CARTESIAN_POINT('Ctrl Pts',(-29.1000300557961,-67.4702032270062,
12.));
#72974=CARTESIAN_POINT('Ctrl Pts',(-29.0998456363687,-67.4437091546869,
12.));
#72975=CARTESIAN_POINT('Ctrl Pts',(-29.0996369822418,-67.4172524429726,
12.));
#72976=CARTESIAN_POINT('Ctrl Pts',(-29.0994041438715,-67.3908331857313,
12.));
#72977=CARTESIAN_POINT('Ctrl Pts',(-29.0991471719172,-67.3644514770373,
12.));
#72978=CARTESIAN_POINT('Ctrl Pts',(-29.0988661172526,-67.3381074112013,
12.));
#72979=CARTESIAN_POINT('Ctrl Pts',(-29.0985610309768,-67.311801082791,12.));
#72980=CARTESIAN_POINT('Ctrl Pts',(-29.0982319644277,-67.2855325866516,
12.));
#72981=CARTESIAN_POINT('Ctrl Pts',(-29.0978789691965,-67.2593020179216,
12.));
#72982=CARTESIAN_POINT('Ctrl Pts',(-29.0975020971474,-67.2331094720482,
12.));
#72983=CARTESIAN_POINT('Ctrl Pts',(-29.0971014004135,-67.2069550447895,
12.));
#72984=CARTESIAN_POINT('Ctrl Pts',(-29.0966769313893,-67.1808388322116,
12.));
#72985=CARTESIAN_POINT('Ctrl Pts',(-29.0962287427274,-67.1547609306845,
12.));
#72986=CARTESIAN_POINT('Ctrl Pts',(-29.0957568873358,-67.1287214368743,
12.));
#72987=CARTESIAN_POINT('Ctrl Pts',(-29.0952614183777,-67.1027204477304,
12.));
#72988=CARTESIAN_POINT('Ctrl Pts',(-29.0947423892725,-67.0767580604872,
12.));
#72989=CARTESIAN_POINT('Ctrl Pts',(-29.0941998536958,-67.0508343726771,
12.));
#72990=CARTESIAN_POINT('Ctrl Pts',(-29.0936338655828,-67.0249494821361,
12.));
#72991=CARTESIAN_POINT('Ctrl Pts',(-29.0930444791329,-66.9991034870084,
12.));
#72992=CARTESIAN_POINT('Ctrl Pts',(-29.092431748817,-66.9732964857467,12.));
#72993=CARTESIAN_POINT('Ctrl Pts',(-29.0917957293824,-66.9475285771133,
12.));
#72994=CARTESIAN_POINT('Ctrl Pts',(-29.0911364758484,-66.9217998601881,
12.));
#72995=CARTESIAN_POINT('Ctrl Pts',(-29.0904540435063,-66.8961104343703,
12.));
#72996=CARTESIAN_POINT('Ctrl Pts',(-29.0897484879208,-66.8704603993794,
12.));
#72997=CARTESIAN_POINT('Ctrl Pts',(-29.0890198649327,-66.8448498552508,
12.));
#72998=CARTESIAN_POINT('Ctrl Pts',(-29.0882682306636,-66.8192789023323,
12.));
#72999=CARTESIAN_POINT('Ctrl Pts',(-29.0874936415138,-66.7937476412941,
12.));
#73000=CARTESIAN_POINT('Ctrl Pts',(-29.086696154163,-66.7682561731348,12.));
#73001=CARTESIAN_POINT('Ctrl Pts',(-29.0858758255729,-66.742804599184,12.));
#73002=CARTESIAN_POINT('Ctrl Pts',(-29.0850327129914,-66.7173930211015,
12.));
#73003=CARTESIAN_POINT('Ctrl Pts',(-29.0841668739585,-66.6920215408744,
12.));
#73004=CARTESIAN_POINT('Ctrl Pts',(-29.0832783663049,-66.6666902608246,
12.));
#73005=CARTESIAN_POINT('Ctrl Pts',(-29.0823672481508,-66.6413992836148,
12.));
#73006=CARTESIAN_POINT('Ctrl Pts',(-29.0814335779086,-66.6161487122504,
12.));
#73007=CARTESIAN_POINT('Ctrl Pts',(-29.0804774142852,-66.5909386500796,
12.));
#73008=CARTESIAN_POINT('Ctrl Pts',(-29.0794988162892,-66.5657692007894,
12.));
#73009=CARTESIAN_POINT('Ctrl Pts',(-29.0784978432294,-66.5406404684116,
12.));
#73010=CARTESIAN_POINT('Ctrl Pts',(-29.0774745547146,-66.5155525573308,
12.));
#73011=CARTESIAN_POINT('Ctrl Pts',(-29.0764290106553,-66.4905055722864,
12.));
#73012=CARTESIAN_POINT('Ctrl Pts',(-29.075361271267,-66.4654996183739,12.));
#73013=CARTESIAN_POINT('Ctrl Pts',(-29.0742713970762,-66.4405348010404,
12.));
#73014=CARTESIAN_POINT('Ctrl Pts',(-29.0731594489219,-66.4156112260904,
12.));
#73015=CARTESIAN_POINT('Ctrl Pts',(-29.0720254879535,-66.3907289996942,
12.));
#73016=CARTESIAN_POINT('Ctrl Pts',(-29.0708695756336,-66.3658882283906,
12.));
#73017=CARTESIAN_POINT('Ctrl Pts',(-29.0696917737398,-66.3410890190879,
12.));
#73018=CARTESIAN_POINT('Ctrl Pts',(-29.0684921443718,-66.3163314790607,
12.));
#73019=CARTESIAN_POINT('Ctrl Pts',(-29.0672707499527,-66.2916157159527,
12.));
#73020=CARTESIAN_POINT('Ctrl Pts',(-29.0660276532272,-66.2669418377865,
12.));
#73021=CARTESIAN_POINT('Ctrl Pts',(-29.0647629172645,-66.2423099529668,
12.));
#73022=CARTESIAN_POINT('Ctrl Pts',(-29.0634766054599,-66.2177201702819,
12.));
#73023=CARTESIAN_POINT('Ctrl Pts',(-29.062168781542,-66.1931725989008,12.));
#73024=CARTESIAN_POINT('Ctrl Pts',(-29.0608395095746,-66.1686673483755,
12.));
#73025=CARTESIAN_POINT('Ctrl Pts',(-29.0594888539556,-66.1442045286516,
12.));
#73026=CARTESIAN_POINT('Ctrl Pts',(-29.058116879419,-66.1197842500711,12.));
#73027=CARTESIAN_POINT('Ctrl Pts',(-29.0567236510374,-66.0954066233754,
12.));
#73028=CARTESIAN_POINT('Ctrl Pts',(-29.0553092342279,-66.0710717597009,
12.));
#73029=CARTESIAN_POINT('Ctrl Pts',(-29.0538736947552,-66.0467797705815,
12.));
#73030=CARTESIAN_POINT('Ctrl Pts',(-29.0524170987307,-66.0225307679591,
12.));
#73031=CARTESIAN_POINT('Ctrl Pts',(-29.0509395126143,-65.9983248641879,
12.));
#73032=CARTESIAN_POINT('Ctrl Pts',(-29.0494410032173,-65.9741621720369,
12.));
#73033=CARTESIAN_POINT('Ctrl Pts',(-29.0479216377081,-65.9500428046868,
12.));
#73034=CARTESIAN_POINT('Ctrl Pts',(-29.0463814836157,-65.9259668757306,
12.));
#73035=CARTESIAN_POINT('Ctrl Pts',(-29.0448206088289,-65.9019344991854,
12.));
#73036=CARTESIAN_POINT('Ctrl Pts',(-29.0432390815978,-65.8779457894961,
12.));
#73037=CARTESIAN_POINT('Ctrl Pts',(-29.0416369705375,-65.854000861539,12.));
#73038=CARTESIAN_POINT('Ctrl Pts',(-29.0400143446338,-65.8300998306191,
12.));
#73039=CARTESIAN_POINT('Ctrl Pts',(-29.0383712732469,-65.8062428124713,
12.));
#73040=CARTESIAN_POINT('Ctrl Pts',(-29.0367078261103,-65.7824299232705,
12.));
#73041=CARTESIAN_POINT('Ctrl Pts',(-29.035024073333,-65.7586612796368,12.));
#73042=CARTESIAN_POINT('Ctrl Pts',(-29.0333200854028,-65.7349369986384,
12.));
#73043=CARTESIAN_POINT('Ctrl Pts',(-29.0315959331919,-65.7112571977891,
12.));
#73044=CARTESIAN_POINT('Ctrl Pts',(-29.0298516879612,-65.6876219950493,
12.));
#73045=CARTESIAN_POINT('Ctrl Pts',(-29.0280874213596,-65.6640315088388,
12.));
#73046=CARTESIAN_POINT('Ctrl Pts',(-29.0263032054266,-65.6404858580403,
12.));
#73047=CARTESIAN_POINT('Ctrl Pts',(-29.0244991125959,-65.6169851620046,
12.));
#73048=CARTESIAN_POINT('Ctrl Pts',(-29.0226752157003,-65.5935295405453,
12.));
#73049=CARTESIAN_POINT('Ctrl Pts',(-29.0208315879764,-65.5701191139418,
12.));
#73050=CARTESIAN_POINT('Ctrl Pts',(-29.0189683030642,-65.5467540029514,
12.));
#73051=CARTESIAN_POINT('Ctrl Pts',(-29.0170854350095,-65.5234343288136,
12.));
#73052=CARTESIAN_POINT('Ctrl Pts',(-29.0151830582675,-65.5001602132535,
12.));
#73053=CARTESIAN_POINT('Ctrl Pts',(-29.013261247709,-65.4769317784789,12.));
#73054=CARTESIAN_POINT('Ctrl Pts',(-29.0113200786239,-65.4537491471828,
12.));
#73055=CARTESIAN_POINT('Ctrl Pts',(-29.0093596267216,-65.4306124425562,
12.));
#73056=CARTESIAN_POINT('Ctrl Pts',(-29.0073799681342,-65.4075217882934,
12.));
#73057=CARTESIAN_POINT('Ctrl Pts',(-29.0053811794207,-65.3844773085961,
12.));
#73058=CARTESIAN_POINT('Ctrl Pts',(-29.003363337573,-65.3614791281692,12.));
#73059=CARTESIAN_POINT('Ctrl Pts',(-29.0013265200185,-65.3385273722241,
12.));
#73060=CARTESIAN_POINT('Ctrl Pts',(-28.9992708046212,-65.3156221664916,
12.));
#73061=CARTESIAN_POINT('Ctrl Pts',(-28.9971962696845,-65.2927636372253,
12.));
#73062=CARTESIAN_POINT('Ctrl Pts',(-28.9951029939557,-65.2699519112064,
12.));
#73063=CARTESIAN_POINT('Ctrl Pts',(-28.9929910566325,-65.2471871157397,
12.));
#73064=CARTESIAN_POINT('Ctrl Pts',(-28.9908605373663,-65.2244693786609,
12.));
#73065=CARTESIAN_POINT('Ctrl Pts',(-28.9887115162634,-65.2017988283479,
12.));
#73066=CARTESIAN_POINT('Ctrl Pts',(-28.9865440738884,-65.1791755937256,
12.));
#73067=CARTESIAN_POINT('Ctrl Pts',(-28.9843582912693,-65.1565998042697,
12.));
#73068=CARTESIAN_POINT('Ctrl Pts',(-28.9821542499043,-65.1340715900028,
12.));
#73069=CARTESIAN_POINT('Ctrl Pts',(-28.9799320317641,-65.1115910815037,
12.));
#73070=CARTESIAN_POINT('Ctrl Pts',(-28.9776917192933,-65.0891584099168,
12.));
#73071=CARTESIAN_POINT('Ctrl Pts',(-28.9754333954135,-65.0667737069563,
12.));
#73072=CARTESIAN_POINT('Ctrl Pts',(-28.9731571435283,-65.0444371049082,
12.));
#73073=CARTESIAN_POINT('Ctrl Pts',(-28.97086304753,-65.022148736628,12.));
#73074=CARTESIAN_POINT('Ctrl Pts',(-28.9685511918018,-64.9999087355504,
12.));
#73075=CARTESIAN_POINT('Ctrl Pts',(-28.9662216612217,-64.9777172357027,
12.));
#73076=CARTESIAN_POINT('Ctrl Pts',(-28.9638745411677,-64.9555743717109,
12.));
#73077=CARTESIAN_POINT('Ctrl Pts',(-28.961509917525,-64.9334802788038,12.));
#73078=CARTESIAN_POINT('Ctrl Pts',(-28.9591278766934,-64.9114350928125,
12.));
#73079=CARTESIAN_POINT('Ctrl Pts',(-28.9567285055867,-64.8894389501801,
12.));
#73080=CARTESIAN_POINT('Ctrl Pts',(-28.9543118916328,-64.8674919879648,
12.));
#73081=CARTESIAN_POINT('Ctrl Pts',(-28.9518781227765,-64.8455943438423,
12.));
#73082=CARTESIAN_POINT('Ctrl Pts',(-28.9494272874832,-64.8237461561018,
12.));
#73083=CARTESIAN_POINT('Ctrl Pts',(-28.9469594747432,-64.8019475636442,
12.));
#73084=CARTESIAN_POINT('Ctrl Pts',(-28.944474774081,-64.7801987060084,12.));
#73085=CARTESIAN_POINT('Ctrl Pts',(-28.9419732755656,-64.758499723388,12.));
#73086=CARTESIAN_POINT('Ctrl Pts',(-28.9394550698204,-64.7368507566467,
12.));
#73087=CARTESIAN_POINT('Ctrl Pts',(-28.9369202480393,-64.715251947329,12.));
#73088=CARTESIAN_POINT('Ctrl Pts',(-28.9343689019882,-64.6937034376617,
12.));
#73089=CARTESIAN_POINT('Ctrl Pts',(-28.9318011239915,-64.672205370541,12.));
#73090=CARTESIAN_POINT('Ctrl Pts',(-28.9292170069222,-64.6507578895161,
12.));
#73091=CARTESIAN_POINT('Ctrl Pts',(-28.9266166441951,-64.629361138774,12.));
#73092=CARTESIAN_POINT('Ctrl Pts',(-28.9240001297542,-64.6080152631039,
12.));
#73093=CARTESIAN_POINT('Ctrl Pts',(-28.9213675580985,-64.5867204079426,
12.));
#73094=CARTESIAN_POINT('Ctrl Pts',(-28.9187190243224,-64.5654767194471,
12.));
#73095=CARTESIAN_POINT('Ctrl Pts',(-28.9160546241538,-64.5442843445559,
12.));
#73096=CARTESIAN_POINT('Ctrl Pts',(-28.9133744539949,-64.523143431047,12.));
#73097=CARTESIAN_POINT('Ctrl Pts',(-28.910678610965,-64.5020541275951,12.));
#73098=CARTESIAN_POINT('Ctrl Pts',(-28.9079671928264,-64.4810165836592,
12.));
#73099=CARTESIAN_POINT('Ctrl Pts',(-28.9052402979062,-64.4600309493583,
12.));
#73100=CARTESIAN_POINT('Ctrl Pts',(-28.9024980250307,-64.4390973753634,
12.));
#73101=CARTESIAN_POINT('Ctrl Pts',(-28.899740473434,-64.4182160127379,12.));
#73102=CARTESIAN_POINT('Ctrl Pts',(-28.8969677427504,-64.3973870129169,
12.));
#73103=CARTESIAN_POINT('Ctrl Pts',(-28.89417993323,-64.3766105280688,12.));
#73104=CARTESIAN_POINT('Ctrl Pts',(-28.8913771459323,-64.3558867114076,
12.));
#73105=CARTESIAN_POINT('Ctrl Pts',(-28.8885594828926,-64.3352157174619,
12.));
#73106=CARTESIAN_POINT('Ctrl Pts',(-28.8857270473959,-64.3145977025037,
12.));
#73107=CARTESIAN_POINT('Ctrl Pts',(-28.882879943794,-64.2940328242521,12.));
#73108=CARTESIAN_POINT('Ctrl Pts',(-28.8800182770065,-64.273521241071,12.));
#73109=CARTESIAN_POINT('Ctrl Pts',(-28.877142152106,-64.2530631112929,12.));
#73110=CARTESIAN_POINT('Ctrl Pts',(-28.8742516738947,-64.2326585925252,
12.));
#73111=CARTESIAN_POINT('Ctrl Pts',(-28.8713469464185,-64.2123078408461,
12.));
#73112=CARTESIAN_POINT('Ctrl Pts',(-28.8684280739014,-64.1920110123299,
12.));
#73113=CARTESIAN_POINT('Ctrl Pts',(-28.8654951618649,-64.1717682648685,
12.));
#73114=CARTESIAN_POINT('Ctrl Pts',(-28.8625483180438,-64.1515797596564,
12.));
#73115=CARTESIAN_POINT('Ctrl Pts',(-28.8595876537148,-64.1314456633381,
12.));
#73116=CARTESIAN_POINT('Ctrl Pts',(-28.8566132838179,-64.1113661481965,
12.));
#73117=CARTESIAN_POINT('Ctrl Pts',(-28.8536253241854,-64.0913413876622,
12.));
#73118=CARTESIAN_POINT('Ctrl Pts',(-28.8506238891093,-64.0713715523599,
12.));
#73119=CARTESIAN_POINT('Ctrl Pts',(-28.8476090892232,-64.0514568066637,
12.));
#73120=CARTESIAN_POINT('Ctrl Pts',(-28.844581028125,-64.0315973031942,12.));
#73121=CARTESIAN_POINT('Ctrl Pts',(-28.8415398056428,-64.0117931881298,
12.));
#73122=CARTESIAN_POINT('Ctrl Pts',(-28.8384855243243,-63.9920446117582,
12.));
#73123=CARTESIAN_POINT('Ctrl Pts',(-28.8354182946601,-63.9723517369614,
12.));
#73124=CARTESIAN_POINT('Ctrl Pts',(-28.8323382413789,-63.9527147494423,
12.));
#73125=CARTESIAN_POINT('Ctrl Pts',(-28.8292455077559,-63.9331338646996,
12.));
#73126=CARTESIAN_POINT('Ctrl Pts',(-28.8261402423291,-63.9136093063786,
12.));
#73127=CARTESIAN_POINT('Ctrl Pts',(-28.823022586318,-63.8941412856923,12.));
#73128=CARTESIAN_POINT('Ctrl Pts',(-28.8198926619858,-63.8747299825313,
12.));
#73129=CARTESIAN_POINT('Ctrl Pts',(-28.8167505576681,-63.8553755207486,
12.));
#73130=CARTESIAN_POINT('Ctrl Pts',(-28.8135963263369,-63.8360779669856,
12.));
#73131=CARTESIAN_POINT('Ctrl Pts',(-28.8110632620958,-63.8206854735027,
12.));
#73132=CARTESIAN_POINT('Ctrl Pts',(-28.8091580239553,-63.8091667271231,
12.));
#73133=CARTESIAN_POINT('Ctrl Pts',(-28.8078854475432,-63.8014989507494,
12.));
#73134=CARTESIAN_POINT('Ctrl Pts',(-28.8072485549237,-63.7976679095314,
12.));
#73135=CARTESIAN_POINT('Ctrl Pts',(-27.6958230985045,-68.8415926175086,
-5.55111512312578E-16));
#73136=CARTESIAN_POINT('Ctrl Pts',(-27.6958230985045,-68.8415926175086,
4.));
#73137=CARTESIAN_POINT('Ctrl Pts',(-27.6958230985045,-68.8415926175086,
8.));
#73138=CARTESIAN_POINT('Ctrl Pts',(-27.6958230985045,-68.8415926175086,
12.));
#73139=CARTESIAN_POINT('Ctrl Pts',(-27.7750822307004,-68.9176987693915,
-5.55111512312578E-16));
#73140=CARTESIAN_POINT('Ctrl Pts',(-27.7750822307004,-68.9176987693915,
3.99999999999999));
#73141=CARTESIAN_POINT('Ctrl Pts',(-27.7750822307004,-68.9176987693915,
8.));
#73142=CARTESIAN_POINT('Ctrl Pts',(-27.7750822307004,-68.9176987693915,
12.));
#73143=CARTESIAN_POINT('Ctrl Pts',(-27.9589320265198,-69.0029745467578,
-5.55111512312578E-16));
#73144=CARTESIAN_POINT('Ctrl Pts',(-27.9589320265198,-69.0029745467578,
4.00000000000001));
#73145=CARTESIAN_POINT('Ctrl Pts',(-27.9589320265198,-69.0029745467578,
7.99999999999999));
#73146=CARTESIAN_POINT('Ctrl Pts',(-27.9589320265198,-69.0029745467578,
12.));
#73147=CARTESIAN_POINT('Ctrl Pts',(-28.155338613888,-68.9748773050757,-5.55111512312578E-16));
#73148=CARTESIAN_POINT('Ctrl Pts',(-28.155338613888,-68.9748773050757,3.99999999999999));
#73149=CARTESIAN_POINT('Ctrl Pts',(-28.155338613888,-68.9748773050757,8.00000000000001));
#73150=CARTESIAN_POINT('Ctrl Pts',(-28.155338613888,-68.9748773050757,12.));
#73151=CARTESIAN_POINT('Ctrl Pts',(-28.231604030224,-68.9436475237611,-5.55111512312578E-16));
#73152=CARTESIAN_POINT('Ctrl Pts',(-28.231604030224,-68.9436475237611,4.));
#73153=CARTESIAN_POINT('Ctrl Pts',(-28.231604030224,-68.9436475237611,8.));
#73154=CARTESIAN_POINT('Ctrl Pts',(-28.231604030224,-68.9436475237611,12.));
#73155=CARTESIAN_POINT('',(-27.6958230985045,-68.8415926175086,-2.77555756156289E-16));
#73156=CARTESIAN_POINT('',(-28.2316040302241,-68.9436475237613,2.77555756156289E-16));
#73157=CARTESIAN_POINT('Ctrl Pts',(-27.6958230985045,-68.8415926175086,
-5.55111512312578E-16));
#73158=CARTESIAN_POINT('Ctrl Pts',(-27.7750822307004,-68.9176987693915,
-5.55111512312578E-16));
#73159=CARTESIAN_POINT('Ctrl Pts',(-27.8801392568829,-68.9664277850294,
-5.55111512312578E-16));
#73160=CARTESIAN_POINT('Ctrl Pts',(-27.9892964598977,-68.9781370393453,
-5.55111512312578E-16));
#73161=CARTESIAN_POINT('Ctrl Pts',(-28.0711643621588,-68.9869189800823,
-5.55111512312578E-16));
#73162=CARTESIAN_POINT('Ctrl Pts',(-28.155338613888,-68.9748773050757,-5.55111512312578E-16));
#73163=CARTESIAN_POINT('Ctrl Pts',(-28.231604030224,-68.9436475237611,-5.55111512312578E-16));
#73164=CARTESIAN_POINT('',(-28.2316040302241,-68.9436475237613,12.));
#73165=CARTESIAN_POINT('Ctrl Pts',(-28.231604030224,-68.9436475237611,-5.55111512312578E-16));
#73166=CARTESIAN_POINT('Ctrl Pts',(-28.231604030224,-68.9436475237611,4.));
#73167=CARTESIAN_POINT('Ctrl Pts',(-28.231604030224,-68.9436475237611,8.));
#73168=CARTESIAN_POINT('Ctrl Pts',(-28.231604030224,-68.9436475237611,12.));
#73169=CARTESIAN_POINT('',(-27.6958230985045,-68.8415926175086,12.));
#73170=CARTESIAN_POINT('Ctrl Pts',(-28.231604030224,-68.9436475237611,12.));
#73171=CARTESIAN_POINT('Ctrl Pts',(-28.155338613888,-68.9748773050757,12.));
#73172=CARTESIAN_POINT('Ctrl Pts',(-28.0711643621588,-68.9869189800823,
12.));
#73173=CARTESIAN_POINT('Ctrl Pts',(-27.9892964598977,-68.9781370393453,
12.));
#73174=CARTESIAN_POINT('Ctrl Pts',(-27.8801392568829,-68.9664277850294,
12.));
#73175=CARTESIAN_POINT('Ctrl Pts',(-27.7750822307004,-68.9176987693915,
12.));
#73176=CARTESIAN_POINT('Ctrl Pts',(-27.6958230985045,-68.8415926175086,
12.));
#73177=CARTESIAN_POINT('Ctrl Pts',(-27.6958230985045,-68.8415926175086,
12.));
#73178=CARTESIAN_POINT('Ctrl Pts',(-27.6958230985045,-68.8415926175086,
8.));
#73179=CARTESIAN_POINT('Ctrl Pts',(-27.6958230985045,-68.8415926175086,
4.));
#73180=CARTESIAN_POINT('Ctrl Pts',(-27.6958230985045,-68.8415926175086,
-5.55111512312578E-16));
#73181=CARTESIAN_POINT('Origin',(-1.43354795624835E-10,-3.4634846687719E-10,
0.));
#73182=CARTESIAN_POINT('Origin',(-1.43354795624835E-10,-3.4634846687719E-10,
12.));
#73183=CARTESIAN_POINT('Origin',(-1.43354795624835E-10,-3.4634846687719E-10,
0.));
#73184=CARTESIAN_POINT('Ctrl Pts',(-34.6669728017237,-65.9427857825597,
-5.55111512312578E-16));
#73185=CARTESIAN_POINT('Ctrl Pts',(-34.6669728017237,-65.9427857825597,
4.));
#73186=CARTESIAN_POINT('Ctrl Pts',(-34.6669728017237,-65.9427857825597,
8.));
#73187=CARTESIAN_POINT('Ctrl Pts',(-34.6669728017237,-65.9427857825597,
12.));
#73188=CARTESIAN_POINT('Ctrl Pts',(-34.7642339552035,-65.8916543400169,
-5.55111512312578E-16));
#73189=CARTESIAN_POINT('Ctrl Pts',(-34.7642339552035,-65.8916543400169,
4.));
#73190=CARTESIAN_POINT('Ctrl Pts',(-34.7642339552036,-65.8916543400169,
8.));
#73191=CARTESIAN_POINT('Ctrl Pts',(-34.7642339552036,-65.8916543400169,
12.));
#73192=CARTESIAN_POINT('Ctrl Pts',(-34.9032616822024,-65.7441961270804,
-5.55111512312578E-16));
#73193=CARTESIAN_POINT('Ctrl Pts',(-34.9032616822024,-65.7441961270804,
4.));
#73194=CARTESIAN_POINT('Ctrl Pts',(-34.9032616822024,-65.7441961270804,
8.));
#73195=CARTESIAN_POINT('Ctrl Pts',(-34.9032616822024,-65.7441961270804,
12.));
#73196=CARTESIAN_POINT('Ctrl Pts',(-34.9387029822717,-65.5489812297286,
-5.55111512312578E-16));
#73197=CARTESIAN_POINT('Ctrl Pts',(-34.9387029822717,-65.5489812297286,
4.));
#73198=CARTESIAN_POINT('Ctrl Pts',(-34.9387029822717,-65.5489812297286,
8.));
#73199=CARTESIAN_POINT('Ctrl Pts',(-34.9387029822717,-65.5489812297286,
12.));
#73200=CARTESIAN_POINT('Ctrl Pts',(-34.9331875523087,-65.4667541477954,
-5.55111512312578E-16));
#73201=CARTESIAN_POINT('Ctrl Pts',(-34.9331875523087,-65.4667541477954,
4.));
#73202=CARTESIAN_POINT('Ctrl Pts',(-34.9331875523087,-65.4667541477954,
8.));
#73203=CARTESIAN_POINT('Ctrl Pts',(-34.9331875523087,-65.4667541477954,
12.));
#73204=CARTESIAN_POINT('',(-34.6669728017237,-65.9427857825597,0.));
#73205=CARTESIAN_POINT('',(-34.9331875523085,-65.4667541477955,2.77555756156289E-16));
#73206=CARTESIAN_POINT('Ctrl Pts',(-34.6669728017237,-65.9427857825597,
-1.38777878078145E-16));
#73207=CARTESIAN_POINT('Ctrl Pts',(-34.7642339552035,-65.8916543400169,
-1.38777878078145E-16));
#73208=CARTESIAN_POINT('Ctrl Pts',(-34.8436783706315,-65.8073925040532,
-1.38777878078144E-16));
#73209=CARTESIAN_POINT('Ctrl Pts',(-34.8892986466538,-65.7075366486885,
-1.38777878078145E-16));
#73210=CARTESIAN_POINT('Ctrl Pts',(-34.9235138536706,-65.6326447571651,
-1.38777878078145E-16));
#73211=CARTESIAN_POINT('Ctrl Pts',(-34.9387029822717,-65.5489812297286,
-1.38777878078145E-16));
#73212=CARTESIAN_POINT('Ctrl Pts',(-34.9331875523087,-65.4667541477954,
-1.38777878078145E-16));
#73213=CARTESIAN_POINT('',(-34.9331875523085,-65.4667541477955,12.));
#73214=CARTESIAN_POINT('Ctrl Pts',(-34.9331875523087,-65.4667541477954,
-5.55111512312578E-16));
#73215=CARTESIAN_POINT('Ctrl Pts',(-34.9331875523087,-65.4667541477954,
4.));
#73216=CARTESIAN_POINT('Ctrl Pts',(-34.9331875523087,-65.4667541477954,
8.));
#73217=CARTESIAN_POINT('Ctrl Pts',(-34.9331875523087,-65.4667541477954,
12.));
#73218=CARTESIAN_POINT('',(-34.6669728017237,-65.9427857825597,12.));
#73219=CARTESIAN_POINT('Ctrl Pts',(-34.9331875523087,-65.4667541477954,
12.));
#73220=CARTESIAN_POINT('Ctrl Pts',(-34.9387029822717,-65.5489812297286,
12.));
#73221=CARTESIAN_POINT('Ctrl Pts',(-34.9235138536706,-65.6326447571651,
12.));
#73222=CARTESIAN_POINT('Ctrl Pts',(-34.8892986466538,-65.7075366486885,
12.));
#73223=CARTESIAN_POINT('Ctrl Pts',(-34.8436783706315,-65.8073925040532,
12.));
#73224=CARTESIAN_POINT('Ctrl Pts',(-34.7642339552036,-65.8916543400169,
12.));
#73225=CARTESIAN_POINT('Ctrl Pts',(-34.6669728017237,-65.9427857825597,
12.));
#73226=CARTESIAN_POINT('Ctrl Pts',(-34.6669728017237,-65.9427857825597,
12.));
#73227=CARTESIAN_POINT('Ctrl Pts',(-34.6669728017237,-65.9427857825597,
8.));
#73228=CARTESIAN_POINT('Ctrl Pts',(-34.6669728017237,-65.9427857825597,
4.));
#73229=CARTESIAN_POINT('Ctrl Pts',(-34.6669728017237,-65.9427857825597,
-5.55111512312578E-16));
#73230=CARTESIAN_POINT('Ctrl Pts',(-34.2579614092497,-61.0441813777723,
0.));
#73231=CARTESIAN_POINT('Ctrl Pts',(-34.2579614092497,-61.0441813777723,
12.));
#73232=CARTESIAN_POINT('Ctrl Pts',(-34.2589297755434,-61.0479423318725,
0.));
#73233=CARTESIAN_POINT('Ctrl Pts',(-34.2589297755434,-61.0479423318725,
12.));
#73234=CARTESIAN_POINT('Ctrl Pts',(-34.2608658001631,-61.0554700176998,
0.));
#73235=CARTESIAN_POINT('Ctrl Pts',(-34.2608658001631,-61.0554700176998,
12.));
#73236=CARTESIAN_POINT('Ctrl Pts',(-34.2637677131935,-61.0667788793266,
0.));
#73237=CARTESIAN_POINT('Ctrl Pts',(-34.2637677131935,-61.0667788793266,
12.));
#73238=CARTESIAN_POINT('Ctrl Pts',(-34.2676326825626,-61.0818920286293,
0.));
#73239=CARTESIAN_POINT('Ctrl Pts',(-34.2676326825626,-61.0818920286293,
12.));
#73240=CARTESIAN_POINT('Ctrl Pts',(-34.2724568037228,-61.1008412399997,
0.));
#73241=CARTESIAN_POINT('Ctrl Pts',(-34.2724568037228,-61.1008412399997,
12.));
#73242=CARTESIAN_POINT('Ctrl Pts',(-34.2772738038771,-61.1198481997764,
0.));
#73243=CARTESIAN_POINT('Ctrl Pts',(-34.2772738038771,-61.1198481997764,
12.));
#73244=CARTESIAN_POINT('Ctrl Pts',(-34.282083624447,-61.1389128461885,0.));
#73245=CARTESIAN_POINT('Ctrl Pts',(-34.282083624447,-61.1389128461885,12.));
#73246=CARTESIAN_POINT('Ctrl Pts',(-34.2868861666384,-61.1580350635532,
0.));
#73247=CARTESIAN_POINT('Ctrl Pts',(-34.2868861666384,-61.1580350635532,
12.));
#73248=CARTESIAN_POINT('Ctrl Pts',(-34.2916812929751,-61.1772146833205,
0.));
#73249=CARTESIAN_POINT('Ctrl Pts',(-34.2916812929751,-61.1772146833205,
12.));
#73250=CARTESIAN_POINT('Ctrl Pts',(-34.2964688443663,-61.1964515073891,
0.));
#73251=CARTESIAN_POINT('Ctrl Pts',(-34.2964688443663,-61.1964515073891,
12.));
#73252=CARTESIAN_POINT('Ctrl Pts',(-34.3012486533474,-61.2157453259107,
0.));
#73253=CARTESIAN_POINT('Ctrl Pts',(-34.3012486533474,-61.2157453259107,
12.));
#73254=CARTESIAN_POINT('Ctrl Pts',(-34.3060205584065,-61.2350959366939,
0.));
#73255=CARTESIAN_POINT('Ctrl Pts',(-34.3060205584065,-61.2350959366939,
12.));
#73256=CARTESIAN_POINT('Ctrl Pts',(-34.3107844191044,-61.2545031656133,
0.));
#73257=CARTESIAN_POINT('Ctrl Pts',(-34.3107844191044,-61.2545031656133,
12.));
#73258=CARTESIAN_POINT('Ctrl Pts',(-34.3155401111747,-61.2739668600365,
0.));
#73259=CARTESIAN_POINT('Ctrl Pts',(-34.3155401111747,-61.2739668600365,
12.));
#73260=CARTESIAN_POINT('Ctrl Pts',(-34.3202875193618,-61.2934868791854,
0.));
#73261=CARTESIAN_POINT('Ctrl Pts',(-34.3202875193618,-61.2934868791854,
12.));
#73262=CARTESIAN_POINT('Ctrl Pts',(-34.3250265314768,-61.3130630861386,
0.));
#73263=CARTESIAN_POINT('Ctrl Pts',(-34.3250265314768,-61.3130630861386,
12.));
#73264=CARTESIAN_POINT('Ctrl Pts',(-34.3297570310146,-61.3326953378851,
0.));
#73265=CARTESIAN_POINT('Ctrl Pts',(-34.3297570310146,-61.3326953378851,
12.));
#73266=CARTESIAN_POINT('Ctrl Pts',(-34.3344788934363,-61.3523834803188,
0.));
#73267=CARTESIAN_POINT('Ctrl Pts',(-34.3344788934363,-61.3523834803188,
12.));
#73268=CARTESIAN_POINT('Ctrl Pts',(-34.339191990014,-61.3721273534256,0.));
#73269=CARTESIAN_POINT('Ctrl Pts',(-34.339191990014,-61.3721273534256,12.));
#73270=CARTESIAN_POINT('Ctrl Pts',(-34.3438961902405,-61.3919267945302,
0.));
#73271=CARTESIAN_POINT('Ctrl Pts',(-34.3438961902405,-61.3919267945302,
12.));
#73272=CARTESIAN_POINT('Ctrl Pts',(-34.3485913645979,-61.4117816420228,
0.));
#73273=CARTESIAN_POINT('Ctrl Pts',(-34.3485913645979,-61.4117816420228,
12.));
#73274=CARTESIAN_POINT('Ctrl Pts',(-34.3532773877089,-61.4316917395918,
0.));
#73275=CARTESIAN_POINT('Ctrl Pts',(-34.3532773877089,-61.4316917395918,
12.));
#73276=CARTESIAN_POINT('Ctrl Pts',(-34.3579541381996,-61.4516569360454,
0.));
#73277=CARTESIAN_POINT('Ctrl Pts',(-34.3579541381996,-61.4516569360454,
12.));
#73278=CARTESIAN_POINT('Ctrl Pts',(-34.3626214971889,-61.4716770832896,
0.));
#73279=CARTESIAN_POINT('Ctrl Pts',(-34.3626214971889,-61.4716770832896,
12.));
#73280=CARTESIAN_POINT('Ctrl Pts',(-34.3672793472466,-61.4917520349278,
0.));
#73281=CARTESIAN_POINT('Ctrl Pts',(-34.3672793472466,-61.4917520349278,
12.));
#73282=CARTESIAN_POINT('Ctrl Pts',(-34.3719275711195,-61.5118816445437,
0.));
#73283=CARTESIAN_POINT('Ctrl Pts',(-34.3719275711195,-61.5118816445437,
12.));
#73284=CARTESIAN_POINT('Ctrl Pts',(-34.376566050668,-61.5320657642638,0.));
#73285=CARTESIAN_POINT('Ctrl Pts',(-34.376566050668,-61.5320657642638,12.));
#73286=CARTESIAN_POINT('Ctrl Pts',(-34.3811946674197,-61.5523042455158,
0.));
#73287=CARTESIAN_POINT('Ctrl Pts',(-34.3811946674197,-61.5523042455158,
12.));
#73288=CARTESIAN_POINT('Ctrl Pts',(-34.3858133030518,-61.5725969396829,
0.));
#73289=CARTESIAN_POINT('Ctrl Pts',(-34.3858133030518,-61.5725969396829,
12.));
#73290=CARTESIAN_POINT('Ctrl Pts',(-34.3904218398637,-61.5929436987409,
0.));
#73291=CARTESIAN_POINT('Ctrl Pts',(-34.3904218398637,-61.5929436987409,
12.));
#73292=CARTESIAN_POINT('Ctrl Pts',(-34.3950201613432,-61.6133443760142,
0.));
#73293=CARTESIAN_POINT('Ctrl Pts',(-34.3950201613432,-61.6133443760142,
12.));
#73294=CARTESIAN_POINT('Ctrl Pts',(-34.3996081523753,-61.6337988264556,
0.));
#73295=CARTESIAN_POINT('Ctrl Pts',(-34.3996081523753,-61.6337988264556,
12.));
#73296=CARTESIAN_POINT('Ctrl Pts',(-34.4041856989317,-61.6543069062416,
0.));
#73297=CARTESIAN_POINT('Ctrl Pts',(-34.4041856989317,-61.6543069062416,
12.));
#73298=CARTESIAN_POINT('Ctrl Pts',(-34.4087526878812,-61.6748684725205,
0.));
#73299=CARTESIAN_POINT('Ctrl Pts',(-34.4087526878812,-61.6748684725205,
12.));
#73300=CARTESIAN_POINT('Ctrl Pts',(-34.4133090067704,-61.695483383117,0.));
#73301=CARTESIAN_POINT('Ctrl Pts',(-34.4133090067704,-61.695483383117,12.));
#73302=CARTESIAN_POINT('Ctrl Pts',(-34.4178545435767,-61.7161514961914,
0.));
#73303=CARTESIAN_POINT('Ctrl Pts',(-34.4178545435767,-61.7161514961914,
12.));
#73304=CARTESIAN_POINT('Ctrl Pts',(-34.422389186718,-61.7368726702596,0.));
#73305=CARTESIAN_POINT('Ctrl Pts',(-34.422389186718,-61.7368726702596,12.));
#73306=CARTESIAN_POINT('Ctrl Pts',(-34.4269128251577,-61.7576467643432,
0.));
#73307=CARTESIAN_POINT('Ctrl Pts',(-34.4269128251577,-61.7576467643432,
12.));
#73308=CARTESIAN_POINT('Ctrl Pts',(-34.4314253484792,-61.7784736380727,
0.));
#73309=CARTESIAN_POINT('Ctrl Pts',(-34.4314253484792,-61.7784736380727,
12.));
#73310=CARTESIAN_POINT('Ctrl Pts',(-34.4359266469749,-61.7993531518036,
0.));
#73311=CARTESIAN_POINT('Ctrl Pts',(-34.4359266469749,-61.7993531518036,
12.));
#73312=CARTESIAN_POINT('Ctrl Pts',(-34.4404166117299,-61.8202851667222,
0.));
#73313=CARTESIAN_POINT('Ctrl Pts',(-34.4404166117299,-61.8202851667222,
12.));
#73314=CARTESIAN_POINT('Ctrl Pts',(-34.444895134574,-61.8412695447926,0.));
#73315=CARTESIAN_POINT('Ctrl Pts',(-34.444895134574,-61.8412695447926,12.));
#73316=CARTESIAN_POINT('Ctrl Pts',(-34.4493621080361,-61.8623061487018,
0.));
#73317=CARTESIAN_POINT('Ctrl Pts',(-34.4493621080361,-61.8623061487018,
12.));
#73318=CARTESIAN_POINT('Ctrl Pts',(-34.4538174253012,-61.8833948418025,
0.));
#73319=CARTESIAN_POINT('Ctrl Pts',(-34.4538174253012,-61.8833948418025,
12.));
#73320=CARTESIAN_POINT('Ctrl Pts',(-34.4582609801637,-61.9045354880444,
0.));
#73321=CARTESIAN_POINT('Ctrl Pts',(-34.4582609801637,-61.9045354880444,
12.));
#73322=CARTESIAN_POINT('Ctrl Pts',(-34.4626926669975,-61.9257279519308,
0.));
#73323=CARTESIAN_POINT('Ctrl Pts',(-34.4626926669975,-61.9257279519308,
12.));
#73324=CARTESIAN_POINT('Ctrl Pts',(-34.4671123807717,-61.9469720985531,
0.));
#73325=CARTESIAN_POINT('Ctrl Pts',(-34.4671123807717,-61.9469720985531,
12.));
#73326=CARTESIAN_POINT('Ctrl Pts',(-34.4715200170592,-61.9682677936053,
0.));
#73327=CARTESIAN_POINT('Ctrl Pts',(-34.4715200170592,-61.9682677936053,
12.));
#73328=CARTESIAN_POINT('Ctrl Pts',(-34.4759154720473,-61.9896149034001,
0.));
#73329=CARTESIAN_POINT('Ctrl Pts',(-34.4759154720473,-61.9896149034001,
12.));
#73330=CARTESIAN_POINT('Ctrl Pts',(-34.4802986425528,-62.0110132948794,
0.));
#73331=CARTESIAN_POINT('Ctrl Pts',(-34.4802986425528,-62.0110132948794,
12.));
#73332=CARTESIAN_POINT('Ctrl Pts',(-34.48466942602,-62.0324628356141,0.));
#73333=CARTESIAN_POINT('Ctrl Pts',(-34.48466942602,-62.0324628356141,12.));
#73334=CARTESIAN_POINT('Ctrl Pts',(-34.489027720504,-62.0539633937939,0.));
#73335=CARTESIAN_POINT('Ctrl Pts',(-34.489027720504,-62.0539633937939,12.));
#73336=CARTESIAN_POINT('Ctrl Pts',(-34.4933734246593,-62.0755148382135,
0.));
#73337=CARTESIAN_POINT('Ctrl Pts',(-34.4933734246593,-62.0755148382135,
12.));
#73338=CARTESIAN_POINT('Ctrl Pts',(-34.4977064377282,-62.0971170382567,
0.));
#73339=CARTESIAN_POINT('Ctrl Pts',(-34.4977064377282,-62.0971170382567,
12.));
#73340=CARTESIAN_POINT('Ctrl Pts',(-34.5020266595293,-62.1187698638707,
0.));
#73341=CARTESIAN_POINT('Ctrl Pts',(-34.5020266595293,-62.1187698638707,
12.));
#73342=CARTESIAN_POINT('Ctrl Pts',(-34.5063339904533,-62.1404731855687,
0.));
#73343=CARTESIAN_POINT('Ctrl Pts',(-34.5063339904533,-62.1404731855687,
12.));
#73344=CARTESIAN_POINT('Ctrl Pts',(-34.5106283314594,-62.1622268744337,
0.));
#73345=CARTESIAN_POINT('Ctrl Pts',(-34.5106283314594,-62.1622268744337,
12.));
#73346=CARTESIAN_POINT('Ctrl Pts',(-34.514909584073,-62.184030802117,0.));
#73347=CARTESIAN_POINT('Ctrl Pts',(-34.514909584073,-62.184030802117,12.));
#73348=CARTESIAN_POINT('Ctrl Pts',(-34.5191776503843,-62.2058848408346,
0.));
#73349=CARTESIAN_POINT('Ctrl Pts',(-34.5191776503843,-62.2058848408346,
12.));
#73350=CARTESIAN_POINT('Ctrl Pts',(-34.5234324330492,-62.2277888633576,
0.));
#73351=CARTESIAN_POINT('Ctrl Pts',(-34.5234324330492,-62.2277888633576,
12.));
#73352=CARTESIAN_POINT('Ctrl Pts',(-34.527673835281,-62.2497427430136,0.));
#73353=CARTESIAN_POINT('Ctrl Pts',(-34.527673835281,-62.2497427430136,12.));
#73354=CARTESIAN_POINT('Ctrl Pts',(-34.5319017608435,-62.2717463536828,
0.));
#73355=CARTESIAN_POINT('Ctrl Pts',(-34.5319017608435,-62.2717463536828,
12.));
#73356=CARTESIAN_POINT('Ctrl Pts',(-34.536116114045,-62.2937995697927,0.));
#73357=CARTESIAN_POINT('Ctrl Pts',(-34.536116114045,-62.2937995697927,12.));
#73358=CARTESIAN_POINT('Ctrl Pts',(-34.5403167997333,-62.3159022663052,
0.));
#73359=CARTESIAN_POINT('Ctrl Pts',(-34.5403167997333,-62.3159022663052,
12.));
#73360=CARTESIAN_POINT('Ctrl Pts',(-34.5445037232928,-62.3380543187067,
0.));
#73361=CARTESIAN_POINT('Ctrl Pts',(-34.5445037232928,-62.3380543187067,
12.));
#73362=CARTESIAN_POINT('Ctrl Pts',(-34.5486767906376,-62.3602556030114,
0.));
#73363=CARTESIAN_POINT('Ctrl Pts',(-34.5486767906376,-62.3602556030114,
12.));
#73364=CARTESIAN_POINT('Ctrl Pts',(-34.552835908207,-62.3825059957593,0.));
#73365=CARTESIAN_POINT('Ctrl Pts',(-34.552835908207,-62.3825059957593,12.));
#73366=CARTESIAN_POINT('Ctrl Pts',(-34.5569809829615,-62.4048053740129,
0.));
#73367=CARTESIAN_POINT('Ctrl Pts',(-34.5569809829615,-62.4048053740129,
12.));
#73368=CARTESIAN_POINT('Ctrl Pts',(-34.5611119223807,-62.4271536153473,
0.));
#73369=CARTESIAN_POINT('Ctrl Pts',(-34.5611119223807,-62.4271536153473,
12.));
#73370=CARTESIAN_POINT('Ctrl Pts',(-34.5652286344606,-62.4495505978415,
0.));
#73371=CARTESIAN_POINT('Ctrl Pts',(-34.5652286344606,-62.4495505978415,
12.));
#73372=CARTESIAN_POINT('Ctrl Pts',(-34.5693310277064,-62.4719962000829,
0.));
#73373=CARTESIAN_POINT('Ctrl Pts',(-34.5693310277064,-62.4719962000829,
12.));
#73374=CARTESIAN_POINT('Ctrl Pts',(-34.5734190111279,-62.494490301164,0.));
#73375=CARTESIAN_POINT('Ctrl Pts',(-34.5734190111279,-62.494490301164,12.));
#73376=CARTESIAN_POINT('Ctrl Pts',(-34.5774924942351,-62.5170327806774,
0.));
#73377=CARTESIAN_POINT('Ctrl Pts',(-34.5774924942351,-62.5170327806774,
12.));
#73378=CARTESIAN_POINT('Ctrl Pts',(-34.5815513870363,-62.5396235187053,
0.));
#73379=CARTESIAN_POINT('Ctrl Pts',(-34.5815513870363,-62.5396235187053,
12.));
#73380=CARTESIAN_POINT('Ctrl Pts',(-34.5855956000344,-62.5622623958125,
0.));
#73381=CARTESIAN_POINT('Ctrl Pts',(-34.5855956000344,-62.5622623958125,
12.));
#73382=CARTESIAN_POINT('Ctrl Pts',(-34.5896250442199,-62.5849492930501,
0.));
#73383=CARTESIAN_POINT('Ctrl Pts',(-34.5896250442199,-62.5849492930501,
12.));
#73384=CARTESIAN_POINT('Ctrl Pts',(-34.5936396310671,-62.6076840919521,
0.));
#73385=CARTESIAN_POINT('Ctrl Pts',(-34.5936396310671,-62.6076840919521,
12.));
#73386=CARTESIAN_POINT('Ctrl Pts',(-34.5976392725303,-62.6304666745319,
0.));
#73387=CARTESIAN_POINT('Ctrl Pts',(-34.5976392725303,-62.6304666745319,
12.));
#73388=CARTESIAN_POINT('Ctrl Pts',(-34.6016238810419,-62.6532969232695,
0.));
#73389=CARTESIAN_POINT('Ctrl Pts',(-34.6016238810419,-62.6532969232695,
12.));
#73390=CARTESIAN_POINT('Ctrl Pts',(-34.6055933695093,-62.6761747211081,
0.));
#73391=CARTESIAN_POINT('Ctrl Pts',(-34.6055933695093,-62.6761747211081,
12.));
#73392=CARTESIAN_POINT('Ctrl Pts',(-34.6095476513095,-62.6990999514597,
0.));
#73393=CARTESIAN_POINT('Ctrl Pts',(-34.6095476513095,-62.6990999514597,
12.));
#73394=CARTESIAN_POINT('Ctrl Pts',(-34.6134866402842,-62.7220724982005,
0.));
#73395=CARTESIAN_POINT('Ctrl Pts',(-34.6134866402842,-62.7220724982005,
12.));
#73396=CARTESIAN_POINT('Ctrl Pts',(-34.6174102507368,-62.7450922456662,
0.));
#73397=CARTESIAN_POINT('Ctrl Pts',(-34.6174102507368,-62.7450922456662,
12.));
#73398=CARTESIAN_POINT('Ctrl Pts',(-34.6213183974303,-62.7681590786398,
0.));
#73399=CARTESIAN_POINT('Ctrl Pts',(-34.6213183974303,-62.7681590786398,
12.));
#73400=CARTESIAN_POINT('Ctrl Pts',(-34.6252109955836,-62.7912728823482,
0.));
#73401=CARTESIAN_POINT('Ctrl Pts',(-34.6252109955836,-62.7912728823482,
12.));
#73402=CARTESIAN_POINT('Ctrl Pts',(-34.629087960866,-62.8144335424671,0.));
#73403=CARTESIAN_POINT('Ctrl Pts',(-34.629087960866,-62.8144335424671,12.));
#73404=CARTESIAN_POINT('Ctrl Pts',(-34.6329492093932,-62.8376409451167,
0.));
#73405=CARTESIAN_POINT('Ctrl Pts',(-34.6329492093932,-62.8376409451167,
12.));
#73406=CARTESIAN_POINT('Ctrl Pts',(-34.6367946577241,-62.8608949768583,
0.));
#73407=CARTESIAN_POINT('Ctrl Pts',(-34.6367946577241,-62.8608949768583,
12.));
#73408=CARTESIAN_POINT('Ctrl Pts',(-34.6406242228606,-62.8841955246819,
0.));
#73409=CARTESIAN_POINT('Ctrl Pts',(-34.6406242228606,-62.8841955246819,
12.));
#73410=CARTESIAN_POINT('Ctrl Pts',(-34.6444378222425,-62.9075424760042,
0.));
#73411=CARTESIAN_POINT('Ctrl Pts',(-34.6444378222425,-62.9075424760042,
12.));
#73412=CARTESIAN_POINT('Ctrl Pts',(-34.6482353737434,-62.9309357186733,
0.));
#73413=CARTESIAN_POINT('Ctrl Pts',(-34.6482353737434,-62.9309357186733,
12.));
#73414=CARTESIAN_POINT('Ctrl Pts',(-34.6520167956657,-62.9543751409647,
0.));
#73415=CARTESIAN_POINT('Ctrl Pts',(-34.6520167956657,-62.9543751409647,
12.));
#73416=CARTESIAN_POINT('Ctrl Pts',(-34.655782006739,-62.9778606315777,0.));
#73417=CARTESIAN_POINT('Ctrl Pts',(-34.655782006739,-62.9778606315777,12.));
#73418=CARTESIAN_POINT('Ctrl Pts',(-34.6595309261186,-63.0013920796225,
0.));
#73419=CARTESIAN_POINT('Ctrl Pts',(-34.6595309261186,-63.0013920796225,
12.));
#73420=CARTESIAN_POINT('Ctrl Pts',(-34.6632634733819,-63.0249693746198,
0.));
#73421=CARTESIAN_POINT('Ctrl Pts',(-34.6632634733819,-63.0249693746198,
12.));
#73422=CARTESIAN_POINT('Ctrl Pts',(-34.6669795685225,-63.0485924065039,
0.));
#73423=CARTESIAN_POINT('Ctrl Pts',(-34.6669795685225,-63.0485924065039,
12.));
#73424=CARTESIAN_POINT('Ctrl Pts',(-34.6706791319471,-63.0722610656194,
0.));
#73425=CARTESIAN_POINT('Ctrl Pts',(-34.6706791319471,-63.0722610656194,
12.));
#73426=CARTESIAN_POINT('Ctrl Pts',(-34.6743620844722,-63.0959752427169,
0.));
#73427=CARTESIAN_POINT('Ctrl Pts',(-34.6743620844722,-63.0959752427169,
12.));
#73428=CARTESIAN_POINT('Ctrl Pts',(-34.6780283473252,-63.119734828943,0.));
#73429=CARTESIAN_POINT('Ctrl Pts',(-34.6780283473252,-63.119734828943,12.));
#73430=CARTESIAN_POINT('Ctrl Pts',(-34.6816778421401,-63.1435397158385,
0.));
#73431=CARTESIAN_POINT('Ctrl Pts',(-34.6816778421401,-63.1435397158385,
12.));
#73432=CARTESIAN_POINT('Ctrl Pts',(-34.6853104909516,-63.1673897953425,
0.));
#73433=CARTESIAN_POINT('Ctrl Pts',(-34.6853104909516,-63.1673897953425,
12.));
#73434=CARTESIAN_POINT('Ctrl Pts',(-34.6889262161923,-63.1912849597885,
0.));
#73435=CARTESIAN_POINT('Ctrl Pts',(-34.6889262161923,-63.1912849597885,
12.));
#73436=CARTESIAN_POINT('Ctrl Pts',(-34.6925249406899,-63.2152251019014,
0.));
#73437=CARTESIAN_POINT('Ctrl Pts',(-34.6925249406899,-63.2152251019014,
12.));
#73438=CARTESIAN_POINT('Ctrl Pts',(-34.6961065876671,-63.2392101147853,
0.));
#73439=CARTESIAN_POINT('Ctrl Pts',(-34.6961065876671,-63.2392101147853,
12.));
#73440=CARTESIAN_POINT('Ctrl Pts',(-34.6996710807384,-63.2632398919234,
0.));
#73441=CARTESIAN_POINT('Ctrl Pts',(-34.6996710807384,-63.2632398919234,
12.));
#73442=CARTESIAN_POINT('Ctrl Pts',(-34.7032183439045,-63.2873143271812,
0.));
#73443=CARTESIAN_POINT('Ctrl Pts',(-34.7032183439045,-63.2873143271812,
12.));
#73444=CARTESIAN_POINT('Ctrl Pts',(-34.7067483015492,-63.311433314805,0.));
#73445=CARTESIAN_POINT('Ctrl Pts',(-34.7067483015492,-63.311433314805,12.));
#73446=CARTESIAN_POINT('Ctrl Pts',(-34.7102608784373,-63.3355967494169,
0.));
#73447=CARTESIAN_POINT('Ctrl Pts',(-34.7102608784373,-63.3355967494169,
12.));
#73448=CARTESIAN_POINT('Ctrl Pts',(-34.7137559997143,-63.3598045260049,
0.));
#73449=CARTESIAN_POINT('Ctrl Pts',(-34.7137559997143,-63.3598045260049,
12.));
#73450=CARTESIAN_POINT('Ctrl Pts',(-34.7172335909037,-63.3840565399206,
0.));
#73451=CARTESIAN_POINT('Ctrl Pts',(-34.7172335909037,-63.3840565399206,
12.));
#73452=CARTESIAN_POINT('Ctrl Pts',(-34.7206935779007,-63.4083526868837,
0.));
#73453=CARTESIAN_POINT('Ctrl Pts',(-34.7206935779007,-63.4083526868837,
12.));
#73454=CARTESIAN_POINT('Ctrl Pts',(-34.7241358869702,-63.4326928629796,
0.));
#73455=CARTESIAN_POINT('Ctrl Pts',(-34.7241358869702,-63.4326928629796,
12.));
#73456=CARTESIAN_POINT('Ctrl Pts',(-34.7275604447439,-63.4570769646568,
0.));
#73457=CARTESIAN_POINT('Ctrl Pts',(-34.7275604447439,-63.4570769646568,
12.));
#73458=CARTESIAN_POINT('Ctrl Pts',(-34.7309671782212,-63.481504888716,0.));
#73459=CARTESIAN_POINT('Ctrl Pts',(-34.7309671782212,-63.481504888716,12.));
#73460=CARTESIAN_POINT('Ctrl Pts',(-34.7343560147663,-63.5059765323082,
0.));
#73461=CARTESIAN_POINT('Ctrl Pts',(-34.7343560147663,-63.5059765323082,
12.));
#73462=CARTESIAN_POINT('Ctrl Pts',(-34.7377268821022,-63.5304917929378,
0.));
#73463=CARTESIAN_POINT('Ctrl Pts',(-34.7377268821022,-63.5304917929378,
12.));
#73464=CARTESIAN_POINT('Ctrl Pts',(-34.7410797083079,-63.5550505684621,
0.));
#73465=CARTESIAN_POINT('Ctrl Pts',(-34.7410797083079,-63.5550505684621,
12.));
#73466=CARTESIAN_POINT('Ctrl Pts',(-34.7444144218162,-63.5796527570874,
0.));
#73467=CARTESIAN_POINT('Ctrl Pts',(-34.7444144218162,-63.5796527570874,
12.));
#73468=CARTESIAN_POINT('Ctrl Pts',(-34.7477309514142,-63.6042982573598,
0.));
#73469=CARTESIAN_POINT('Ctrl Pts',(-34.7477309514142,-63.6042982573598,
12.));
#73470=CARTESIAN_POINT('Ctrl Pts',(-34.7510292262415,-63.628986968162,0.));
#73471=CARTESIAN_POINT('Ctrl Pts',(-34.7510292262415,-63.628986968162,12.));
#73472=CARTESIAN_POINT('Ctrl Pts',(-34.7543091757842,-63.6537187887174,
0.));
#73473=CARTESIAN_POINT('Ctrl Pts',(-34.7543091757842,-63.6537187887174,
12.));
#73474=CARTESIAN_POINT('Ctrl Pts',(-34.7575707298718,-63.6784936185893,
0.));
#73475=CARTESIAN_POINT('Ctrl Pts',(-34.7575707298718,-63.6784936185893,
12.));
#73476=CARTESIAN_POINT('Ctrl Pts',(-34.7608138186758,-63.7033113576782,
0.));
#73477=CARTESIAN_POINT('Ctrl Pts',(-34.7608138186758,-63.7033113576782,
12.));
#73478=CARTESIAN_POINT('Ctrl Pts',(-34.7640383727094,-63.7281719062135,
0.));
#73479=CARTESIAN_POINT('Ctrl Pts',(-34.7640383727094,-63.7281719062135,
12.));
#73480=CARTESIAN_POINT('Ctrl Pts',(-34.7672443228267,-63.7530751647478,
0.));
#73481=CARTESIAN_POINT('Ctrl Pts',(-34.7672443228267,-63.7530751647478,
12.));
#73482=CARTESIAN_POINT('Ctrl Pts',(-34.7704316002165,-63.7780210341618,
0.));
#73483=CARTESIAN_POINT('Ctrl Pts',(-34.7704316002165,-63.7780210341618,
12.));
#73484=CARTESIAN_POINT('Ctrl Pts',(-34.7736001363991,-63.8030094156635,
0.));
#73485=CARTESIAN_POINT('Ctrl Pts',(-34.7736001363991,-63.8030094156635,
12.));
#73486=CARTESIAN_POINT('Ctrl Pts',(-34.7767498632244,-63.8280402107858,
0.));
#73487=CARTESIAN_POINT('Ctrl Pts',(-34.7767498632244,-63.8280402107858,
12.));
#73488=CARTESIAN_POINT('Ctrl Pts',(-34.7798807128716,-63.8531133213794,
0.));
#73489=CARTESIAN_POINT('Ctrl Pts',(-34.7798807128716,-63.8531133213794,
12.));
#73490=CARTESIAN_POINT('Ctrl Pts',(-34.7829926178495,-63.8782286496059,
0.));
#73491=CARTESIAN_POINT('Ctrl Pts',(-34.7829926178495,-63.8782286496059,
12.));
#73492=CARTESIAN_POINT('Ctrl Pts',(-34.7860855109908,-63.9033860979428,
0.));
#73493=CARTESIAN_POINT('Ctrl Pts',(-34.7860855109908,-63.9033860979428,
12.));
#73494=CARTESIAN_POINT('Ctrl Pts',(-34.7891593254485,-63.9285855691838,
0.));
#73495=CARTESIAN_POINT('Ctrl Pts',(-34.7891593254485,-63.9285855691838,
12.));
#73496=CARTESIAN_POINT('Ctrl Pts',(-34.7922139946943,-63.9538269664365,
0.));
#73497=CARTESIAN_POINT('Ctrl Pts',(-34.7922139946943,-63.9538269664365,
12.));
#73498=CARTESIAN_POINT('Ctrl Pts',(-34.7952494525182,-63.9791101931169,
0.));
#73499=CARTESIAN_POINT('Ctrl Pts',(-34.7952494525182,-63.9791101931169,
12.));
#73500=CARTESIAN_POINT('Ctrl Pts',(-34.79826563303,-64.0044351529413,0.));
#73501=CARTESIAN_POINT('Ctrl Pts',(-34.79826563303,-64.0044351529413,12.));
#73502=CARTESIAN_POINT('Ctrl Pts',(-34.8012624706534,-64.0298017499304,
0.));
#73503=CARTESIAN_POINT('Ctrl Pts',(-34.8012624706534,-64.0298017499304,
12.));
#73504=CARTESIAN_POINT('Ctrl Pts',(-34.8042399001215,-64.05520988841,0.));
#73505=CARTESIAN_POINT('Ctrl Pts',(-34.8042399001215,-64.05520988841,12.));
#73506=CARTESIAN_POINT('Ctrl Pts',(-34.8071978564748,-64.0806594730084,
0.));
#73507=CARTESIAN_POINT('Ctrl Pts',(-34.8071978564748,-64.0806594730084,
12.));
#73508=CARTESIAN_POINT('Ctrl Pts',(-34.8101362750595,-64.1061504086512,
0.));
#73509=CARTESIAN_POINT('Ctrl Pts',(-34.8101362750595,-64.1061504086512,
12.));
#73510=CARTESIAN_POINT('Ctrl Pts',(-34.8130550915284,-64.1316826005502,
0.));
#73511=CARTESIAN_POINT('Ctrl Pts',(-34.8130550915284,-64.1316826005502,
12.));
#73512=CARTESIAN_POINT('Ctrl Pts',(-34.8159542418372,-64.1572559542084,
0.));
#73513=CARTESIAN_POINT('Ctrl Pts',(-34.8159542418372,-64.1572559542084,
12.));
#73514=CARTESIAN_POINT('Ctrl Pts',(-34.8188336622419,-64.1828703754237,
0.));
#73515=CARTESIAN_POINT('Ctrl Pts',(-34.8188336622419,-64.1828703754237,
12.));
#73516=CARTESIAN_POINT('Ctrl Pts',(-34.8216932892969,-64.2085257702885,
0.));
#73517=CARTESIAN_POINT('Ctrl Pts',(-34.8216932892969,-64.2085257702885,
12.));
#73518=CARTESIAN_POINT('Ctrl Pts',(-34.8245330598559,-64.2342220451878,
0.));
#73519=CARTESIAN_POINT('Ctrl Pts',(-34.8245330598559,-64.2342220451878,
12.));
#73520=CARTESIAN_POINT('Ctrl Pts',(-34.8273529110742,-64.259959106791,0.));
#73521=CARTESIAN_POINT('Ctrl Pts',(-34.8273529110742,-64.259959106791,12.));
#73522=CARTESIAN_POINT('Ctrl Pts',(-34.8301527804052,-64.2857368620513,
0.));
#73523=CARTESIAN_POINT('Ctrl Pts',(-34.8301527804052,-64.2857368620513,
12.));
#73524=CARTESIAN_POINT('Ctrl Pts',(-34.8329326055916,-64.3115552182056,
0.));
#73525=CARTESIAN_POINT('Ctrl Pts',(-34.8329326055916,-64.3115552182056,
12.));
#73526=CARTESIAN_POINT('Ctrl Pts',(-34.8356923246617,-64.3374140827708,
0.));
#73527=CARTESIAN_POINT('Ctrl Pts',(-34.8356923246617,-64.3374140827708,
12.));
#73528=CARTESIAN_POINT('Ctrl Pts',(-34.838431875925,-64.3633133635384,0.));
#73529=CARTESIAN_POINT('Ctrl Pts',(-34.838431875925,-64.3633133635384,12.));
#73530=CARTESIAN_POINT('Ctrl Pts',(-34.8411511979705,-64.3892529685614,
0.));
#73531=CARTESIAN_POINT('Ctrl Pts',(-34.8411511979705,-64.3892529685614,
12.));
#73532=CARTESIAN_POINT('Ctrl Pts',(-34.8438502296669,-64.4152328061526,
0.));
#73533=CARTESIAN_POINT('Ctrl Pts',(-34.8438502296669,-64.4152328061526,
12.));
#73534=CARTESIAN_POINT('Ctrl Pts',(-34.8465289101626,-64.4412527848979,
0.));
#73535=CARTESIAN_POINT('Ctrl Pts',(-34.8465289101626,-64.4412527848979,
12.));
#73536=CARTESIAN_POINT('Ctrl Pts',(-34.8491871788899,-64.4673128136631,
0.));
#73537=CARTESIAN_POINT('Ctrl Pts',(-34.8491871788899,-64.4673128136631,
12.));
#73538=CARTESIAN_POINT('Ctrl Pts',(-34.851824975568,-64.4934128015983,0.));
#73539=CARTESIAN_POINT('Ctrl Pts',(-34.851824975568,-64.4934128015983,12.));
#73540=CARTESIAN_POINT('Ctrl Pts',(-34.8544422402114,-64.5195526581398,
0.));
#73541=CARTESIAN_POINT('Ctrl Pts',(-34.8544422402114,-64.5195526581398,
12.));
#73542=CARTESIAN_POINT('Ctrl Pts',(-34.8570389131334,-64.5457322930074,
0.));
#73543=CARTESIAN_POINT('Ctrl Pts',(-34.8570389131334,-64.5457322930074,
12.));
#73544=CARTESIAN_POINT('Ctrl Pts',(-34.8596149349251,-64.5719516161913,
0.));
#73545=CARTESIAN_POINT('Ctrl Pts',(-34.8596149349251,-64.5719516161913,
12.));
#73546=CARTESIAN_POINT('Ctrl Pts',(-34.8621702464397,-64.5982105379374,
0.));
#73547=CARTESIAN_POINT('Ctrl Pts',(-34.8621702464397,-64.5982105379374,
12.));
#73548=CARTESIAN_POINT('Ctrl Pts',(-34.8647047887774,-64.6245089687276,
0.));
#73549=CARTESIAN_POINT('Ctrl Pts',(-34.8647047887774,-64.6245089687276,
12.));
#73550=CARTESIAN_POINT('Ctrl Pts',(-34.8672185032725,-64.6508468192609,
0.));
#73551=CARTESIAN_POINT('Ctrl Pts',(-34.8672185032725,-64.6508468192609,
12.));
#73552=CARTESIAN_POINT('Ctrl Pts',(-34.8697113314797,-64.6772240004241,
0.));
#73553=CARTESIAN_POINT('Ctrl Pts',(-34.8697113314797,-64.6772240004241,
12.));
#73554=CARTESIAN_POINT('Ctrl Pts',(-34.8721832151982,-64.7036404233319,
0.));
#73555=CARTESIAN_POINT('Ctrl Pts',(-34.8721832151982,-64.7036404233319,
12.));
#73556=CARTESIAN_POINT('Ctrl Pts',(-34.8746340964977,-64.7300959993662,
0.));
#73557=CARTESIAN_POINT('Ctrl Pts',(-34.8746340964977,-64.7300959993662,
12.));
#73558=CARTESIAN_POINT('Ctrl Pts',(-34.8770639177494,-64.7565906402153,
0.));
#73559=CARTESIAN_POINT('Ctrl Pts',(-34.8770639177494,-64.7565906402153,
12.));
#73560=CARTESIAN_POINT('Ctrl Pts',(-34.8794726216511,-64.7831242579023,
0.));
#73561=CARTESIAN_POINT('Ctrl Pts',(-34.8794726216511,-64.7831242579023,
12.));
#73562=CARTESIAN_POINT('Ctrl Pts',(-34.8818601512726,-64.8096967648299,
0.));
#73563=CARTESIAN_POINT('Ctrl Pts',(-34.8818601512726,-64.8096967648299,
12.));
#73564=CARTESIAN_POINT('Ctrl Pts',(-34.8842264500184,-64.8363080737369,
0.));
#73565=CARTESIAN_POINT('Ctrl Pts',(-34.8842264500184,-64.8363080737369,
12.));
#73566=CARTESIAN_POINT('Ctrl Pts',(-34.8865714615433,-64.8629580976057,
0.));
#73567=CARTESIAN_POINT('Ctrl Pts',(-34.8865714615433,-64.8629580976057,
12.));
#73568=CARTESIAN_POINT('Ctrl Pts',(-34.888895129681,-64.8896467495754,0.));
#73569=CARTESIAN_POINT('Ctrl Pts',(-34.888895129681,-64.8896467495754,12.));
#73570=CARTESIAN_POINT('Ctrl Pts',(-34.8911973983785,-64.9163739428606,
0.));
#73571=CARTESIAN_POINT('Ctrl Pts',(-34.8911973983785,-64.9163739428606,
12.));
#73572=CARTESIAN_POINT('Ctrl Pts',(-34.8934782116097,-64.943139590634,0.));
#73573=CARTESIAN_POINT('Ctrl Pts',(-34.8934782116097,-64.943139590634,12.));
#73574=CARTESIAN_POINT('Ctrl Pts',(-34.8957375133702,-64.9699436060178,
0.));
#73575=CARTESIAN_POINT('Ctrl Pts',(-34.8957375133702,-64.9699436060178,
12.));
#73576=CARTESIAN_POINT('Ctrl Pts',(-34.8979752478623,-64.9967859023225,
0.));
#73577=CARTESIAN_POINT('Ctrl Pts',(-34.8979752478623,-64.9967859023225,
12.));
#73578=CARTESIAN_POINT('Ctrl Pts',(-34.9001913596422,-65.0236663932338,
0.));
#73579=CARTESIAN_POINT('Ctrl Pts',(-34.9001913596422,-65.0236663932338,
12.));
#73580=CARTESIAN_POINT('Ctrl Pts',(-34.9023857937866,-65.0505849930172,
0.));
#73581=CARTESIAN_POINT('Ctrl Pts',(-34.9023857937866,-65.0505849930172,
12.));
#73582=CARTESIAN_POINT('Ctrl Pts',(-34.9045584960503,-65.0775416167073,
0.));
#73583=CARTESIAN_POINT('Ctrl Pts',(-34.9045584960503,-65.0775416167073,
12.));
#73584=CARTESIAN_POINT('Ctrl Pts',(-34.9067094130387,-65.1045361803097,
0.));
#73585=CARTESIAN_POINT('Ctrl Pts',(-34.9067094130387,-65.1045361803097,
12.));
#73586=CARTESIAN_POINT('Ctrl Pts',(-34.9088384918322,-65.1315686003485,
0.));
#73587=CARTESIAN_POINT('Ctrl Pts',(-34.9088384918322,-65.1315686003485,
12.));
#73588=CARTESIAN_POINT('Ctrl Pts',(-34.9109456796201,-65.1586387934216,
0.));
#73589=CARTESIAN_POINT('Ctrl Pts',(-34.9109456796201,-65.1586387934216,
12.));
#73590=CARTESIAN_POINT('Ctrl Pts',(-34.9130309233017,-65.1857466757082,
0.));
#73591=CARTESIAN_POINT('Ctrl Pts',(-34.9130309233017,-65.1857466757082,
12.));
#73592=CARTESIAN_POINT('Ctrl Pts',(-34.9150941691754,-65.2128921625837,
0.));
#73593=CARTESIAN_POINT('Ctrl Pts',(-34.9150941691754,-65.2128921625837,
12.));
#73594=CARTESIAN_POINT('Ctrl Pts',(-34.9171353624131,-65.2400751679586,
0.));
#73595=CARTESIAN_POINT('Ctrl Pts',(-34.9171353624131,-65.2400751679586,
12.));
#73596=CARTESIAN_POINT('Ctrl Pts',(-34.9191544474898,-65.2672956048121,
0.));
#73597=CARTESIAN_POINT('Ctrl Pts',(-34.9191544474898,-65.2672956048121,
12.));
#73598=CARTESIAN_POINT('Ctrl Pts',(-34.921151369138,-65.2945533863812,0.));
#73599=CARTESIAN_POINT('Ctrl Pts',(-34.921151369138,-65.2945533863812,12.));
#73600=CARTESIAN_POINT('Ctrl Pts',(-34.9231260731846,-65.3218484271941,
0.));
#73601=CARTESIAN_POINT('Ctrl Pts',(-34.9231260731846,-65.3218484271941,
12.));
#73602=CARTESIAN_POINT('Ctrl Pts',(-34.9250785073473,-65.3491806440529,
0.));
#73603=CARTESIAN_POINT('Ctrl Pts',(-34.9250785073473,-65.3491806440529,
12.));
#73604=CARTESIAN_POINT('Ctrl Pts',(-34.9270086222703,-65.3765499573019,
0.));
#73605=CARTESIAN_POINT('Ctrl Pts',(-34.9270086222703,-65.3765499573019,
12.));
#73606=CARTESIAN_POINT('Ctrl Pts',(-34.92891637177,-65.4039562911254,0.));
#73607=CARTESIAN_POINT('Ctrl Pts',(-34.92891637177,-65.4039562911254,12.));
#73608=CARTESIAN_POINT('Ctrl Pts',(-34.9308017105481,-65.4313995707423,
0.));
#73609=CARTESIAN_POINT('Ctrl Pts',(-34.9308017105481,-65.4313995707423,
12.));
#73610=CARTESIAN_POINT('Ctrl Pts',(-34.9326645923897,-65.4588797201884,
0.));
#73611=CARTESIAN_POINT('Ctrl Pts',(-34.9326645923897,-65.4588797201884,
12.));
#73612=CARTESIAN_POINT('Ctrl Pts',(-34.9345049680816,-65.4863966597523,
0.));
#73613=CARTESIAN_POINT('Ctrl Pts',(-34.9345049680816,-65.4863966597523,
12.));
#73614=CARTESIAN_POINT('Ctrl Pts',(-34.9363227836621,-65.5139503038116,
0.));
#73615=CARTESIAN_POINT('Ctrl Pts',(-34.9363227836621,-65.5139503038116,
12.));
#73616=CARTESIAN_POINT('Ctrl Pts',(-34.9381179779763,-65.5415405578138,
0.));
#73617=CARTESIAN_POINT('Ctrl Pts',(-34.9381179779763,-65.5415405578138,
12.));
#73618=CARTESIAN_POINT('Ctrl Pts',(-34.9398904862279,-65.5691673226051,
0.));
#73619=CARTESIAN_POINT('Ctrl Pts',(-34.9398904862279,-65.5691673226051,
12.));
#73620=CARTESIAN_POINT('Ctrl Pts',(-34.9416402443551,-65.5968304997821,
0.));
#73621=CARTESIAN_POINT('Ctrl Pts',(-34.9416402443551,-65.5968304997821,
12.));
#73622=CARTESIAN_POINT('Ctrl Pts',(-34.9433671932982,-65.6245299968635,
0.));
#73623=CARTESIAN_POINT('Ctrl Pts',(-34.9433671932982,-65.6245299968635,
12.));
#73624=CARTESIAN_POINT('Ctrl Pts',(-34.9450712829143,-65.6522657321239,
0.));
#73625=CARTESIAN_POINT('Ctrl Pts',(-34.9450712829143,-65.6522657321239,
12.));
#73626=CARTESIAN_POINT('Ctrl Pts',(-34.9467524770271,-65.6800376405722,
0.));
#73627=CARTESIAN_POINT('Ctrl Pts',(-34.9467524770271,-65.6800376405722,
12.));
#73628=CARTESIAN_POINT('Ctrl Pts',(-34.9484107543857,-65.707845675746,0.));
#73629=CARTESIAN_POINT('Ctrl Pts',(-34.9484107543857,-65.707845675746,12.));
#73630=CARTESIAN_POINT('Ctrl Pts',(-34.9500461042919,-65.7356898060478,
0.));
#73631=CARTESIAN_POINT('Ctrl Pts',(-34.9500461042919,-65.7356898060478,
12.));
#73632=CARTESIAN_POINT('Ctrl Pts',(-34.9513360397181,-65.757993971173,0.));
#73633=CARTESIAN_POINT('Ctrl Pts',(-34.9513360397181,-65.757993971173,12.));
#73634=CARTESIAN_POINT('Ctrl Pts',(-34.9522931728594,-65.7747383250775,
0.));
#73635=CARTESIAN_POINT('Ctrl Pts',(-34.9522931728594,-65.7747383250775,
12.));
#73636=CARTESIAN_POINT('Ctrl Pts',(-34.9529266758406,-65.7859084407494,
0.));
#73637=CARTESIAN_POINT('Ctrl Pts',(-34.9529266758406,-65.7859084407494,
12.));
#73638=CARTESIAN_POINT('Ctrl Pts',(-34.9532422808861,-65.7914953018524,
0.));
#73639=CARTESIAN_POINT('Ctrl Pts',(-34.9532422808861,-65.7914953018524,
12.));
#73640=CARTESIAN_POINT('',(-34.2579614092497,-61.0441813777723,0.));
#73641=CARTESIAN_POINT('Ctrl Pts',(-34.2579614092497,-61.0441813777723,
0.));
#73642=CARTESIAN_POINT('Ctrl Pts',(-34.2589297755434,-61.0479423318725,
0.));
#73643=CARTESIAN_POINT('Ctrl Pts',(-34.2608658001631,-61.0554700176998,
0.));
#73644=CARTESIAN_POINT('Ctrl Pts',(-34.2637677131935,-61.0667788793266,
0.));
#73645=CARTESIAN_POINT('Ctrl Pts',(-34.2676326825626,-61.0818920286293,
0.));
#73646=CARTESIAN_POINT('Ctrl Pts',(-34.2724568037228,-61.1008412399997,
0.));
#73647=CARTESIAN_POINT('Ctrl Pts',(-34.2772738038771,-61.1198481997764,
0.));
#73648=CARTESIAN_POINT('Ctrl Pts',(-34.282083624447,-61.1389128461885,0.));
#73649=CARTESIAN_POINT('Ctrl Pts',(-34.2868861666384,-61.1580350635532,
0.));
#73650=CARTESIAN_POINT('Ctrl Pts',(-34.2916812929751,-61.1772146833205,
0.));
#73651=CARTESIAN_POINT('Ctrl Pts',(-34.2964688443663,-61.1964515073891,
0.));
#73652=CARTESIAN_POINT('Ctrl Pts',(-34.3012486533474,-61.2157453259107,
0.));
#73653=CARTESIAN_POINT('Ctrl Pts',(-34.3060205584065,-61.2350959366939,
0.));
#73654=CARTESIAN_POINT('Ctrl Pts',(-34.3107844191044,-61.2545031656133,
0.));
#73655=CARTESIAN_POINT('Ctrl Pts',(-34.3155401111747,-61.2739668600365,
0.));
#73656=CARTESIAN_POINT('Ctrl Pts',(-34.3202875193618,-61.2934868791854,
0.));
#73657=CARTESIAN_POINT('Ctrl Pts',(-34.3250265314768,-61.3130630861386,
0.));
#73658=CARTESIAN_POINT('Ctrl Pts',(-34.3297570310146,-61.3326953378851,
0.));
#73659=CARTESIAN_POINT('Ctrl Pts',(-34.3344788934363,-61.3523834803188,
0.));
#73660=CARTESIAN_POINT('Ctrl Pts',(-34.339191990014,-61.3721273534256,0.));
#73661=CARTESIAN_POINT('Ctrl Pts',(-34.3438961902405,-61.3919267945302,
0.));
#73662=CARTESIAN_POINT('Ctrl Pts',(-34.3485913645979,-61.4117816420228,
0.));
#73663=CARTESIAN_POINT('Ctrl Pts',(-34.3532773877089,-61.4316917395918,
0.));
#73664=CARTESIAN_POINT('Ctrl Pts',(-34.3579541381996,-61.4516569360454,
0.));
#73665=CARTESIAN_POINT('Ctrl Pts',(-34.3626214971889,-61.4716770832896,
0.));
#73666=CARTESIAN_POINT('Ctrl Pts',(-34.3672793472466,-61.4917520349278,
0.));
#73667=CARTESIAN_POINT('Ctrl Pts',(-34.3719275711195,-61.5118816445437,
0.));
#73668=CARTESIAN_POINT('Ctrl Pts',(-34.376566050668,-61.5320657642638,0.));
#73669=CARTESIAN_POINT('Ctrl Pts',(-34.3811946674197,-61.5523042455158,
0.));
#73670=CARTESIAN_POINT('Ctrl Pts',(-34.3858133030518,-61.5725969396829,
0.));
#73671=CARTESIAN_POINT('Ctrl Pts',(-34.3904218398637,-61.5929436987409,
0.));
#73672=CARTESIAN_POINT('Ctrl Pts',(-34.3950201613432,-61.6133443760142,
0.));
#73673=CARTESIAN_POINT('Ctrl Pts',(-34.3996081523753,-61.6337988264556,
0.));
#73674=CARTESIAN_POINT('Ctrl Pts',(-34.4041856989317,-61.6543069062416,
0.));
#73675=CARTESIAN_POINT('Ctrl Pts',(-34.4087526878812,-61.6748684725205,
0.));
#73676=CARTESIAN_POINT('Ctrl Pts',(-34.4133090067704,-61.695483383117,0.));
#73677=CARTESIAN_POINT('Ctrl Pts',(-34.4178545435767,-61.7161514961914,
0.));
#73678=CARTESIAN_POINT('Ctrl Pts',(-34.422389186718,-61.7368726702596,0.));
#73679=CARTESIAN_POINT('Ctrl Pts',(-34.4269128251577,-61.7576467643432,
0.));
#73680=CARTESIAN_POINT('Ctrl Pts',(-34.4314253484792,-61.7784736380727,
0.));
#73681=CARTESIAN_POINT('Ctrl Pts',(-34.4359266469749,-61.7993531518036,
0.));
#73682=CARTESIAN_POINT('Ctrl Pts',(-34.4404166117299,-61.8202851667222,
0.));
#73683=CARTESIAN_POINT('Ctrl Pts',(-34.444895134574,-61.8412695447926,0.));
#73684=CARTESIAN_POINT('Ctrl Pts',(-34.4493621080361,-61.8623061487018,
0.));
#73685=CARTESIAN_POINT('Ctrl Pts',(-34.4538174253012,-61.8833948418025,
0.));
#73686=CARTESIAN_POINT('Ctrl Pts',(-34.4582609801637,-61.9045354880444,
0.));
#73687=CARTESIAN_POINT('Ctrl Pts',(-34.4626926669975,-61.9257279519308,
0.));
#73688=CARTESIAN_POINT('Ctrl Pts',(-34.4671123807717,-61.9469720985531,
0.));
#73689=CARTESIAN_POINT('Ctrl Pts',(-34.4715200170592,-61.9682677936053,
0.));
#73690=CARTESIAN_POINT('Ctrl Pts',(-34.4759154720473,-61.9896149034001,
0.));
#73691=CARTESIAN_POINT('Ctrl Pts',(-34.4802986425528,-62.0110132948794,
0.));
#73692=CARTESIAN_POINT('Ctrl Pts',(-34.48466942602,-62.0324628356141,0.));
#73693=CARTESIAN_POINT('Ctrl Pts',(-34.489027720504,-62.0539633937939,0.));
#73694=CARTESIAN_POINT('Ctrl Pts',(-34.4933734246593,-62.0755148382135,
0.));
#73695=CARTESIAN_POINT('Ctrl Pts',(-34.4977064377282,-62.0971170382567,
0.));
#73696=CARTESIAN_POINT('Ctrl Pts',(-34.5020266595293,-62.1187698638707,
0.));
#73697=CARTESIAN_POINT('Ctrl Pts',(-34.5063339904533,-62.1404731855687,
0.));
#73698=CARTESIAN_POINT('Ctrl Pts',(-34.5106283314594,-62.1622268744337,
0.));
#73699=CARTESIAN_POINT('Ctrl Pts',(-34.514909584073,-62.184030802117,0.));
#73700=CARTESIAN_POINT('Ctrl Pts',(-34.5191776503843,-62.2058848408346,
0.));
#73701=CARTESIAN_POINT('Ctrl Pts',(-34.5234324330492,-62.2277888633576,
0.));
#73702=CARTESIAN_POINT('Ctrl Pts',(-34.527673835281,-62.2497427430136,0.));
#73703=CARTESIAN_POINT('Ctrl Pts',(-34.5319017608435,-62.2717463536828,
0.));
#73704=CARTESIAN_POINT('Ctrl Pts',(-34.536116114045,-62.2937995697927,0.));
#73705=CARTESIAN_POINT('Ctrl Pts',(-34.5403167997333,-62.3159022663052,
0.));
#73706=CARTESIAN_POINT('Ctrl Pts',(-34.5445037232928,-62.3380543187067,
0.));
#73707=CARTESIAN_POINT('Ctrl Pts',(-34.5486767906376,-62.3602556030114,
0.));
#73708=CARTESIAN_POINT('Ctrl Pts',(-34.552835908207,-62.3825059957593,0.));
#73709=CARTESIAN_POINT('Ctrl Pts',(-34.5569809829615,-62.4048053740129,
0.));
#73710=CARTESIAN_POINT('Ctrl Pts',(-34.5611119223807,-62.4271536153473,
0.));
#73711=CARTESIAN_POINT('Ctrl Pts',(-34.5652286344606,-62.4495505978415,
0.));
#73712=CARTESIAN_POINT('Ctrl Pts',(-34.5693310277064,-62.4719962000829,
0.));
#73713=CARTESIAN_POINT('Ctrl Pts',(-34.5734190111279,-62.494490301164,0.));
#73714=CARTESIAN_POINT('Ctrl Pts',(-34.5774924942351,-62.5170327806774,
0.));
#73715=CARTESIAN_POINT('Ctrl Pts',(-34.5815513870363,-62.5396235187053,
0.));
#73716=CARTESIAN_POINT('Ctrl Pts',(-34.5855956000344,-62.5622623958125,
0.));
#73717=CARTESIAN_POINT('Ctrl Pts',(-34.5896250442199,-62.5849492930501,
0.));
#73718=CARTESIAN_POINT('Ctrl Pts',(-34.5936396310671,-62.6076840919521,
0.));
#73719=CARTESIAN_POINT('Ctrl Pts',(-34.5976392725303,-62.6304666745319,
0.));
#73720=CARTESIAN_POINT('Ctrl Pts',(-34.6016238810419,-62.6532969232695,
0.));
#73721=CARTESIAN_POINT('Ctrl Pts',(-34.6055933695093,-62.6761747211081,
0.));
#73722=CARTESIAN_POINT('Ctrl Pts',(-34.6095476513095,-62.6990999514597,
0.));
#73723=CARTESIAN_POINT('Ctrl Pts',(-34.6134866402842,-62.7220724982005,
0.));
#73724=CARTESIAN_POINT('Ctrl Pts',(-34.6174102507368,-62.7450922456662,
0.));
#73725=CARTESIAN_POINT('Ctrl Pts',(-34.6213183974303,-62.7681590786398,
0.));
#73726=CARTESIAN_POINT('Ctrl Pts',(-34.6252109955836,-62.7912728823482,
0.));
#73727=CARTESIAN_POINT('Ctrl Pts',(-34.629087960866,-62.8144335424671,0.));
#73728=CARTESIAN_POINT('Ctrl Pts',(-34.6329492093932,-62.8376409451167,
0.));
#73729=CARTESIAN_POINT('Ctrl Pts',(-34.6367946577241,-62.8608949768583,
0.));
#73730=CARTESIAN_POINT('Ctrl Pts',(-34.6406242228606,-62.8841955246819,
0.));
#73731=CARTESIAN_POINT('Ctrl Pts',(-34.6444378222425,-62.9075424760042,
0.));
#73732=CARTESIAN_POINT('Ctrl Pts',(-34.6482353737434,-62.9309357186733,
0.));
#73733=CARTESIAN_POINT('Ctrl Pts',(-34.6520167956657,-62.9543751409647,
0.));
#73734=CARTESIAN_POINT('Ctrl Pts',(-34.655782006739,-62.9778606315777,0.));
#73735=CARTESIAN_POINT('Ctrl Pts',(-34.6595309261186,-63.0013920796225,
0.));
#73736=CARTESIAN_POINT('Ctrl Pts',(-34.6632634733819,-63.0249693746198,
0.));
#73737=CARTESIAN_POINT('Ctrl Pts',(-34.6669795685225,-63.0485924065039,
0.));
#73738=CARTESIAN_POINT('Ctrl Pts',(-34.6706791319471,-63.0722610656194,
0.));
#73739=CARTESIAN_POINT('Ctrl Pts',(-34.6743620844722,-63.0959752427169,
0.));
#73740=CARTESIAN_POINT('Ctrl Pts',(-34.6780283473252,-63.119734828943,0.));
#73741=CARTESIAN_POINT('Ctrl Pts',(-34.6816778421401,-63.1435397158385,
0.));
#73742=CARTESIAN_POINT('Ctrl Pts',(-34.6853104909516,-63.1673897953425,
0.));
#73743=CARTESIAN_POINT('Ctrl Pts',(-34.6889262161923,-63.1912849597885,
0.));
#73744=CARTESIAN_POINT('Ctrl Pts',(-34.6925249406899,-63.2152251019014,
0.));
#73745=CARTESIAN_POINT('Ctrl Pts',(-34.6961065876671,-63.2392101147853,
0.));
#73746=CARTESIAN_POINT('Ctrl Pts',(-34.6996710807384,-63.2632398919234,
0.));
#73747=CARTESIAN_POINT('Ctrl Pts',(-34.7032183439045,-63.2873143271812,
0.));
#73748=CARTESIAN_POINT('Ctrl Pts',(-34.7067483015492,-63.311433314805,0.));
#73749=CARTESIAN_POINT('Ctrl Pts',(-34.7102608784373,-63.3355967494169,
0.));
#73750=CARTESIAN_POINT('Ctrl Pts',(-34.7137559997143,-63.3598045260049,
0.));
#73751=CARTESIAN_POINT('Ctrl Pts',(-34.7172335909037,-63.3840565399206,
0.));
#73752=CARTESIAN_POINT('Ctrl Pts',(-34.7206935779007,-63.4083526868837,
0.));
#73753=CARTESIAN_POINT('Ctrl Pts',(-34.7241358869702,-63.4326928629796,
0.));
#73754=CARTESIAN_POINT('Ctrl Pts',(-34.7275604447439,-63.4570769646568,
0.));
#73755=CARTESIAN_POINT('Ctrl Pts',(-34.7309671782212,-63.481504888716,0.));
#73756=CARTESIAN_POINT('Ctrl Pts',(-34.7343560147663,-63.5059765323082,
0.));
#73757=CARTESIAN_POINT('Ctrl Pts',(-34.7377268821022,-63.5304917929378,
0.));
#73758=CARTESIAN_POINT('Ctrl Pts',(-34.7410797083079,-63.5550505684621,
0.));
#73759=CARTESIAN_POINT('Ctrl Pts',(-34.7444144218162,-63.5796527570874,
0.));
#73760=CARTESIAN_POINT('Ctrl Pts',(-34.7477309514142,-63.6042982573598,
0.));
#73761=CARTESIAN_POINT('Ctrl Pts',(-34.7510292262415,-63.628986968162,0.));
#73762=CARTESIAN_POINT('Ctrl Pts',(-34.7543091757842,-63.6537187887174,
0.));
#73763=CARTESIAN_POINT('Ctrl Pts',(-34.7575707298718,-63.6784936185893,
0.));
#73764=CARTESIAN_POINT('Ctrl Pts',(-34.7608138186758,-63.7033113576782,
0.));
#73765=CARTESIAN_POINT('Ctrl Pts',(-34.7640383727094,-63.7281719062135,
0.));
#73766=CARTESIAN_POINT('Ctrl Pts',(-34.7672443228267,-63.7530751647478,
0.));
#73767=CARTESIAN_POINT('Ctrl Pts',(-34.7704316002165,-63.7780210341618,
0.));
#73768=CARTESIAN_POINT('Ctrl Pts',(-34.7736001363991,-63.8030094156635,
0.));
#73769=CARTESIAN_POINT('Ctrl Pts',(-34.7767498632244,-63.8280402107858,
0.));
#73770=CARTESIAN_POINT('Ctrl Pts',(-34.7798807128716,-63.8531133213794,
0.));
#73771=CARTESIAN_POINT('Ctrl Pts',(-34.7829926178495,-63.8782286496059,
0.));
#73772=CARTESIAN_POINT('Ctrl Pts',(-34.7860855109908,-63.9033860979428,
0.));
#73773=CARTESIAN_POINT('Ctrl Pts',(-34.7891593254485,-63.9285855691838,
0.));
#73774=CARTESIAN_POINT('Ctrl Pts',(-34.7922139946943,-63.9538269664365,
0.));
#73775=CARTESIAN_POINT('Ctrl Pts',(-34.7952494525182,-63.9791101931169,
0.));
#73776=CARTESIAN_POINT('Ctrl Pts',(-34.79826563303,-64.0044351529413,0.));
#73777=CARTESIAN_POINT('Ctrl Pts',(-34.8012624706534,-64.0298017499304,
0.));
#73778=CARTESIAN_POINT('Ctrl Pts',(-34.8042399001215,-64.05520988841,0.));
#73779=CARTESIAN_POINT('Ctrl Pts',(-34.8071978564748,-64.0806594730084,
0.));
#73780=CARTESIAN_POINT('Ctrl Pts',(-34.8101362750595,-64.1061504086512,
0.));
#73781=CARTESIAN_POINT('Ctrl Pts',(-34.8130550915284,-64.1316826005502,
0.));
#73782=CARTESIAN_POINT('Ctrl Pts',(-34.8159542418372,-64.1572559542084,
0.));
#73783=CARTESIAN_POINT('Ctrl Pts',(-34.8188336622419,-64.1828703754237,
0.));
#73784=CARTESIAN_POINT('Ctrl Pts',(-34.8216932892969,-64.2085257702885,
0.));
#73785=CARTESIAN_POINT('Ctrl Pts',(-34.8245330598559,-64.2342220451878,
0.));
#73786=CARTESIAN_POINT('Ctrl Pts',(-34.8273529110742,-64.259959106791,0.));
#73787=CARTESIAN_POINT('Ctrl Pts',(-34.8301527804052,-64.2857368620513,
0.));
#73788=CARTESIAN_POINT('Ctrl Pts',(-34.8329326055916,-64.3115552182056,
0.));
#73789=CARTESIAN_POINT('Ctrl Pts',(-34.8356923246617,-64.3374140827708,
0.));
#73790=CARTESIAN_POINT('Ctrl Pts',(-34.838431875925,-64.3633133635384,0.));
#73791=CARTESIAN_POINT('Ctrl Pts',(-34.8411511979705,-64.3892529685614,
0.));
#73792=CARTESIAN_POINT('Ctrl Pts',(-34.8438502296669,-64.4152328061526,
0.));
#73793=CARTESIAN_POINT('Ctrl Pts',(-34.8465289101626,-64.4412527848979,
0.));
#73794=CARTESIAN_POINT('Ctrl Pts',(-34.8491871788899,-64.4673128136631,
0.));
#73795=CARTESIAN_POINT('Ctrl Pts',(-34.851824975568,-64.4934128015983,0.));
#73796=CARTESIAN_POINT('Ctrl Pts',(-34.8544422402114,-64.5195526581398,
0.));
#73797=CARTESIAN_POINT('Ctrl Pts',(-34.8570389131334,-64.5457322930074,
0.));
#73798=CARTESIAN_POINT('Ctrl Pts',(-34.8596149349251,-64.5719516161913,
0.));
#73799=CARTESIAN_POINT('Ctrl Pts',(-34.8621702464397,-64.5982105379374,
0.));
#73800=CARTESIAN_POINT('Ctrl Pts',(-34.8647047887774,-64.6245089687276,
0.));
#73801=CARTESIAN_POINT('Ctrl Pts',(-34.8672185032725,-64.6508468192609,
0.));
#73802=CARTESIAN_POINT('Ctrl Pts',(-34.8697113314797,-64.6772240004241,
0.));
#73803=CARTESIAN_POINT('Ctrl Pts',(-34.8721832151982,-64.7036404233319,
0.));
#73804=CARTESIAN_POINT('Ctrl Pts',(-34.8746340964977,-64.7300959993662,
0.));
#73805=CARTESIAN_POINT('Ctrl Pts',(-34.8770639177494,-64.7565906402153,
0.));
#73806=CARTESIAN_POINT('Ctrl Pts',(-34.8794726216511,-64.7831242579023,
0.));
#73807=CARTESIAN_POINT('Ctrl Pts',(-34.8818601512726,-64.8096967648299,
0.));
#73808=CARTESIAN_POINT('Ctrl Pts',(-34.8842264500184,-64.8363080737369,
0.));
#73809=CARTESIAN_POINT('Ctrl Pts',(-34.8865714615433,-64.8629580976057,
0.));
#73810=CARTESIAN_POINT('Ctrl Pts',(-34.888895129681,-64.8896467495754,0.));
#73811=CARTESIAN_POINT('Ctrl Pts',(-34.8911973983785,-64.9163739428606,
0.));
#73812=CARTESIAN_POINT('Ctrl Pts',(-34.8934782116097,-64.943139590634,0.));
#73813=CARTESIAN_POINT('Ctrl Pts',(-34.8957375133702,-64.9699436060178,
0.));
#73814=CARTESIAN_POINT('Ctrl Pts',(-34.8979752478623,-64.9967859023225,
0.));
#73815=CARTESIAN_POINT('Ctrl Pts',(-34.9001913596422,-65.0236663932338,
0.));
#73816=CARTESIAN_POINT('Ctrl Pts',(-34.9023857937866,-65.0505849930172,
0.));
#73817=CARTESIAN_POINT('Ctrl Pts',(-34.9045584960503,-65.0775416167073,
0.));
#73818=CARTESIAN_POINT('Ctrl Pts',(-34.9067094130387,-65.1045361803097,
0.));
#73819=CARTESIAN_POINT('Ctrl Pts',(-34.9088384918322,-65.1315686003485,
0.));
#73820=CARTESIAN_POINT('Ctrl Pts',(-34.9109456796201,-65.1586387934216,
0.));
#73821=CARTESIAN_POINT('Ctrl Pts',(-34.9130309233017,-65.1857466757082,
0.));
#73822=CARTESIAN_POINT('Ctrl Pts',(-34.9150941691754,-65.2128921625837,
0.));
#73823=CARTESIAN_POINT('Ctrl Pts',(-34.9171353624131,-65.2400751679586,
0.));
#73824=CARTESIAN_POINT('Ctrl Pts',(-34.9191544474898,-65.2672956048121,
0.));
#73825=CARTESIAN_POINT('Ctrl Pts',(-34.921151369138,-65.2945533863812,0.));
#73826=CARTESIAN_POINT('Ctrl Pts',(-34.9231260731846,-65.3218484271941,
0.));
#73827=CARTESIAN_POINT('Ctrl Pts',(-34.9250785073473,-65.3491806440529,
0.));
#73828=CARTESIAN_POINT('Ctrl Pts',(-34.9270086222703,-65.3765499573019,
0.));
#73829=CARTESIAN_POINT('Ctrl Pts',(-34.92891637177,-65.4039562911254,0.));
#73830=CARTESIAN_POINT('Ctrl Pts',(-34.9305324724386,-65.4274804996405,
0.));
#73831=CARTESIAN_POINT('Ctrl Pts',(-34.9317593813103,-65.4455359574999,
0.));
#73832=CARTESIAN_POINT('Ctrl Pts',(-34.9326070346592,-65.4581063193583,
0.));
#73833=CARTESIAN_POINT('Ctrl Pts',(-34.9330820191484,-65.4651808010451,
0.));
#73834=CARTESIAN_POINT('Ctrl Pts',(-34.9331875523085,-65.4667541477954,
0.));
#73835=CARTESIAN_POINT('',(-34.2579614092497,-61.0441813777723,12.));
#73836=CARTESIAN_POINT('',(-34.2579614092497,-61.0441813777723,0.));
#73837=CARTESIAN_POINT('Ctrl Pts',(-34.9331875523085,-65.4667541477954,
12.));
#73838=CARTESIAN_POINT('Ctrl Pts',(-34.9330820191484,-65.4651808010451,
12.));
#73839=CARTESIAN_POINT('Ctrl Pts',(-34.9326070346592,-65.4581063193583,
12.));
#73840=CARTESIAN_POINT('Ctrl Pts',(-34.9317593813103,-65.4455359574999,
12.));
#73841=CARTESIAN_POINT('Ctrl Pts',(-34.9305324724386,-65.4274804996405,
12.));
#73842=CARTESIAN_POINT('Ctrl Pts',(-34.92891637177,-65.4039562911254,12.));
#73843=CARTESIAN_POINT('Ctrl Pts',(-34.9270086222703,-65.3765499573019,
12.));
#73844=CARTESIAN_POINT('Ctrl Pts',(-34.9250785073473,-65.3491806440529,
12.));
#73845=CARTESIAN_POINT('Ctrl Pts',(-34.9231260731846,-65.3218484271941,
12.));
#73846=CARTESIAN_POINT('Ctrl Pts',(-34.921151369138,-65.2945533863812,12.));
#73847=CARTESIAN_POINT('Ctrl Pts',(-34.9191544474898,-65.2672956048121,
12.));
#73848=CARTESIAN_POINT('Ctrl Pts',(-34.9171353624131,-65.2400751679586,
12.));
#73849=CARTESIAN_POINT('Ctrl Pts',(-34.9150941691754,-65.2128921625837,
12.));
#73850=CARTESIAN_POINT('Ctrl Pts',(-34.9130309233017,-65.1857466757082,
12.));
#73851=CARTESIAN_POINT('Ctrl Pts',(-34.9109456796201,-65.1586387934216,
12.));
#73852=CARTESIAN_POINT('Ctrl Pts',(-34.9088384918322,-65.1315686003485,
12.));
#73853=CARTESIAN_POINT('Ctrl Pts',(-34.9067094130387,-65.1045361803097,
12.));
#73854=CARTESIAN_POINT('Ctrl Pts',(-34.9045584960503,-65.0775416167073,
12.));
#73855=CARTESIAN_POINT('Ctrl Pts',(-34.9023857937866,-65.0505849930172,
12.));
#73856=CARTESIAN_POINT('Ctrl Pts',(-34.9001913596422,-65.0236663932338,
12.));
#73857=CARTESIAN_POINT('Ctrl Pts',(-34.8979752478623,-64.9967859023225,
12.));
#73858=CARTESIAN_POINT('Ctrl Pts',(-34.8957375133702,-64.9699436060178,
12.));
#73859=CARTESIAN_POINT('Ctrl Pts',(-34.8934782116097,-64.943139590634,12.));
#73860=CARTESIAN_POINT('Ctrl Pts',(-34.8911973983785,-64.9163739428606,
12.));
#73861=CARTESIAN_POINT('Ctrl Pts',(-34.888895129681,-64.8896467495754,12.));
#73862=CARTESIAN_POINT('Ctrl Pts',(-34.8865714615433,-64.8629580976057,
12.));
#73863=CARTESIAN_POINT('Ctrl Pts',(-34.8842264500184,-64.8363080737369,
12.));
#73864=CARTESIAN_POINT('Ctrl Pts',(-34.8818601512726,-64.8096967648299,
12.));
#73865=CARTESIAN_POINT('Ctrl Pts',(-34.8794726216511,-64.7831242579023,
12.));
#73866=CARTESIAN_POINT('Ctrl Pts',(-34.8770639177494,-64.7565906402153,
12.));
#73867=CARTESIAN_POINT('Ctrl Pts',(-34.8746340964977,-64.7300959993662,
12.));
#73868=CARTESIAN_POINT('Ctrl Pts',(-34.8721832151982,-64.7036404233319,
12.));
#73869=CARTESIAN_POINT('Ctrl Pts',(-34.8697113314797,-64.6772240004241,
12.));
#73870=CARTESIAN_POINT('Ctrl Pts',(-34.8672185032725,-64.6508468192609,
12.));
#73871=CARTESIAN_POINT('Ctrl Pts',(-34.8647047887774,-64.6245089687276,
12.));
#73872=CARTESIAN_POINT('Ctrl Pts',(-34.8621702464397,-64.5982105379374,
12.));
#73873=CARTESIAN_POINT('Ctrl Pts',(-34.8596149349251,-64.5719516161913,
12.));
#73874=CARTESIAN_POINT('Ctrl Pts',(-34.8570389131334,-64.5457322930074,
12.));
#73875=CARTESIAN_POINT('Ctrl Pts',(-34.8544422402114,-64.5195526581398,
12.));
#73876=CARTESIAN_POINT('Ctrl Pts',(-34.851824975568,-64.4934128015983,12.));
#73877=CARTESIAN_POINT('Ctrl Pts',(-34.8491871788899,-64.4673128136631,
12.));
#73878=CARTESIAN_POINT('Ctrl Pts',(-34.8465289101626,-64.4412527848979,
12.));
#73879=CARTESIAN_POINT('Ctrl Pts',(-34.8438502296669,-64.4152328061526,
12.));
#73880=CARTESIAN_POINT('Ctrl Pts',(-34.8411511979705,-64.3892529685614,
12.));
#73881=CARTESIAN_POINT('Ctrl Pts',(-34.838431875925,-64.3633133635384,12.));
#73882=CARTESIAN_POINT('Ctrl Pts',(-34.8356923246617,-64.3374140827708,
12.));
#73883=CARTESIAN_POINT('Ctrl Pts',(-34.8329326055916,-64.3115552182056,
12.));
#73884=CARTESIAN_POINT('Ctrl Pts',(-34.8301527804052,-64.2857368620513,
12.));
#73885=CARTESIAN_POINT('Ctrl Pts',(-34.8273529110742,-64.259959106791,12.));
#73886=CARTESIAN_POINT('Ctrl Pts',(-34.8245330598559,-64.2342220451878,
12.));
#73887=CARTESIAN_POINT('Ctrl Pts',(-34.8216932892969,-64.2085257702885,
12.));
#73888=CARTESIAN_POINT('Ctrl Pts',(-34.8188336622419,-64.1828703754237,
12.));
#73889=CARTESIAN_POINT('Ctrl Pts',(-34.8159542418372,-64.1572559542084,
12.));
#73890=CARTESIAN_POINT('Ctrl Pts',(-34.8130550915284,-64.1316826005502,
12.));
#73891=CARTESIAN_POINT('Ctrl Pts',(-34.8101362750595,-64.1061504086512,
12.));
#73892=CARTESIAN_POINT('Ctrl Pts',(-34.8071978564748,-64.0806594730084,
12.));
#73893=CARTESIAN_POINT('Ctrl Pts',(-34.8042399001215,-64.05520988841,12.));
#73894=CARTESIAN_POINT('Ctrl Pts',(-34.8012624706534,-64.0298017499304,
12.));
#73895=CARTESIAN_POINT('Ctrl Pts',(-34.79826563303,-64.0044351529413,12.));
#73896=CARTESIAN_POINT('Ctrl Pts',(-34.7952494525182,-63.9791101931169,
12.));
#73897=CARTESIAN_POINT('Ctrl Pts',(-34.7922139946943,-63.9538269664365,
12.));
#73898=CARTESIAN_POINT('Ctrl Pts',(-34.7891593254485,-63.9285855691838,
12.));
#73899=CARTESIAN_POINT('Ctrl Pts',(-34.7860855109908,-63.9033860979428,
12.));
#73900=CARTESIAN_POINT('Ctrl Pts',(-34.7829926178495,-63.8782286496059,
12.));
#73901=CARTESIAN_POINT('Ctrl Pts',(-34.7798807128716,-63.8531133213794,
12.));
#73902=CARTESIAN_POINT('Ctrl Pts',(-34.7767498632244,-63.8280402107858,
12.));
#73903=CARTESIAN_POINT('Ctrl Pts',(-34.7736001363991,-63.8030094156635,
12.));
#73904=CARTESIAN_POINT('Ctrl Pts',(-34.7704316002165,-63.7780210341618,
12.));
#73905=CARTESIAN_POINT('Ctrl Pts',(-34.7672443228267,-63.7530751647478,
12.));
#73906=CARTESIAN_POINT('Ctrl Pts',(-34.7640383727094,-63.7281719062135,
12.));
#73907=CARTESIAN_POINT('Ctrl Pts',(-34.7608138186758,-63.7033113576782,
12.));
#73908=CARTESIAN_POINT('Ctrl Pts',(-34.7575707298718,-63.6784936185893,
12.));
#73909=CARTESIAN_POINT('Ctrl Pts',(-34.7543091757842,-63.6537187887174,
12.));
#73910=CARTESIAN_POINT('Ctrl Pts',(-34.7510292262415,-63.628986968162,12.));
#73911=CARTESIAN_POINT('Ctrl Pts',(-34.7477309514142,-63.6042982573598,
12.));
#73912=CARTESIAN_POINT('Ctrl Pts',(-34.7444144218162,-63.5796527570874,
12.));
#73913=CARTESIAN_POINT('Ctrl Pts',(-34.7410797083079,-63.5550505684621,
12.));
#73914=CARTESIAN_POINT('Ctrl Pts',(-34.7377268821022,-63.5304917929378,
12.));
#73915=CARTESIAN_POINT('Ctrl Pts',(-34.7343560147663,-63.5059765323082,
12.));
#73916=CARTESIAN_POINT('Ctrl Pts',(-34.7309671782212,-63.481504888716,12.));
#73917=CARTESIAN_POINT('Ctrl Pts',(-34.7275604447439,-63.4570769646568,
12.));
#73918=CARTESIAN_POINT('Ctrl Pts',(-34.7241358869702,-63.4326928629796,
12.));
#73919=CARTESIAN_POINT('Ctrl Pts',(-34.7206935779007,-63.4083526868837,
12.));
#73920=CARTESIAN_POINT('Ctrl Pts',(-34.7172335909037,-63.3840565399206,
12.));
#73921=CARTESIAN_POINT('Ctrl Pts',(-34.7137559997143,-63.3598045260049,
12.));
#73922=CARTESIAN_POINT('Ctrl Pts',(-34.7102608784373,-63.3355967494169,
12.));
#73923=CARTESIAN_POINT('Ctrl Pts',(-34.7067483015492,-63.311433314805,12.));
#73924=CARTESIAN_POINT('Ctrl Pts',(-34.7032183439045,-63.2873143271812,
12.));
#73925=CARTESIAN_POINT('Ctrl Pts',(-34.6996710807384,-63.2632398919234,
12.));
#73926=CARTESIAN_POINT('Ctrl Pts',(-34.6961065876671,-63.2392101147853,
12.));
#73927=CARTESIAN_POINT('Ctrl Pts',(-34.6925249406899,-63.2152251019014,
12.));
#73928=CARTESIAN_POINT('Ctrl Pts',(-34.6889262161923,-63.1912849597885,
12.));
#73929=CARTESIAN_POINT('Ctrl Pts',(-34.6853104909516,-63.1673897953425,
12.));
#73930=CARTESIAN_POINT('Ctrl Pts',(-34.6816778421401,-63.1435397158385,
12.));
#73931=CARTESIAN_POINT('Ctrl Pts',(-34.6780283473252,-63.119734828943,12.));
#73932=CARTESIAN_POINT('Ctrl Pts',(-34.6743620844722,-63.0959752427169,
12.));
#73933=CARTESIAN_POINT('Ctrl Pts',(-34.6706791319471,-63.0722610656194,
12.));
#73934=CARTESIAN_POINT('Ctrl Pts',(-34.6669795685225,-63.0485924065039,
12.));
#73935=CARTESIAN_POINT('Ctrl Pts',(-34.6632634733819,-63.0249693746198,
12.));
#73936=CARTESIAN_POINT('Ctrl Pts',(-34.6595309261186,-63.0013920796225,
12.));
#73937=CARTESIAN_POINT('Ctrl Pts',(-34.655782006739,-62.9778606315777,12.));
#73938=CARTESIAN_POINT('Ctrl Pts',(-34.6520167956657,-62.9543751409647,
12.));
#73939=CARTESIAN_POINT('Ctrl Pts',(-34.6482353737434,-62.9309357186733,
12.));
#73940=CARTESIAN_POINT('Ctrl Pts',(-34.6444378222425,-62.9075424760042,
12.));
#73941=CARTESIAN_POINT('Ctrl Pts',(-34.6406242228606,-62.8841955246819,
12.));
#73942=CARTESIAN_POINT('Ctrl Pts',(-34.6367946577241,-62.8608949768583,
12.));
#73943=CARTESIAN_POINT('Ctrl Pts',(-34.6329492093932,-62.8376409451167,
12.));
#73944=CARTESIAN_POINT('Ctrl Pts',(-34.629087960866,-62.8144335424671,12.));
#73945=CARTESIAN_POINT('Ctrl Pts',(-34.6252109955836,-62.7912728823482,
12.));
#73946=CARTESIAN_POINT('Ctrl Pts',(-34.6213183974303,-62.7681590786398,
12.));
#73947=CARTESIAN_POINT('Ctrl Pts',(-34.6174102507368,-62.7450922456662,
12.));
#73948=CARTESIAN_POINT('Ctrl Pts',(-34.6134866402842,-62.7220724982005,
12.));
#73949=CARTESIAN_POINT('Ctrl Pts',(-34.6095476513095,-62.6990999514597,
12.));
#73950=CARTESIAN_POINT('Ctrl Pts',(-34.6055933695093,-62.6761747211081,
12.));
#73951=CARTESIAN_POINT('Ctrl Pts',(-34.6016238810419,-62.6532969232695,
12.));
#73952=CARTESIAN_POINT('Ctrl Pts',(-34.5976392725303,-62.6304666745319,
12.));
#73953=CARTESIAN_POINT('Ctrl Pts',(-34.5936396310671,-62.6076840919521,
12.));
#73954=CARTESIAN_POINT('Ctrl Pts',(-34.5896250442199,-62.5849492930501,
12.));
#73955=CARTESIAN_POINT('Ctrl Pts',(-34.5855956000344,-62.5622623958125,
12.));
#73956=CARTESIAN_POINT('Ctrl Pts',(-34.5815513870363,-62.5396235187053,
12.));
#73957=CARTESIAN_POINT('Ctrl Pts',(-34.5774924942351,-62.5170327806774,
12.));
#73958=CARTESIAN_POINT('Ctrl Pts',(-34.5734190111279,-62.494490301164,12.));
#73959=CARTESIAN_POINT('Ctrl Pts',(-34.5693310277064,-62.4719962000829,
12.));
#73960=CARTESIAN_POINT('Ctrl Pts',(-34.5652286344606,-62.4495505978415,
12.));
#73961=CARTESIAN_POINT('Ctrl Pts',(-34.5611119223807,-62.4271536153473,
12.));
#73962=CARTESIAN_POINT('Ctrl Pts',(-34.5569809829615,-62.4048053740129,
12.));
#73963=CARTESIAN_POINT('Ctrl Pts',(-34.552835908207,-62.3825059957593,12.));
#73964=CARTESIAN_POINT('Ctrl Pts',(-34.5486767906376,-62.3602556030114,
12.));
#73965=CARTESIAN_POINT('Ctrl Pts',(-34.5445037232928,-62.3380543187067,
12.));
#73966=CARTESIAN_POINT('Ctrl Pts',(-34.5403167997333,-62.3159022663052,
12.));
#73967=CARTESIAN_POINT('Ctrl Pts',(-34.536116114045,-62.2937995697927,12.));
#73968=CARTESIAN_POINT('Ctrl Pts',(-34.5319017608435,-62.2717463536828,
12.));
#73969=CARTESIAN_POINT('Ctrl Pts',(-34.527673835281,-62.2497427430136,12.));
#73970=CARTESIAN_POINT('Ctrl Pts',(-34.5234324330492,-62.2277888633576,
12.));
#73971=CARTESIAN_POINT('Ctrl Pts',(-34.5191776503843,-62.2058848408346,
12.));
#73972=CARTESIAN_POINT('Ctrl Pts',(-34.514909584073,-62.184030802117,12.));
#73973=CARTESIAN_POINT('Ctrl Pts',(-34.5106283314594,-62.1622268744337,
12.));
#73974=CARTESIAN_POINT('Ctrl Pts',(-34.5063339904533,-62.1404731855687,
12.));
#73975=CARTESIAN_POINT('Ctrl Pts',(-34.5020266595293,-62.1187698638707,
12.));
#73976=CARTESIAN_POINT('Ctrl Pts',(-34.4977064377282,-62.0971170382567,
12.));
#73977=CARTESIAN_POINT('Ctrl Pts',(-34.4933734246593,-62.0755148382135,
12.));
#73978=CARTESIAN_POINT('Ctrl Pts',(-34.489027720504,-62.0539633937939,12.));
#73979=CARTESIAN_POINT('Ctrl Pts',(-34.48466942602,-62.0324628356141,12.));
#73980=CARTESIAN_POINT('Ctrl Pts',(-34.4802986425528,-62.0110132948794,
12.));
#73981=CARTESIAN_POINT('Ctrl Pts',(-34.4759154720473,-61.9896149034001,
12.));
#73982=CARTESIAN_POINT('Ctrl Pts',(-34.4715200170592,-61.9682677936053,
12.));
#73983=CARTESIAN_POINT('Ctrl Pts',(-34.4671123807717,-61.9469720985531,
12.));
#73984=CARTESIAN_POINT('Ctrl Pts',(-34.4626926669975,-61.9257279519308,
12.));
#73985=CARTESIAN_POINT('Ctrl Pts',(-34.4582609801637,-61.9045354880444,
12.));
#73986=CARTESIAN_POINT('Ctrl Pts',(-34.4538174253012,-61.8833948418025,
12.));
#73987=CARTESIAN_POINT('Ctrl Pts',(-34.4493621080361,-61.8623061487018,
12.));
#73988=CARTESIAN_POINT('Ctrl Pts',(-34.444895134574,-61.8412695447926,12.));
#73989=CARTESIAN_POINT('Ctrl Pts',(-34.4404166117299,-61.8202851667222,
12.));
#73990=CARTESIAN_POINT('Ctrl Pts',(-34.4359266469749,-61.7993531518036,
12.));
#73991=CARTESIAN_POINT('Ctrl Pts',(-34.4314253484792,-61.7784736380727,
12.));
#73992=CARTESIAN_POINT('Ctrl Pts',(-34.4269128251577,-61.7576467643432,
12.));
#73993=CARTESIAN_POINT('Ctrl Pts',(-34.422389186718,-61.7368726702596,12.));
#73994=CARTESIAN_POINT('Ctrl Pts',(-34.4178545435767,-61.7161514961914,
12.));
#73995=CARTESIAN_POINT('Ctrl Pts',(-34.4133090067704,-61.695483383117,12.));
#73996=CARTESIAN_POINT('Ctrl Pts',(-34.4087526878812,-61.6748684725205,
12.));
#73997=CARTESIAN_POINT('Ctrl Pts',(-34.4041856989317,-61.6543069062416,
12.));
#73998=CARTESIAN_POINT('Ctrl Pts',(-34.3996081523753,-61.6337988264556,
12.));
#73999=CARTESIAN_POINT('Ctrl Pts',(-34.3950201613432,-61.6133443760142,
12.));
#74000=CARTESIAN_POINT('Ctrl Pts',(-34.3904218398637,-61.5929436987409,
12.));
#74001=CARTESIAN_POINT('Ctrl Pts',(-34.3858133030518,-61.5725969396829,
12.));
#74002=CARTESIAN_POINT('Ctrl Pts',(-34.3811946674197,-61.5523042455158,
12.));
#74003=CARTESIAN_POINT('Ctrl Pts',(-34.376566050668,-61.5320657642638,12.));
#74004=CARTESIAN_POINT('Ctrl Pts',(-34.3719275711195,-61.5118816445437,
12.));
#74005=CARTESIAN_POINT('Ctrl Pts',(-34.3672793472466,-61.4917520349278,
12.));
#74006=CARTESIAN_POINT('Ctrl Pts',(-34.3626214971889,-61.4716770832896,
12.));
#74007=CARTESIAN_POINT('Ctrl Pts',(-34.3579541381996,-61.4516569360454,
12.));
#74008=CARTESIAN_POINT('Ctrl Pts',(-34.3532773877089,-61.4316917395918,
12.));
#74009=CARTESIAN_POINT('Ctrl Pts',(-34.3485913645979,-61.4117816420228,
12.));
#74010=CARTESIAN_POINT('Ctrl Pts',(-34.3438961902405,-61.3919267945302,
12.));
#74011=CARTESIAN_POINT('Ctrl Pts',(-34.339191990014,-61.3721273534256,12.));
#74012=CARTESIAN_POINT('Ctrl Pts',(-34.3344788934363,-61.3523834803188,
12.));
#74013=CARTESIAN_POINT('Ctrl Pts',(-34.3297570310146,-61.3326953378851,
12.));
#74014=CARTESIAN_POINT('Ctrl Pts',(-34.3250265314768,-61.3130630861386,
12.));
#74015=CARTESIAN_POINT('Ctrl Pts',(-34.3202875193618,-61.2934868791854,
12.));
#74016=CARTESIAN_POINT('Ctrl Pts',(-34.3155401111747,-61.2739668600365,
12.));
#74017=CARTESIAN_POINT('Ctrl Pts',(-34.3107844191044,-61.2545031656133,
12.));
#74018=CARTESIAN_POINT('Ctrl Pts',(-34.3060205584065,-61.2350959366939,
12.));
#74019=CARTESIAN_POINT('Ctrl Pts',(-34.3012486533474,-61.2157453259107,
12.));
#74020=CARTESIAN_POINT('Ctrl Pts',(-34.2964688443663,-61.1964515073891,
12.));
#74021=CARTESIAN_POINT('Ctrl Pts',(-34.2916812929751,-61.1772146833205,
12.));
#74022=CARTESIAN_POINT('Ctrl Pts',(-34.2868861666384,-61.1580350635532,
12.));
#74023=CARTESIAN_POINT('Ctrl Pts',(-34.282083624447,-61.1389128461885,12.));
#74024=CARTESIAN_POINT('Ctrl Pts',(-34.2772738038771,-61.1198481997764,
12.));
#74025=CARTESIAN_POINT('Ctrl Pts',(-34.2724568037228,-61.1008412399997,
12.));
#74026=CARTESIAN_POINT('Ctrl Pts',(-34.2676326825626,-61.0818920286293,
12.));
#74027=CARTESIAN_POINT('Ctrl Pts',(-34.2637677131935,-61.0667788793266,
12.));
#74028=CARTESIAN_POINT('Ctrl Pts',(-34.2608658001631,-61.0554700176998,
12.));
#74029=CARTESIAN_POINT('Ctrl Pts',(-34.2589297755434,-61.0479423318725,
12.));
#74030=CARTESIAN_POINT('Ctrl Pts',(-34.2579614092497,-61.0441813777723,
12.));
#74031=CARTESIAN_POINT('Ctrl Pts',(-33.590372266528,-66.1657795405962,-5.55111512312578E-16));
#74032=CARTESIAN_POINT('Ctrl Pts',(-33.590372266528,-66.1657795405962,4.));
#74033=CARTESIAN_POINT('Ctrl Pts',(-33.590372266528,-66.1657795405962,8.));
#74034=CARTESIAN_POINT('Ctrl Pts',(-33.590372266528,-66.1657795405962,12.));
#74035=CARTESIAN_POINT('Ctrl Pts',(-33.6759628819919,-66.2346881970582,
-5.55111512312578E-16));
#74036=CARTESIAN_POINT('Ctrl Pts',(-33.6759628819919,-66.2346881970582,
4.));
#74037=CARTESIAN_POINT('Ctrl Pts',(-33.675962881992,-66.2346881970582,8.));
#74038=CARTESIAN_POINT('Ctrl Pts',(-33.675962881992,-66.2346881970582,12.));
#74039=CARTESIAN_POINT('Ctrl Pts',(-33.8665453669335,-66.3036153738448,
-5.55111512312578E-16));
#74040=CARTESIAN_POINT('Ctrl Pts',(-33.8665453669335,-66.3036153738448,
4.));
#74041=CARTESIAN_POINT('Ctrl Pts',(-33.8665453669334,-66.3036153738447,
8.));
#74042=CARTESIAN_POINT('Ctrl Pts',(-33.8665453669334,-66.3036153738447,
12.));
#74043=CARTESIAN_POINT('Ctrl Pts',(-34.0597557125863,-66.2585076236406,
-5.55111512312578E-16));
#74044=CARTESIAN_POINT('Ctrl Pts',(-34.0597557125863,-66.2585076236406,
4.));
#74045=CARTESIAN_POINT('Ctrl Pts',(-34.0597557125862,-66.2585076236405,
8.));
#74046=CARTESIAN_POINT('Ctrl Pts',(-34.0597557125862,-66.2585076236405,
12.));
#74047=CARTESIAN_POINT('Ctrl Pts',(-34.1330090612018,-66.2207497120656,
-5.55111512312578E-16));
#74048=CARTESIAN_POINT('Ctrl Pts',(-34.1330090612018,-66.2207497120656,
4.));
#74049=CARTESIAN_POINT('Ctrl Pts',(-34.1330090612017,-66.2207497120656,
8.));
#74050=CARTESIAN_POINT('Ctrl Pts',(-34.1330090612017,-66.2207497120656,
12.));
#74051=CARTESIAN_POINT('',(-33.590372266528,-66.1657795405962,-2.77555756156289E-16));
#74052=CARTESIAN_POINT('',(-34.1330090612014,-66.2207497120649,2.77555756156289E-16));
#74053=CARTESIAN_POINT('Ctrl Pts',(-33.590372266528,-66.1657795405962,-5.44214888274584E-16));
#74054=CARTESIAN_POINT('Ctrl Pts',(-33.6759628819919,-66.2346881970582,
-5.44214888274584E-16));
#74055=CARTESIAN_POINT('Ctrl Pts',(-33.7848671591014,-66.274075155222,-5.44214888274584E-16));
#74056=CARTESIAN_POINT('Ctrl Pts',(-33.8946295131778,-66.2762262188581,
-5.44214888274584E-16));
#74057=CARTESIAN_POINT('Ctrl Pts',(-33.9769512787351,-66.2778395165852,
-5.44214888274584E-16));
#74058=CARTESIAN_POINT('Ctrl Pts',(-34.0597557125863,-66.2585076236406,
-5.44214888274584E-16));
#74059=CARTESIAN_POINT('Ctrl Pts',(-34.1330090612018,-66.2207497120656,
-5.44214888274584E-16));
#74060=CARTESIAN_POINT('',(-34.1330090612013,-66.2207497120649,12.));
#74061=CARTESIAN_POINT('Ctrl Pts',(-34.1330090612018,-66.2207497120656,
-5.55111512312578E-16));
#74062=CARTESIAN_POINT('Ctrl Pts',(-34.1330090612018,-66.2207497120656,
4.));
#74063=CARTESIAN_POINT('Ctrl Pts',(-34.1330090612017,-66.2207497120656,
8.));
#74064=CARTESIAN_POINT('Ctrl Pts',(-34.1330090612017,-66.2207497120656,
12.));
#74065=CARTESIAN_POINT('',(-33.590372266528,-66.1657795405962,12.));
#74066=CARTESIAN_POINT('Ctrl Pts',(-34.1330090612017,-66.2207497120656,
12.));
#74067=CARTESIAN_POINT('Ctrl Pts',(-34.0597557125862,-66.2585076236405,
12.));
#74068=CARTESIAN_POINT('Ctrl Pts',(-33.976951278735,-66.2778395165851,12.));
#74069=CARTESIAN_POINT('Ctrl Pts',(-33.8946295131777,-66.2762262188581,
12.));
#74070=CARTESIAN_POINT('Ctrl Pts',(-33.7848671591014,-66.2740751552219,
12.));
#74071=CARTESIAN_POINT('Ctrl Pts',(-33.675962881992,-66.2346881970582,12.));
#74072=CARTESIAN_POINT('Ctrl Pts',(-33.590372266528,-66.1657795405962,12.));
#74073=CARTESIAN_POINT('Ctrl Pts',(-33.590372266528,-66.1657795405962,12.));
#74074=CARTESIAN_POINT('Ctrl Pts',(-33.590372266528,-66.1657795405962,8.));
#74075=CARTESIAN_POINT('Ctrl Pts',(-33.590372266528,-66.1657795405962,4.));
#74076=CARTESIAN_POINT('Ctrl Pts',(-33.590372266528,-66.1657795405962,-5.55111512312578E-16));
#74077=CARTESIAN_POINT('Origin',(-1.72995545227681E-10,-3.3253631270614E-10,
0.));
#74078=CARTESIAN_POINT('Origin',(-1.72995545227681E-10,-3.3253631270614E-10,
12.));
#74079=CARTESIAN_POINT('Origin',(-1.72995545227681E-10,-3.3253631270614E-10,
0.));
#74080=CARTESIAN_POINT('Ctrl Pts',(-40.2823469776966,-62.6704278106386,
0.));
#74081=CARTESIAN_POINT('Ctrl Pts',(-40.2823469776966,-62.6704278106386,
4.));
#74082=CARTESIAN_POINT('Ctrl Pts',(-40.2823469776966,-62.6704278106386,
8.));
#74083=CARTESIAN_POINT('Ctrl Pts',(-40.2823469776966,-62.6704278106386,
12.));
#74084=CARTESIAN_POINT('Ctrl Pts',(-40.3747816242709,-62.6110140705996,
0.));
#74085=CARTESIAN_POINT('Ctrl Pts',(-40.3747816242709,-62.6110140705996,
4.));
#74086=CARTESIAN_POINT('Ctrl Pts',(-40.3747816242709,-62.6110140705997,
8.00000000000001));
#74087=CARTESIAN_POINT('Ctrl Pts',(-40.3747816242709,-62.6110140705997,
12.));
#74088=CARTESIAN_POINT('Ctrl Pts',(-40.5004281293558,-62.4519997852061,
0.));
#74089=CARTESIAN_POINT('Ctrl Pts',(-40.5004281293558,-62.4519997852061,
4.));
#74090=CARTESIAN_POINT('Ctrl Pts',(-40.5004281293557,-62.4519997852062,
7.99999999999999));
#74091=CARTESIAN_POINT('Ctrl Pts',(-40.5004281293557,-62.4519997852062,
12.));
#74092=CARTESIAN_POINT('Ctrl Pts',(-40.5187208145706,-62.2544389573114,
0.));
#74093=CARTESIAN_POINT('Ctrl Pts',(-40.5187208145706,-62.2544389573114,
4.));
#74094=CARTESIAN_POINT('Ctrl Pts',(-40.5187208145705,-62.2544389573115,
8.00000000000001));
#74095=CARTESIAN_POINT('Ctrl Pts',(-40.5187208145705,-62.2544389573115,
12.));
#74096=CARTESIAN_POINT('Ctrl Pts',(-40.506059810084,-62.173005475645,0.));
#74097=CARTESIAN_POINT('Ctrl Pts',(-40.506059810084,-62.173005475645,4.));
#74098=CARTESIAN_POINT('Ctrl Pts',(-40.5060598100839,-62.1730054756452,
8.));
#74099=CARTESIAN_POINT('Ctrl Pts',(-40.5060598100839,-62.1730054756452,
12.));
#74100=CARTESIAN_POINT('',(-40.2823469776966,-62.6704278106386,0.));
#74101=CARTESIAN_POINT('',(-40.5060598100838,-62.1730054756451,0.));
#74102=CARTESIAN_POINT('Ctrl Pts',(-40.2823469776966,-62.6704278106386,
0.));
#74103=CARTESIAN_POINT('Ctrl Pts',(-40.3747816242709,-62.6110140705996,
0.));
#74104=CARTESIAN_POINT('Ctrl Pts',(-40.4465796271766,-62.5201487646605,
0.));
#74105=CARTESIAN_POINT('Ctrl Pts',(-40.4833233215532,-62.4166968325985,
0.));
#74106=CARTESIAN_POINT('Ctrl Pts',(-40.5108810923357,-62.339107883552,0.));
#74107=CARTESIAN_POINT('Ctrl Pts',(-40.5187208145706,-62.2544389573114,
0.));
#74108=CARTESIAN_POINT('Ctrl Pts',(-40.506059810084,-62.173005475645,0.));
#74109=CARTESIAN_POINT('',(-40.5060598100838,-62.1730054756452,12.));
#74110=CARTESIAN_POINT('Ctrl Pts',(-40.506059810084,-62.173005475645,0.));
#74111=CARTESIAN_POINT('Ctrl Pts',(-40.506059810084,-62.173005475645,4.));
#74112=CARTESIAN_POINT('Ctrl Pts',(-40.5060598100839,-62.1730054756452,
8.));
#74113=CARTESIAN_POINT('Ctrl Pts',(-40.5060598100839,-62.1730054756452,
12.));
#74114=CARTESIAN_POINT('',(-40.2823469776966,-62.6704278106386,12.));
#74115=CARTESIAN_POINT('Ctrl Pts',(-40.5060598100839,-62.1730054756452,
12.));
#74116=CARTESIAN_POINT('Ctrl Pts',(-40.5187208145705,-62.2544389573115,
12.));
#74117=CARTESIAN_POINT('Ctrl Pts',(-40.5108810923356,-62.3391078835521,
12.));
#74118=CARTESIAN_POINT('Ctrl Pts',(-40.4833233215531,-62.4166968325986,
12.));
#74119=CARTESIAN_POINT('Ctrl Pts',(-40.4465796271765,-62.5201487646605,
12.));
#74120=CARTESIAN_POINT('Ctrl Pts',(-40.3747816242709,-62.6110140705997,
12.));
#74121=CARTESIAN_POINT('Ctrl Pts',(-40.2823469776966,-62.6704278106386,
12.));
#74122=CARTESIAN_POINT('Ctrl Pts',(-40.2823469776966,-62.6704278106386,
12.));
#74123=CARTESIAN_POINT('Ctrl Pts',(-40.2823469776966,-62.6704278106386,
8.));
#74124=CARTESIAN_POINT('Ctrl Pts',(-40.2823469776966,-62.6704278106386,
4.));
#74125=CARTESIAN_POINT('Ctrl Pts',(-40.2823469776966,-62.6704278106386,
0.));
#74126=CARTESIAN_POINT('Ctrl Pts',(-39.4479504917287,-57.8261117662438,
0.));
#74127=CARTESIAN_POINT('Ctrl Pts',(-39.4479504917287,-57.8261117662438,
12.));
#74128=CARTESIAN_POINT('Ctrl Pts',(-39.4492429618443,-57.8297740100947,
0.));
#74129=CARTESIAN_POINT('Ctrl Pts',(-39.4492429618443,-57.8297740100947,
12.));
#74130=CARTESIAN_POINT('Ctrl Pts',(-39.4518277003553,-57.837104315141,0.));
#74131=CARTESIAN_POINT('Ctrl Pts',(-39.4518277003553,-57.837104315141,12.));
#74132=CARTESIAN_POINT('Ctrl Pts',(-39.4557042029652,-57.8481172247495,
0.));
#74133=CARTESIAN_POINT('Ctrl Pts',(-39.4557042029652,-57.8481172247495,
12.));
#74134=CARTESIAN_POINT('Ctrl Pts',(-39.4608716627118,-57.8628360096803,
0.));
#74135=CARTESIAN_POINT('Ctrl Pts',(-39.4608716627118,-57.8628360096803,
12.));
#74136=CARTESIAN_POINT('Ctrl Pts',(-39.4673289592259,-57.8812926637177,
0.));
#74137=CARTESIAN_POINT('Ctrl Pts',(-39.4673289592259,-57.8812926637177,
12.));
#74138=CARTESIAN_POINT('Ctrl Pts',(-39.473784194937,-57.8998074670478,0.));
#74139=CARTESIAN_POINT('Ctrl Pts',(-39.473784194937,-57.8998074670478,12.));
#74140=CARTESIAN_POINT('Ctrl Pts',(-39.4802373061058,-57.9183803632403,
0.));
#74141=CARTESIAN_POINT('Ctrl Pts',(-39.4802373061058,-57.9183803632403,
12.));
#74142=CARTESIAN_POINT('Ctrl Pts',(-39.4866881842317,-57.937011245663,0.));
#74143=CARTESIAN_POINT('Ctrl Pts',(-39.4866881842317,-57.937011245663,12.));
#74144=CARTESIAN_POINT('Ctrl Pts',(-39.4931366776714,-57.9556999583892,
0.));
#74145=CARTESIAN_POINT('Ctrl Pts',(-39.4931366776714,-57.9556999583892,
12.));
#74146=CARTESIAN_POINT('Ctrl Pts',(-39.499582610674,-57.974446317937,0.));
#74147=CARTESIAN_POINT('Ctrl Pts',(-39.499582610674,-57.974446317937,12.));
#74148=CARTESIAN_POINT('Ctrl Pts',(-39.5060257981225,-57.9932501298522,
0.));
#74149=CARTESIAN_POINT('Ctrl Pts',(-39.5060257981225,-57.9932501298522,
12.));
#74150=CARTESIAN_POINT('Ctrl Pts',(-39.5124660614976,-58.0121112067895,
0.));
#74151=CARTESIAN_POINT('Ctrl Pts',(-39.5124660614976,-58.0121112067895,
12.));
#74152=CARTESIAN_POINT('Ctrl Pts',(-39.5189032457184,-58.0310293875262,
0.));
#74153=CARTESIAN_POINT('Ctrl Pts',(-39.5189032457184,-58.0310293875262,
12.));
#74154=CARTESIAN_POINT('Ctrl Pts',(-39.5253372136887,-58.0500045308412,
0.));
#74155=CARTESIAN_POINT('Ctrl Pts',(-39.5253372136887,-58.0500045308412,
12.));
#74156=CARTESIAN_POINT('Ctrl Pts',(-39.5317678383217,-58.0690365065374,
0.));
#74157=CARTESIAN_POINT('Ctrl Pts',(-39.5317678383217,-58.0690365065374,
12.));
#74158=CARTESIAN_POINT('Ctrl Pts',(-39.5381949959221,-58.088125187992,0.));
#74159=CARTESIAN_POINT('Ctrl Pts',(-39.5381949959221,-58.088125187992,12.));
#74160=CARTESIAN_POINT('Ctrl Pts',(-39.5446185579638,-58.1072704428928,
0.));
#74161=CARTESIAN_POINT('Ctrl Pts',(-39.5446185579638,-58.1072704428928,
12.));
#74162=CARTESIAN_POINT('Ctrl Pts',(-39.5510383869505,-58.126472128574,0.));
#74163=CARTESIAN_POINT('Ctrl Pts',(-39.5510383869505,-58.126472128574,12.));
#74164=CARTESIAN_POINT('Ctrl Pts',(-39.5574543406982,-58.1457300968499,
0.));
#74165=CARTESIAN_POINT('Ctrl Pts',(-39.5574543406982,-58.1457300968499,
12.));
#74166=CARTESIAN_POINT('Ctrl Pts',(-39.563866275018,-58.1650441970387,0.));
#74167=CARTESIAN_POINT('Ctrl Pts',(-39.563866275018,-58.1650441970387,12.));
#74168=CARTESIAN_POINT('Ctrl Pts',(-39.5702740467999,-58.1844142794338,
0.));
#74169=CARTESIAN_POINT('Ctrl Pts',(-39.5702740467999,-58.1844142794338,
12.));
#74170=CARTESIAN_POINT('Ctrl Pts',(-39.57667751752,-58.2038401992457,0.));
#74171=CARTESIAN_POINT('Ctrl Pts',(-39.57667751752,-58.2038401992457,12.));
#74172=CARTESIAN_POINT('Ctrl Pts',(-39.5830765530891,-58.2233218164365,
0.));
#74173=CARTESIAN_POINT('Ctrl Pts',(-39.5830765530891,-58.2233218164365,
12.));
#74174=CARTESIAN_POINT('Ctrl Pts',(-39.5894710221713,-58.2428589938369,
0.));
#74175=CARTESIAN_POINT('Ctrl Pts',(-39.5894710221713,-58.2428589938369,
12.));
#74176=CARTESIAN_POINT('Ctrl Pts',(-39.5958607950239,-58.2624515958419,
0.));
#74177=CARTESIAN_POINT('Ctrl Pts',(-39.5958607950239,-58.2624515958419,
12.));
#74178=CARTESIAN_POINT('Ctrl Pts',(-39.602245742079,-58.2820994868118,0.));
#74179=CARTESIAN_POINT('Ctrl Pts',(-39.602245742079,-58.2820994868118,12.));
#74180=CARTESIAN_POINT('Ctrl Pts',(-39.6086257327583,-58.3018025297323,
0.));
#74181=CARTESIAN_POINT('Ctrl Pts',(-39.6086257327583,-58.3018025297323,
12.));
#74182=CARTESIAN_POINT('Ctrl Pts',(-39.6150006360914,-58.3215605869221,
0.));
#74183=CARTESIAN_POINT('Ctrl Pts',(-39.6150006360914,-58.3215605869221,
12.));
#74184=CARTESIAN_POINT('Ctrl Pts',(-39.6213703212531,-58.3413735206423,
0.));
#74185=CARTESIAN_POINT('Ctrl Pts',(-39.6213703212531,-58.3413735206423,
12.));
#74186=CARTESIAN_POINT('Ctrl Pts',(-39.6277346580892,-58.3612411936904,
0.));
#74187=CARTESIAN_POINT('Ctrl Pts',(-39.6277346580892,-58.3612411936904,
12.));
#74188=CARTESIAN_POINT('Ctrl Pts',(-39.6340935177476,-58.3811634701037,
0.));
#74189=CARTESIAN_POINT('Ctrl Pts',(-39.6340935177476,-58.3811634701037,
12.));
#74190=CARTESIAN_POINT('Ctrl Pts',(-39.6404467729094,-58.4011402154196,
0.));
#74191=CARTESIAN_POINT('Ctrl Pts',(-39.6404467729094,-58.4011402154196,
12.));
#74192=CARTESIAN_POINT('Ctrl Pts',(-39.6467942974451,-58.4211712963004,
0.));
#74193=CARTESIAN_POINT('Ctrl Pts',(-39.6467942974451,-58.4211712963004,
12.));
#74194=CARTESIAN_POINT('Ctrl Pts',(-39.653135966204,-58.4412565802979,0.));
#74195=CARTESIAN_POINT('Ctrl Pts',(-39.653135966204,-58.4412565802979,12.));
#74196=CARTESIAN_POINT('Ctrl Pts',(-39.6594716547689,-58.4613959355788,
0.));
#74197=CARTESIAN_POINT('Ctrl Pts',(-39.6594716547689,-58.4613959355788,
12.));
#74198=CARTESIAN_POINT('Ctrl Pts',(-39.6658012391815,-58.4815892306066,
0.));
#74199=CARTESIAN_POINT('Ctrl Pts',(-39.6658012391815,-58.4815892306066,
12.));
#74200=CARTESIAN_POINT('Ctrl Pts',(-39.6721245959531,-58.5018363341604,
0.));
#74201=CARTESIAN_POINT('Ctrl Pts',(-39.6721245959531,-58.5018363341604,
12.));
#74202=CARTESIAN_POINT('Ctrl Pts',(-39.6784416021826,-58.522137115476,0.));
#74203=CARTESIAN_POINT('Ctrl Pts',(-39.6784416021826,-58.522137115476,12.));
#74204=CARTESIAN_POINT('Ctrl Pts',(-39.6847521356395,-58.5424914443415,
0.));
#74205=CARTESIAN_POINT('Ctrl Pts',(-39.6847521356395,-58.5424914443415,
12.));
#74206=CARTESIAN_POINT('Ctrl Pts',(-39.6910560748629,-58.5628991912052,
0.));
#74207=CARTESIAN_POINT('Ctrl Pts',(-39.6910560748629,-58.5628991912052,
12.));
#74208=CARTESIAN_POINT('Ctrl Pts',(-39.6973532992539,-58.5833602272743,
0.));
#74209=CARTESIAN_POINT('Ctrl Pts',(-39.6973532992539,-58.5833602272743,
12.));
#74210=CARTESIAN_POINT('Ctrl Pts',(-39.7036436890233,-58.6038744244659,
0.));
#74211=CARTESIAN_POINT('Ctrl Pts',(-39.7036436890233,-58.6038744244659,
12.));
#74212=CARTESIAN_POINT('Ctrl Pts',(-39.7099271251413,-58.6244416553562,
0.));
#74213=CARTESIAN_POINT('Ctrl Pts',(-39.7099271251413,-58.6244416553562,
12.));
#74214=CARTESIAN_POINT('Ctrl Pts',(-39.7162034892899,-58.6450617931274,
0.));
#74215=CARTESIAN_POINT('Ctrl Pts',(-39.7162034892899,-58.6450617931274,
12.));
#74216=CARTESIAN_POINT('Ctrl Pts',(-39.7224726638101,-58.6657347115034,
0.));
#74217=CARTESIAN_POINT('Ctrl Pts',(-39.7224726638101,-58.6657347115034,
12.));
#74218=CARTESIAN_POINT('Ctrl Pts',(-39.7287345316681,-58.6864602847088,
0.));
#74219=CARTESIAN_POINT('Ctrl Pts',(-39.7287345316681,-58.6864602847088,
12.));
#74220=CARTESIAN_POINT('Ctrl Pts',(-39.734988976475,-58.7072383875027,0.));
#74221=CARTESIAN_POINT('Ctrl Pts',(-39.734988976475,-58.7072383875027,12.));
#74222=CARTESIAN_POINT('Ctrl Pts',(-39.7412358824953,-58.7280688951916,
0.));
#74223=CARTESIAN_POINT('Ctrl Pts',(-39.7412358824953,-58.7280688951916,
12.));
#74224=CARTESIAN_POINT('Ctrl Pts',(-39.7474751346598,-58.7489516836445,
0.));
#74225=CARTESIAN_POINT('Ctrl Pts',(-39.7474751346598,-58.7489516836445,
12.));
#74226=CARTESIAN_POINT('Ctrl Pts',(-39.7537066185813,-58.7698866293029,
0.));
#74227=CARTESIAN_POINT('Ctrl Pts',(-39.7537066185813,-58.7698866293029,
12.));
#74228=CARTESIAN_POINT('Ctrl Pts',(-39.7599302205521,-58.7908736091798,
0.));
#74229=CARTESIAN_POINT('Ctrl Pts',(-39.7599302205521,-58.7908736091798,
12.));
#74230=CARTESIAN_POINT('Ctrl Pts',(-39.7661458275274,-58.8119125008517,
0.));
#74231=CARTESIAN_POINT('Ctrl Pts',(-39.7661458275274,-58.8119125008517,
12.));
#74232=CARTESIAN_POINT('Ctrl Pts',(-39.772353327112,-58.8330031824453,0.));
#74233=CARTESIAN_POINT('Ctrl Pts',(-39.772353327112,-58.8330031824453,12.));
#74234=CARTESIAN_POINT('Ctrl Pts',(-39.7785526075478,-58.8541455326231,
0.));
#74235=CARTESIAN_POINT('Ctrl Pts',(-39.7785526075478,-58.8541455326231,
12.));
#74236=CARTESIAN_POINT('Ctrl Pts',(-39.7847435576996,-58.8753394305585,
0.));
#74237=CARTESIAN_POINT('Ctrl Pts',(-39.7847435576996,-58.8753394305585,
12.));
#74238=CARTESIAN_POINT('Ctrl Pts',(-39.7909260670517,-58.8965847559391,
0.));
#74239=CARTESIAN_POINT('Ctrl Pts',(-39.7909260670517,-58.8965847559391,
12.));
#74240=CARTESIAN_POINT('Ctrl Pts',(-39.7971000257044,-58.9178813889703,
0.));
#74241=CARTESIAN_POINT('Ctrl Pts',(-39.7971000257044,-58.9178813889703,
12.));
#74242=CARTESIAN_POINT('Ctrl Pts',(-39.8032653243712,-58.9392292103747,
0.));
#74243=CARTESIAN_POINT('Ctrl Pts',(-39.8032653243712,-58.9392292103747,
12.));
#74244=CARTESIAN_POINT('Ctrl Pts',(-39.8094218543782,-58.9606281013875,
0.));
#74245=CARTESIAN_POINT('Ctrl Pts',(-39.8094218543782,-58.9606281013875,
12.));
#74246=CARTESIAN_POINT('Ctrl Pts',(-39.8155695076626,-58.9820779437484,
0.));
#74247=CARTESIAN_POINT('Ctrl Pts',(-39.8155695076626,-58.9820779437484,
12.));
#74248=CARTESIAN_POINT('Ctrl Pts',(-39.821708176766,-59.0035786197024,0.));
#74249=CARTESIAN_POINT('Ctrl Pts',(-39.821708176766,-59.0035786197024,12.));
#74250=CARTESIAN_POINT('Ctrl Pts',(-39.8278377548262,-59.0251300119973,
0.));
#74251=CARTESIAN_POINT('Ctrl Pts',(-39.8278377548262,-59.0251300119973,
12.));
#74252=CARTESIAN_POINT('Ctrl Pts',(-39.8339581355716,-59.0467320038784,
0.));
#74253=CARTESIAN_POINT('Ctrl Pts',(-39.8339581355716,-59.0467320038784,
12.));
#74254=CARTESIAN_POINT('Ctrl Pts',(-39.8400692133139,-59.0683844790764,
0.));
#74255=CARTESIAN_POINT('Ctrl Pts',(-39.8400692133139,-59.0683844790764,
12.));
#74256=CARTESIAN_POINT('Ctrl Pts',(-39.8461708829456,-59.090087321798,0.));
#74257=CARTESIAN_POINT('Ctrl Pts',(-39.8461708829456,-59.090087321798,12.));
#74258=CARTESIAN_POINT('Ctrl Pts',(-39.8522630399328,-59.1118404167292,
0.));
#74259=CARTESIAN_POINT('Ctrl Pts',(-39.8522630399328,-59.1118404167292,
12.));
#74260=CARTESIAN_POINT('Ctrl Pts',(-39.8583455803105,-59.1336436490342,
0.));
#74261=CARTESIAN_POINT('Ctrl Pts',(-39.8583455803105,-59.1336436490342,
12.));
#74262=CARTESIAN_POINT('Ctrl Pts',(-39.8644184006787,-59.1554969043522,
0.));
#74263=CARTESIAN_POINT('Ctrl Pts',(-39.8644184006787,-59.1554969043522,
12.));
#74264=CARTESIAN_POINT('Ctrl Pts',(-39.8704813981988,-59.1774000687879,
0.));
#74265=CARTESIAN_POINT('Ctrl Pts',(-39.8704813981988,-59.1774000687879,
12.));
#74266=CARTESIAN_POINT('Ctrl Pts',(-39.876534470591,-59.1993530289028,0.));
#74267=CARTESIAN_POINT('Ctrl Pts',(-39.876534470591,-59.1993530289028,12.));
#74268=CARTESIAN_POINT('Ctrl Pts',(-39.8825775161267,-59.2213556717209,
0.));
#74269=CARTESIAN_POINT('Ctrl Pts',(-39.8825775161267,-59.2213556717209,
12.));
#74270=CARTESIAN_POINT('Ctrl Pts',(-39.8886104336242,-59.2434078847247,
0.));
#74271=CARTESIAN_POINT('Ctrl Pts',(-39.8886104336242,-59.2434078847247,
12.));
#74272=CARTESIAN_POINT('Ctrl Pts',(-39.8946331224438,-59.2655095558521,
0.));
#74273=CARTESIAN_POINT('Ctrl Pts',(-39.8946331224438,-59.2655095558521,
12.));
#74274=CARTESIAN_POINT('Ctrl Pts',(-39.9006454824845,-59.2876605734846,
0.));
#74275=CARTESIAN_POINT('Ctrl Pts',(-39.9006454824845,-59.2876605734846,
12.));
#74276=CARTESIAN_POINT('Ctrl Pts',(-39.9066474141803,-59.3098608264419,
0.));
#74277=CARTESIAN_POINT('Ctrl Pts',(-39.9066474141803,-59.3098608264419,
12.));
#74278=CARTESIAN_POINT('Ctrl Pts',(-39.9126388184936,-59.3321102039852,
0.));
#74279=CARTESIAN_POINT('Ctrl Pts',(-39.9126388184936,-59.3321102039852,
12.));
#74280=CARTESIAN_POINT('Ctrl Pts',(-39.9186195969104,-59.3544085958151,
0.));
#74281=CARTESIAN_POINT('Ctrl Pts',(-39.9186195969104,-59.3544085958151,
12.));
#74282=CARTESIAN_POINT('Ctrl Pts',(-39.9245896514367,-59.3767558920675,
0.));
#74283=CARTESIAN_POINT('Ctrl Pts',(-39.9245896514367,-59.3767558920675,
12.));
#74284=CARTESIAN_POINT('Ctrl Pts',(-39.9305488845958,-59.3991519833016,
0.));
#74285=CARTESIAN_POINT('Ctrl Pts',(-39.9305488845958,-59.3991519833016,
12.));
#74286=CARTESIAN_POINT('Ctrl Pts',(-39.9364971994242,-59.4215967604967,
0.));
#74287=CARTESIAN_POINT('Ctrl Pts',(-39.9364971994242,-59.4215967604967,
12.));
#74288=CARTESIAN_POINT('Ctrl Pts',(-39.9424344994672,-59.4440901150582,
0.));
#74289=CARTESIAN_POINT('Ctrl Pts',(-39.9424344994672,-59.4440901150582,
12.));
#74290=CARTESIAN_POINT('Ctrl Pts',(-39.9483606887737,-59.4666319388133,
0.));
#74291=CARTESIAN_POINT('Ctrl Pts',(-39.9483606887737,-59.4666319388133,
12.));
#74292=CARTESIAN_POINT('Ctrl Pts',(-39.9542756718922,-59.4892221240068,
0.));
#74293=CARTESIAN_POINT('Ctrl Pts',(-39.9542756718922,-59.4892221240068,
12.));
#74294=CARTESIAN_POINT('Ctrl Pts',(-39.9601793538682,-59.511860563289,0.));
#74295=CARTESIAN_POINT('Ctrl Pts',(-39.9601793538682,-59.511860563289,12.));
#74296=CARTESIAN_POINT('Ctrl Pts',(-39.9660716402403,-59.5345471497128,
0.));
#74297=CARTESIAN_POINT('Ctrl Pts',(-39.9660716402403,-59.5345471497128,
12.));
#74298=CARTESIAN_POINT('Ctrl Pts',(-39.9719524370345,-59.5572817767388,
0.));
#74299=CARTESIAN_POINT('Ctrl Pts',(-39.9719524370345,-59.5572817767388,
12.));
#74300=CARTESIAN_POINT('Ctrl Pts',(-39.9778216507605,-59.5800643382314,
0.));
#74301=CARTESIAN_POINT('Ctrl Pts',(-39.9778216507605,-59.5800643382314,
12.));
#74302=CARTESIAN_POINT('Ctrl Pts',(-39.9836791884079,-59.6028947284562,
0.));
#74303=CARTESIAN_POINT('Ctrl Pts',(-39.9836791884079,-59.6028947284562,
12.));
#74304=CARTESIAN_POINT('Ctrl Pts',(-39.9895249574448,-59.6257728420669,
0.));
#74305=CARTESIAN_POINT('Ctrl Pts',(-39.9895249574448,-59.6257728420669,
12.));
#74306=CARTESIAN_POINT('Ctrl Pts',(-39.9953588658132,-59.6486985741041,
0.));
#74307=CARTESIAN_POINT('Ctrl Pts',(-39.9953588658132,-59.6486985741041,
12.));
#74308=CARTESIAN_POINT('Ctrl Pts',(-40.0011808219241,-59.6716718200005,
0.));
#74309=CARTESIAN_POINT('Ctrl Pts',(-40.0011808219241,-59.6716718200005,
12.));
#74310=CARTESIAN_POINT('Ctrl Pts',(-40.0069907346537,-59.6946924755773,
0.));
#74311=CARTESIAN_POINT('Ctrl Pts',(-40.0069907346537,-59.6946924755773,
12.));
#74312=CARTESIAN_POINT('Ctrl Pts',(-40.0127885133403,-59.7177604370403,
0.));
#74313=CARTESIAN_POINT('Ctrl Pts',(-40.0127885133403,-59.7177604370403,
12.));
#74314=CARTESIAN_POINT('Ctrl Pts',(-40.0185740677821,-59.7408756009679,
0.));
#74315=CARTESIAN_POINT('Ctrl Pts',(-40.0185740677821,-59.7408756009679,
12.));
#74316=CARTESIAN_POINT('Ctrl Pts',(-40.0243473082337,-59.7640378643106,
0.));
#74317=CARTESIAN_POINT('Ctrl Pts',(-40.0243473082337,-59.7640378643106,
12.));
#74318=CARTESIAN_POINT('Ctrl Pts',(-40.0301081454002,-59.7872471243942,
0.));
#74319=CARTESIAN_POINT('Ctrl Pts',(-40.0301081454002,-59.7872471243942,
12.));
#74320=CARTESIAN_POINT('Ctrl Pts',(-40.0358564904341,-59.8105032789179,
0.));
#74321=CARTESIAN_POINT('Ctrl Pts',(-40.0358564904341,-59.8105032789179,
12.));
#74322=CARTESIAN_POINT('Ctrl Pts',(-40.0415922549315,-59.8338062259492,
0.));
#74323=CARTESIAN_POINT('Ctrl Pts',(-40.0415922549315,-59.8338062259492,
12.));
#74324=CARTESIAN_POINT('Ctrl Pts',(-40.0473153509324,-59.8571558639145,
0.));
#74325=CARTESIAN_POINT('Ctrl Pts',(-40.0473153509324,-59.8571558639145,
12.));
#74326=CARTESIAN_POINT('Ctrl Pts',(-40.0530256909161,-59.8805520915972,
0.));
#74327=CARTESIAN_POINT('Ctrl Pts',(-40.0530256909161,-59.8805520915972,
12.));
#74328=CARTESIAN_POINT('Ctrl Pts',(-40.0587231877959,-59.9039948081428,
0.));
#74329=CARTESIAN_POINT('Ctrl Pts',(-40.0587231877959,-59.9039948081428,
12.));
#74330=CARTESIAN_POINT('Ctrl Pts',(-40.0644077549158,-59.927483913055,0.));
#74331=CARTESIAN_POINT('Ctrl Pts',(-40.0644077549158,-59.927483913055,12.));
#74332=CARTESIAN_POINT('Ctrl Pts',(-40.0700793060475,-59.9510193061929,
0.));
#74333=CARTESIAN_POINT('Ctrl Pts',(-40.0700793060475,-59.9510193061929,
12.));
#74334=CARTESIAN_POINT('Ctrl Pts',(-40.0757377553893,-59.974600887759,0.));
#74335=CARTESIAN_POINT('Ctrl Pts',(-40.0757377553893,-59.974600887759,12.));
#74336=CARTESIAN_POINT('Ctrl Pts',(-40.0813830175629,-59.9982285582991,
0.));
#74337=CARTESIAN_POINT('Ctrl Pts',(-40.0813830175629,-59.9982285582991,
12.));
#74338=CARTESIAN_POINT('Ctrl Pts',(-40.0870150076078,-60.0219022187066,
0.));
#74339=CARTESIAN_POINT('Ctrl Pts',(-40.0870150076078,-60.0219022187066,
12.));
#74340=CARTESIAN_POINT('Ctrl Pts',(-40.0926336409787,-60.0456217702203,
0.));
#74341=CARTESIAN_POINT('Ctrl Pts',(-40.0926336409787,-60.0456217702203,
12.));
#74342=CARTESIAN_POINT('Ctrl Pts',(-40.0982388335421,-60.0693871144207,
0.));
#74343=CARTESIAN_POINT('Ctrl Pts',(-40.0982388335421,-60.0693871144207,
12.));
#74344=CARTESIAN_POINT('Ctrl Pts',(-40.1038305015763,-60.0931981532194,
0.));
#74345=CARTESIAN_POINT('Ctrl Pts',(-40.1038305015763,-60.0931981532194,
12.));
#74346=CARTESIAN_POINT('Ctrl Pts',(-40.1094085617672,-60.1170547888572,
0.));
#74347=CARTESIAN_POINT('Ctrl Pts',(-40.1094085617672,-60.1170547888572,
12.));
#74348=CARTESIAN_POINT('Ctrl Pts',(-40.1149729312036,-60.1409569239092,
0.));
#74349=CARTESIAN_POINT('Ctrl Pts',(-40.1149729312036,-60.1409569239092,
12.));
#74350=CARTESIAN_POINT('Ctrl Pts',(-40.120523527374,-60.1649044612829,0.));
#74351=CARTESIAN_POINT('Ctrl Pts',(-40.120523527374,-60.1649044612829,12.));
#74352=CARTESIAN_POINT('Ctrl Pts',(-40.1260602681644,-60.1888973042151,
0.));
#74353=CARTESIAN_POINT('Ctrl Pts',(-40.1260602681644,-60.1888973042151,
12.));
#74354=CARTESIAN_POINT('Ctrl Pts',(-40.1315830718575,-60.2129353562617,
0.));
#74355=CARTESIAN_POINT('Ctrl Pts',(-40.1315830718575,-60.2129353562617,
12.));
#74356=CARTESIAN_POINT('Ctrl Pts',(-40.13709185713,-60.2370185212957,0.));
#74357=CARTESIAN_POINT('Ctrl Pts',(-40.13709185713,-60.2370185212957,12.));
#74358=CARTESIAN_POINT('Ctrl Pts',(-40.1425865430468,-60.2611467035109,
0.));
#74359=CARTESIAN_POINT('Ctrl Pts',(-40.1425865430468,-60.2611467035109,
12.));
#74360=CARTESIAN_POINT('Ctrl Pts',(-40.1480670490583,-60.2853198074215,
0.));
#74361=CARTESIAN_POINT('Ctrl Pts',(-40.1480670490583,-60.2853198074215,
12.));
#74362=CARTESIAN_POINT('Ctrl Pts',(-40.1535332949978,-60.3095377378589,
0.));
#74363=CARTESIAN_POINT('Ctrl Pts',(-40.1535332949978,-60.3095377378589,
12.));
#74364=CARTESIAN_POINT('Ctrl Pts',(-40.1589852010811,-60.3338003999616,
0.));
#74365=CARTESIAN_POINT('Ctrl Pts',(-40.1589852010811,-60.3338003999616,
12.));
#74366=CARTESIAN_POINT('Ctrl Pts',(-40.1644226879043,-60.3581076991731,
0.));
#74367=CARTESIAN_POINT('Ctrl Pts',(-40.1644226879043,-60.3581076991731,
12.));
#74368=CARTESIAN_POINT('Ctrl Pts',(-40.1698456764387,-60.382459541246,0.));
#74369=CARTESIAN_POINT('Ctrl Pts',(-40.1698456764387,-60.382459541246,12.));
#74370=CARTESIAN_POINT('Ctrl Pts',(-40.1752540880273,-60.4068558322414,
0.));
#74371=CARTESIAN_POINT('Ctrl Pts',(-40.1752540880273,-60.4068558322414,
12.));
#74372=CARTESIAN_POINT('Ctrl Pts',(-40.1806478443828,-60.4312964785269,
0.));
#74373=CARTESIAN_POINT('Ctrl Pts',(-40.1806478443828,-60.4312964785269,
12.));
#74374=CARTESIAN_POINT('Ctrl Pts',(-40.1860268675875,-60.4557813867677,
0.));
#74375=CARTESIAN_POINT('Ctrl Pts',(-40.1860268675875,-60.4557813867677,
12.));
#74376=CARTESIAN_POINT('Ctrl Pts',(-40.1913910800911,-60.4803104639211,
0.));
#74377=CARTESIAN_POINT('Ctrl Pts',(-40.1913910800911,-60.4803104639211,
12.));
#74378=CARTESIAN_POINT('Ctrl Pts',(-40.1967404047055,-60.5048836172423,
0.));
#74379=CARTESIAN_POINT('Ctrl Pts',(-40.1967404047055,-60.5048836172423,
12.));
#74380=CARTESIAN_POINT('Ctrl Pts',(-40.2020747646012,-60.5295007542838,
0.));
#74381=CARTESIAN_POINT('Ctrl Pts',(-40.2020747646012,-60.5295007542838,
12.));
#74382=CARTESIAN_POINT('Ctrl Pts',(-40.2073940833054,-60.5541617828927,
0.));
#74383=CARTESIAN_POINT('Ctrl Pts',(-40.2073940833054,-60.5541617828927,
12.));
#74384=CARTESIAN_POINT('Ctrl Pts',(-40.2126982847012,-60.5788666112043,
0.));
#74385=CARTESIAN_POINT('Ctrl Pts',(-40.2126982847012,-60.5788666112043,
12.));
#74386=CARTESIAN_POINT('Ctrl Pts',(-40.2179872930272,-60.6036151476347,
0.));
#74387=CARTESIAN_POINT('Ctrl Pts',(-40.2179872930272,-60.6036151476347,
12.));
#74388=CARTESIAN_POINT('Ctrl Pts',(-40.2232610328717,-60.6284073008865,
0.));
#74389=CARTESIAN_POINT('Ctrl Pts',(-40.2232610328717,-60.6284073008865,
12.));
#74390=CARTESIAN_POINT('Ctrl Pts',(-40.2285194291702,-60.6532429799493,
0.));
#74391=CARTESIAN_POINT('Ctrl Pts',(-40.2285194291702,-60.6532429799493,
12.));
#74392=CARTESIAN_POINT('Ctrl Pts',(-40.2337624072029,-60.6781220940979,
0.));
#74393=CARTESIAN_POINT('Ctrl Pts',(-40.2337624072029,-60.6781220940979,
12.));
#74394=CARTESIAN_POINT('Ctrl Pts',(-40.2389898925937,-60.7030445528863,
0.));
#74395=CARTESIAN_POINT('Ctrl Pts',(-40.2389898925937,-60.7030445528863,
12.));
#74396=CARTESIAN_POINT('Ctrl Pts',(-40.2442018113116,-60.72801026614,0.));
#74397=CARTESIAN_POINT('Ctrl Pts',(-40.2442018113116,-60.72801026614,12.));
#74398=CARTESIAN_POINT('Ctrl Pts',(-40.2493980896646,-60.7530191439603,
0.));
#74399=CARTESIAN_POINT('Ctrl Pts',(-40.2493980896646,-60.7530191439603,
12.));
#74400=CARTESIAN_POINT('Ctrl Pts',(-40.2545786542957,-60.7780710967253,
0.));
#74401=CARTESIAN_POINT('Ctrl Pts',(-40.2545786542957,-60.7780710967253,
12.));
#74402=CARTESIAN_POINT('Ctrl Pts',(-40.2597434321804,-60.8031660350878,
0.));
#74403=CARTESIAN_POINT('Ctrl Pts',(-40.2597434321804,-60.8031660350878,
12.));
#74404=CARTESIAN_POINT('Ctrl Pts',(-40.2648923506245,-60.8283038699703,
0.));
#74405=CARTESIAN_POINT('Ctrl Pts',(-40.2648923506245,-60.8283038699703,
12.));
#74406=CARTESIAN_POINT('Ctrl Pts',(-40.2700253372644,-60.8534845125535,
0.));
#74407=CARTESIAN_POINT('Ctrl Pts',(-40.2700253372644,-60.8534845125535,
12.));
#74408=CARTESIAN_POINT('Ctrl Pts',(-40.2751423200637,-60.8787078742817,
0.));
#74409=CARTESIAN_POINT('Ctrl Pts',(-40.2751423200637,-60.8787078742817,
12.));
#74410=CARTESIAN_POINT('Ctrl Pts',(-40.2802432273105,-60.903973866867,0.));
#74411=CARTESIAN_POINT('Ctrl Pts',(-40.2802432273105,-60.903973866867,12.));
#74412=CARTESIAN_POINT('Ctrl Pts',(-40.2853279876162,-60.9292824022888,
0.));
#74413=CARTESIAN_POINT('Ctrl Pts',(-40.2853279876162,-60.9292824022888,
12.));
#74414=CARTESIAN_POINT('Ctrl Pts',(-40.2903965299155,-60.9546333927919,
0.));
#74415=CARTESIAN_POINT('Ctrl Pts',(-40.2903965299155,-60.9546333927919,
12.));
#74416=CARTESIAN_POINT('Ctrl Pts',(-40.2954487834688,-60.9800267508781,
0.));
#74417=CARTESIAN_POINT('Ctrl Pts',(-40.2954487834688,-60.9800267508781,
12.));
#74418=CARTESIAN_POINT('Ctrl Pts',(-40.3004846778577,-61.0054623893059,
0.));
#74419=CARTESIAN_POINT('Ctrl Pts',(-40.3004846778577,-61.0054623893059,
12.));
#74420=CARTESIAN_POINT('Ctrl Pts',(-40.3055041429772,-61.0309402210915,
0.));
#74421=CARTESIAN_POINT('Ctrl Pts',(-40.3055041429772,-61.0309402210915,
12.));
#74422=CARTESIAN_POINT('Ctrl Pts',(-40.3105071090308,-61.0564601595047,
0.));
#74423=CARTESIAN_POINT('Ctrl Pts',(-40.3105071090308,-61.0564601595047,
12.));
#74424=CARTESIAN_POINT('Ctrl Pts',(-40.3154935065264,-61.0820221180646,
0.));
#74425=CARTESIAN_POINT('Ctrl Pts',(-40.3154935065264,-61.0820221180646,
12.));
#74426=CARTESIAN_POINT('Ctrl Pts',(-40.3204632662729,-61.1076260105265,
0.));
#74427=CARTESIAN_POINT('Ctrl Pts',(-40.3204632662729,-61.1076260105265,
12.));
#74428=CARTESIAN_POINT('Ctrl Pts',(-40.3254163193806,-61.1332717508799,
0.));
#74429=CARTESIAN_POINT('Ctrl Pts',(-40.3254163193806,-61.1332717508799,
12.));
#74430=CARTESIAN_POINT('Ctrl Pts',(-40.3303525972621,-61.1589592533623,
0.));
#74431=CARTESIAN_POINT('Ctrl Pts',(-40.3303525972621,-61.1589592533623,
12.));
#74432=CARTESIAN_POINT('Ctrl Pts',(-40.3352720316373,-61.184688432465,0.));
#74433=CARTESIAN_POINT('Ctrl Pts',(-40.3352720316373,-61.184688432465,12.));
#74434=CARTESIAN_POINT('Ctrl Pts',(-40.3401745545369,-61.2104592029375,
0.));
#74435=CARTESIAN_POINT('Ctrl Pts',(-40.3401745545369,-61.2104592029375,
12.));
#74436=CARTESIAN_POINT('Ctrl Pts',(-40.3450600983104,-61.236271479789,0.));
#74437=CARTESIAN_POINT('Ctrl Pts',(-40.3450600983104,-61.236271479789,12.));
#74438=CARTESIAN_POINT('Ctrl Pts',(-40.3499285956297,-61.2621251782849,
0.));
#74439=CARTESIAN_POINT('Ctrl Pts',(-40.3499285956297,-61.2621251782849,
12.));
#74440=CARTESIAN_POINT('Ctrl Pts',(-40.3547799794672,-61.2880202139358,
0.));
#74441=CARTESIAN_POINT('Ctrl Pts',(-40.3547799794672,-61.2880202139358,
12.));
#74442=CARTESIAN_POINT('Ctrl Pts',(-40.3596141830786,-61.3139565024838,
0.));
#74443=CARTESIAN_POINT('Ctrl Pts',(-40.3596141830786,-61.3139565024838,
12.));
#74444=CARTESIAN_POINT('Ctrl Pts',(-40.3644311399861,-61.3399339598851,
0.));
#74445=CARTESIAN_POINT('Ctrl Pts',(-40.3644311399861,-61.3399339598851,
12.));
#74446=CARTESIAN_POINT('Ctrl Pts',(-40.3692307839642,-61.3659525022917,
0.));
#74447=CARTESIAN_POINT('Ctrl Pts',(-40.3692307839642,-61.3659525022917,
12.));
#74448=CARTESIAN_POINT('Ctrl Pts',(-40.3740130490233,-61.3920120460232,
0.));
#74449=CARTESIAN_POINT('Ctrl Pts',(-40.3740130490233,-61.3920120460232,
12.));
#74450=CARTESIAN_POINT('Ctrl Pts',(-40.3787778694373,-61.418112507605,0.));
#74451=CARTESIAN_POINT('Ctrl Pts',(-40.3787778694373,-61.418112507605,12.));
#74452=CARTESIAN_POINT('Ctrl Pts',(-40.3835251797725,-61.4442538038053,
0.));
#74453=CARTESIAN_POINT('Ctrl Pts',(-40.3835251797725,-61.4442538038053,
12.));
#74454=CARTESIAN_POINT('Ctrl Pts',(-40.3882549149229,-61.4704358516711,
0.));
#74455=CARTESIAN_POINT('Ctrl Pts',(-40.3882549149229,-61.4704358516711,
12.));
#74456=CARTESIAN_POINT('Ctrl Pts',(-40.3929670101363,-61.4966585685544,
0.));
#74457=CARTESIAN_POINT('Ctrl Pts',(-40.3929670101363,-61.4966585685544,
12.));
#74458=CARTESIAN_POINT('Ctrl Pts',(-40.3976614010648,-61.5229218721532,
0.));
#74459=CARTESIAN_POINT('Ctrl Pts',(-40.3976614010648,-61.5229218721532,
12.));
#74460=CARTESIAN_POINT('Ctrl Pts',(-40.4023380237227,-61.5492256804709,
0.));
#74461=CARTESIAN_POINT('Ctrl Pts',(-40.4023380237227,-61.5492256804709,
12.));
#74462=CARTESIAN_POINT('Ctrl Pts',(-40.4069968143953,-61.5755699117318,
0.));
#74463=CARTESIAN_POINT('Ctrl Pts',(-40.4069968143953,-61.5755699117318,
12.));
#74464=CARTESIAN_POINT('Ctrl Pts',(-40.4116377095595,-61.6019544843008,
0.));
#74465=CARTESIAN_POINT('Ctrl Pts',(-40.4116377095595,-61.6019544843008,
12.));
#74466=CARTESIAN_POINT('Ctrl Pts',(-40.4162606458119,-61.628379316608,0.));
#74467=CARTESIAN_POINT('Ctrl Pts',(-40.4162606458119,-61.628379316608,12.));
#74468=CARTESIAN_POINT('Ctrl Pts',(-40.420865559772,-61.6548443270397,0.));
#74469=CARTESIAN_POINT('Ctrl Pts',(-40.420865559772,-61.6548443270397,12.));
#74470=CARTESIAN_POINT('Ctrl Pts',(-40.4254523880766,-61.6813494339295,
0.));
#74471=CARTESIAN_POINT('Ctrl Pts',(-40.4254523880766,-61.6813494339295,
12.));
#74472=CARTESIAN_POINT('Ctrl Pts',(-40.4300210675848,-61.7078945557812,
0.));
#74473=CARTESIAN_POINT('Ctrl Pts',(-40.4300210675848,-61.7078945557812,
12.));
#74474=CARTESIAN_POINT('Ctrl Pts',(-40.4345715355411,-61.7344796114409,
0.));
#74475=CARTESIAN_POINT('Ctrl Pts',(-40.4345715355411,-61.7344796114409,
12.));
#74476=CARTESIAN_POINT('Ctrl Pts',(-40.439103729759,-61.7611045202875,0.));
#74477=CARTESIAN_POINT('Ctrl Pts',(-40.439103729759,-61.7611045202875,12.));
#74478=CARTESIAN_POINT('Ctrl Pts',(-40.4436175887943,-61.7877692024064,
0.));
#74479=CARTESIAN_POINT('Ctrl Pts',(-40.4436175887943,-61.7877692024064,
12.));
#74480=CARTESIAN_POINT('Ctrl Pts',(-40.448113052135,-61.8144735787767,0.));
#74481=CARTESIAN_POINT('Ctrl Pts',(-40.448113052135,-61.8144735787767,12.));
#74482=CARTESIAN_POINT('Ctrl Pts',(-40.4525900597877,-61.8412175708523,
0.));
#74483=CARTESIAN_POINT('Ctrl Pts',(-40.4525900597877,-61.8412175708523,
12.));
#74484=CARTESIAN_POINT('Ctrl Pts',(-40.4570485518735,-61.8680011001513,
0.));
#74485=CARTESIAN_POINT('Ctrl Pts',(-40.4570485518735,-61.8680011001513,
12.));
#74486=CARTESIAN_POINT('Ctrl Pts',(-40.4614884681884,-61.8948240877998,
0.));
#74487=CARTESIAN_POINT('Ctrl Pts',(-40.4614884681884,-61.8948240877998,
12.));
#74488=CARTESIAN_POINT('Ctrl Pts',(-40.4659097478595,-61.9216864541758,
0.));
#74489=CARTESIAN_POINT('Ctrl Pts',(-40.4659097478595,-61.9216864541758,
12.));
#74490=CARTESIAN_POINT('Ctrl Pts',(-40.4703123287642,-61.9485881182957,
0.));
#74491=CARTESIAN_POINT('Ctrl Pts',(-40.4703123287642,-61.9485881182957,
12.));
#74492=CARTESIAN_POINT('Ctrl Pts',(-40.4746961480045,-61.9755289983093,
0.));
#74493=CARTESIAN_POINT('Ctrl Pts',(-40.4746961480045,-61.9755289983093,
12.));
#74494=CARTESIAN_POINT('Ctrl Pts',(-40.4790611429613,-62.0025090126008,
0.));
#74495=CARTESIAN_POINT('Ctrl Pts',(-40.4790611429613,-62.0025090126008,
12.));
#74496=CARTESIAN_POINT('Ctrl Pts',(-40.4834072522181,-62.0295280807449,
0.));
#74497=CARTESIAN_POINT('Ctrl Pts',(-40.4834072522181,-62.0295280807449,
12.));
#74498=CARTESIAN_POINT('Ctrl Pts',(-40.4877344164407,-62.0565861244171,
0.));
#74499=CARTESIAN_POINT('Ctrl Pts',(-40.4877344164407,-62.0565861244171,
12.));
#74500=CARTESIAN_POINT('Ctrl Pts',(-40.4920425795184,-62.0836830685665,
0.));
#74501=CARTESIAN_POINT('Ctrl Pts',(-40.4920425795184,-62.0836830685665,
12.));
#74502=CARTESIAN_POINT('Ctrl Pts',(-40.4963316888357,-62.110818841691,0.));
#74503=CARTESIAN_POINT('Ctrl Pts',(-40.4963316888357,-62.110818841691,12.));
#74504=CARTESIAN_POINT('Ctrl Pts',(-40.5006016927489,-62.137993373242,0.));
#74505=CARTESIAN_POINT('Ctrl Pts',(-40.5006016927489,-62.137993373242,12.));
#74506=CARTESIAN_POINT('Ctrl Pts',(-40.5048525385985,-62.1652065915724,
0.));
#74507=CARTESIAN_POINT('Ctrl Pts',(-40.5048525385985,-62.1652065915724,
12.));
#74508=CARTESIAN_POINT('Ctrl Pts',(-40.5090841704111,-62.1924584215634,
0.));
#74509=CARTESIAN_POINT('Ctrl Pts',(-40.5090841704111,-62.1924584215634,
12.));
#74510=CARTESIAN_POINT('Ctrl Pts',(-40.5132965269679,-62.2197487826212,
0.));
#74511=CARTESIAN_POINT('Ctrl Pts',(-40.5132965269679,-62.2197487826212,
12.));
#74512=CARTESIAN_POINT('Ctrl Pts',(-40.5174895391059,-62.2470775858834,
0.));
#74513=CARTESIAN_POINT('Ctrl Pts',(-40.5174895391059,-62.2470775858834,
12.));
#74514=CARTESIAN_POINT('Ctrl Pts',(-40.5216631336335,-62.2744447382207,
0.));
#74515=CARTESIAN_POINT('Ctrl Pts',(-40.5216631336335,-62.2744447382207,
12.));
#74516=CARTESIAN_POINT('Ctrl Pts',(-40.5258172381565,-62.3018501471876,
0.));
#74517=CARTESIAN_POINT('Ctrl Pts',(-40.5258172381565,-62.3018501471876,
12.));
#74518=CARTESIAN_POINT('Ctrl Pts',(-40.5299517857793,-62.3292937258021,
0.));
#74519=CARTESIAN_POINT('Ctrl Pts',(-40.5299517857793,-62.3292937258021,
12.));
#74520=CARTESIAN_POINT('Ctrl Pts',(-40.5340667194272,-62.35677539702,0.));
#74521=CARTESIAN_POINT('Ctrl Pts',(-40.5340667194272,-62.35677539702,12.));
#74522=CARTESIAN_POINT('Ctrl Pts',(-40.5381619973972,-62.3842950992504,
0.));
#74523=CARTESIAN_POINT('Ctrl Pts',(-40.5381619973972,-62.3842950992504,
12.));
#74524=CARTESIAN_POINT('Ctrl Pts',(-40.5422375944697,-62.4118527880601,
0.));
#74525=CARTESIAN_POINT('Ctrl Pts',(-40.5422375944697,-62.4118527880601,
12.));
#74526=CARTESIAN_POINT('Ctrl Pts',(-40.5462934972334,-62.439448432904,0.));
#74527=CARTESIAN_POINT('Ctrl Pts',(-40.5462934972334,-62.439448432904,12.));
#74528=CARTESIAN_POINT('Ctrl Pts',(-40.5495224601437,-62.4615552986668,
0.));
#74529=CARTESIAN_POINT('Ctrl Pts',(-40.5495224601437,-62.4615552986668,
12.));
#74530=CARTESIAN_POINT('Ctrl Pts',(-40.5519353177058,-62.4781525155997,
0.));
#74531=CARTESIAN_POINT('Ctrl Pts',(-40.5519353177058,-62.4781525155997,
12.));
#74532=CARTESIAN_POINT('Ctrl Pts',(-40.5535399497449,-62.4892249121863,
0.));
#74533=CARTESIAN_POINT('Ctrl Pts',(-40.5535399497449,-62.4892249121863,
12.));
#74534=CARTESIAN_POINT('Ctrl Pts',(-40.554341280847,-62.4947630068039,0.));
#74535=CARTESIAN_POINT('Ctrl Pts',(-40.554341280847,-62.4947630068039,12.));
#74536=CARTESIAN_POINT('',(-39.4479504917287,-57.8261117662438,0.));
#74537=CARTESIAN_POINT('Ctrl Pts',(-39.4479504917287,-57.8261117662438,
0.));
#74538=CARTESIAN_POINT('Ctrl Pts',(-39.4492429618443,-57.8297740100947,
0.));
#74539=CARTESIAN_POINT('Ctrl Pts',(-39.4518277003553,-57.837104315141,0.));
#74540=CARTESIAN_POINT('Ctrl Pts',(-39.4557042029652,-57.8481172247495,
0.));
#74541=CARTESIAN_POINT('Ctrl Pts',(-39.4608716627118,-57.8628360096803,
0.));
#74542=CARTESIAN_POINT('Ctrl Pts',(-39.4673289592259,-57.8812926637177,
0.));
#74543=CARTESIAN_POINT('Ctrl Pts',(-39.473784194937,-57.8998074670478,0.));
#74544=CARTESIAN_POINT('Ctrl Pts',(-39.4802373061058,-57.9183803632403,
0.));
#74545=CARTESIAN_POINT('Ctrl Pts',(-39.4866881842317,-57.937011245663,0.));
#74546=CARTESIAN_POINT('Ctrl Pts',(-39.4931366776714,-57.9556999583892,
0.));
#74547=CARTESIAN_POINT('Ctrl Pts',(-39.499582610674,-57.974446317937,0.));
#74548=CARTESIAN_POINT('Ctrl Pts',(-39.5060257981225,-57.9932501298522,
0.));
#74549=CARTESIAN_POINT('Ctrl Pts',(-39.5124660614976,-58.0121112067895,
0.));
#74550=CARTESIAN_POINT('Ctrl Pts',(-39.5189032457184,-58.0310293875262,
0.));
#74551=CARTESIAN_POINT('Ctrl Pts',(-39.5253372136887,-58.0500045308412,
0.));
#74552=CARTESIAN_POINT('Ctrl Pts',(-39.5317678383217,-58.0690365065374,
0.));
#74553=CARTESIAN_POINT('Ctrl Pts',(-39.5381949959221,-58.088125187992,0.));
#74554=CARTESIAN_POINT('Ctrl Pts',(-39.5446185579638,-58.1072704428928,
0.));
#74555=CARTESIAN_POINT('Ctrl Pts',(-39.5510383869505,-58.126472128574,0.));
#74556=CARTESIAN_POINT('Ctrl Pts',(-39.5574543406982,-58.1457300968499,
0.));
#74557=CARTESIAN_POINT('Ctrl Pts',(-39.563866275018,-58.1650441970387,0.));
#74558=CARTESIAN_POINT('Ctrl Pts',(-39.5702740467999,-58.1844142794338,
0.));
#74559=CARTESIAN_POINT('Ctrl Pts',(-39.57667751752,-58.2038401992457,0.));
#74560=CARTESIAN_POINT('Ctrl Pts',(-39.5830765530891,-58.2233218164365,
0.));
#74561=CARTESIAN_POINT('Ctrl Pts',(-39.5894710221713,-58.2428589938369,
0.));
#74562=CARTESIAN_POINT('Ctrl Pts',(-39.5958607950239,-58.2624515958419,
0.));
#74563=CARTESIAN_POINT('Ctrl Pts',(-39.602245742079,-58.2820994868118,0.));
#74564=CARTESIAN_POINT('Ctrl Pts',(-39.6086257327583,-58.3018025297323,
0.));
#74565=CARTESIAN_POINT('Ctrl Pts',(-39.6150006360914,-58.3215605869221,
0.));
#74566=CARTESIAN_POINT('Ctrl Pts',(-39.6213703212531,-58.3413735206423,
0.));
#74567=CARTESIAN_POINT('Ctrl Pts',(-39.6277346580892,-58.3612411936904,
0.));
#74568=CARTESIAN_POINT('Ctrl Pts',(-39.6340935177476,-58.3811634701037,
0.));
#74569=CARTESIAN_POINT('Ctrl Pts',(-39.6404467729094,-58.4011402154196,
0.));
#74570=CARTESIAN_POINT('Ctrl Pts',(-39.6467942974451,-58.4211712963004,
0.));
#74571=CARTESIAN_POINT('Ctrl Pts',(-39.653135966204,-58.4412565802979,0.));
#74572=CARTESIAN_POINT('Ctrl Pts',(-39.6594716547689,-58.4613959355788,
0.));
#74573=CARTESIAN_POINT('Ctrl Pts',(-39.6658012391815,-58.4815892306066,
0.));
#74574=CARTESIAN_POINT('Ctrl Pts',(-39.6721245959531,-58.5018363341604,
0.));
#74575=CARTESIAN_POINT('Ctrl Pts',(-39.6784416021826,-58.522137115476,0.));
#74576=CARTESIAN_POINT('Ctrl Pts',(-39.6847521356395,-58.5424914443415,
0.));
#74577=CARTESIAN_POINT('Ctrl Pts',(-39.6910560748629,-58.5628991912052,
0.));
#74578=CARTESIAN_POINT('Ctrl Pts',(-39.6973532992539,-58.5833602272743,
0.));
#74579=CARTESIAN_POINT('Ctrl Pts',(-39.7036436890233,-58.6038744244659,
0.));
#74580=CARTESIAN_POINT('Ctrl Pts',(-39.7099271251413,-58.6244416553562,
0.));
#74581=CARTESIAN_POINT('Ctrl Pts',(-39.7162034892899,-58.6450617931274,
0.));
#74582=CARTESIAN_POINT('Ctrl Pts',(-39.7224726638101,-58.6657347115034,
0.));
#74583=CARTESIAN_POINT('Ctrl Pts',(-39.7287345316681,-58.6864602847088,
0.));
#74584=CARTESIAN_POINT('Ctrl Pts',(-39.734988976475,-58.7072383875027,0.));
#74585=CARTESIAN_POINT('Ctrl Pts',(-39.7412358824953,-58.7280688951916,
0.));
#74586=CARTESIAN_POINT('Ctrl Pts',(-39.7474751346598,-58.7489516836445,
0.));
#74587=CARTESIAN_POINT('Ctrl Pts',(-39.7537066185813,-58.7698866293029,
0.));
#74588=CARTESIAN_POINT('Ctrl Pts',(-39.7599302205521,-58.7908736091798,
0.));
#74589=CARTESIAN_POINT('Ctrl Pts',(-39.7661458275274,-58.8119125008517,
0.));
#74590=CARTESIAN_POINT('Ctrl Pts',(-39.772353327112,-58.8330031824453,0.));
#74591=CARTESIAN_POINT('Ctrl Pts',(-39.7785526075478,-58.8541455326231,
0.));
#74592=CARTESIAN_POINT('Ctrl Pts',(-39.7847435576996,-58.8753394305585,
0.));
#74593=CARTESIAN_POINT('Ctrl Pts',(-39.7909260670517,-58.8965847559391,
0.));
#74594=CARTESIAN_POINT('Ctrl Pts',(-39.7971000257044,-58.9178813889703,
0.));
#74595=CARTESIAN_POINT('Ctrl Pts',(-39.8032653243712,-58.9392292103747,
0.));
#74596=CARTESIAN_POINT('Ctrl Pts',(-39.8094218543782,-58.9606281013875,
0.));
#74597=CARTESIAN_POINT('Ctrl Pts',(-39.8155695076626,-58.9820779437484,
0.));
#74598=CARTESIAN_POINT('Ctrl Pts',(-39.821708176766,-59.0035786197024,0.));
#74599=CARTESIAN_POINT('Ctrl Pts',(-39.8278377548262,-59.0251300119973,
0.));
#74600=CARTESIAN_POINT('Ctrl Pts',(-39.8339581355716,-59.0467320038784,
0.));
#74601=CARTESIAN_POINT('Ctrl Pts',(-39.8400692133139,-59.0683844790764,
0.));
#74602=CARTESIAN_POINT('Ctrl Pts',(-39.8461708829456,-59.090087321798,0.));
#74603=CARTESIAN_POINT('Ctrl Pts',(-39.8522630399328,-59.1118404167292,
0.));
#74604=CARTESIAN_POINT('Ctrl Pts',(-39.8583455803105,-59.1336436490342,
0.));
#74605=CARTESIAN_POINT('Ctrl Pts',(-39.8644184006787,-59.1554969043522,
0.));
#74606=CARTESIAN_POINT('Ctrl Pts',(-39.8704813981988,-59.1774000687879,
0.));
#74607=CARTESIAN_POINT('Ctrl Pts',(-39.876534470591,-59.1993530289028,0.));
#74608=CARTESIAN_POINT('Ctrl Pts',(-39.8825775161267,-59.2213556717209,
0.));
#74609=CARTESIAN_POINT('Ctrl Pts',(-39.8886104336242,-59.2434078847247,
0.));
#74610=CARTESIAN_POINT('Ctrl Pts',(-39.8946331224438,-59.2655095558521,
0.));
#74611=CARTESIAN_POINT('Ctrl Pts',(-39.9006454824845,-59.2876605734846,
0.));
#74612=CARTESIAN_POINT('Ctrl Pts',(-39.9066474141803,-59.3098608264419,
0.));
#74613=CARTESIAN_POINT('Ctrl Pts',(-39.9126388184936,-59.3321102039852,
0.));
#74614=CARTESIAN_POINT('Ctrl Pts',(-39.9186195969104,-59.3544085958151,
0.));
#74615=CARTESIAN_POINT('Ctrl Pts',(-39.9245896514367,-59.3767558920675,
0.));
#74616=CARTESIAN_POINT('Ctrl Pts',(-39.9305488845958,-59.3991519833016,
0.));
#74617=CARTESIAN_POINT('Ctrl Pts',(-39.9364971994242,-59.4215967604967,
0.));
#74618=CARTESIAN_POINT('Ctrl Pts',(-39.9424344994672,-59.4440901150582,
0.));
#74619=CARTESIAN_POINT('Ctrl Pts',(-39.9483606887737,-59.4666319388133,
0.));
#74620=CARTESIAN_POINT('Ctrl Pts',(-39.9542756718922,-59.4892221240068,
0.));
#74621=CARTESIAN_POINT('Ctrl Pts',(-39.9601793538682,-59.511860563289,0.));
#74622=CARTESIAN_POINT('Ctrl Pts',(-39.9660716402403,-59.5345471497128,
0.));
#74623=CARTESIAN_POINT('Ctrl Pts',(-39.9719524370345,-59.5572817767388,
0.));
#74624=CARTESIAN_POINT('Ctrl Pts',(-39.9778216507605,-59.5800643382314,
0.));
#74625=CARTESIAN_POINT('Ctrl Pts',(-39.9836791884079,-59.6028947284562,
0.));
#74626=CARTESIAN_POINT('Ctrl Pts',(-39.9895249574448,-59.6257728420669,
0.));
#74627=CARTESIAN_POINT('Ctrl Pts',(-39.9953588658132,-59.6486985741041,
0.));
#74628=CARTESIAN_POINT('Ctrl Pts',(-40.0011808219241,-59.6716718200005,
0.));
#74629=CARTESIAN_POINT('Ctrl Pts',(-40.0069907346537,-59.6946924755773,
0.));
#74630=CARTESIAN_POINT('Ctrl Pts',(-40.0127885133403,-59.7177604370403,
0.));
#74631=CARTESIAN_POINT('Ctrl Pts',(-40.0185740677821,-59.7408756009679,
0.));
#74632=CARTESIAN_POINT('Ctrl Pts',(-40.0243473082337,-59.7640378643106,
0.));
#74633=CARTESIAN_POINT('Ctrl Pts',(-40.0301081454002,-59.7872471243942,
0.));
#74634=CARTESIAN_POINT('Ctrl Pts',(-40.0358564904341,-59.8105032789179,
0.));
#74635=CARTESIAN_POINT('Ctrl Pts',(-40.0415922549315,-59.8338062259492,
0.));
#74636=CARTESIAN_POINT('Ctrl Pts',(-40.0473153509324,-59.8571558639145,
0.));
#74637=CARTESIAN_POINT('Ctrl Pts',(-40.0530256909161,-59.8805520915972,
0.));
#74638=CARTESIAN_POINT('Ctrl Pts',(-40.0587231877959,-59.9039948081428,
0.));
#74639=CARTESIAN_POINT('Ctrl Pts',(-40.0644077549158,-59.927483913055,0.));
#74640=CARTESIAN_POINT('Ctrl Pts',(-40.0700793060475,-59.9510193061929,
0.));
#74641=CARTESIAN_POINT('Ctrl Pts',(-40.0757377553893,-59.974600887759,0.));
#74642=CARTESIAN_POINT('Ctrl Pts',(-40.0813830175629,-59.9982285582991,
0.));
#74643=CARTESIAN_POINT('Ctrl Pts',(-40.0870150076078,-60.0219022187066,
0.));
#74644=CARTESIAN_POINT('Ctrl Pts',(-40.0926336409787,-60.0456217702203,
0.));
#74645=CARTESIAN_POINT('Ctrl Pts',(-40.0982388335421,-60.0693871144207,
0.));
#74646=CARTESIAN_POINT('Ctrl Pts',(-40.1038305015763,-60.0931981532194,
0.));
#74647=CARTESIAN_POINT('Ctrl Pts',(-40.1094085617672,-60.1170547888572,
0.));
#74648=CARTESIAN_POINT('Ctrl Pts',(-40.1149729312036,-60.1409569239092,
0.));
#74649=CARTESIAN_POINT('Ctrl Pts',(-40.120523527374,-60.1649044612829,0.));
#74650=CARTESIAN_POINT('Ctrl Pts',(-40.1260602681644,-60.1888973042151,
0.));
#74651=CARTESIAN_POINT('Ctrl Pts',(-40.1315830718575,-60.2129353562617,
0.));
#74652=CARTESIAN_POINT('Ctrl Pts',(-40.13709185713,-60.2370185212957,0.));
#74653=CARTESIAN_POINT('Ctrl Pts',(-40.1425865430468,-60.2611467035109,
0.));
#74654=CARTESIAN_POINT('Ctrl Pts',(-40.1480670490583,-60.2853198074215,
0.));
#74655=CARTESIAN_POINT('Ctrl Pts',(-40.1535332949978,-60.3095377378589,
0.));
#74656=CARTESIAN_POINT('Ctrl Pts',(-40.1589852010811,-60.3338003999616,
0.));
#74657=CARTESIAN_POINT('Ctrl Pts',(-40.1644226879043,-60.3581076991731,
0.));
#74658=CARTESIAN_POINT('Ctrl Pts',(-40.1698456764387,-60.382459541246,0.));
#74659=CARTESIAN_POINT('Ctrl Pts',(-40.1752540880273,-60.4068558322414,
0.));
#74660=CARTESIAN_POINT('Ctrl Pts',(-40.1806478443828,-60.4312964785269,
0.));
#74661=CARTESIAN_POINT('Ctrl Pts',(-40.1860268675875,-60.4557813867677,
0.));
#74662=CARTESIAN_POINT('Ctrl Pts',(-40.1913910800911,-60.4803104639211,
0.));
#74663=CARTESIAN_POINT('Ctrl Pts',(-40.1967404047055,-60.5048836172423,
0.));
#74664=CARTESIAN_POINT('Ctrl Pts',(-40.2020747646012,-60.5295007542838,
0.));
#74665=CARTESIAN_POINT('Ctrl Pts',(-40.2073940833054,-60.5541617828927,
0.));
#74666=CARTESIAN_POINT('Ctrl Pts',(-40.2126982847012,-60.5788666112043,
0.));
#74667=CARTESIAN_POINT('Ctrl Pts',(-40.2179872930272,-60.6036151476347,
0.));
#74668=CARTESIAN_POINT('Ctrl Pts',(-40.2232610328717,-60.6284073008865,
0.));
#74669=CARTESIAN_POINT('Ctrl Pts',(-40.2285194291702,-60.6532429799493,
0.));
#74670=CARTESIAN_POINT('Ctrl Pts',(-40.2337624072029,-60.6781220940979,
0.));
#74671=CARTESIAN_POINT('Ctrl Pts',(-40.2389898925937,-60.7030445528863,
0.));
#74672=CARTESIAN_POINT('Ctrl Pts',(-40.2442018113116,-60.72801026614,0.));
#74673=CARTESIAN_POINT('Ctrl Pts',(-40.2493980896646,-60.7530191439603,
0.));
#74674=CARTESIAN_POINT('Ctrl Pts',(-40.2545786542957,-60.7780710967253,
0.));
#74675=CARTESIAN_POINT('Ctrl Pts',(-40.2597434321804,-60.8031660350878,
0.));
#74676=CARTESIAN_POINT('Ctrl Pts',(-40.2648923506245,-60.8283038699703,
0.));
#74677=CARTESIAN_POINT('Ctrl Pts',(-40.2700253372644,-60.8534845125535,
0.));
#74678=CARTESIAN_POINT('Ctrl Pts',(-40.2751423200637,-60.8787078742817,
0.));
#74679=CARTESIAN_POINT('Ctrl Pts',(-40.2802432273105,-60.903973866867,0.));
#74680=CARTESIAN_POINT('Ctrl Pts',(-40.2853279876162,-60.9292824022888,
0.));
#74681=CARTESIAN_POINT('Ctrl Pts',(-40.2903965299155,-60.9546333927919,
0.));
#74682=CARTESIAN_POINT('Ctrl Pts',(-40.2954487834688,-60.9800267508781,
0.));
#74683=CARTESIAN_POINT('Ctrl Pts',(-40.3004846778577,-61.0054623893059,
0.));
#74684=CARTESIAN_POINT('Ctrl Pts',(-40.3055041429772,-61.0309402210915,
0.));
#74685=CARTESIAN_POINT('Ctrl Pts',(-40.3105071090308,-61.0564601595047,
0.));
#74686=CARTESIAN_POINT('Ctrl Pts',(-40.3154935065264,-61.0820221180646,
0.));
#74687=CARTESIAN_POINT('Ctrl Pts',(-40.3204632662729,-61.1076260105265,
0.));
#74688=CARTESIAN_POINT('Ctrl Pts',(-40.3254163193806,-61.1332717508799,
0.));
#74689=CARTESIAN_POINT('Ctrl Pts',(-40.3303525972621,-61.1589592533623,
0.));
#74690=CARTESIAN_POINT('Ctrl Pts',(-40.3352720316373,-61.184688432465,0.));
#74691=CARTESIAN_POINT('Ctrl Pts',(-40.3401745545369,-61.2104592029375,
0.));
#74692=CARTESIAN_POINT('Ctrl Pts',(-40.3450600983104,-61.236271479789,0.));
#74693=CARTESIAN_POINT('Ctrl Pts',(-40.3499285956297,-61.2621251782849,
0.));
#74694=CARTESIAN_POINT('Ctrl Pts',(-40.3547799794672,-61.2880202139358,
0.));
#74695=CARTESIAN_POINT('Ctrl Pts',(-40.3596141830786,-61.3139565024838,
0.));
#74696=CARTESIAN_POINT('Ctrl Pts',(-40.3644311399861,-61.3399339598851,
0.));
#74697=CARTESIAN_POINT('Ctrl Pts',(-40.3692307839642,-61.3659525022917,
0.));
#74698=CARTESIAN_POINT('Ctrl Pts',(-40.3740130490233,-61.3920120460232,
0.));
#74699=CARTESIAN_POINT('Ctrl Pts',(-40.3787778694373,-61.418112507605,0.));
#74700=CARTESIAN_POINT('Ctrl Pts',(-40.3835251797725,-61.4442538038053,
0.));
#74701=CARTESIAN_POINT('Ctrl Pts',(-40.3882549149229,-61.4704358516711,
0.));
#74702=CARTESIAN_POINT('Ctrl Pts',(-40.3929670101363,-61.4966585685544,
0.));
#74703=CARTESIAN_POINT('Ctrl Pts',(-40.3976614010648,-61.5229218721532,
0.));
#74704=CARTESIAN_POINT('Ctrl Pts',(-40.4023380237227,-61.5492256804709,
0.));
#74705=CARTESIAN_POINT('Ctrl Pts',(-40.4069968143953,-61.5755699117318,
0.));
#74706=CARTESIAN_POINT('Ctrl Pts',(-40.4116377095595,-61.6019544843008,
0.));
#74707=CARTESIAN_POINT('Ctrl Pts',(-40.4162606458119,-61.628379316608,0.));
#74708=CARTESIAN_POINT('Ctrl Pts',(-40.420865559772,-61.6548443270397,0.));
#74709=CARTESIAN_POINT('Ctrl Pts',(-40.4254523880766,-61.6813494339295,
0.));
#74710=CARTESIAN_POINT('Ctrl Pts',(-40.4300210675848,-61.7078945557812,
0.));
#74711=CARTESIAN_POINT('Ctrl Pts',(-40.4345715355411,-61.7344796114409,
0.));
#74712=CARTESIAN_POINT('Ctrl Pts',(-40.439103729759,-61.7611045202875,0.));
#74713=CARTESIAN_POINT('Ctrl Pts',(-40.4436175887943,-61.7877692024064,
0.));
#74714=CARTESIAN_POINT('Ctrl Pts',(-40.448113052135,-61.8144735787767,0.));
#74715=CARTESIAN_POINT('Ctrl Pts',(-40.4525900597877,-61.8412175708523,
0.));
#74716=CARTESIAN_POINT('Ctrl Pts',(-40.4570485518735,-61.8680011001513,
0.));
#74717=CARTESIAN_POINT('Ctrl Pts',(-40.4614884681884,-61.8948240877998,
0.));
#74718=CARTESIAN_POINT('Ctrl Pts',(-40.4659097478595,-61.9216864541758,
0.));
#74719=CARTESIAN_POINT('Ctrl Pts',(-40.4703123287642,-61.9485881182957,
0.));
#74720=CARTESIAN_POINT('Ctrl Pts',(-40.4746961480045,-61.9755289983093,
0.));
#74721=CARTESIAN_POINT('Ctrl Pts',(-40.4790611429613,-62.0025090126008,
0.));
#74722=CARTESIAN_POINT('Ctrl Pts',(-40.4834072522181,-62.0295280807449,
0.));
#74723=CARTESIAN_POINT('Ctrl Pts',(-40.4877344164407,-62.0565861244171,
0.));
#74724=CARTESIAN_POINT('Ctrl Pts',(-40.4920425795184,-62.0836830685665,
0.));
#74725=CARTESIAN_POINT('Ctrl Pts',(-40.4963316888357,-62.110818841691,0.));
#74726=CARTESIAN_POINT('Ctrl Pts',(-40.499991909619,-62.1341126810364,0.));
#74727=CARTESIAN_POINT('Ctrl Pts',(-40.5027877865723,-62.1519925002736,
0.));
#74728=CARTESIAN_POINT('Ctrl Pts',(-40.5047277935687,-62.1644411502528,
0.));
#74729=CARTESIAN_POINT('Ctrl Pts',(-40.5058175523045,-62.171447313775,0.));
#74730=CARTESIAN_POINT('Ctrl Pts',(-40.5060598100838,-62.1730054756451,
0.));
#74731=CARTESIAN_POINT('',(-39.4479504917287,-57.8261117662438,12.));
#74732=CARTESIAN_POINT('',(-39.4479504917287,-57.8261117662438,0.));
#74733=CARTESIAN_POINT('Ctrl Pts',(-40.5060598100838,-62.1730054756452,
12.));
#74734=CARTESIAN_POINT('Ctrl Pts',(-40.5058175523045,-62.1714473137751,
12.));
#74735=CARTESIAN_POINT('Ctrl Pts',(-40.5047277935688,-62.1644411502529,
12.));
#74736=CARTESIAN_POINT('Ctrl Pts',(-40.5027877865724,-62.1519925002736,
12.));
#74737=CARTESIAN_POINT('Ctrl Pts',(-40.499991909619,-62.1341126810364,12.));
#74738=CARTESIAN_POINT('Ctrl Pts',(-40.4963316888357,-62.110818841691,12.));
#74739=CARTESIAN_POINT('Ctrl Pts',(-40.4920425795184,-62.0836830685665,
12.));
#74740=CARTESIAN_POINT('Ctrl Pts',(-40.4877344164407,-62.0565861244171,
12.));
#74741=CARTESIAN_POINT('Ctrl Pts',(-40.4834072522181,-62.0295280807449,
12.));
#74742=CARTESIAN_POINT('Ctrl Pts',(-40.4790611429613,-62.0025090126008,
12.));
#74743=CARTESIAN_POINT('Ctrl Pts',(-40.4746961480045,-61.9755289983093,
12.));
#74744=CARTESIAN_POINT('Ctrl Pts',(-40.4703123287642,-61.9485881182957,
12.));
#74745=CARTESIAN_POINT('Ctrl Pts',(-40.4659097478595,-61.9216864541758,
12.));
#74746=CARTESIAN_POINT('Ctrl Pts',(-40.4614884681884,-61.8948240877998,
12.));
#74747=CARTESIAN_POINT('Ctrl Pts',(-40.4570485518735,-61.8680011001513,
12.));
#74748=CARTESIAN_POINT('Ctrl Pts',(-40.4525900597877,-61.8412175708523,
12.));
#74749=CARTESIAN_POINT('Ctrl Pts',(-40.448113052135,-61.8144735787767,12.));
#74750=CARTESIAN_POINT('Ctrl Pts',(-40.4436175887943,-61.7877692024064,
12.));
#74751=CARTESIAN_POINT('Ctrl Pts',(-40.439103729759,-61.7611045202875,12.));
#74752=CARTESIAN_POINT('Ctrl Pts',(-40.4345715355411,-61.7344796114409,
12.));
#74753=CARTESIAN_POINT('Ctrl Pts',(-40.4300210675848,-61.7078945557812,
12.));
#74754=CARTESIAN_POINT('Ctrl Pts',(-40.4254523880766,-61.6813494339295,
12.));
#74755=CARTESIAN_POINT('Ctrl Pts',(-40.420865559772,-61.6548443270397,12.));
#74756=CARTESIAN_POINT('Ctrl Pts',(-40.4162606458119,-61.628379316608,12.));
#74757=CARTESIAN_POINT('Ctrl Pts',(-40.4116377095595,-61.6019544843008,
12.));
#74758=CARTESIAN_POINT('Ctrl Pts',(-40.4069968143953,-61.5755699117318,
12.));
#74759=CARTESIAN_POINT('Ctrl Pts',(-40.4023380237227,-61.5492256804709,
12.));
#74760=CARTESIAN_POINT('Ctrl Pts',(-40.3976614010648,-61.5229218721532,
12.));
#74761=CARTESIAN_POINT('Ctrl Pts',(-40.3929670101363,-61.4966585685544,
12.));
#74762=CARTESIAN_POINT('Ctrl Pts',(-40.3882549149229,-61.4704358516711,
12.));
#74763=CARTESIAN_POINT('Ctrl Pts',(-40.3835251797725,-61.4442538038053,
12.));
#74764=CARTESIAN_POINT('Ctrl Pts',(-40.3787778694373,-61.418112507605,12.));
#74765=CARTESIAN_POINT('Ctrl Pts',(-40.3740130490233,-61.3920120460232,
12.));
#74766=CARTESIAN_POINT('Ctrl Pts',(-40.3692307839642,-61.3659525022917,
12.));
#74767=CARTESIAN_POINT('Ctrl Pts',(-40.3644311399861,-61.3399339598851,
12.));
#74768=CARTESIAN_POINT('Ctrl Pts',(-40.3596141830786,-61.3139565024838,
12.));
#74769=CARTESIAN_POINT('Ctrl Pts',(-40.3547799794672,-61.2880202139358,
12.));
#74770=CARTESIAN_POINT('Ctrl Pts',(-40.3499285956297,-61.2621251782849,
12.));
#74771=CARTESIAN_POINT('Ctrl Pts',(-40.3450600983104,-61.236271479789,12.));
#74772=CARTESIAN_POINT('Ctrl Pts',(-40.3401745545369,-61.2104592029375,
12.));
#74773=CARTESIAN_POINT('Ctrl Pts',(-40.3352720316373,-61.184688432465,12.));
#74774=CARTESIAN_POINT('Ctrl Pts',(-40.3303525972621,-61.1589592533623,
12.));
#74775=CARTESIAN_POINT('Ctrl Pts',(-40.3254163193806,-61.1332717508799,
12.));
#74776=CARTESIAN_POINT('Ctrl Pts',(-40.3204632662729,-61.1076260105265,
12.));
#74777=CARTESIAN_POINT('Ctrl Pts',(-40.3154935065264,-61.0820221180646,
12.));
#74778=CARTESIAN_POINT('Ctrl Pts',(-40.3105071090308,-61.0564601595047,
12.));
#74779=CARTESIAN_POINT('Ctrl Pts',(-40.3055041429772,-61.0309402210915,
12.));
#74780=CARTESIAN_POINT('Ctrl Pts',(-40.3004846778577,-61.0054623893059,
12.));
#74781=CARTESIAN_POINT('Ctrl Pts',(-40.2954487834688,-60.9800267508781,
12.));
#74782=CARTESIAN_POINT('Ctrl Pts',(-40.2903965299155,-60.9546333927919,
12.));
#74783=CARTESIAN_POINT('Ctrl Pts',(-40.2853279876162,-60.9292824022888,
12.));
#74784=CARTESIAN_POINT('Ctrl Pts',(-40.2802432273105,-60.903973866867,12.));
#74785=CARTESIAN_POINT('Ctrl Pts',(-40.2751423200637,-60.8787078742817,
12.));
#74786=CARTESIAN_POINT('Ctrl Pts',(-40.2700253372644,-60.8534845125535,
12.));
#74787=CARTESIAN_POINT('Ctrl Pts',(-40.2648923506245,-60.8283038699703,
12.));
#74788=CARTESIAN_POINT('Ctrl Pts',(-40.2597434321804,-60.8031660350878,
12.));
#74789=CARTESIAN_POINT('Ctrl Pts',(-40.2545786542957,-60.7780710967253,
12.));
#74790=CARTESIAN_POINT('Ctrl Pts',(-40.2493980896646,-60.7530191439603,
12.));
#74791=CARTESIAN_POINT('Ctrl Pts',(-40.2442018113116,-60.72801026614,12.));
#74792=CARTESIAN_POINT('Ctrl Pts',(-40.2389898925937,-60.7030445528863,
12.));
#74793=CARTESIAN_POINT('Ctrl Pts',(-40.2337624072029,-60.6781220940979,
12.));
#74794=CARTESIAN_POINT('Ctrl Pts',(-40.2285194291702,-60.6532429799493,
12.));
#74795=CARTESIAN_POINT('Ctrl Pts',(-40.2232610328717,-60.6284073008865,
12.));
#74796=CARTESIAN_POINT('Ctrl Pts',(-40.2179872930272,-60.6036151476347,
12.));
#74797=CARTESIAN_POINT('Ctrl Pts',(-40.2126982847012,-60.5788666112043,
12.));
#74798=CARTESIAN_POINT('Ctrl Pts',(-40.2073940833054,-60.5541617828927,
12.));
#74799=CARTESIAN_POINT('Ctrl Pts',(-40.2020747646012,-60.5295007542838,
12.));
#74800=CARTESIAN_POINT('Ctrl Pts',(-40.1967404047055,-60.5048836172423,
12.));
#74801=CARTESIAN_POINT('Ctrl Pts',(-40.1913910800911,-60.4803104639211,
12.));
#74802=CARTESIAN_POINT('Ctrl Pts',(-40.1860268675875,-60.4557813867677,
12.));
#74803=CARTESIAN_POINT('Ctrl Pts',(-40.1806478443828,-60.4312964785269,
12.));
#74804=CARTESIAN_POINT('Ctrl Pts',(-40.1752540880273,-60.4068558322414,
12.));
#74805=CARTESIAN_POINT('Ctrl Pts',(-40.1698456764387,-60.382459541246,12.));
#74806=CARTESIAN_POINT('Ctrl Pts',(-40.1644226879043,-60.3581076991731,
12.));
#74807=CARTESIAN_POINT('Ctrl Pts',(-40.1589852010811,-60.3338003999616,
12.));
#74808=CARTESIAN_POINT('Ctrl Pts',(-40.1535332949978,-60.3095377378589,
12.));
#74809=CARTESIAN_POINT('Ctrl Pts',(-40.1480670490583,-60.2853198074215,
12.));
#74810=CARTESIAN_POINT('Ctrl Pts',(-40.1425865430468,-60.2611467035109,
12.));
#74811=CARTESIAN_POINT('Ctrl Pts',(-40.13709185713,-60.2370185212957,12.));
#74812=CARTESIAN_POINT('Ctrl Pts',(-40.1315830718575,-60.2129353562617,
12.));
#74813=CARTESIAN_POINT('Ctrl Pts',(-40.1260602681644,-60.1888973042151,
12.));
#74814=CARTESIAN_POINT('Ctrl Pts',(-40.120523527374,-60.1649044612829,12.));
#74815=CARTESIAN_POINT('Ctrl Pts',(-40.1149729312036,-60.1409569239092,
12.));
#74816=CARTESIAN_POINT('Ctrl Pts',(-40.1094085617672,-60.1170547888572,
12.));
#74817=CARTESIAN_POINT('Ctrl Pts',(-40.1038305015763,-60.0931981532194,
12.));
#74818=CARTESIAN_POINT('Ctrl Pts',(-40.0982388335421,-60.0693871144207,
12.));
#74819=CARTESIAN_POINT('Ctrl Pts',(-40.0926336409787,-60.0456217702203,
12.));
#74820=CARTESIAN_POINT('Ctrl Pts',(-40.0870150076078,-60.0219022187066,
12.));
#74821=CARTESIAN_POINT('Ctrl Pts',(-40.0813830175629,-59.9982285582991,
12.));
#74822=CARTESIAN_POINT('Ctrl Pts',(-40.0757377553893,-59.974600887759,12.));
#74823=CARTESIAN_POINT('Ctrl Pts',(-40.0700793060475,-59.9510193061929,
12.));
#74824=CARTESIAN_POINT('Ctrl Pts',(-40.0644077549158,-59.927483913055,12.));
#74825=CARTESIAN_POINT('Ctrl Pts',(-40.0587231877959,-59.9039948081428,
12.));
#74826=CARTESIAN_POINT('Ctrl Pts',(-40.0530256909161,-59.8805520915972,
12.));
#74827=CARTESIAN_POINT('Ctrl Pts',(-40.0473153509324,-59.8571558639145,
12.));
#74828=CARTESIAN_POINT('Ctrl Pts',(-40.0415922549315,-59.8338062259492,
12.));
#74829=CARTESIAN_POINT('Ctrl Pts',(-40.0358564904341,-59.8105032789179,
12.));
#74830=CARTESIAN_POINT('Ctrl Pts',(-40.0301081454002,-59.7872471243942,
12.));
#74831=CARTESIAN_POINT('Ctrl Pts',(-40.0243473082337,-59.7640378643106,
12.));
#74832=CARTESIAN_POINT('Ctrl Pts',(-40.0185740677821,-59.7408756009679,
12.));
#74833=CARTESIAN_POINT('Ctrl Pts',(-40.0127885133403,-59.7177604370403,
12.));
#74834=CARTESIAN_POINT('Ctrl Pts',(-40.0069907346537,-59.6946924755773,
12.));
#74835=CARTESIAN_POINT('Ctrl Pts',(-40.0011808219241,-59.6716718200005,
12.));
#74836=CARTESIAN_POINT('Ctrl Pts',(-39.9953588658132,-59.6486985741041,
12.));
#74837=CARTESIAN_POINT('Ctrl Pts',(-39.9895249574448,-59.6257728420669,
12.));
#74838=CARTESIAN_POINT('Ctrl Pts',(-39.9836791884079,-59.6028947284562,
12.));
#74839=CARTESIAN_POINT('Ctrl Pts',(-39.9778216507605,-59.5800643382314,
12.));
#74840=CARTESIAN_POINT('Ctrl Pts',(-39.9719524370345,-59.5572817767388,
12.));
#74841=CARTESIAN_POINT('Ctrl Pts',(-39.9660716402403,-59.5345471497128,
12.));
#74842=CARTESIAN_POINT('Ctrl Pts',(-39.9601793538682,-59.511860563289,12.));
#74843=CARTESIAN_POINT('Ctrl Pts',(-39.9542756718922,-59.4892221240068,
12.));
#74844=CARTESIAN_POINT('Ctrl Pts',(-39.9483606887737,-59.4666319388133,
12.));
#74845=CARTESIAN_POINT('Ctrl Pts',(-39.9424344994672,-59.4440901150582,
12.));
#74846=CARTESIAN_POINT('Ctrl Pts',(-39.9364971994242,-59.4215967604967,
12.));
#74847=CARTESIAN_POINT('Ctrl Pts',(-39.9305488845958,-59.3991519833016,
12.));
#74848=CARTESIAN_POINT('Ctrl Pts',(-39.9245896514367,-59.3767558920675,
12.));
#74849=CARTESIAN_POINT('Ctrl Pts',(-39.9186195969104,-59.3544085958151,
12.));
#74850=CARTESIAN_POINT('Ctrl Pts',(-39.9126388184936,-59.3321102039852,
12.));
#74851=CARTESIAN_POINT('Ctrl Pts',(-39.9066474141803,-59.3098608264419,
12.));
#74852=CARTESIAN_POINT('Ctrl Pts',(-39.9006454824845,-59.2876605734846,
12.));
#74853=CARTESIAN_POINT('Ctrl Pts',(-39.8946331224438,-59.2655095558521,
12.));
#74854=CARTESIAN_POINT('Ctrl Pts',(-39.8886104336242,-59.2434078847247,
12.));
#74855=CARTESIAN_POINT('Ctrl Pts',(-39.8825775161267,-59.2213556717209,
12.));
#74856=CARTESIAN_POINT('Ctrl Pts',(-39.876534470591,-59.1993530289028,12.));
#74857=CARTESIAN_POINT('Ctrl Pts',(-39.8704813981988,-59.1774000687879,
12.));
#74858=CARTESIAN_POINT('Ctrl Pts',(-39.8644184006787,-59.1554969043522,
12.));
#74859=CARTESIAN_POINT('Ctrl Pts',(-39.8583455803105,-59.1336436490342,
12.));
#74860=CARTESIAN_POINT('Ctrl Pts',(-39.8522630399328,-59.1118404167292,
12.));
#74861=CARTESIAN_POINT('Ctrl Pts',(-39.8461708829456,-59.090087321798,12.));
#74862=CARTESIAN_POINT('Ctrl Pts',(-39.8400692133139,-59.0683844790764,
12.));
#74863=CARTESIAN_POINT('Ctrl Pts',(-39.8339581355716,-59.0467320038784,
12.));
#74864=CARTESIAN_POINT('Ctrl Pts',(-39.8278377548262,-59.0251300119973,
12.));
#74865=CARTESIAN_POINT('Ctrl Pts',(-39.821708176766,-59.0035786197024,12.));
#74866=CARTESIAN_POINT('Ctrl Pts',(-39.8155695076626,-58.9820779437484,
12.));
#74867=CARTESIAN_POINT('Ctrl Pts',(-39.8094218543782,-58.9606281013875,
12.));
#74868=CARTESIAN_POINT('Ctrl Pts',(-39.8032653243712,-58.9392292103747,
12.));
#74869=CARTESIAN_POINT('Ctrl Pts',(-39.7971000257044,-58.9178813889703,
12.));
#74870=CARTESIAN_POINT('Ctrl Pts',(-39.7909260670517,-58.8965847559391,
12.));
#74871=CARTESIAN_POINT('Ctrl Pts',(-39.7847435576996,-58.8753394305585,
12.));
#74872=CARTESIAN_POINT('Ctrl Pts',(-39.7785526075478,-58.8541455326231,
12.));
#74873=CARTESIAN_POINT('Ctrl Pts',(-39.772353327112,-58.8330031824453,12.));
#74874=CARTESIAN_POINT('Ctrl Pts',(-39.7661458275274,-58.8119125008517,
12.));
#74875=CARTESIAN_POINT('Ctrl Pts',(-39.7599302205521,-58.7908736091798,
12.));
#74876=CARTESIAN_POINT('Ctrl Pts',(-39.7537066185813,-58.7698866293029,
12.));
#74877=CARTESIAN_POINT('Ctrl Pts',(-39.7474751346598,-58.7489516836445,
12.));
#74878=CARTESIAN_POINT('Ctrl Pts',(-39.7412358824953,-58.7280688951916,
12.));
#74879=CARTESIAN_POINT('Ctrl Pts',(-39.734988976475,-58.7072383875027,12.));
#74880=CARTESIAN_POINT('Ctrl Pts',(-39.7287345316681,-58.6864602847088,
12.));
#74881=CARTESIAN_POINT('Ctrl Pts',(-39.7224726638101,-58.6657347115034,
12.));
#74882=CARTESIAN_POINT('Ctrl Pts',(-39.7162034892899,-58.6450617931274,
12.));
#74883=CARTESIAN_POINT('Ctrl Pts',(-39.7099271251413,-58.6244416553562,
12.));
#74884=CARTESIAN_POINT('Ctrl Pts',(-39.7036436890233,-58.6038744244659,
12.));
#74885=CARTESIAN_POINT('Ctrl Pts',(-39.6973532992539,-58.5833602272743,
12.));
#74886=CARTESIAN_POINT('Ctrl Pts',(-39.6910560748629,-58.5628991912052,
12.));
#74887=CARTESIAN_POINT('Ctrl Pts',(-39.6847521356395,-58.5424914443415,
12.));
#74888=CARTESIAN_POINT('Ctrl Pts',(-39.6784416021826,-58.522137115476,12.));
#74889=CARTESIAN_POINT('Ctrl Pts',(-39.6721245959531,-58.5018363341604,
12.));
#74890=CARTESIAN_POINT('Ctrl Pts',(-39.6658012391815,-58.4815892306066,
12.));
#74891=CARTESIAN_POINT('Ctrl Pts',(-39.6594716547689,-58.4613959355788,
12.));
#74892=CARTESIAN_POINT('Ctrl Pts',(-39.653135966204,-58.4412565802979,12.));
#74893=CARTESIAN_POINT('Ctrl Pts',(-39.6467942974451,-58.4211712963004,
12.));
#74894=CARTESIAN_POINT('Ctrl Pts',(-39.6404467729094,-58.4011402154196,
12.));
#74895=CARTESIAN_POINT('Ctrl Pts',(-39.6340935177476,-58.3811634701037,
12.));
#74896=CARTESIAN_POINT('Ctrl Pts',(-39.6277346580892,-58.3612411936904,
12.));
#74897=CARTESIAN_POINT('Ctrl Pts',(-39.6213703212531,-58.3413735206423,
12.));
#74898=CARTESIAN_POINT('Ctrl Pts',(-39.6150006360914,-58.3215605869221,
12.));
#74899=CARTESIAN_POINT('Ctrl Pts',(-39.6086257327583,-58.3018025297323,
12.));
#74900=CARTESIAN_POINT('Ctrl Pts',(-39.602245742079,-58.2820994868118,12.));
#74901=CARTESIAN_POINT('Ctrl Pts',(-39.5958607950239,-58.2624515958419,
12.));
#74902=CARTESIAN_POINT('Ctrl Pts',(-39.5894710221713,-58.2428589938369,
12.));
#74903=CARTESIAN_POINT('Ctrl Pts',(-39.5830765530891,-58.2233218164365,
12.));
#74904=CARTESIAN_POINT('Ctrl Pts',(-39.57667751752,-58.2038401992457,12.));
#74905=CARTESIAN_POINT('Ctrl Pts',(-39.5702740467999,-58.1844142794338,
12.));
#74906=CARTESIAN_POINT('Ctrl Pts',(-39.563866275018,-58.1650441970387,12.));
#74907=CARTESIAN_POINT('Ctrl Pts',(-39.5574543406982,-58.1457300968499,
12.));
#74908=CARTESIAN_POINT('Ctrl Pts',(-39.5510383869505,-58.126472128574,12.));
#74909=CARTESIAN_POINT('Ctrl Pts',(-39.5446185579638,-58.1072704428928,
12.));
#74910=CARTESIAN_POINT('Ctrl Pts',(-39.5381949959221,-58.088125187992,12.));
#74911=CARTESIAN_POINT('Ctrl Pts',(-39.5317678383217,-58.0690365065374,
12.));
#74912=CARTESIAN_POINT('Ctrl Pts',(-39.5253372136887,-58.0500045308412,
12.));
#74913=CARTESIAN_POINT('Ctrl Pts',(-39.5189032457184,-58.0310293875262,
12.));
#74914=CARTESIAN_POINT('Ctrl Pts',(-39.5124660614976,-58.0121112067895,
12.));
#74915=CARTESIAN_POINT('Ctrl Pts',(-39.5060257981225,-57.9932501298522,
12.));
#74916=CARTESIAN_POINT('Ctrl Pts',(-39.499582610674,-57.974446317937,12.));
#74917=CARTESIAN_POINT('Ctrl Pts',(-39.4931366776714,-57.9556999583892,
12.));
#74918=CARTESIAN_POINT('Ctrl Pts',(-39.4866881842317,-57.937011245663,12.));
#74919=CARTESIAN_POINT('Ctrl Pts',(-39.4802373061058,-57.9183803632403,
12.));
#74920=CARTESIAN_POINT('Ctrl Pts',(-39.473784194937,-57.8998074670478,12.));
#74921=CARTESIAN_POINT('Ctrl Pts',(-39.4673289592259,-57.8812926637177,
12.));
#74922=CARTESIAN_POINT('Ctrl Pts',(-39.4608716627118,-57.8628360096803,
12.));
#74923=CARTESIAN_POINT('Ctrl Pts',(-39.4557042029652,-57.8481172247495,
12.));
#74924=CARTESIAN_POINT('Ctrl Pts',(-39.4518277003553,-57.837104315141,12.));
#74925=CARTESIAN_POINT('Ctrl Pts',(-39.4492429618443,-57.8297740100947,
12.));
#74926=CARTESIAN_POINT('Ctrl Pts',(-39.4479504917287,-57.8261117662438,
12.));
#74927=CARTESIAN_POINT('Ctrl Pts',(-39.2292784191817,-62.9864049293897,
0.));
#74928=CARTESIAN_POINT('Ctrl Pts',(-39.2292784191817,-62.9864049293897,
4.));
#74929=CARTESIAN_POINT('Ctrl Pts',(-39.2292784191818,-62.9864049293897,
8.));
#74930=CARTESIAN_POINT('Ctrl Pts',(-39.2292784191818,-62.9864049293897,
12.));
#74931=CARTESIAN_POINT('Ctrl Pts',(-39.3205491216489,-63.0475916539463,
0.));
#74932=CARTESIAN_POINT('Ctrl Pts',(-39.3205491216489,-63.0475916539463,
4.));
#74933=CARTESIAN_POINT('Ctrl Pts',(-39.320549121649,-63.0475916539464,8.));
#74934=CARTESIAN_POINT('Ctrl Pts',(-39.320549121649,-63.0475916539464,12.));
#74935=CARTESIAN_POINT('Ctrl Pts',(-39.5164137621549,-63.0996457958578,
0.));
#74936=CARTESIAN_POINT('Ctrl Pts',(-39.5164137621549,-63.0996457958578,
4.00000000000001));
#74937=CARTESIAN_POINT('Ctrl Pts',(-39.516413762155,-63.0996457958578,7.99999999999999));
#74938=CARTESIAN_POINT('Ctrl Pts',(-39.516413762155,-63.0996457958578,12.));
#74939=CARTESIAN_POINT('Ctrl Pts',(-39.7049575044671,-63.037870691207,0.));
#74940=CARTESIAN_POINT('Ctrl Pts',(-39.7049575044671,-63.037870691207,3.99999999999999));
#74941=CARTESIAN_POINT('Ctrl Pts',(-39.7049575044672,-63.0378706912071,
8.00000000000001));
#74942=CARTESIAN_POINT('Ctrl Pts',(-39.7049575044672,-63.0378706912071,
12.));
#74943=CARTESIAN_POINT('Ctrl Pts',(-39.7746412831472,-62.9938720098778,
0.));
#74944=CARTESIAN_POINT('Ctrl Pts',(-39.7746412831472,-62.9938720098778,
4.));
#74945=CARTESIAN_POINT('Ctrl Pts',(-39.7746412831473,-62.9938720098779,
8.));
#74946=CARTESIAN_POINT('Ctrl Pts',(-39.7746412831473,-62.9938720098779,
12.));
#74947=CARTESIAN_POINT('',(-39.2292784191817,-62.9864049293897,0.));
#74948=CARTESIAN_POINT('',(-39.7746412831476,-62.9938720098783,0.));
#74949=CARTESIAN_POINT('Ctrl Pts',(-39.2292784191817,-62.9864049293897,
0.));
#74950=CARTESIAN_POINT('Ctrl Pts',(-39.3205491216489,-63.0475916539463,
0.));
#74951=CARTESIAN_POINT('Ctrl Pts',(-39.4324717733666,-63.0773368778958,
0.));
#74952=CARTESIAN_POINT('Ctrl Pts',(-39.5420039277149,-63.0699133682738,
0.));
#74953=CARTESIAN_POINT('Ctrl Pts',(-39.6241530434762,-63.0643457360574,
0.));
#74954=CARTESIAN_POINT('Ctrl Pts',(-39.7049575044671,-63.037870691207,0.));
#74955=CARTESIAN_POINT('Ctrl Pts',(-39.7746412831472,-62.9938720098778,
0.));
#74956=CARTESIAN_POINT('',(-39.7746412831476,-62.9938720098783,12.));
#74957=CARTESIAN_POINT('Ctrl Pts',(-39.7746412831472,-62.9938720098778,
0.));
#74958=CARTESIAN_POINT('Ctrl Pts',(-39.7746412831472,-62.9938720098778,
4.));
#74959=CARTESIAN_POINT('Ctrl Pts',(-39.7746412831473,-62.9938720098779,
8.));
#74960=CARTESIAN_POINT('Ctrl Pts',(-39.7746412831473,-62.9938720098779,
12.));
#74961=CARTESIAN_POINT('',(-39.2292784191818,-62.9864049293897,12.));
#74962=CARTESIAN_POINT('Ctrl Pts',(-39.7746412831473,-62.9938720098779,
12.));
#74963=CARTESIAN_POINT('Ctrl Pts',(-39.7049575044672,-63.0378706912071,
12.));
#74964=CARTESIAN_POINT('Ctrl Pts',(-39.6241530434763,-63.0643457360574,
12.));
#74965=CARTESIAN_POINT('Ctrl Pts',(-39.542003927715,-63.0699133682739,12.));
#74966=CARTESIAN_POINT('Ctrl Pts',(-39.4324717733667,-63.0773368778958,
12.));
#74967=CARTESIAN_POINT('Ctrl Pts',(-39.320549121649,-63.0475916539464,12.));
#74968=CARTESIAN_POINT('Ctrl Pts',(-39.2292784191818,-62.9864049293897,
12.));
#74969=CARTESIAN_POINT('Ctrl Pts',(-39.2292784191818,-62.9864049293897,
12.));
#74970=CARTESIAN_POINT('Ctrl Pts',(-39.2292784191818,-62.9864049293897,
8.));
#74971=CARTESIAN_POINT('Ctrl Pts',(-39.2292784191817,-62.9864049293897,
4.));
#74972=CARTESIAN_POINT('Ctrl Pts',(-39.2292784191817,-62.9864049293897,
0.));
#74973=CARTESIAN_POINT('Origin',(-2.01319694273778E-10,-3.16193356404481E-10,
0.));
#74974=CARTESIAN_POINT('Origin',(-2.01319694273778E-10,-3.16193356404481E-10,
12.));
#74975=CARTESIAN_POINT('Origin',(-2.01319694273778E-10,-3.16193356404481E-10,
0.));
#74976=CARTESIAN_POINT('Ctrl Pts',(-45.591148170023,-58.9211100416396,0.));
#74977=CARTESIAN_POINT('Ctrl Pts',(-45.591148170023,-58.9211100416396,4.));
#74978=CARTESIAN_POINT('Ctrl Pts',(-45.5911481700231,-58.9211100416396,
8.));
#74979=CARTESIAN_POINT('Ctrl Pts',(-45.5911481700231,-58.9211100416396,
12.));
#74980=CARTESIAN_POINT('Ctrl Pts',(-45.6780528262179,-58.8538661785413,
0.));
#74981=CARTESIAN_POINT('Ctrl Pts',(-45.6780528262179,-58.8538661785413,
4.));
#74982=CARTESIAN_POINT('Ctrl Pts',(-45.6780528262179,-58.8538661785413,
8.));
#74983=CARTESIAN_POINT('Ctrl Pts',(-45.6780528262179,-58.8538661785413,
12.));
#74984=CARTESIAN_POINT('Ctrl Pts',(-45.7893619681937,-58.6845061116499,
0.));
#74985=CARTESIAN_POINT('Ctrl Pts',(-45.7893619681937,-58.6845061116499,
4.00000000000001));
#74986=CARTESIAN_POINT('Ctrl Pts',(-45.7893619681937,-58.6845061116498,
7.99999999999999));
#74987=CARTESIAN_POINT('Ctrl Pts',(-45.7893619681937,-58.6845061116498,
12.));
#74988=CARTESIAN_POINT('Ctrl Pts',(-45.790366715598,-58.486102814171,0.));
#74989=CARTESIAN_POINT('Ctrl Pts',(-45.790366715598,-58.486102814171,4.));
#74990=CARTESIAN_POINT('Ctrl Pts',(-45.7903667155981,-58.486102814171,8.00000000000001));
#74991=CARTESIAN_POINT('Ctrl Pts',(-45.7903667155981,-58.486102814171,12.));
#74992=CARTESIAN_POINT('Ctrl Pts',(-45.7706564944768,-58.4060826907379,
0.));
#74993=CARTESIAN_POINT('Ctrl Pts',(-45.7706564944768,-58.4060826907379,
4.));
#74994=CARTESIAN_POINT('Ctrl Pts',(-45.7706564944768,-58.4060826907378,
8.));
#74995=CARTESIAN_POINT('Ctrl Pts',(-45.7706564944768,-58.4060826907378,
12.));
#74996=CARTESIAN_POINT('',(-45.591148170023,-58.9211100416396,0.));
#74997=CARTESIAN_POINT('',(-45.7706564944767,-58.4060826907379,0.));
#74998=CARTESIAN_POINT('Ctrl Pts',(-45.591148170023,-58.9211100416396,0.));
#74999=CARTESIAN_POINT('Ctrl Pts',(-45.6780528262179,-58.8538661785413,
0.));
#75000=CARTESIAN_POINT('Ctrl Pts',(-45.741658050204,-58.7570889974605,0.));
#75001=CARTESIAN_POINT('Ctrl Pts',(-45.7692455126975,-58.6508283125144,
0.));
#75002=CARTESIAN_POINT('Ctrl Pts',(-45.7899361095676,-58.5711327988048,
0.));
#75003=CARTESIAN_POINT('Ctrl Pts',(-45.790366715598,-58.486102814171,0.));
#75004=CARTESIAN_POINT('Ctrl Pts',(-45.7706564944768,-58.4060826907379,
0.));
#75005=CARTESIAN_POINT('',(-45.7706564944767,-58.4060826907378,12.));
#75006=CARTESIAN_POINT('Ctrl Pts',(-45.7706564944768,-58.4060826907379,
0.));
#75007=CARTESIAN_POINT('Ctrl Pts',(-45.7706564944768,-58.4060826907379,
4.));
#75008=CARTESIAN_POINT('Ctrl Pts',(-45.7706564944768,-58.4060826907378,
8.));
#75009=CARTESIAN_POINT('Ctrl Pts',(-45.7706564944768,-58.4060826907378,
12.));
#75010=CARTESIAN_POINT('',(-45.5911481700231,-58.9211100416396,12.));
#75011=CARTESIAN_POINT('Ctrl Pts',(-45.7706564944768,-58.4060826907378,
12.));
#75012=CARTESIAN_POINT('Ctrl Pts',(-45.7903667155981,-58.486102814171,12.));
#75013=CARTESIAN_POINT('Ctrl Pts',(-45.7899361095676,-58.5711327988048,
12.));
#75014=CARTESIAN_POINT('Ctrl Pts',(-45.7692455126975,-58.6508283125143,
12.));
#75015=CARTESIAN_POINT('Ctrl Pts',(-45.7416580502041,-58.7570889974604,
12.));
#75016=CARTESIAN_POINT('Ctrl Pts',(-45.6780528262179,-58.8538661785413,
12.));
#75017=CARTESIAN_POINT('Ctrl Pts',(-45.5911481700231,-58.9211100416396,
12.));
#75018=CARTESIAN_POINT('Ctrl Pts',(-45.5911481700231,-58.9211100416396,
12.));
#75019=CARTESIAN_POINT('Ctrl Pts',(-45.5911481700231,-58.9211100416396,
8.));
#75020=CARTESIAN_POINT('Ctrl Pts',(-45.591148170023,-58.9211100416396,4.));
#75021=CARTESIAN_POINT('Ctrl Pts',(-45.591148170023,-58.9211100416396,0.));
#75022=CARTESIAN_POINT('Ctrl Pts',(-44.3377168516418,-54.1679505278134,
0.));
#75023=CARTESIAN_POINT('Ctrl Pts',(-44.3377168516418,-54.1679505278134,
12.));
#75024=CARTESIAN_POINT('Ctrl Pts',(-44.3393235891014,-54.1714861895278,
0.));
#75025=CARTESIAN_POINT('Ctrl Pts',(-44.3393235891014,-54.1714861895278,
12.));
#75026=CARTESIAN_POINT('Ctrl Pts',(-44.3425373700829,-54.1785633257456,
0.));
#75027=CARTESIAN_POINT('Ctrl Pts',(-44.3425373700829,-54.1785633257456,
12.));
#75028=CARTESIAN_POINT('Ctrl Pts',(-44.3473589597468,-54.1891964684439,
0.));
#75029=CARTESIAN_POINT('Ctrl Pts',(-44.3473589597468,-54.1891964684439,
12.));
#75030=CARTESIAN_POINT('Ctrl Pts',(-44.3537895823819,-54.203408870162,0.));
#75031=CARTESIAN_POINT('Ctrl Pts',(-44.3537895823819,-54.203408870162,12.));
#75032=CARTESIAN_POINT('Ctrl Pts',(-44.3618309103245,-54.2212325005847,
0.));
#75033=CARTESIAN_POINT('Ctrl Pts',(-44.3618309103245,-54.2212325005847,
12.));
#75034=CARTESIAN_POINT('Ctrl Pts',(-44.369875253351,-54.2391142386354,0.));
#75035=CARTESIAN_POINT('Ctrl Pts',(-44.369875253351,-54.2391142386354,12.));
#75036=CARTESIAN_POINT('Ctrl Pts',(-44.3779225430461,-54.2570540336536,
0.));
#75037=CARTESIAN_POINT('Ctrl Pts',(-44.3779225430461,-54.2570540336536,
12.));
#75038=CARTESIAN_POINT('Ctrl Pts',(-44.3859726620288,-54.2750517888695,
0.));
#75039=CARTESIAN_POINT('Ctrl Pts',(-44.3859726620288,-54.2750517888695,
12.));
#75040=CARTESIAN_POINT('Ctrl Pts',(-44.3940254456427,-54.2931073621661,
0.));
#75041=CARTESIAN_POINT('Ctrl Pts',(-44.3940254456427,-54.2931073621661,
12.));
#75042=CARTESIAN_POINT('Ctrl Pts',(-44.4020807028144,-54.3112205860776,
0.));
#75043=CARTESIAN_POINT('Ctrl Pts',(-44.4020807028144,-54.3112205860776,
12.));
#75044=CARTESIAN_POINT('Ctrl Pts',(-44.4101382321834,-54.3293912830237,
0.));
#75045=CARTESIAN_POINT('Ctrl Pts',(-44.4101382321834,-54.3293912830237,
12.));
#75046=CARTESIAN_POINT('Ctrl Pts',(-44.4181978395814,-54.347619281931,0.));
#75047=CARTESIAN_POINT('Ctrl Pts',(-44.4181978395814,-54.347619281931,12.));
#75048=CARTESIAN_POINT('Ctrl Pts',(-44.4262593564664,-54.3659044357064,
0.));
#75049=CARTESIAN_POINT('Ctrl Pts',(-44.4262593564664,-54.3659044357064,
12.));
#75050=CARTESIAN_POINT('Ctrl Pts',(-44.4343226339555,-54.3842466156151,
0.));
#75051=CARTESIAN_POINT('Ctrl Pts',(-44.4343226339555,-54.3842466156151,
12.));
#75052=CARTESIAN_POINT('Ctrl Pts',(-44.442387534098,-54.4026457030316,0.));
#75053=CARTESIAN_POINT('Ctrl Pts',(-44.442387534098,-54.4026457030316,12.));
#75054=CARTESIAN_POINT('Ctrl Pts',(-44.4504539226336,-54.4211015825959,
0.));
#75055=CARTESIAN_POINT('Ctrl Pts',(-44.4504539226336,-54.4211015825959,
12.));
#75056=CARTESIAN_POINT('Ctrl Pts',(-44.4585216599933,-54.4396141337008,
0.));
#75057=CARTESIAN_POINT('Ctrl Pts',(-44.4585216599933,-54.4396141337008,
12.));
#75058=CARTESIAN_POINT('Ctrl Pts',(-44.4665905967701,-54.4581832262072,
0.));
#75059=CARTESIAN_POINT('Ctrl Pts',(-44.4665905967701,-54.4581832262072,
12.));
#75060=CARTESIAN_POINT('Ctrl Pts',(-44.4746605784056,-54.4768087248854,
0.));
#75061=CARTESIAN_POINT('Ctrl Pts',(-44.4746605784056,-54.4768087248854,
12.));
#75062=CARTESIAN_POINT('Ctrl Pts',(-44.482731448127,-54.4954904921938,0.));
#75063=CARTESIAN_POINT('Ctrl Pts',(-44.482731448127,-54.4954904921938,12.));
#75064=CARTESIAN_POINT('Ctrl Pts',(-44.4908030503209,-54.5142283914684,
0.));
#75065=CARTESIAN_POINT('Ctrl Pts',(-44.4908030503209,-54.5142283914684,
12.));
#75066=CARTESIAN_POINT('Ctrl Pts',(-44.4988752343715,-54.5330222905438,
0.));
#75067=CARTESIAN_POINT('Ctrl Pts',(-44.4988752343715,-54.5330222905438,
12.));
#75068=CARTESIAN_POINT('Ctrl Pts',(-44.5069478544945,-54.5518720616016,
0.));
#75069=CARTESIAN_POINT('Ctrl Pts',(-44.5069478544945,-54.5518720616016,
12.));
#75070=CARTESIAN_POINT('Ctrl Pts',(-44.5150207678988,-54.5707775794412,
0.));
#75071=CARTESIAN_POINT('Ctrl Pts',(-44.5150207678988,-54.5707775794412,
12.));
#75072=CARTESIAN_POINT('Ctrl Pts',(-44.5230938335167,-54.5897387202815,
0.));
#75073=CARTESIAN_POINT('Ctrl Pts',(-44.5230938335167,-54.5897387202815,
12.));
#75074=CARTESIAN_POINT('Ctrl Pts',(-44.5311669104515,-54.6087553602914,
0.));
#75075=CARTESIAN_POINT('Ctrl Pts',(-44.5311669104515,-54.6087553602914,
12.));
#75076=CARTESIAN_POINT('Ctrl Pts',(-44.5392398566802,-54.6278273743587,
0.));
#75077=CARTESIAN_POINT('Ctrl Pts',(-44.5392398566802,-54.6278273743587,
12.));
#75078=CARTESIAN_POINT('Ctrl Pts',(-44.5473125297311,-54.6469546367408,
0.));
#75079=CARTESIAN_POINT('Ctrl Pts',(-44.5473125297311,-54.6469546367408,
12.));
#75080=CARTESIAN_POINT('Ctrl Pts',(-44.5553847872721,-54.6661370216252,
0.));
#75081=CARTESIAN_POINT('Ctrl Pts',(-44.5553847872721,-54.6661370216252,
12.));
#75082=CARTESIAN_POINT('Ctrl Pts',(-44.5634564876863,-54.6853744036751,
0.));
#75083=CARTESIAN_POINT('Ctrl Pts',(-44.5634564876863,-54.6853744036751,
12.));
#75084=CARTESIAN_POINT('Ctrl Pts',(-44.5715274907619,-54.7046666586754,
0.));
#75085=CARTESIAN_POINT('Ctrl Pts',(-44.5715274907619,-54.7046666586754,
12.));
#75086=CARTESIAN_POINT('Ctrl Pts',(-44.5795976579454,-54.7240136637717,
0.));
#75087=CARTESIAN_POINT('Ctrl Pts',(-44.5795976579454,-54.7240136637717,
12.));
#75088=CARTESIAN_POINT('Ctrl Pts',(-44.5876668519661,-54.7434152971267,
0.));
#75089=CARTESIAN_POINT('Ctrl Pts',(-44.5876668519661,-54.7434152971267,
12.));
#75090=CARTESIAN_POINT('Ctrl Pts',(-44.5957349366059,-54.7628714377037,
0.));
#75091=CARTESIAN_POINT('Ctrl Pts',(-44.5957349366059,-54.7628714377037,
12.));
#75092=CARTESIAN_POINT('Ctrl Pts',(-44.6038017764309,-54.7823819650149,
0.));
#75093=CARTESIAN_POINT('Ctrl Pts',(-44.6038017764309,-54.7823819650149,
12.));
#75094=CARTESIAN_POINT('Ctrl Pts',(-44.6118672364906,-54.8019467588278,
0.));
#75095=CARTESIAN_POINT('Ctrl Pts',(-44.6118672364906,-54.8019467588278,
12.));
#75096=CARTESIAN_POINT('Ctrl Pts',(-44.6199311823293,-54.8215656991837,
0.));
#75097=CARTESIAN_POINT('Ctrl Pts',(-44.6199311823293,-54.8215656991837,
12.));
#75098=CARTESIAN_POINT('Ctrl Pts',(-44.6279934801169,-54.8412386665276,
0.));
#75099=CARTESIAN_POINT('Ctrl Pts',(-44.6279934801169,-54.8412386665276,
12.));
#75100=CARTESIAN_POINT('Ctrl Pts',(-44.6360539967392,-54.860965541796,0.));
#75101=CARTESIAN_POINT('Ctrl Pts',(-44.6360539967392,-54.860965541796,12.));
#75102=CARTESIAN_POINT('Ctrl Pts',(-44.6441125999063,-54.8807462065164,
0.));
#75103=CARTESIAN_POINT('Ctrl Pts',(-44.6441125999063,-54.8807462065164,
12.));
#75104=CARTESIAN_POINT('Ctrl Pts',(-44.6521691582533,-54.9005805428969,
0.));
#75105=CARTESIAN_POINT('Ctrl Pts',(-44.6521691582533,-54.9005805428969,
12.));
#75106=CARTESIAN_POINT('Ctrl Pts',(-44.6602235412836,-54.9204684337822,
0.));
#75107=CARTESIAN_POINT('Ctrl Pts',(-44.6602235412836,-54.9204684337822,
12.));
#75108=CARTESIAN_POINT('Ctrl Pts',(-44.6682756193147,-54.9404097626077,
0.));
#75109=CARTESIAN_POINT('Ctrl Pts',(-44.6682756193147,-54.9404097626077,
12.));
#75110=CARTESIAN_POINT('Ctrl Pts',(-44.6763252634258,-54.9604044133501,
0.));
#75111=CARTESIAN_POINT('Ctrl Pts',(-44.6763252634258,-54.9604044133501,
12.));
#75112=CARTESIAN_POINT('Ctrl Pts',(-44.6843723454,-54.9804522704686,0.));
#75113=CARTESIAN_POINT('Ctrl Pts',(-44.6843723454,-54.9804522704686,12.));
#75114=CARTESIAN_POINT('Ctrl Pts',(-44.6924167376869,-55.0005532188667,
0.));
#75115=CARTESIAN_POINT('Ctrl Pts',(-44.6924167376869,-55.0005532188667,
12.));
#75116=CARTESIAN_POINT('Ctrl Pts',(-44.7004583134249,-55.0207071439237,
0.));
#75117=CARTESIAN_POINT('Ctrl Pts',(-44.7004583134249,-55.0207071439237,
12.));
#75118=CARTESIAN_POINT('Ctrl Pts',(-44.7084969464513,-55.0409139315078,
0.));
#75119=CARTESIAN_POINT('Ctrl Pts',(-44.7084969464513,-55.0409139315078,
12.));
#75120=CARTESIAN_POINT('Ctrl Pts',(-44.7165325113159,-55.0611734679894,
0.));
#75121=CARTESIAN_POINT('Ctrl Pts',(-44.7165325113159,-55.0611734679894,
12.));
#75122=CARTESIAN_POINT('Ctrl Pts',(-44.7245648832979,-55.0814856402496,
0.));
#75123=CARTESIAN_POINT('Ctrl Pts',(-44.7245648832979,-55.0814856402496,
12.));
#75124=CARTESIAN_POINT('Ctrl Pts',(-44.7325939384035,-55.1018503356796,
0.));
#75125=CARTESIAN_POINT('Ctrl Pts',(-44.7325939384035,-55.1018503356796,
12.));
#75126=CARTESIAN_POINT('Ctrl Pts',(-44.740619553348,-55.1222674421743,0.));
#75127=CARTESIAN_POINT('Ctrl Pts',(-44.740619553348,-55.1222674421743,12.));
#75128=CARTESIAN_POINT('Ctrl Pts',(-44.748641605542,-55.14273684812,0.));
#75129=CARTESIAN_POINT('Ctrl Pts',(-44.748641605542,-55.14273684812,12.));
#75130=CARTESIAN_POINT('Ctrl Pts',(-44.7566599730773,-55.1632584423815,
0.));
#75131=CARTESIAN_POINT('Ctrl Pts',(-44.7566599730773,-55.1632584423815,
12.));
#75132=CARTESIAN_POINT('Ctrl Pts',(-44.7646745347109,-55.1838321142779,
0.));
#75133=CARTESIAN_POINT('Ctrl Pts',(-44.7646745347109,-55.1838321142779,
12.));
#75134=CARTESIAN_POINT('Ctrl Pts',(-44.7726851698619,-55.2044577535866,
0.));
#75135=CARTESIAN_POINT('Ctrl Pts',(-44.7726851698619,-55.2044577535866,
12.));
#75136=CARTESIAN_POINT('Ctrl Pts',(-44.7806917586077,-55.2251352505475,
0.));
#75137=CARTESIAN_POINT('Ctrl Pts',(-44.7806917586077,-55.2251352505475,
12.));
#75138=CARTESIAN_POINT('Ctrl Pts',(-44.7886941816823,-55.2458644958617,
0.));
#75139=CARTESIAN_POINT('Ctrl Pts',(-44.7886941816823,-55.2458644958617,
12.));
#75140=CARTESIAN_POINT('Ctrl Pts',(-44.7966923204741,-55.2666453806883,
0.));
#75141=CARTESIAN_POINT('Ctrl Pts',(-44.7966923204741,-55.2666453806883,
12.));
#75142=CARTESIAN_POINT('Ctrl Pts',(-44.8046860570245,-55.287477796635,0.));
#75143=CARTESIAN_POINT('Ctrl Pts',(-44.8046860570245,-55.287477796635,12.));
#75144=CARTESIAN_POINT('Ctrl Pts',(-44.812675274021,-55.3083616357605,0.));
#75145=CARTESIAN_POINT('Ctrl Pts',(-44.812675274021,-55.3083616357605,12.));
#75146=CARTESIAN_POINT('Ctrl Pts',(-44.8206598547889,-55.3292967905726,
0.));
#75147=CARTESIAN_POINT('Ctrl Pts',(-44.8206598547889,-55.3292967905726,
12.));
#75148=CARTESIAN_POINT('Ctrl Pts',(-44.8286396832849,-55.350283154023,0.));
#75149=CARTESIAN_POINT('Ctrl Pts',(-44.8286396832849,-55.350283154023,12.));
#75150=CARTESIAN_POINT('Ctrl Pts',(-44.8366146440896,-55.3713206194962,
0.));
#75151=CARTESIAN_POINT('Ctrl Pts',(-44.8366146440896,-55.3713206194962,
12.));
#75152=CARTESIAN_POINT('Ctrl Pts',(-44.8445846224034,-55.3924090808002,
0.));
#75153=CARTESIAN_POINT('Ctrl Pts',(-44.8445846224034,-55.3924090808002,
12.));
#75154=CARTESIAN_POINT('Ctrl Pts',(-44.8525495040397,-55.4135484321706,
0.));
#75155=CARTESIAN_POINT('Ctrl Pts',(-44.8525495040397,-55.4135484321706,
12.));
#75156=CARTESIAN_POINT('Ctrl Pts',(-44.8605091754208,-55.4347385682697,
0.));
#75157=CARTESIAN_POINT('Ctrl Pts',(-44.8605091754208,-55.4347385682697,
12.));
#75158=CARTESIAN_POINT('Ctrl Pts',(-44.8684635235727,-55.4559793841838,
0.));
#75159=CARTESIAN_POINT('Ctrl Pts',(-44.8684635235727,-55.4559793841838,
12.));
#75160=CARTESIAN_POINT('Ctrl Pts',(-44.8764124361218,-55.4772707754139,
0.));
#75161=CARTESIAN_POINT('Ctrl Pts',(-44.8764124361218,-55.4772707754139,
12.));
#75162=CARTESIAN_POINT('Ctrl Pts',(-44.8843558012903,-55.4986126378676,
0.));
#75163=CARTESIAN_POINT('Ctrl Pts',(-44.8843558012903,-55.4986126378676,
12.));
#75164=CARTESIAN_POINT('Ctrl Pts',(-44.8922935078905,-55.5200048678648,
0.));
#75165=CARTESIAN_POINT('Ctrl Pts',(-44.8922935078905,-55.5200048678648,
12.));
#75166=CARTESIAN_POINT('Ctrl Pts',(-44.9002254453192,-55.541447362135,0.));
#75167=CARTESIAN_POINT('Ctrl Pts',(-44.9002254453192,-55.541447362135,12.));
#75168=CARTESIAN_POINT('Ctrl Pts',(-44.9081515035525,-55.5629400178136,
0.));
#75169=CARTESIAN_POINT('Ctrl Pts',(-44.9081515035525,-55.5629400178136,
12.));
#75170=CARTESIAN_POINT('Ctrl Pts',(-44.9160715731425,-55.5844827324315,
0.));
#75171=CARTESIAN_POINT('Ctrl Pts',(-44.9160715731425,-55.5844827324315,
12.));
#75172=CARTESIAN_POINT('Ctrl Pts',(-44.9239855452119,-55.6060754039089,
0.));
#75173=CARTESIAN_POINT('Ctrl Pts',(-44.9239855452119,-55.6060754039089,
12.));
#75174=CARTESIAN_POINT('Ctrl Pts',(-44.9318933114483,-55.6277179305604,
0.));
#75175=CARTESIAN_POINT('Ctrl Pts',(-44.9318933114483,-55.6277179305604,
12.));
#75176=CARTESIAN_POINT('Ctrl Pts',(-44.9397947640996,-55.6494102110922,
0.));
#75177=CARTESIAN_POINT('Ctrl Pts',(-44.9397947640996,-55.6494102110922,
12.));
#75178=CARTESIAN_POINT('Ctrl Pts',(-44.9476897959694,-55.671152144599,0.));
#75179=CARTESIAN_POINT('Ctrl Pts',(-44.9476897959694,-55.671152144599,12.));
#75180=CARTESIAN_POINT('Ctrl Pts',(-44.9555783004133,-55.6929436305522,
0.));
#75181=CARTESIAN_POINT('Ctrl Pts',(-44.9555783004133,-55.6929436305522,
12.));
#75182=CARTESIAN_POINT('Ctrl Pts',(-44.9634601713352,-55.7147845687969,
0.));
#75183=CARTESIAN_POINT('Ctrl Pts',(-44.9634601713352,-55.7147845687969,
12.));
#75184=CARTESIAN_POINT('Ctrl Pts',(-44.9713353031827,-55.7366748595582,
0.));
#75185=CARTESIAN_POINT('Ctrl Pts',(-44.9713353031827,-55.7366748595582,
12.));
#75186=CARTESIAN_POINT('Ctrl Pts',(-44.979203590942,-55.7586144034376,0.));
#75187=CARTESIAN_POINT('Ctrl Pts',(-44.979203590942,-55.7586144034376,12.));
#75188=CARTESIAN_POINT('Ctrl Pts',(-44.9870649301333,-55.7806031014093,
0.));
#75189=CARTESIAN_POINT('Ctrl Pts',(-44.9870649301333,-55.7806031014093,
12.));
#75190=CARTESIAN_POINT('Ctrl Pts',(-44.9949192168073,-55.8026408548078,
0.));
#75191=CARTESIAN_POINT('Ctrl Pts',(-44.9949192168073,-55.8026408548078,
12.));
#75192=CARTESIAN_POINT('Ctrl Pts',(-45.002766347541,-55.8247275653257,0.));
#75193=CARTESIAN_POINT('Ctrl Pts',(-45.002766347541,-55.8247275653257,12.));
#75194=CARTESIAN_POINT('Ctrl Pts',(-45.0106062194325,-55.8468631350195,
0.));
#75195=CARTESIAN_POINT('Ctrl Pts',(-45.0106062194325,-55.8468631350195,
12.));
#75196=CARTESIAN_POINT('Ctrl Pts',(-45.0184387300968,-55.8690474663058,
0.));
#75197=CARTESIAN_POINT('Ctrl Pts',(-45.0184387300968,-55.8690474663058,
12.));
#75198=CARTESIAN_POINT('Ctrl Pts',(-45.0262637776623,-55.8912804619588,
0.));
#75199=CARTESIAN_POINT('Ctrl Pts',(-45.0262637776623,-55.8912804619588,
12.));
#75200=CARTESIAN_POINT('Ctrl Pts',(-45.0340812607676,-55.9135620250977,
0.));
#75201=CARTESIAN_POINT('Ctrl Pts',(-45.0340812607676,-55.9135620250977,
12.));
#75202=CARTESIAN_POINT('Ctrl Pts',(-45.041891078557,-55.9358920591861,0.));
#75203=CARTESIAN_POINT('Ctrl Pts',(-45.041891078557,-55.9358920591861,12.));
#75204=CARTESIAN_POINT('Ctrl Pts',(-45.0496931306766,-55.958270468037,0.));
#75205=CARTESIAN_POINT('Ctrl Pts',(-45.0496931306766,-55.958270468037,12.));
#75206=CARTESIAN_POINT('Ctrl Pts',(-45.0574873172696,-55.9806971558099,
0.));
#75207=CARTESIAN_POINT('Ctrl Pts',(-45.0574873172696,-55.9806971558099,
12.));
#75208=CARTESIAN_POINT('Ctrl Pts',(-45.0652735389729,-56.0031720270074,
0.));
#75209=CARTESIAN_POINT('Ctrl Pts',(-45.0652735389729,-56.0031720270074,
12.));
#75210=CARTESIAN_POINT('Ctrl Pts',(-45.0730516969142,-56.025694986463,0.));
#75211=CARTESIAN_POINT('Ctrl Pts',(-45.0730516969142,-56.025694986463,12.));
#75212=CARTESIAN_POINT('Ctrl Pts',(-45.0808216927082,-56.0482659393412,
0.));
#75213=CARTESIAN_POINT('Ctrl Pts',(-45.0808216927082,-56.0482659393412,
12.));
#75214=CARTESIAN_POINT('Ctrl Pts',(-45.0885834284513,-56.070884791141,0.));
#75215=CARTESIAN_POINT('Ctrl Pts',(-45.0885834284513,-56.070884791141,12.));
#75216=CARTESIAN_POINT('Ctrl Pts',(-45.0963368067177,-56.0935514476945,
0.));
#75217=CARTESIAN_POINT('Ctrl Pts',(-45.0963368067177,-56.0935514476945,
12.));
#75218=CARTESIAN_POINT('Ctrl Pts',(-45.1040817305563,-56.1162658151621,
0.));
#75219=CARTESIAN_POINT('Ctrl Pts',(-45.1040817305563,-56.1162658151621,
12.));
#75220=CARTESIAN_POINT('Ctrl Pts',(-45.1118181034888,-56.1390278000226,
0.));
#75221=CARTESIAN_POINT('Ctrl Pts',(-45.1118181034888,-56.1390278000226,
12.));
#75222=CARTESIAN_POINT('Ctrl Pts',(-45.119545829506,-56.1618373090729,0.));
#75223=CARTESIAN_POINT('Ctrl Pts',(-45.119545829506,-56.1618373090729,12.));
#75224=CARTESIAN_POINT('Ctrl Pts',(-45.1272648130627,-56.1846942494321,
0.));
#75225=CARTESIAN_POINT('Ctrl Pts',(-45.1272648130627,-56.1846942494321,
12.));
#75226=CARTESIAN_POINT('Ctrl Pts',(-45.1349749590736,-56.2075985285391,
0.));
#75227=CARTESIAN_POINT('Ctrl Pts',(-45.1349749590736,-56.2075985285391,
12.));
#75228=CARTESIAN_POINT('Ctrl Pts',(-45.1426761729107,-56.2305500541491,
0.));
#75229=CARTESIAN_POINT('Ctrl Pts',(-45.1426761729107,-56.2305500541491,
12.));
#75230=CARTESIAN_POINT('Ctrl Pts',(-45.150368360401,-56.2535487343227,0.));
#75231=CARTESIAN_POINT('Ctrl Pts',(-45.150368360401,-56.2535487343227,12.));
#75232=CARTESIAN_POINT('Ctrl Pts',(-45.158051427823,-56.2765944774252,0.));
#75233=CARTESIAN_POINT('Ctrl Pts',(-45.158051427823,-56.2765944774252,12.));
#75234=CARTESIAN_POINT('Ctrl Pts',(-45.1657252819018,-56.2996871921321,
0.));
#75235=CARTESIAN_POINT('Ctrl Pts',(-45.1657252819018,-56.2996871921321,
12.));
#75236=CARTESIAN_POINT('Ctrl Pts',(-45.1733898298062,-56.3228267874265,
0.));
#75237=CARTESIAN_POINT('Ctrl Pts',(-45.1733898298062,-56.3228267874265,
12.));
#75238=CARTESIAN_POINT('Ctrl Pts',(-45.1810449791451,-56.3460131725962,
0.));
#75239=CARTESIAN_POINT('Ctrl Pts',(-45.1810449791451,-56.3460131725962,
12.));
#75240=CARTESIAN_POINT('Ctrl Pts',(-45.1886906379664,-56.3692462572228,
0.));
#75241=CARTESIAN_POINT('Ctrl Pts',(-45.1886906379664,-56.3692462572228,
12.));
#75242=CARTESIAN_POINT('Ctrl Pts',(-45.1963267147527,-56.3925259511804,
0.));
#75243=CARTESIAN_POINT('Ctrl Pts',(-45.1963267147527,-56.3925259511804,
12.));
#75244=CARTESIAN_POINT('Ctrl Pts',(-45.2039531184172,-56.4158521646412,
0.));
#75245=CARTESIAN_POINT('Ctrl Pts',(-45.2039531184172,-56.4158521646412,
12.));
#75246=CARTESIAN_POINT('Ctrl Pts',(-45.2115697583002,-56.4392248080733,
0.));
#75247=CARTESIAN_POINT('Ctrl Pts',(-45.2115697583002,-56.4392248080733,
12.));
#75248=CARTESIAN_POINT('Ctrl Pts',(-45.2191765441666,-56.4626437922385,
0.));
#75249=CARTESIAN_POINT('Ctrl Pts',(-45.2191765441666,-56.4626437922385,
12.));
#75250=CARTESIAN_POINT('Ctrl Pts',(-45.2267733862046,-56.4861090281819,
0.));
#75251=CARTESIAN_POINT('Ctrl Pts',(-45.2267733862046,-56.4861090281819,
12.));
#75252=CARTESIAN_POINT('Ctrl Pts',(-45.2343601950222,-56.5096204272299,
0.));
#75253=CARTESIAN_POINT('Ctrl Pts',(-45.2343601950222,-56.5096204272299,
12.));
#75254=CARTESIAN_POINT('Ctrl Pts',(-45.2419368816423,-56.533177900995,0.));
#75255=CARTESIAN_POINT('Ctrl Pts',(-45.2419368816423,-56.533177900995,12.));
#75256=CARTESIAN_POINT('Ctrl Pts',(-45.2495033574997,-56.5567813613752,
0.));
#75257=CARTESIAN_POINT('Ctrl Pts',(-45.2495033574997,-56.5567813613752,
12.));
#75258=CARTESIAN_POINT('Ctrl Pts',(-45.2570595344382,-56.5804307205507,
0.));
#75259=CARTESIAN_POINT('Ctrl Pts',(-45.2570595344382,-56.5804307205507,
12.));
#75260=CARTESIAN_POINT('Ctrl Pts',(-45.2646053247094,-56.604125890975,0.));
#75261=CARTESIAN_POINT('Ctrl Pts',(-45.2646053247094,-56.604125890975,12.));
#75262=CARTESIAN_POINT('Ctrl Pts',(-45.2721406409706,-56.6278667853716,
0.));
#75263=CARTESIAN_POINT('Ctrl Pts',(-45.2721406409706,-56.6278667853716,
12.));
#75264=CARTESIAN_POINT('Ctrl Pts',(-45.2796653962796,-56.6516533167398,
0.));
#75265=CARTESIAN_POINT('Ctrl Pts',(-45.2796653962796,-56.6516533167398,
12.));
#75266=CARTESIAN_POINT('Ctrl Pts',(-45.2871795040912,-56.6754853983535,
0.));
#75267=CARTESIAN_POINT('Ctrl Pts',(-45.2871795040912,-56.6754853983535,
12.));
#75268=CARTESIAN_POINT('Ctrl Pts',(-45.2946828782557,-56.6993629437596,
0.));
#75269=CARTESIAN_POINT('Ctrl Pts',(-45.2946828782557,-56.6993629437596,
12.));
#75270=CARTESIAN_POINT('Ctrl Pts',(-45.3021754330169,-56.7232858667697,
0.));
#75271=CARTESIAN_POINT('Ctrl Pts',(-45.3021754330169,-56.7232858667697,
12.));
#75272=CARTESIAN_POINT('Ctrl Pts',(-45.3096570830107,-56.747254081454,0.));
#75273=CARTESIAN_POINT('Ctrl Pts',(-45.3096570830107,-56.747254081454,12.));
#75274=CARTESIAN_POINT('Ctrl Pts',(-45.3171277432592,-56.771267502148,0.));
#75275=CARTESIAN_POINT('Ctrl Pts',(-45.3171277432592,-56.771267502148,12.));
#75276=CARTESIAN_POINT('Ctrl Pts',(-45.3245873291682,-56.7953260434521,
0.));
#75277=CARTESIAN_POINT('Ctrl Pts',(-45.3245873291682,-56.7953260434521,
12.));
#75278=CARTESIAN_POINT('Ctrl Pts',(-45.3320357565241,-56.8194296202293,
0.));
#75279=CARTESIAN_POINT('Ctrl Pts',(-45.3320357565241,-56.8194296202293,
12.));
#75280=CARTESIAN_POINT('Ctrl Pts',(-45.3394729414932,-56.8435781475982,
0.));
#75281=CARTESIAN_POINT('Ctrl Pts',(-45.3394729414932,-56.8435781475982,
12.));
#75282=CARTESIAN_POINT('Ctrl Pts',(-45.3468988006202,-56.8677715409266,
0.));
#75283=CARTESIAN_POINT('Ctrl Pts',(-45.3468988006202,-56.8677715409266,
12.));
#75284=CARTESIAN_POINT('Ctrl Pts',(-45.3543132508234,-56.8920097158371,
0.));
#75285=CARTESIAN_POINT('Ctrl Pts',(-45.3543132508234,-56.8920097158371,
12.));
#75286=CARTESIAN_POINT('Ctrl Pts',(-45.3617162093918,-56.916292588208,0.));
#75287=CARTESIAN_POINT('Ctrl Pts',(-45.3617162093918,-56.916292588208,12.));
#75288=CARTESIAN_POINT('Ctrl Pts',(-45.3691075939827,-56.9406200741714,
0.));
#75289=CARTESIAN_POINT('Ctrl Pts',(-45.3691075939827,-56.9406200741714,
12.));
#75290=CARTESIAN_POINT('Ctrl Pts',(-45.3764873226202,-56.9649920901079,
0.));
#75291=CARTESIAN_POINT('Ctrl Pts',(-45.3764873226202,-56.9649920901079,
12.));
#75292=CARTESIAN_POINT('Ctrl Pts',(-45.3838553136957,-56.9894085526383,
0.));
#75293=CARTESIAN_POINT('Ctrl Pts',(-45.3838553136957,-56.9894085526383,
12.));
#75294=CARTESIAN_POINT('Ctrl Pts',(-45.3912114859625,-57.0138693786287,
0.));
#75295=CARTESIAN_POINT('Ctrl Pts',(-45.3912114859625,-57.0138693786287,
12.));
#75296=CARTESIAN_POINT('Ctrl Pts',(-45.3985557585316,-57.0383744851917,
0.));
#75297=CARTESIAN_POINT('Ctrl Pts',(-45.3985557585316,-57.0383744851917,
12.));
#75298=CARTESIAN_POINT('Ctrl Pts',(-45.4058880508693,-57.0629237896848,
0.));
#75299=CARTESIAN_POINT('Ctrl Pts',(-45.4058880508693,-57.0629237896848,
12.));
#75300=CARTESIAN_POINT('Ctrl Pts',(-45.4132082827945,-57.0875172097048,
0.));
#75301=CARTESIAN_POINT('Ctrl Pts',(-45.4132082827945,-57.0875172097048,
12.));
#75302=CARTESIAN_POINT('Ctrl Pts',(-45.4205163744778,-57.1121546630776,
0.));
#75303=CARTESIAN_POINT('Ctrl Pts',(-45.4205163744778,-57.1121546630776,
12.));
#75304=CARTESIAN_POINT('Ctrl Pts',(-45.4278122464387,-57.1368360678629,
0.));
#75305=CARTESIAN_POINT('Ctrl Pts',(-45.4278122464387,-57.1368360678629,
12.));
#75306=CARTESIAN_POINT('Ctrl Pts',(-45.4350958195434,-57.1615613423586,
0.));
#75307=CARTESIAN_POINT('Ctrl Pts',(-45.4350958195434,-57.1615613423586,
12.));
#75308=CARTESIAN_POINT('Ctrl Pts',(-45.4423670150035,-57.1863304051011,
0.));
#75309=CARTESIAN_POINT('Ctrl Pts',(-45.4423670150035,-57.1863304051011,
12.));
#75310=CARTESIAN_POINT('Ctrl Pts',(-45.4496257543759,-57.2111431748629,
0.));
#75311=CARTESIAN_POINT('Ctrl Pts',(-45.4496257543759,-57.2111431748629,
12.));
#75312=CARTESIAN_POINT('Ctrl Pts',(-45.4568719595639,-57.2359995706441,
0.));
#75313=CARTESIAN_POINT('Ctrl Pts',(-45.4568719595639,-57.2359995706441,
12.));
#75314=CARTESIAN_POINT('Ctrl Pts',(-45.4641055528138,-57.2608995116727,
0.));
#75315=CARTESIAN_POINT('Ctrl Pts',(-45.4641055528138,-57.2608995116727,
12.));
#75316=CARTESIAN_POINT('Ctrl Pts',(-45.4713264567059,-57.2858429174056,
0.));
#75317=CARTESIAN_POINT('Ctrl Pts',(-45.4713264567059,-57.2858429174056,
12.));
#75318=CARTESIAN_POINT('Ctrl Pts',(-45.4785345941505,-57.3108297075262,
0.));
#75319=CARTESIAN_POINT('Ctrl Pts',(-45.4785345941505,-57.3108297075262,
12.));
#75320=CARTESIAN_POINT('Ctrl Pts',(-45.4857298883826,-57.3358598019391,
0.));
#75321=CARTESIAN_POINT('Ctrl Pts',(-45.4857298883826,-57.3358598019391,
12.));
#75322=CARTESIAN_POINT('Ctrl Pts',(-45.4929122629576,-57.360933120758,0.));
#75323=CARTESIAN_POINT('Ctrl Pts',(-45.4929122629576,-57.360933120758,12.));
#75324=CARTESIAN_POINT('Ctrl Pts',(-45.5000816417516,-57.3860495843043,
0.));
#75325=CARTESIAN_POINT('Ctrl Pts',(-45.5000816417516,-57.3860495843043,
12.));
#75326=CARTESIAN_POINT('Ctrl Pts',(-45.5072379489637,-57.4112091131193,
0.));
#75327=CARTESIAN_POINT('Ctrl Pts',(-45.5072379489637,-57.4112091131193,
12.));
#75328=CARTESIAN_POINT('Ctrl Pts',(-45.5143811091209,-57.4364116279708,
0.));
#75329=CARTESIAN_POINT('Ctrl Pts',(-45.5143811091209,-57.4364116279708,
12.));
#75330=CARTESIAN_POINT('Ctrl Pts',(-45.5215110470825,-57.4616570498566,
0.));
#75331=CARTESIAN_POINT('Ctrl Pts',(-45.5215110470825,-57.4616570498566,
12.));
#75332=CARTESIAN_POINT('Ctrl Pts',(-45.5286276880479,-57.4869453000055,
0.));
#75333=CARTESIAN_POINT('Ctrl Pts',(-45.5286276880479,-57.4869453000055,
12.));
#75334=CARTESIAN_POINT('Ctrl Pts',(-45.5357309575603,-57.5122762998732,
0.));
#75335=CARTESIAN_POINT('Ctrl Pts',(-45.5357309575603,-57.5122762998732,
12.));
#75336=CARTESIAN_POINT('Ctrl Pts',(-45.5428207814832,-57.5376499711338,
0.));
#75337=CARTESIAN_POINT('Ctrl Pts',(-45.5428207814832,-57.5376499711338,
12.));
#75338=CARTESIAN_POINT('Ctrl Pts',(-45.5498970859829,-57.5630662356671,
0.));
#75339=CARTESIAN_POINT('Ctrl Pts',(-45.5498970859829,-57.5630662356671,
12.));
#75340=CARTESIAN_POINT('Ctrl Pts',(-45.5569597975096,-57.5885250155432,
0.));
#75341=CARTESIAN_POINT('Ctrl Pts',(-45.5569597975096,-57.5885250155432,
12.));
#75342=CARTESIAN_POINT('Ctrl Pts',(-45.5640088427819,-57.6140262330048,
0.));
#75343=CARTESIAN_POINT('Ctrl Pts',(-45.5640088427819,-57.6140262330048,
12.));
#75344=CARTESIAN_POINT('Ctrl Pts',(-45.5710441487683,-57.6395698104416,
0.));
#75345=CARTESIAN_POINT('Ctrl Pts',(-45.5710441487683,-57.6395698104416,
12.));
#75346=CARTESIAN_POINT('Ctrl Pts',(-45.5780656427172,-57.6651556704249,
0.));
#75347=CARTESIAN_POINT('Ctrl Pts',(-45.5780656427172,-57.6651556704249,
12.));
#75348=CARTESIAN_POINT('Ctrl Pts',(-45.5850732521902,-57.6907837357425,
0.));
#75349=CARTESIAN_POINT('Ctrl Pts',(-45.5850732521902,-57.6907837357425,
12.));
#75350=CARTESIAN_POINT('Ctrl Pts',(-45.5920669050988,-57.7164539294316,
0.));
#75351=CARTESIAN_POINT('Ctrl Pts',(-45.5920669050988,-57.7164539294316,
12.));
#75352=CARTESIAN_POINT('Ctrl Pts',(-45.5990465297341,-57.7421661748022,
0.));
#75353=CARTESIAN_POINT('Ctrl Pts',(-45.5990465297341,-57.7421661748022,
12.));
#75354=CARTESIAN_POINT('Ctrl Pts',(-45.6060120548199,-57.7679203954735,
0.));
#75355=CARTESIAN_POINT('Ctrl Pts',(-45.6060120548199,-57.7679203954735,
12.));
#75356=CARTESIAN_POINT('Ctrl Pts',(-45.6129634094677,-57.7937165153379,
0.));
#75357=CARTESIAN_POINT('Ctrl Pts',(-45.6129634094677,-57.7937165153379,
12.));
#75358=CARTESIAN_POINT('Ctrl Pts',(-45.619900523078,-57.819554458484,0.));
#75359=CARTESIAN_POINT('Ctrl Pts',(-45.619900523078,-57.819554458484,12.));
#75360=CARTESIAN_POINT('Ctrl Pts',(-45.6268233252543,-57.8454341491236,
0.));
#75361=CARTESIAN_POINT('Ctrl Pts',(-45.6268233252543,-57.8454341491236,
12.));
#75362=CARTESIAN_POINT('Ctrl Pts',(-45.6337317457253,-57.8713555115232,
0.));
#75363=CARTESIAN_POINT('Ctrl Pts',(-45.6337317457253,-57.8713555115232,
12.));
#75364=CARTESIAN_POINT('Ctrl Pts',(-45.6406257142385,-57.8973184699037,
0.));
#75365=CARTESIAN_POINT('Ctrl Pts',(-45.6406257142385,-57.8973184699037,
12.));
#75366=CARTESIAN_POINT('Ctrl Pts',(-45.6475051605542,-57.923322948432,0.));
#75367=CARTESIAN_POINT('Ctrl Pts',(-45.6475051605542,-57.923322948432,12.));
#75368=CARTESIAN_POINT('Ctrl Pts',(-45.6543700146689,-57.9493688714249,
0.));
#75369=CARTESIAN_POINT('Ctrl Pts',(-45.6543700146689,-57.9493688714249,
12.));
#75370=CARTESIAN_POINT('Ctrl Pts',(-45.6612202069927,-57.975456163507,0.));
#75371=CARTESIAN_POINT('Ctrl Pts',(-45.6612202069927,-57.975456163507,12.));
#75372=CARTESIAN_POINT('Ctrl Pts',(-45.6680556685494,-58.0015847497838,
0.));
#75373=CARTESIAN_POINT('Ctrl Pts',(-45.6680556685494,-58.0015847497838,
12.));
#75374=CARTESIAN_POINT('Ctrl Pts',(-45.6748763311635,-58.0277545560001,
0.));
#75375=CARTESIAN_POINT('Ctrl Pts',(-45.6748763311635,-58.0277545560001,
12.));
#75376=CARTESIAN_POINT('Ctrl Pts',(-45.6816821276662,-58.0539655087095,
0.));
#75377=CARTESIAN_POINT('Ctrl Pts',(-45.6816821276662,-58.0539655087095,
12.));
#75378=CARTESIAN_POINT('Ctrl Pts',(-45.6884729914465,-58.0802175348939,
0.));
#75379=CARTESIAN_POINT('Ctrl Pts',(-45.6884729914465,-58.0802175348939,
12.));
#75380=CARTESIAN_POINT('Ctrl Pts',(-45.6952488560133,-58.1065105615884,
0.));
#75381=CARTESIAN_POINT('Ctrl Pts',(-45.6952488560133,-58.1065105615884,
12.));
#75382=CARTESIAN_POINT('Ctrl Pts',(-45.7020096545174,-58.1328445154667,
0.));
#75383=CARTESIAN_POINT('Ctrl Pts',(-45.7020096545174,-58.1328445154667,
12.));
#75384=CARTESIAN_POINT('Ctrl Pts',(-45.708755319378,-58.159219322515,0.));
#75385=CARTESIAN_POINT('Ctrl Pts',(-45.708755319378,-58.159219322515,12.));
#75386=CARTESIAN_POINT('Ctrl Pts',(-45.7154857816507,-58.1856349074723,
0.));
#75387=CARTESIAN_POINT('Ctrl Pts',(-45.7154857816507,-58.1856349074723,
12.));
#75388=CARTESIAN_POINT('Ctrl Pts',(-45.7222009715431,-58.2120911942819,
0.));
#75389=CARTESIAN_POINT('Ctrl Pts',(-45.7222009715431,-58.2120911942819,
12.));
#75390=CARTESIAN_POINT('Ctrl Pts',(-45.7289008195612,-58.2385881070959,
0.));
#75391=CARTESIAN_POINT('Ctrl Pts',(-45.7289008195612,-58.2385881070959,
12.));
#75392=CARTESIAN_POINT('Ctrl Pts',(-45.7355852575127,-58.2651255711481,
0.));
#75393=CARTESIAN_POINT('Ctrl Pts',(-45.7355852575127,-58.2651255711481,
12.));
#75394=CARTESIAN_POINT('Ctrl Pts',(-45.7422542194625,-58.2917035135833,
0.));
#75395=CARTESIAN_POINT('Ctrl Pts',(-45.7422542194625,-58.2917035135833,
12.));
#75396=CARTESIAN_POINT('Ctrl Pts',(-45.7489076429725,-58.3183218645265,
0.));
#75397=CARTESIAN_POINT('Ctrl Pts',(-45.7489076429725,-58.3183218645265,
12.));
#75398=CARTESIAN_POINT('Ctrl Pts',(-45.7555454693956,-58.3449805573335,
0.));
#75399=CARTESIAN_POINT('Ctrl Pts',(-45.7555454693956,-58.3449805573335,
12.));
#75400=CARTESIAN_POINT('Ctrl Pts',(-45.762167641136,-58.3716795262251,0.));
#75401=CARTESIAN_POINT('Ctrl Pts',(-45.762167641136,-58.3716795262251,12.));
#75402=CARTESIAN_POINT('Ctrl Pts',(-45.7687740994899,-58.3984187044166,
0.));
#75403=CARTESIAN_POINT('Ctrl Pts',(-45.7687740994899,-58.3984187044166,
12.));
#75404=CARTESIAN_POINT('Ctrl Pts',(-45.77536478215,-58.4251980219532,0.));
#75405=CARTESIAN_POINT('Ctrl Pts',(-45.77536478215,-58.4251980219532,12.));
#75406=CARTESIAN_POINT('Ctrl Pts',(-45.7819396211062,-58.4520174038836,
0.));
#75407=CARTESIAN_POINT('Ctrl Pts',(-45.7819396211062,-58.4520174038836,
12.));
#75408=CARTESIAN_POINT('Ctrl Pts',(-45.7884985397138,-58.4788767677114,
0.));
#75409=CARTESIAN_POINT('Ctrl Pts',(-45.7884985397138,-58.4788767677114,
12.));
#75410=CARTESIAN_POINT('Ctrl Pts',(-45.7950414569431,-58.5057760270407,
0.));
#75411=CARTESIAN_POINT('Ctrl Pts',(-45.7950414569431,-58.5057760270407,
12.));
#75412=CARTESIAN_POINT('Ctrl Pts',(-45.801568292618,-58.5327150960874,0.));
#75413=CARTESIAN_POINT('Ctrl Pts',(-45.801568292618,-58.5327150960874,12.));
#75414=CARTESIAN_POINT('Ctrl Pts',(-45.8080789725167,-58.5596938940308,
0.));
#75415=CARTESIAN_POINT('Ctrl Pts',(-45.8080789725167,-58.5596938940308,
12.));
#75416=CARTESIAN_POINT('Ctrl Pts',(-45.8145734330666,-58.5867123490943,
0.));
#75417=CARTESIAN_POINT('Ctrl Pts',(-45.8145734330666,-58.5867123490943,
12.));
#75418=CARTESIAN_POINT('Ctrl Pts',(-45.8210516273556,-58.6137704035561,
0.));
#75419=CARTESIAN_POINT('Ctrl Pts',(-45.8210516273556,-58.6137704035561,
12.));
#75420=CARTESIAN_POINT('Ctrl Pts',(-45.8275135263874,-58.64086801535,0.));
#75421=CARTESIAN_POINT('Ctrl Pts',(-45.8275135263874,-58.64086801535,12.));
#75422=CARTESIAN_POINT('Ctrl Pts',(-45.8339591141396,-58.668005155216,0.));
#75423=CARTESIAN_POINT('Ctrl Pts',(-45.8339591141396,-58.668005155216,12.));
#75424=CARTESIAN_POINT('Ctrl Pts',(-45.8391025301766,-58.6897464750196,
0.));
#75425=CARTESIAN_POINT('Ctrl Pts',(-45.8391025301766,-58.6897464750196,
12.));
#75426=CARTESIAN_POINT('Ctrl Pts',(-45.8429527488565,-58.7060702401382,
0.));
#75427=CARTESIAN_POINT('Ctrl Pts',(-45.8429527488565,-58.7060702401382,
12.));
#75428=CARTESIAN_POINT('Ctrl Pts',(-45.8455162977347,-58.7169606500157,
0.));
#75429=CARTESIAN_POINT('Ctrl Pts',(-45.8455162977347,-58.7169606500157,
12.));
#75430=CARTESIAN_POINT('Ctrl Pts',(-45.8467972562798,-58.722407829904,0.));
#75431=CARTESIAN_POINT('Ctrl Pts',(-45.8467972562798,-58.722407829904,12.));
#75432=CARTESIAN_POINT('',(-44.3377168516418,-54.1679505278134,0.));
#75433=CARTESIAN_POINT('Ctrl Pts',(-44.3377168516418,-54.1679505278134,
0.));
#75434=CARTESIAN_POINT('Ctrl Pts',(-44.3393235891014,-54.1714861895278,
0.));
#75435=CARTESIAN_POINT('Ctrl Pts',(-44.3425373700829,-54.1785633257456,
0.));
#75436=CARTESIAN_POINT('Ctrl Pts',(-44.3473589597468,-54.1891964684439,
0.));
#75437=CARTESIAN_POINT('Ctrl Pts',(-44.3537895823819,-54.203408870162,0.));
#75438=CARTESIAN_POINT('Ctrl Pts',(-44.3618309103245,-54.2212325005847,
0.));
#75439=CARTESIAN_POINT('Ctrl Pts',(-44.369875253351,-54.2391142386354,0.));
#75440=CARTESIAN_POINT('Ctrl Pts',(-44.3779225430461,-54.2570540336536,
0.));
#75441=CARTESIAN_POINT('Ctrl Pts',(-44.3859726620288,-54.2750517888695,
0.));
#75442=CARTESIAN_POINT('Ctrl Pts',(-44.3940254456427,-54.2931073621661,
0.));
#75443=CARTESIAN_POINT('Ctrl Pts',(-44.4020807028144,-54.3112205860776,
0.));
#75444=CARTESIAN_POINT('Ctrl Pts',(-44.4101382321834,-54.3293912830237,
0.));
#75445=CARTESIAN_POINT('Ctrl Pts',(-44.4181978395814,-54.347619281931,0.));
#75446=CARTESIAN_POINT('Ctrl Pts',(-44.4262593564664,-54.3659044357064,
0.));
#75447=CARTESIAN_POINT('Ctrl Pts',(-44.4343226339555,-54.3842466156151,
0.));
#75448=CARTESIAN_POINT('Ctrl Pts',(-44.442387534098,-54.4026457030316,0.));
#75449=CARTESIAN_POINT('Ctrl Pts',(-44.4504539226336,-54.4211015825959,
0.));
#75450=CARTESIAN_POINT('Ctrl Pts',(-44.4585216599933,-54.4396141337008,
0.));
#75451=CARTESIAN_POINT('Ctrl Pts',(-44.4665905967701,-54.4581832262072,
0.));
#75452=CARTESIAN_POINT('Ctrl Pts',(-44.4746605784056,-54.4768087248854,
0.));
#75453=CARTESIAN_POINT('Ctrl Pts',(-44.482731448127,-54.4954904921938,0.));
#75454=CARTESIAN_POINT('Ctrl Pts',(-44.4908030503209,-54.5142283914684,
0.));
#75455=CARTESIAN_POINT('Ctrl Pts',(-44.4988752343715,-54.5330222905438,
0.));
#75456=CARTESIAN_POINT('Ctrl Pts',(-44.5069478544945,-54.5518720616016,
0.));
#75457=CARTESIAN_POINT('Ctrl Pts',(-44.5150207678988,-54.5707775794412,
0.));
#75458=CARTESIAN_POINT('Ctrl Pts',(-44.5230938335167,-54.5897387202815,
0.));
#75459=CARTESIAN_POINT('Ctrl Pts',(-44.5311669104515,-54.6087553602914,
0.));
#75460=CARTESIAN_POINT('Ctrl Pts',(-44.5392398566802,-54.6278273743587,
0.));
#75461=CARTESIAN_POINT('Ctrl Pts',(-44.5473125297311,-54.6469546367408,
0.));
#75462=CARTESIAN_POINT('Ctrl Pts',(-44.5553847872721,-54.6661370216252,
0.));
#75463=CARTESIAN_POINT('Ctrl Pts',(-44.5634564876863,-54.6853744036751,
0.));
#75464=CARTESIAN_POINT('Ctrl Pts',(-44.5715274907619,-54.7046666586754,
0.));
#75465=CARTESIAN_POINT('Ctrl Pts',(-44.5795976579454,-54.7240136637717,
0.));
#75466=CARTESIAN_POINT('Ctrl Pts',(-44.5876668519661,-54.7434152971267,
0.));
#75467=CARTESIAN_POINT('Ctrl Pts',(-44.5957349366059,-54.7628714377037,
0.));
#75468=CARTESIAN_POINT('Ctrl Pts',(-44.6038017764309,-54.7823819650149,
0.));
#75469=CARTESIAN_POINT('Ctrl Pts',(-44.6118672364906,-54.8019467588278,
0.));
#75470=CARTESIAN_POINT('Ctrl Pts',(-44.6199311823293,-54.8215656991837,
0.));
#75471=CARTESIAN_POINT('Ctrl Pts',(-44.6279934801169,-54.8412386665276,
0.));
#75472=CARTESIAN_POINT('Ctrl Pts',(-44.6360539967392,-54.860965541796,0.));
#75473=CARTESIAN_POINT('Ctrl Pts',(-44.6441125999063,-54.8807462065164,
0.));
#75474=CARTESIAN_POINT('Ctrl Pts',(-44.6521691582533,-54.9005805428969,
0.));
#75475=CARTESIAN_POINT('Ctrl Pts',(-44.6602235412836,-54.9204684337822,
0.));
#75476=CARTESIAN_POINT('Ctrl Pts',(-44.6682756193147,-54.9404097626077,
0.));
#75477=CARTESIAN_POINT('Ctrl Pts',(-44.6763252634258,-54.9604044133501,
0.));
#75478=CARTESIAN_POINT('Ctrl Pts',(-44.6843723454,-54.9804522704686,0.));
#75479=CARTESIAN_POINT('Ctrl Pts',(-44.6924167376869,-55.0005532188667,
0.));
#75480=CARTESIAN_POINT('Ctrl Pts',(-44.7004583134249,-55.0207071439237,
0.));
#75481=CARTESIAN_POINT('Ctrl Pts',(-44.7084969464513,-55.0409139315078,
0.));
#75482=CARTESIAN_POINT('Ctrl Pts',(-44.7165325113159,-55.0611734679894,
0.));
#75483=CARTESIAN_POINT('Ctrl Pts',(-44.7245648832979,-55.0814856402496,
0.));
#75484=CARTESIAN_POINT('Ctrl Pts',(-44.7325939384035,-55.1018503356796,
0.));
#75485=CARTESIAN_POINT('Ctrl Pts',(-44.740619553348,-55.1222674421743,0.));
#75486=CARTESIAN_POINT('Ctrl Pts',(-44.748641605542,-55.14273684812,0.));
#75487=CARTESIAN_POINT('Ctrl Pts',(-44.7566599730773,-55.1632584423815,
0.));
#75488=CARTESIAN_POINT('Ctrl Pts',(-44.7646745347109,-55.1838321142779,
0.));
#75489=CARTESIAN_POINT('Ctrl Pts',(-44.7726851698619,-55.2044577535866,
0.));
#75490=CARTESIAN_POINT('Ctrl Pts',(-44.7806917586077,-55.2251352505475,
0.));
#75491=CARTESIAN_POINT('Ctrl Pts',(-44.7886941816823,-55.2458644958617,
0.));
#75492=CARTESIAN_POINT('Ctrl Pts',(-44.7966923204741,-55.2666453806883,
0.));
#75493=CARTESIAN_POINT('Ctrl Pts',(-44.8046860570245,-55.287477796635,0.));
#75494=CARTESIAN_POINT('Ctrl Pts',(-44.812675274021,-55.3083616357605,0.));
#75495=CARTESIAN_POINT('Ctrl Pts',(-44.8206598547889,-55.3292967905726,
0.));
#75496=CARTESIAN_POINT('Ctrl Pts',(-44.8286396832849,-55.350283154023,0.));
#75497=CARTESIAN_POINT('Ctrl Pts',(-44.8366146440896,-55.3713206194962,
0.));
#75498=CARTESIAN_POINT('Ctrl Pts',(-44.8445846224034,-55.3924090808002,
0.));
#75499=CARTESIAN_POINT('Ctrl Pts',(-44.8525495040397,-55.4135484321706,
0.));
#75500=CARTESIAN_POINT('Ctrl Pts',(-44.8605091754208,-55.4347385682697,
0.));
#75501=CARTESIAN_POINT('Ctrl Pts',(-44.8684635235727,-55.4559793841838,
0.));
#75502=CARTESIAN_POINT('Ctrl Pts',(-44.8764124361218,-55.4772707754139,
0.));
#75503=CARTESIAN_POINT('Ctrl Pts',(-44.8843558012903,-55.4986126378676,
0.));
#75504=CARTESIAN_POINT('Ctrl Pts',(-44.8922935078905,-55.5200048678648,
0.));
#75505=CARTESIAN_POINT('Ctrl Pts',(-44.9002254453192,-55.541447362135,0.));
#75506=CARTESIAN_POINT('Ctrl Pts',(-44.9081515035525,-55.5629400178136,
0.));
#75507=CARTESIAN_POINT('Ctrl Pts',(-44.9160715731425,-55.5844827324315,
0.));
#75508=CARTESIAN_POINT('Ctrl Pts',(-44.9239855452119,-55.6060754039089,
0.));
#75509=CARTESIAN_POINT('Ctrl Pts',(-44.9318933114483,-55.6277179305604,
0.));
#75510=CARTESIAN_POINT('Ctrl Pts',(-44.9397947640996,-55.6494102110922,
0.));
#75511=CARTESIAN_POINT('Ctrl Pts',(-44.9476897959694,-55.671152144599,0.));
#75512=CARTESIAN_POINT('Ctrl Pts',(-44.9555783004133,-55.6929436305522,
0.));
#75513=CARTESIAN_POINT('Ctrl Pts',(-44.9634601713352,-55.7147845687969,
0.));
#75514=CARTESIAN_POINT('Ctrl Pts',(-44.9713353031827,-55.7366748595582,
0.));
#75515=CARTESIAN_POINT('Ctrl Pts',(-44.979203590942,-55.7586144034376,0.));
#75516=CARTESIAN_POINT('Ctrl Pts',(-44.9870649301333,-55.7806031014093,
0.));
#75517=CARTESIAN_POINT('Ctrl Pts',(-44.9949192168073,-55.8026408548078,
0.));
#75518=CARTESIAN_POINT('Ctrl Pts',(-45.002766347541,-55.8247275653257,0.));
#75519=CARTESIAN_POINT('Ctrl Pts',(-45.0106062194325,-55.8468631350195,
0.));
#75520=CARTESIAN_POINT('Ctrl Pts',(-45.0184387300968,-55.8690474663058,
0.));
#75521=CARTESIAN_POINT('Ctrl Pts',(-45.0262637776623,-55.8912804619588,
0.));
#75522=CARTESIAN_POINT('Ctrl Pts',(-45.0340812607676,-55.9135620250977,
0.));
#75523=CARTESIAN_POINT('Ctrl Pts',(-45.041891078557,-55.9358920591861,0.));
#75524=CARTESIAN_POINT('Ctrl Pts',(-45.0496931306766,-55.958270468037,0.));
#75525=CARTESIAN_POINT('Ctrl Pts',(-45.0574873172696,-55.9806971558099,
0.));
#75526=CARTESIAN_POINT('Ctrl Pts',(-45.0652735389729,-56.0031720270074,
0.));
#75527=CARTESIAN_POINT('Ctrl Pts',(-45.0730516969142,-56.025694986463,0.));
#75528=CARTESIAN_POINT('Ctrl Pts',(-45.0808216927082,-56.0482659393412,
0.));
#75529=CARTESIAN_POINT('Ctrl Pts',(-45.0885834284513,-56.070884791141,0.));
#75530=CARTESIAN_POINT('Ctrl Pts',(-45.0963368067177,-56.0935514476945,
0.));
#75531=CARTESIAN_POINT('Ctrl Pts',(-45.1040817305563,-56.1162658151621,
0.));
#75532=CARTESIAN_POINT('Ctrl Pts',(-45.1118181034888,-56.1390278000226,
0.));
#75533=CARTESIAN_POINT('Ctrl Pts',(-45.119545829506,-56.1618373090729,0.));
#75534=CARTESIAN_POINT('Ctrl Pts',(-45.1272648130627,-56.1846942494321,
0.));
#75535=CARTESIAN_POINT('Ctrl Pts',(-45.1349749590736,-56.2075985285391,
0.));
#75536=CARTESIAN_POINT('Ctrl Pts',(-45.1426761729107,-56.2305500541491,
0.));
#75537=CARTESIAN_POINT('Ctrl Pts',(-45.150368360401,-56.2535487343227,0.));
#75538=CARTESIAN_POINT('Ctrl Pts',(-45.158051427823,-56.2765944774252,0.));
#75539=CARTESIAN_POINT('Ctrl Pts',(-45.1657252819018,-56.2996871921321,
0.));
#75540=CARTESIAN_POINT('Ctrl Pts',(-45.1733898298062,-56.3228267874265,
0.));
#75541=CARTESIAN_POINT('Ctrl Pts',(-45.1810449791451,-56.3460131725962,
0.));
#75542=CARTESIAN_POINT('Ctrl Pts',(-45.1886906379664,-56.3692462572228,
0.));
#75543=CARTESIAN_POINT('Ctrl Pts',(-45.1963267147527,-56.3925259511804,
0.));
#75544=CARTESIAN_POINT('Ctrl Pts',(-45.2039531184172,-56.4158521646412,
0.));
#75545=CARTESIAN_POINT('Ctrl Pts',(-45.2115697583002,-56.4392248080733,
0.));
#75546=CARTESIAN_POINT('Ctrl Pts',(-45.2191765441666,-56.4626437922385,
0.));
#75547=CARTESIAN_POINT('Ctrl Pts',(-45.2267733862046,-56.4861090281819,
0.));
#75548=CARTESIAN_POINT('Ctrl Pts',(-45.2343601950222,-56.5096204272299,
0.));
#75549=CARTESIAN_POINT('Ctrl Pts',(-45.2419368816423,-56.533177900995,0.));
#75550=CARTESIAN_POINT('Ctrl Pts',(-45.2495033574997,-56.5567813613752,
0.));
#75551=CARTESIAN_POINT('Ctrl Pts',(-45.2570595344382,-56.5804307205507,
0.));
#75552=CARTESIAN_POINT('Ctrl Pts',(-45.2646053247094,-56.604125890975,0.));
#75553=CARTESIAN_POINT('Ctrl Pts',(-45.2721406409706,-56.6278667853716,
0.));
#75554=CARTESIAN_POINT('Ctrl Pts',(-45.2796653962796,-56.6516533167398,
0.));
#75555=CARTESIAN_POINT('Ctrl Pts',(-45.2871795040912,-56.6754853983535,
0.));
#75556=CARTESIAN_POINT('Ctrl Pts',(-45.2946828782557,-56.6993629437596,
0.));
#75557=CARTESIAN_POINT('Ctrl Pts',(-45.3021754330169,-56.7232858667697,
0.));
#75558=CARTESIAN_POINT('Ctrl Pts',(-45.3096570830107,-56.747254081454,0.));
#75559=CARTESIAN_POINT('Ctrl Pts',(-45.3171277432592,-56.771267502148,0.));
#75560=CARTESIAN_POINT('Ctrl Pts',(-45.3245873291682,-56.7953260434521,
0.));
#75561=CARTESIAN_POINT('Ctrl Pts',(-45.3320357565241,-56.8194296202293,
0.));
#75562=CARTESIAN_POINT('Ctrl Pts',(-45.3394729414932,-56.8435781475982,
0.));
#75563=CARTESIAN_POINT('Ctrl Pts',(-45.3468988006202,-56.8677715409266,
0.));
#75564=CARTESIAN_POINT('Ctrl Pts',(-45.3543132508234,-56.8920097158371,
0.));
#75565=CARTESIAN_POINT('Ctrl Pts',(-45.3617162093918,-56.916292588208,0.));
#75566=CARTESIAN_POINT('Ctrl Pts',(-45.3691075939827,-56.9406200741714,
0.));
#75567=CARTESIAN_POINT('Ctrl Pts',(-45.3764873226202,-56.9649920901079,
0.));
#75568=CARTESIAN_POINT('Ctrl Pts',(-45.3838553136957,-56.9894085526383,
0.));
#75569=CARTESIAN_POINT('Ctrl Pts',(-45.3912114859625,-57.0138693786287,
0.));
#75570=CARTESIAN_POINT('Ctrl Pts',(-45.3985557585316,-57.0383744851917,
0.));
#75571=CARTESIAN_POINT('Ctrl Pts',(-45.4058880508693,-57.0629237896848,
0.));
#75572=CARTESIAN_POINT('Ctrl Pts',(-45.4132082827945,-57.0875172097048,
0.));
#75573=CARTESIAN_POINT('Ctrl Pts',(-45.4205163744778,-57.1121546630776,
0.));
#75574=CARTESIAN_POINT('Ctrl Pts',(-45.4278122464387,-57.1368360678629,
0.));
#75575=CARTESIAN_POINT('Ctrl Pts',(-45.4350958195434,-57.1615613423586,
0.));
#75576=CARTESIAN_POINT('Ctrl Pts',(-45.4423670150035,-57.1863304051011,
0.));
#75577=CARTESIAN_POINT('Ctrl Pts',(-45.4496257543759,-57.2111431748629,
0.));
#75578=CARTESIAN_POINT('Ctrl Pts',(-45.4568719595639,-57.2359995706441,
0.));
#75579=CARTESIAN_POINT('Ctrl Pts',(-45.4641055528138,-57.2608995116727,
0.));
#75580=CARTESIAN_POINT('Ctrl Pts',(-45.4713264567059,-57.2858429174056,
0.));
#75581=CARTESIAN_POINT('Ctrl Pts',(-45.4785345941505,-57.3108297075262,
0.));
#75582=CARTESIAN_POINT('Ctrl Pts',(-45.4857298883826,-57.3358598019391,
0.));
#75583=CARTESIAN_POINT('Ctrl Pts',(-45.4929122629576,-57.360933120758,0.));
#75584=CARTESIAN_POINT('Ctrl Pts',(-45.5000816417516,-57.3860495843043,
0.));
#75585=CARTESIAN_POINT('Ctrl Pts',(-45.5072379489637,-57.4112091131193,
0.));
#75586=CARTESIAN_POINT('Ctrl Pts',(-45.5143811091209,-57.4364116279708,
0.));
#75587=CARTESIAN_POINT('Ctrl Pts',(-45.5215110470825,-57.4616570498566,
0.));
#75588=CARTESIAN_POINT('Ctrl Pts',(-45.5286276880479,-57.4869453000055,
0.));
#75589=CARTESIAN_POINT('Ctrl Pts',(-45.5357309575603,-57.5122762998732,
0.));
#75590=CARTESIAN_POINT('Ctrl Pts',(-45.5428207814832,-57.5376499711338,
0.));
#75591=CARTESIAN_POINT('Ctrl Pts',(-45.5498970859829,-57.5630662356671,
0.));
#75592=CARTESIAN_POINT('Ctrl Pts',(-45.5569597975096,-57.5885250155432,
0.));
#75593=CARTESIAN_POINT('Ctrl Pts',(-45.5640088427819,-57.6140262330048,
0.));
#75594=CARTESIAN_POINT('Ctrl Pts',(-45.5710441487683,-57.6395698104416,
0.));
#75595=CARTESIAN_POINT('Ctrl Pts',(-45.5780656427172,-57.6651556704249,
0.));
#75596=CARTESIAN_POINT('Ctrl Pts',(-45.5850732521902,-57.6907837357425,
0.));
#75597=CARTESIAN_POINT('Ctrl Pts',(-45.5920669050988,-57.7164539294316,
0.));
#75598=CARTESIAN_POINT('Ctrl Pts',(-45.5990465297341,-57.7421661748022,
0.));
#75599=CARTESIAN_POINT('Ctrl Pts',(-45.6060120548199,-57.7679203954735,
0.));
#75600=CARTESIAN_POINT('Ctrl Pts',(-45.6129634094677,-57.7937165153379,
0.));
#75601=CARTESIAN_POINT('Ctrl Pts',(-45.619900523078,-57.819554458484,0.));
#75602=CARTESIAN_POINT('Ctrl Pts',(-45.6268233252543,-57.8454341491236,
0.));
#75603=CARTESIAN_POINT('Ctrl Pts',(-45.6337317457253,-57.8713555115232,
0.));
#75604=CARTESIAN_POINT('Ctrl Pts',(-45.6406257142385,-57.8973184699037,
0.));
#75605=CARTESIAN_POINT('Ctrl Pts',(-45.6475051605542,-57.923322948432,0.));
#75606=CARTESIAN_POINT('Ctrl Pts',(-45.6543700146689,-57.9493688714249,
0.));
#75607=CARTESIAN_POINT('Ctrl Pts',(-45.6612202069927,-57.975456163507,0.));
#75608=CARTESIAN_POINT('Ctrl Pts',(-45.6680556685494,-58.0015847497838,
0.));
#75609=CARTESIAN_POINT('Ctrl Pts',(-45.6748763311635,-58.0277545560001,
0.));
#75610=CARTESIAN_POINT('Ctrl Pts',(-45.6816821276662,-58.0539655087095,
0.));
#75611=CARTESIAN_POINT('Ctrl Pts',(-45.6884729914465,-58.0802175348939,
0.));
#75612=CARTESIAN_POINT('Ctrl Pts',(-45.6952488560133,-58.1065105615884,
0.));
#75613=CARTESIAN_POINT('Ctrl Pts',(-45.7020096545174,-58.1328445154667,
0.));
#75614=CARTESIAN_POINT('Ctrl Pts',(-45.708755319378,-58.159219322515,0.));
#75615=CARTESIAN_POINT('Ctrl Pts',(-45.7154857816507,-58.1856349074723,
0.));
#75616=CARTESIAN_POINT('Ctrl Pts',(-45.7222009715431,-58.2120911942819,
0.));
#75617=CARTESIAN_POINT('Ctrl Pts',(-45.7289008195612,-58.2385881070959,
0.));
#75618=CARTESIAN_POINT('Ctrl Pts',(-45.7355852575127,-58.2651255711481,
0.));
#75619=CARTESIAN_POINT('Ctrl Pts',(-45.7422542194625,-58.2917035135833,
0.));
#75620=CARTESIAN_POINT('Ctrl Pts',(-45.7489076429725,-58.3183218645265,
0.));
#75621=CARTESIAN_POINT('Ctrl Pts',(-45.7555454693956,-58.3449805573335,
0.));
#75622=CARTESIAN_POINT('Ctrl Pts',(-45.7612219538034,-58.3678667473266,
0.));
#75623=CARTESIAN_POINT('Ctrl Pts',(-45.7655655205267,-58.385434851721,0.));
#75624=CARTESIAN_POINT('Ctrl Pts',(-45.7685831165459,-58.3976670480781,
0.));
#75625=CARTESIAN_POINT('Ctrl Pts',(-45.7702793558063,-58.4045515723008,
0.));
#75626=CARTESIAN_POINT('Ctrl Pts',(-45.7706564944767,-58.4060826907379,
0.));
#75627=CARTESIAN_POINT('',(-44.3377168516418,-54.1679505278134,12.));
#75628=CARTESIAN_POINT('',(-44.3377168516418,-54.1679505278134,0.));
#75629=CARTESIAN_POINT('Ctrl Pts',(-45.7706564944767,-58.4060826907378,
12.));
#75630=CARTESIAN_POINT('Ctrl Pts',(-45.7702793558063,-58.4045515723008,
12.));
#75631=CARTESIAN_POINT('Ctrl Pts',(-45.7685831165459,-58.397667048078,12.));
#75632=CARTESIAN_POINT('Ctrl Pts',(-45.7655655205267,-58.385434851721,12.));
#75633=CARTESIAN_POINT('Ctrl Pts',(-45.7612219538034,-58.3678667473265,
12.));
#75634=CARTESIAN_POINT('Ctrl Pts',(-45.7555454693956,-58.3449805573335,
12.));
#75635=CARTESIAN_POINT('Ctrl Pts',(-45.7489076429725,-58.3183218645265,
12.));
#75636=CARTESIAN_POINT('Ctrl Pts',(-45.7422542194625,-58.2917035135833,
12.));
#75637=CARTESIAN_POINT('Ctrl Pts',(-45.7355852575127,-58.2651255711481,
12.));
#75638=CARTESIAN_POINT('Ctrl Pts',(-45.7289008195612,-58.2385881070959,
12.));
#75639=CARTESIAN_POINT('Ctrl Pts',(-45.7222009715431,-58.2120911942819,
12.));
#75640=CARTESIAN_POINT('Ctrl Pts',(-45.7154857816507,-58.1856349074723,
12.));
#75641=CARTESIAN_POINT('Ctrl Pts',(-45.708755319378,-58.159219322515,12.));
#75642=CARTESIAN_POINT('Ctrl Pts',(-45.7020096545174,-58.1328445154667,
12.));
#75643=CARTESIAN_POINT('Ctrl Pts',(-45.6952488560133,-58.1065105615884,
12.));
#75644=CARTESIAN_POINT('Ctrl Pts',(-45.6884729914465,-58.0802175348939,
12.));
#75645=CARTESIAN_POINT('Ctrl Pts',(-45.6816821276662,-58.0539655087095,
12.));
#75646=CARTESIAN_POINT('Ctrl Pts',(-45.6748763311635,-58.0277545560001,
12.));
#75647=CARTESIAN_POINT('Ctrl Pts',(-45.6680556685494,-58.0015847497838,
12.));
#75648=CARTESIAN_POINT('Ctrl Pts',(-45.6612202069927,-57.975456163507,12.));
#75649=CARTESIAN_POINT('Ctrl Pts',(-45.6543700146689,-57.9493688714249,
12.));
#75650=CARTESIAN_POINT('Ctrl Pts',(-45.6475051605542,-57.923322948432,12.));
#75651=CARTESIAN_POINT('Ctrl Pts',(-45.6406257142385,-57.8973184699037,
12.));
#75652=CARTESIAN_POINT('Ctrl Pts',(-45.6337317457253,-57.8713555115232,
12.));
#75653=CARTESIAN_POINT('Ctrl Pts',(-45.6268233252543,-57.8454341491236,
12.));
#75654=CARTESIAN_POINT('Ctrl Pts',(-45.619900523078,-57.819554458484,12.));
#75655=CARTESIAN_POINT('Ctrl Pts',(-45.6129634094677,-57.7937165153379,
12.));
#75656=CARTESIAN_POINT('Ctrl Pts',(-45.6060120548199,-57.7679203954735,
12.));
#75657=CARTESIAN_POINT('Ctrl Pts',(-45.5990465297341,-57.7421661748022,
12.));
#75658=CARTESIAN_POINT('Ctrl Pts',(-45.5920669050988,-57.7164539294316,
12.));
#75659=CARTESIAN_POINT('Ctrl Pts',(-45.5850732521902,-57.6907837357425,
12.));
#75660=CARTESIAN_POINT('Ctrl Pts',(-45.5780656427172,-57.6651556704249,
12.));
#75661=CARTESIAN_POINT('Ctrl Pts',(-45.5710441487683,-57.6395698104416,
12.));
#75662=CARTESIAN_POINT('Ctrl Pts',(-45.5640088427819,-57.6140262330048,
12.));
#75663=CARTESIAN_POINT('Ctrl Pts',(-45.5569597975096,-57.5885250155432,
12.));
#75664=CARTESIAN_POINT('Ctrl Pts',(-45.5498970859829,-57.5630662356671,
12.));
#75665=CARTESIAN_POINT('Ctrl Pts',(-45.5428207814832,-57.5376499711338,
12.));
#75666=CARTESIAN_POINT('Ctrl Pts',(-45.5357309575603,-57.5122762998732,
12.));
#75667=CARTESIAN_POINT('Ctrl Pts',(-45.5286276880479,-57.4869453000055,
12.));
#75668=CARTESIAN_POINT('Ctrl Pts',(-45.5215110470825,-57.4616570498566,
12.));
#75669=CARTESIAN_POINT('Ctrl Pts',(-45.5143811091209,-57.4364116279708,
12.));
#75670=CARTESIAN_POINT('Ctrl Pts',(-45.5072379489637,-57.4112091131193,
12.));
#75671=CARTESIAN_POINT('Ctrl Pts',(-45.5000816417516,-57.3860495843043,
12.));
#75672=CARTESIAN_POINT('Ctrl Pts',(-45.4929122629576,-57.360933120758,12.));
#75673=CARTESIAN_POINT('Ctrl Pts',(-45.4857298883826,-57.3358598019391,
12.));
#75674=CARTESIAN_POINT('Ctrl Pts',(-45.4785345941505,-57.3108297075262,
12.));
#75675=CARTESIAN_POINT('Ctrl Pts',(-45.4713264567059,-57.2858429174056,
12.));
#75676=CARTESIAN_POINT('Ctrl Pts',(-45.4641055528138,-57.2608995116727,
12.));
#75677=CARTESIAN_POINT('Ctrl Pts',(-45.4568719595639,-57.2359995706441,
12.));
#75678=CARTESIAN_POINT('Ctrl Pts',(-45.4496257543759,-57.2111431748629,
12.));
#75679=CARTESIAN_POINT('Ctrl Pts',(-45.4423670150035,-57.1863304051011,
12.));
#75680=CARTESIAN_POINT('Ctrl Pts',(-45.4350958195434,-57.1615613423586,
12.));
#75681=CARTESIAN_POINT('Ctrl Pts',(-45.4278122464387,-57.1368360678629,
12.));
#75682=CARTESIAN_POINT('Ctrl Pts',(-45.4205163744778,-57.1121546630776,
12.));
#75683=CARTESIAN_POINT('Ctrl Pts',(-45.4132082827945,-57.0875172097048,
12.));
#75684=CARTESIAN_POINT('Ctrl Pts',(-45.4058880508693,-57.0629237896848,
12.));
#75685=CARTESIAN_POINT('Ctrl Pts',(-45.3985557585316,-57.0383744851917,
12.));
#75686=CARTESIAN_POINT('Ctrl Pts',(-45.3912114859625,-57.0138693786287,
12.));
#75687=CARTESIAN_POINT('Ctrl Pts',(-45.3838553136957,-56.9894085526383,
12.));
#75688=CARTESIAN_POINT('Ctrl Pts',(-45.3764873226202,-56.9649920901079,
12.));
#75689=CARTESIAN_POINT('Ctrl Pts',(-45.3691075939827,-56.9406200741714,
12.));
#75690=CARTESIAN_POINT('Ctrl Pts',(-45.3617162093918,-56.916292588208,12.));
#75691=CARTESIAN_POINT('Ctrl Pts',(-45.3543132508234,-56.8920097158371,
12.));
#75692=CARTESIAN_POINT('Ctrl Pts',(-45.3468988006202,-56.8677715409266,
12.));
#75693=CARTESIAN_POINT('Ctrl Pts',(-45.3394729414932,-56.8435781475982,
12.));
#75694=CARTESIAN_POINT('Ctrl Pts',(-45.3320357565241,-56.8194296202293,
12.));
#75695=CARTESIAN_POINT('Ctrl Pts',(-45.3245873291682,-56.7953260434521,
12.));
#75696=CARTESIAN_POINT('Ctrl Pts',(-45.3171277432592,-56.771267502148,12.));
#75697=CARTESIAN_POINT('Ctrl Pts',(-45.3096570830107,-56.747254081454,12.));
#75698=CARTESIAN_POINT('Ctrl Pts',(-45.3021754330169,-56.7232858667697,
12.));
#75699=CARTESIAN_POINT('Ctrl Pts',(-45.2946828782557,-56.6993629437596,
12.));
#75700=CARTESIAN_POINT('Ctrl Pts',(-45.2871795040912,-56.6754853983535,
12.));
#75701=CARTESIAN_POINT('Ctrl Pts',(-45.2796653962796,-56.6516533167398,
12.));
#75702=CARTESIAN_POINT('Ctrl Pts',(-45.2721406409706,-56.6278667853716,
12.));
#75703=CARTESIAN_POINT('Ctrl Pts',(-45.2646053247094,-56.604125890975,12.));
#75704=CARTESIAN_POINT('Ctrl Pts',(-45.2570595344382,-56.5804307205507,
12.));
#75705=CARTESIAN_POINT('Ctrl Pts',(-45.2495033574997,-56.5567813613752,
12.));
#75706=CARTESIAN_POINT('Ctrl Pts',(-45.2419368816423,-56.533177900995,12.));
#75707=CARTESIAN_POINT('Ctrl Pts',(-45.2343601950222,-56.5096204272299,
12.));
#75708=CARTESIAN_POINT('Ctrl Pts',(-45.2267733862046,-56.4861090281819,
12.));
#75709=CARTESIAN_POINT('Ctrl Pts',(-45.2191765441666,-56.4626437922385,
12.));
#75710=CARTESIAN_POINT('Ctrl Pts',(-45.2115697583002,-56.4392248080733,
12.));
#75711=CARTESIAN_POINT('Ctrl Pts',(-45.2039531184172,-56.4158521646412,
12.));
#75712=CARTESIAN_POINT('Ctrl Pts',(-45.1963267147527,-56.3925259511804,
12.));
#75713=CARTESIAN_POINT('Ctrl Pts',(-45.1886906379664,-56.3692462572228,
12.));
#75714=CARTESIAN_POINT('Ctrl Pts',(-45.1810449791451,-56.3460131725962,
12.));
#75715=CARTESIAN_POINT('Ctrl Pts',(-45.1733898298062,-56.3228267874265,
12.));
#75716=CARTESIAN_POINT('Ctrl Pts',(-45.1657252819018,-56.2996871921321,
12.));
#75717=CARTESIAN_POINT('Ctrl Pts',(-45.158051427823,-56.2765944774252,12.));
#75718=CARTESIAN_POINT('Ctrl Pts',(-45.150368360401,-56.2535487343227,12.));
#75719=CARTESIAN_POINT('Ctrl Pts',(-45.1426761729107,-56.2305500541491,
12.));
#75720=CARTESIAN_POINT('Ctrl Pts',(-45.1349749590736,-56.2075985285391,
12.));
#75721=CARTESIAN_POINT('Ctrl Pts',(-45.1272648130627,-56.1846942494321,
12.));
#75722=CARTESIAN_POINT('Ctrl Pts',(-45.119545829506,-56.1618373090729,12.));
#75723=CARTESIAN_POINT('Ctrl Pts',(-45.1118181034888,-56.1390278000226,
12.));
#75724=CARTESIAN_POINT('Ctrl Pts',(-45.1040817305563,-56.1162658151621,
12.));
#75725=CARTESIAN_POINT('Ctrl Pts',(-45.0963368067177,-56.0935514476945,
12.));
#75726=CARTESIAN_POINT('Ctrl Pts',(-45.0885834284513,-56.070884791141,12.));
#75727=CARTESIAN_POINT('Ctrl Pts',(-45.0808216927082,-56.0482659393412,
12.));
#75728=CARTESIAN_POINT('Ctrl Pts',(-45.0730516969142,-56.025694986463,12.));
#75729=CARTESIAN_POINT('Ctrl Pts',(-45.0652735389729,-56.0031720270074,
12.));
#75730=CARTESIAN_POINT('Ctrl Pts',(-45.0574873172696,-55.9806971558099,
12.));
#75731=CARTESIAN_POINT('Ctrl Pts',(-45.0496931306766,-55.958270468037,12.));
#75732=CARTESIAN_POINT('Ctrl Pts',(-45.041891078557,-55.9358920591861,12.));
#75733=CARTESIAN_POINT('Ctrl Pts',(-45.0340812607676,-55.9135620250977,
12.));
#75734=CARTESIAN_POINT('Ctrl Pts',(-45.0262637776623,-55.8912804619588,
12.));
#75735=CARTESIAN_POINT('Ctrl Pts',(-45.0184387300968,-55.8690474663058,
12.));
#75736=CARTESIAN_POINT('Ctrl Pts',(-45.0106062194325,-55.8468631350195,
12.));
#75737=CARTESIAN_POINT('Ctrl Pts',(-45.002766347541,-55.8247275653257,12.));
#75738=CARTESIAN_POINT('Ctrl Pts',(-44.9949192168073,-55.8026408548078,
12.));
#75739=CARTESIAN_POINT('Ctrl Pts',(-44.9870649301333,-55.7806031014093,
12.));
#75740=CARTESIAN_POINT('Ctrl Pts',(-44.979203590942,-55.7586144034376,12.));
#75741=CARTESIAN_POINT('Ctrl Pts',(-44.9713353031827,-55.7366748595582,
12.));
#75742=CARTESIAN_POINT('Ctrl Pts',(-44.9634601713352,-55.7147845687969,
12.));
#75743=CARTESIAN_POINT('Ctrl Pts',(-44.9555783004133,-55.6929436305522,
12.));
#75744=CARTESIAN_POINT('Ctrl Pts',(-44.9476897959694,-55.671152144599,12.));
#75745=CARTESIAN_POINT('Ctrl Pts',(-44.9397947640996,-55.6494102110922,
12.));
#75746=CARTESIAN_POINT('Ctrl Pts',(-44.9318933114483,-55.6277179305604,
12.));
#75747=CARTESIAN_POINT('Ctrl Pts',(-44.9239855452119,-55.6060754039089,
12.));
#75748=CARTESIAN_POINT('Ctrl Pts',(-44.9160715731425,-55.5844827324315,
12.));
#75749=CARTESIAN_POINT('Ctrl Pts',(-44.9081515035525,-55.5629400178136,
12.));
#75750=CARTESIAN_POINT('Ctrl Pts',(-44.9002254453192,-55.541447362135,12.));
#75751=CARTESIAN_POINT('Ctrl Pts',(-44.8922935078905,-55.5200048678648,
12.));
#75752=CARTESIAN_POINT('Ctrl Pts',(-44.8843558012903,-55.4986126378676,
12.));
#75753=CARTESIAN_POINT('Ctrl Pts',(-44.8764124361218,-55.4772707754139,
12.));
#75754=CARTESIAN_POINT('Ctrl Pts',(-44.8684635235727,-55.4559793841838,
12.));
#75755=CARTESIAN_POINT('Ctrl Pts',(-44.8605091754208,-55.4347385682697,
12.));
#75756=CARTESIAN_POINT('Ctrl Pts',(-44.8525495040397,-55.4135484321706,
12.));
#75757=CARTESIAN_POINT('Ctrl Pts',(-44.8445846224034,-55.3924090808002,
12.));
#75758=CARTESIAN_POINT('Ctrl Pts',(-44.8366146440896,-55.3713206194962,
12.));
#75759=CARTESIAN_POINT('Ctrl Pts',(-44.8286396832849,-55.350283154023,12.));
#75760=CARTESIAN_POINT('Ctrl Pts',(-44.8206598547889,-55.3292967905726,
12.));
#75761=CARTESIAN_POINT('Ctrl Pts',(-44.812675274021,-55.3083616357605,12.));
#75762=CARTESIAN_POINT('Ctrl Pts',(-44.8046860570245,-55.287477796635,12.));
#75763=CARTESIAN_POINT('Ctrl Pts',(-44.7966923204741,-55.2666453806883,
12.));
#75764=CARTESIAN_POINT('Ctrl Pts',(-44.7886941816823,-55.2458644958617,
12.));
#75765=CARTESIAN_POINT('Ctrl Pts',(-44.7806917586077,-55.2251352505475,
12.));
#75766=CARTESIAN_POINT('Ctrl Pts',(-44.7726851698619,-55.2044577535866,
12.));
#75767=CARTESIAN_POINT('Ctrl Pts',(-44.7646745347109,-55.1838321142779,
12.));
#75768=CARTESIAN_POINT('Ctrl Pts',(-44.7566599730773,-55.1632584423815,
12.));
#75769=CARTESIAN_POINT('Ctrl Pts',(-44.748641605542,-55.14273684812,12.));
#75770=CARTESIAN_POINT('Ctrl Pts',(-44.740619553348,-55.1222674421743,12.));
#75771=CARTESIAN_POINT('Ctrl Pts',(-44.7325939384035,-55.1018503356796,
12.));
#75772=CARTESIAN_POINT('Ctrl Pts',(-44.7245648832979,-55.0814856402496,
12.));
#75773=CARTESIAN_POINT('Ctrl Pts',(-44.7165325113159,-55.0611734679894,
12.));
#75774=CARTESIAN_POINT('Ctrl Pts',(-44.7084969464513,-55.0409139315078,
12.));
#75775=CARTESIAN_POINT('Ctrl Pts',(-44.7004583134249,-55.0207071439237,
12.));
#75776=CARTESIAN_POINT('Ctrl Pts',(-44.6924167376869,-55.0005532188667,
12.));
#75777=CARTESIAN_POINT('Ctrl Pts',(-44.6843723454,-54.9804522704686,12.));
#75778=CARTESIAN_POINT('Ctrl Pts',(-44.6763252634258,-54.9604044133501,
12.));
#75779=CARTESIAN_POINT('Ctrl Pts',(-44.6682756193147,-54.9404097626077,
12.));
#75780=CARTESIAN_POINT('Ctrl Pts',(-44.6602235412836,-54.9204684337822,
12.));
#75781=CARTESIAN_POINT('Ctrl Pts',(-44.6521691582533,-54.9005805428969,
12.));
#75782=CARTESIAN_POINT('Ctrl Pts',(-44.6441125999063,-54.8807462065164,
12.));
#75783=CARTESIAN_POINT('Ctrl Pts',(-44.6360539967392,-54.860965541796,12.));
#75784=CARTESIAN_POINT('Ctrl Pts',(-44.6279934801169,-54.8412386665276,
12.));
#75785=CARTESIAN_POINT('Ctrl Pts',(-44.6199311823293,-54.8215656991837,
12.));
#75786=CARTESIAN_POINT('Ctrl Pts',(-44.6118672364906,-54.8019467588278,
12.));
#75787=CARTESIAN_POINT('Ctrl Pts',(-44.6038017764309,-54.7823819650149,
12.));
#75788=CARTESIAN_POINT('Ctrl Pts',(-44.5957349366059,-54.7628714377037,
12.));
#75789=CARTESIAN_POINT('Ctrl Pts',(-44.5876668519661,-54.7434152971267,
12.));
#75790=CARTESIAN_POINT('Ctrl Pts',(-44.5795976579454,-54.7240136637717,
12.));
#75791=CARTESIAN_POINT('Ctrl Pts',(-44.5715274907619,-54.7046666586754,
12.));
#75792=CARTESIAN_POINT('Ctrl Pts',(-44.5634564876863,-54.6853744036751,
12.));
#75793=CARTESIAN_POINT('Ctrl Pts',(-44.5553847872721,-54.6661370216252,
12.));
#75794=CARTESIAN_POINT('Ctrl Pts',(-44.5473125297311,-54.6469546367408,
12.));
#75795=CARTESIAN_POINT('Ctrl Pts',(-44.5392398566802,-54.6278273743587,
12.));
#75796=CARTESIAN_POINT('Ctrl Pts',(-44.5311669104515,-54.6087553602914,
12.));
#75797=CARTESIAN_POINT('Ctrl Pts',(-44.5230938335167,-54.5897387202815,
12.));
#75798=CARTESIAN_POINT('Ctrl Pts',(-44.5150207678988,-54.5707775794412,
12.));
#75799=CARTESIAN_POINT('Ctrl Pts',(-44.5069478544945,-54.5518720616016,
12.));
#75800=CARTESIAN_POINT('Ctrl Pts',(-44.4988752343715,-54.5330222905438,
12.));
#75801=CARTESIAN_POINT('Ctrl Pts',(-44.4908030503209,-54.5142283914684,
12.));
#75802=CARTESIAN_POINT('Ctrl Pts',(-44.482731448127,-54.4954904921938,12.));
#75803=CARTESIAN_POINT('Ctrl Pts',(-44.4746605784056,-54.4768087248854,
12.));
#75804=CARTESIAN_POINT('Ctrl Pts',(-44.4665905967701,-54.4581832262072,
12.));
#75805=CARTESIAN_POINT('Ctrl Pts',(-44.4585216599933,-54.4396141337008,
12.));
#75806=CARTESIAN_POINT('Ctrl Pts',(-44.4504539226336,-54.4211015825959,
12.));
#75807=CARTESIAN_POINT('Ctrl Pts',(-44.442387534098,-54.4026457030316,12.));
#75808=CARTESIAN_POINT('Ctrl Pts',(-44.4343226339555,-54.3842466156151,
12.));
#75809=CARTESIAN_POINT('Ctrl Pts',(-44.4262593564664,-54.3659044357064,
12.));
#75810=CARTESIAN_POINT('Ctrl Pts',(-44.4181978395814,-54.347619281931,12.));
#75811=CARTESIAN_POINT('Ctrl Pts',(-44.4101382321834,-54.3293912830237,
12.));
#75812=CARTESIAN_POINT('Ctrl Pts',(-44.4020807028144,-54.3112205860776,
12.));
#75813=CARTESIAN_POINT('Ctrl Pts',(-44.3940254456427,-54.2931073621661,
12.));
#75814=CARTESIAN_POINT('Ctrl Pts',(-44.3859726620288,-54.2750517888695,
12.));
#75815=CARTESIAN_POINT('Ctrl Pts',(-44.3779225430461,-54.2570540336536,
12.));
#75816=CARTESIAN_POINT('Ctrl Pts',(-44.369875253351,-54.2391142386354,12.));
#75817=CARTESIAN_POINT('Ctrl Pts',(-44.3618309103245,-54.2212325005847,
12.));
#75818=CARTESIAN_POINT('Ctrl Pts',(-44.3537895823819,-54.203408870162,12.));
#75819=CARTESIAN_POINT('Ctrl Pts',(-44.3473589597468,-54.1891964684439,
12.));
#75820=CARTESIAN_POINT('Ctrl Pts',(-44.3425373700829,-54.1785633257456,
12.));
#75821=CARTESIAN_POINT('Ctrl Pts',(-44.3393235891014,-54.1714861895278,
12.));
#75822=CARTESIAN_POINT('Ctrl Pts',(-44.3377168516418,-54.1679505278134,
12.));
#75823=CARTESIAN_POINT('Ctrl Pts',(-44.5696260757792,-59.3276657444392,
-1.11022302462516E-15));
#75824=CARTESIAN_POINT('Ctrl Pts',(-44.5696260757792,-59.3276657444392,
4.));
#75825=CARTESIAN_POINT('Ctrl Pts',(-44.5696260757792,-59.3276657444392,
8.));
#75826=CARTESIAN_POINT('Ctrl Pts',(-44.5696260757792,-59.3276657444392,
12.));
#75827=CARTESIAN_POINT('Ctrl Pts',(-44.6658822400933,-59.3806648691719,
-1.11022302462516E-15));
#75828=CARTESIAN_POINT('Ctrl Pts',(-44.6658822400933,-59.3806648691719,
4.));
#75829=CARTESIAN_POINT('Ctrl Pts',(-44.6658822400933,-59.3806648691719,
8.));
#75830=CARTESIAN_POINT('Ctrl Pts',(-44.6658822400933,-59.3806648691719,
12.));
#75831=CARTESIAN_POINT('Ctrl Pts',(-44.8655383388341,-59.4154499491518,
-1.03713949455603E-15));
#75832=CARTESIAN_POINT('Ctrl Pts',(-44.8655383388341,-59.4154499491518,
4.));
#75833=CARTESIAN_POINT('Ctrl Pts',(-44.8655383388341,-59.4154499491518,
7.99999999999999));
#75834=CARTESIAN_POINT('Ctrl Pts',(-44.8655383388341,-59.4154499491518,
12.));
#75835=CARTESIAN_POINT('Ctrl Pts',(-45.047980595232,-59.3374774995081,-8.63611844427577E-16));
#75836=CARTESIAN_POINT('Ctrl Pts',(-45.047980595232,-59.3374774995081,4.));
#75837=CARTESIAN_POINT('Ctrl Pts',(-45.0479805952321,-59.3374774995081,
8.00000000000001));
#75838=CARTESIAN_POINT('Ctrl Pts',(-45.0479805952321,-59.3374774995081,
12.));
#75839=CARTESIAN_POINT('Ctrl Pts',(-45.1135644683452,-59.2875729049565,
-7.79957864199761E-16));
#75840=CARTESIAN_POINT('Ctrl Pts',(-45.1135644683452,-59.2875729049565,
4.));
#75841=CARTESIAN_POINT('Ctrl Pts',(-45.1135644683452,-59.2875729049565,
8.));
#75842=CARTESIAN_POINT('Ctrl Pts',(-45.1135644683452,-59.2875729049565,
12.));
#75843=CARTESIAN_POINT('',(-44.5696260757792,-59.3276657444392,2.77555756156289E-16));
#75844=CARTESIAN_POINT('',(-45.1135644683449,-59.2875729049561,2.77555756156289E-16));
#75845=CARTESIAN_POINT('Ctrl Pts',(-44.5696260757792,-59.3276657444392,
-3.21795698712167E-17));
#75846=CARTESIAN_POINT('Ctrl Pts',(-44.6658822400933,-59.3806648691719,
-3.2179569871217E-17));
#75847=CARTESIAN_POINT('Ctrl Pts',(-44.7799714393737,-59.4005420577319,
9.58244731114085E-18));
#75848=CARTESIAN_POINT('Ctrl Pts',(-44.8884397921749,-59.3836004611086,
8.41425445128705E-17));
#75849=CARTESIAN_POINT('Ctrl Pts',(-44.9697910567758,-59.3708942636411,
1.40062617414167E-16));
#75850=CARTESIAN_POINT('Ctrl Pts',(-45.047980595232,-59.3374774995081,2.14431610326361E-16));
#75851=CARTESIAN_POINT('Ctrl Pts',(-45.1135644683452,-59.2875729049565,
2.98085590554179E-16));
#75852=CARTESIAN_POINT('',(-45.1135644683449,-59.2875729049561,12.));
#75853=CARTESIAN_POINT('Ctrl Pts',(-45.1135644683452,-59.2875729049565,
-7.79957864199761E-16));
#75854=CARTESIAN_POINT('Ctrl Pts',(-45.1135644683452,-59.2875729049565,
4.));
#75855=CARTESIAN_POINT('Ctrl Pts',(-45.1135644683452,-59.2875729049565,
8.));
#75856=CARTESIAN_POINT('Ctrl Pts',(-45.1135644683452,-59.2875729049565,
12.));
#75857=CARTESIAN_POINT('',(-44.5696260757792,-59.3276657444392,12.));
#75858=CARTESIAN_POINT('Ctrl Pts',(-45.1135644683452,-59.2875729049565,
12.));
#75859=CARTESIAN_POINT('Ctrl Pts',(-45.0479805952321,-59.3374774995081,
12.));
#75860=CARTESIAN_POINT('Ctrl Pts',(-44.9697910567758,-59.3708942636412,
12.));
#75861=CARTESIAN_POINT('Ctrl Pts',(-44.8884397921749,-59.3836004611086,
12.));
#75862=CARTESIAN_POINT('Ctrl Pts',(-44.7799714393738,-59.4005420577319,
12.));
#75863=CARTESIAN_POINT('Ctrl Pts',(-44.6658822400933,-59.3806648691719,
12.));
#75864=CARTESIAN_POINT('Ctrl Pts',(-44.5696260757792,-59.3276657444392,
12.));
#75865=CARTESIAN_POINT('Ctrl Pts',(-44.5696260757792,-59.3276657444392,
12.));
#75866=CARTESIAN_POINT('Ctrl Pts',(-44.5696260757792,-59.3276657444392,
8.));
#75867=CARTESIAN_POINT('Ctrl Pts',(-44.5696260757792,-59.3276657444392,
4.));
#75868=CARTESIAN_POINT('Ctrl Pts',(-44.5696260757792,-59.3276657444392,
-1.11022302462516E-15));
#75869=CARTESIAN_POINT('Origin',(-2.28111678886296E-10,-2.97443977737815E-10,
0.));
#75870=CARTESIAN_POINT('Origin',(-2.28111678886296E-10,-2.97443977737815E-10,
12.));
#75871=CARTESIAN_POINT('Origin',(-2.28111678886296E-10,-2.97443977737815E-10,
0.));
#75872=CARTESIAN_POINT('Ctrl Pts',(-50.5529731960877,-54.7233670476848,
0.));
#75873=CARTESIAN_POINT('Ctrl Pts',(-50.5529731960877,-54.7233670476848,
4.));
#75874=CARTESIAN_POINT('Ctrl Pts',(-50.5529731960877,-54.7233670476848,
8.));
#75875=CARTESIAN_POINT('Ctrl Pts',(-50.5529731960877,-54.7233670476848,
12.));
#75876=CARTESIAN_POINT('Ctrl Pts',(-50.6336864649948,-54.6488048279282,
0.));
#75877=CARTESIAN_POINT('Ctrl Pts',(-50.6336864649948,-54.6488048279282,
4.));
#75878=CARTESIAN_POINT('Ctrl Pts',(-50.6336864649948,-54.6488048279283,
8.));
#75879=CARTESIAN_POINT('Ctrl Pts',(-50.6336864649948,-54.6488048279283,
12.));
#75880=CARTESIAN_POINT('Ctrl Pts',(-50.7298112257546,-54.4703879751554,
0.));
#75881=CARTESIAN_POINT('Ctrl Pts',(-50.7298112257546,-54.4703879751554,
4.00000000000001));
#75882=CARTESIAN_POINT('Ctrl Pts',(-50.7298112257546,-54.4703879751553,
8.));
#75883=CARTESIAN_POINT('Ctrl Pts',(-50.7298112257546,-54.4703879751553,
12.));
#75884=CARTESIAN_POINT('Ctrl Pts',(-50.7135202769404,-54.2726521137409,
0.));
#75885=CARTESIAN_POINT('Ctrl Pts',(-50.7135202769404,-54.2726521137409,
4.));
#75886=CARTESIAN_POINT('Ctrl Pts',(-50.7135202769404,-54.2726521137408,
8.00000000000001));
#75887=CARTESIAN_POINT('Ctrl Pts',(-50.7135202769404,-54.2726521137408,
12.));
#75888=CARTESIAN_POINT('Ctrl Pts',(-50.6869108458687,-54.1946543499977,
0.));
#75889=CARTESIAN_POINT('Ctrl Pts',(-50.6869108458687,-54.1946543499977,
4.));
#75890=CARTESIAN_POINT('Ctrl Pts',(-50.6869108458687,-54.1946543499977,
8.));
#75891=CARTESIAN_POINT('Ctrl Pts',(-50.6869108458687,-54.1946543499977,
12.));
#75892=CARTESIAN_POINT('',(-50.5529731960877,-54.7233670476848,0.));
#75893=CARTESIAN_POINT('',(-50.6869108458688,-54.1946543499977,0.));
#75894=CARTESIAN_POINT('Ctrl Pts',(-50.5529731960877,-54.7233670476848,
0.));
#75895=CARTESIAN_POINT('Ctrl Pts',(-50.6336864649948,-54.6488048279282,
0.));
#75896=CARTESIAN_POINT('Ctrl Pts',(-50.6886148997147,-54.5468523406295,
0.));
#75897=CARTESIAN_POINT('Ctrl Pts',(-50.7068361639614,-54.438591605611,0.));
#75898=CARTESIAN_POINT('Ctrl Pts',(-50.7205021121465,-54.3573960543471,
0.));
#75899=CARTESIAN_POINT('Ctrl Pts',(-50.7135202769404,-54.2726521137409,
0.));
#75900=CARTESIAN_POINT('Ctrl Pts',(-50.6869108458687,-54.1946543499977,
0.));
#75901=CARTESIAN_POINT('',(-50.6869108458688,-54.1946543499976,12.));
#75902=CARTESIAN_POINT('Ctrl Pts',(-50.6869108458687,-54.1946543499977,
0.));
#75903=CARTESIAN_POINT('Ctrl Pts',(-50.6869108458687,-54.1946543499977,
4.));
#75904=CARTESIAN_POINT('Ctrl Pts',(-50.6869108458687,-54.1946543499977,
8.));
#75905=CARTESIAN_POINT('Ctrl Pts',(-50.6869108458687,-54.1946543499977,
12.));
#75906=CARTESIAN_POINT('',(-50.5529731960877,-54.7233670476848,12.));
#75907=CARTESIAN_POINT('Ctrl Pts',(-50.6869108458687,-54.1946543499977,
12.));
#75908=CARTESIAN_POINT('Ctrl Pts',(-50.7135202769404,-54.2726521137408,
12.));
#75909=CARTESIAN_POINT('Ctrl Pts',(-50.7205021121465,-54.357396054347,12.));
#75910=CARTESIAN_POINT('Ctrl Pts',(-50.7068361639614,-54.4385916056109,
12.));
#75911=CARTESIAN_POINT('Ctrl Pts',(-50.6886148997147,-54.5468523406294,
12.));
#75912=CARTESIAN_POINT('Ctrl Pts',(-50.6336864649948,-54.6488048279283,
12.));
#75913=CARTESIAN_POINT('Ctrl Pts',(-50.5529731960877,-54.7233670476848,
12.));
#75914=CARTESIAN_POINT('Ctrl Pts',(-50.5529731960877,-54.7233670476848,
12.));
#75915=CARTESIAN_POINT('Ctrl Pts',(-50.5529731960877,-54.7233670476848,
8.));
#75916=CARTESIAN_POINT('Ctrl Pts',(-50.5529731960877,-54.7233670476848,
4.));
#75917=CARTESIAN_POINT('Ctrl Pts',(-50.5529731960877,-54.7233670476848,
0.));
#75918=CARTESIAN_POINT('Ctrl Pts',(-48.8900464144686,-50.0975384783634,
0.));
#75919=CARTESIAN_POINT('Ctrl Pts',(-48.8900464144686,-50.0975384783634,
12.));
#75920=CARTESIAN_POINT('Ctrl Pts',(-48.8919551910299,-50.1009206494209,
0.));
#75921=CARTESIAN_POINT('Ctrl Pts',(-48.8919551910299,-50.1009206494209,
12.));
#75922=CARTESIAN_POINT('Ctrl Pts',(-48.8957735556681,-50.1076907555303,
0.));
#75923=CARTESIAN_POINT('Ctrl Pts',(-48.8957735556681,-50.1076907555303,
12.));
#75924=CARTESIAN_POINT('Ctrl Pts',(-48.9015035371772,-50.1178632066821,
0.));
#75925=CARTESIAN_POINT('Ctrl Pts',(-48.9015035371772,-50.1178632066821,
12.));
#75926=CARTESIAN_POINT('Ctrl Pts',(-48.9091483817797,-50.1314610602286,
0.));
#75927=CARTESIAN_POINT('Ctrl Pts',(-48.9091483817797,-50.1314610602286,
12.));
#75928=CARTESIAN_POINT('Ctrl Pts',(-48.9187125417897,-50.148516018447,0.));
#75929=CARTESIAN_POINT('Ctrl Pts',(-48.9187125417897,-50.148516018447,12.));
#75930=CARTESIAN_POINT('Ctrl Pts',(-48.9282847698237,-50.1656286003943,
0.));
#75931=CARTESIAN_POINT('Ctrl Pts',(-48.9282847698237,-50.1656286003943,
12.));
#75932=CARTESIAN_POINT('Ctrl Pts',(-48.9378649933116,-50.1827987615659,
0.));
#75933=CARTESIAN_POINT('Ctrl Pts',(-48.9378649933116,-50.1827987615659,
12.));
#75934=CARTESIAN_POINT('Ctrl Pts',(-48.9474530868847,-50.2000264157903,
0.));
#75935=CARTESIAN_POINT('Ctrl Pts',(-48.9474530868847,-50.2000264157903,
12.));
#75936=CARTESIAN_POINT('Ctrl Pts',(-48.9570488741273,-50.2173114358423,
0.));
#75937=CARTESIAN_POINT('Ctrl Pts',(-48.9570488741273,-50.2173114358423,
12.));
#75938=CARTESIAN_POINT('Ctrl Pts',(-48.9666521500969,-50.2346536715465,
0.));
#75939=CARTESIAN_POINT('Ctrl Pts',(-48.9666521500969,-50.2346536715465,
12.));
#75940=CARTESIAN_POINT('Ctrl Pts',(-48.9762626987227,-50.252052963548,0.));
#75941=CARTESIAN_POINT('Ctrl Pts',(-48.9762626987227,-50.252052963548,12.));
#75942=CARTESIAN_POINT('Ctrl Pts',(-48.9858803116649,-50.2695091583473,
0.));
#75943=CARTESIAN_POINT('Ctrl Pts',(-48.9858803116649,-50.2695091583473,
12.));
#75944=CARTESIAN_POINT('Ctrl Pts',(-48.9955048082028,-50.2870221241003,
0.));
#75945=CARTESIAN_POINT('Ctrl Pts',(-48.9955048082028,-50.2870221241003,
12.));
#75946=CARTESIAN_POINT('Ctrl Pts',(-49.0051360288002,-50.3045917455383,
0.));
#75947=CARTESIAN_POINT('Ctrl Pts',(-49.0051360288002,-50.3045917455383,
12.));
#75948=CARTESIAN_POINT('Ctrl Pts',(-49.0147738256925,-50.3222179165102,
0.));
#75949=CARTESIAN_POINT('Ctrl Pts',(-49.0147738256925,-50.3222179165102,
12.));
#75950=CARTESIAN_POINT('Ctrl Pts',(-49.0244180550759,-50.3399005337967,
0.));
#75951=CARTESIAN_POINT('Ctrl Pts',(-49.0244180550759,-50.3399005337967,
12.));
#75952=CARTESIAN_POINT('Ctrl Pts',(-49.034068567401,-50.3576394894136,0.));
#75953=CARTESIAN_POINT('Ctrl Pts',(-49.034068567401,-50.3576394894136,12.));
#75954=CARTESIAN_POINT('Ctrl Pts',(-49.0437252024868,-50.3754346667389,
0.));
#75955=CARTESIAN_POINT('Ctrl Pts',(-49.0437252024868,-50.3754346667389,
12.));
#75956=CARTESIAN_POINT('Ctrl Pts',(-49.0533877945771,-50.393285944528,0.));
#75957=CARTESIAN_POINT('Ctrl Pts',(-49.0533877945771,-50.393285944528,12.));
#75958=CARTESIAN_POINT('Ctrl Pts',(-49.0630561755082,-50.4111931994264,
0.));
#75959=CARTESIAN_POINT('Ctrl Pts',(-49.0630561755082,-50.4111931994264,
12.));
#75960=CARTESIAN_POINT('Ctrl Pts',(-49.0727301783477,-50.4291563088528,
0.));
#75961=CARTESIAN_POINT('Ctrl Pts',(-49.0727301783477,-50.4291563088528,
12.));
#75962=CARTESIAN_POINT('Ctrl Pts',(-49.0824096415339,-50.4471751542717,
0.));
#75963=CARTESIAN_POINT('Ctrl Pts',(-49.0824096415339,-50.4471751542717,
12.));
#75964=CARTESIAN_POINT('Ctrl Pts',(-49.0920944086973,-50.465249621057,0.));
#75965=CARTESIAN_POINT('Ctrl Pts',(-49.0920944086973,-50.465249621057,12.));
#75966=CARTESIAN_POINT('Ctrl Pts',(-49.1017843266782,-50.4833795969296,
0.));
#75967=CARTESIAN_POINT('Ctrl Pts',(-49.1017843266782,-50.4833795969296,
12.));
#75968=CARTESIAN_POINT('Ctrl Pts',(-49.1114792441573,-50.5015649708742,
0.));
#75969=CARTESIAN_POINT('Ctrl Pts',(-49.1114792441573,-50.5015649708742,
12.));
#75970=CARTESIAN_POINT('Ctrl Pts',(-49.1211790099817,-50.5198056318111,
0.));
#75971=CARTESIAN_POINT('Ctrl Pts',(-49.1211790099817,-50.5198056318111,
12.));
#75972=CARTESIAN_POINT('Ctrl Pts',(-49.1308834717645,-50.5381014674822,
0.));
#75973=CARTESIAN_POINT('Ctrl Pts',(-49.1308834717645,-50.5381014674822,
12.));
#75974=CARTESIAN_POINT('Ctrl Pts',(-49.1405924766169,-50.5564523650406,
0.));
#75975=CARTESIAN_POINT('Ctrl Pts',(-49.1405924766169,-50.5564523650406,
12.));
#75976=CARTESIAN_POINT('Ctrl Pts',(-49.1503058717831,-50.5748582115575,
0.));
#75977=CARTESIAN_POINT('Ctrl Pts',(-49.1503058717831,-50.5748582115575,
12.));
#75978=CARTESIAN_POINT('Ctrl Pts',(-49.1600235052613,-50.593318894516,0.));
#75979=CARTESIAN_POINT('Ctrl Pts',(-49.1600235052613,-50.593318894516,12.));
#75980=CARTESIAN_POINT('Ctrl Pts',(-49.1697452265473,-50.6118343023937,
0.));
#75981=CARTESIAN_POINT('Ctrl Pts',(-49.1697452265473,-50.6118343023937,
12.));
#75982=CARTESIAN_POINT('Ctrl Pts',(-49.1794708869074,-50.6304043248796,
0.));
#75983=CARTESIAN_POINT('Ctrl Pts',(-49.1794708869074,-50.6304043248796,
12.));
#75984=CARTESIAN_POINT('Ctrl Pts',(-49.1892003389743,-50.6490288525639,
0.));
#75985=CARTESIAN_POINT('Ctrl Pts',(-49.1892003389743,-50.6490288525639,
12.));
#75986=CARTESIAN_POINT('Ctrl Pts',(-49.1989334364992,-50.6677077767427,
0.));
#75987=CARTESIAN_POINT('Ctrl Pts',(-49.1989334364992,-50.6677077767427,
12.));
#75988=CARTESIAN_POINT('Ctrl Pts',(-49.2086700340625,-50.6864409891905,
0.));
#75989=CARTESIAN_POINT('Ctrl Pts',(-49.2086700340625,-50.6864409891905,
12.));
#75990=CARTESIAN_POINT('Ctrl Pts',(-49.218409986748,-50.7052283818941,0.));
#75991=CARTESIAN_POINT('Ctrl Pts',(-49.218409986748,-50.7052283818941,12.));
#75992=CARTESIAN_POINT('Ctrl Pts',(-49.2281531501569,-50.7240698470698,
0.));
#75993=CARTESIAN_POINT('Ctrl Pts',(-49.2281531501569,-50.7240698470698,
12.));
#75994=CARTESIAN_POINT('Ctrl Pts',(-49.2378993805482,-50.7429652772816,
0.));
#75995=CARTESIAN_POINT('Ctrl Pts',(-49.2378993805482,-50.7429652772816,
12.));
#75996=CARTESIAN_POINT('Ctrl Pts',(-49.2476485349373,-50.7619145655207,
0.));
#75997=CARTESIAN_POINT('Ctrl Pts',(-49.2476485349373,-50.7619145655207,
12.));
#75998=CARTESIAN_POINT('Ctrl Pts',(-49.2574004712122,-50.7809176052954,
0.));
#75999=CARTESIAN_POINT('Ctrl Pts',(-49.2574004712122,-50.7809176052954,
12.));
#76000=CARTESIAN_POINT('Ctrl Pts',(-49.2671550482415,-50.7999742907111,
0.));
#76001=CARTESIAN_POINT('Ctrl Pts',(-49.2671550482415,-50.7999742907111,
12.));
#76002=CARTESIAN_POINT('Ctrl Pts',(-49.2769121258144,-50.8190845164319,
0.));
#76003=CARTESIAN_POINT('Ctrl Pts',(-49.2769121258144,-50.8190845164319,
12.));
#76004=CARTESIAN_POINT('Ctrl Pts',(-49.2866715645828,-50.8382481776392,
0.));
#76005=CARTESIAN_POINT('Ctrl Pts',(-49.2866715645828,-50.8382481776392,
12.));
#76006=CARTESIAN_POINT('Ctrl Pts',(-49.2964332260043,-50.8574651699877,
0.));
#76007=CARTESIAN_POINT('Ctrl Pts',(-49.2964332260043,-50.8574651699877,
12.));
#76008=CARTESIAN_POINT('Ctrl Pts',(-49.3061969722798,-50.8767353895509,
0.));
#76009=CARTESIAN_POINT('Ctrl Pts',(-49.3061969722798,-50.8767353895509,
12.));
#76010=CARTESIAN_POINT('Ctrl Pts',(-49.3159626663129,-50.8960587327869,
0.));
#76011=CARTESIAN_POINT('Ctrl Pts',(-49.3159626663129,-50.8960587327869,
12.));
#76012=CARTESIAN_POINT('Ctrl Pts',(-49.325730171735,-50.9154350965681,0.));
#76013=CARTESIAN_POINT('Ctrl Pts',(-49.325730171735,-50.9154350965681,12.));
#76014=CARTESIAN_POINT('Ctrl Pts',(-49.3354993529163,-50.9348643781928,
0.));
#76015=CARTESIAN_POINT('Ctrl Pts',(-49.3354993529163,-50.9348643781928,
12.));
#76016=CARTESIAN_POINT('Ctrl Pts',(-49.3452700749804,-50.9543464753974,
0.));
#76017=CARTESIAN_POINT('Ctrl Pts',(-49.3452700749804,-50.9543464753974,
12.));
#76018=CARTESIAN_POINT('Ctrl Pts',(-49.3550422038221,-50.9738812863636,
0.));
#76019=CARTESIAN_POINT('Ctrl Pts',(-49.3550422038221,-50.9738812863636,
12.));
#76020=CARTESIAN_POINT('Ctrl Pts',(-49.3648156061049,-50.9934687097179,
0.));
#76021=CARTESIAN_POINT('Ctrl Pts',(-49.3648156061049,-50.9934687097179,
12.));
#76022=CARTESIAN_POINT('Ctrl Pts',(-49.3745901492429,-51.0131086445268,
0.));
#76023=CARTESIAN_POINT('Ctrl Pts',(-49.3745901492429,-51.0131086445268,
12.));
#76024=CARTESIAN_POINT('Ctrl Pts',(-49.3843657013851,-51.0328009902857,
0.));
#76025=CARTESIAN_POINT('Ctrl Pts',(-49.3843657013851,-51.0328009902857,
12.));
#76026=CARTESIAN_POINT('Ctrl Pts',(-49.3941421314014,-51.0525456469072,
0.));
#76027=CARTESIAN_POINT('Ctrl Pts',(-49.3941421314014,-51.0525456469072,
12.));
#76028=CARTESIAN_POINT('Ctrl Pts',(-49.4039193088636,-51.0723425146987,
0.));
#76029=CARTESIAN_POINT('Ctrl Pts',(-49.4039193088636,-51.0723425146987,
12.));
#76030=CARTESIAN_POINT('Ctrl Pts',(-49.4136971040428,-51.0921914943663,
0.));
#76031=CARTESIAN_POINT('Ctrl Pts',(-49.4136971040428,-51.0921914943663,
12.));
#76032=CARTESIAN_POINT('Ctrl Pts',(-49.4234753879071,-51.1120924870196,
0.));
#76033=CARTESIAN_POINT('Ctrl Pts',(-49.4234753879071,-51.1120924870196,
12.));
#76034=CARTESIAN_POINT('Ctrl Pts',(-49.4332540321178,-51.1320453941702,
0.));
#76035=CARTESIAN_POINT('Ctrl Pts',(-49.4332540321178,-51.1320453941702,
12.));
#76036=CARTESIAN_POINT('Ctrl Pts',(-49.4430329090288,-51.1520501177291,
0.));
#76037=CARTESIAN_POINT('Ctrl Pts',(-49.4430329090288,-51.1520501177291,
12.));
#76038=CARTESIAN_POINT('Ctrl Pts',(-49.4528118916833,-51.1721065599972,
0.));
#76039=CARTESIAN_POINT('Ctrl Pts',(-49.4528118916833,-51.1721065599972,
12.));
#76040=CARTESIAN_POINT('Ctrl Pts',(-49.4625908538076,-51.1922146236686,
0.));
#76041=CARTESIAN_POINT('Ctrl Pts',(-49.4625908538076,-51.1922146236686,
12.));
#76042=CARTESIAN_POINT('Ctrl Pts',(-49.4723696698022,-51.2123742118288,
0.));
#76043=CARTESIAN_POINT('Ctrl Pts',(-49.4723696698022,-51.2123742118288,
12.));
#76044=CARTESIAN_POINT('Ctrl Pts',(-49.4821482147357,-51.2325852279507,
0.));
#76045=CARTESIAN_POINT('Ctrl Pts',(-49.4821482147357,-51.2325852279507,
12.));
#76046=CARTESIAN_POINT('Ctrl Pts',(-49.4919263643357,-51.2528475758841,
0.));
#76047=CARTESIAN_POINT('Ctrl Pts',(-49.4919263643357,-51.2528475758841,
12.));
#76048=CARTESIAN_POINT('Ctrl Pts',(-49.5017039949841,-51.2731611598465,
0.));
#76049=CARTESIAN_POINT('Ctrl Pts',(-49.5017039949841,-51.2731611598465,
12.));
#76050=CARTESIAN_POINT('Ctrl Pts',(-49.5114809837111,-51.2935258844278,
0.));
#76051=CARTESIAN_POINT('Ctrl Pts',(-49.5114809837111,-51.2935258844278,
12.));
#76052=CARTESIAN_POINT('Ctrl Pts',(-49.5212572081901,-51.3139416545903,
0.));
#76053=CARTESIAN_POINT('Ctrl Pts',(-49.5212572081901,-51.3139416545903,
12.));
#76054=CARTESIAN_POINT('Ctrl Pts',(-49.5310325467334,-51.3344083756659,
0.));
#76055=CARTESIAN_POINT('Ctrl Pts',(-49.5310325467334,-51.3344083756659,
12.));
#76056=CARTESIAN_POINT('Ctrl Pts',(-49.5408068782871,-51.354925953347,0.));
#76057=CARTESIAN_POINT('Ctrl Pts',(-49.5408068782871,-51.354925953347,12.));
#76058=CARTESIAN_POINT('Ctrl Pts',(-49.5505800824268,-51.3754942936796,
0.));
#76059=CARTESIAN_POINT('Ctrl Pts',(-49.5505800824268,-51.3754942936796,
12.));
#76060=CARTESIAN_POINT('Ctrl Pts',(-49.5603520393514,-51.3961133030688,
0.));
#76061=CARTESIAN_POINT('Ctrl Pts',(-49.5603520393514,-51.3961133030688,
12.));
#76062=CARTESIAN_POINT('Ctrl Pts',(-49.5701226298779,-51.4167828882765,
0.));
#76063=CARTESIAN_POINT('Ctrl Pts',(-49.5701226298779,-51.4167828882765,
12.));
#76064=CARTESIAN_POINT('Ctrl Pts',(-49.579891735436,-51.4375029564191,0.));
#76065=CARTESIAN_POINT('Ctrl Pts',(-49.579891735436,-51.4375029564191,12.));
#76066=CARTESIAN_POINT('Ctrl Pts',(-49.5896592380634,-51.4582734149562,
0.));
#76067=CARTESIAN_POINT('Ctrl Pts',(-49.5896592380634,-51.4582734149562,
12.));
#76068=CARTESIAN_POINT('Ctrl Pts',(-49.5994250204003,-51.4790941716859,
0.));
#76069=CARTESIAN_POINT('Ctrl Pts',(-49.5994250204003,-51.4790941716859,
12.));
#76070=CARTESIAN_POINT('Ctrl Pts',(-49.609188965684,-51.4999651347496,0.));
#76071=CARTESIAN_POINT('Ctrl Pts',(-49.609188965684,-51.4999651347496,12.));
#76072=CARTESIAN_POINT('Ctrl Pts',(-49.6189509577441,-51.5208862126303,
0.));
#76073=CARTESIAN_POINT('Ctrl Pts',(-49.6189509577441,-51.5208862126303,
12.));
#76074=CARTESIAN_POINT('Ctrl Pts',(-49.6287108809975,-51.5418573141494,
0.));
#76075=CARTESIAN_POINT('Ctrl Pts',(-49.6287108809975,-51.5418573141494,
12.));
#76076=CARTESIAN_POINT('Ctrl Pts',(-49.6384686204443,-51.5628783484556,
0.));
#76077=CARTESIAN_POINT('Ctrl Pts',(-49.6384686204443,-51.5628783484556,
12.));
#76078=CARTESIAN_POINT('Ctrl Pts',(-49.6482240616627,-51.5839492250218,
0.));
#76079=CARTESIAN_POINT('Ctrl Pts',(-49.6482240616627,-51.5839492250218,
12.));
#76080=CARTESIAN_POINT('Ctrl Pts',(-49.6579770908063,-51.6050698536525,
0.));
#76081=CARTESIAN_POINT('Ctrl Pts',(-49.6579770908063,-51.6050698536525,
12.));
#76082=CARTESIAN_POINT('Ctrl Pts',(-49.6677275945975,-51.6262401444799,
0.));
#76083=CARTESIAN_POINT('Ctrl Pts',(-49.6677275945975,-51.6262401444799,
12.));
#76084=CARTESIAN_POINT('Ctrl Pts',(-49.6774754603235,-51.6474600079611,
0.));
#76085=CARTESIAN_POINT('Ctrl Pts',(-49.6774754603235,-51.6474600079611,
12.));
#76086=CARTESIAN_POINT('Ctrl Pts',(-49.6872205758314,-51.6687293548656,
0.));
#76087=CARTESIAN_POINT('Ctrl Pts',(-49.6872205758314,-51.6687293548656,
12.));
#76088=CARTESIAN_POINT('Ctrl Pts',(-49.6969628295236,-51.6900480962744,
0.));
#76089=CARTESIAN_POINT('Ctrl Pts',(-49.6969628295236,-51.6900480962744,
12.));
#76090=CARTESIAN_POINT('Ctrl Pts',(-49.7067021103534,-51.7114161435848,
0.));
#76091=CARTESIAN_POINT('Ctrl Pts',(-49.7067021103534,-51.7114161435848,
12.));
#76092=CARTESIAN_POINT('Ctrl Pts',(-49.7164383078206,-51.7328334085084,
0.));
#76093=CARTESIAN_POINT('Ctrl Pts',(-49.7164383078206,-51.7328334085084,
12.));
#76094=CARTESIAN_POINT('Ctrl Pts',(-49.7261713119672,-51.754299803068,0.));
#76095=CARTESIAN_POINT('Ctrl Pts',(-49.7261713119672,-51.754299803068,12.));
#76096=CARTESIAN_POINT('Ctrl Pts',(-49.7359010133741,-51.7758152395857,
0.));
#76097=CARTESIAN_POINT('Ctrl Pts',(-49.7359010133741,-51.7758152395857,
12.));
#76098=CARTESIAN_POINT('Ctrl Pts',(-49.7456273031555,-51.7973796306826,
0.));
#76099=CARTESIAN_POINT('Ctrl Pts',(-49.7456273031555,-51.7973796306826,
12.));
#76100=CARTESIAN_POINT('Ctrl Pts',(-49.7553500729563,-51.8189928892841,
0.));
#76101=CARTESIAN_POINT('Ctrl Pts',(-49.7553500729563,-51.8189928892841,
12.));
#76102=CARTESIAN_POINT('Ctrl Pts',(-49.7650692149464,-51.8406549286177,
0.));
#76103=CARTESIAN_POINT('Ctrl Pts',(-49.7650692149464,-51.8406549286177,
12.));
#76104=CARTESIAN_POINT('Ctrl Pts',(-49.7747846218177,-51.8623656622092,
0.));
#76105=CARTESIAN_POINT('Ctrl Pts',(-49.7747846218177,-51.8623656622092,
12.));
#76106=CARTESIAN_POINT('Ctrl Pts',(-49.78449618678,-51.8841250038716,0.));
#76107=CARTESIAN_POINT('Ctrl Pts',(-49.78449618678,-51.8841250038716,12.));
#76108=CARTESIAN_POINT('Ctrl Pts',(-49.7942038035568,-51.9059328677051,
0.));
#76109=CARTESIAN_POINT('Ctrl Pts',(-49.7942038035568,-51.9059328677051,
12.));
#76110=CARTESIAN_POINT('Ctrl Pts',(-49.8039073663808,-51.9277891681014,
0.));
#76111=CARTESIAN_POINT('Ctrl Pts',(-49.8039073663808,-51.9277891681014,
12.));
#76112=CARTESIAN_POINT('Ctrl Pts',(-49.8136067699896,-51.9496938197418,
0.));
#76113=CARTESIAN_POINT('Ctrl Pts',(-49.8136067699896,-51.9496938197418,
12.));
#76114=CARTESIAN_POINT('Ctrl Pts',(-49.8233019096224,-51.9716467375938,
0.));
#76115=CARTESIAN_POINT('Ctrl Pts',(-49.8233019096224,-51.9716467375938,
12.));
#76116=CARTESIAN_POINT('Ctrl Pts',(-49.8329926810172,-51.9936478369008,
0.));
#76117=CARTESIAN_POINT('Ctrl Pts',(-49.8329926810172,-51.9936478369008,
12.));
#76118=CARTESIAN_POINT('Ctrl Pts',(-49.8426789804068,-52.015697033182,0.));
#76119=CARTESIAN_POINT('Ctrl Pts',(-49.8426789804068,-52.015697033182,12.));
#76120=CARTESIAN_POINT('Ctrl Pts',(-49.8523607045146,-52.0377942422373,
0.));
#76121=CARTESIAN_POINT('Ctrl Pts',(-49.8523607045146,-52.0377942422373,
12.));
#76122=CARTESIAN_POINT('Ctrl Pts',(-49.8620377505498,-52.059939380145,0.));
#76123=CARTESIAN_POINT('Ctrl Pts',(-49.8620377505498,-52.059939380145,12.));
#76124=CARTESIAN_POINT('Ctrl Pts',(-49.871710016205,-52.0821323632588,0.));
#76125=CARTESIAN_POINT('Ctrl Pts',(-49.871710016205,-52.0821323632588,12.));
#76126=CARTESIAN_POINT('Ctrl Pts',(-49.8813773996523,-52.1043731081968,
0.));
#76127=CARTESIAN_POINT('Ctrl Pts',(-49.8813773996523,-52.1043731081968,
12.));
#76128=CARTESIAN_POINT('Ctrl Pts',(-49.8910397995404,-52.1266615318414,
0.));
#76129=CARTESIAN_POINT('Ctrl Pts',(-49.8910397995404,-52.1266615318414,
12.));
#76130=CARTESIAN_POINT('Ctrl Pts',(-49.90069711499,-52.1489975513449,0.));
#76131=CARTESIAN_POINT('Ctrl Pts',(-49.90069711499,-52.1489975513449,12.));
#76132=CARTESIAN_POINT('Ctrl Pts',(-49.9103492455904,-52.1713810841277,
0.));
#76133=CARTESIAN_POINT('Ctrl Pts',(-49.9103492455904,-52.1713810841277,
12.));
#76134=CARTESIAN_POINT('Ctrl Pts',(-49.919996091396,-52.1938120478752,0.));
#76135=CARTESIAN_POINT('Ctrl Pts',(-49.919996091396,-52.1938120478752,12.));
#76136=CARTESIAN_POINT('Ctrl Pts',(-49.9296375529241,-52.2162903605272,
0.));
#76137=CARTESIAN_POINT('Ctrl Pts',(-49.9296375529241,-52.2162903605272,
12.));
#76138=CARTESIAN_POINT('Ctrl Pts',(-49.9392735311507,-52.238815940277,0.));
#76139=CARTESIAN_POINT('Ctrl Pts',(-49.9392735311507,-52.238815940277,12.));
#76140=CARTESIAN_POINT('Ctrl Pts',(-49.9489039275064,-52.2613887055773,
0.));
#76141=CARTESIAN_POINT('Ctrl Pts',(-49.9489039275064,-52.2613887055773,
12.));
#76142=CARTESIAN_POINT('Ctrl Pts',(-49.9585286438734,-52.2840085751385,
0.));
#76143=CARTESIAN_POINT('Ctrl Pts',(-49.9585286438734,-52.2840085751385,
12.));
#76144=CARTESIAN_POINT('Ctrl Pts',(-49.9681475825824,-52.3066754679265,
0.));
#76145=CARTESIAN_POINT('Ctrl Pts',(-49.9681475825824,-52.3066754679265,
12.));
#76146=CARTESIAN_POINT('Ctrl Pts',(-49.9777606464103,-52.3293893031524,
0.));
#76147=CARTESIAN_POINT('Ctrl Pts',(-49.9777606464103,-52.3293893031524,
12.));
#76148=CARTESIAN_POINT('Ctrl Pts',(-49.9873677385769,-52.3521500002711,
0.));
#76149=CARTESIAN_POINT('Ctrl Pts',(-49.9873677385769,-52.3521500002711,
12.));
#76150=CARTESIAN_POINT('Ctrl Pts',(-49.9969687627402,-52.3749574789865,
0.));
#76151=CARTESIAN_POINT('Ctrl Pts',(-49.9969687627402,-52.3749574789865,
12.));
#76152=CARTESIAN_POINT('Ctrl Pts',(-50.0065636229934,-52.3978116592505,
0.));
#76153=CARTESIAN_POINT('Ctrl Pts',(-50.0065636229934,-52.3978116592505,
12.));
#76154=CARTESIAN_POINT('Ctrl Pts',(-50.0161522238619,-52.420712461261,0.));
#76155=CARTESIAN_POINT('Ctrl Pts',(-50.0161522238619,-52.420712461261,12.));
#76156=CARTESIAN_POINT('Ctrl Pts',(-50.0257344703008,-52.4436598054523,
0.));
#76157=CARTESIAN_POINT('Ctrl Pts',(-50.0257344703008,-52.4436598054523,
12.));
#76158=CARTESIAN_POINT('Ctrl Pts',(-50.0353102676933,-52.4666536124926,
0.));
#76159=CARTESIAN_POINT('Ctrl Pts',(-50.0353102676933,-52.4666536124926,
12.));
#76160=CARTESIAN_POINT('Ctrl Pts',(-50.0448795218453,-52.4896938032896,
0.));
#76161=CARTESIAN_POINT('Ctrl Pts',(-50.0448795218453,-52.4896938032896,
12.));
#76162=CARTESIAN_POINT('Ctrl Pts',(-50.0544421389824,-52.5127802989903,
0.));
#76163=CARTESIAN_POINT('Ctrl Pts',(-50.0544421389824,-52.5127802989903,
12.));
#76164=CARTESIAN_POINT('Ctrl Pts',(-50.0639980257477,-52.5359130209789,
0.));
#76165=CARTESIAN_POINT('Ctrl Pts',(-50.0639980257477,-52.5359130209789,
12.));
#76166=CARTESIAN_POINT('Ctrl Pts',(-50.0735470891996,-52.5590918908691,
0.));
#76167=CARTESIAN_POINT('Ctrl Pts',(-50.0735470891996,-52.5590918908691,
12.));
#76168=CARTESIAN_POINT('Ctrl Pts',(-50.0830892368095,-52.5823168304981,
0.));
#76169=CARTESIAN_POINT('Ctrl Pts',(-50.0830892368095,-52.5823168304981,
12.));
#76170=CARTESIAN_POINT('Ctrl Pts',(-50.0926243764569,-52.6055877619338,
0.));
#76171=CARTESIAN_POINT('Ctrl Pts',(-50.0926243764569,-52.6055877619338,
12.));
#76172=CARTESIAN_POINT('Ctrl Pts',(-50.1021524164261,-52.6289046074743,
0.));
#76173=CARTESIAN_POINT('Ctrl Pts',(-50.1021524164261,-52.6289046074743,
12.));
#76174=CARTESIAN_POINT('Ctrl Pts',(-50.1116732654041,-52.6522672896462,
0.));
#76175=CARTESIAN_POINT('Ctrl Pts',(-50.1116732654041,-52.6522672896462,
12.));
#76176=CARTESIAN_POINT('Ctrl Pts',(-50.1211868324781,-52.6756757311979,
0.));
#76177=CARTESIAN_POINT('Ctrl Pts',(-50.1211868324781,-52.6756757311979,
12.));
#76178=CARTESIAN_POINT('Ctrl Pts',(-50.1306930271343,-52.6991298550928,
0.));
#76179=CARTESIAN_POINT('Ctrl Pts',(-50.1306930271343,-52.6991298550928,
12.));
#76180=CARTESIAN_POINT('Ctrl Pts',(-50.1401917592532,-52.7226295845156,
0.));
#76181=CARTESIAN_POINT('Ctrl Pts',(-50.1401917592532,-52.7226295845156,
12.));
#76182=CARTESIAN_POINT('Ctrl Pts',(-50.1496829391068,-52.7461748428733,
0.));
#76183=CARTESIAN_POINT('Ctrl Pts',(-50.1496829391068,-52.7461748428733,
12.));
#76184=CARTESIAN_POINT('Ctrl Pts',(-50.1591664773561,-52.769765553794,0.));
#76185=CARTESIAN_POINT('Ctrl Pts',(-50.1591664773561,-52.769765553794,12.));
#76186=CARTESIAN_POINT('Ctrl Pts',(-50.1686422850493,-52.793401641121,0.));
#76187=CARTESIAN_POINT('Ctrl Pts',(-50.1686422850493,-52.793401641121,12.));
#76188=CARTESIAN_POINT('Ctrl Pts',(-50.1781102736215,-52.8170830289052,
0.));
#76189=CARTESIAN_POINT('Ctrl Pts',(-50.1781102736215,-52.8170830289052,
12.));
#76190=CARTESIAN_POINT('Ctrl Pts',(-50.1875703548893,-52.8408096414101,
0.));
#76191=CARTESIAN_POINT('Ctrl Pts',(-50.1875703548893,-52.8408096414101,
12.));
#76192=CARTESIAN_POINT('Ctrl Pts',(-50.1970224410476,-52.8645814031137,
0.));
#76193=CARTESIAN_POINT('Ctrl Pts',(-50.1970224410476,-52.8645814031137,
12.));
#76194=CARTESIAN_POINT('Ctrl Pts',(-50.2064664446663,-52.8883982387068,
0.));
#76195=CARTESIAN_POINT('Ctrl Pts',(-50.2064664446663,-52.8883982387068,
12.));
#76196=CARTESIAN_POINT('Ctrl Pts',(-50.2159022786876,-52.9122600730882,
0.));
#76197=CARTESIAN_POINT('Ctrl Pts',(-50.2159022786876,-52.9122600730882,
12.));
#76198=CARTESIAN_POINT('Ctrl Pts',(-50.2253298564237,-52.9361668313539,
0.));
#76199=CARTESIAN_POINT('Ctrl Pts',(-50.2253298564237,-52.9361668313539,
12.));
#76200=CARTESIAN_POINT('Ctrl Pts',(-50.2347490915553,-52.9601184388027,
0.));
#76201=CARTESIAN_POINT('Ctrl Pts',(-50.2347490915553,-52.9601184388027,
12.));
#76202=CARTESIAN_POINT('Ctrl Pts',(-50.2441598981286,-52.9841148209404,
0.));
#76203=CARTESIAN_POINT('Ctrl Pts',(-50.2441598981286,-52.9841148209404,
12.));
#76204=CARTESIAN_POINT('Ctrl Pts',(-50.2535621905553,-53.0081559034802,
0.));
#76205=CARTESIAN_POINT('Ctrl Pts',(-50.2535621905553,-53.0081559034802,
12.));
#76206=CARTESIAN_POINT('Ctrl Pts',(-50.262955883611,-53.0322416123404,0.));
#76207=CARTESIAN_POINT('Ctrl Pts',(-50.262955883611,-53.0322416123404,12.));
#76208=CARTESIAN_POINT('Ctrl Pts',(-50.272340892437,-53.0563718736361,0.));
#76209=CARTESIAN_POINT('Ctrl Pts',(-50.272340892437,-53.0563718736361,12.));
#76210=CARTESIAN_POINT('Ctrl Pts',(-50.2817171325354,-53.0805466136791,
0.));
#76211=CARTESIAN_POINT('Ctrl Pts',(-50.2817171325354,-53.0805466136791,
12.));
#76212=CARTESIAN_POINT('Ctrl Pts',(-50.2910845197615,-53.1047657589806,
0.));
#76213=CARTESIAN_POINT('Ctrl Pts',(-50.2910845197615,-53.1047657589806,
12.));
#76214=CARTESIAN_POINT('Ctrl Pts',(-50.3004429703188,-53.1290292362482,
0.));
#76215=CARTESIAN_POINT('Ctrl Pts',(-50.3004429703188,-53.1290292362482,
12.));
#76216=CARTESIAN_POINT('Ctrl Pts',(-50.3097924007536,-53.153336972382,0.));
#76217=CARTESIAN_POINT('Ctrl Pts',(-50.3097924007536,-53.153336972382,12.));
#76218=CARTESIAN_POINT('Ctrl Pts',(-50.3191327279497,-53.1776888944622,
0.));
#76219=CARTESIAN_POINT('Ctrl Pts',(-50.3191327279497,-53.1776888944622,
12.));
#76220=CARTESIAN_POINT('Ctrl Pts',(-50.3284638691285,-53.202084929748,0.));
#76221=CARTESIAN_POINT('Ctrl Pts',(-50.3284638691285,-53.202084929748,12.));
#76222=CARTESIAN_POINT('Ctrl Pts',(-50.3377857418522,-53.2265250056896,
0.));
#76223=CARTESIAN_POINT('Ctrl Pts',(-50.3377857418522,-53.2265250056896,
12.));
#76224=CARTESIAN_POINT('Ctrl Pts',(-50.3470982640294,-53.2510090499341,
0.));
#76225=CARTESIAN_POINT('Ctrl Pts',(-50.3470982640294,-53.2510090499341,
12.));
#76226=CARTESIAN_POINT('Ctrl Pts',(-50.3564013539198,-53.2755369903291,
0.));
#76227=CARTESIAN_POINT('Ctrl Pts',(-50.3564013539198,-53.2755369903291,
12.));
#76228=CARTESIAN_POINT('Ctrl Pts',(-50.3656949301424,-53.3001087549222,
0.));
#76229=CARTESIAN_POINT('Ctrl Pts',(-50.3656949301424,-53.3001087549222,
12.));
#76230=CARTESIAN_POINT('Ctrl Pts',(-50.3749789116777,-53.3247242719575,
0.));
#76231=CARTESIAN_POINT('Ctrl Pts',(-50.3749789116777,-53.3247242719575,
12.));
#76232=CARTESIAN_POINT('Ctrl Pts',(-50.3842532178451,-53.3493834698685,
0.));
#76233=CARTESIAN_POINT('Ctrl Pts',(-50.3842532178451,-53.3493834698685,
12.));
#76234=CARTESIAN_POINT('Ctrl Pts',(-50.393517768283,-53.3740862772673,0.));
#76235=CARTESIAN_POINT('Ctrl Pts',(-50.393517768283,-53.3740862772673,12.));
#76236=CARTESIAN_POINT('Ctrl Pts',(-50.4027724829296,-53.3988326229308,
0.));
#76237=CARTESIAN_POINT('Ctrl Pts',(-50.4027724829296,-53.3988326229308,
12.));
#76238=CARTESIAN_POINT('Ctrl Pts',(-50.4120172820054,-53.4236224357846,
0.));
#76239=CARTESIAN_POINT('Ctrl Pts',(-50.4120172820054,-53.4236224357846,
12.));
#76240=CARTESIAN_POINT('Ctrl Pts',(-50.4212520859924,-53.4484556448787,
0.));
#76241=CARTESIAN_POINT('Ctrl Pts',(-50.4212520859924,-53.4484556448787,
12.));
#76242=CARTESIAN_POINT('Ctrl Pts',(-50.4304768156677,-53.4733321794199,
0.));
#76243=CARTESIAN_POINT('Ctrl Pts',(-50.4304768156677,-53.4733321794199,
12.));
#76244=CARTESIAN_POINT('Ctrl Pts',(-50.4396913921389,-53.4982519688032,
0.));
#76245=CARTESIAN_POINT('Ctrl Pts',(-50.4396913921389,-53.4982519688032,
12.));
#76246=CARTESIAN_POINT('Ctrl Pts',(-50.4488957368841,-53.5232149426415,
0.));
#76247=CARTESIAN_POINT('Ctrl Pts',(-50.4488957368841,-53.5232149426415,
12.));
#76248=CARTESIAN_POINT('Ctrl Pts',(-50.4580897717835,-53.5482210307864,
0.));
#76249=CARTESIAN_POINT('Ctrl Pts',(-50.4580897717835,-53.5482210307864,
12.));
#76250=CARTESIAN_POINT('Ctrl Pts',(-50.467273419175,-53.5732701633603,0.));
#76251=CARTESIAN_POINT('Ctrl Pts',(-50.467273419175,-53.5732701633603,12.));
#76252=CARTESIAN_POINT('Ctrl Pts',(-50.4764466018064,-53.5983622707231,
0.));
#76253=CARTESIAN_POINT('Ctrl Pts',(-50.4764466018064,-53.5983622707231,
12.));
#76254=CARTESIAN_POINT('Ctrl Pts',(-50.485609242731,-53.6234972834055,0.));
#76255=CARTESIAN_POINT('Ctrl Pts',(-50.485609242731,-53.6234972834055,12.));
#76256=CARTESIAN_POINT('Ctrl Pts',(-50.4947612652147,-53.6486751320434,
0.));
#76257=CARTESIAN_POINT('Ctrl Pts',(-50.4947612652147,-53.6486751320434,
12.));
#76258=CARTESIAN_POINT('Ctrl Pts',(-50.5039025926531,-53.6738957473158,
0.));
#76259=CARTESIAN_POINT('Ctrl Pts',(-50.5039025926531,-53.6738957473158,
12.));
#76260=CARTESIAN_POINT('Ctrl Pts',(-50.5130331484563,-53.6991590598551,
0.));
#76261=CARTESIAN_POINT('Ctrl Pts',(-50.5130331484563,-53.6991590598551,
12.));
#76262=CARTESIAN_POINT('Ctrl Pts',(-50.5221528560427,-53.7244650002382,
0.));
#76263=CARTESIAN_POINT('Ctrl Pts',(-50.5221528560427,-53.7244650002382,
12.));
#76264=CARTESIAN_POINT('Ctrl Pts',(-50.5312616390789,-53.7498134991714,
0.));
#76265=CARTESIAN_POINT('Ctrl Pts',(-50.5312616390789,-53.7498134991714,
12.));
#76266=CARTESIAN_POINT('Ctrl Pts',(-50.5403594216706,-53.7752044876313,
0.));
#76267=CARTESIAN_POINT('Ctrl Pts',(-50.5403594216706,-53.7752044876313,
12.));
#76268=CARTESIAN_POINT('Ctrl Pts',(-50.5494461285762,-53.8006378970198,
0.));
#76269=CARTESIAN_POINT('Ctrl Pts',(-50.5494461285762,-53.8006378970198,
12.));
#76270=CARTESIAN_POINT('Ctrl Pts',(-50.5585216854082,-53.8261136593064,
0.));
#76271=CARTESIAN_POINT('Ctrl Pts',(-50.5585216854082,-53.8261136593064,
12.));
#76272=CARTESIAN_POINT('Ctrl Pts',(-50.567586018852,-53.8516317071783,0.));
#76273=CARTESIAN_POINT('Ctrl Pts',(-50.567586018852,-53.8516317071783,12.));
#76274=CARTESIAN_POINT('Ctrl Pts',(-50.5766390561861,-53.8771919737007,
0.));
#76275=CARTESIAN_POINT('Ctrl Pts',(-50.5766390561861,-53.8771919737007,
12.));
#76276=CARTESIAN_POINT('Ctrl Pts',(-50.5856807248133,-53.9027943919814,
0.));
#76277=CARTESIAN_POINT('Ctrl Pts',(-50.5856807248133,-53.9027943919814,
12.));
#76278=CARTESIAN_POINT('Ctrl Pts',(-50.5947109517476,-53.9284388947996,
0.));
#76279=CARTESIAN_POINT('Ctrl Pts',(-50.5947109517476,-53.9284388947996,
12.));
#76280=CARTESIAN_POINT('Ctrl Pts',(-50.603729663215,-53.9541254143131,0.));
#76281=CARTESIAN_POINT('Ctrl Pts',(-50.603729663215,-53.9541254143131,12.));
#76282=CARTESIAN_POINT('Ctrl Pts',(-50.6127367839738,-53.9798538815561,
0.));
#76283=CARTESIAN_POINT('Ctrl Pts',(-50.6127367839738,-53.9798538815561,
12.));
#76284=CARTESIAN_POINT('Ctrl Pts',(-50.6217322378686,-54.0056242268443,
0.));
#76285=CARTESIAN_POINT('Ctrl Pts',(-50.6217322378686,-54.0056242268443,
12.));
#76286=CARTESIAN_POINT('Ctrl Pts',(-50.630715949059,-54.0314363806751,0.));
#76287=CARTESIAN_POINT('Ctrl Pts',(-50.630715949059,-54.0314363806751,12.));
#76288=CARTESIAN_POINT('Ctrl Pts',(-50.6396878430961,-54.0572902745101,
0.));
#76289=CARTESIAN_POINT('Ctrl Pts',(-50.6396878430961,-54.0572902745101,
12.));
#76290=CARTESIAN_POINT('Ctrl Pts',(-50.6486478479459,-54.0831858415182,
0.));
#76291=CARTESIAN_POINT('Ctrl Pts',(-50.6486478479459,-54.0831858415182,
12.));
#76292=CARTESIAN_POINT('Ctrl Pts',(-50.657595895318,-54.1091230175319,0.));
#76293=CARTESIAN_POINT('Ctrl Pts',(-50.657595895318,-54.1091230175319,12.));
#76294=CARTESIAN_POINT('Ctrl Pts',(-50.6665319209798,-54.1351017412722,
0.));
#76295=CARTESIAN_POINT('Ctrl Pts',(-50.6665319209798,-54.1351017412722,
12.));
#76296=CARTESIAN_POINT('Ctrl Pts',(-50.6754558618218,-54.1611219522299,
0.));
#76297=CARTESIAN_POINT('Ctrl Pts',(-50.6754558618218,-54.1611219522299,
12.));
#76298=CARTESIAN_POINT('Ctrl Pts',(-50.6843676535428,-54.1871835889908,
0.));
#76299=CARTESIAN_POINT('Ctrl Pts',(-50.6843676535428,-54.1871835889908,
12.));
#76300=CARTESIAN_POINT('Ctrl Pts',(-50.6932672279758,-54.2132865872968,
0.));
#76301=CARTESIAN_POINT('Ctrl Pts',(-50.6932672279758,-54.2132865872968,
12.));
#76302=CARTESIAN_POINT('Ctrl Pts',(-50.7021545108369,-54.2394308784093,
0.));
#76303=CARTESIAN_POINT('Ctrl Pts',(-50.7021545108369,-54.2394308784093,
12.));
#76304=CARTESIAN_POINT('Ctrl Pts',(-50.7110294185832,-54.2656163868258,
0.));
#76305=CARTESIAN_POINT('Ctrl Pts',(-50.7110294185832,-54.2656163868258,
12.));
#76306=CARTESIAN_POINT('Ctrl Pts',(-50.7198918629632,-54.2918430335414,
0.));
#76307=CARTESIAN_POINT('Ctrl Pts',(-50.7198918629632,-54.2918430335414,
12.));
#76308=CARTESIAN_POINT('Ctrl Pts',(-50.7287417566296,-54.3181107400862,
0.));
#76309=CARTESIAN_POINT('Ctrl Pts',(-50.7287417566296,-54.3181107400862,
12.));
#76310=CARTESIAN_POINT('Ctrl Pts',(-50.7375790185988,-54.344419432416,0.));
#76311=CARTESIAN_POINT('Ctrl Pts',(-50.7375790185988,-54.344419432416,12.));
#76312=CARTESIAN_POINT('Ctrl Pts',(-50.7464035792846,-54.3707690445679,
0.));
#76313=CARTESIAN_POINT('Ctrl Pts',(-50.7464035792846,-54.3707690445679,
12.));
#76314=CARTESIAN_POINT('Ctrl Pts',(-50.7552153869224,-54.3971595231285,
0.));
#76315=CARTESIAN_POINT('Ctrl Pts',(-50.7552153869224,-54.3971595231285,
12.));
#76316=CARTESIAN_POINT('Ctrl Pts',(-50.7640144089601,-54.4235908287188,
0.));
#76317=CARTESIAN_POINT('Ctrl Pts',(-50.7640144089601,-54.4235908287188,
12.));
#76318=CARTESIAN_POINT('Ctrl Pts',(-50.772800626886,-54.4500629335867,0.));
#76319=CARTESIAN_POINT('Ctrl Pts',(-50.772800626886,-54.4500629335867,12.));
#76320=CARTESIAN_POINT('Ctrl Pts',(-50.7798193515479,-54.4712732428597,
0.));
#76321=CARTESIAN_POINT('Ctrl Pts',(-50.7798193515479,-54.4712732428597,
12.));
#76322=CARTESIAN_POINT('Ctrl Pts',(-50.7850776288567,-54.4871993224549,
0.));
#76323=CARTESIAN_POINT('Ctrl Pts',(-50.7850776288567,-54.4871993224549,
12.));
#76324=CARTESIAN_POINT('Ctrl Pts',(-50.7885805844191,-54.4978248630284,
0.));
#76325=CARTESIAN_POINT('Ctrl Pts',(-50.7885805844191,-54.4978248630284,
12.));
#76326=CARTESIAN_POINT('Ctrl Pts',(-50.7903314215393,-54.5031396718592,
0.));
#76327=CARTESIAN_POINT('Ctrl Pts',(-50.7903314215393,-54.5031396718592,
12.));
#76328=CARTESIAN_POINT('',(-48.8900464144686,-50.0975384783634,0.));
#76329=CARTESIAN_POINT('Ctrl Pts',(-48.8900464144686,-50.0975384783634,
0.));
#76330=CARTESIAN_POINT('Ctrl Pts',(-48.8919551910299,-50.1009206494209,
0.));
#76331=CARTESIAN_POINT('Ctrl Pts',(-48.8957735556681,-50.1076907555303,
0.));
#76332=CARTESIAN_POINT('Ctrl Pts',(-48.9015035371772,-50.1178632066821,
0.));
#76333=CARTESIAN_POINT('Ctrl Pts',(-48.9091483817797,-50.1314610602286,
0.));
#76334=CARTESIAN_POINT('Ctrl Pts',(-48.9187125417897,-50.148516018447,0.));
#76335=CARTESIAN_POINT('Ctrl Pts',(-48.9282847698237,-50.1656286003943,
0.));
#76336=CARTESIAN_POINT('Ctrl Pts',(-48.9378649933116,-50.1827987615659,
0.));
#76337=CARTESIAN_POINT('Ctrl Pts',(-48.9474530868847,-50.2000264157903,
0.));
#76338=CARTESIAN_POINT('Ctrl Pts',(-48.9570488741273,-50.2173114358423,
0.));
#76339=CARTESIAN_POINT('Ctrl Pts',(-48.9666521500969,-50.2346536715465,
0.));
#76340=CARTESIAN_POINT('Ctrl Pts',(-48.9762626987227,-50.252052963548,0.));
#76341=CARTESIAN_POINT('Ctrl Pts',(-48.9858803116649,-50.2695091583473,
0.));
#76342=CARTESIAN_POINT('Ctrl Pts',(-48.9955048082028,-50.2870221241003,
0.));
#76343=CARTESIAN_POINT('Ctrl Pts',(-49.0051360288002,-50.3045917455383,
0.));
#76344=CARTESIAN_POINT('Ctrl Pts',(-49.0147738256925,-50.3222179165102,
0.));
#76345=CARTESIAN_POINT('Ctrl Pts',(-49.0244180550759,-50.3399005337967,
0.));
#76346=CARTESIAN_POINT('Ctrl Pts',(-49.034068567401,-50.3576394894136,0.));
#76347=CARTESIAN_POINT('Ctrl Pts',(-49.0437252024868,-50.3754346667389,
0.));
#76348=CARTESIAN_POINT('Ctrl Pts',(-49.0533877945771,-50.393285944528,0.));
#76349=CARTESIAN_POINT('Ctrl Pts',(-49.0630561755082,-50.4111931994264,
0.));
#76350=CARTESIAN_POINT('Ctrl Pts',(-49.0727301783477,-50.4291563088528,
0.));
#76351=CARTESIAN_POINT('Ctrl Pts',(-49.0824096415339,-50.4471751542717,
0.));
#76352=CARTESIAN_POINT('Ctrl Pts',(-49.0920944086973,-50.465249621057,0.));
#76353=CARTESIAN_POINT('Ctrl Pts',(-49.1017843266782,-50.4833795969296,
0.));
#76354=CARTESIAN_POINT('Ctrl Pts',(-49.1114792441573,-50.5015649708742,
0.));
#76355=CARTESIAN_POINT('Ctrl Pts',(-49.1211790099817,-50.5198056318111,
0.));
#76356=CARTESIAN_POINT('Ctrl Pts',(-49.1308834717645,-50.5381014674822,
0.));
#76357=CARTESIAN_POINT('Ctrl Pts',(-49.1405924766169,-50.5564523650406,
0.));
#76358=CARTESIAN_POINT('Ctrl Pts',(-49.1503058717831,-50.5748582115575,
0.));
#76359=CARTESIAN_POINT('Ctrl Pts',(-49.1600235052613,-50.593318894516,0.));
#76360=CARTESIAN_POINT('Ctrl Pts',(-49.1697452265473,-50.6118343023937,
0.));
#76361=CARTESIAN_POINT('Ctrl Pts',(-49.1794708869074,-50.6304043248796,
0.));
#76362=CARTESIAN_POINT('Ctrl Pts',(-49.1892003389743,-50.6490288525639,
0.));
#76363=CARTESIAN_POINT('Ctrl Pts',(-49.1989334364992,-50.6677077767427,
0.));
#76364=CARTESIAN_POINT('Ctrl Pts',(-49.2086700340625,-50.6864409891905,
0.));
#76365=CARTESIAN_POINT('Ctrl Pts',(-49.218409986748,-50.7052283818941,0.));
#76366=CARTESIAN_POINT('Ctrl Pts',(-49.2281531501569,-50.7240698470698,
0.));
#76367=CARTESIAN_POINT('Ctrl Pts',(-49.2378993805482,-50.7429652772816,
0.));
#76368=CARTESIAN_POINT('Ctrl Pts',(-49.2476485349373,-50.7619145655207,
0.));
#76369=CARTESIAN_POINT('Ctrl Pts',(-49.2574004712122,-50.7809176052954,
0.));
#76370=CARTESIAN_POINT('Ctrl Pts',(-49.2671550482415,-50.7999742907111,
0.));
#76371=CARTESIAN_POINT('Ctrl Pts',(-49.2769121258144,-50.8190845164319,
0.));
#76372=CARTESIAN_POINT('Ctrl Pts',(-49.2866715645828,-50.8382481776392,
0.));
#76373=CARTESIAN_POINT('Ctrl Pts',(-49.2964332260043,-50.8574651699877,
0.));
#76374=CARTESIAN_POINT('Ctrl Pts',(-49.3061969722798,-50.8767353895509,
0.));
#76375=CARTESIAN_POINT('Ctrl Pts',(-49.3159626663129,-50.8960587327869,
0.));
#76376=CARTESIAN_POINT('Ctrl Pts',(-49.325730171735,-50.9154350965681,0.));
#76377=CARTESIAN_POINT('Ctrl Pts',(-49.3354993529163,-50.9348643781928,
0.));
#76378=CARTESIAN_POINT('Ctrl Pts',(-49.3452700749804,-50.9543464753974,
0.));
#76379=CARTESIAN_POINT('Ctrl Pts',(-49.3550422038221,-50.9738812863636,
0.));
#76380=CARTESIAN_POINT('Ctrl Pts',(-49.3648156061049,-50.9934687097179,
0.));
#76381=CARTESIAN_POINT('Ctrl Pts',(-49.3745901492429,-51.0131086445268,
0.));
#76382=CARTESIAN_POINT('Ctrl Pts',(-49.3843657013851,-51.0328009902857,
0.));
#76383=CARTESIAN_POINT('Ctrl Pts',(-49.3941421314014,-51.0525456469072,
0.));
#76384=CARTESIAN_POINT('Ctrl Pts',(-49.4039193088636,-51.0723425146987,
0.));
#76385=CARTESIAN_POINT('Ctrl Pts',(-49.4136971040428,-51.0921914943663,
0.));
#76386=CARTESIAN_POINT('Ctrl Pts',(-49.4234753879071,-51.1120924870196,
0.));
#76387=CARTESIAN_POINT('Ctrl Pts',(-49.4332540321178,-51.1320453941702,
0.));
#76388=CARTESIAN_POINT('Ctrl Pts',(-49.4430329090288,-51.1520501177291,
0.));
#76389=CARTESIAN_POINT('Ctrl Pts',(-49.4528118916833,-51.1721065599972,
0.));
#76390=CARTESIAN_POINT('Ctrl Pts',(-49.4625908538076,-51.1922146236686,
0.));
#76391=CARTESIAN_POINT('Ctrl Pts',(-49.4723696698022,-51.2123742118288,
0.));
#76392=CARTESIAN_POINT('Ctrl Pts',(-49.4821482147357,-51.2325852279507,
0.));
#76393=CARTESIAN_POINT('Ctrl Pts',(-49.4919263643357,-51.2528475758841,
0.));
#76394=CARTESIAN_POINT('Ctrl Pts',(-49.5017039949841,-51.2731611598465,
0.));
#76395=CARTESIAN_POINT('Ctrl Pts',(-49.5114809837111,-51.2935258844278,
0.));
#76396=CARTESIAN_POINT('Ctrl Pts',(-49.5212572081901,-51.3139416545903,
0.));
#76397=CARTESIAN_POINT('Ctrl Pts',(-49.5310325467334,-51.3344083756659,
0.));
#76398=CARTESIAN_POINT('Ctrl Pts',(-49.5408068782871,-51.354925953347,0.));
#76399=CARTESIAN_POINT('Ctrl Pts',(-49.5505800824268,-51.3754942936796,
0.));
#76400=CARTESIAN_POINT('Ctrl Pts',(-49.5603520393514,-51.3961133030688,
0.));
#76401=CARTESIAN_POINT('Ctrl Pts',(-49.5701226298779,-51.4167828882765,
0.));
#76402=CARTESIAN_POINT('Ctrl Pts',(-49.579891735436,-51.4375029564191,0.));
#76403=CARTESIAN_POINT('Ctrl Pts',(-49.5896592380634,-51.4582734149562,
0.));
#76404=CARTESIAN_POINT('Ctrl Pts',(-49.5994250204003,-51.4790941716859,
0.));
#76405=CARTESIAN_POINT('Ctrl Pts',(-49.609188965684,-51.4999651347496,0.));
#76406=CARTESIAN_POINT('Ctrl Pts',(-49.6189509577441,-51.5208862126303,
0.));
#76407=CARTESIAN_POINT('Ctrl Pts',(-49.6287108809975,-51.5418573141494,
0.));
#76408=CARTESIAN_POINT('Ctrl Pts',(-49.6384686204443,-51.5628783484556,
0.));
#76409=CARTESIAN_POINT('Ctrl Pts',(-49.6482240616627,-51.5839492250218,
0.));
#76410=CARTESIAN_POINT('Ctrl Pts',(-49.6579770908063,-51.6050698536525,
0.));
#76411=CARTESIAN_POINT('Ctrl Pts',(-49.6677275945975,-51.6262401444799,
0.));
#76412=CARTESIAN_POINT('Ctrl Pts',(-49.6774754603235,-51.6474600079611,
0.));
#76413=CARTESIAN_POINT('Ctrl Pts',(-49.6872205758314,-51.6687293548656,
0.));
#76414=CARTESIAN_POINT('Ctrl Pts',(-49.6969628295236,-51.6900480962744,
0.));
#76415=CARTESIAN_POINT('Ctrl Pts',(-49.7067021103534,-51.7114161435848,
0.));
#76416=CARTESIAN_POINT('Ctrl Pts',(-49.7164383078206,-51.7328334085084,
0.));
#76417=CARTESIAN_POINT('Ctrl Pts',(-49.7261713119672,-51.754299803068,0.));
#76418=CARTESIAN_POINT('Ctrl Pts',(-49.7359010133741,-51.7758152395857,
0.));
#76419=CARTESIAN_POINT('Ctrl Pts',(-49.7456273031555,-51.7973796306826,
0.));
#76420=CARTESIAN_POINT('Ctrl Pts',(-49.7553500729563,-51.8189928892841,
0.));
#76421=CARTESIAN_POINT('Ctrl Pts',(-49.7650692149464,-51.8406549286177,
0.));
#76422=CARTESIAN_POINT('Ctrl Pts',(-49.7747846218177,-51.8623656622092,
0.));
#76423=CARTESIAN_POINT('Ctrl Pts',(-49.78449618678,-51.8841250038716,0.));
#76424=CARTESIAN_POINT('Ctrl Pts',(-49.7942038035568,-51.9059328677051,
0.));
#76425=CARTESIAN_POINT('Ctrl Pts',(-49.8039073663808,-51.9277891681014,
0.));
#76426=CARTESIAN_POINT('Ctrl Pts',(-49.8136067699896,-51.9496938197418,
0.));
#76427=CARTESIAN_POINT('Ctrl Pts',(-49.8233019096224,-51.9716467375938,
0.));
#76428=CARTESIAN_POINT('Ctrl Pts',(-49.8329926810172,-51.9936478369008,
0.));
#76429=CARTESIAN_POINT('Ctrl Pts',(-49.8426789804068,-52.015697033182,0.));
#76430=CARTESIAN_POINT('Ctrl Pts',(-49.8523607045146,-52.0377942422373,
0.));
#76431=CARTESIAN_POINT('Ctrl Pts',(-49.8620377505498,-52.059939380145,0.));
#76432=CARTESIAN_POINT('Ctrl Pts',(-49.871710016205,-52.0821323632588,0.));
#76433=CARTESIAN_POINT('Ctrl Pts',(-49.8813773996523,-52.1043731081968,
0.));
#76434=CARTESIAN_POINT('Ctrl Pts',(-49.8910397995404,-52.1266615318414,
0.));
#76435=CARTESIAN_POINT('Ctrl Pts',(-49.90069711499,-52.1489975513449,0.));
#76436=CARTESIAN_POINT('Ctrl Pts',(-49.9103492455904,-52.1713810841277,
0.));
#76437=CARTESIAN_POINT('Ctrl Pts',(-49.919996091396,-52.1938120478752,0.));
#76438=CARTESIAN_POINT('Ctrl Pts',(-49.9296375529241,-52.2162903605272,
0.));
#76439=CARTESIAN_POINT('Ctrl Pts',(-49.9392735311507,-52.238815940277,0.));
#76440=CARTESIAN_POINT('Ctrl Pts',(-49.9489039275064,-52.2613887055773,
0.));
#76441=CARTESIAN_POINT('Ctrl Pts',(-49.9585286438734,-52.2840085751385,
0.));
#76442=CARTESIAN_POINT('Ctrl Pts',(-49.9681475825824,-52.3066754679265,
0.));
#76443=CARTESIAN_POINT('Ctrl Pts',(-49.9777606464103,-52.3293893031524,
0.));
#76444=CARTESIAN_POINT('Ctrl Pts',(-49.9873677385769,-52.3521500002711,
0.));
#76445=CARTESIAN_POINT('Ctrl Pts',(-49.9969687627402,-52.3749574789865,
0.));
#76446=CARTESIAN_POINT('Ctrl Pts',(-50.0065636229934,-52.3978116592505,
0.));
#76447=CARTESIAN_POINT('Ctrl Pts',(-50.0161522238619,-52.420712461261,0.));
#76448=CARTESIAN_POINT('Ctrl Pts',(-50.0257344703008,-52.4436598054523,
0.));
#76449=CARTESIAN_POINT('Ctrl Pts',(-50.0353102676933,-52.4666536124926,
0.));
#76450=CARTESIAN_POINT('Ctrl Pts',(-50.0448795218453,-52.4896938032896,
0.));
#76451=CARTESIAN_POINT('Ctrl Pts',(-50.0544421389824,-52.5127802989903,
0.));
#76452=CARTESIAN_POINT('Ctrl Pts',(-50.0639980257477,-52.5359130209789,
0.));
#76453=CARTESIAN_POINT('Ctrl Pts',(-50.0735470891996,-52.5590918908691,
0.));
#76454=CARTESIAN_POINT('Ctrl Pts',(-50.0830892368095,-52.5823168304981,
0.));
#76455=CARTESIAN_POINT('Ctrl Pts',(-50.0926243764569,-52.6055877619338,
0.));
#76456=CARTESIAN_POINT('Ctrl Pts',(-50.1021524164261,-52.6289046074743,
0.));
#76457=CARTESIAN_POINT('Ctrl Pts',(-50.1116732654041,-52.6522672896462,
0.));
#76458=CARTESIAN_POINT('Ctrl Pts',(-50.1211868324781,-52.6756757311979,
0.));
#76459=CARTESIAN_POINT('Ctrl Pts',(-50.1306930271343,-52.6991298550928,
0.));
#76460=CARTESIAN_POINT('Ctrl Pts',(-50.1401917592532,-52.7226295845156,
0.));
#76461=CARTESIAN_POINT('Ctrl Pts',(-50.1496829391068,-52.7461748428733,
0.));
#76462=CARTESIAN_POINT('Ctrl Pts',(-50.1591664773561,-52.769765553794,0.));
#76463=CARTESIAN_POINT('Ctrl Pts',(-50.1686422850493,-52.793401641121,0.));
#76464=CARTESIAN_POINT('Ctrl Pts',(-50.1781102736215,-52.8170830289052,
0.));
#76465=CARTESIAN_POINT('Ctrl Pts',(-50.1875703548893,-52.8408096414101,
0.));
#76466=CARTESIAN_POINT('Ctrl Pts',(-50.1970224410476,-52.8645814031137,
0.));
#76467=CARTESIAN_POINT('Ctrl Pts',(-50.2064664446663,-52.8883982387068,
0.));
#76468=CARTESIAN_POINT('Ctrl Pts',(-50.2159022786876,-52.9122600730882,
0.));
#76469=CARTESIAN_POINT('Ctrl Pts',(-50.2253298564237,-52.9361668313539,
0.));
#76470=CARTESIAN_POINT('Ctrl Pts',(-50.2347490915553,-52.9601184388027,
0.));
#76471=CARTESIAN_POINT('Ctrl Pts',(-50.2441598981286,-52.9841148209404,
0.));
#76472=CARTESIAN_POINT('Ctrl Pts',(-50.2535621905553,-53.0081559034802,
0.));
#76473=CARTESIAN_POINT('Ctrl Pts',(-50.262955883611,-53.0322416123404,0.));
#76474=CARTESIAN_POINT('Ctrl Pts',(-50.272340892437,-53.0563718736361,0.));
#76475=CARTESIAN_POINT('Ctrl Pts',(-50.2817171325354,-53.0805466136791,
0.));
#76476=CARTESIAN_POINT('Ctrl Pts',(-50.2910845197615,-53.1047657589806,
0.));
#76477=CARTESIAN_POINT('Ctrl Pts',(-50.3004429703188,-53.1290292362482,
0.));
#76478=CARTESIAN_POINT('Ctrl Pts',(-50.3097924007536,-53.153336972382,0.));
#76479=CARTESIAN_POINT('Ctrl Pts',(-50.3191327279497,-53.1776888944622,
0.));
#76480=CARTESIAN_POINT('Ctrl Pts',(-50.3284638691285,-53.202084929748,0.));
#76481=CARTESIAN_POINT('Ctrl Pts',(-50.3377857418522,-53.2265250056896,
0.));
#76482=CARTESIAN_POINT('Ctrl Pts',(-50.3470982640294,-53.2510090499341,
0.));
#76483=CARTESIAN_POINT('Ctrl Pts',(-50.3564013539198,-53.2755369903291,
0.));
#76484=CARTESIAN_POINT('Ctrl Pts',(-50.3656949301424,-53.3001087549222,
0.));
#76485=CARTESIAN_POINT('Ctrl Pts',(-50.3749789116777,-53.3247242719575,
0.));
#76486=CARTESIAN_POINT('Ctrl Pts',(-50.3842532178451,-53.3493834698685,
0.));
#76487=CARTESIAN_POINT('Ctrl Pts',(-50.393517768283,-53.3740862772673,0.));
#76488=CARTESIAN_POINT('Ctrl Pts',(-50.4027724829296,-53.3988326229308,
0.));
#76489=CARTESIAN_POINT('Ctrl Pts',(-50.4120172820054,-53.4236224357846,
0.));
#76490=CARTESIAN_POINT('Ctrl Pts',(-50.4212520859924,-53.4484556448787,
0.));
#76491=CARTESIAN_POINT('Ctrl Pts',(-50.4304768156677,-53.4733321794199,
0.));
#76492=CARTESIAN_POINT('Ctrl Pts',(-50.4396913921389,-53.4982519688032,
0.));
#76493=CARTESIAN_POINT('Ctrl Pts',(-50.4488957368841,-53.5232149426415,
0.));
#76494=CARTESIAN_POINT('Ctrl Pts',(-50.4580897717835,-53.5482210307864,
0.));
#76495=CARTESIAN_POINT('Ctrl Pts',(-50.467273419175,-53.5732701633603,0.));
#76496=CARTESIAN_POINT('Ctrl Pts',(-50.4764466018064,-53.5983622707231,
0.));
#76497=CARTESIAN_POINT('Ctrl Pts',(-50.485609242731,-53.6234972834055,0.));
#76498=CARTESIAN_POINT('Ctrl Pts',(-50.4947612652147,-53.6486751320434,
0.));
#76499=CARTESIAN_POINT('Ctrl Pts',(-50.5039025926531,-53.6738957473158,
0.));
#76500=CARTESIAN_POINT('Ctrl Pts',(-50.5130331484563,-53.6991590598551,
0.));
#76501=CARTESIAN_POINT('Ctrl Pts',(-50.5221528560427,-53.7244650002382,
0.));
#76502=CARTESIAN_POINT('Ctrl Pts',(-50.5312616390789,-53.7498134991714,
0.));
#76503=CARTESIAN_POINT('Ctrl Pts',(-50.5403594216706,-53.7752044876313,
0.));
#76504=CARTESIAN_POINT('Ctrl Pts',(-50.5494461285762,-53.8006378970198,
0.));
#76505=CARTESIAN_POINT('Ctrl Pts',(-50.5585216854082,-53.8261136593064,
0.));
#76506=CARTESIAN_POINT('Ctrl Pts',(-50.567586018852,-53.8516317071783,0.));
#76507=CARTESIAN_POINT('Ctrl Pts',(-50.5766390561861,-53.8771919737007,
0.));
#76508=CARTESIAN_POINT('Ctrl Pts',(-50.5856807248133,-53.9027943919814,
0.));
#76509=CARTESIAN_POINT('Ctrl Pts',(-50.5947109517476,-53.9284388947996,
0.));
#76510=CARTESIAN_POINT('Ctrl Pts',(-50.603729663215,-53.9541254143131,0.));
#76511=CARTESIAN_POINT('Ctrl Pts',(-50.6127367839738,-53.9798538815561,
0.));
#76512=CARTESIAN_POINT('Ctrl Pts',(-50.6217322378686,-54.0056242268443,
0.));
#76513=CARTESIAN_POINT('Ctrl Pts',(-50.630715949059,-54.0314363806751,0.));
#76514=CARTESIAN_POINT('Ctrl Pts',(-50.6396878430961,-54.0572902745101,
0.));
#76515=CARTESIAN_POINT('Ctrl Pts',(-50.6486478479459,-54.0831858415182,
0.));
#76516=CARTESIAN_POINT('Ctrl Pts',(-50.657595895318,-54.1091230175319,0.));
#76517=CARTESIAN_POINT('Ctrl Pts',(-50.6665319209798,-54.1351017412722,
0.));
#76518=CARTESIAN_POINT('Ctrl Pts',(-50.6741814675382,-54.1574061041881,
0.));
#76519=CARTESIAN_POINT('Ctrl Pts',(-50.6800396668659,-54.1745287898576,
0.));
#76520=CARTESIAN_POINT('Ctrl Pts',(-50.6841118861802,-54.1864514381923,
0.));
#76521=CARTESIAN_POINT('Ctrl Pts',(-50.6864016965602,-54.1931619277294,
0.));
#76522=CARTESIAN_POINT('Ctrl Pts',(-50.6869108458688,-54.1946543499977,
0.));
#76523=CARTESIAN_POINT('',(-48.8900464144686,-50.0975384783634,12.));
#76524=CARTESIAN_POINT('',(-48.8900464144686,-50.0975384783634,0.));
#76525=CARTESIAN_POINT('Ctrl Pts',(-50.6869108458688,-54.1946543499976,
12.));
#76526=CARTESIAN_POINT('Ctrl Pts',(-50.6864016965602,-54.1931619277293,
12.));
#76527=CARTESIAN_POINT('Ctrl Pts',(-50.6841118861802,-54.1864514381923,
12.));
#76528=CARTESIAN_POINT('Ctrl Pts',(-50.6800396668659,-54.1745287898576,
12.));
#76529=CARTESIAN_POINT('Ctrl Pts',(-50.6741814675382,-54.1574061041882,
12.));
#76530=CARTESIAN_POINT('Ctrl Pts',(-50.6665319209798,-54.1351017412722,
12.));
#76531=CARTESIAN_POINT('Ctrl Pts',(-50.657595895318,-54.1091230175319,12.));
#76532=CARTESIAN_POINT('Ctrl Pts',(-50.6486478479459,-54.0831858415182,
12.));
#76533=CARTESIAN_POINT('Ctrl Pts',(-50.6396878430961,-54.0572902745101,
12.));
#76534=CARTESIAN_POINT('Ctrl Pts',(-50.630715949059,-54.0314363806751,12.));
#76535=CARTESIAN_POINT('Ctrl Pts',(-50.6217322378686,-54.0056242268443,
12.));
#76536=CARTESIAN_POINT('Ctrl Pts',(-50.6127367839738,-53.9798538815561,
12.));
#76537=CARTESIAN_POINT('Ctrl Pts',(-50.603729663215,-53.9541254143131,12.));
#76538=CARTESIAN_POINT('Ctrl Pts',(-50.5947109517476,-53.9284388947996,
12.));
#76539=CARTESIAN_POINT('Ctrl Pts',(-50.5856807248133,-53.9027943919814,
12.));
#76540=CARTESIAN_POINT('Ctrl Pts',(-50.5766390561861,-53.8771919737007,
12.));
#76541=CARTESIAN_POINT('Ctrl Pts',(-50.567586018852,-53.8516317071783,12.));
#76542=CARTESIAN_POINT('Ctrl Pts',(-50.5585216854082,-53.8261136593064,
12.));
#76543=CARTESIAN_POINT('Ctrl Pts',(-50.5494461285762,-53.8006378970198,
12.));
#76544=CARTESIAN_POINT('Ctrl Pts',(-50.5403594216706,-53.7752044876313,
12.));
#76545=CARTESIAN_POINT('Ctrl Pts',(-50.5312616390789,-53.7498134991714,
12.));
#76546=CARTESIAN_POINT('Ctrl Pts',(-50.5221528560427,-53.7244650002382,
12.));
#76547=CARTESIAN_POINT('Ctrl Pts',(-50.5130331484563,-53.6991590598551,
12.));
#76548=CARTESIAN_POINT('Ctrl Pts',(-50.5039025926531,-53.6738957473158,
12.));
#76549=CARTESIAN_POINT('Ctrl Pts',(-50.4947612652147,-53.6486751320434,
12.));
#76550=CARTESIAN_POINT('Ctrl Pts',(-50.485609242731,-53.6234972834055,12.));
#76551=CARTESIAN_POINT('Ctrl Pts',(-50.4764466018064,-53.5983622707231,
12.));
#76552=CARTESIAN_POINT('Ctrl Pts',(-50.467273419175,-53.5732701633603,12.));
#76553=CARTESIAN_POINT('Ctrl Pts',(-50.4580897717835,-53.5482210307864,
12.));
#76554=CARTESIAN_POINT('Ctrl Pts',(-50.4488957368841,-53.5232149426415,
12.));
#76555=CARTESIAN_POINT('Ctrl Pts',(-50.4396913921389,-53.4982519688032,
12.));
#76556=CARTESIAN_POINT('Ctrl Pts',(-50.4304768156677,-53.4733321794199,
12.));
#76557=CARTESIAN_POINT('Ctrl Pts',(-50.4212520859924,-53.4484556448787,
12.));
#76558=CARTESIAN_POINT('Ctrl Pts',(-50.4120172820054,-53.4236224357846,
12.));
#76559=CARTESIAN_POINT('Ctrl Pts',(-50.4027724829296,-53.3988326229308,
12.));
#76560=CARTESIAN_POINT('Ctrl Pts',(-50.393517768283,-53.3740862772673,12.));
#76561=CARTESIAN_POINT('Ctrl Pts',(-50.3842532178451,-53.3493834698685,
12.));
#76562=CARTESIAN_POINT('Ctrl Pts',(-50.3749789116777,-53.3247242719575,
12.));
#76563=CARTESIAN_POINT('Ctrl Pts',(-50.3656949301424,-53.3001087549222,
12.));
#76564=CARTESIAN_POINT('Ctrl Pts',(-50.3564013539198,-53.2755369903291,
12.));
#76565=CARTESIAN_POINT('Ctrl Pts',(-50.3470982640294,-53.2510090499341,
12.));
#76566=CARTESIAN_POINT('Ctrl Pts',(-50.3377857418522,-53.2265250056896,
12.));
#76567=CARTESIAN_POINT('Ctrl Pts',(-50.3284638691285,-53.202084929748,12.));
#76568=CARTESIAN_POINT('Ctrl Pts',(-50.3191327279497,-53.1776888944622,
12.));
#76569=CARTESIAN_POINT('Ctrl Pts',(-50.3097924007536,-53.153336972382,12.));
#76570=CARTESIAN_POINT('Ctrl Pts',(-50.3004429703188,-53.1290292362482,
12.));
#76571=CARTESIAN_POINT('Ctrl Pts',(-50.2910845197615,-53.1047657589806,
12.));
#76572=CARTESIAN_POINT('Ctrl Pts',(-50.2817171325354,-53.0805466136791,
12.));
#76573=CARTESIAN_POINT('Ctrl Pts',(-50.272340892437,-53.0563718736361,12.));
#76574=CARTESIAN_POINT('Ctrl Pts',(-50.262955883611,-53.0322416123404,12.));
#76575=CARTESIAN_POINT('Ctrl Pts',(-50.2535621905553,-53.0081559034802,
12.));
#76576=CARTESIAN_POINT('Ctrl Pts',(-50.2441598981286,-52.9841148209404,
12.));
#76577=CARTESIAN_POINT('Ctrl Pts',(-50.2347490915553,-52.9601184388027,
12.));
#76578=CARTESIAN_POINT('Ctrl Pts',(-50.2253298564237,-52.9361668313539,
12.));
#76579=CARTESIAN_POINT('Ctrl Pts',(-50.2159022786876,-52.9122600730882,
12.));
#76580=CARTESIAN_POINT('Ctrl Pts',(-50.2064664446663,-52.8883982387068,
12.));
#76581=CARTESIAN_POINT('Ctrl Pts',(-50.1970224410476,-52.8645814031137,
12.));
#76582=CARTESIAN_POINT('Ctrl Pts',(-50.1875703548893,-52.8408096414101,
12.));
#76583=CARTESIAN_POINT('Ctrl Pts',(-50.1781102736215,-52.8170830289052,
12.));
#76584=CARTESIAN_POINT('Ctrl Pts',(-50.1686422850493,-52.793401641121,12.));
#76585=CARTESIAN_POINT('Ctrl Pts',(-50.1591664773561,-52.769765553794,12.));
#76586=CARTESIAN_POINT('Ctrl Pts',(-50.1496829391068,-52.7461748428733,
12.));
#76587=CARTESIAN_POINT('Ctrl Pts',(-50.1401917592532,-52.7226295845156,
12.));
#76588=CARTESIAN_POINT('Ctrl Pts',(-50.1306930271343,-52.6991298550928,
12.));
#76589=CARTESIAN_POINT('Ctrl Pts',(-50.1211868324781,-52.6756757311979,
12.));
#76590=CARTESIAN_POINT('Ctrl Pts',(-50.1116732654041,-52.6522672896462,
12.));
#76591=CARTESIAN_POINT('Ctrl Pts',(-50.1021524164261,-52.6289046074743,
12.));
#76592=CARTESIAN_POINT('Ctrl Pts',(-50.0926243764569,-52.6055877619338,
12.));
#76593=CARTESIAN_POINT('Ctrl Pts',(-50.0830892368095,-52.5823168304981,
12.));
#76594=CARTESIAN_POINT('Ctrl Pts',(-50.0735470891996,-52.5590918908691,
12.));
#76595=CARTESIAN_POINT('Ctrl Pts',(-50.0639980257477,-52.5359130209789,
12.));
#76596=CARTESIAN_POINT('Ctrl Pts',(-50.0544421389824,-52.5127802989903,
12.));
#76597=CARTESIAN_POINT('Ctrl Pts',(-50.0448795218453,-52.4896938032896,
12.));
#76598=CARTESIAN_POINT('Ctrl Pts',(-50.0353102676933,-52.4666536124926,
12.));
#76599=CARTESIAN_POINT('Ctrl Pts',(-50.0257344703008,-52.4436598054523,
12.));
#76600=CARTESIAN_POINT('Ctrl Pts',(-50.0161522238619,-52.420712461261,12.));
#76601=CARTESIAN_POINT('Ctrl Pts',(-50.0065636229934,-52.3978116592505,
12.));
#76602=CARTESIAN_POINT('Ctrl Pts',(-49.9969687627402,-52.3749574789865,
12.));
#76603=CARTESIAN_POINT('Ctrl Pts',(-49.9873677385769,-52.3521500002711,
12.));
#76604=CARTESIAN_POINT('Ctrl Pts',(-49.9777606464103,-52.3293893031524,
12.));
#76605=CARTESIAN_POINT('Ctrl Pts',(-49.9681475825824,-52.3066754679265,
12.));
#76606=CARTESIAN_POINT('Ctrl Pts',(-49.9585286438734,-52.2840085751385,
12.));
#76607=CARTESIAN_POINT('Ctrl Pts',(-49.9489039275064,-52.2613887055773,
12.));
#76608=CARTESIAN_POINT('Ctrl Pts',(-49.9392735311507,-52.238815940277,12.));
#76609=CARTESIAN_POINT('Ctrl Pts',(-49.9296375529241,-52.2162903605272,
12.));
#76610=CARTESIAN_POINT('Ctrl Pts',(-49.919996091396,-52.1938120478752,12.));
#76611=CARTESIAN_POINT('Ctrl Pts',(-49.9103492455904,-52.1713810841277,
12.));
#76612=CARTESIAN_POINT('Ctrl Pts',(-49.90069711499,-52.1489975513449,12.));
#76613=CARTESIAN_POINT('Ctrl Pts',(-49.8910397995404,-52.1266615318414,
12.));
#76614=CARTESIAN_POINT('Ctrl Pts',(-49.8813773996523,-52.1043731081968,
12.));
#76615=CARTESIAN_POINT('Ctrl Pts',(-49.871710016205,-52.0821323632588,12.));
#76616=CARTESIAN_POINT('Ctrl Pts',(-49.8620377505498,-52.059939380145,12.));
#76617=CARTESIAN_POINT('Ctrl Pts',(-49.8523607045146,-52.0377942422373,
12.));
#76618=CARTESIAN_POINT('Ctrl Pts',(-49.8426789804068,-52.015697033182,12.));
#76619=CARTESIAN_POINT('Ctrl Pts',(-49.8329926810172,-51.9936478369008,
12.));
#76620=CARTESIAN_POINT('Ctrl Pts',(-49.8233019096224,-51.9716467375938,
12.));
#76621=CARTESIAN_POINT('Ctrl Pts',(-49.8136067699896,-51.9496938197418,
12.));
#76622=CARTESIAN_POINT('Ctrl Pts',(-49.8039073663808,-51.9277891681014,
12.));
#76623=CARTESIAN_POINT('Ctrl Pts',(-49.7942038035568,-51.9059328677051,
12.));
#76624=CARTESIAN_POINT('Ctrl Pts',(-49.78449618678,-51.8841250038716,12.));
#76625=CARTESIAN_POINT('Ctrl Pts',(-49.7747846218177,-51.8623656622092,
12.));
#76626=CARTESIAN_POINT('Ctrl Pts',(-49.7650692149464,-51.8406549286177,
12.));
#76627=CARTESIAN_POINT('Ctrl Pts',(-49.7553500729563,-51.8189928892841,
12.));
#76628=CARTESIAN_POINT('Ctrl Pts',(-49.7456273031555,-51.7973796306826,
12.));
#76629=CARTESIAN_POINT('Ctrl Pts',(-49.7359010133741,-51.7758152395857,
12.));
#76630=CARTESIAN_POINT('Ctrl Pts',(-49.7261713119672,-51.754299803068,12.));
#76631=CARTESIAN_POINT('Ctrl Pts',(-49.7164383078206,-51.7328334085084,
12.));
#76632=CARTESIAN_POINT('Ctrl Pts',(-49.7067021103534,-51.7114161435848,
12.));
#76633=CARTESIAN_POINT('Ctrl Pts',(-49.6969628295236,-51.6900480962744,
12.));
#76634=CARTESIAN_POINT('Ctrl Pts',(-49.6872205758314,-51.6687293548656,
12.));
#76635=CARTESIAN_POINT('Ctrl Pts',(-49.6774754603235,-51.6474600079611,
12.));
#76636=CARTESIAN_POINT('Ctrl Pts',(-49.6677275945975,-51.6262401444799,
12.));
#76637=CARTESIAN_POINT('Ctrl Pts',(-49.6579770908063,-51.6050698536525,
12.));
#76638=CARTESIAN_POINT('Ctrl Pts',(-49.6482240616627,-51.5839492250218,
12.));
#76639=CARTESIAN_POINT('Ctrl Pts',(-49.6384686204443,-51.5628783484556,
12.));
#76640=CARTESIAN_POINT('Ctrl Pts',(-49.6287108809975,-51.5418573141494,
12.));
#76641=CARTESIAN_POINT('Ctrl Pts',(-49.6189509577441,-51.5208862126303,
12.));
#76642=CARTESIAN_POINT('Ctrl Pts',(-49.609188965684,-51.4999651347496,12.));
#76643=CARTESIAN_POINT('Ctrl Pts',(-49.5994250204003,-51.4790941716859,
12.));
#76644=CARTESIAN_POINT('Ctrl Pts',(-49.5896592380634,-51.4582734149562,
12.));
#76645=CARTESIAN_POINT('Ctrl Pts',(-49.579891735436,-51.4375029564191,12.));
#76646=CARTESIAN_POINT('Ctrl Pts',(-49.5701226298779,-51.4167828882765,
12.));
#76647=CARTESIAN_POINT('Ctrl Pts',(-49.5603520393514,-51.3961133030688,
12.));
#76648=CARTESIAN_POINT('Ctrl Pts',(-49.5505800824268,-51.3754942936796,
12.));
#76649=CARTESIAN_POINT('Ctrl Pts',(-49.5408068782871,-51.354925953347,12.));
#76650=CARTESIAN_POINT('Ctrl Pts',(-49.5310325467334,-51.3344083756659,
12.));
#76651=CARTESIAN_POINT('Ctrl Pts',(-49.5212572081901,-51.3139416545903,
12.));
#76652=CARTESIAN_POINT('Ctrl Pts',(-49.5114809837111,-51.2935258844278,
12.));
#76653=CARTESIAN_POINT('Ctrl Pts',(-49.5017039949841,-51.2731611598465,
12.));
#76654=CARTESIAN_POINT('Ctrl Pts',(-49.4919263643357,-51.2528475758841,
12.));
#76655=CARTESIAN_POINT('Ctrl Pts',(-49.4821482147357,-51.2325852279507,
12.));
#76656=CARTESIAN_POINT('Ctrl Pts',(-49.4723696698022,-51.2123742118288,
12.));
#76657=CARTESIAN_POINT('Ctrl Pts',(-49.4625908538076,-51.1922146236686,
12.));
#76658=CARTESIAN_POINT('Ctrl Pts',(-49.4528118916833,-51.1721065599972,
12.));
#76659=CARTESIAN_POINT('Ctrl Pts',(-49.4430329090288,-51.1520501177291,
12.));
#76660=CARTESIAN_POINT('Ctrl Pts',(-49.4332540321178,-51.1320453941702,
12.));
#76661=CARTESIAN_POINT('Ctrl Pts',(-49.4234753879071,-51.1120924870196,
12.));
#76662=CARTESIAN_POINT('Ctrl Pts',(-49.4136971040428,-51.0921914943663,
12.));
#76663=CARTESIAN_POINT('Ctrl Pts',(-49.4039193088636,-51.0723425146987,
12.));
#76664=CARTESIAN_POINT('Ctrl Pts',(-49.3941421314014,-51.0525456469072,
12.));
#76665=CARTESIAN_POINT('Ctrl Pts',(-49.3843657013851,-51.0328009902857,
12.));
#76666=CARTESIAN_POINT('Ctrl Pts',(-49.3745901492429,-51.0131086445268,
12.));
#76667=CARTESIAN_POINT('Ctrl Pts',(-49.3648156061049,-50.9934687097179,
12.));
#76668=CARTESIAN_POINT('Ctrl Pts',(-49.3550422038221,-50.9738812863636,
12.));
#76669=CARTESIAN_POINT('Ctrl Pts',(-49.3452700749804,-50.9543464753974,
12.));
#76670=CARTESIAN_POINT('Ctrl Pts',(-49.3354993529163,-50.9348643781928,
12.));
#76671=CARTESIAN_POINT('Ctrl Pts',(-49.325730171735,-50.9154350965681,12.));
#76672=CARTESIAN_POINT('Ctrl Pts',(-49.3159626663129,-50.8960587327869,
12.));
#76673=CARTESIAN_POINT('Ctrl Pts',(-49.3061969722798,-50.8767353895509,
12.));
#76674=CARTESIAN_POINT('Ctrl Pts',(-49.2964332260043,-50.8574651699877,
12.));
#76675=CARTESIAN_POINT('Ctrl Pts',(-49.2866715645828,-50.8382481776392,
12.));
#76676=CARTESIAN_POINT('Ctrl Pts',(-49.2769121258144,-50.8190845164319,
12.));
#76677=CARTESIAN_POINT('Ctrl Pts',(-49.2671550482415,-50.7999742907111,
12.));
#76678=CARTESIAN_POINT('Ctrl Pts',(-49.2574004712122,-50.7809176052954,
12.));
#76679=CARTESIAN_POINT('Ctrl Pts',(-49.2476485349373,-50.7619145655207,
12.));
#76680=CARTESIAN_POINT('Ctrl Pts',(-49.2378993805482,-50.7429652772816,
12.));
#76681=CARTESIAN_POINT('Ctrl Pts',(-49.2281531501569,-50.7240698470698,
12.));
#76682=CARTESIAN_POINT('Ctrl Pts',(-49.218409986748,-50.7052283818941,12.));
#76683=CARTESIAN_POINT('Ctrl Pts',(-49.2086700340625,-50.6864409891905,
12.));
#76684=CARTESIAN_POINT('Ctrl Pts',(-49.1989334364992,-50.6677077767427,
12.));
#76685=CARTESIAN_POINT('Ctrl Pts',(-49.1892003389743,-50.6490288525639,
12.));
#76686=CARTESIAN_POINT('Ctrl Pts',(-49.1794708869074,-50.6304043248796,
12.));
#76687=CARTESIAN_POINT('Ctrl Pts',(-49.1697452265473,-50.6118343023937,
12.));
#76688=CARTESIAN_POINT('Ctrl Pts',(-49.1600235052613,-50.593318894516,12.));
#76689=CARTESIAN_POINT('Ctrl Pts',(-49.1503058717831,-50.5748582115575,
12.));
#76690=CARTESIAN_POINT('Ctrl Pts',(-49.1405924766169,-50.5564523650406,
12.));
#76691=CARTESIAN_POINT('Ctrl Pts',(-49.1308834717645,-50.5381014674822,
12.));
#76692=CARTESIAN_POINT('Ctrl Pts',(-49.1211790099817,-50.5198056318111,
12.));
#76693=CARTESIAN_POINT('Ctrl Pts',(-49.1114792441573,-50.5015649708742,
12.));
#76694=CARTESIAN_POINT('Ctrl Pts',(-49.1017843266782,-50.4833795969296,
12.));
#76695=CARTESIAN_POINT('Ctrl Pts',(-49.0920944086973,-50.465249621057,12.));
#76696=CARTESIAN_POINT('Ctrl Pts',(-49.0824096415339,-50.4471751542717,
12.));
#76697=CARTESIAN_POINT('Ctrl Pts',(-49.0727301783477,-50.4291563088528,
12.));
#76698=CARTESIAN_POINT('Ctrl Pts',(-49.0630561755082,-50.4111931994264,
12.));
#76699=CARTESIAN_POINT('Ctrl Pts',(-49.0533877945771,-50.393285944528,12.));
#76700=CARTESIAN_POINT('Ctrl Pts',(-49.0437252024868,-50.3754346667389,
12.));
#76701=CARTESIAN_POINT('Ctrl Pts',(-49.034068567401,-50.3576394894136,12.));
#76702=CARTESIAN_POINT('Ctrl Pts',(-49.0244180550759,-50.3399005337967,
12.));
#76703=CARTESIAN_POINT('Ctrl Pts',(-49.0147738256925,-50.3222179165102,
12.));
#76704=CARTESIAN_POINT('Ctrl Pts',(-49.0051360288002,-50.3045917455383,
12.));
#76705=CARTESIAN_POINT('Ctrl Pts',(-48.9955048082028,-50.2870221241003,
12.));
#76706=CARTESIAN_POINT('Ctrl Pts',(-48.9858803116649,-50.2695091583473,
12.));
#76707=CARTESIAN_POINT('Ctrl Pts',(-48.9762626987227,-50.252052963548,12.));
#76708=CARTESIAN_POINT('Ctrl Pts',(-48.9666521500969,-50.2346536715465,
12.));
#76709=CARTESIAN_POINT('Ctrl Pts',(-48.9570488741273,-50.2173114358423,
12.));
#76710=CARTESIAN_POINT('Ctrl Pts',(-48.9474530868847,-50.2000264157903,
12.));
#76711=CARTESIAN_POINT('Ctrl Pts',(-48.9378649933116,-50.1827987615659,
12.));
#76712=CARTESIAN_POINT('Ctrl Pts',(-48.9282847698237,-50.1656286003943,
12.));
#76713=CARTESIAN_POINT('Ctrl Pts',(-48.9187125417897,-50.148516018447,12.));
#76714=CARTESIAN_POINT('Ctrl Pts',(-48.9091483817797,-50.1314610602286,
12.));
#76715=CARTESIAN_POINT('Ctrl Pts',(-48.9015035371772,-50.1178632066821,
12.));
#76716=CARTESIAN_POINT('Ctrl Pts',(-48.8957735556681,-50.1076907555303,
12.));
#76717=CARTESIAN_POINT('Ctrl Pts',(-48.8919551910299,-50.1009206494209,
12.));
#76718=CARTESIAN_POINT('Ctrl Pts',(-48.8900464144686,-50.0975384783634,
12.));
#76719=CARTESIAN_POINT('Ctrl Pts',(-49.5707719660638,-55.2174072001495,
0.));
#76720=CARTESIAN_POINT('Ctrl Pts',(-49.5707719660638,-55.2174072001495,
4.));
#76721=CARTESIAN_POINT('Ctrl Pts',(-49.5707719660638,-55.2174072001495,
8.));
#76722=CARTESIAN_POINT('Ctrl Pts',(-49.5707719660638,-55.2174072001495,
12.));
#76723=CARTESIAN_POINT('Ctrl Pts',(-49.6712810246932,-55.2618153697169,
0.));
#76724=CARTESIAN_POINT('Ctrl Pts',(-49.6712810246932,-55.2618153697169,
4.));
#76725=CARTESIAN_POINT('Ctrl Pts',(-49.6712810246932,-55.2618153697169,
8.));
#76726=CARTESIAN_POINT('Ctrl Pts',(-49.6712810246932,-55.2618153697169,
12.));
#76727=CARTESIAN_POINT('Ctrl Pts',(-49.8732090625341,-55.2790667815473,
0.));
#76728=CARTESIAN_POINT('Ctrl Pts',(-49.8732090625341,-55.2790667815473,
4.));
#76729=CARTESIAN_POINT('Ctrl Pts',(-49.8732090625341,-55.2790667815473,
7.99999999999999));
#76730=CARTESIAN_POINT('Ctrl Pts',(-49.8732090625341,-55.2790667815473,
12.));
#76731=CARTESIAN_POINT('Ctrl Pts',(-50.0481613529516,-55.1854902750885,
0.));
#76732=CARTESIAN_POINT('Ctrl Pts',(-50.0481613529516,-55.1854902750885,
4.));
#76733=CARTESIAN_POINT('Ctrl Pts',(-50.0481613529516,-55.1854902750885,
8.00000000000001));
#76734=CARTESIAN_POINT('Ctrl Pts',(-50.0481613529516,-55.1854902750885,
12.));
#76735=CARTESIAN_POINT('Ctrl Pts',(-50.1091461876225,-55.1300595714123,
0.));
#76736=CARTESIAN_POINT('Ctrl Pts',(-50.1091461876225,-55.1300595714123,
4.));
#76737=CARTESIAN_POINT('Ctrl Pts',(-50.1091461876225,-55.1300595714123,
8.));
#76738=CARTESIAN_POINT('Ctrl Pts',(-50.1091461876225,-55.1300595714123,
12.));
#76739=CARTESIAN_POINT('',(-49.5707719660638,-55.2174072001495,0.));
#76740=CARTESIAN_POINT('',(-50.1091461876226,-55.1300595714123,0.));
#76741=CARTESIAN_POINT('Ctrl Pts',(-49.5707719660638,-55.2174072001495,
2.77555756156289E-16));
#76742=CARTESIAN_POINT('Ctrl Pts',(-49.6712810246932,-55.2618153697169,
2.77555756156289E-16));
#76743=CARTESIAN_POINT('Ctrl Pts',(-49.786668474888,-55.2716733193343,2.77555756156289E-16));
#76744=CARTESIAN_POINT('Ctrl Pts',(-49.8932475177609,-55.2453425609388,
2.77555756156289E-16));
#76745=CARTESIAN_POINT('Ctrl Pts',(-49.9731817999155,-55.2255944921423,
2.77555756156289E-16));
#76746=CARTESIAN_POINT('Ctrl Pts',(-50.0481613529516,-55.1854902750885,
2.77555756156289E-16));
#76747=CARTESIAN_POINT('Ctrl Pts',(-50.1091461876225,-55.1300595714123,
2.77555756156289E-16));
#76748=CARTESIAN_POINT('',(-50.1091461876226,-55.1300595714123,12.));
#76749=CARTESIAN_POINT('Ctrl Pts',(-50.1091461876225,-55.1300595714123,
0.));
#76750=CARTESIAN_POINT('Ctrl Pts',(-50.1091461876225,-55.1300595714123,
4.));
#76751=CARTESIAN_POINT('Ctrl Pts',(-50.1091461876225,-55.1300595714123,
8.));
#76752=CARTESIAN_POINT('Ctrl Pts',(-50.1091461876225,-55.1300595714123,
12.));
#76753=CARTESIAN_POINT('',(-49.5707719660638,-55.2174072001495,12.));
#76754=CARTESIAN_POINT('Ctrl Pts',(-50.1091461876225,-55.1300595714123,
12.));
#76755=CARTESIAN_POINT('Ctrl Pts',(-50.0481613529516,-55.1854902750885,
12.));
#76756=CARTESIAN_POINT('Ctrl Pts',(-49.9731817999155,-55.2255944921423,
12.));
#76757=CARTESIAN_POINT('Ctrl Pts',(-49.8932475177609,-55.2453425609389,
12.));
#76758=CARTESIAN_POINT('Ctrl Pts',(-49.786668474888,-55.2716733193343,12.));
#76759=CARTESIAN_POINT('Ctrl Pts',(-49.6712810246932,-55.2618153697169,
12.));
#76760=CARTESIAN_POINT('Ctrl Pts',(-49.5707719660638,-55.2174072001495,
12.));
#76761=CARTESIAN_POINT('Ctrl Pts',(-49.5707719660638,-55.2174072001495,
12.));
#76762=CARTESIAN_POINT('Ctrl Pts',(-49.5707719660638,-55.2174072001495,
8.));
#76763=CARTESIAN_POINT('Ctrl Pts',(-49.5707719660638,-55.2174072001495,
4.));
#76764=CARTESIAN_POINT('Ctrl Pts',(-49.5707719660638,-55.2174072001495,
0.));
#76765=CARTESIAN_POINT('Origin',(-2.53167595884892E-10,-2.7643087079898E-10,
0.));
#76766=CARTESIAN_POINT('Origin',(-2.53167595884892E-10,-2.7643087079898E-10,
12.));
#76767=CARTESIAN_POINT('Origin',(-2.53167595884892E-10,-2.7643087079898E-10,
0.));
#76768=CARTESIAN_POINT('Ctrl Pts',(-55.1300595714105,-50.1091461876246,
0.));
#76769=CARTESIAN_POINT('Ctrl Pts',(-55.1300595714105,-50.1091461876246,
4.));
#76770=CARTESIAN_POINT('Ctrl Pts',(-55.1300595714105,-50.1091461876246,
8.));
#76771=CARTESIAN_POINT('Ctrl Pts',(-55.1300595714105,-50.1091461876246,
12.));
#76772=CARTESIAN_POINT('Ctrl Pts',(-55.2039671763178,-50.0278330747237,
0.));
#76773=CARTESIAN_POINT('Ctrl Pts',(-55.2039671763178,-50.0278330747237,
4.));
#76774=CARTESIAN_POINT('Ctrl Pts',(-55.2039671763178,-50.0278330747237,
8.));
#76775=CARTESIAN_POINT('Ctrl Pts',(-55.2039671763178,-50.0278330747237,
12.));
#76776=CARTESIAN_POINT('Ctrl Pts',(-55.2841761056306,-49.8417173275612,
0.));
#76777=CARTESIAN_POINT('Ctrl Pts',(-55.2841761056306,-49.8417173275612,
4.));
#76778=CARTESIAN_POINT('Ctrl Pts',(-55.2841761056306,-49.8417173275612,
7.99999999999999));
#76779=CARTESIAN_POINT('Ctrl Pts',(-55.2841761056306,-49.8417173275612,
12.));
#76780=CARTESIAN_POINT('Ctrl Pts',(-55.2507133273147,-49.6461537600002,
0.));
#76781=CARTESIAN_POINT('Ctrl Pts',(-55.2507133273147,-49.6461537600002,
4.));
#76782=CARTESIAN_POINT('Ctrl Pts',(-55.2507133273147,-49.6461537600002,
8.00000000000001));
#76783=CARTESIAN_POINT('Ctrl Pts',(-55.2507133273147,-49.6461537600002,
12.));
#76784=CARTESIAN_POINT('Ctrl Pts',(-55.21740720013,-49.5707719660253,0.));
#76785=CARTESIAN_POINT('Ctrl Pts',(-55.21740720013,-49.5707719660253,4.));
#76786=CARTESIAN_POINT('Ctrl Pts',(-55.21740720013,-49.5707719660253,8.));
#76787=CARTESIAN_POINT('Ctrl Pts',(-55.21740720013,-49.5707719660253,12.));
#76788=CARTESIAN_POINT('',(-55.1300595714105,-50.1091461876246,0.));
#76789=CARTESIAN_POINT('',(-55.2174072001297,-49.5707719660254,0.));
#76790=CARTESIAN_POINT('Ctrl Pts',(-55.1300595714105,-50.1091461876246,
1.38777878078145E-16));
#76791=CARTESIAN_POINT('Ctrl Pts',(-55.2039671763178,-50.0278330747237,
1.38777878078145E-16));
#76792=CARTESIAN_POINT('Ctrl Pts',(-55.2498008502108,-49.9214812192023,
1.38777878078145E-16));
#76793=CARTESIAN_POINT('Ctrl Pts',(-55.2585172318169,-49.8120443611017,
1.38777878078145E-16));
#76794=CARTESIAN_POINT('Ctrl Pts',(-55.2650545180215,-49.7299667175263,
1.38777878078145E-16));
#76795=CARTESIAN_POINT('Ctrl Pts',(-55.2507133273147,-49.6461537600002,
1.38777878078144E-16));
#76796=CARTESIAN_POINT('Ctrl Pts',(-55.21740720013,-49.5707719660253,1.38777878078145E-16));
#76797=CARTESIAN_POINT('',(-55.2174072001297,-49.5707719660254,12.));
#76798=CARTESIAN_POINT('Ctrl Pts',(-55.21740720013,-49.5707719660253,0.));
#76799=CARTESIAN_POINT('Ctrl Pts',(-55.21740720013,-49.5707719660253,4.));
#76800=CARTESIAN_POINT('Ctrl Pts',(-55.21740720013,-49.5707719660253,8.));
#76801=CARTESIAN_POINT('Ctrl Pts',(-55.21740720013,-49.5707719660253,12.));
#76802=CARTESIAN_POINT('',(-55.1300595714105,-50.1091461876246,12.));
#76803=CARTESIAN_POINT('Ctrl Pts',(-55.21740720013,-49.5707719660253,12.));
#76804=CARTESIAN_POINT('Ctrl Pts',(-55.2507133273147,-49.6461537600002,
12.));
#76805=CARTESIAN_POINT('Ctrl Pts',(-55.2650545180215,-49.7299667175263,
12.));
#76806=CARTESIAN_POINT('Ctrl Pts',(-55.2585172318169,-49.8120443611017,
12.));
#76807=CARTESIAN_POINT('Ctrl Pts',(-55.2498008502108,-49.9214812192023,
12.));
#76808=CARTESIAN_POINT('Ctrl Pts',(-55.2039671763178,-50.0278330747237,
12.));
#76809=CARTESIAN_POINT('Ctrl Pts',(-55.1300595714105,-50.1091461876246,
12.));
#76810=CARTESIAN_POINT('Ctrl Pts',(-55.1300595714105,-50.1091461876246,
12.));
#76811=CARTESIAN_POINT('Ctrl Pts',(-55.1300595714105,-50.1091461876246,
8.));
#76812=CARTESIAN_POINT('Ctrl Pts',(-55.1300595714105,-50.1091461876246,
4.));
#76813=CARTESIAN_POINT('Ctrl Pts',(-55.1300595714105,-50.1091461876246,
0.));
#76814=CARTESIAN_POINT('Ctrl Pts',(-53.0702932034641,-45.6458539113724,
0.));
#76815=CARTESIAN_POINT('Ctrl Pts',(-53.0702932034641,-45.6458539113724,
12.));
#76816=CARTESIAN_POINT('Ctrl Pts',(-53.0724894921849,-45.6490568514089,
0.));
#76817=CARTESIAN_POINT('Ctrl Pts',(-53.0724894921849,-45.6490568514089,
12.));
#76818=CARTESIAN_POINT('Ctrl Pts',(-53.0768833804193,-45.6554684028145,
0.));
#76819=CARTESIAN_POINT('Ctrl Pts',(-53.0768833804193,-45.6554684028145,
12.));
#76820=CARTESIAN_POINT('Ctrl Pts',(-53.0834781451546,-45.6651027439241,
0.));
#76821=CARTESIAN_POINT('Ctrl Pts',(-53.0834781451546,-45.6651027439241,
12.));
#76822=CARTESIAN_POINT('Ctrl Pts',(-53.0922790298409,-45.6779825614231,
0.));
#76823=CARTESIAN_POINT('Ctrl Pts',(-53.0922790298409,-45.6779825614231,
12.));
#76824=CARTESIAN_POINT('Ctrl Pts',(-53.1032932328857,-45.694139048907,0.));
#76825=CARTESIAN_POINT('Ctrl Pts',(-53.1032932328857,-45.694139048907,12.));
#76826=CARTESIAN_POINT('Ctrl Pts',(-53.114320495492,-45.7103522376696,0.));
#76827=CARTESIAN_POINT('Ctrl Pts',(-53.114320495492,-45.7103522376696,12.));
#76828=CARTESIAN_POINT('Ctrl Pts',(-53.1253607414872,-45.7266220897003,
0.));
#76829=CARTESIAN_POINT('Ctrl Pts',(-53.1253607414872,-45.7266220897003,
12.));
#76830=CARTESIAN_POINT('Ctrl Pts',(-53.1364138384693,-45.7429485300823,
0.));
#76831=CARTESIAN_POINT('Ctrl Pts',(-53.1364138384693,-45.7429485300823,
12.));
#76832=CARTESIAN_POINT('Ctrl Pts',(-53.1474795996053,-45.7593314474501,
0.));
#76833=CARTESIAN_POINT('Ctrl Pts',(-53.1474795996053,-45.7593314474501,
12.));
#76834=CARTESIAN_POINT('Ctrl Pts',(-53.1585578076444,-45.7757707100618,
0.));
#76835=CARTESIAN_POINT('Ctrl Pts',(-53.1585578076444,-45.7757707100618,
12.));
#76836=CARTESIAN_POINT('Ctrl Pts',(-53.1696482334487,-45.7922661780005,
0.));
#76837=CARTESIAN_POINT('Ctrl Pts',(-53.1696482334487,-45.7922661780005,
12.));
#76838=CARTESIAN_POINT('Ctrl Pts',(-53.1807506560933,-45.808817716509,0.));
#76839=CARTESIAN_POINT('Ctrl Pts',(-53.1807506560933,-45.808817716509,12.));
#76840=CARTESIAN_POINT('Ctrl Pts',(-53.1918648840541,-45.8254252099957,
0.));
#76841=CARTESIAN_POINT('Ctrl Pts',(-53.1918648840541,-45.8254252099957,
12.));
#76842=CARTESIAN_POINT('Ctrl Pts',(-53.2029907483557,-45.8420885575349,
0.));
#76843=CARTESIAN_POINT('Ctrl Pts',(-53.2029907483557,-45.8420885575349,
12.));
#76844=CARTESIAN_POINT('Ctrl Pts',(-53.2141280925439,-45.8588076662582,
0.));
#76845=CARTESIAN_POINT('Ctrl Pts',(-53.2141280925439,-45.8588076662582,
12.));
#76846=CARTESIAN_POINT('Ctrl Pts',(-53.2252767643662,-45.8755824458723,
0.));
#76847=CARTESIAN_POINT('Ctrl Pts',(-53.2252767643662,-45.8755824458723,
12.));
#76848=CARTESIAN_POINT('Ctrl Pts',(-53.2364366054306,-45.892412801838,0.));
#76849=CARTESIAN_POINT('Ctrl Pts',(-53.2364366054306,-45.892412801838,12.));
#76850=CARTESIAN_POINT('Ctrl Pts',(-53.2476074460017,-45.9092986319377,
0.));
#76851=CARTESIAN_POINT('Ctrl Pts',(-53.2476074460017,-45.9092986319377,
12.));
#76852=CARTESIAN_POINT('Ctrl Pts',(-53.2587891103866,-45.9262398298349,
0.));
#76853=CARTESIAN_POINT('Ctrl Pts',(-53.2587891103866,-45.9262398298349,
12.));
#76854=CARTESIAN_POINT('Ctrl Pts',(-53.2699814203105,-45.9432362873008,
0.));
#76855=CARTESIAN_POINT('Ctrl Pts',(-53.2699814203105,-45.9432362873008,
12.));
#76856=CARTESIAN_POINT('Ctrl Pts',(-53.2811841987926,-45.9602878967698,
0.));
#76857=CARTESIAN_POINT('Ctrl Pts',(-53.2811841987926,-45.9602878967698,
12.));
#76858=CARTESIAN_POINT('Ctrl Pts',(-53.292397274555,-45.9773945542384,0.));
#76859=CARTESIAN_POINT('Ctrl Pts',(-53.292397274555,-45.9773945542384,12.));
#76860=CARTESIAN_POINT('Ctrl Pts',(-53.3036204818329,-45.9945561591453,
0.));
#76861=CARTESIAN_POINT('Ctrl Pts',(-53.3036204818329,-45.9945561591453,
12.));
#76862=CARTESIAN_POINT('Ctrl Pts',(-53.3148536582635,-46.0117726129873,
0.));
#76863=CARTESIAN_POINT('Ctrl Pts',(-53.3148536582635,-46.0117726129873,
12.));
#76864=CARTESIAN_POINT('Ctrl Pts',(-53.326096643428,-46.02904381836,0.));
#76865=CARTESIAN_POINT('Ctrl Pts',(-53.326096643428,-46.02904381836,12.));
#76866=CARTESIAN_POINT('Ctrl Pts',(-53.3373492770671,-46.0463696777801,
0.));
#76867=CARTESIAN_POINT('Ctrl Pts',(-53.3373492770671,-46.0463696777801,
12.));
#76868=CARTESIAN_POINT('Ctrl Pts',(-53.3486113975901,-46.0637500926982,
0.));
#76869=CARTESIAN_POINT('Ctrl Pts',(-53.3486113975901,-46.0637500926982,
12.));
#76870=CARTESIAN_POINT('Ctrl Pts',(-53.3598828428546,-46.0811849640218,
0.));
#76871=CARTESIAN_POINT('Ctrl Pts',(-53.3598828428546,-46.0811849640218,
12.));
#76872=CARTESIAN_POINT('Ctrl Pts',(-53.3711634508437,-46.0986741925656,
0.));
#76873=CARTESIAN_POINT('Ctrl Pts',(-53.3711634508437,-46.0986741925656,
12.));
#76874=CARTESIAN_POINT('Ctrl Pts',(-53.3824530603276,-46.1162176794884,
0.));
#76875=CARTESIAN_POINT('Ctrl Pts',(-53.3824530603276,-46.1162176794884,
12.));
#76876=CARTESIAN_POINT('Ctrl Pts',(-53.3937515116549,-46.1338153268097,
0.));
#76877=CARTESIAN_POINT('Ctrl Pts',(-53.3937515116549,-46.1338153268097,
12.));
#76878=CARTESIAN_POINT('Ctrl Pts',(-53.4050586470436,-46.1514670376012,
0.));
#76879=CARTESIAN_POINT('Ctrl Pts',(-53.4050586470436,-46.1514670376012,
12.));
#76880=CARTESIAN_POINT('Ctrl Pts',(-53.4163743101517,-46.1691727157134,
0.));
#76881=CARTESIAN_POINT('Ctrl Pts',(-53.4163743101517,-46.1691727157134,
12.));
#76882=CARTESIAN_POINT('Ctrl Pts',(-53.4276983458125,-46.1869322656024,
0.));
#76883=CARTESIAN_POINT('Ctrl Pts',(-53.4276983458125,-46.1869322656024,
12.));
#76884=CARTESIAN_POINT('Ctrl Pts',(-53.4390305997274,-46.2047455921286,
0.));
#76885=CARTESIAN_POINT('Ctrl Pts',(-53.4390305997274,-46.2047455921286,
12.));
#76886=CARTESIAN_POINT('Ctrl Pts',(-53.4503709181178,-46.2226126003202,
0.));
#76887=CARTESIAN_POINT('Ctrl Pts',(-53.4503709181178,-46.2226126003202,
12.));
#76888=CARTESIAN_POINT('Ctrl Pts',(-53.4617191477402,-46.2405331953889,
0.));
#76889=CARTESIAN_POINT('Ctrl Pts',(-53.4617191477402,-46.2405331953889,
12.));
#76890=CARTESIAN_POINT('Ctrl Pts',(-53.4730751360371,-46.2585072828353,
0.));
#76891=CARTESIAN_POINT('Ctrl Pts',(-53.4730751360371,-46.2585072828353,
12.));
#76892=CARTESIAN_POINT('Ctrl Pts',(-53.4844387312414,-46.2765347685198,
0.));
#76893=CARTESIAN_POINT('Ctrl Pts',(-53.4844387312414,-46.2765347685198,
12.));
#76894=CARTESIAN_POINT('Ctrl Pts',(-53.4958097825006,-46.2946155587417,
0.));
#76895=CARTESIAN_POINT('Ctrl Pts',(-53.4958097825006,-46.2946155587417,
12.));
#76896=CARTESIAN_POINT('Ctrl Pts',(-53.5071881399911,-46.3127495603098,
0.));
#76897=CARTESIAN_POINT('Ctrl Pts',(-53.5071881399911,-46.3127495603098,
12.));
#76898=CARTESIAN_POINT('Ctrl Pts',(-53.5185736548548,-46.3309366805093,
0.));
#76899=CARTESIAN_POINT('Ctrl Pts',(-53.5185736548548,-46.3309366805093,
12.));
#76900=CARTESIAN_POINT('Ctrl Pts',(-53.5299661791385,-46.3491768270655,
0.));
#76901=CARTESIAN_POINT('Ctrl Pts',(-53.5299661791385,-46.3491768270655,
12.));
#76902=CARTESIAN_POINT('Ctrl Pts',(-53.5413655657327,-46.3674699081046,
0.));
#76903=CARTESIAN_POINT('Ctrl Pts',(-53.5413655657327,-46.3674699081046,
12.));
#76904=CARTESIAN_POINT('Ctrl Pts',(-53.5527716683048,-46.3858158321059,
0.));
#76905=CARTESIAN_POINT('Ctrl Pts',(-53.5527716683048,-46.3858158321059,
12.));
#76906=CARTESIAN_POINT('Ctrl Pts',(-53.5641843412559,-46.4042145078701,
0.));
#76907=CARTESIAN_POINT('Ctrl Pts',(-53.5641843412559,-46.4042145078701,
12.));
#76908=CARTESIAN_POINT('Ctrl Pts',(-53.5756034397481,-46.4226658445474,
0.));
#76909=CARTESIAN_POINT('Ctrl Pts',(-53.5756034397481,-46.4226658445474,
12.));
#76910=CARTESIAN_POINT('Ctrl Pts',(-53.5870288197166,-46.4411697516478,
0.));
#76911=CARTESIAN_POINT('Ctrl Pts',(-53.5870288197166,-46.4411697516478,
12.));
#76912=CARTESIAN_POINT('Ctrl Pts',(-53.5984603378855,-46.459726139052,0.));
#76913=CARTESIAN_POINT('Ctrl Pts',(-53.5984603378855,-46.459726139052,12.));
#76914=CARTESIAN_POINT('Ctrl Pts',(-53.6098978517859,-46.4783349170173,
0.));
#76915=CARTESIAN_POINT('Ctrl Pts',(-53.6098978517859,-46.4783349170173,
12.));
#76916=CARTESIAN_POINT('Ctrl Pts',(-53.6213412197533,-46.496995996177,0.));
#76917=CARTESIAN_POINT('Ctrl Pts',(-53.6213412197533,-46.496995996177,12.));
#76918=CARTESIAN_POINT('Ctrl Pts',(-53.6327903009094,-46.5157092875373,
0.));
#76919=CARTESIAN_POINT('Ctrl Pts',(-53.6327903009094,-46.5157092875373,
12.));
#76920=CARTESIAN_POINT('Ctrl Pts',(-53.6442449551455,-46.5344747024676,
0.));
#76921=CARTESIAN_POINT('Ctrl Pts',(-53.6442449551455,-46.5344747024676,
12.));
#76922=CARTESIAN_POINT('Ctrl Pts',(-53.6557050431071,-46.5532921526901,
0.));
#76923=CARTESIAN_POINT('Ctrl Pts',(-53.6557050431071,-46.5532921526901,
12.));
#76924=CARTESIAN_POINT('Ctrl Pts',(-53.6671704261737,-46.5721615502591,
0.));
#76925=CARTESIAN_POINT('Ctrl Pts',(-53.6671704261737,-46.5721615502591,
12.));
#76926=CARTESIAN_POINT('Ctrl Pts',(-53.678640966456,-46.5910828075653,0.));
#76927=CARTESIAN_POINT('Ctrl Pts',(-53.678640966456,-46.5910828075653,12.));
#76928=CARTESIAN_POINT('Ctrl Pts',(-53.6901165267941,-46.6100558373402,
0.));
#76929=CARTESIAN_POINT('Ctrl Pts',(-53.6901165267941,-46.6100558373402,
12.));
#76930=CARTESIAN_POINT('Ctrl Pts',(-53.701596970754,-46.6290805526559,0.));
#76931=CARTESIAN_POINT('Ctrl Pts',(-53.701596970754,-46.6290805526559,12.));
#76932=CARTESIAN_POINT('Ctrl Pts',(-53.7130821626263,-46.6481568669216,
0.));
#76933=CARTESIAN_POINT('Ctrl Pts',(-53.7130821626263,-46.6481568669216,
12.));
#76934=CARTESIAN_POINT('Ctrl Pts',(-53.7245719674222,-46.6672846938752,
0.));
#76935=CARTESIAN_POINT('Ctrl Pts',(-53.7245719674222,-46.6672846938752,
12.));
#76936=CARTESIAN_POINT('Ctrl Pts',(-53.7360662508677,-46.6864639475863,
0.));
#76937=CARTESIAN_POINT('Ctrl Pts',(-53.7360662508677,-46.6864639475863,
12.));
#76938=CARTESIAN_POINT('Ctrl Pts',(-53.7475648793948,-46.7056945424559,
0.));
#76939=CARTESIAN_POINT('Ctrl Pts',(-53.7475648793948,-46.7056945424559,
12.));
#76940=CARTESIAN_POINT('Ctrl Pts',(-53.7590677201344,-46.724976393213,0.));
#76941=CARTESIAN_POINT('Ctrl Pts',(-53.7590677201344,-46.724976393213,12.));
#76942=CARTESIAN_POINT('Ctrl Pts',(-53.770574640907,-46.7443094149041,0.));
#76943=CARTESIAN_POINT('Ctrl Pts',(-53.770574640907,-46.7443094149041,12.));
#76944=CARTESIAN_POINT('Ctrl Pts',(-53.782085510217,-46.7636935228851,0.));
#76945=CARTESIAN_POINT('Ctrl Pts',(-53.782085510217,-46.7636935228851,12.));
#76946=CARTESIAN_POINT('Ctrl Pts',(-53.7936001972468,-46.7831286328268,
0.));
#76947=CARTESIAN_POINT('Ctrl Pts',(-53.7936001972468,-46.7831286328268,
12.));
#76948=CARTESIAN_POINT('Ctrl Pts',(-53.8051185718525,-46.8026146607144,
0.));
#76949=CARTESIAN_POINT('Ctrl Pts',(-53.8051185718525,-46.8026146607144,
12.));
#76950=CARTESIAN_POINT('Ctrl Pts',(-53.8166405045582,-46.8221515228459,
0.));
#76951=CARTESIAN_POINT('Ctrl Pts',(-53.8166405045582,-46.8221515228459,
12.));
#76952=CARTESIAN_POINT('Ctrl Pts',(-53.8281658665517,-46.8417391358231,
0.));
#76953=CARTESIAN_POINT('Ctrl Pts',(-53.8281658665517,-46.8417391358231,
12.));
#76954=CARTESIAN_POINT('Ctrl Pts',(-53.8396945296777,-46.8613774165452,
0.));
#76955=CARTESIAN_POINT('Ctrl Pts',(-53.8396945296777,-46.8613774165452,
12.));
#76956=CARTESIAN_POINT('Ctrl Pts',(-53.851226366434,-46.8810662822147,0.));
#76957=CARTESIAN_POINT('Ctrl Pts',(-53.851226366434,-46.8810662822147,12.));
#76958=CARTESIAN_POINT('Ctrl Pts',(-53.8627612499648,-46.900805650336,0.));
#76959=CARTESIAN_POINT('Ctrl Pts',(-53.8627612499648,-46.900805650336,12.));
#76960=CARTESIAN_POINT('Ctrl Pts',(-53.8742990540557,-46.9205954387128,
0.));
#76961=CARTESIAN_POINT('Ctrl Pts',(-53.8742990540557,-46.9205954387128,
12.));
#76962=CARTESIAN_POINT('Ctrl Pts',(-53.8858396531277,-46.9404355654381,
0.));
#76963=CARTESIAN_POINT('Ctrl Pts',(-53.8858396531277,-46.9404355654381,
12.));
#76964=CARTESIAN_POINT('Ctrl Pts',(-53.8973829222317,-46.9603259488894,
0.));
#76965=CARTESIAN_POINT('Ctrl Pts',(-53.8973829222317,-46.9603259488894,
12.));
#76966=CARTESIAN_POINT('Ctrl Pts',(-53.9089287370436,-46.9802665077342,
0.));
#76967=CARTESIAN_POINT('Ctrl Pts',(-53.9089287370436,-46.9802665077342,
12.));
#76968=CARTESIAN_POINT('Ctrl Pts',(-53.9204769738584,-47.0002571609286,
0.));
#76969=CARTESIAN_POINT('Ctrl Pts',(-53.9204769738584,-47.0002571609286,
12.));
#76970=CARTESIAN_POINT('Ctrl Pts',(-53.9320275095864,-47.0202978277148,
0.));
#76971=CARTESIAN_POINT('Ctrl Pts',(-53.9320275095864,-47.0202978277148,
12.));
#76972=CARTESIAN_POINT('Ctrl Pts',(-53.9435802217468,-47.04038842761,0.));
#76973=CARTESIAN_POINT('Ctrl Pts',(-53.9435802217468,-47.04038842761,12.));
#76974=CARTESIAN_POINT('Ctrl Pts',(-53.9551349884637,-47.0605288804042,
0.));
#76975=CARTESIAN_POINT('Ctrl Pts',(-53.9551349884637,-47.0605288804042,
12.));
#76976=CARTESIAN_POINT('Ctrl Pts',(-53.9666916884624,-47.0807191061674,
0.));
#76977=CARTESIAN_POINT('Ctrl Pts',(-53.9666916884624,-47.0807191061674,
12.));
#76978=CARTESIAN_POINT('Ctrl Pts',(-53.9782502010642,-47.1009590252466,
0.));
#76979=CARTESIAN_POINT('Ctrl Pts',(-53.9782502010642,-47.1009590252466,
12.));
#76980=CARTESIAN_POINT('Ctrl Pts',(-53.9898104061809,-47.1212485582632,
0.));
#76981=CARTESIAN_POINT('Ctrl Pts',(-53.9898104061809,-47.1212485582632,
12.));
#76982=CARTESIAN_POINT('Ctrl Pts',(-54.0013721843094,-47.1415876261012,
0.));
#76983=CARTESIAN_POINT('Ctrl Pts',(-54.0013721843094,-47.1415876261012,
12.));
#76984=CARTESIAN_POINT('Ctrl Pts',(-54.0129354165269,-47.161976149906,0.));
#76985=CARTESIAN_POINT('Ctrl Pts',(-54.0129354165269,-47.161976149906,12.));
#76986=CARTESIAN_POINT('Ctrl Pts',(-54.0244999844872,-47.1824140510906,
0.));
#76987=CARTESIAN_POINT('Ctrl Pts',(-54.0244999844872,-47.1824140510906,
12.));
#76988=CARTESIAN_POINT('Ctrl Pts',(-54.0360657704156,-47.2029012513334,
0.));
#76989=CARTESIAN_POINT('Ctrl Pts',(-54.0360657704156,-47.2029012513334,
12.));
#76990=CARTESIAN_POINT('Ctrl Pts',(-54.047632657105,-47.2234376725752,0.));
#76991=CARTESIAN_POINT('Ctrl Pts',(-54.047632657105,-47.2234376725752,12.));
#76992=CARTESIAN_POINT('Ctrl Pts',(-54.0592005279108,-47.2440232370085,
0.));
#76993=CARTESIAN_POINT('Ctrl Pts',(-54.0592005279108,-47.2440232370085,
12.));
#76994=CARTESIAN_POINT('Ctrl Pts',(-54.0707692667461,-47.2646578670767,
0.));
#76995=CARTESIAN_POINT('Ctrl Pts',(-54.0707692667461,-47.2646578670767,
12.));
#76996=CARTESIAN_POINT('Ctrl Pts',(-54.082338758079,-47.2853414854805,0.));
#76997=CARTESIAN_POINT('Ctrl Pts',(-54.082338758079,-47.2853414854805,12.));
#76998=CARTESIAN_POINT('Ctrl Pts',(-54.0939088869271,-47.3060740151754,
0.));
#76999=CARTESIAN_POINT('Ctrl Pts',(-54.0939088869271,-47.3060740151754,
12.));
#77000=CARTESIAN_POINT('Ctrl Pts',(-54.1054795388538,-47.326855379369,0.));
#77001=CARTESIAN_POINT('Ctrl Pts',(-54.1054795388538,-47.326855379369,12.));
#77002=CARTESIAN_POINT('Ctrl Pts',(-54.1170505999637,-47.3476855015095,
0.));
#77003=CARTESIAN_POINT('Ctrl Pts',(-54.1170505999637,-47.3476855015095,
12.));
#77004=CARTESIAN_POINT('Ctrl Pts',(-54.1286219568981,-47.3685643052867,
0.));
#77005=CARTESIAN_POINT('Ctrl Pts',(-54.1286219568981,-47.3685643052867,
12.));
#77006=CARTESIAN_POINT('Ctrl Pts',(-54.1401934968306,-47.3894917146361,
0.));
#77007=CARTESIAN_POINT('Ctrl Pts',(-54.1401934968306,-47.3894917146361,
12.));
#77008=CARTESIAN_POINT('Ctrl Pts',(-54.1517651074638,-47.4104676537381,
0.));
#77009=CARTESIAN_POINT('Ctrl Pts',(-54.1517651074638,-47.4104676537381,
12.));
#77010=CARTESIAN_POINT('Ctrl Pts',(-54.163336677024,-47.4314920470142,0.));
#77011=CARTESIAN_POINT('Ctrl Pts',(-54.163336677024,-47.4314920470142,12.));
#77012=CARTESIAN_POINT('Ctrl Pts',(-54.1749080942593,-47.4525648191173,
0.));
#77013=CARTESIAN_POINT('Ctrl Pts',(-54.1749080942593,-47.4525648191173,
12.));
#77014=CARTESIAN_POINT('Ctrl Pts',(-54.1864792484343,-47.473685894932,0.));
#77015=CARTESIAN_POINT('Ctrl Pts',(-54.1864792484343,-47.473685894932,12.));
#77016=CARTESIAN_POINT('Ctrl Pts',(-54.1980500293267,-47.4948551995799,
0.));
#77017=CARTESIAN_POINT('Ctrl Pts',(-54.1980500293267,-47.4948551995799,
12.));
#77018=CARTESIAN_POINT('Ctrl Pts',(-54.2096203272228,-47.5160726584172,
0.));
#77019=CARTESIAN_POINT('Ctrl Pts',(-54.2096203272228,-47.5160726584172,
12.));
#77020=CARTESIAN_POINT('Ctrl Pts',(-54.2211900329141,-47.5373381970328,
0.));
#77021=CARTESIAN_POINT('Ctrl Pts',(-54.2211900329141,-47.5373381970328,
12.));
#77022=CARTESIAN_POINT('Ctrl Pts',(-54.232759037693,-47.5586517412368,0.));
#77023=CARTESIAN_POINT('Ctrl Pts',(-54.232759037693,-47.5586517412368,12.));
#77024=CARTESIAN_POINT('Ctrl Pts',(-54.2443272333498,-47.5800132170614,
0.));
#77025=CARTESIAN_POINT('Ctrl Pts',(-54.2443272333498,-47.5800132170614,
12.));
#77026=CARTESIAN_POINT('Ctrl Pts',(-54.2558945121684,-47.6014225507664,
0.));
#77027=CARTESIAN_POINT('Ctrl Pts',(-54.2558945121684,-47.6014225507664,
12.));
#77028=CARTESIAN_POINT('Ctrl Pts',(-54.2674607669228,-47.6228796688376,
0.));
#77029=CARTESIAN_POINT('Ctrl Pts',(-54.2674607669228,-47.6228796688376,
12.));
#77030=CARTESIAN_POINT('Ctrl Pts',(-54.2790258908736,-47.6443844979846,
0.));
#77031=CARTESIAN_POINT('Ctrl Pts',(-54.2790258908736,-47.6443844979846,
12.));
#77032=CARTESIAN_POINT('Ctrl Pts',(-54.2905897777647,-47.6659369651299,
0.));
#77033=CARTESIAN_POINT('Ctrl Pts',(-54.2905897777647,-47.6659369651299,
12.));
#77034=CARTESIAN_POINT('Ctrl Pts',(-54.3021523218188,-47.6875369974086,
0.));
#77035=CARTESIAN_POINT('Ctrl Pts',(-54.3021523218188,-47.6875369974086,
12.));
#77036=CARTESIAN_POINT('Ctrl Pts',(-54.3137134177345,-47.7091845221748,
0.));
#77037=CARTESIAN_POINT('Ctrl Pts',(-54.3137134177345,-47.7091845221748,
12.));
#77038=CARTESIAN_POINT('Ctrl Pts',(-54.3252729606824,-47.7308794669994,
0.));
#77039=CARTESIAN_POINT('Ctrl Pts',(-54.3252729606824,-47.7308794669994,
12.));
#77040=CARTESIAN_POINT('Ctrl Pts',(-54.3368308463023,-47.7526217596694,
0.));
#77041=CARTESIAN_POINT('Ctrl Pts',(-54.3368308463023,-47.7526217596694,
12.));
#77042=CARTESIAN_POINT('Ctrl Pts',(-54.3483869706998,-47.7744113281768,
0.));
#77043=CARTESIAN_POINT('Ctrl Pts',(-54.3483869706998,-47.7744113281768,
12.));
#77044=CARTESIAN_POINT('Ctrl Pts',(-54.3599412304431,-47.7962481007179,
0.));
#77045=CARTESIAN_POINT('Ctrl Pts',(-54.3599412304431,-47.7962481007179,
12.));
#77046=CARTESIAN_POINT('Ctrl Pts',(-54.3714935225585,-47.8181320056988,
0.));
#77047=CARTESIAN_POINT('Ctrl Pts',(-54.3714935225585,-47.8181320056988,
12.));
#77048=CARTESIAN_POINT('Ctrl Pts',(-54.3830437445275,-47.8400629717352,
0.));
#77049=CARTESIAN_POINT('Ctrl Pts',(-54.3830437445275,-47.8400629717352,
12.));
#77050=CARTESIAN_POINT('Ctrl Pts',(-54.3945917942835,-47.8620409276495,
0.));
#77051=CARTESIAN_POINT('Ctrl Pts',(-54.3945917942835,-47.8620409276495,
12.));
#77052=CARTESIAN_POINT('Ctrl Pts',(-54.4061375702088,-47.8840658024626,
0.));
#77053=CARTESIAN_POINT('Ctrl Pts',(-54.4061375702088,-47.8840658024626,
12.));
#77054=CARTESIAN_POINT('Ctrl Pts',(-54.4176809711324,-47.9061375253909,
0.));
#77055=CARTESIAN_POINT('Ctrl Pts',(-54.4176809711324,-47.9061375253909,
12.));
#77056=CARTESIAN_POINT('Ctrl Pts',(-54.4292218963253,-47.9282560258528,
0.));
#77057=CARTESIAN_POINT('Ctrl Pts',(-54.4292218963253,-47.9282560258528,
12.));
#77058=CARTESIAN_POINT('Ctrl Pts',(-54.4407602454974,-47.9504212334681,
0.));
#77059=CARTESIAN_POINT('Ctrl Pts',(-54.4407602454974,-47.9504212334681,
12.));
#77060=CARTESIAN_POINT('Ctrl Pts',(-54.4522959187952,-47.972633078057,0.));
#77061=CARTESIAN_POINT('Ctrl Pts',(-54.4522959187952,-47.972633078057,12.));
#77062=CARTESIAN_POINT('Ctrl Pts',(-54.4638288167991,-47.9948914896316,
0.));
#77063=CARTESIAN_POINT('Ctrl Pts',(-54.4638288167991,-47.9948914896316,
12.));
#77064=CARTESIAN_POINT('Ctrl Pts',(-54.4753588405202,-48.0171963983912,
0.));
#77065=CARTESIAN_POINT('Ctrl Pts',(-54.4753588405202,-48.0171963983912,
12.));
#77066=CARTESIAN_POINT('Ctrl Pts',(-54.4868858913961,-48.039547734729,0.));
#77067=CARTESIAN_POINT('Ctrl Pts',(-54.4868858913961,-48.039547734729,12.));
#77068=CARTESIAN_POINT('Ctrl Pts',(-54.4984098712883,-48.0619454292321,
0.));
#77069=CARTESIAN_POINT('Ctrl Pts',(-54.4984098712883,-48.0619454292321,
12.));
#77070=CARTESIAN_POINT('Ctrl Pts',(-54.5099306824788,-48.0843894126807,
0.));
#77071=CARTESIAN_POINT('Ctrl Pts',(-54.5099306824788,-48.0843894126807,
12.));
#77072=CARTESIAN_POINT('Ctrl Pts',(-54.5214482276679,-48.1068796160406,
0.));
#77073=CARTESIAN_POINT('Ctrl Pts',(-54.5214482276679,-48.1068796160406,
12.));
#77074=CARTESIAN_POINT('Ctrl Pts',(-54.5329624099719,-48.1294159704571,
0.));
#77075=CARTESIAN_POINT('Ctrl Pts',(-54.5329624099719,-48.1294159704571,
12.));
#77076=CARTESIAN_POINT('Ctrl Pts',(-54.5444731329196,-48.1519984072617,
0.));
#77077=CARTESIAN_POINT('Ctrl Pts',(-54.5444731329196,-48.1519984072617,
12.));
#77078=CARTESIAN_POINT('Ctrl Pts',(-54.5559803004487,-48.1746268579732,
0.));
#77079=CARTESIAN_POINT('Ctrl Pts',(-54.5559803004487,-48.1746268579732,
12.));
#77080=CARTESIAN_POINT('Ctrl Pts',(-54.5674838169041,-48.1973012542966,
0.));
#77081=CARTESIAN_POINT('Ctrl Pts',(-54.5674838169041,-48.1973012542966,
12.));
#77082=CARTESIAN_POINT('Ctrl Pts',(-54.5789835870348,-48.2200215281178,
0.));
#77083=CARTESIAN_POINT('Ctrl Pts',(-54.5789835870348,-48.2200215281178,
12.));
#77084=CARTESIAN_POINT('Ctrl Pts',(-54.5904795159936,-48.2427876114956,
0.));
#77085=CARTESIAN_POINT('Ctrl Pts',(-54.5904795159936,-48.2427876114956,
12.));
#77086=CARTESIAN_POINT('Ctrl Pts',(-54.6019715093319,-48.2655994366672,
0.));
#77087=CARTESIAN_POINT('Ctrl Pts',(-54.6019715093319,-48.2655994366672,
12.));
#77088=CARTESIAN_POINT('Ctrl Pts',(-54.6134594729964,-48.288456936051,0.));
#77089=CARTESIAN_POINT('Ctrl Pts',(-54.6134594729964,-48.288456936051,12.));
#77090=CARTESIAN_POINT('Ctrl Pts',(-54.6249433133262,-48.3113600422443,
0.));
#77091=CARTESIAN_POINT('Ctrl Pts',(-54.6249433133262,-48.3113600422443,
12.));
#77092=CARTESIAN_POINT('Ctrl Pts',(-54.636422937049,-48.3343086880192,0.));
#77093=CARTESIAN_POINT('Ctrl Pts',(-54.636422937049,-48.3343086880192,12.));
#77094=CARTESIAN_POINT('Ctrl Pts',(-54.647898251279,-48.3573028063122,0.));
#77095=CARTESIAN_POINT('Ctrl Pts',(-54.647898251279,-48.3573028063122,12.));
#77096=CARTESIAN_POINT('Ctrl Pts',(-54.6593691635143,-48.3803423302294,
0.));
#77097=CARTESIAN_POINT('Ctrl Pts',(-54.6593691635143,-48.3803423302294,
12.));
#77098=CARTESIAN_POINT('Ctrl Pts',(-54.6708355816359,-48.4034271930516,
0.));
#77099=CARTESIAN_POINT('Ctrl Pts',(-54.6708355816359,-48.4034271930516,
12.));
#77100=CARTESIAN_POINT('Ctrl Pts',(-54.6822974139065,-48.4265573282342,
0.));
#77101=CARTESIAN_POINT('Ctrl Pts',(-54.6822974139065,-48.4265573282342,
12.));
#77102=CARTESIAN_POINT('Ctrl Pts',(-54.6937545689694,-48.4497326694051,
0.));
#77103=CARTESIAN_POINT('Ctrl Pts',(-54.6937545689694,-48.4497326694051,
12.));
#77104=CARTESIAN_POINT('Ctrl Pts',(-54.7052069558493,-48.4729531503565,
0.));
#77105=CARTESIAN_POINT('Ctrl Pts',(-54.7052069558493,-48.4729531503565,
12.));
#77106=CARTESIAN_POINT('Ctrl Pts',(-54.7166544839475,-48.4962187050452,
0.));
#77107=CARTESIAN_POINT('Ctrl Pts',(-54.7166544839475,-48.4962187050452,
12.));
#77108=CARTESIAN_POINT('Ctrl Pts',(-54.7280970630346,-48.5195292675955,
0.));
#77109=CARTESIAN_POINT('Ctrl Pts',(-54.7280970630346,-48.5195292675955,
12.));
#77110=CARTESIAN_POINT('Ctrl Pts',(-54.7395346032451,-48.5428847722975,
0.));
#77111=CARTESIAN_POINT('Ctrl Pts',(-54.7395346032451,-48.5428847722975,
12.));
#77112=CARTESIAN_POINT('Ctrl Pts',(-54.7509670150716,-48.5662851536027,
0.));
#77113=CARTESIAN_POINT('Ctrl Pts',(-54.7509670150716,-48.5662851536027,
12.));
#77114=CARTESIAN_POINT('Ctrl Pts',(-54.7623942093591,-48.5897303461131,
0.));
#77115=CARTESIAN_POINT('Ctrl Pts',(-54.7623942093591,-48.5897303461131,
12.));
#77116=CARTESIAN_POINT('Ctrl Pts',(-54.773816097304,-48.6132202845792,0.));
#77117=CARTESIAN_POINT('Ctrl Pts',(-54.773816097304,-48.6132202845792,12.));
#77118=CARTESIAN_POINT('Ctrl Pts',(-54.7852325904591,-48.6367549039121,
0.));
#77119=CARTESIAN_POINT('Ctrl Pts',(-54.7852325904591,-48.6367549039121,
12.));
#77120=CARTESIAN_POINT('Ctrl Pts',(-54.7966436007395,-48.6603341391891,
0.));
#77121=CARTESIAN_POINT('Ctrl Pts',(-54.7966436007395,-48.6603341391891,
12.));
#77122=CARTESIAN_POINT('Ctrl Pts',(-54.8080490404274,-48.6839579256565,
0.));
#77123=CARTESIAN_POINT('Ctrl Pts',(-54.8080490404274,-48.6839579256565,
12.));
#77124=CARTESIAN_POINT('Ctrl Pts',(-54.8194488221803,-48.7076261987284,
0.));
#77125=CARTESIAN_POINT('Ctrl Pts',(-54.8194488221803,-48.7076261987284,
12.));
#77126=CARTESIAN_POINT('Ctrl Pts',(-54.8308428590334,-48.7313388939834,
0.));
#77127=CARTESIAN_POINT('Ctrl Pts',(-54.8308428590334,-48.7313388939834,
12.));
#77128=CARTESIAN_POINT('Ctrl Pts',(-54.8422310643752,-48.755095947159,0.));
#77129=CARTESIAN_POINT('Ctrl Pts',(-54.8422310643752,-48.755095947159,12.));
#77130=CARTESIAN_POINT('Ctrl Pts',(-54.8536133519285,-48.7788972941431,
0.));
#77131=CARTESIAN_POINT('Ctrl Pts',(-54.8536133519285,-48.7788972941431,
12.));
#77132=CARTESIAN_POINT('Ctrl Pts',(-54.8649896357284,-48.8027428709613,
0.));
#77133=CARTESIAN_POINT('Ctrl Pts',(-54.8649896357284,-48.8027428709613,
12.));
#77134=CARTESIAN_POINT('Ctrl Pts',(-54.8763598301045,-48.8266326137629,
0.));
#77135=CARTESIAN_POINT('Ctrl Pts',(-54.8763598301045,-48.8266326137629,
12.));
#77136=CARTESIAN_POINT('Ctrl Pts',(-54.8877238496577,-48.8505664587985,
0.));
#77137=CARTESIAN_POINT('Ctrl Pts',(-54.8877238496577,-48.8505664587985,
12.));
#77138=CARTESIAN_POINT('Ctrl Pts',(-54.8990816092964,-48.8745443424488,
0.));
#77139=CARTESIAN_POINT('Ctrl Pts',(-54.8990816092964,-48.8745443424488,
12.));
#77140=CARTESIAN_POINT('Ctrl Pts',(-54.910433024275,-48.8985662012535,0.));
#77141=CARTESIAN_POINT('Ctrl Pts',(-54.910433024275,-48.8985662012535,12.));
#77142=CARTESIAN_POINT('Ctrl Pts',(-54.9217780102357,-48.922631971937,0.));
#77143=CARTESIAN_POINT('Ctrl Pts',(-54.9217780102357,-48.922631971937,12.));
#77144=CARTESIAN_POINT('Ctrl Pts',(-54.933116483242,-48.9467415914266,0.));
#77145=CARTESIAN_POINT('Ctrl Pts',(-54.933116483242,-48.9467415914266,12.));
#77146=CARTESIAN_POINT('Ctrl Pts',(-54.9444483598372,-48.9708949968789,
0.));
#77147=CARTESIAN_POINT('Ctrl Pts',(-54.9444483598372,-48.9708949968789,
12.));
#77148=CARTESIAN_POINT('Ctrl Pts',(-54.9557735569936,-48.995092125652,0.));
#77149=CARTESIAN_POINT('Ctrl Pts',(-54.9557735569936,-48.995092125652,12.));
#77150=CARTESIAN_POINT('Ctrl Pts',(-54.9670919920024,-49.0193329152475,
0.));
#77151=CARTESIAN_POINT('Ctrl Pts',(-54.9670919920024,-49.0193329152475,
12.));
#77152=CARTESIAN_POINT('Ctrl Pts',(-54.9784035823764,-49.0436173032527,
0.));
#77153=CARTESIAN_POINT('Ctrl Pts',(-54.9784035823764,-49.0436173032527,
12.));
#77154=CARTESIAN_POINT('Ctrl Pts',(-54.9897082457606,-49.0679452272871,
0.));
#77155=CARTESIAN_POINT('Ctrl Pts',(-54.9897082457606,-49.0679452272871,
12.));
#77156=CARTESIAN_POINT('Ctrl Pts',(-55.0010058998111,-49.0923166249222,
0.));
#77157=CARTESIAN_POINT('Ctrl Pts',(-55.0010058998111,-49.0923166249222,
12.));
#77158=CARTESIAN_POINT('Ctrl Pts',(-55.0122964621868,-49.1167314336737,
0.));
#77159=CARTESIAN_POINT('Ctrl Pts',(-55.0122964621868,-49.1167314336737,
12.));
#77160=CARTESIAN_POINT('Ctrl Pts',(-55.0235798508056,-49.1411895911646,
0.));
#77161=CARTESIAN_POINT('Ctrl Pts',(-55.0235798508056,-49.1411895911646,
12.));
#77162=CARTESIAN_POINT('Ctrl Pts',(-55.0348559840462,-49.1656910352484,
0.));
#77163=CARTESIAN_POINT('Ctrl Pts',(-55.0348559840462,-49.1656910352484,
12.));
#77164=CARTESIAN_POINT('Ctrl Pts',(-55.0461247809745,-49.1902357041462,
0.));
#77165=CARTESIAN_POINT('Ctrl Pts',(-55.0461247809745,-49.1902357041462,
12.));
#77166=CARTESIAN_POINT('Ctrl Pts',(-55.0573861615569,-49.2148235365694,
0.));
#77167=CARTESIAN_POINT('Ctrl Pts',(-55.0573861615569,-49.2148235365694,
12.));
#77168=CARTESIAN_POINT('Ctrl Pts',(-55.0686400468911,-49.2394544718513,
0.));
#77169=CARTESIAN_POINT('Ctrl Pts',(-55.0686400468911,-49.2394544718513,
12.));
#77170=CARTESIAN_POINT('Ctrl Pts',(-55.0798863586986,-49.2641284496496,
0.));
#77171=CARTESIAN_POINT('Ctrl Pts',(-55.0798863586986,-49.2641284496496,
12.));
#77172=CARTESIAN_POINT('Ctrl Pts',(-55.0911250188282,-49.2888454096544,
0.));
#77173=CARTESIAN_POINT('Ctrl Pts',(-55.0911250188282,-49.2888454096544,
12.));
#77174=CARTESIAN_POINT('Ctrl Pts',(-55.1023559487133,-49.3136052912614,
0.));
#77175=CARTESIAN_POINT('Ctrl Pts',(-55.1023559487133,-49.3136052912614,
12.));
#77176=CARTESIAN_POINT('Ctrl Pts',(-55.1135790689475,-49.3384080333166,
0.));
#77177=CARTESIAN_POINT('Ctrl Pts',(-55.1135790689475,-49.3384080333166,
12.));
#77178=CARTESIAN_POINT('Ctrl Pts',(-55.1247942985649,-49.3632535736744,
0.));
#77179=CARTESIAN_POINT('Ctrl Pts',(-55.1247942985649,-49.3632535736744,
12.));
#77180=CARTESIAN_POINT('Ctrl Pts',(-55.1360015556262,-49.3881418495529,
0.));
#77181=CARTESIAN_POINT('Ctrl Pts',(-55.1360015556262,-49.3881418495529,
12.));
#77182=CARTESIAN_POINT('Ctrl Pts',(-55.1472007585224,-49.413072798324,0.));
#77183=CARTESIAN_POINT('Ctrl Pts',(-55.1472007585224,-49.413072798324,12.));
#77184=CARTESIAN_POINT('Ctrl Pts',(-55.158391827114,-49.4380463581989,0.));
#77185=CARTESIAN_POINT('Ctrl Pts',(-55.158391827114,-49.4380463581989,12.));
#77186=CARTESIAN_POINT('Ctrl Pts',(-55.1695746838168,-49.4630624688787,
0.));
#77187=CARTESIAN_POINT('Ctrl Pts',(-55.1695746838168,-49.4630624688787,
12.));
#77188=CARTESIAN_POINT('Ctrl Pts',(-55.1807492550073,-49.4881210723921,
0.));
#77189=CARTESIAN_POINT('Ctrl Pts',(-55.1807492550073,-49.4881210723921,
12.));
#77190=CARTESIAN_POINT('Ctrl Pts',(-55.1919154713569,-49.5132221132916,
0.));
#77191=CARTESIAN_POINT('Ctrl Pts',(-55.1919154713569,-49.5132221132916,
12.));
#77192=CARTESIAN_POINT('Ctrl Pts',(-55.2030732647222,-49.5383655367987,
0.));
#77193=CARTESIAN_POINT('Ctrl Pts',(-55.2030732647222,-49.5383655367987,
12.));
#77194=CARTESIAN_POINT('Ctrl Pts',(-55.2142225656943,-49.5635512873368,
0.));
#77195=CARTESIAN_POINT('Ctrl Pts',(-55.2142225656943,-49.5635512873368,
12.));
#77196=CARTESIAN_POINT('Ctrl Pts',(-55.225363300765,-49.5887793068337,0.));
#77197=CARTESIAN_POINT('Ctrl Pts',(-55.225363300765,-49.5887793068337,12.));
#77198=CARTESIAN_POINT('Ctrl Pts',(-55.2364953899423,-49.6140495332865,
0.));
#77199=CARTESIAN_POINT('Ctrl Pts',(-55.2364953899423,-49.6140495332865,
12.));
#77200=CARTESIAN_POINT('Ctrl Pts',(-55.2476187434204,-49.6393618987614,
0.));
#77201=CARTESIAN_POINT('Ctrl Pts',(-55.2476187434204,-49.6393618987614,
12.));
#77202=CARTESIAN_POINT('Ctrl Pts',(-55.2587332663982,-49.6647163322457,
0.));
#77203=CARTESIAN_POINT('Ctrl Pts',(-55.2587332663982,-49.6647163322457,
12.));
#77204=CARTESIAN_POINT('Ctrl Pts',(-55.2698388650215,-49.690112763181,0.));
#77205=CARTESIAN_POINT('Ctrl Pts',(-55.2698388650215,-49.690112763181,12.));
#77206=CARTESIAN_POINT('Ctrl Pts',(-55.2809354521616,-49.7155511248629,
0.));
#77207=CARTESIAN_POINT('Ctrl Pts',(-55.2809354521616,-49.7155511248629,
12.));
#77208=CARTESIAN_POINT('Ctrl Pts',(-55.292022952748,-49.7410313576444,0.));
#77209=CARTESIAN_POINT('Ctrl Pts',(-55.292022952748,-49.7410313576444,12.));
#77210=CARTESIAN_POINT('Ctrl Pts',(-55.3031013105578,-49.7665534128269,
0.));
#77211=CARTESIAN_POINT('Ctrl Pts',(-55.3031013105578,-49.7665534128269,
12.));
#77212=CARTESIAN_POINT('Ctrl Pts',(-55.3141704897307,-49.7921172540185,
0.));
#77213=CARTESIAN_POINT('Ctrl Pts',(-55.3141704897307,-49.7921172540185,
12.));
#77214=CARTESIAN_POINT('Ctrl Pts',(-55.3252304694066,-49.817722855186,0.));
#77215=CARTESIAN_POINT('Ctrl Pts',(-55.3252304694066,-49.817722855186,12.));
#77216=CARTESIAN_POINT('Ctrl Pts',(-55.3340710859607,-49.8382407306675,
0.));
#77217=CARTESIAN_POINT('Ctrl Pts',(-55.3340710859607,-49.8382407306675,
12.));
#77218=CARTESIAN_POINT('Ctrl Pts',(-55.340697403233,-49.8536479176573,0.));
#77219=CARTESIAN_POINT('Ctrl Pts',(-55.340697403233,-49.8536479176573,12.));
#77220=CARTESIAN_POINT('Ctrl Pts',(-55.3451131058727,-49.8639277221471,
0.));
#77221=CARTESIAN_POINT('Ctrl Pts',(-55.3451131058727,-49.8639277221471,
12.));
#77222=CARTESIAN_POINT('Ctrl Pts',(-55.3473204966403,-49.8690697110161,
0.));
#77223=CARTESIAN_POINT('Ctrl Pts',(-55.3473204966403,-49.8690697110161,
12.));
#77224=CARTESIAN_POINT('',(-53.0702932034641,-45.6458539113724,0.));
#77225=CARTESIAN_POINT('Ctrl Pts',(-53.0702932034641,-45.6458539113724,
0.));
#77226=CARTESIAN_POINT('Ctrl Pts',(-53.0724894921849,-45.6490568514089,
0.));
#77227=CARTESIAN_POINT('Ctrl Pts',(-53.0768833804193,-45.6554684028145,
0.));
#77228=CARTESIAN_POINT('Ctrl Pts',(-53.0834781451546,-45.6651027439241,
0.));
#77229=CARTESIAN_POINT('Ctrl Pts',(-53.0922790298409,-45.6779825614231,
0.));
#77230=CARTESIAN_POINT('Ctrl Pts',(-53.1032932328857,-45.694139048907,0.));
#77231=CARTESIAN_POINT('Ctrl Pts',(-53.114320495492,-45.7103522376696,0.));
#77232=CARTESIAN_POINT('Ctrl Pts',(-53.1253607414872,-45.7266220897003,
0.));
#77233=CARTESIAN_POINT('Ctrl Pts',(-53.1364138384693,-45.7429485300823,
0.));
#77234=CARTESIAN_POINT('Ctrl Pts',(-53.1474795996053,-45.7593314474501,
0.));
#77235=CARTESIAN_POINT('Ctrl Pts',(-53.1585578076444,-45.7757707100618,
0.));
#77236=CARTESIAN_POINT('Ctrl Pts',(-53.1696482334487,-45.7922661780005,
0.));
#77237=CARTESIAN_POINT('Ctrl Pts',(-53.1807506560933,-45.808817716509,0.));
#77238=CARTESIAN_POINT('Ctrl Pts',(-53.1918648840541,-45.8254252099957,
0.));
#77239=CARTESIAN_POINT('Ctrl Pts',(-53.2029907483557,-45.8420885575349,
0.));
#77240=CARTESIAN_POINT('Ctrl Pts',(-53.2141280925439,-45.8588076662582,
0.));
#77241=CARTESIAN_POINT('Ctrl Pts',(-53.2252767643662,-45.8755824458723,
0.));
#77242=CARTESIAN_POINT('Ctrl Pts',(-53.2364366054306,-45.892412801838,0.));
#77243=CARTESIAN_POINT('Ctrl Pts',(-53.2476074460017,-45.9092986319377,
0.));
#77244=CARTESIAN_POINT('Ctrl Pts',(-53.2587891103866,-45.9262398298349,
0.));
#77245=CARTESIAN_POINT('Ctrl Pts',(-53.2699814203105,-45.9432362873008,
0.));
#77246=CARTESIAN_POINT('Ctrl Pts',(-53.2811841987926,-45.9602878967698,
0.));
#77247=CARTESIAN_POINT('Ctrl Pts',(-53.292397274555,-45.9773945542384,0.));
#77248=CARTESIAN_POINT('Ctrl Pts',(-53.3036204818329,-45.9945561591453,
0.));
#77249=CARTESIAN_POINT('Ctrl Pts',(-53.3148536582635,-46.0117726129873,
0.));
#77250=CARTESIAN_POINT('Ctrl Pts',(-53.326096643428,-46.02904381836,0.));
#77251=CARTESIAN_POINT('Ctrl Pts',(-53.3373492770671,-46.0463696777801,
0.));
#77252=CARTESIAN_POINT('Ctrl Pts',(-53.3486113975901,-46.0637500926982,
0.));
#77253=CARTESIAN_POINT('Ctrl Pts',(-53.3598828428546,-46.0811849640218,
0.));
#77254=CARTESIAN_POINT('Ctrl Pts',(-53.3711634508437,-46.0986741925656,
0.));
#77255=CARTESIAN_POINT('Ctrl Pts',(-53.3824530603276,-46.1162176794884,
0.));
#77256=CARTESIAN_POINT('Ctrl Pts',(-53.3937515116549,-46.1338153268097,
0.));
#77257=CARTESIAN_POINT('Ctrl Pts',(-53.4050586470436,-46.1514670376012,
0.));
#77258=CARTESIAN_POINT('Ctrl Pts',(-53.4163743101517,-46.1691727157134,
0.));
#77259=CARTESIAN_POINT('Ctrl Pts',(-53.4276983458125,-46.1869322656024,
0.));
#77260=CARTESIAN_POINT('Ctrl Pts',(-53.4390305997274,-46.2047455921286,
0.));
#77261=CARTESIAN_POINT('Ctrl Pts',(-53.4503709181178,-46.2226126003202,
0.));
#77262=CARTESIAN_POINT('Ctrl Pts',(-53.4617191477402,-46.2405331953889,
0.));
#77263=CARTESIAN_POINT('Ctrl Pts',(-53.4730751360371,-46.2585072828353,
0.));
#77264=CARTESIAN_POINT('Ctrl Pts',(-53.4844387312414,-46.2765347685198,
0.));
#77265=CARTESIAN_POINT('Ctrl Pts',(-53.4958097825006,-46.2946155587417,
0.));
#77266=CARTESIAN_POINT('Ctrl Pts',(-53.5071881399911,-46.3127495603098,
0.));
#77267=CARTESIAN_POINT('Ctrl Pts',(-53.5185736548548,-46.3309366805093,
0.));
#77268=CARTESIAN_POINT('Ctrl Pts',(-53.5299661791385,-46.3491768270655,
0.));
#77269=CARTESIAN_POINT('Ctrl Pts',(-53.5413655657327,-46.3674699081046,
0.));
#77270=CARTESIAN_POINT('Ctrl Pts',(-53.5527716683048,-46.3858158321059,
0.));
#77271=CARTESIAN_POINT('Ctrl Pts',(-53.5641843412559,-46.4042145078701,
0.));
#77272=CARTESIAN_POINT('Ctrl Pts',(-53.5756034397481,-46.4226658445474,
0.));
#77273=CARTESIAN_POINT('Ctrl Pts',(-53.5870288197166,-46.4411697516478,
0.));
#77274=CARTESIAN_POINT('Ctrl Pts',(-53.5984603378855,-46.459726139052,0.));
#77275=CARTESIAN_POINT('Ctrl Pts',(-53.6098978517859,-46.4783349170173,
0.));
#77276=CARTESIAN_POINT('Ctrl Pts',(-53.6213412197533,-46.496995996177,0.));
#77277=CARTESIAN_POINT('Ctrl Pts',(-53.6327903009094,-46.5157092875373,
0.));
#77278=CARTESIAN_POINT('Ctrl Pts',(-53.6442449551455,-46.5344747024676,
0.));
#77279=CARTESIAN_POINT('Ctrl Pts',(-53.6557050431071,-46.5532921526901,
0.));
#77280=CARTESIAN_POINT('Ctrl Pts',(-53.6671704261737,-46.5721615502591,
0.));
#77281=CARTESIAN_POINT('Ctrl Pts',(-53.678640966456,-46.5910828075653,0.));
#77282=CARTESIAN_POINT('Ctrl Pts',(-53.6901165267941,-46.6100558373402,
0.));
#77283=CARTESIAN_POINT('Ctrl Pts',(-53.701596970754,-46.6290805526559,0.));
#77284=CARTESIAN_POINT('Ctrl Pts',(-53.7130821626263,-46.6481568669216,
0.));
#77285=CARTESIAN_POINT('Ctrl Pts',(-53.7245719674222,-46.6672846938752,
0.));
#77286=CARTESIAN_POINT('Ctrl Pts',(-53.7360662508677,-46.6864639475863,
0.));
#77287=CARTESIAN_POINT('Ctrl Pts',(-53.7475648793948,-46.7056945424559,
0.));
#77288=CARTESIAN_POINT('Ctrl Pts',(-53.7590677201344,-46.724976393213,0.));
#77289=CARTESIAN_POINT('Ctrl Pts',(-53.770574640907,-46.7443094149041,0.));
#77290=CARTESIAN_POINT('Ctrl Pts',(-53.782085510217,-46.7636935228851,0.));
#77291=CARTESIAN_POINT('Ctrl Pts',(-53.7936001972468,-46.7831286328268,
0.));
#77292=CARTESIAN_POINT('Ctrl Pts',(-53.8051185718525,-46.8026146607144,
0.));
#77293=CARTESIAN_POINT('Ctrl Pts',(-53.8166405045582,-46.8221515228459,
0.));
#77294=CARTESIAN_POINT('Ctrl Pts',(-53.8281658665517,-46.8417391358231,
0.));
#77295=CARTESIAN_POINT('Ctrl Pts',(-53.8396945296777,-46.8613774165452,
0.));
#77296=CARTESIAN_POINT('Ctrl Pts',(-53.851226366434,-46.8810662822147,0.));
#77297=CARTESIAN_POINT('Ctrl Pts',(-53.8627612499648,-46.900805650336,0.));
#77298=CARTESIAN_POINT('Ctrl Pts',(-53.8742990540557,-46.9205954387128,
0.));
#77299=CARTESIAN_POINT('Ctrl Pts',(-53.8858396531277,-46.9404355654381,
0.));
#77300=CARTESIAN_POINT('Ctrl Pts',(-53.8973829222317,-46.9603259488894,
0.));
#77301=CARTESIAN_POINT('Ctrl Pts',(-53.9089287370436,-46.9802665077342,
0.));
#77302=CARTESIAN_POINT('Ctrl Pts',(-53.9204769738584,-47.0002571609286,
0.));
#77303=CARTESIAN_POINT('Ctrl Pts',(-53.9320275095864,-47.0202978277148,
0.));
#77304=CARTESIAN_POINT('Ctrl Pts',(-53.9435802217468,-47.04038842761,0.));
#77305=CARTESIAN_POINT('Ctrl Pts',(-53.9551349884637,-47.0605288804042,
0.));
#77306=CARTESIAN_POINT('Ctrl Pts',(-53.9666916884624,-47.0807191061674,
0.));
#77307=CARTESIAN_POINT('Ctrl Pts',(-53.9782502010642,-47.1009590252466,
0.));
#77308=CARTESIAN_POINT('Ctrl Pts',(-53.9898104061809,-47.1212485582632,
0.));
#77309=CARTESIAN_POINT('Ctrl Pts',(-54.0013721843094,-47.1415876261012,
0.));
#77310=CARTESIAN_POINT('Ctrl Pts',(-54.0129354165269,-47.161976149906,0.));
#77311=CARTESIAN_POINT('Ctrl Pts',(-54.0244999844872,-47.1824140510906,
0.));
#77312=CARTESIAN_POINT('Ctrl Pts',(-54.0360657704156,-47.2029012513334,
0.));
#77313=CARTESIAN_POINT('Ctrl Pts',(-54.047632657105,-47.2234376725752,0.));
#77314=CARTESIAN_POINT('Ctrl Pts',(-54.0592005279108,-47.2440232370085,
0.));
#77315=CARTESIAN_POINT('Ctrl Pts',(-54.0707692667461,-47.2646578670767,
0.));
#77316=CARTESIAN_POINT('Ctrl Pts',(-54.082338758079,-47.2853414854805,0.));
#77317=CARTESIAN_POINT('Ctrl Pts',(-54.0939088869271,-47.3060740151754,
0.));
#77318=CARTESIAN_POINT('Ctrl Pts',(-54.1054795388538,-47.326855379369,0.));
#77319=CARTESIAN_POINT('Ctrl Pts',(-54.1170505999637,-47.3476855015095,
0.));
#77320=CARTESIAN_POINT('Ctrl Pts',(-54.1286219568981,-47.3685643052867,
0.));
#77321=CARTESIAN_POINT('Ctrl Pts',(-54.1401934968306,-47.3894917146361,
0.));
#77322=CARTESIAN_POINT('Ctrl Pts',(-54.1517651074638,-47.4104676537381,
0.));
#77323=CARTESIAN_POINT('Ctrl Pts',(-54.163336677024,-47.4314920470142,0.));
#77324=CARTESIAN_POINT('Ctrl Pts',(-54.1749080942593,-47.4525648191173,
0.));
#77325=CARTESIAN_POINT('Ctrl Pts',(-54.1864792484343,-47.473685894932,0.));
#77326=CARTESIAN_POINT('Ctrl Pts',(-54.1980500293267,-47.4948551995799,
0.));
#77327=CARTESIAN_POINT('Ctrl Pts',(-54.2096203272228,-47.5160726584172,
0.));
#77328=CARTESIAN_POINT('Ctrl Pts',(-54.2211900329141,-47.5373381970328,
0.));
#77329=CARTESIAN_POINT('Ctrl Pts',(-54.232759037693,-47.5586517412368,0.));
#77330=CARTESIAN_POINT('Ctrl Pts',(-54.2443272333498,-47.5800132170614,
0.));
#77331=CARTESIAN_POINT('Ctrl Pts',(-54.2558945121684,-47.6014225507664,
0.));
#77332=CARTESIAN_POINT('Ctrl Pts',(-54.2674607669228,-47.6228796688376,
0.));
#77333=CARTESIAN_POINT('Ctrl Pts',(-54.2790258908736,-47.6443844979846,
0.));
#77334=CARTESIAN_POINT('Ctrl Pts',(-54.2905897777647,-47.6659369651299,
0.));
#77335=CARTESIAN_POINT('Ctrl Pts',(-54.3021523218188,-47.6875369974086,
0.));
#77336=CARTESIAN_POINT('Ctrl Pts',(-54.3137134177345,-47.7091845221748,
0.));
#77337=CARTESIAN_POINT('Ctrl Pts',(-54.3252729606824,-47.7308794669994,
0.));
#77338=CARTESIAN_POINT('Ctrl Pts',(-54.3368308463023,-47.7526217596694,
0.));
#77339=CARTESIAN_POINT('Ctrl Pts',(-54.3483869706998,-47.7744113281768,
0.));
#77340=CARTESIAN_POINT('Ctrl Pts',(-54.3599412304431,-47.7962481007179,
0.));
#77341=CARTESIAN_POINT('Ctrl Pts',(-54.3714935225585,-47.8181320056988,
0.));
#77342=CARTESIAN_POINT('Ctrl Pts',(-54.3830437445275,-47.8400629717352,
0.));
#77343=CARTESIAN_POINT('Ctrl Pts',(-54.3945917942835,-47.8620409276495,
0.));
#77344=CARTESIAN_POINT('Ctrl Pts',(-54.4061375702088,-47.8840658024626,
0.));
#77345=CARTESIAN_POINT('Ctrl Pts',(-54.4176809711324,-47.9061375253909,
0.));
#77346=CARTESIAN_POINT('Ctrl Pts',(-54.4292218963253,-47.9282560258528,
0.));
#77347=CARTESIAN_POINT('Ctrl Pts',(-54.4407602454974,-47.9504212334681,
0.));
#77348=CARTESIAN_POINT('Ctrl Pts',(-54.4522959187952,-47.972633078057,0.));
#77349=CARTESIAN_POINT('Ctrl Pts',(-54.4638288167991,-47.9948914896316,
0.));
#77350=CARTESIAN_POINT('Ctrl Pts',(-54.4753588405202,-48.0171963983912,
0.));
#77351=CARTESIAN_POINT('Ctrl Pts',(-54.4868858913961,-48.039547734729,0.));
#77352=CARTESIAN_POINT('Ctrl Pts',(-54.4984098712883,-48.0619454292321,
0.));
#77353=CARTESIAN_POINT('Ctrl Pts',(-54.5099306824788,-48.0843894126807,
0.));
#77354=CARTESIAN_POINT('Ctrl Pts',(-54.5214482276679,-48.1068796160406,
0.));
#77355=CARTESIAN_POINT('Ctrl Pts',(-54.5329624099719,-48.1294159704571,
0.));
#77356=CARTESIAN_POINT('Ctrl Pts',(-54.5444731329196,-48.1519984072617,
0.));
#77357=CARTESIAN_POINT('Ctrl Pts',(-54.5559803004487,-48.1746268579732,
0.));
#77358=CARTESIAN_POINT('Ctrl Pts',(-54.5674838169041,-48.1973012542966,
0.));
#77359=CARTESIAN_POINT('Ctrl Pts',(-54.5789835870348,-48.2200215281178,
0.));
#77360=CARTESIAN_POINT('Ctrl Pts',(-54.5904795159936,-48.2427876114956,
0.));
#77361=CARTESIAN_POINT('Ctrl Pts',(-54.6019715093319,-48.2655994366672,
0.));
#77362=CARTESIAN_POINT('Ctrl Pts',(-54.6134594729964,-48.288456936051,0.));
#77363=CARTESIAN_POINT('Ctrl Pts',(-54.6249433133262,-48.3113600422443,
0.));
#77364=CARTESIAN_POINT('Ctrl Pts',(-54.636422937049,-48.3343086880192,0.));
#77365=CARTESIAN_POINT('Ctrl Pts',(-54.647898251279,-48.3573028063122,0.));
#77366=CARTESIAN_POINT('Ctrl Pts',(-54.6593691635143,-48.3803423302294,
0.));
#77367=CARTESIAN_POINT('Ctrl Pts',(-54.6708355816359,-48.4034271930516,
0.));
#77368=CARTESIAN_POINT('Ctrl Pts',(-54.6822974139065,-48.4265573282342,
0.));
#77369=CARTESIAN_POINT('Ctrl Pts',(-54.6937545689694,-48.4497326694051,
0.));
#77370=CARTESIAN_POINT('Ctrl Pts',(-54.7052069558493,-48.4729531503565,
0.));
#77371=CARTESIAN_POINT('Ctrl Pts',(-54.7166544839475,-48.4962187050452,
0.));
#77372=CARTESIAN_POINT('Ctrl Pts',(-54.7280970630346,-48.5195292675955,
0.));
#77373=CARTESIAN_POINT('Ctrl Pts',(-54.7395346032451,-48.5428847722975,
0.));
#77374=CARTESIAN_POINT('Ctrl Pts',(-54.7509670150716,-48.5662851536027,
0.));
#77375=CARTESIAN_POINT('Ctrl Pts',(-54.7623942093591,-48.5897303461131,
0.));
#77376=CARTESIAN_POINT('Ctrl Pts',(-54.773816097304,-48.6132202845792,0.));
#77377=CARTESIAN_POINT('Ctrl Pts',(-54.7852325904591,-48.6367549039121,
0.));
#77378=CARTESIAN_POINT('Ctrl Pts',(-54.7966436007395,-48.6603341391891,
0.));
#77379=CARTESIAN_POINT('Ctrl Pts',(-54.8080490404274,-48.6839579256565,
0.));
#77380=CARTESIAN_POINT('Ctrl Pts',(-54.8194488221803,-48.7076261987284,
0.));
#77381=CARTESIAN_POINT('Ctrl Pts',(-54.8308428590334,-48.7313388939834,
0.));
#77382=CARTESIAN_POINT('Ctrl Pts',(-54.8422310643752,-48.755095947159,0.));
#77383=CARTESIAN_POINT('Ctrl Pts',(-54.8536133519285,-48.7788972941431,
0.));
#77384=CARTESIAN_POINT('Ctrl Pts',(-54.8649896357284,-48.8027428709613,
0.));
#77385=CARTESIAN_POINT('Ctrl Pts',(-54.8763598301045,-48.8266326137629,
0.));
#77386=CARTESIAN_POINT('Ctrl Pts',(-54.8877238496577,-48.8505664587985,
0.));
#77387=CARTESIAN_POINT('Ctrl Pts',(-54.8990816092964,-48.8745443424488,
0.));
#77388=CARTESIAN_POINT('Ctrl Pts',(-54.910433024275,-48.8985662012535,0.));
#77389=CARTESIAN_POINT('Ctrl Pts',(-54.9217780102357,-48.922631971937,0.));
#77390=CARTESIAN_POINT('Ctrl Pts',(-54.933116483242,-48.9467415914266,0.));
#77391=CARTESIAN_POINT('Ctrl Pts',(-54.9444483598372,-48.9708949968789,
0.));
#77392=CARTESIAN_POINT('Ctrl Pts',(-54.9557735569936,-48.995092125652,0.));
#77393=CARTESIAN_POINT('Ctrl Pts',(-54.9670919920024,-49.0193329152475,
0.));
#77394=CARTESIAN_POINT('Ctrl Pts',(-54.9784035823764,-49.0436173032527,
0.));
#77395=CARTESIAN_POINT('Ctrl Pts',(-54.9897082457606,-49.0679452272871,
0.));
#77396=CARTESIAN_POINT('Ctrl Pts',(-55.0010058998111,-49.0923166249222,
0.));
#77397=CARTESIAN_POINT('Ctrl Pts',(-55.0122964621868,-49.1167314336737,
0.));
#77398=CARTESIAN_POINT('Ctrl Pts',(-55.0235798508056,-49.1411895911646,
0.));
#77399=CARTESIAN_POINT('Ctrl Pts',(-55.0348559840462,-49.1656910352484,
0.));
#77400=CARTESIAN_POINT('Ctrl Pts',(-55.0461247809745,-49.1902357041462,
0.));
#77401=CARTESIAN_POINT('Ctrl Pts',(-55.0573861615569,-49.2148235365694,
0.));
#77402=CARTESIAN_POINT('Ctrl Pts',(-55.0686400468911,-49.2394544718513,
0.));
#77403=CARTESIAN_POINT('Ctrl Pts',(-55.0798863586986,-49.2641284496496,
0.));
#77404=CARTESIAN_POINT('Ctrl Pts',(-55.0911250188282,-49.2888454096544,
0.));
#77405=CARTESIAN_POINT('Ctrl Pts',(-55.1023559487133,-49.3136052912614,
0.));
#77406=CARTESIAN_POINT('Ctrl Pts',(-55.1135790689475,-49.3384080333166,
0.));
#77407=CARTESIAN_POINT('Ctrl Pts',(-55.1247942985649,-49.3632535736744,
0.));
#77408=CARTESIAN_POINT('Ctrl Pts',(-55.1360015556262,-49.3881418495529,
0.));
#77409=CARTESIAN_POINT('Ctrl Pts',(-55.1472007585224,-49.413072798324,0.));
#77410=CARTESIAN_POINT('Ctrl Pts',(-55.158391827114,-49.4380463581989,0.));
#77411=CARTESIAN_POINT('Ctrl Pts',(-55.1695746838168,-49.4630624688787,
0.));
#77412=CARTESIAN_POINT('Ctrl Pts',(-55.1807492550073,-49.4881210723921,
0.));
#77413=CARTESIAN_POINT('Ctrl Pts',(-55.1919154713569,-49.5132221132916,
0.));
#77414=CARTESIAN_POINT('Ctrl Pts',(-55.2014798623975,-49.5347748994607,
0.));
#77415=CARTESIAN_POINT('Ctrl Pts',(-55.2088081098955,-49.5513218524279,
0.));
#77416=CARTESIAN_POINT('Ctrl Pts',(-55.2139039604569,-49.5628442141869,
0.));
#77417=CARTESIAN_POINT('Ctrl Pts',(-55.2167699151168,-49.5693295981608,
0.));
#77418=CARTESIAN_POINT('Ctrl Pts',(-55.2174072001297,-49.5707719660254,
0.));
#77419=CARTESIAN_POINT('',(-53.0702932034641,-45.6458539113724,12.));
#77420=CARTESIAN_POINT('',(-53.0702932034641,-45.6458539113724,0.));
#77421=CARTESIAN_POINT('Ctrl Pts',(-55.2174072001297,-49.5707719660254,
12.));
#77422=CARTESIAN_POINT('Ctrl Pts',(-55.2167699151168,-49.5693295981608,
12.));
#77423=CARTESIAN_POINT('Ctrl Pts',(-55.2139039604569,-49.5628442141869,
12.));
#77424=CARTESIAN_POINT('Ctrl Pts',(-55.2088081098955,-49.5513218524279,
12.));
#77425=CARTESIAN_POINT('Ctrl Pts',(-55.2014798623975,-49.5347748994607,
12.));
#77426=CARTESIAN_POINT('Ctrl Pts',(-55.1919154713569,-49.5132221132916,
12.));
#77427=CARTESIAN_POINT('Ctrl Pts',(-55.1807492550073,-49.4881210723921,
12.));
#77428=CARTESIAN_POINT('Ctrl Pts',(-55.1695746838168,-49.4630624688787,
12.));
#77429=CARTESIAN_POINT('Ctrl Pts',(-55.158391827114,-49.4380463581989,12.));
#77430=CARTESIAN_POINT('Ctrl Pts',(-55.1472007585224,-49.413072798324,12.));
#77431=CARTESIAN_POINT('Ctrl Pts',(-55.1360015556262,-49.3881418495529,
12.));
#77432=CARTESIAN_POINT('Ctrl Pts',(-55.1247942985649,-49.3632535736744,
12.));
#77433=CARTESIAN_POINT('Ctrl Pts',(-55.1135790689475,-49.3384080333166,
12.));
#77434=CARTESIAN_POINT('Ctrl Pts',(-55.1023559487133,-49.3136052912614,
12.));
#77435=CARTESIAN_POINT('Ctrl Pts',(-55.0911250188282,-49.2888454096544,
12.));
#77436=CARTESIAN_POINT('Ctrl Pts',(-55.0798863586986,-49.2641284496496,
12.));
#77437=CARTESIAN_POINT('Ctrl Pts',(-55.0686400468911,-49.2394544718513,
12.));
#77438=CARTESIAN_POINT('Ctrl Pts',(-55.0573861615569,-49.2148235365694,
12.));
#77439=CARTESIAN_POINT('Ctrl Pts',(-55.0461247809745,-49.1902357041462,
12.));
#77440=CARTESIAN_POINT('Ctrl Pts',(-55.0348559840462,-49.1656910352484,
12.));
#77441=CARTESIAN_POINT('Ctrl Pts',(-55.0235798508056,-49.1411895911646,
12.));
#77442=CARTESIAN_POINT('Ctrl Pts',(-55.0122964621868,-49.1167314336737,
12.));
#77443=CARTESIAN_POINT('Ctrl Pts',(-55.0010058998111,-49.0923166249222,
12.));
#77444=CARTESIAN_POINT('Ctrl Pts',(-54.9897082457606,-49.0679452272871,
12.));
#77445=CARTESIAN_POINT('Ctrl Pts',(-54.9784035823764,-49.0436173032527,
12.));
#77446=CARTESIAN_POINT('Ctrl Pts',(-54.9670919920024,-49.0193329152475,
12.));
#77447=CARTESIAN_POINT('Ctrl Pts',(-54.9557735569936,-48.995092125652,12.));
#77448=CARTESIAN_POINT('Ctrl Pts',(-54.9444483598372,-48.9708949968789,
12.));
#77449=CARTESIAN_POINT('Ctrl Pts',(-54.933116483242,-48.9467415914266,12.));
#77450=CARTESIAN_POINT('Ctrl Pts',(-54.9217780102357,-48.922631971937,12.));
#77451=CARTESIAN_POINT('Ctrl Pts',(-54.910433024275,-48.8985662012535,12.));
#77452=CARTESIAN_POINT('Ctrl Pts',(-54.8990816092964,-48.8745443424488,
12.));
#77453=CARTESIAN_POINT('Ctrl Pts',(-54.8877238496577,-48.8505664587985,
12.));
#77454=CARTESIAN_POINT('Ctrl Pts',(-54.8763598301045,-48.8266326137629,
12.));
#77455=CARTESIAN_POINT('Ctrl Pts',(-54.8649896357284,-48.8027428709613,
12.));
#77456=CARTESIAN_POINT('Ctrl Pts',(-54.8536133519285,-48.7788972941431,
12.));
#77457=CARTESIAN_POINT('Ctrl Pts',(-54.8422310643752,-48.755095947159,12.));
#77458=CARTESIAN_POINT('Ctrl Pts',(-54.8308428590334,-48.7313388939834,
12.));
#77459=CARTESIAN_POINT('Ctrl Pts',(-54.8194488221803,-48.7076261987284,
12.));
#77460=CARTESIAN_POINT('Ctrl Pts',(-54.8080490404274,-48.6839579256565,
12.));
#77461=CARTESIAN_POINT('Ctrl Pts',(-54.7966436007395,-48.6603341391891,
12.));
#77462=CARTESIAN_POINT('Ctrl Pts',(-54.7852325904591,-48.6367549039121,
12.));
#77463=CARTESIAN_POINT('Ctrl Pts',(-54.773816097304,-48.6132202845792,12.));
#77464=CARTESIAN_POINT('Ctrl Pts',(-54.7623942093591,-48.5897303461131,
12.));
#77465=CARTESIAN_POINT('Ctrl Pts',(-54.7509670150716,-48.5662851536027,
12.));
#77466=CARTESIAN_POINT('Ctrl Pts',(-54.7395346032451,-48.5428847722975,
12.));
#77467=CARTESIAN_POINT('Ctrl Pts',(-54.7280970630346,-48.5195292675955,
12.));
#77468=CARTESIAN_POINT('Ctrl Pts',(-54.7166544839475,-48.4962187050452,
12.));
#77469=CARTESIAN_POINT('Ctrl Pts',(-54.7052069558493,-48.4729531503565,
12.));
#77470=CARTESIAN_POINT('Ctrl Pts',(-54.6937545689694,-48.4497326694051,
12.));
#77471=CARTESIAN_POINT('Ctrl Pts',(-54.6822974139065,-48.4265573282342,
12.));
#77472=CARTESIAN_POINT('Ctrl Pts',(-54.6708355816359,-48.4034271930516,
12.));
#77473=CARTESIAN_POINT('Ctrl Pts',(-54.6593691635143,-48.3803423302294,
12.));
#77474=CARTESIAN_POINT('Ctrl Pts',(-54.647898251279,-48.3573028063122,12.));
#77475=CARTESIAN_POINT('Ctrl Pts',(-54.636422937049,-48.3343086880192,12.));
#77476=CARTESIAN_POINT('Ctrl Pts',(-54.6249433133262,-48.3113600422443,
12.));
#77477=CARTESIAN_POINT('Ctrl Pts',(-54.6134594729964,-48.288456936051,12.));
#77478=CARTESIAN_POINT('Ctrl Pts',(-54.6019715093319,-48.2655994366672,
12.));
#77479=CARTESIAN_POINT('Ctrl Pts',(-54.5904795159936,-48.2427876114956,
12.));
#77480=CARTESIAN_POINT('Ctrl Pts',(-54.5789835870348,-48.2200215281178,
12.));
#77481=CARTESIAN_POINT('Ctrl Pts',(-54.5674838169041,-48.1973012542966,
12.));
#77482=CARTESIAN_POINT('Ctrl Pts',(-54.5559803004487,-48.1746268579732,
12.));
#77483=CARTESIAN_POINT('Ctrl Pts',(-54.5444731329196,-48.1519984072617,
12.));
#77484=CARTESIAN_POINT('Ctrl Pts',(-54.5329624099719,-48.1294159704571,
12.));
#77485=CARTESIAN_POINT('Ctrl Pts',(-54.5214482276679,-48.1068796160406,
12.));
#77486=CARTESIAN_POINT('Ctrl Pts',(-54.5099306824788,-48.0843894126807,
12.));
#77487=CARTESIAN_POINT('Ctrl Pts',(-54.4984098712883,-48.0619454292321,
12.));
#77488=CARTESIAN_POINT('Ctrl Pts',(-54.4868858913961,-48.039547734729,12.));
#77489=CARTESIAN_POINT('Ctrl Pts',(-54.4753588405202,-48.0171963983912,
12.));
#77490=CARTESIAN_POINT('Ctrl Pts',(-54.4638288167991,-47.9948914896316,
12.));
#77491=CARTESIAN_POINT('Ctrl Pts',(-54.4522959187952,-47.972633078057,12.));
#77492=CARTESIAN_POINT('Ctrl Pts',(-54.4407602454974,-47.9504212334681,
12.));
#77493=CARTESIAN_POINT('Ctrl Pts',(-54.4292218963253,-47.9282560258528,
12.));
#77494=CARTESIAN_POINT('Ctrl Pts',(-54.4176809711324,-47.9061375253909,
12.));
#77495=CARTESIAN_POINT('Ctrl Pts',(-54.4061375702088,-47.8840658024626,
12.));
#77496=CARTESIAN_POINT('Ctrl Pts',(-54.3945917942835,-47.8620409276495,
12.));
#77497=CARTESIAN_POINT('Ctrl Pts',(-54.3830437445275,-47.8400629717352,
12.));
#77498=CARTESIAN_POINT('Ctrl Pts',(-54.3714935225585,-47.8181320056988,
12.));
#77499=CARTESIAN_POINT('Ctrl Pts',(-54.3599412304431,-47.7962481007179,
12.));
#77500=CARTESIAN_POINT('Ctrl Pts',(-54.3483869706998,-47.7744113281768,
12.));
#77501=CARTESIAN_POINT('Ctrl Pts',(-54.3368308463023,-47.7526217596694,
12.));
#77502=CARTESIAN_POINT('Ctrl Pts',(-54.3252729606824,-47.7308794669994,
12.));
#77503=CARTESIAN_POINT('Ctrl Pts',(-54.3137134177345,-47.7091845221748,
12.));
#77504=CARTESIAN_POINT('Ctrl Pts',(-54.3021523218188,-47.6875369974086,
12.));
#77505=CARTESIAN_POINT('Ctrl Pts',(-54.2905897777647,-47.6659369651299,
12.));
#77506=CARTESIAN_POINT('Ctrl Pts',(-54.2790258908736,-47.6443844979846,
12.));
#77507=CARTESIAN_POINT('Ctrl Pts',(-54.2674607669228,-47.6228796688376,
12.));
#77508=CARTESIAN_POINT('Ctrl Pts',(-54.2558945121684,-47.6014225507664,
12.));
#77509=CARTESIAN_POINT('Ctrl Pts',(-54.2443272333498,-47.5800132170614,
12.));
#77510=CARTESIAN_POINT('Ctrl Pts',(-54.232759037693,-47.5586517412368,12.));
#77511=CARTESIAN_POINT('Ctrl Pts',(-54.2211900329141,-47.5373381970328,
12.));
#77512=CARTESIAN_POINT('Ctrl Pts',(-54.2096203272228,-47.5160726584172,
12.));
#77513=CARTESIAN_POINT('Ctrl Pts',(-54.1980500293267,-47.4948551995799,
12.));
#77514=CARTESIAN_POINT('Ctrl Pts',(-54.1864792484343,-47.473685894932,12.));
#77515=CARTESIAN_POINT('Ctrl Pts',(-54.1749080942593,-47.4525648191173,
12.));
#77516=CARTESIAN_POINT('Ctrl Pts',(-54.163336677024,-47.4314920470142,12.));
#77517=CARTESIAN_POINT('Ctrl Pts',(-54.1517651074638,-47.4104676537381,
12.));
#77518=CARTESIAN_POINT('Ctrl Pts',(-54.1401934968306,-47.3894917146361,
12.));
#77519=CARTESIAN_POINT('Ctrl Pts',(-54.1286219568981,-47.3685643052867,
12.));
#77520=CARTESIAN_POINT('Ctrl Pts',(-54.1170505999637,-47.3476855015095,
12.));
#77521=CARTESIAN_POINT('Ctrl Pts',(-54.1054795388538,-47.326855379369,12.));
#77522=CARTESIAN_POINT('Ctrl Pts',(-54.0939088869271,-47.3060740151754,
12.));
#77523=CARTESIAN_POINT('Ctrl Pts',(-54.082338758079,-47.2853414854805,12.));
#77524=CARTESIAN_POINT('Ctrl Pts',(-54.0707692667461,-47.2646578670767,
12.));
#77525=CARTESIAN_POINT('Ctrl Pts',(-54.0592005279108,-47.2440232370085,
12.));
#77526=CARTESIAN_POINT('Ctrl Pts',(-54.047632657105,-47.2234376725752,12.));
#77527=CARTESIAN_POINT('Ctrl Pts',(-54.0360657704156,-47.2029012513334,
12.));
#77528=CARTESIAN_POINT('Ctrl Pts',(-54.0244999844872,-47.1824140510906,
12.));
#77529=CARTESIAN_POINT('Ctrl Pts',(-54.0129354165269,-47.161976149906,12.));
#77530=CARTESIAN_POINT('Ctrl Pts',(-54.0013721843094,-47.1415876261012,
12.));
#77531=CARTESIAN_POINT('Ctrl Pts',(-53.9898104061809,-47.1212485582632,
12.));
#77532=CARTESIAN_POINT('Ctrl Pts',(-53.9782502010642,-47.1009590252466,
12.));
#77533=CARTESIAN_POINT('Ctrl Pts',(-53.9666916884624,-47.0807191061674,
12.));
#77534=CARTESIAN_POINT('Ctrl Pts',(-53.9551349884637,-47.0605288804042,
12.));
#77535=CARTESIAN_POINT('Ctrl Pts',(-53.9435802217468,-47.04038842761,12.));
#77536=CARTESIAN_POINT('Ctrl Pts',(-53.9320275095864,-47.0202978277148,
12.));
#77537=CARTESIAN_POINT('Ctrl Pts',(-53.9204769738584,-47.0002571609286,
12.));
#77538=CARTESIAN_POINT('Ctrl Pts',(-53.9089287370436,-46.9802665077342,
12.));
#77539=CARTESIAN_POINT('Ctrl Pts',(-53.8973829222317,-46.9603259488894,
12.));
#77540=CARTESIAN_POINT('Ctrl Pts',(-53.8858396531277,-46.9404355654381,
12.));
#77541=CARTESIAN_POINT('Ctrl Pts',(-53.8742990540557,-46.9205954387128,
12.));
#77542=CARTESIAN_POINT('Ctrl Pts',(-53.8627612499648,-46.900805650336,12.));
#77543=CARTESIAN_POINT('Ctrl Pts',(-53.851226366434,-46.8810662822147,12.));
#77544=CARTESIAN_POINT('Ctrl Pts',(-53.8396945296777,-46.8613774165452,
12.));
#77545=CARTESIAN_POINT('Ctrl Pts',(-53.8281658665517,-46.8417391358231,
12.));
#77546=CARTESIAN_POINT('Ctrl Pts',(-53.8166405045582,-46.8221515228459,
12.));
#77547=CARTESIAN_POINT('Ctrl Pts',(-53.8051185718525,-46.8026146607144,
12.));
#77548=CARTESIAN_POINT('Ctrl Pts',(-53.7936001972468,-46.7831286328268,
12.));
#77549=CARTESIAN_POINT('Ctrl Pts',(-53.782085510217,-46.7636935228851,12.));
#77550=CARTESIAN_POINT('Ctrl Pts',(-53.770574640907,-46.7443094149041,12.));
#77551=CARTESIAN_POINT('Ctrl Pts',(-53.7590677201344,-46.724976393213,12.));
#77552=CARTESIAN_POINT('Ctrl Pts',(-53.7475648793948,-46.7056945424559,
12.));
#77553=CARTESIAN_POINT('Ctrl Pts',(-53.7360662508677,-46.6864639475863,
12.));
#77554=CARTESIAN_POINT('Ctrl Pts',(-53.7245719674222,-46.6672846938752,
12.));
#77555=CARTESIAN_POINT('Ctrl Pts',(-53.7130821626263,-46.6481568669216,
12.));
#77556=CARTESIAN_POINT('Ctrl Pts',(-53.701596970754,-46.6290805526559,12.));
#77557=CARTESIAN_POINT('Ctrl Pts',(-53.6901165267941,-46.6100558373402,
12.));
#77558=CARTESIAN_POINT('Ctrl Pts',(-53.678640966456,-46.5910828075653,12.));
#77559=CARTESIAN_POINT('Ctrl Pts',(-53.6671704261737,-46.5721615502591,
12.));
#77560=CARTESIAN_POINT('Ctrl Pts',(-53.6557050431071,-46.5532921526901,
12.));
#77561=CARTESIAN_POINT('Ctrl Pts',(-53.6442449551455,-46.5344747024676,
12.));
#77562=CARTESIAN_POINT('Ctrl Pts',(-53.6327903009094,-46.5157092875373,
12.));
#77563=CARTESIAN_POINT('Ctrl Pts',(-53.6213412197533,-46.496995996177,12.));
#77564=CARTESIAN_POINT('Ctrl Pts',(-53.6098978517859,-46.4783349170173,
12.));
#77565=CARTESIAN_POINT('Ctrl Pts',(-53.5984603378855,-46.459726139052,12.));
#77566=CARTESIAN_POINT('Ctrl Pts',(-53.5870288197166,-46.4411697516478,
12.));
#77567=CARTESIAN_POINT('Ctrl Pts',(-53.5756034397481,-46.4226658445474,
12.));
#77568=CARTESIAN_POINT('Ctrl Pts',(-53.5641843412559,-46.4042145078701,
12.));
#77569=CARTESIAN_POINT('Ctrl Pts',(-53.5527716683048,-46.3858158321059,
12.));
#77570=CARTESIAN_POINT('Ctrl Pts',(-53.5413655657327,-46.3674699081046,
12.));
#77571=CARTESIAN_POINT('Ctrl Pts',(-53.5299661791385,-46.3491768270655,
12.));
#77572=CARTESIAN_POINT('Ctrl Pts',(-53.5185736548548,-46.3309366805093,
12.));
#77573=CARTESIAN_POINT('Ctrl Pts',(-53.5071881399911,-46.3127495603098,
12.));
#77574=CARTESIAN_POINT('Ctrl Pts',(-53.4958097825006,-46.2946155587417,
12.));
#77575=CARTESIAN_POINT('Ctrl Pts',(-53.4844387312414,-46.2765347685198,
12.));
#77576=CARTESIAN_POINT('Ctrl Pts',(-53.4730751360371,-46.2585072828353,
12.));
#77577=CARTESIAN_POINT('Ctrl Pts',(-53.4617191477402,-46.2405331953889,
12.));
#77578=CARTESIAN_POINT('Ctrl Pts',(-53.4503709181178,-46.2226126003202,
12.));
#77579=CARTESIAN_POINT('Ctrl Pts',(-53.4390305997274,-46.2047455921286,
12.));
#77580=CARTESIAN_POINT('Ctrl Pts',(-53.4276983458125,-46.1869322656024,
12.));
#77581=CARTESIAN_POINT('Ctrl Pts',(-53.4163743101517,-46.1691727157134,
12.));
#77582=CARTESIAN_POINT('Ctrl Pts',(-53.4050586470436,-46.1514670376012,
12.));
#77583=CARTESIAN_POINT('Ctrl Pts',(-53.3937515116549,-46.1338153268097,
12.));
#77584=CARTESIAN_POINT('Ctrl Pts',(-53.3824530603276,-46.1162176794884,
12.));
#77585=CARTESIAN_POINT('Ctrl Pts',(-53.3711634508437,-46.0986741925656,
12.));
#77586=CARTESIAN_POINT('Ctrl Pts',(-53.3598828428546,-46.0811849640218,
12.));
#77587=CARTESIAN_POINT('Ctrl Pts',(-53.3486113975901,-46.0637500926982,
12.));
#77588=CARTESIAN_POINT('Ctrl Pts',(-53.3373492770671,-46.0463696777801,
12.));
#77589=CARTESIAN_POINT('Ctrl Pts',(-53.326096643428,-46.02904381836,12.));
#77590=CARTESIAN_POINT('Ctrl Pts',(-53.3148536582635,-46.0117726129873,
12.));
#77591=CARTESIAN_POINT('Ctrl Pts',(-53.3036204818329,-45.9945561591453,
12.));
#77592=CARTESIAN_POINT('Ctrl Pts',(-53.292397274555,-45.9773945542384,12.));
#77593=CARTESIAN_POINT('Ctrl Pts',(-53.2811841987926,-45.9602878967698,
12.));
#77594=CARTESIAN_POINT('Ctrl Pts',(-53.2699814203105,-45.9432362873008,
12.));
#77595=CARTESIAN_POINT('Ctrl Pts',(-53.2587891103866,-45.9262398298349,
12.));
#77596=CARTESIAN_POINT('Ctrl Pts',(-53.2476074460017,-45.9092986319377,
12.));
#77597=CARTESIAN_POINT('Ctrl Pts',(-53.2364366054306,-45.892412801838,12.));
#77598=CARTESIAN_POINT('Ctrl Pts',(-53.2252767643662,-45.8755824458723,
12.));
#77599=CARTESIAN_POINT('Ctrl Pts',(-53.2141280925439,-45.8588076662582,
12.));
#77600=CARTESIAN_POINT('Ctrl Pts',(-53.2029907483557,-45.8420885575349,
12.));
#77601=CARTESIAN_POINT('Ctrl Pts',(-53.1918648840541,-45.8254252099957,
12.));
#77602=CARTESIAN_POINT('Ctrl Pts',(-53.1807506560933,-45.808817716509,12.));
#77603=CARTESIAN_POINT('Ctrl Pts',(-53.1696482334487,-45.7922661780005,
12.));
#77604=CARTESIAN_POINT('Ctrl Pts',(-53.1585578076444,-45.7757707100618,
12.));
#77605=CARTESIAN_POINT('Ctrl Pts',(-53.1474795996053,-45.7593314474501,
12.));
#77606=CARTESIAN_POINT('Ctrl Pts',(-53.1364138384693,-45.7429485300823,
12.));
#77607=CARTESIAN_POINT('Ctrl Pts',(-53.1253607414872,-45.7266220897003,
12.));
#77608=CARTESIAN_POINT('Ctrl Pts',(-53.114320495492,-45.7103522376696,12.));
#77609=CARTESIAN_POINT('Ctrl Pts',(-53.1032932328857,-45.694139048907,12.));
#77610=CARTESIAN_POINT('Ctrl Pts',(-53.0922790298409,-45.6779825614231,
12.));
#77611=CARTESIAN_POINT('Ctrl Pts',(-53.0834781451546,-45.6651027439241,
12.));
#77612=CARTESIAN_POINT('Ctrl Pts',(-53.0768833804193,-45.6554684028145,
12.));
#77613=CARTESIAN_POINT('Ctrl Pts',(-53.0724894921849,-45.6490568514089,
12.));
#77614=CARTESIAN_POINT('Ctrl Pts',(-53.0702932034641,-45.6458539113724,
12.));
#77615=CARTESIAN_POINT('Ctrl Pts',(-54.1946543500373,-50.6869108458851,
-1.11022302462516E-15));
#77616=CARTESIAN_POINT('Ctrl Pts',(-54.1946543500373,-50.6869108458851,
4.));
#77617=CARTESIAN_POINT('Ctrl Pts',(-54.1946543500373,-50.6869108458851,
8.));
#77618=CARTESIAN_POINT('Ctrl Pts',(-54.1946543500373,-50.6869108458851,
12.));
#77619=CARTESIAN_POINT('Ctrl Pts',(-54.2986513683568,-50.7223900873023,
-1.11022302462516E-15));
#77620=CARTESIAN_POINT('Ctrl Pts',(-54.2986513683568,-50.7223900873023,
4.));
#77621=CARTESIAN_POINT('Ctrl Pts',(-54.2986513683568,-50.7223900873023,
8.));
#77622=CARTESIAN_POINT('Ctrl Pts',(-54.2986513683568,-50.7223900873023,
12.));
#77623=CARTESIAN_POINT('Ctrl Pts',(-54.5013145669267,-50.7219766588197,
-1.03713937562159E-15));
#77624=CARTESIAN_POINT('Ctrl Pts',(-54.5013145669267,-50.7219766588197,
4.));
#77625=CARTESIAN_POINT('Ctrl Pts',(-54.5013145669267,-50.7219766588197,
7.99999999999999));
#77626=CARTESIAN_POINT('Ctrl Pts',(-54.5013145669267,-50.7219766588197,
12.));
#77627=CARTESIAN_POINT('Ctrl Pts',(-54.6674453828701,-50.6135081477658,
-8.63611844427818E-16));
#77628=CARTESIAN_POINT('Ctrl Pts',(-54.6674453828701,-50.6135081477658,
4.));
#77629=CARTESIAN_POINT('Ctrl Pts',(-54.6674453828701,-50.6135081477658,
8.));
#77630=CARTESIAN_POINT('Ctrl Pts',(-54.6674453828701,-50.6135081477658,
12.));
#77631=CARTESIAN_POINT('Ctrl Pts',(-54.7233670476834,-50.55297319609,-7.79957864200068E-16));
#77632=CARTESIAN_POINT('Ctrl Pts',(-54.7233670476834,-50.55297319609,4.));
#77633=CARTESIAN_POINT('Ctrl Pts',(-54.7233670476834,-50.55297319609,8.));
#77634=CARTESIAN_POINT('Ctrl Pts',(-54.7233670476834,-50.55297319609,12.));
#77635=CARTESIAN_POINT('',(-54.1946543500373,-50.6869108458851,0.));
#77636=CARTESIAN_POINT('',(-54.723367047683,-50.5529731960897,0.));
#77637=CARTESIAN_POINT('Ctrl Pts',(-54.1946543500373,-50.6869108458851,
8.74764948622162E-18));
#77638=CARTESIAN_POINT('Ctrl Pts',(-54.2986513683568,-50.7223900873023,
8.74764948622131E-18));
#77639=CARTESIAN_POINT('Ctrl Pts',(-54.4144589103968,-50.7221538424551,
5.05097346311187E-17));
#77640=CARTESIAN_POINT('Ctrl Pts',(-54.5183375111709,-50.6866343053397,
1.25069822123835E-16));
#77641=CARTESIAN_POINT('Ctrl Pts',(-54.5962464617515,-50.6599946525032,
1.80989887743373E-16));
#77642=CARTESIAN_POINT('Ctrl Pts',(-54.6674453828701,-50.6135081477658,
2.55358829683559E-16));
#77643=CARTESIAN_POINT('Ctrl Pts',(-54.7233670476834,-50.55297319609,3.3901280991131E-16));
#77644=CARTESIAN_POINT('',(-54.723367047683,-50.5529731960897,12.));
#77645=CARTESIAN_POINT('Ctrl Pts',(-54.7233670476834,-50.55297319609,-7.79957864200068E-16));
#77646=CARTESIAN_POINT('Ctrl Pts',(-54.7233670476834,-50.55297319609,4.));
#77647=CARTESIAN_POINT('Ctrl Pts',(-54.7233670476834,-50.55297319609,8.));
#77648=CARTESIAN_POINT('Ctrl Pts',(-54.7233670476834,-50.55297319609,12.));
#77649=CARTESIAN_POINT('',(-54.1946543500373,-50.6869108458851,12.));
#77650=CARTESIAN_POINT('Ctrl Pts',(-54.7233670476834,-50.55297319609,12.));
#77651=CARTESIAN_POINT('Ctrl Pts',(-54.6674453828701,-50.6135081477658,
12.));
#77652=CARTESIAN_POINT('Ctrl Pts',(-54.5962464617515,-50.6599946525032,
12.));
#77653=CARTESIAN_POINT('Ctrl Pts',(-54.5183375111709,-50.6866343053397,
12.));
#77654=CARTESIAN_POINT('Ctrl Pts',(-54.4144589103968,-50.7221538424551,
12.));
#77655=CARTESIAN_POINT('Ctrl Pts',(-54.2986513683568,-50.7223900873023,
12.));
#77656=CARTESIAN_POINT('Ctrl Pts',(-54.1946543500373,-50.6869108458851,
12.));
#77657=CARTESIAN_POINT('Ctrl Pts',(-54.1946543500373,-50.6869108458851,
12.));
#77658=CARTESIAN_POINT('Ctrl Pts',(-54.1946543500373,-50.6869108458851,
8.));
#77659=CARTESIAN_POINT('Ctrl Pts',(-54.1946543500373,-50.6869108458851,
4.));
#77660=CARTESIAN_POINT('Ctrl Pts',(-54.1946543500373,-50.6869108458851,
-1.11022302462516E-15));
#77661=CARTESIAN_POINT('Origin',(-2.7629675461203E-10,-2.53313958019842E-10,
0.));
#77662=CARTESIAN_POINT('Origin',(-2.7629675461203E-10,-2.53313958019842E-10,
12.));
#77663=CARTESIAN_POINT('Origin',(-2.7629675461203E-10,-2.53313958019842E-10,
0.));
#77664=CARTESIAN_POINT('Ctrl Pts',(-59.2875729049545,-45.1135644683471,
-5.55111512312578E-16));
#77665=CARTESIAN_POINT('Ctrl Pts',(-59.2875729049545,-45.1135644683471,
4.));
#77666=CARTESIAN_POINT('Ctrl Pts',(-59.2875729049545,-45.113564468347,8.));
#77667=CARTESIAN_POINT('Ctrl Pts',(-59.2875729049545,-45.113564468347,12.));
#77668=CARTESIAN_POINT('Ctrl Pts',(-59.3541123643618,-45.0261193041895,
-5.55111512312578E-16));
#77669=CARTESIAN_POINT('Ctrl Pts',(-59.3541123643618,-45.0261193041895,
4.));
#77670=CARTESIAN_POINT('Ctrl Pts',(-59.3541123643618,-45.0261193041895,
8.));
#77671=CARTESIAN_POINT('Ctrl Pts',(-59.3541123643618,-45.0261193041895,
12.));
#77672=CARTESIAN_POINT('Ctrl Pts',(-59.4177951463802,-44.8337211159574,
-5.55111512312578E-16));
#77673=CARTESIAN_POINT('Ctrl Pts',(-59.4177951463802,-44.8337211159574,
4.));
#77674=CARTESIAN_POINT('Ctrl Pts',(-59.4177951463802,-44.8337211159573,
8.));
#77675=CARTESIAN_POINT('Ctrl Pts',(-59.4177951463802,-44.8337211159573,
12.));
#77676=CARTESIAN_POINT('Ctrl Pts',(-59.3674150879747,-44.6418181989797,
-5.55111512312578E-16));
#77677=CARTESIAN_POINT('Ctrl Pts',(-59.3674150879747,-44.6418181989797,
4.));
#77678=CARTESIAN_POINT('Ctrl Pts',(-59.3674150879747,-44.6418181989796,
8.00000000000001));
#77679=CARTESIAN_POINT('Ctrl Pts',(-59.3674150879747,-44.6418181989796,
12.));
#77680=CARTESIAN_POINT('Ctrl Pts',(-59.3276657444156,-44.5696260757421,
-5.55111512312578E-16));
#77681=CARTESIAN_POINT('Ctrl Pts',(-59.3276657444156,-44.5696260757421,
4.));
#77682=CARTESIAN_POINT('Ctrl Pts',(-59.3276657444156,-44.5696260757421,
8.));
#77683=CARTESIAN_POINT('Ctrl Pts',(-59.3276657444156,-44.5696260757421,
12.));
#77684=CARTESIAN_POINT('',(-59.2875729049545,-45.1135644683471,0.));
#77685=CARTESIAN_POINT('',(-59.3276657444158,-44.5696260757421,0.));
#77686=CARTESIAN_POINT('Ctrl Pts',(-59.2875729049545,-45.1135644683471,
-5.55111512312578E-16));
#77687=CARTESIAN_POINT('Ctrl Pts',(-59.3541123643618,-45.0261193041895,
-5.55111512312578E-16));
#77688=CARTESIAN_POINT('Ctrl Pts',(-59.3905025255151,-44.9161774823426,
-5.55111512312578E-16));
#77689=CARTESIAN_POINT('Ctrl Pts',(-59.3896476775505,-44.8063973817216,
-5.55111512312578E-16));
#77690=CARTESIAN_POINT('Ctrl Pts',(-59.389006541577,-44.7240623062559,-5.55111512312578E-16));
#77691=CARTESIAN_POINT('Ctrl Pts',(-59.3674150879747,-44.6418181989797,
-5.55111512312578E-16));
#77692=CARTESIAN_POINT('Ctrl Pts',(-59.3276657444156,-44.5696260757421,
-5.55111512312578E-16));
#77693=CARTESIAN_POINT('',(-59.3276657444158,-44.569626075742,12.));
#77694=CARTESIAN_POINT('Ctrl Pts',(-59.3276657444156,-44.5696260757421,
-5.55111512312578E-16));
#77695=CARTESIAN_POINT('Ctrl Pts',(-59.3276657444156,-44.5696260757421,
4.));
#77696=CARTESIAN_POINT('Ctrl Pts',(-59.3276657444156,-44.5696260757421,
8.));
#77697=CARTESIAN_POINT('Ctrl Pts',(-59.3276657444156,-44.5696260757421,
12.));
#77698=CARTESIAN_POINT('',(-59.2875729049545,-45.113564468347,12.));
#77699=CARTESIAN_POINT('Ctrl Pts',(-59.3276657444156,-44.5696260757421,
12.));
#77700=CARTESIAN_POINT('Ctrl Pts',(-59.3674150879747,-44.6418181989796,
12.));
#77701=CARTESIAN_POINT('Ctrl Pts',(-59.3890065415771,-44.7240623062558,
12.));
#77702=CARTESIAN_POINT('Ctrl Pts',(-59.3896476775505,-44.8063973817216,
12.));
#77703=CARTESIAN_POINT('Ctrl Pts',(-59.3905025255152,-44.9161774823425,
12.));
#77704=CARTESIAN_POINT('Ctrl Pts',(-59.3541123643618,-45.0261193041895,
12.));
#77705=CARTESIAN_POINT('Ctrl Pts',(-59.2875729049545,-45.113564468347,12.));
#77706=CARTESIAN_POINT('Ctrl Pts',(-59.2875729049545,-45.113564468347,12.));
#77707=CARTESIAN_POINT('Ctrl Pts',(-59.2875729049545,-45.113564468347,8.));
#77708=CARTESIAN_POINT('Ctrl Pts',(-59.2875729049545,-45.1135644683471,
4.));
#77709=CARTESIAN_POINT('Ctrl Pts',(-59.2875729049545,-45.1135644683471,
-5.55111512312578E-16));
#77710=CARTESIAN_POINT('Ctrl Pts',(-56.8466430164621,-40.8467768343956,
0.));
#77711=CARTESIAN_POINT('Ctrl Pts',(-56.8466430164621,-40.8467768343956,
12.));
#77712=CARTESIAN_POINT('Ctrl Pts',(-56.8491101022591,-40.8497761671036,
0.));
#77713=CARTESIAN_POINT('Ctrl Pts',(-56.8491101022591,-40.8497761671036,
12.));
#77714=CARTESIAN_POINT('Ctrl Pts',(-56.8540460739472,-40.8557803680277,
0.));
#77715=CARTESIAN_POINT('Ctrl Pts',(-56.8540460739472,-40.8557803680277,
12.));
#77716=CARTESIAN_POINT('Ctrl Pts',(-56.8614554317668,-40.864803275942,0.));
#77717=CARTESIAN_POINT('Ctrl Pts',(-56.8614554317668,-40.864803275942,12.));
#77718=CARTESIAN_POINT('Ctrl Pts',(-56.8713453764905,-40.8768670342052,
0.));
#77719=CARTESIAN_POINT('Ctrl Pts',(-56.8713453764905,-40.8768670342052,
12.));
#77720=CARTESIAN_POINT('Ctrl Pts',(-56.8837257978343,-40.8920020903293,
0.));
#77721=CARTESIAN_POINT('Ctrl Pts',(-56.8837257978343,-40.8920020903293,
12.));
#77722=CARTESIAN_POINT('Ctrl Pts',(-56.8961241708861,-40.9071924937508,
0.));
#77723=CARTESIAN_POINT('Ctrl Pts',(-56.8961241708861,-40.9071924937508,
12.));
#77724=CARTESIAN_POINT('Ctrl Pts',(-56.9085404164502,-40.9224382132427,
0.));
#77725=CARTESIAN_POINT('Ctrl Pts',(-56.9085404164502,-40.9224382132427,
12.));
#77726=CARTESIAN_POINT('Ctrl Pts',(-56.9209743960992,-40.9377391857128,
0.));
#77727=CARTESIAN_POINT('Ctrl Pts',(-56.9209743960992,-40.9377391857128,
12.));
#77728=CARTESIAN_POINT('Ctrl Pts',(-56.9334259140049,-40.9530953165031,
0.));
#77729=CARTESIAN_POINT('Ctrl Pts',(-56.9334259140049,-40.9530953165031,
12.));
#77730=CARTESIAN_POINT('Ctrl Pts',(-56.9458947422608,-40.9685064933074,
0.));
#77731=CARTESIAN_POINT('Ctrl Pts',(-56.9458947422608,-40.9685064933074,
12.));
#77732=CARTESIAN_POINT('Ctrl Pts',(-56.9583806404069,-40.9839725967121,
0.));
#77733=CARTESIAN_POINT('Ctrl Pts',(-56.9583806404069,-40.9839725967121,
12.));
#77734=CARTESIAN_POINT('Ctrl Pts',(-56.9708833766137,-40.9994935117276,
0.));
#77735=CARTESIAN_POINT('Ctrl Pts',(-56.9708833766137,-40.9994935117276,
12.));
#77736=CARTESIAN_POINT('Ctrl Pts',(-56.9834027500117,-41.0150691398947,
0.));
#77737=CARTESIAN_POINT('Ctrl Pts',(-56.9834027500117,-41.0150691398947,
12.));
#77738=CARTESIAN_POINT('Ctrl Pts',(-56.995938583472,-41.0306993953988,0.));
#77739=CARTESIAN_POINT('Ctrl Pts',(-56.995938583472,-41.0306993953988,12.));
#77740=CARTESIAN_POINT('Ctrl Pts',(-57.008490713042,-41.0463841993608,0.));
#77741=CARTESIAN_POINT('Ctrl Pts',(-57.008490713042,-41.0463841993608,12.));
#77742=CARTESIAN_POINT('Ctrl Pts',(-57.0210589791788,-41.0621234751007,
0.));
#77743=CARTESIAN_POINT('Ctrl Pts',(-57.0210589791788,-41.0621234751007,
12.));
#77744=CARTESIAN_POINT('Ctrl Pts',(-57.0336432158536,-41.0779171422438,
0.));
#77745=CARTESIAN_POINT('Ctrl Pts',(-57.0336432158536,-41.0779171422438,
12.));
#77746=CARTESIAN_POINT('Ctrl Pts',(-57.046243245068,-41.0937651137549,0.));
#77747=CARTESIAN_POINT('Ctrl Pts',(-57.046243245068,-41.0937651137549,12.));
#77748=CARTESIAN_POINT('Ctrl Pts',(-57.0588588825298,-41.1096672990148,
0.));
#77749=CARTESIAN_POINT('Ctrl Pts',(-57.0588588825298,-41.1096672990148,
12.));
#77750=CARTESIAN_POINT('Ctrl Pts',(-57.0714899412099,-41.1256236057442,
0.));
#77751=CARTESIAN_POINT('Ctrl Pts',(-57.0714899412099,-41.1256236057442,
12.));
#77752=CARTESIAN_POINT('Ctrl Pts',(-57.084136235426,-41.1416339422117,0.));
#77753=CARTESIAN_POINT('Ctrl Pts',(-57.084136235426,-41.1416339422117,12.));
#77754=CARTESIAN_POINT('Ctrl Pts',(-57.0967975854874,-41.1576982197374,
0.));
#77755=CARTESIAN_POINT('Ctrl Pts',(-57.0967975854874,-41.1576982197374,
12.));
#77756=CARTESIAN_POINT('Ctrl Pts',(-57.1094738174957,-41.1738163525901,
0.));
#77757=CARTESIAN_POINT('Ctrl Pts',(-57.1094738174957,-41.1738163525901,
12.));
#77758=CARTESIAN_POINT('Ctrl Pts',(-57.1221647611207,-41.1899882567923,
0.));
#77759=CARTESIAN_POINT('Ctrl Pts',(-57.1221647611207,-41.1899882567923,
12.));
#77760=CARTESIAN_POINT('Ctrl Pts',(-57.1348702480647,-41.2062138492915,
0.));
#77761=CARTESIAN_POINT('Ctrl Pts',(-57.1348702480647,-41.2062138492915,
12.));
#77762=CARTESIAN_POINT('Ctrl Pts',(-57.147590110182,-41.222493046943,0.));
#77763=CARTESIAN_POINT('Ctrl Pts',(-57.147590110182,-41.222493046943,12.));
#77764=CARTESIAN_POINT('Ctrl Pts',(-57.1603241779077,-41.2388257656559,
0.));
#77765=CARTESIAN_POINT('Ctrl Pts',(-57.1603241779077,-41.2388257656559,
12.));
#77766=CARTESIAN_POINT('Ctrl Pts',(-57.17307228108,-41.2552119208465,0.));
#77767=CARTESIAN_POINT('Ctrl Pts',(-57.17307228108,-41.2552119208465,12.));
#77768=CARTESIAN_POINT('Ctrl Pts',(-57.1858342496538,-41.2716514278276,
0.));
#77769=CARTESIAN_POINT('Ctrl Pts',(-57.1858342496538,-41.2716514278276,
12.));
#77770=CARTESIAN_POINT('Ctrl Pts',(-57.1986099143983,-41.2881442021863,
0.));
#77771=CARTESIAN_POINT('Ctrl Pts',(-57.1986099143983,-41.2881442021863,
12.));
#77772=CARTESIAN_POINT('Ctrl Pts',(-57.2113991077302,-41.3046901602293,
0.));
#77773=CARTESIAN_POINT('Ctrl Pts',(-57.2113991077302,-41.3046901602293,
12.));
#77774=CARTESIAN_POINT('Ctrl Pts',(-57.2242016640198,-41.321289219149,0.));
#77775=CARTESIAN_POINT('Ctrl Pts',(-57.2242016640198,-41.321289219149,12.));
#77776=CARTESIAN_POINT('Ctrl Pts',(-57.2370174191401,-41.3379412967875,
0.));
#77777=CARTESIAN_POINT('Ctrl Pts',(-57.2370174191401,-41.3379412967875,
12.));
#77778=CARTESIAN_POINT('Ctrl Pts',(-57.2498462101879,-41.3546463114885,
0.));
#77779=CARTESIAN_POINT('Ctrl Pts',(-57.2498462101879,-41.3546463114885,
12.));
#77780=CARTESIAN_POINT('Ctrl Pts',(-57.2626878751596,-41.3714041819223,
0.));
#77781=CARTESIAN_POINT('Ctrl Pts',(-57.2626878751596,-41.3714041819223,
12.));
#77782=CARTESIAN_POINT('Ctrl Pts',(-57.2755422525844,-41.3882148268813,
0.));
#77783=CARTESIAN_POINT('Ctrl Pts',(-57.2755422525844,-41.3882148268813,
12.));
#77784=CARTESIAN_POINT('Ctrl Pts',(-57.2884091815406,-41.4050781652938,
0.));
#77785=CARTESIAN_POINT('Ctrl Pts',(-57.2884091815406,-41.4050781652938,
12.));
#77786=CARTESIAN_POINT('Ctrl Pts',(-57.3012885018151,-41.4219941163163,
0.));
#77787=CARTESIAN_POINT('Ctrl Pts',(-57.3012885018151,-41.4219941163163,
12.));
#77788=CARTESIAN_POINT('Ctrl Pts',(-57.3141800540137,-41.4389625993948,
0.));
#77789=CARTESIAN_POINT('Ctrl Pts',(-57.3141800540137,-41.4389625993948,
12.));
#77790=CARTESIAN_POINT('Ctrl Pts',(-57.3270836796911,-41.4559835343328,
0.));
#77791=CARTESIAN_POINT('Ctrl Pts',(-57.3270836796911,-41.4559835343328,
12.));
#77792=CARTESIAN_POINT('Ctrl Pts',(-57.3399992214717,-41.4730568413518,
0.));
#77793=CARTESIAN_POINT('Ctrl Pts',(-57.3399992214717,-41.4730568413518,
12.));
#77794=CARTESIAN_POINT('Ctrl Pts',(-57.3529265229835,-41.4901824410636,
0.));
#77795=CARTESIAN_POINT('Ctrl Pts',(-57.3529265229835,-41.4901824410636,
12.));
#77796=CARTESIAN_POINT('Ctrl Pts',(-57.3658654287937,-41.5073602544396,
0.));
#77797=CARTESIAN_POINT('Ctrl Pts',(-57.3658654287937,-41.5073602544396,
12.));
#77798=CARTESIAN_POINT('Ctrl Pts',(-57.3788157843454,-41.524590202777,0.));
#77799=CARTESIAN_POINT('Ctrl Pts',(-57.3788157843454,-41.524590202777,12.));
#77800=CARTESIAN_POINT('Ctrl Pts',(-57.3917774358863,-41.5418722076572,
0.));
#77801=CARTESIAN_POINT('Ctrl Pts',(-57.3917774358863,-41.5418722076572,
12.));
#77802=CARTESIAN_POINT('Ctrl Pts',(-57.4047502304231,-41.5592061909176,
0.));
#77803=CARTESIAN_POINT('Ctrl Pts',(-57.4047502304231,-41.5592061909176,
12.));
#77804=CARTESIAN_POINT('Ctrl Pts',(-57.4177340157508,-41.5765920746777,
0.));
#77805=CARTESIAN_POINT('Ctrl Pts',(-57.4177340157508,-41.5765920746777,
12.));
#77806=CARTESIAN_POINT('Ctrl Pts',(-57.4307286404662,-41.5940297813477,
0.));
#77807=CARTESIAN_POINT('Ctrl Pts',(-57.4307286404662,-41.5940297813477,
12.));
#77808=CARTESIAN_POINT('Ctrl Pts',(-57.4437339539841,-41.6115192336388,
0.));
#77809=CARTESIAN_POINT('Ctrl Pts',(-57.4437339539841,-41.6115192336388,
12.));
#77810=CARTESIAN_POINT('Ctrl Pts',(-57.4567498065562,-41.6290603545666,
0.));
#77811=CARTESIAN_POINT('Ctrl Pts',(-57.4567498065562,-41.6290603545666,
12.));
#77812=CARTESIAN_POINT('Ctrl Pts',(-57.4697760492683,-41.6466530674514,
0.));
#77813=CARTESIAN_POINT('Ctrl Pts',(-57.4697760492683,-41.6466530674514,
12.));
#77814=CARTESIAN_POINT('Ctrl Pts',(-57.4828125340218,-41.6642972959165,
0.));
#77815=CARTESIAN_POINT('Ctrl Pts',(-57.4828125340218,-41.6642972959165,
12.));
#77816=CARTESIAN_POINT('Ctrl Pts',(-57.4958591135165,-41.6819929638797,
0.));
#77817=CARTESIAN_POINT('Ctrl Pts',(-57.4958591135165,-41.6819929638797,
12.));
#77818=CARTESIAN_POINT('Ctrl Pts',(-57.5089156412343,-41.6997399955447,
0.));
#77819=CARTESIAN_POINT('Ctrl Pts',(-57.5089156412343,-41.6997399955447,
12.));
#77820=CARTESIAN_POINT('Ctrl Pts',(-57.5219819714171,-41.7175383153821,
0.));
#77821=CARTESIAN_POINT('Ctrl Pts',(-57.5219819714171,-41.7175383153821,
12.));
#77822=CARTESIAN_POINT('Ctrl Pts',(-57.5350579590649,-41.7353878481336,
0.));
#77823=CARTESIAN_POINT('Ctrl Pts',(-57.5350579590649,-41.7353878481336,
12.));
#77824=CARTESIAN_POINT('Ctrl Pts',(-57.5481434599335,-41.7532885188174,
0.));
#77825=CARTESIAN_POINT('Ctrl Pts',(-57.5481434599335,-41.7532885188174,
12.));
#77826=CARTESIAN_POINT('Ctrl Pts',(-57.561238330532,-41.7712402527273,0.));
#77827=CARTESIAN_POINT('Ctrl Pts',(-57.561238330532,-41.7712402527273,12.));
#77828=CARTESIAN_POINT('Ctrl Pts',(-57.5743424281205,-41.7892429754297,
0.));
#77829=CARTESIAN_POINT('Ctrl Pts',(-57.5743424281205,-41.7892429754297,
12.));
#77830=CARTESIAN_POINT('Ctrl Pts',(-57.5874556107056,-41.8072966127558,
0.));
#77831=CARTESIAN_POINT('Ctrl Pts',(-57.5874556107056,-41.8072966127558,
12.));
#77832=CARTESIAN_POINT('Ctrl Pts',(-57.6005777370349,-41.8254010908051,
0.));
#77833=CARTESIAN_POINT('Ctrl Pts',(-57.6005777370349,-41.8254010908051,
12.));
#77834=CARTESIAN_POINT('Ctrl Pts',(-57.6137086665882,-41.8435563359456,
0.));
#77835=CARTESIAN_POINT('Ctrl Pts',(-57.6137086665882,-41.8435563359456,
12.));
#77836=CARTESIAN_POINT('Ctrl Pts',(-57.6268482595702,-41.8617622748108,
0.));
#77837=CARTESIAN_POINT('Ctrl Pts',(-57.6268482595702,-41.8617622748108,
12.));
#77838=CARTESIAN_POINT('Ctrl Pts',(-57.6399963769003,-41.8800188342908,
0.));
#77839=CARTESIAN_POINT('Ctrl Pts',(-57.6399963769003,-41.8800188342908,
12.));
#77840=CARTESIAN_POINT('Ctrl Pts',(-57.6531528802059,-41.8983259415244,
0.));
#77841=CARTESIAN_POINT('Ctrl Pts',(-57.6531528802059,-41.8983259415244,
12.));
#77842=CARTESIAN_POINT('Ctrl Pts',(-57.6663176318176,-41.9166835239046,
0.));
#77843=CARTESIAN_POINT('Ctrl Pts',(-57.6663176318176,-41.9166835239046,
12.));
#77844=CARTESIAN_POINT('Ctrl Pts',(-57.6794904947641,-41.9350915090791,
0.));
#77845=CARTESIAN_POINT('Ctrl Pts',(-57.6794904947641,-41.9350915090791,
12.));
#77846=CARTESIAN_POINT('Ctrl Pts',(-57.6926713327674,-41.9535498249489,
0.));
#77847=CARTESIAN_POINT('Ctrl Pts',(-57.6926713327674,-41.9535498249489,
12.));
#77848=CARTESIAN_POINT('Ctrl Pts',(-57.7058600102365,-41.9720583996601,
0.));
#77849=CARTESIAN_POINT('Ctrl Pts',(-57.7058600102365,-41.9720583996601,
12.));
#77850=CARTESIAN_POINT('Ctrl Pts',(-57.7190563922614,-41.9906171615974,
0.));
#77851=CARTESIAN_POINT('Ctrl Pts',(-57.7190563922614,-41.9906171615974,
12.));
#77852=CARTESIAN_POINT('Ctrl Pts',(-57.7322603446086,-42.0092260393911,
0.));
#77853=CARTESIAN_POINT('Ctrl Pts',(-57.7322603446086,-42.0092260393911,
12.));
#77854=CARTESIAN_POINT('Ctrl Pts',(-57.7454717337151,-42.0278849619156,
0.));
#77855=CARTESIAN_POINT('Ctrl Pts',(-57.7454717337151,-42.0278849619156,
12.));
#77856=CARTESIAN_POINT('Ctrl Pts',(-57.7586904266828,-42.0465938582877,
0.));
#77857=CARTESIAN_POINT('Ctrl Pts',(-57.7586904266828,-42.0465938582877,
12.));
#77858=CARTESIAN_POINT('Ctrl Pts',(-57.7719162912721,-42.0653526578571,
0.));
#77859=CARTESIAN_POINT('Ctrl Pts',(-57.7719162912721,-42.0653526578571,
12.));
#77860=CARTESIAN_POINT('Ctrl Pts',(-57.7851491958954,-42.0841612902018,
0.));
#77861=CARTESIAN_POINT('Ctrl Pts',(-57.7851491958954,-42.0841612902018,
12.));
#77862=CARTESIAN_POINT('Ctrl Pts',(-57.798389009613,-42.1030196851344,0.));
#77863=CARTESIAN_POINT('Ctrl Pts',(-57.798389009613,-42.1030196851344,12.));
#77864=CARTESIAN_POINT('Ctrl Pts',(-57.8116356021274,-42.121927772701,0.));
#77865=CARTESIAN_POINT('Ctrl Pts',(-57.8116356021274,-42.121927772701,12.));
#77866=CARTESIAN_POINT('Ctrl Pts',(-57.8248888437787,-42.1408854831791,
0.));
#77867=CARTESIAN_POINT('Ctrl Pts',(-57.8248888437787,-42.1408854831791,
12.));
#77868=CARTESIAN_POINT('Ctrl Pts',(-57.8381486055376,-42.1598927470671,
0.));
#77869=CARTESIAN_POINT('Ctrl Pts',(-57.8381486055376,-42.1598927470671,
12.));
#77870=CARTESIAN_POINT('Ctrl Pts',(-57.8514147590012,-42.1789494950824,
0.));
#77871=CARTESIAN_POINT('Ctrl Pts',(-57.8514147590012,-42.1789494950824,
12.));
#77872=CARTESIAN_POINT('Ctrl Pts',(-57.86468717639,-42.1980556581688,0.));
#77873=CARTESIAN_POINT('Ctrl Pts',(-57.86468717639,-42.1980556581688,12.));
#77874=CARTESIAN_POINT('Ctrl Pts',(-57.8779657305423,-42.2172111674945,
0.));
#77875=CARTESIAN_POINT('Ctrl Pts',(-57.8779657305423,-42.2172111674945,
12.));
#77876=CARTESIAN_POINT('Ctrl Pts',(-57.8912502949084,-42.2364159544492,
0.));
#77877=CARTESIAN_POINT('Ctrl Pts',(-57.8912502949084,-42.2364159544492,
12.));
#77878=CARTESIAN_POINT('Ctrl Pts',(-57.9045407435447,-42.2556699506332,
0.));
#77879=CARTESIAN_POINT('Ctrl Pts',(-57.9045407435447,-42.2556699506332,
12.));
#77880=CARTESIAN_POINT('Ctrl Pts',(-57.9178369511084,-42.274973087857,0.));
#77881=CARTESIAN_POINT('Ctrl Pts',(-57.9178369511084,-42.274973087857,12.));
#77882=CARTESIAN_POINT('Ctrl Pts',(-57.9311387928541,-42.2943252981471,
0.));
#77883=CARTESIAN_POINT('Ctrl Pts',(-57.9311387928541,-42.2943252981471,
12.));
#77884=CARTESIAN_POINT('Ctrl Pts',(-57.9444461446292,-42.3137265137446,
0.));
#77885=CARTESIAN_POINT('Ctrl Pts',(-57.9444461446292,-42.3137265137446,
12.));
#77886=CARTESIAN_POINT('Ctrl Pts',(-57.9577588828693,-42.3331766671028,
0.));
#77887=CARTESIAN_POINT('Ctrl Pts',(-57.9577588828693,-42.3331766671028,
12.));
#77888=CARTESIAN_POINT('Ctrl Pts',(-57.9710768845923,-42.3526756908764,
0.));
#77889=CARTESIAN_POINT('Ctrl Pts',(-57.9710768845923,-42.3526756908764,
12.));
#77890=CARTESIAN_POINT('Ctrl Pts',(-57.9844000273936,-42.3722235179216,
0.));
#77891=CARTESIAN_POINT('Ctrl Pts',(-57.9844000273936,-42.3722235179216,
12.));
#77892=CARTESIAN_POINT('Ctrl Pts',(-57.9977281894437,-42.3918200813024,
0.));
#77893=CARTESIAN_POINT('Ctrl Pts',(-57.9977281894437,-42.3918200813024,
12.));
#77894=CARTESIAN_POINT('Ctrl Pts',(-58.011061249483,-42.4114653142891,0.));
#77895=CARTESIAN_POINT('Ctrl Pts',(-58.011061249483,-42.4114653142891,12.));
#77896=CARTESIAN_POINT('Ctrl Pts',(-58.0243990868175,-42.4311591503551,
0.));
#77897=CARTESIAN_POINT('Ctrl Pts',(-58.0243990868175,-42.4311591503551,
12.));
#77898=CARTESIAN_POINT('Ctrl Pts',(-58.0377415813132,-42.4509015231667,
0.));
#77899=CARTESIAN_POINT('Ctrl Pts',(-58.0377415813132,-42.4509015231667,
12.));
#77900=CARTESIAN_POINT('Ctrl Pts',(-58.0510886133917,-42.4706923665838,
0.));
#77901=CARTESIAN_POINT('Ctrl Pts',(-58.0510886133917,-42.4706923665838,
12.));
#77902=CARTESIAN_POINT('Ctrl Pts',(-58.064440064027,-42.4905316146649,0.));
#77903=CARTESIAN_POINT('Ctrl Pts',(-58.064440064027,-42.4905316146649,12.));
#77904=CARTESIAN_POINT('Ctrl Pts',(-58.0777958147404,-42.5104192016664,
0.));
#77905=CARTESIAN_POINT('Ctrl Pts',(-58.0777958147404,-42.5104192016664,
12.));
#77906=CARTESIAN_POINT('Ctrl Pts',(-58.0911557475967,-42.5303550620388,
0.));
#77907=CARTESIAN_POINT('Ctrl Pts',(-58.0911557475967,-42.5303550620388,
12.));
#77908=CARTESIAN_POINT('Ctrl Pts',(-58.1045197452003,-42.5503391304182,
0.));
#77909=CARTESIAN_POINT('Ctrl Pts',(-58.1045197452003,-42.5503391304182,
12.));
#77910=CARTESIAN_POINT('Ctrl Pts',(-58.1178876906905,-42.5703713416263,
0.));
#77911=CARTESIAN_POINT('Ctrl Pts',(-58.1178876906905,-42.5703713416263,
12.));
#77912=CARTESIAN_POINT('Ctrl Pts',(-58.1312594677383,-42.5904516306759,
0.));
#77913=CARTESIAN_POINT('Ctrl Pts',(-58.1312594677383,-42.5904516306759,
12.));
#77914=CARTESIAN_POINT('Ctrl Pts',(-58.1446349605419,-42.6105799327697,
0.));
#77915=CARTESIAN_POINT('Ctrl Pts',(-58.1446349605419,-42.6105799327697,
12.));
#77916=CARTESIAN_POINT('Ctrl Pts',(-58.158014053823,-42.6307561832977,0.));
#77917=CARTESIAN_POINT('Ctrl Pts',(-58.158014053823,-42.6307561832977,12.));
#77918=CARTESIAN_POINT('Ctrl Pts',(-58.1713966328217,-42.6509803178269,
0.));
#77919=CARTESIAN_POINT('Ctrl Pts',(-58.1713966328217,-42.6509803178269,
12.));
#77920=CARTESIAN_POINT('Ctrl Pts',(-58.1847825832932,-42.6712522721021,
0.));
#77921=CARTESIAN_POINT('Ctrl Pts',(-58.1847825832932,-42.6712522721021,
12.));
#77922=CARTESIAN_POINT('Ctrl Pts',(-58.1981717915043,-42.6915719820516,
0.));
#77923=CARTESIAN_POINT('Ctrl Pts',(-58.1981717915043,-42.6915719820516,
12.));
#77924=CARTESIAN_POINT('Ctrl Pts',(-58.2115641442302,-42.7119393837866,
0.));
#77925=CARTESIAN_POINT('Ctrl Pts',(-58.2115641442302,-42.7119393837866,
12.));
#77926=CARTESIAN_POINT('Ctrl Pts',(-58.2249595287497,-42.7323544135983,
0.));
#77927=CARTESIAN_POINT('Ctrl Pts',(-58.2249595287497,-42.7323544135983,
12.));
#77928=CARTESIAN_POINT('Ctrl Pts',(-58.238357832842,-42.7528170079482,0.));
#77929=CARTESIAN_POINT('Ctrl Pts',(-58.238357832842,-42.7528170079482,12.));
#77930=CARTESIAN_POINT('Ctrl Pts',(-58.2517589447818,-42.7733271034678,
0.));
#77931=CARTESIAN_POINT('Ctrl Pts',(-58.2517589447818,-42.7733271034678,
12.));
#77932=CARTESIAN_POINT('Ctrl Pts',(-58.2651627533368,-42.7938846369651,
0.));
#77933=CARTESIAN_POINT('Ctrl Pts',(-58.2651627533368,-42.7938846369651,
12.));
#77934=CARTESIAN_POINT('Ctrl Pts',(-58.278569147764,-42.8144895454234,0.));
#77935=CARTESIAN_POINT('Ctrl Pts',(-58.278569147764,-42.8144895454234,12.));
#77936=CARTESIAN_POINT('Ctrl Pts',(-58.2919780178063,-42.8351417659998,
0.));
#77937=CARTESIAN_POINT('Ctrl Pts',(-58.2919780178063,-42.8351417659998,
12.));
#77938=CARTESIAN_POINT('Ctrl Pts',(-58.305389253689,-42.8558412360154,0.));
#77939=CARTESIAN_POINT('Ctrl Pts',(-58.305389253689,-42.8558412360154,12.));
#77940=CARTESIAN_POINT('Ctrl Pts',(-58.3188027461158,-42.8765878929545,
0.));
#77941=CARTESIAN_POINT('Ctrl Pts',(-58.3188027461158,-42.8765878929545,
12.));
#77942=CARTESIAN_POINT('Ctrl Pts',(-58.3322183862647,-42.8973816744703,
0.));
#77943=CARTESIAN_POINT('Ctrl Pts',(-58.3322183862647,-42.8973816744703,
12.));
#77944=CARTESIAN_POINT('Ctrl Pts',(-58.3456360657861,-42.9182225183851,
0.));
#77945=CARTESIAN_POINT('Ctrl Pts',(-58.3456360657861,-42.9182225183851,
12.));
#77946=CARTESIAN_POINT('Ctrl Pts',(-58.3590556767981,-42.9391103626881,
0.));
#77947=CARTESIAN_POINT('Ctrl Pts',(-58.3590556767981,-42.9391103626881,
12.));
#77948=CARTESIAN_POINT('Ctrl Pts',(-58.3724771118835,-42.9600451455267,
0.));
#77949=CARTESIAN_POINT('Ctrl Pts',(-58.3724771118835,-42.9600451455267,
12.));
#77950=CARTESIAN_POINT('Ctrl Pts',(-58.3859002640871,-42.9810268052043,
0.));
#77951=CARTESIAN_POINT('Ctrl Pts',(-58.3859002640871,-42.9810268052043,
12.));
#77952=CARTESIAN_POINT('Ctrl Pts',(-58.3993250269115,-43.0020552801869,
0.));
#77953=CARTESIAN_POINT('Ctrl Pts',(-58.3993250269115,-43.0020552801869,
12.));
#77954=CARTESIAN_POINT('Ctrl Pts',(-58.4127512943144,-43.0231305091032,
0.));
#77955=CARTESIAN_POINT('Ctrl Pts',(-58.4127512943144,-43.0231305091032,
12.));
#77956=CARTESIAN_POINT('Ctrl Pts',(-58.4261789607055,-43.0442524307432,
0.));
#77957=CARTESIAN_POINT('Ctrl Pts',(-58.4261789607055,-43.0442524307432,
12.));
#77958=CARTESIAN_POINT('Ctrl Pts',(-58.4396079209438,-43.0654209840502,
0.));
#77959=CARTESIAN_POINT('Ctrl Pts',(-58.4396079209438,-43.0654209840502,
12.));
#77960=CARTESIAN_POINT('Ctrl Pts',(-58.4530380703335,-43.0866361081166,
0.));
#77961=CARTESIAN_POINT('Ctrl Pts',(-58.4530380703335,-43.0866361081166,
12.));
#77962=CARTESIAN_POINT('Ctrl Pts',(-58.4664693046206,-43.1078977421908,
0.));
#77963=CARTESIAN_POINT('Ctrl Pts',(-58.4664693046206,-43.1078977421908,
12.));
#77964=CARTESIAN_POINT('Ctrl Pts',(-58.4799015199904,-43.1292058256774,
0.));
#77965=CARTESIAN_POINT('Ctrl Pts',(-58.4799015199904,-43.1292058256774,
12.));
#77966=CARTESIAN_POINT('Ctrl Pts',(-58.4933346130638,-43.1505602981366,
0.));
#77967=CARTESIAN_POINT('Ctrl Pts',(-58.4933346130638,-43.1505602981366,
12.));
#77968=CARTESIAN_POINT('Ctrl Pts',(-58.5067684808946,-43.1719610992771,
0.));
#77969=CARTESIAN_POINT('Ctrl Pts',(-58.5067684808946,-43.1719610992771,
12.));
#77970=CARTESIAN_POINT('Ctrl Pts',(-58.5202030209667,-43.1934081689503,
0.));
#77971=CARTESIAN_POINT('Ctrl Pts',(-58.5202030209667,-43.1934081689503,
12.));
#77972=CARTESIAN_POINT('Ctrl Pts',(-58.5336381311911,-43.214901447157,0.));
#77973=CARTESIAN_POINT('Ctrl Pts',(-58.5336381311911,-43.214901447157,12.));
#77974=CARTESIAN_POINT('Ctrl Pts',(-58.5470737099027,-43.2364408740488,
0.));
#77975=CARTESIAN_POINT('Ctrl Pts',(-58.5470737099027,-43.2364408740488,
12.));
#77976=CARTESIAN_POINT('Ctrl Pts',(-58.5605096558578,-43.2580263899278,
0.));
#77977=CARTESIAN_POINT('Ctrl Pts',(-58.5605096558578,-43.2580263899278,
12.));
#77978=CARTESIAN_POINT('Ctrl Pts',(-58.5739458682317,-43.2796579352405,
0.));
#77979=CARTESIAN_POINT('Ctrl Pts',(-58.5739458682317,-43.2796579352405,
12.));
#77980=CARTESIAN_POINT('Ctrl Pts',(-58.5873822466163,-43.3013354505707,
0.));
#77981=CARTESIAN_POINT('Ctrl Pts',(-58.5873822466163,-43.3013354505707,
12.));
#77982=CARTESIAN_POINT('Ctrl Pts',(-58.6008186910166,-43.3230588766455,
0.));
#77983=CARTESIAN_POINT('Ctrl Pts',(-58.6008186910166,-43.3230588766455,
12.));
#77984=CARTESIAN_POINT('Ctrl Pts',(-58.6142551018473,-43.3448281543374,
0.));
#77985=CARTESIAN_POINT('Ctrl Pts',(-58.6142551018473,-43.3448281543374,
12.));
#77986=CARTESIAN_POINT('Ctrl Pts',(-58.627691379929,-43.3666432246634,0.));
#77987=CARTESIAN_POINT('Ctrl Pts',(-58.627691379929,-43.3666432246634,12.));
#77988=CARTESIAN_POINT('Ctrl Pts',(-58.6411274264854,-43.3885040287808,
0.));
#77989=CARTESIAN_POINT('Ctrl Pts',(-58.6411274264854,-43.3885040287808,
12.));
#77990=CARTESIAN_POINT('Ctrl Pts',(-58.6545631431388,-43.4104105079766,
0.));
#77991=CARTESIAN_POINT('Ctrl Pts',(-58.6545631431388,-43.4104105079766,
12.));
#77992=CARTESIAN_POINT('Ctrl Pts',(-58.6679984319095,-43.4323626036736,
0.));
#77993=CARTESIAN_POINT('Ctrl Pts',(-58.6679984319095,-43.4323626036736,
12.));
#77994=CARTESIAN_POINT('Ctrl Pts',(-58.6814331952138,-43.4543602574352,
0.));
#77995=CARTESIAN_POINT('Ctrl Pts',(-58.6814331952138,-43.4543602574352,
12.));
#77996=CARTESIAN_POINT('Ctrl Pts',(-58.6948673358639,-43.4764034109654,
0.));
#77997=CARTESIAN_POINT('Ctrl Pts',(-58.6948673358639,-43.4764034109654,
12.));
#77998=CARTESIAN_POINT('Ctrl Pts',(-58.708300757066,-43.4984920061071,0.));
#77999=CARTESIAN_POINT('Ctrl Pts',(-58.708300757066,-43.4984920061071,12.));
#78000=CARTESIAN_POINT('Ctrl Pts',(-58.7217333624206,-43.5206259848333,
0.));
#78001=CARTESIAN_POINT('Ctrl Pts',(-58.7217333624206,-43.5206259848333,
12.));
#78002=CARTESIAN_POINT('Ctrl Pts',(-58.7351650559176,-43.5428052892483,
0.));
#78003=CARTESIAN_POINT('Ctrl Pts',(-58.7351650559176,-43.5428052892483,
12.));
#78004=CARTESIAN_POINT('Ctrl Pts',(-58.7485957419296,-43.5650298615911,
0.));
#78005=CARTESIAN_POINT('Ctrl Pts',(-58.7485957419296,-43.5650298615911,
12.));
#78006=CARTESIAN_POINT('Ctrl Pts',(-58.7620253252059,-43.5872996442343,
0.));
#78007=CARTESIAN_POINT('Ctrl Pts',(-58.7620253252059,-43.5872996442343,
12.));
#78008=CARTESIAN_POINT('Ctrl Pts',(-58.7754537108672,-43.6096145796798,
0.));
#78009=CARTESIAN_POINT('Ctrl Pts',(-58.7754537108672,-43.6096145796798,
12.));
#78010=CARTESIAN_POINT('Ctrl Pts',(-58.7888808043976,-43.6319746105487,
0.));
#78011=CARTESIAN_POINT('Ctrl Pts',(-58.7888808043976,-43.6319746105487,
12.));
#78012=CARTESIAN_POINT('Ctrl Pts',(-58.8023065116446,-43.6543796795797,
0.));
#78013=CARTESIAN_POINT('Ctrl Pts',(-58.8023065116446,-43.6543796795797,
12.));
#78014=CARTESIAN_POINT('Ctrl Pts',(-58.8157307388247,-43.6768297296402,
0.));
#78015=CARTESIAN_POINT('Ctrl Pts',(-58.8157307388247,-43.6768297296402,
12.));
#78016=CARTESIAN_POINT('Ctrl Pts',(-58.8291533925299,-43.6993247037318,
0.));
#78017=CARTESIAN_POINT('Ctrl Pts',(-58.8291533925299,-43.6993247037318,
12.));
#78018=CARTESIAN_POINT('Ctrl Pts',(-58.8425743797325,-43.7218645449921,
0.));
#78019=CARTESIAN_POINT('Ctrl Pts',(-58.8425743797325,-43.7218645449921,
12.));
#78020=CARTESIAN_POINT('Ctrl Pts',(-58.8559936077933,-43.7444491966935,
0.));
#78021=CARTESIAN_POINT('Ctrl Pts',(-58.8559936077933,-43.7444491966935,
12.));
#78022=CARTESIAN_POINT('Ctrl Pts',(-58.8694109844636,-43.7670786022392,
0.));
#78023=CARTESIAN_POINT('Ctrl Pts',(-58.8694109844636,-43.7670786022392,
12.));
#78024=CARTESIAN_POINT('Ctrl Pts',(-58.882826417861,-43.7897527051599,0.));
#78025=CARTESIAN_POINT('Ctrl Pts',(-58.882826417861,-43.7897527051599,12.));
#78026=CARTESIAN_POINT('Ctrl Pts',(-58.8962398164486,-43.8124714491069,
0.));
#78027=CARTESIAN_POINT('Ctrl Pts',(-58.8962398164486,-43.8124714491069,
12.));
#78028=CARTESIAN_POINT('Ctrl Pts',(-58.9096510890128,-43.8352347778419,
0.));
#78029=CARTESIAN_POINT('Ctrl Pts',(-58.9096510890128,-43.8352347778419,
12.));
#78030=CARTESIAN_POINT('Ctrl Pts',(-58.9230601446445,-43.8580426352236,
0.));
#78031=CARTESIAN_POINT('Ctrl Pts',(-58.9230601446445,-43.8580426352236,
12.));
#78032=CARTESIAN_POINT('Ctrl Pts',(-58.9364668927132,-43.8808949651882,
0.));
#78033=CARTESIAN_POINT('Ctrl Pts',(-58.9364668927132,-43.8808949651882,
12.));
#78034=CARTESIAN_POINT('Ctrl Pts',(-58.9498712429066,-43.9037917117748,
0.));
#78035=CARTESIAN_POINT('Ctrl Pts',(-58.9498712429066,-43.9037917117748,
12.));
#78036=CARTESIAN_POINT('Ctrl Pts',(-58.9632731052704,-43.9267328191507,
0.));
#78037=CARTESIAN_POINT('Ctrl Pts',(-58.9632731052704,-43.9267328191507,
12.));
#78038=CARTESIAN_POINT('Ctrl Pts',(-58.9766723902531,-43.9497182316333,
0.));
#78039=CARTESIAN_POINT('Ctrl Pts',(-58.9766723902531,-43.9497182316333,
12.));
#78040=CARTESIAN_POINT('Ctrl Pts',(-58.9900690087404,-43.9727478937053,
0.));
#78041=CARTESIAN_POINT('Ctrl Pts',(-58.9900690087404,-43.9727478937053,
12.));
#78042=CARTESIAN_POINT('Ctrl Pts',(-59.0034628721161,-43.9958217500363,
0.));
#78043=CARTESIAN_POINT('Ctrl Pts',(-59.0034628721161,-43.9958217500363,
12.));
#78044=CARTESIAN_POINT('Ctrl Pts',(-59.0168538922087,-44.0189397454593,
0.));
#78045=CARTESIAN_POINT('Ctrl Pts',(-59.0168538922087,-44.0189397454593,
12.));
#78046=CARTESIAN_POINT('Ctrl Pts',(-59.0302419811772,-44.0421018249219,
0.));
#78047=CARTESIAN_POINT('Ctrl Pts',(-59.0302419811772,-44.0421018249219,
12.));
#78048=CARTESIAN_POINT('Ctrl Pts',(-59.0436270514085,-44.0653079334384,
0.));
#78049=CARTESIAN_POINT('Ctrl Pts',(-59.0436270514085,-44.0653079334384,
12.));
#78050=CARTESIAN_POINT('Ctrl Pts',(-59.0570090154243,-44.0885580160433,
0.));
#78051=CARTESIAN_POINT('Ctrl Pts',(-59.0570090154243,-44.0885580160433,
12.));
#78052=CARTESIAN_POINT('Ctrl Pts',(-59.0703877857529,-44.1118520177223,
0.));
#78053=CARTESIAN_POINT('Ctrl Pts',(-59.0703877857529,-44.1118520177223,
12.));
#78054=CARTESIAN_POINT('Ctrl Pts',(-59.0837632749209,-44.1351898834057,
0.));
#78055=CARTESIAN_POINT('Ctrl Pts',(-59.0837632749209,-44.1351898834057,
12.));
#78056=CARTESIAN_POINT('Ctrl Pts',(-59.0971353957218,-44.1585715581073,
0.));
#78057=CARTESIAN_POINT('Ctrl Pts',(-59.0971353957218,-44.1585715581073,
12.));
#78058=CARTESIAN_POINT('Ctrl Pts',(-59.1105040614285,-44.1819969870314,
0.));
#78059=CARTESIAN_POINT('Ctrl Pts',(-59.1105040614285,-44.1819969870314,
12.));
#78060=CARTESIAN_POINT('Ctrl Pts',(-59.1238691860307,-44.2054661156876,
0.));
#78061=CARTESIAN_POINT('Ctrl Pts',(-59.1238691860307,-44.2054661156876,
12.));
#78062=CARTESIAN_POINT('Ctrl Pts',(-59.1372306844575,-44.2289788899962,
0.));
#78063=CARTESIAN_POINT('Ctrl Pts',(-59.1372306844575,-44.2289788899962,
12.));
#78064=CARTESIAN_POINT('Ctrl Pts',(-59.1505884728194,-44.2525352563979,
0.));
#78065=CARTESIAN_POINT('Ctrl Pts',(-59.1505884728194,-44.2525352563979,
12.));
#78066=CARTESIAN_POINT('Ctrl Pts',(-59.1639424678766,-44.2761351616027,
0.));
#78067=CARTESIAN_POINT('Ctrl Pts',(-59.1639424678766,-44.2761351616027,
12.));
#78068=CARTESIAN_POINT('Ctrl Pts',(-59.1772925865191,-44.2997785523413,
0.));
#78069=CARTESIAN_POINT('Ctrl Pts',(-59.1772925865191,-44.2997785523413,
12.));
#78070=CARTESIAN_POINT('Ctrl Pts',(-59.1906387451971,-44.3234653750877,
0.));
#78071=CARTESIAN_POINT('Ctrl Pts',(-59.1906387451971,-44.3234653750877,
12.));
#78072=CARTESIAN_POINT('Ctrl Pts',(-59.2039808594765,-44.3471955758412,
0.));
#78073=CARTESIAN_POINT('Ctrl Pts',(-59.2039808594765,-44.3471955758412,
12.));
#78074=CARTESIAN_POINT('Ctrl Pts',(-59.217318843283,-44.3709690997495,0.));
#78075=CARTESIAN_POINT('Ctrl Pts',(-59.217318843283,-44.3709690997495,12.));
#78076=CARTESIAN_POINT('Ctrl Pts',(-59.2306526095175,-44.394785891411,0.));
#78077=CARTESIAN_POINT('Ctrl Pts',(-59.2306526095175,-44.394785891411,12.));
#78078=CARTESIAN_POINT('Ctrl Pts',(-59.2439820714231,-44.4186458955486,
0.));
#78079=CARTESIAN_POINT('Ctrl Pts',(-59.2439820714231,-44.4186458955486,
12.));
#78080=CARTESIAN_POINT('Ctrl Pts',(-59.2573071437801,-44.4425490575932,
0.));
#78081=CARTESIAN_POINT('Ctrl Pts',(-59.2573071437801,-44.4425490575932,
12.));
#78082=CARTESIAN_POINT('Ctrl Pts',(-59.2706277440438,-44.4664953242373,
0.));
#78083=CARTESIAN_POINT('Ctrl Pts',(-59.2706277440438,-44.4664953242373,
12.));
#78084=CARTESIAN_POINT('Ctrl Pts',(-59.2839437938187,-44.490484644147,0.));
#78085=CARTESIAN_POINT('Ctrl Pts',(-59.2839437938187,-44.490484644147,12.));
#78086=CARTESIAN_POINT('Ctrl Pts',(-59.2972552192072,-44.514516968128,0.));
#78087=CARTESIAN_POINT('Ctrl Pts',(-59.2972552192072,-44.514516968128,12.));
#78088=CARTESIAN_POINT('Ctrl Pts',(-59.3105619475512,-44.5385922475494,
0.));
#78089=CARTESIAN_POINT('Ctrl Pts',(-59.3105619475512,-44.5385922475494,
12.));
#78090=CARTESIAN_POINT('Ctrl Pts',(-59.3238639048618,-44.5627104330956,
0.));
#78091=CARTESIAN_POINT('Ctrl Pts',(-59.3238639048618,-44.5627104330956,
12.));
#78092=CARTESIAN_POINT('Ctrl Pts',(-59.3371610128494,-44.5868714733219,
0.));
#78093=CARTESIAN_POINT('Ctrl Pts',(-59.3371610128494,-44.5868714733219,
12.));
#78094=CARTESIAN_POINT('Ctrl Pts',(-59.3504531864223,-44.6110753134333,
0.));
#78095=CARTESIAN_POINT('Ctrl Pts',(-59.3504531864223,-44.6110753134333,
12.));
#78096=CARTESIAN_POINT('Ctrl Pts',(-59.3637403301959,-44.6353218935813,
0.));
#78097=CARTESIAN_POINT('Ctrl Pts',(-59.3637403301959,-44.6353218935813,
12.));
#78098=CARTESIAN_POINT('Ctrl Pts',(-59.3770223435405,-44.659611151286,0.));
#78099=CARTESIAN_POINT('Ctrl Pts',(-59.3770223435405,-44.659611151286,12.));
#78100=CARTESIAN_POINT('Ctrl Pts',(-59.3902991268094,-44.6839430244375,
0.));
#78101=CARTESIAN_POINT('Ctrl Pts',(-59.3902991268094,-44.6839430244375,
12.));
#78102=CARTESIAN_POINT('Ctrl Pts',(-59.403570587392,-44.708317454179,0.));
#78103=CARTESIAN_POINT('Ctrl Pts',(-59.403570587392,-44.708317454179,12.));
#78104=CARTESIAN_POINT('Ctrl Pts',(-59.4168366453047,-44.7327343876333,
0.));
#78105=CARTESIAN_POINT('Ctrl Pts',(-59.4168366453047,-44.7327343876333,
12.));
#78106=CARTESIAN_POINT('Ctrl Pts',(-59.4300972402943,-44.7571937811872,
0.));
#78107=CARTESIAN_POINT('Ctrl Pts',(-59.4300972402943,-44.7571937811872,
12.));
#78108=CARTESIAN_POINT('Ctrl Pts',(-59.4433523334651,-44.7816956017126,
0.));
#78109=CARTESIAN_POINT('Ctrl Pts',(-59.4433523334651,-44.7816956017126,
12.));
#78110=CARTESIAN_POINT('Ctrl Pts',(-59.4566019017674,-44.8062398250937,
0.));
#78111=CARTESIAN_POINT('Ctrl Pts',(-59.4566019017674,-44.8062398250937,
12.));
#78112=CARTESIAN_POINT('Ctrl Pts',(-59.4671971277837,-44.8259091133624,
0.));
#78113=CARTESIAN_POINT('Ctrl Pts',(-59.4671971277837,-44.8259091133624,
12.));
#78114=CARTESIAN_POINT('Ctrl Pts',(-59.475141054744,-44.8406801497506,0.));
#78115=CARTESIAN_POINT('Ctrl Pts',(-59.475141054744,-44.8406801497506,12.));
#78116=CARTESIAN_POINT('Ctrl Pts',(-59.4804358982977,-44.8505359826374,
0.));
#78117=CARTESIAN_POINT('Ctrl Pts',(-59.4804358982977,-44.8505359826374,
12.));
#78118=CARTESIAN_POINT('Ctrl Pts',(-59.483083043136,-44.8554660179045,0.));
#78119=CARTESIAN_POINT('Ctrl Pts',(-59.483083043136,-44.8554660179045,12.));
#78120=CARTESIAN_POINT('',(-56.8466430164621,-40.8467768343956,0.));
#78121=CARTESIAN_POINT('Ctrl Pts',(-56.8466430164621,-40.8467768343956,
0.));
#78122=CARTESIAN_POINT('Ctrl Pts',(-56.8491101022591,-40.8497761671036,
0.));
#78123=CARTESIAN_POINT('Ctrl Pts',(-56.8540460739472,-40.8557803680277,
0.));
#78124=CARTESIAN_POINT('Ctrl Pts',(-56.8614554317668,-40.864803275942,0.));
#78125=CARTESIAN_POINT('Ctrl Pts',(-56.8713453764905,-40.8768670342052,
0.));
#78126=CARTESIAN_POINT('Ctrl Pts',(-56.8837257978343,-40.8920020903293,
0.));
#78127=CARTESIAN_POINT('Ctrl Pts',(-56.8961241708861,-40.9071924937508,
0.));
#78128=CARTESIAN_POINT('Ctrl Pts',(-56.9085404164502,-40.9224382132427,
0.));
#78129=CARTESIAN_POINT('Ctrl Pts',(-56.9209743960992,-40.9377391857128,
0.));
#78130=CARTESIAN_POINT('Ctrl Pts',(-56.9334259140049,-40.9530953165031,
0.));
#78131=CARTESIAN_POINT('Ctrl Pts',(-56.9458947422608,-40.9685064933074,
0.));
#78132=CARTESIAN_POINT('Ctrl Pts',(-56.9583806404069,-40.9839725967121,
0.));
#78133=CARTESIAN_POINT('Ctrl Pts',(-56.9708833766137,-40.9994935117276,
0.));
#78134=CARTESIAN_POINT('Ctrl Pts',(-56.9834027500117,-41.0150691398947,
0.));
#78135=CARTESIAN_POINT('Ctrl Pts',(-56.995938583472,-41.0306993953988,0.));
#78136=CARTESIAN_POINT('Ctrl Pts',(-57.008490713042,-41.0463841993608,0.));
#78137=CARTESIAN_POINT('Ctrl Pts',(-57.0210589791788,-41.0621234751007,
0.));
#78138=CARTESIAN_POINT('Ctrl Pts',(-57.0336432158536,-41.0779171422438,
0.));
#78139=CARTESIAN_POINT('Ctrl Pts',(-57.046243245068,-41.0937651137549,0.));
#78140=CARTESIAN_POINT('Ctrl Pts',(-57.0588588825298,-41.1096672990148,
0.));
#78141=CARTESIAN_POINT('Ctrl Pts',(-57.0714899412099,-41.1256236057442,
0.));
#78142=CARTESIAN_POINT('Ctrl Pts',(-57.084136235426,-41.1416339422117,0.));
#78143=CARTESIAN_POINT('Ctrl Pts',(-57.0967975854874,-41.1576982197374,
0.));
#78144=CARTESIAN_POINT('Ctrl Pts',(-57.1094738174957,-41.1738163525901,
0.));
#78145=CARTESIAN_POINT('Ctrl Pts',(-57.1221647611207,-41.1899882567923,
0.));
#78146=CARTESIAN_POINT('Ctrl Pts',(-57.1348702480647,-41.2062138492915,
0.));
#78147=CARTESIAN_POINT('Ctrl Pts',(-57.147590110182,-41.222493046943,0.));
#78148=CARTESIAN_POINT('Ctrl Pts',(-57.1603241779077,-41.2388257656559,
0.));
#78149=CARTESIAN_POINT('Ctrl Pts',(-57.17307228108,-41.2552119208465,0.));
#78150=CARTESIAN_POINT('Ctrl Pts',(-57.1858342496538,-41.2716514278276,
0.));
#78151=CARTESIAN_POINT('Ctrl Pts',(-57.1986099143983,-41.2881442021863,
0.));
#78152=CARTESIAN_POINT('Ctrl Pts',(-57.2113991077302,-41.3046901602293,
0.));
#78153=CARTESIAN_POINT('Ctrl Pts',(-57.2242016640198,-41.321289219149,0.));
#78154=CARTESIAN_POINT('Ctrl Pts',(-57.2370174191401,-41.3379412967875,
0.));
#78155=CARTESIAN_POINT('Ctrl Pts',(-57.2498462101879,-41.3546463114885,
0.));
#78156=CARTESIAN_POINT('Ctrl Pts',(-57.2626878751596,-41.3714041819223,
0.));
#78157=CARTESIAN_POINT('Ctrl Pts',(-57.2755422525844,-41.3882148268813,
0.));
#78158=CARTESIAN_POINT('Ctrl Pts',(-57.2884091815406,-41.4050781652938,
0.));
#78159=CARTESIAN_POINT('Ctrl Pts',(-57.3012885018151,-41.4219941163163,
0.));
#78160=CARTESIAN_POINT('Ctrl Pts',(-57.3141800540137,-41.4389625993948,
0.));
#78161=CARTESIAN_POINT('Ctrl Pts',(-57.3270836796911,-41.4559835343328,
0.));
#78162=CARTESIAN_POINT('Ctrl Pts',(-57.3399992214717,-41.4730568413518,
0.));
#78163=CARTESIAN_POINT('Ctrl Pts',(-57.3529265229835,-41.4901824410636,
0.));
#78164=CARTESIAN_POINT('Ctrl Pts',(-57.3658654287937,-41.5073602544396,
0.));
#78165=CARTESIAN_POINT('Ctrl Pts',(-57.3788157843454,-41.524590202777,0.));
#78166=CARTESIAN_POINT('Ctrl Pts',(-57.3917774358863,-41.5418722076572,
0.));
#78167=CARTESIAN_POINT('Ctrl Pts',(-57.4047502304231,-41.5592061909176,
0.));
#78168=CARTESIAN_POINT('Ctrl Pts',(-57.4177340157508,-41.5765920746777,
0.));
#78169=CARTESIAN_POINT('Ctrl Pts',(-57.4307286404662,-41.5940297813477,
0.));
#78170=CARTESIAN_POINT('Ctrl Pts',(-57.4437339539841,-41.6115192336388,
0.));
#78171=CARTESIAN_POINT('Ctrl Pts',(-57.4567498065562,-41.6290603545666,
0.));
#78172=CARTESIAN_POINT('Ctrl Pts',(-57.4697760492683,-41.6466530674514,
0.));
#78173=CARTESIAN_POINT('Ctrl Pts',(-57.4828125340218,-41.6642972959165,
0.));
#78174=CARTESIAN_POINT('Ctrl Pts',(-57.4958591135165,-41.6819929638797,
0.));
#78175=CARTESIAN_POINT('Ctrl Pts',(-57.5089156412343,-41.6997399955447,
0.));
#78176=CARTESIAN_POINT('Ctrl Pts',(-57.5219819714171,-41.7175383153821,
0.));
#78177=CARTESIAN_POINT('Ctrl Pts',(-57.5350579590649,-41.7353878481336,
0.));
#78178=CARTESIAN_POINT('Ctrl Pts',(-57.5481434599335,-41.7532885188174,
0.));
#78179=CARTESIAN_POINT('Ctrl Pts',(-57.561238330532,-41.7712402527273,0.));
#78180=CARTESIAN_POINT('Ctrl Pts',(-57.5743424281205,-41.7892429754297,
0.));
#78181=CARTESIAN_POINT('Ctrl Pts',(-57.5874556107056,-41.8072966127558,
0.));
#78182=CARTESIAN_POINT('Ctrl Pts',(-57.6005777370349,-41.8254010908051,
0.));
#78183=CARTESIAN_POINT('Ctrl Pts',(-57.6137086665882,-41.8435563359456,
0.));
#78184=CARTESIAN_POINT('Ctrl Pts',(-57.6268482595702,-41.8617622748108,
0.));
#78185=CARTESIAN_POINT('Ctrl Pts',(-57.6399963769003,-41.8800188342908,
0.));
#78186=CARTESIAN_POINT('Ctrl Pts',(-57.6531528802059,-41.8983259415244,
0.));
#78187=CARTESIAN_POINT('Ctrl Pts',(-57.6663176318176,-41.9166835239046,
0.));
#78188=CARTESIAN_POINT('Ctrl Pts',(-57.6794904947641,-41.9350915090791,
0.));
#78189=CARTESIAN_POINT('Ctrl Pts',(-57.6926713327674,-41.9535498249489,
0.));
#78190=CARTESIAN_POINT('Ctrl Pts',(-57.7058600102365,-41.9720583996601,
0.));
#78191=CARTESIAN_POINT('Ctrl Pts',(-57.7190563922614,-41.9906171615974,
0.));
#78192=CARTESIAN_POINT('Ctrl Pts',(-57.7322603446086,-42.0092260393911,
0.));
#78193=CARTESIAN_POINT('Ctrl Pts',(-57.7454717337151,-42.0278849619156,
0.));
#78194=CARTESIAN_POINT('Ctrl Pts',(-57.7586904266828,-42.0465938582877,
0.));
#78195=CARTESIAN_POINT('Ctrl Pts',(-57.7719162912721,-42.0653526578571,
0.));
#78196=CARTESIAN_POINT('Ctrl Pts',(-57.7851491958954,-42.0841612902018,
0.));
#78197=CARTESIAN_POINT('Ctrl Pts',(-57.798389009613,-42.1030196851344,0.));
#78198=CARTESIAN_POINT('Ctrl Pts',(-57.8116356021274,-42.121927772701,0.));
#78199=CARTESIAN_POINT('Ctrl Pts',(-57.8248888437787,-42.1408854831791,
0.));
#78200=CARTESIAN_POINT('Ctrl Pts',(-57.8381486055376,-42.1598927470671,
0.));
#78201=CARTESIAN_POINT('Ctrl Pts',(-57.8514147590012,-42.1789494950824,
0.));
#78202=CARTESIAN_POINT('Ctrl Pts',(-57.86468717639,-42.1980556581688,0.));
#78203=CARTESIAN_POINT('Ctrl Pts',(-57.8779657305423,-42.2172111674945,
0.));
#78204=CARTESIAN_POINT('Ctrl Pts',(-57.8912502949084,-42.2364159544492,
0.));
#78205=CARTESIAN_POINT('Ctrl Pts',(-57.9045407435447,-42.2556699506332,
0.));
#78206=CARTESIAN_POINT('Ctrl Pts',(-57.9178369511084,-42.274973087857,0.));
#78207=CARTESIAN_POINT('Ctrl Pts',(-57.9311387928541,-42.2943252981471,
0.));
#78208=CARTESIAN_POINT('Ctrl Pts',(-57.9444461446292,-42.3137265137446,
0.));
#78209=CARTESIAN_POINT('Ctrl Pts',(-57.9577588828693,-42.3331766671028,
0.));
#78210=CARTESIAN_POINT('Ctrl Pts',(-57.9710768845923,-42.3526756908764,
0.));
#78211=CARTESIAN_POINT('Ctrl Pts',(-57.9844000273936,-42.3722235179216,
0.));
#78212=CARTESIAN_POINT('Ctrl Pts',(-57.9977281894437,-42.3918200813024,
0.));
#78213=CARTESIAN_POINT('Ctrl Pts',(-58.011061249483,-42.4114653142891,0.));
#78214=CARTESIAN_POINT('Ctrl Pts',(-58.0243990868175,-42.4311591503551,
0.));
#78215=CARTESIAN_POINT('Ctrl Pts',(-58.0377415813132,-42.4509015231667,
0.));
#78216=CARTESIAN_POINT('Ctrl Pts',(-58.0510886133917,-42.4706923665838,
0.));
#78217=CARTESIAN_POINT('Ctrl Pts',(-58.064440064027,-42.4905316146649,0.));
#78218=CARTESIAN_POINT('Ctrl Pts',(-58.0777958147404,-42.5104192016664,
0.));
#78219=CARTESIAN_POINT('Ctrl Pts',(-58.0911557475967,-42.5303550620388,
0.));
#78220=CARTESIAN_POINT('Ctrl Pts',(-58.1045197452003,-42.5503391304182,
0.));
#78221=CARTESIAN_POINT('Ctrl Pts',(-58.1178876906905,-42.5703713416263,
0.));
#78222=CARTESIAN_POINT('Ctrl Pts',(-58.1312594677383,-42.5904516306759,
0.));
#78223=CARTESIAN_POINT('Ctrl Pts',(-58.1446349605419,-42.6105799327697,
0.));
#78224=CARTESIAN_POINT('Ctrl Pts',(-58.158014053823,-42.6307561832977,0.));
#78225=CARTESIAN_POINT('Ctrl Pts',(-58.1713966328217,-42.6509803178269,
0.));
#78226=CARTESIAN_POINT('Ctrl Pts',(-58.1847825832932,-42.6712522721021,
0.));
#78227=CARTESIAN_POINT('Ctrl Pts',(-58.1981717915043,-42.6915719820516,
0.));
#78228=CARTESIAN_POINT('Ctrl Pts',(-58.2115641442302,-42.7119393837866,
0.));
#78229=CARTESIAN_POINT('Ctrl Pts',(-58.2249595287497,-42.7323544135983,
0.));
#78230=CARTESIAN_POINT('Ctrl Pts',(-58.238357832842,-42.7528170079482,0.));
#78231=CARTESIAN_POINT('Ctrl Pts',(-58.2517589447818,-42.7733271034678,
0.));
#78232=CARTESIAN_POINT('Ctrl Pts',(-58.2651627533368,-42.7938846369651,
0.));
#78233=CARTESIAN_POINT('Ctrl Pts',(-58.278569147764,-42.8144895454234,0.));
#78234=CARTESIAN_POINT('Ctrl Pts',(-58.2919780178063,-42.8351417659998,
0.));
#78235=CARTESIAN_POINT('Ctrl Pts',(-58.305389253689,-42.8558412360154,0.));
#78236=CARTESIAN_POINT('Ctrl Pts',(-58.3188027461158,-42.8765878929545,
0.));
#78237=CARTESIAN_POINT('Ctrl Pts',(-58.3322183862647,-42.8973816744703,
0.));
#78238=CARTESIAN_POINT('Ctrl Pts',(-58.3456360657861,-42.9182225183851,
0.));
#78239=CARTESIAN_POINT('Ctrl Pts',(-58.3590556767981,-42.9391103626881,
0.));
#78240=CARTESIAN_POINT('Ctrl Pts',(-58.3724771118835,-42.9600451455267,
0.));
#78241=CARTESIAN_POINT('Ctrl Pts',(-58.3859002640871,-42.9810268052043,
0.));
#78242=CARTESIAN_POINT('Ctrl Pts',(-58.3993250269115,-43.0020552801869,
0.));
#78243=CARTESIAN_POINT('Ctrl Pts',(-58.4127512943144,-43.0231305091032,
0.));
#78244=CARTESIAN_POINT('Ctrl Pts',(-58.4261789607055,-43.0442524307432,
0.));
#78245=CARTESIAN_POINT('Ctrl Pts',(-58.4396079209438,-43.0654209840502,
0.));
#78246=CARTESIAN_POINT('Ctrl Pts',(-58.4530380703335,-43.0866361081166,
0.));
#78247=CARTESIAN_POINT('Ctrl Pts',(-58.4664693046206,-43.1078977421908,
0.));
#78248=CARTESIAN_POINT('Ctrl Pts',(-58.4799015199904,-43.1292058256774,
0.));
#78249=CARTESIAN_POINT('Ctrl Pts',(-58.4933346130638,-43.1505602981366,
0.));
#78250=CARTESIAN_POINT('Ctrl Pts',(-58.5067684808946,-43.1719610992771,
0.));
#78251=CARTESIAN_POINT('Ctrl Pts',(-58.5202030209667,-43.1934081689503,
0.));
#78252=CARTESIAN_POINT('Ctrl Pts',(-58.5336381311911,-43.214901447157,0.));
#78253=CARTESIAN_POINT('Ctrl Pts',(-58.5470737099027,-43.2364408740488,
0.));
#78254=CARTESIAN_POINT('Ctrl Pts',(-58.5605096558578,-43.2580263899278,
0.));
#78255=CARTESIAN_POINT('Ctrl Pts',(-58.5739458682317,-43.2796579352405,
0.));
#78256=CARTESIAN_POINT('Ctrl Pts',(-58.5873822466163,-43.3013354505707,
0.));
#78257=CARTESIAN_POINT('Ctrl Pts',(-58.6008186910166,-43.3230588766455,
0.));
#78258=CARTESIAN_POINT('Ctrl Pts',(-58.6142551018473,-43.3448281543374,
0.));
#78259=CARTESIAN_POINT('Ctrl Pts',(-58.627691379929,-43.3666432246634,0.));
#78260=CARTESIAN_POINT('Ctrl Pts',(-58.6411274264854,-43.3885040287808,
0.));
#78261=CARTESIAN_POINT('Ctrl Pts',(-58.6545631431388,-43.4104105079766,
0.));
#78262=CARTESIAN_POINT('Ctrl Pts',(-58.6679984319095,-43.4323626036736,
0.));
#78263=CARTESIAN_POINT('Ctrl Pts',(-58.6814331952138,-43.4543602574352,
0.));
#78264=CARTESIAN_POINT('Ctrl Pts',(-58.6948673358639,-43.4764034109654,
0.));
#78265=CARTESIAN_POINT('Ctrl Pts',(-58.708300757066,-43.4984920061071,0.));
#78266=CARTESIAN_POINT('Ctrl Pts',(-58.7217333624206,-43.5206259848333,
0.));
#78267=CARTESIAN_POINT('Ctrl Pts',(-58.7351650559176,-43.5428052892483,
0.));
#78268=CARTESIAN_POINT('Ctrl Pts',(-58.7485957419296,-43.5650298615911,
0.));
#78269=CARTESIAN_POINT('Ctrl Pts',(-58.7620253252059,-43.5872996442343,
0.));
#78270=CARTESIAN_POINT('Ctrl Pts',(-58.7754537108672,-43.6096145796798,
0.));
#78271=CARTESIAN_POINT('Ctrl Pts',(-58.7888808043976,-43.6319746105487,
0.));
#78272=CARTESIAN_POINT('Ctrl Pts',(-58.8023065116446,-43.6543796795797,
0.));
#78273=CARTESIAN_POINT('Ctrl Pts',(-58.8157307388247,-43.6768297296402,
0.));
#78274=CARTESIAN_POINT('Ctrl Pts',(-58.8291533925299,-43.6993247037318,
0.));
#78275=CARTESIAN_POINT('Ctrl Pts',(-58.8425743797325,-43.7218645449921,
0.));
#78276=CARTESIAN_POINT('Ctrl Pts',(-58.8559936077933,-43.7444491966935,
0.));
#78277=CARTESIAN_POINT('Ctrl Pts',(-58.8694109844636,-43.7670786022392,
0.));
#78278=CARTESIAN_POINT('Ctrl Pts',(-58.882826417861,-43.7897527051599,0.));
#78279=CARTESIAN_POINT('Ctrl Pts',(-58.8962398164486,-43.8124714491069,
0.));
#78280=CARTESIAN_POINT('Ctrl Pts',(-58.9096510890128,-43.8352347778419,
0.));
#78281=CARTESIAN_POINT('Ctrl Pts',(-58.9230601446445,-43.8580426352236,
0.));
#78282=CARTESIAN_POINT('Ctrl Pts',(-58.9364668927132,-43.8808949651882,
0.));
#78283=CARTESIAN_POINT('Ctrl Pts',(-58.9498712429066,-43.9037917117748,
0.));
#78284=CARTESIAN_POINT('Ctrl Pts',(-58.9632731052704,-43.9267328191507,
0.));
#78285=CARTESIAN_POINT('Ctrl Pts',(-58.9766723902531,-43.9497182316333,
0.));
#78286=CARTESIAN_POINT('Ctrl Pts',(-58.9900690087404,-43.9727478937053,
0.));
#78287=CARTESIAN_POINT('Ctrl Pts',(-59.0034628721161,-43.9958217500363,
0.));
#78288=CARTESIAN_POINT('Ctrl Pts',(-59.0168538922087,-44.0189397454593,
0.));
#78289=CARTESIAN_POINT('Ctrl Pts',(-59.0302419811772,-44.0421018249219,
0.));
#78290=CARTESIAN_POINT('Ctrl Pts',(-59.0436270514085,-44.0653079334384,
0.));
#78291=CARTESIAN_POINT('Ctrl Pts',(-59.0570090154243,-44.0885580160433,
0.));
#78292=CARTESIAN_POINT('Ctrl Pts',(-59.0703877857529,-44.1118520177223,
0.));
#78293=CARTESIAN_POINT('Ctrl Pts',(-59.0837632749209,-44.1351898834057,
0.));
#78294=CARTESIAN_POINT('Ctrl Pts',(-59.0971353957218,-44.1585715581073,
0.));
#78295=CARTESIAN_POINT('Ctrl Pts',(-59.1105040614285,-44.1819969870314,
0.));
#78296=CARTESIAN_POINT('Ctrl Pts',(-59.1238691860307,-44.2054661156876,
0.));
#78297=CARTESIAN_POINT('Ctrl Pts',(-59.1372306844575,-44.2289788899962,
0.));
#78298=CARTESIAN_POINT('Ctrl Pts',(-59.1505884728194,-44.2525352563979,
0.));
#78299=CARTESIAN_POINT('Ctrl Pts',(-59.1639424678766,-44.2761351616027,
0.));
#78300=CARTESIAN_POINT('Ctrl Pts',(-59.1772925865191,-44.2997785523413,
0.));
#78301=CARTESIAN_POINT('Ctrl Pts',(-59.1906387451971,-44.3234653750877,
0.));
#78302=CARTESIAN_POINT('Ctrl Pts',(-59.2039808594765,-44.3471955758412,
0.));
#78303=CARTESIAN_POINT('Ctrl Pts',(-59.217318843283,-44.3709690997495,0.));
#78304=CARTESIAN_POINT('Ctrl Pts',(-59.2306526095175,-44.394785891411,0.));
#78305=CARTESIAN_POINT('Ctrl Pts',(-59.2439820714231,-44.4186458955486,
0.));
#78306=CARTESIAN_POINT('Ctrl Pts',(-59.2573071437801,-44.4425490575932,
0.));
#78307=CARTESIAN_POINT('Ctrl Pts',(-59.2706277440438,-44.4664953242373,
0.));
#78308=CARTESIAN_POINT('Ctrl Pts',(-59.2839437938187,-44.490484644147,0.));
#78309=CARTESIAN_POINT('Ctrl Pts',(-59.2972552192072,-44.514516968128,0.));
#78310=CARTESIAN_POINT('Ctrl Pts',(-59.3086616639392,-44.5351541478336,
0.));
#78311=CARTESIAN_POINT('Ctrl Pts',(-59.317404187219,-44.5509994357954,0.));
#78312=CARTESIAN_POINT('Ctrl Pts',(-59.3234848865278,-44.5620338188485,
0.));
#78313=CARTESIAN_POINT('Ctrl Pts',(-59.3269051738222,-44.5682447395713,
0.));
#78314=CARTESIAN_POINT('Ctrl Pts',(-59.3276657444158,-44.569626075742,0.));
#78315=CARTESIAN_POINT('',(-56.8466430164621,-40.8467768343956,12.));
#78316=CARTESIAN_POINT('',(-56.8466430164621,-40.8467768343956,0.));
#78317=CARTESIAN_POINT('Ctrl Pts',(-59.3276657444158,-44.569626075742,12.));
#78318=CARTESIAN_POINT('Ctrl Pts',(-59.3269051738222,-44.5682447395712,
12.));
#78319=CARTESIAN_POINT('Ctrl Pts',(-59.3234848865278,-44.5620338188485,
12.));
#78320=CARTESIAN_POINT('Ctrl Pts',(-59.317404187219,-44.5509994357953,12.));
#78321=CARTESIAN_POINT('Ctrl Pts',(-59.3086616639392,-44.5351541478336,
12.));
#78322=CARTESIAN_POINT('Ctrl Pts',(-59.2972552192072,-44.514516968128,12.));
#78323=CARTESIAN_POINT('Ctrl Pts',(-59.2839437938187,-44.490484644147,12.));
#78324=CARTESIAN_POINT('Ctrl Pts',(-59.2706277440438,-44.4664953242373,
12.));
#78325=CARTESIAN_POINT('Ctrl Pts',(-59.2573071437801,-44.4425490575932,
12.));
#78326=CARTESIAN_POINT('Ctrl Pts',(-59.2439820714231,-44.4186458955486,
12.));
#78327=CARTESIAN_POINT('Ctrl Pts',(-59.2306526095175,-44.394785891411,12.));
#78328=CARTESIAN_POINT('Ctrl Pts',(-59.217318843283,-44.3709690997495,12.));
#78329=CARTESIAN_POINT('Ctrl Pts',(-59.2039808594765,-44.3471955758412,
12.));
#78330=CARTESIAN_POINT('Ctrl Pts',(-59.1906387451971,-44.3234653750877,
12.));
#78331=CARTESIAN_POINT('Ctrl Pts',(-59.1772925865191,-44.2997785523413,
12.));
#78332=CARTESIAN_POINT('Ctrl Pts',(-59.1639424678766,-44.2761351616027,
12.));
#78333=CARTESIAN_POINT('Ctrl Pts',(-59.1505884728194,-44.2525352563979,
12.));
#78334=CARTESIAN_POINT('Ctrl Pts',(-59.1372306844575,-44.2289788899962,
12.));
#78335=CARTESIAN_POINT('Ctrl Pts',(-59.1238691860307,-44.2054661156876,
12.));
#78336=CARTESIAN_POINT('Ctrl Pts',(-59.1105040614285,-44.1819969870314,
12.));
#78337=CARTESIAN_POINT('Ctrl Pts',(-59.0971353957218,-44.1585715581073,
12.));
#78338=CARTESIAN_POINT('Ctrl Pts',(-59.0837632749209,-44.1351898834057,
12.));
#78339=CARTESIAN_POINT('Ctrl Pts',(-59.0703877857529,-44.1118520177223,
12.));
#78340=CARTESIAN_POINT('Ctrl Pts',(-59.0570090154243,-44.0885580160433,
12.));
#78341=CARTESIAN_POINT('Ctrl Pts',(-59.0436270514085,-44.0653079334384,
12.));
#78342=CARTESIAN_POINT('Ctrl Pts',(-59.0302419811772,-44.0421018249219,
12.));
#78343=CARTESIAN_POINT('Ctrl Pts',(-59.0168538922087,-44.0189397454593,
12.));
#78344=CARTESIAN_POINT('Ctrl Pts',(-59.0034628721161,-43.9958217500363,
12.));
#78345=CARTESIAN_POINT('Ctrl Pts',(-58.9900690087404,-43.9727478937053,
12.));
#78346=CARTESIAN_POINT('Ctrl Pts',(-58.9766723902531,-43.9497182316333,
12.));
#78347=CARTESIAN_POINT('Ctrl Pts',(-58.9632731052704,-43.9267328191507,
12.));
#78348=CARTESIAN_POINT('Ctrl Pts',(-58.9498712429066,-43.9037917117748,
12.));
#78349=CARTESIAN_POINT('Ctrl Pts',(-58.9364668927132,-43.8808949651882,
12.));
#78350=CARTESIAN_POINT('Ctrl Pts',(-58.9230601446445,-43.8580426352236,
12.));
#78351=CARTESIAN_POINT('Ctrl Pts',(-58.9096510890128,-43.8352347778419,
12.));
#78352=CARTESIAN_POINT('Ctrl Pts',(-58.8962398164486,-43.8124714491069,
12.));
#78353=CARTESIAN_POINT('Ctrl Pts',(-58.882826417861,-43.7897527051599,12.));
#78354=CARTESIAN_POINT('Ctrl Pts',(-58.8694109844636,-43.7670786022392,
12.));
#78355=CARTESIAN_POINT('Ctrl Pts',(-58.8559936077933,-43.7444491966935,
12.));
#78356=CARTESIAN_POINT('Ctrl Pts',(-58.8425743797325,-43.7218645449921,
12.));
#78357=CARTESIAN_POINT('Ctrl Pts',(-58.8291533925299,-43.6993247037318,
12.));
#78358=CARTESIAN_POINT('Ctrl Pts',(-58.8157307388247,-43.6768297296402,
12.));
#78359=CARTESIAN_POINT('Ctrl Pts',(-58.8023065116446,-43.6543796795797,
12.));
#78360=CARTESIAN_POINT('Ctrl Pts',(-58.7888808043976,-43.6319746105487,
12.));
#78361=CARTESIAN_POINT('Ctrl Pts',(-58.7754537108672,-43.6096145796798,
12.));
#78362=CARTESIAN_POINT('Ctrl Pts',(-58.7620253252059,-43.5872996442343,
12.));
#78363=CARTESIAN_POINT('Ctrl Pts',(-58.7485957419296,-43.5650298615911,
12.));
#78364=CARTESIAN_POINT('Ctrl Pts',(-58.7351650559176,-43.5428052892483,
12.));
#78365=CARTESIAN_POINT('Ctrl Pts',(-58.7217333624206,-43.5206259848333,
12.));
#78366=CARTESIAN_POINT('Ctrl Pts',(-58.708300757066,-43.4984920061071,12.));
#78367=CARTESIAN_POINT('Ctrl Pts',(-58.6948673358639,-43.4764034109654,
12.));
#78368=CARTESIAN_POINT('Ctrl Pts',(-58.6814331952138,-43.4543602574352,
12.));
#78369=CARTESIAN_POINT('Ctrl Pts',(-58.6679984319095,-43.4323626036736,
12.));
#78370=CARTESIAN_POINT('Ctrl Pts',(-58.6545631431388,-43.4104105079766,
12.));
#78371=CARTESIAN_POINT('Ctrl Pts',(-58.6411274264854,-43.3885040287808,
12.));
#78372=CARTESIAN_POINT('Ctrl Pts',(-58.627691379929,-43.3666432246634,12.));
#78373=CARTESIAN_POINT('Ctrl Pts',(-58.6142551018473,-43.3448281543374,
12.));
#78374=CARTESIAN_POINT('Ctrl Pts',(-58.6008186910166,-43.3230588766455,
12.));
#78375=CARTESIAN_POINT('Ctrl Pts',(-58.5873822466163,-43.3013354505707,
12.));
#78376=CARTESIAN_POINT('Ctrl Pts',(-58.5739458682317,-43.2796579352405,
12.));
#78377=CARTESIAN_POINT('Ctrl Pts',(-58.5605096558578,-43.2580263899278,
12.));
#78378=CARTESIAN_POINT('Ctrl Pts',(-58.5470737099027,-43.2364408740488,
12.));
#78379=CARTESIAN_POINT('Ctrl Pts',(-58.5336381311911,-43.214901447157,12.));
#78380=CARTESIAN_POINT('Ctrl Pts',(-58.5202030209667,-43.1934081689503,
12.));
#78381=CARTESIAN_POINT('Ctrl Pts',(-58.5067684808946,-43.1719610992771,
12.));
#78382=CARTESIAN_POINT('Ctrl Pts',(-58.4933346130638,-43.1505602981366,
12.));
#78383=CARTESIAN_POINT('Ctrl Pts',(-58.4799015199904,-43.1292058256774,
12.));
#78384=CARTESIAN_POINT('Ctrl Pts',(-58.4664693046206,-43.1078977421908,
12.));
#78385=CARTESIAN_POINT('Ctrl Pts',(-58.4530380703335,-43.0866361081166,
12.));
#78386=CARTESIAN_POINT('Ctrl Pts',(-58.4396079209438,-43.0654209840502,
12.));
#78387=CARTESIAN_POINT('Ctrl Pts',(-58.4261789607055,-43.0442524307432,
12.));
#78388=CARTESIAN_POINT('Ctrl Pts',(-58.4127512943144,-43.0231305091032,
12.));
#78389=CARTESIAN_POINT('Ctrl Pts',(-58.3993250269115,-43.0020552801869,
12.));
#78390=CARTESIAN_POINT('Ctrl Pts',(-58.3859002640871,-42.9810268052043,
12.));
#78391=CARTESIAN_POINT('Ctrl Pts',(-58.3724771118835,-42.9600451455267,
12.));
#78392=CARTESIAN_POINT('Ctrl Pts',(-58.3590556767981,-42.9391103626881,
12.));
#78393=CARTESIAN_POINT('Ctrl Pts',(-58.3456360657861,-42.9182225183851,
12.));
#78394=CARTESIAN_POINT('Ctrl Pts',(-58.3322183862647,-42.8973816744703,
12.));
#78395=CARTESIAN_POINT('Ctrl Pts',(-58.3188027461158,-42.8765878929545,
12.));
#78396=CARTESIAN_POINT('Ctrl Pts',(-58.305389253689,-42.8558412360154,12.));
#78397=CARTESIAN_POINT('Ctrl Pts',(-58.2919780178063,-42.8351417659998,
12.));
#78398=CARTESIAN_POINT('Ctrl Pts',(-58.278569147764,-42.8144895454234,12.));
#78399=CARTESIAN_POINT('Ctrl Pts',(-58.2651627533368,-42.7938846369651,
12.));
#78400=CARTESIAN_POINT('Ctrl Pts',(-58.2517589447818,-42.7733271034678,
12.));
#78401=CARTESIAN_POINT('Ctrl Pts',(-58.238357832842,-42.7528170079482,12.));
#78402=CARTESIAN_POINT('Ctrl Pts',(-58.2249595287497,-42.7323544135983,
12.));
#78403=CARTESIAN_POINT('Ctrl Pts',(-58.2115641442302,-42.7119393837866,
12.));
#78404=CARTESIAN_POINT('Ctrl Pts',(-58.1981717915043,-42.6915719820516,
12.));
#78405=CARTESIAN_POINT('Ctrl Pts',(-58.1847825832932,-42.6712522721021,
12.));
#78406=CARTESIAN_POINT('Ctrl Pts',(-58.1713966328217,-42.6509803178269,
12.));
#78407=CARTESIAN_POINT('Ctrl Pts',(-58.158014053823,-42.6307561832977,12.));
#78408=CARTESIAN_POINT('Ctrl Pts',(-58.1446349605419,-42.6105799327697,
12.));
#78409=CARTESIAN_POINT('Ctrl Pts',(-58.1312594677383,-42.5904516306759,
12.));
#78410=CARTESIAN_POINT('Ctrl Pts',(-58.1178876906905,-42.5703713416263,
12.));
#78411=CARTESIAN_POINT('Ctrl Pts',(-58.1045197452003,-42.5503391304182,
12.));
#78412=CARTESIAN_POINT('Ctrl Pts',(-58.0911557475967,-42.5303550620388,
12.));
#78413=CARTESIAN_POINT('Ctrl Pts',(-58.0777958147404,-42.5104192016664,
12.));
#78414=CARTESIAN_POINT('Ctrl Pts',(-58.064440064027,-42.4905316146649,12.));
#78415=CARTESIAN_POINT('Ctrl Pts',(-58.0510886133917,-42.4706923665838,
12.));
#78416=CARTESIAN_POINT('Ctrl Pts',(-58.0377415813132,-42.4509015231667,
12.));
#78417=CARTESIAN_POINT('Ctrl Pts',(-58.0243990868175,-42.4311591503551,
12.));
#78418=CARTESIAN_POINT('Ctrl Pts',(-58.011061249483,-42.4114653142891,12.));
#78419=CARTESIAN_POINT('Ctrl Pts',(-57.9977281894437,-42.3918200813024,
12.));
#78420=CARTESIAN_POINT('Ctrl Pts',(-57.9844000273936,-42.3722235179216,
12.));
#78421=CARTESIAN_POINT('Ctrl Pts',(-57.9710768845923,-42.3526756908764,
12.));
#78422=CARTESIAN_POINT('Ctrl Pts',(-57.9577588828693,-42.3331766671028,
12.));
#78423=CARTESIAN_POINT('Ctrl Pts',(-57.9444461446292,-42.3137265137446,
12.));
#78424=CARTESIAN_POINT('Ctrl Pts',(-57.9311387928541,-42.2943252981471,
12.));
#78425=CARTESIAN_POINT('Ctrl Pts',(-57.9178369511084,-42.274973087857,12.));
#78426=CARTESIAN_POINT('Ctrl Pts',(-57.9045407435447,-42.2556699506332,
12.));
#78427=CARTESIAN_POINT('Ctrl Pts',(-57.8912502949084,-42.2364159544492,
12.));
#78428=CARTESIAN_POINT('Ctrl Pts',(-57.8779657305423,-42.2172111674945,
12.));
#78429=CARTESIAN_POINT('Ctrl Pts',(-57.86468717639,-42.1980556581688,12.));
#78430=CARTESIAN_POINT('Ctrl Pts',(-57.8514147590012,-42.1789494950824,
12.));
#78431=CARTESIAN_POINT('Ctrl Pts',(-57.8381486055376,-42.1598927470671,
12.));
#78432=CARTESIAN_POINT('Ctrl Pts',(-57.8248888437787,-42.1408854831791,
12.));
#78433=CARTESIAN_POINT('Ctrl Pts',(-57.8116356021274,-42.121927772701,12.));
#78434=CARTESIAN_POINT('Ctrl Pts',(-57.798389009613,-42.1030196851344,12.));
#78435=CARTESIAN_POINT('Ctrl Pts',(-57.7851491958954,-42.0841612902018,
12.));
#78436=CARTESIAN_POINT('Ctrl Pts',(-57.7719162912721,-42.0653526578571,
12.));
#78437=CARTESIAN_POINT('Ctrl Pts',(-57.7586904266828,-42.0465938582877,
12.));
#78438=CARTESIAN_POINT('Ctrl Pts',(-57.7454717337151,-42.0278849619156,
12.));
#78439=CARTESIAN_POINT('Ctrl Pts',(-57.7322603446086,-42.0092260393911,
12.));
#78440=CARTESIAN_POINT('Ctrl Pts',(-57.7190563922614,-41.9906171615974,
12.));
#78441=CARTESIAN_POINT('Ctrl Pts',(-57.7058600102365,-41.9720583996601,
12.));
#78442=CARTESIAN_POINT('Ctrl Pts',(-57.6926713327674,-41.9535498249489,
12.));
#78443=CARTESIAN_POINT('Ctrl Pts',(-57.6794904947641,-41.9350915090791,
12.));
#78444=CARTESIAN_POINT('Ctrl Pts',(-57.6663176318176,-41.9166835239046,
12.));
#78445=CARTESIAN_POINT('Ctrl Pts',(-57.6531528802059,-41.8983259415244,
12.));
#78446=CARTESIAN_POINT('Ctrl Pts',(-57.6399963769003,-41.8800188342908,
12.));
#78447=CARTESIAN_POINT('Ctrl Pts',(-57.6268482595702,-41.8617622748108,
12.));
#78448=CARTESIAN_POINT('Ctrl Pts',(-57.6137086665882,-41.8435563359456,
12.));
#78449=CARTESIAN_POINT('Ctrl Pts',(-57.6005777370349,-41.8254010908051,
12.));
#78450=CARTESIAN_POINT('Ctrl Pts',(-57.5874556107056,-41.8072966127558,
12.));
#78451=CARTESIAN_POINT('Ctrl Pts',(-57.5743424281205,-41.7892429754297,
12.));
#78452=CARTESIAN_POINT('Ctrl Pts',(-57.561238330532,-41.7712402527273,12.));
#78453=CARTESIAN_POINT('Ctrl Pts',(-57.5481434599335,-41.7532885188174,
12.));
#78454=CARTESIAN_POINT('Ctrl Pts',(-57.5350579590649,-41.7353878481336,
12.));
#78455=CARTESIAN_POINT('Ctrl Pts',(-57.5219819714171,-41.7175383153821,
12.));
#78456=CARTESIAN_POINT('Ctrl Pts',(-57.5089156412343,-41.6997399955447,
12.));
#78457=CARTESIAN_POINT('Ctrl Pts',(-57.4958591135165,-41.6819929638797,
12.));
#78458=CARTESIAN_POINT('Ctrl Pts',(-57.4828125340218,-41.6642972959165,
12.));
#78459=CARTESIAN_POINT('Ctrl Pts',(-57.4697760492683,-41.6466530674514,
12.));
#78460=CARTESIAN_POINT('Ctrl Pts',(-57.4567498065562,-41.6290603545666,
12.));
#78461=CARTESIAN_POINT('Ctrl Pts',(-57.4437339539841,-41.6115192336388,
12.));
#78462=CARTESIAN_POINT('Ctrl Pts',(-57.4307286404662,-41.5940297813477,
12.));
#78463=CARTESIAN_POINT('Ctrl Pts',(-57.4177340157508,-41.5765920746777,
12.));
#78464=CARTESIAN_POINT('Ctrl Pts',(-57.4047502304231,-41.5592061909176,
12.));
#78465=CARTESIAN_POINT('Ctrl Pts',(-57.3917774358863,-41.5418722076572,
12.));
#78466=CARTESIAN_POINT('Ctrl Pts',(-57.3788157843454,-41.524590202777,12.));
#78467=CARTESIAN_POINT('Ctrl Pts',(-57.3658654287937,-41.5073602544396,
12.));
#78468=CARTESIAN_POINT('Ctrl Pts',(-57.3529265229835,-41.4901824410636,
12.));
#78469=CARTESIAN_POINT('Ctrl Pts',(-57.3399992214717,-41.4730568413518,
12.));
#78470=CARTESIAN_POINT('Ctrl Pts',(-57.3270836796911,-41.4559835343328,
12.));
#78471=CARTESIAN_POINT('Ctrl Pts',(-57.3141800540137,-41.4389625993948,
12.));
#78472=CARTESIAN_POINT('Ctrl Pts',(-57.3012885018151,-41.4219941163163,
12.));
#78473=CARTESIAN_POINT('Ctrl Pts',(-57.2884091815406,-41.4050781652938,
12.));
#78474=CARTESIAN_POINT('Ctrl Pts',(-57.2755422525844,-41.3882148268813,
12.));
#78475=CARTESIAN_POINT('Ctrl Pts',(-57.2626878751596,-41.3714041819223,
12.));
#78476=CARTESIAN_POINT('Ctrl Pts',(-57.2498462101879,-41.3546463114885,
12.));
#78477=CARTESIAN_POINT('Ctrl Pts',(-57.2370174191401,-41.3379412967875,
12.));
#78478=CARTESIAN_POINT('Ctrl Pts',(-57.2242016640198,-41.321289219149,12.));
#78479=CARTESIAN_POINT('Ctrl Pts',(-57.2113991077302,-41.3046901602293,
12.));
#78480=CARTESIAN_POINT('Ctrl Pts',(-57.1986099143983,-41.2881442021863,
12.));
#78481=CARTESIAN_POINT('Ctrl Pts',(-57.1858342496538,-41.2716514278276,
12.));
#78482=CARTESIAN_POINT('Ctrl Pts',(-57.17307228108,-41.2552119208465,12.));
#78483=CARTESIAN_POINT('Ctrl Pts',(-57.1603241779077,-41.2388257656559,
12.));
#78484=CARTESIAN_POINT('Ctrl Pts',(-57.147590110182,-41.222493046943,12.));
#78485=CARTESIAN_POINT('Ctrl Pts',(-57.1348702480647,-41.2062138492915,
12.));
#78486=CARTESIAN_POINT('Ctrl Pts',(-57.1221647611207,-41.1899882567923,
12.));
#78487=CARTESIAN_POINT('Ctrl Pts',(-57.1094738174957,-41.1738163525901,
12.));
#78488=CARTESIAN_POINT('Ctrl Pts',(-57.0967975854874,-41.1576982197374,
12.));
#78489=CARTESIAN_POINT('Ctrl Pts',(-57.084136235426,-41.1416339422117,12.));
#78490=CARTESIAN_POINT('Ctrl Pts',(-57.0714899412099,-41.1256236057442,
12.));
#78491=CARTESIAN_POINT('Ctrl Pts',(-57.0588588825298,-41.1096672990148,
12.));
#78492=CARTESIAN_POINT('Ctrl Pts',(-57.046243245068,-41.0937651137549,12.));
#78493=CARTESIAN_POINT('Ctrl Pts',(-57.0336432158536,-41.0779171422438,
12.));
#78494=CARTESIAN_POINT('Ctrl Pts',(-57.0210589791788,-41.0621234751007,
12.));
#78495=CARTESIAN_POINT('Ctrl Pts',(-57.008490713042,-41.0463841993608,12.));
#78496=CARTESIAN_POINT('Ctrl Pts',(-56.995938583472,-41.0306993953988,12.));
#78497=CARTESIAN_POINT('Ctrl Pts',(-56.9834027500117,-41.0150691398947,
12.));
#78498=CARTESIAN_POINT('Ctrl Pts',(-56.9708833766137,-40.9994935117276,
12.));
#78499=CARTESIAN_POINT('Ctrl Pts',(-56.9583806404069,-40.9839725967121,
12.));
#78500=CARTESIAN_POINT('Ctrl Pts',(-56.9458947422608,-40.9685064933074,
12.));
#78501=CARTESIAN_POINT('Ctrl Pts',(-56.9334259140049,-40.9530953165031,
12.));
#78502=CARTESIAN_POINT('Ctrl Pts',(-56.9209743960992,-40.9377391857128,
12.));
#78503=CARTESIAN_POINT('Ctrl Pts',(-56.9085404164502,-40.9224382132427,
12.));
#78504=CARTESIAN_POINT('Ctrl Pts',(-56.8961241708861,-40.9071924937508,
12.));
#78505=CARTESIAN_POINT('Ctrl Pts',(-56.8837257978343,-40.8920020903293,
12.));
#78506=CARTESIAN_POINT('Ctrl Pts',(-56.8713453764905,-40.8768670342052,
12.));
#78507=CARTESIAN_POINT('Ctrl Pts',(-56.8614554317668,-40.864803275942,12.));
#78508=CARTESIAN_POINT('Ctrl Pts',(-56.8540460739472,-40.8557803680277,
12.));
#78509=CARTESIAN_POINT('Ctrl Pts',(-56.8491101022591,-40.8497761671036,
12.));
#78510=CARTESIAN_POINT('Ctrl Pts',(-56.8466430164621,-40.8467768343956,
12.));
#78511=CARTESIAN_POINT('Ctrl Pts',(-58.4060826907797,-45.7706564944896,
-5.55111512312578E-16));
#78512=CARTESIAN_POINT('Ctrl Pts',(-58.4060826907797,-45.7706564944896,
4.));
#78513=CARTESIAN_POINT('Ctrl Pts',(-58.4060826907797,-45.7706564944896,
8.));
#78514=CARTESIAN_POINT('Ctrl Pts',(-58.4060826907797,-45.7706564944896,
12.));
#78515=CARTESIAN_POINT('Ctrl Pts',(-58.5127761886847,-45.7969367893064,
-5.55111512312578E-16));
#78516=CARTESIAN_POINT('Ctrl Pts',(-58.5127761886847,-45.7969367893064,
4.));
#78517=CARTESIAN_POINT('Ctrl Pts',(-58.5127761886847,-45.7969367893064,
8.00000000000001));
#78518=CARTESIAN_POINT('Ctrl Pts',(-58.5127761886847,-45.7969367893064,
12.));
#78519=CARTESIAN_POINT('Ctrl Pts',(-58.714632205056,-45.7788617791411,-5.55111512312578E-16));
#78520=CARTESIAN_POINT('Ctrl Pts',(-58.714632205056,-45.7788617791411,4.));
#78521=CARTESIAN_POINT('Ctrl Pts',(-58.714632205056,-45.7788617791411,7.99999999999999));
#78522=CARTESIAN_POINT('Ctrl Pts',(-58.714632205056,-45.7788617791411,12.));
#78523=CARTESIAN_POINT('Ctrl Pts',(-58.870677144318,-45.6563266621663,-5.55111512312578E-16));
#78524=CARTESIAN_POINT('Ctrl Pts',(-58.870677144318,-45.6563266621663,4.));
#78525=CARTESIAN_POINT('Ctrl Pts',(-58.870677144318,-45.6563266621663,8.00000000000001));
#78526=CARTESIAN_POINT('Ctrl Pts',(-58.870677144318,-45.6563266621663,12.));
#78527=CARTESIAN_POINT('Ctrl Pts',(-58.9211100416378,-45.5911481700252,
-5.55111512312578E-16));
#78528=CARTESIAN_POINT('Ctrl Pts',(-58.9211100416378,-45.5911481700252,
4.));
#78529=CARTESIAN_POINT('Ctrl Pts',(-58.9211100416378,-45.5911481700252,
8.));
#78530=CARTESIAN_POINT('Ctrl Pts',(-58.9211100416378,-45.5911481700252,
12.));
#78531=CARTESIAN_POINT('',(-58.4060826907797,-45.7706564944896,2.77555756156289E-16));
#78532=CARTESIAN_POINT('',(-58.9211100416379,-45.5911481700253,0.));
#78533=CARTESIAN_POINT('Ctrl Pts',(-58.4060826907797,-45.7706564944896,
-1.38777878078145E-16));
#78534=CARTESIAN_POINT('Ctrl Pts',(-58.5127761886847,-45.7969367893064,
-1.38777878078145E-16));
#78535=CARTESIAN_POINT('Ctrl Pts',(-58.628122483754,-45.7866082120691,-1.38777878078144E-16));
#78536=CARTESIAN_POINT('Ctrl Pts',(-58.7285100597672,-45.7421702122001,
-1.38777878078145E-16));
#78537=CARTESIAN_POINT('Ctrl Pts',(-58.8038007417772,-45.7088417122983,
-1.38777878078145E-16));
#78538=CARTESIAN_POINT('Ctrl Pts',(-58.870677144318,-45.6563266621663,-1.38777878078145E-16));
#78539=CARTESIAN_POINT('Ctrl Pts',(-58.9211100416378,-45.5911481700252,
-1.38777878078145E-16));
#78540=CARTESIAN_POINT('',(-58.9211100416379,-45.5911481700253,12.));
#78541=CARTESIAN_POINT('Ctrl Pts',(-58.9211100416378,-45.5911481700252,
-5.55111512312578E-16));
#78542=CARTESIAN_POINT('Ctrl Pts',(-58.9211100416378,-45.5911481700252,
4.));
#78543=CARTESIAN_POINT('Ctrl Pts',(-58.9211100416378,-45.5911481700252,
8.));
#78544=CARTESIAN_POINT('Ctrl Pts',(-58.9211100416378,-45.5911481700252,
12.));
#78545=CARTESIAN_POINT('',(-58.4060826907797,-45.7706564944896,12.));
#78546=CARTESIAN_POINT('Ctrl Pts',(-58.9211100416378,-45.5911481700252,
12.));
#78547=CARTESIAN_POINT('Ctrl Pts',(-58.870677144318,-45.6563266621663,12.));
#78548=CARTESIAN_POINT('Ctrl Pts',(-58.8038007417772,-45.7088417122983,
12.));
#78549=CARTESIAN_POINT('Ctrl Pts',(-58.7285100597672,-45.7421702122001,
12.));
#78550=CARTESIAN_POINT('Ctrl Pts',(-58.628122483754,-45.7866082120691,12.));
#78551=CARTESIAN_POINT('Ctrl Pts',(-58.5127761886847,-45.7969367893064,
12.));
#78552=CARTESIAN_POINT('Ctrl Pts',(-58.4060826907797,-45.7706564944896,
12.));
#78553=CARTESIAN_POINT('Ctrl Pts',(-58.4060826907797,-45.7706564944896,
12.));
#78554=CARTESIAN_POINT('Ctrl Pts',(-58.4060826907797,-45.7706564944896,
8.));
#78555=CARTESIAN_POINT('Ctrl Pts',(-58.4060826907797,-45.7706564944896,
4.));
#78556=CARTESIAN_POINT('Ctrl Pts',(-58.4060826907797,-45.7706564944896,
-5.55111512312578E-16));
#78557=CARTESIAN_POINT('Origin',(-2.97323128204029E-10,-2.28269173065022E-10,
0.));
#78558=CARTESIAN_POINT('Origin',(-2.97323128204029E-10,-2.28269173065022E-10,
12.));
#78559=CARTESIAN_POINT('Origin',(-2.97323128204029E-10,-2.28269173065022E-10,
0.));
#78560=CARTESIAN_POINT('Ctrl Pts',(-62.9938720098768,-39.77464128315,0.));
#78561=CARTESIAN_POINT('Ctrl Pts',(-62.9938720098768,-39.77464128315,4.));
#78562=CARTESIAN_POINT('Ctrl Pts',(-62.9938720098768,-39.7746412831501,
8.));
#78563=CARTESIAN_POINT('Ctrl Pts',(-62.9938720098768,-39.7746412831501,
12.));
#78564=CARTESIAN_POINT('Ctrl Pts',(-63.0525369183205,-39.6817295782357,
0.));
#78565=CARTESIAN_POINT('Ctrl Pts',(-63.0525369183205,-39.6817295782357,
4.));
#78566=CARTESIAN_POINT('Ctrl Pts',(-63.0525369183204,-39.6817295782358,
8.00000000000001));
#78567=CARTESIAN_POINT('Ctrl Pts',(-63.0525369183204,-39.6817295782358,
12.));
#78568=CARTESIAN_POINT('Ctrl Pts',(-63.0992090147611,-39.4845131830964,
-7.30833037965888E-17));
#78569=CARTESIAN_POINT('Ctrl Pts',(-63.0992090147611,-39.4845131830964,
4.00000000000001));
#78570=CARTESIAN_POINT('Ctrl Pts',(-63.099209014761,-39.4845131830966,7.99999999999999));
#78571=CARTESIAN_POINT('Ctrl Pts',(-63.099209014761,-39.4845131830966,12.));
#78572=CARTESIAN_POINT('Ctrl Pts',(-63.0322949727907,-39.2977314459977,
-2.46611180232692E-16));
#78573=CARTESIAN_POINT('Ctrl Pts',(-63.0322949727907,-39.2977314459977,
4.));
#78574=CARTESIAN_POINT('Ctrl Pts',(-63.0322949727907,-39.2977314459979,
8.00000000000001));
#78575=CARTESIAN_POINT('Ctrl Pts',(-63.0322949727907,-39.2977314459979,
12.));
#78576=CARTESIAN_POINT('Ctrl Pts',(-62.9864049293633,-39.2292784191459,
-3.30265160470176E-16));
#78577=CARTESIAN_POINT('Ctrl Pts',(-62.9864049293633,-39.2292784191459,
4.));
#78578=CARTESIAN_POINT('Ctrl Pts',(-62.9864049293633,-39.2292784191462,
8.));
#78579=CARTESIAN_POINT('Ctrl Pts',(-62.9864049293633,-39.2292784191462,
12.));
#78580=CARTESIAN_POINT('',(-62.9938720098768,-39.77464128315,0.));
#78581=CARTESIAN_POINT('',(-62.9864049293628,-39.2292784191463,0.));
#78582=CARTESIAN_POINT('Ctrl Pts',(-62.9938720098768,-39.77464128315,2.74425517504379E-17));
#78583=CARTESIAN_POINT('Ctrl Pts',(-63.0525369183205,-39.6817295782357,
2.74425517504379E-17));
#78584=CARTESIAN_POINT('Ctrl Pts',(-63.0792066877151,-39.569034495299,-1.43193361333271E-17));
#78585=CARTESIAN_POINT('Ctrl Pts',(-63.0687871057919,-39.4597466476407,
-8.887945181775E-17));
#78586=CARTESIAN_POINT('Ctrl Pts',(-63.0609724193495,-39.3777807618971,
-1.44799538581067E-16));
#78587=CARTESIAN_POINT('Ctrl Pts',(-63.0322949727907,-39.2977314459977,
-2.19168628482255E-16));
#78588=CARTESIAN_POINT('Ctrl Pts',(-62.9864049293633,-39.2292784191459,
-3.02822608719738E-16));
#78589=CARTESIAN_POINT('',(-62.9864049293629,-39.2292784191464,12.));
#78590=CARTESIAN_POINT('Ctrl Pts',(-62.9864049293633,-39.2292784191459,
-3.30265160470176E-16));
#78591=CARTESIAN_POINT('Ctrl Pts',(-62.9864049293633,-39.2292784191459,
4.));
#78592=CARTESIAN_POINT('Ctrl Pts',(-62.9864049293633,-39.2292784191462,
8.));
#78593=CARTESIAN_POINT('Ctrl Pts',(-62.9864049293633,-39.2292784191462,
12.));
#78594=CARTESIAN_POINT('',(-62.9938720098768,-39.7746412831501,12.));
#78595=CARTESIAN_POINT('Ctrl Pts',(-62.9864049293633,-39.2292784191462,
12.));
#78596=CARTESIAN_POINT('Ctrl Pts',(-63.0322949727907,-39.2977314459979,
12.));
#78597=CARTESIAN_POINT('Ctrl Pts',(-63.0609724193494,-39.3777807618974,
12.));
#78598=CARTESIAN_POINT('Ctrl Pts',(-63.0687871057918,-39.459746647641,12.));
#78599=CARTESIAN_POINT('Ctrl Pts',(-63.079206687715,-39.5690344952991,12.));
#78600=CARTESIAN_POINT('Ctrl Pts',(-63.0525369183204,-39.6817295782358,
12.));
#78601=CARTESIAN_POINT('Ctrl Pts',(-62.9938720098768,-39.7746412831501,
12.));
#78602=CARTESIAN_POINT('Ctrl Pts',(-62.9938720098768,-39.7746412831501,
12.));
#78603=CARTESIAN_POINT('Ctrl Pts',(-62.9938720098768,-39.7746412831501,
8.));
#78604=CARTESIAN_POINT('Ctrl Pts',(-62.9938720098768,-39.77464128315,4.));
#78605=CARTESIAN_POINT('Ctrl Pts',(-62.9938720098768,-39.77464128315,0.));
#78606=CARTESIAN_POINT('Ctrl Pts',(-60.1903555511633,-35.7368311217509,
0.));
#78607=CARTESIAN_POINT('Ctrl Pts',(-60.1903555511633,-35.7368311217509,
12.));
#78608=CARTESIAN_POINT('Ctrl Pts',(-60.1930746580239,-35.7396040203973,
0.));
#78609=CARTESIAN_POINT('Ctrl Pts',(-60.1930746580239,-35.7396040203973,
12.));
#78610=CARTESIAN_POINT('Ctrl Pts',(-60.1985151474406,-35.7451551752456,
0.));
#78611=CARTESIAN_POINT('Ctrl Pts',(-60.1985151474406,-35.7451551752456,
12.));
#78612=CARTESIAN_POINT('Ctrl Pts',(-60.2066827086579,-35.7534979801871,
0.));
#78613=CARTESIAN_POINT('Ctrl Pts',(-60.2066827086579,-35.7534979801871,
12.));
#78614=CARTESIAN_POINT('Ctrl Pts',(-60.2175864449678,-35.7646538667299,
0.));
#78615=CARTESIAN_POINT('Ctrl Pts',(-60.2175864449678,-35.7646538667299,
12.));
#78616=CARTESIAN_POINT('Ctrl Pts',(-60.2312388621286,-35.7786523045782,
0.));
#78617=CARTESIAN_POINT('Ctrl Pts',(-60.2312388621286,-35.7786523045782,
12.));
#78618=CARTESIAN_POINT('Ctrl Pts',(-60.2449139865206,-35.7927043145164,
0.));
#78619=CARTESIAN_POINT('Ctrl Pts',(-60.2449139865206,-35.7927043145164,
12.));
#78620=CARTESIAN_POINT('Ctrl Pts',(-60.2586117365278,-35.8068098723386,
0.));
#78621=CARTESIAN_POINT('Ctrl Pts',(-60.2586117365278,-35.8068098723386,
12.));
#78622=CARTESIAN_POINT('Ctrl Pts',(-60.2723319687507,-35.8209689272574,
0.));
#78623=CARTESIAN_POINT('Ctrl Pts',(-60.2723319687507,-35.8209689272574,
12.));
#78624=CARTESIAN_POINT('Ctrl Pts',(-60.2860744798563,-35.8351814020424,
0.));
#78625=CARTESIAN_POINT('Ctrl Pts',(-60.2860744798563,-35.8351814020424,
12.));
#78626=CARTESIAN_POINT('Ctrl Pts',(-60.2998390330173,-35.8494472046783,
0.));
#78627=CARTESIAN_POINT('Ctrl Pts',(-60.2998390330173,-35.8494472046783,
12.));
#78628=CARTESIAN_POINT('Ctrl Pts',(-60.313625378281,-35.8637662371635,0.));
#78629=CARTESIAN_POINT('Ctrl Pts',(-60.313625378281,-35.8637662371635,12.));
#78630=CARTESIAN_POINT('Ctrl Pts',(-60.3274332746782,-35.878138405151,0.));
#78631=CARTESIAN_POINT('Ctrl Pts',(-60.3274332746782,-35.878138405151,12.));
#78632=CARTESIAN_POINT('Ctrl Pts',(-60.3412625135223,-35.8925636280632,
0.));
#78633=CARTESIAN_POINT('Ctrl Pts',(-60.3412625135223,-35.8925636280632,
12.));
#78634=CARTESIAN_POINT('Ctrl Pts',(-60.3551129108794,-35.9070418358501,
0.));
#78635=CARTESIAN_POINT('Ctrl Pts',(-60.3551129108794,-35.9070418358501,
12.));
#78636=CARTESIAN_POINT('Ctrl Pts',(-60.368984296546,-35.9215729642219,0.));
#78637=CARTESIAN_POINT('Ctrl Pts',(-60.368984296546,-35.9215729642219,12.));
#78638=CARTESIAN_POINT('Ctrl Pts',(-60.3828765049031,-35.9361569506955,
0.));
#78639=CARTESIAN_POINT('Ctrl Pts',(-60.3828765049031,-35.9361569506955,
12.));
#78640=CARTESIAN_POINT('Ctrl Pts',(-60.3967893635487,-35.9507937296726,
0.));
#78641=CARTESIAN_POINT('Ctrl Pts',(-60.3967893635487,-35.9507937296726,
12.));
#78642=CARTESIAN_POINT('Ctrl Pts',(-60.4107226875759,-35.9654832299627,
0.));
#78643=CARTESIAN_POINT('Ctrl Pts',(-60.4107226875759,-35.9654832299627,
12.));
#78644=CARTESIAN_POINT('Ctrl Pts',(-60.4246762854961,-35.9802253773534,
0.));
#78645=CARTESIAN_POINT('Ctrl Pts',(-60.4246762854961,-35.9802253773534,
12.));
#78646=CARTESIAN_POINT('Ctrl Pts',(-60.438649962949,-35.9950200962175,0.));
#78647=CARTESIAN_POINT('Ctrl Pts',(-60.438649962949,-35.9950200962175,12.));
#78648=CARTESIAN_POINT('Ctrl Pts',(-60.452643526964,-36.0098673113556,0.));
#78649=CARTESIAN_POINT('Ctrl Pts',(-60.452643526964,-36.0098673113556,12.));
#78650=CARTESIAN_POINT('Ctrl Pts',(-60.4666567908053,-36.0247669500867,
0.));
#78651=CARTESIAN_POINT('Ctrl Pts',(-60.4666567908053,-36.0247669500867,
12.));
#78652=CARTESIAN_POINT('Ctrl Pts',(-60.4806895737643,-36.0397189421617,
0.));
#78653=CARTESIAN_POINT('Ctrl Pts',(-60.4806895737643,-36.0397189421617,
12.));
#78654=CARTESIAN_POINT('Ctrl Pts',(-60.4947416988396,-36.0547232187681,
0.));
#78655=CARTESIAN_POINT('Ctrl Pts',(-60.4947416988396,-36.0547232187681,
12.));
#78656=CARTESIAN_POINT('Ctrl Pts',(-60.5088129911357,-36.0697797118377,
0.));
#78657=CARTESIAN_POINT('Ctrl Pts',(-60.5088129911357,-36.0697797118377,
12.));
#78658=CARTESIAN_POINT('Ctrl Pts',(-60.5229032759001,-36.0848883531968,
0.));
#78659=CARTESIAN_POINT('Ctrl Pts',(-60.5229032759001,-36.0848883531968,
12.));
#78660=CARTESIAN_POINT('Ctrl Pts',(-60.5370123768841,-36.1000490738532,
0.));
#78661=CARTESIAN_POINT('Ctrl Pts',(-60.5370123768841,-36.1000490738532,
12.));
#78662=CARTESIAN_POINT('Ctrl Pts',(-60.5511401172014,-36.1152618043756,
0.));
#78663=CARTESIAN_POINT('Ctrl Pts',(-60.5511401172014,-36.1152618043756,
12.));
#78664=CARTESIAN_POINT('Ctrl Pts',(-60.5652863200732,-36.1305264752195,
0.));
#78665=CARTESIAN_POINT('Ctrl Pts',(-60.5652863200732,-36.1305264752195,
12.));
#78666=CARTESIAN_POINT('Ctrl Pts',(-60.5794508095555,-36.1458430170425,
0.));
#78667=CARTESIAN_POINT('Ctrl Pts',(-60.5794508095555,-36.1458430170425,
12.));
#78668=CARTESIAN_POINT('Ctrl Pts',(-60.5936334114083,-36.1612113610758,
0.));
#78669=CARTESIAN_POINT('Ctrl Pts',(-60.5936334114083,-36.1612113610758,
12.));
#78670=CARTESIAN_POINT('Ctrl Pts',(-60.6078339534151,-36.1766314392624,
0.));
#78671=CARTESIAN_POINT('Ctrl Pts',(-60.6078339534151,-36.1766314392624,
12.));
#78672=CARTESIAN_POINT('Ctrl Pts',(-60.6220522649129,-36.1921031840617,
0.));
#78673=CARTESIAN_POINT('Ctrl Pts',(-60.6220522649129,-36.1921031840617,
12.));
#78674=CARTESIAN_POINT('Ctrl Pts',(-60.6362881765014,-36.2076265283261,
0.));
#78675=CARTESIAN_POINT('Ctrl Pts',(-60.6362881765014,-36.2076265283261,
12.));
#78676=CARTESIAN_POINT('Ctrl Pts',(-60.6505415197055,-36.2232014051549,
0.));
#78677=CARTESIAN_POINT('Ctrl Pts',(-60.6505415197055,-36.2232014051549,
12.));
#78678=CARTESIAN_POINT('Ctrl Pts',(-60.6648121265908,-36.2388277477225,
0.));
#78679=CARTESIAN_POINT('Ctrl Pts',(-60.6648121265908,-36.2388277477225,
12.));
#78680=CARTESIAN_POINT('Ctrl Pts',(-60.6790998297823,-36.2545054892911,
0.));
#78681=CARTESIAN_POINT('Ctrl Pts',(-60.6790998297823,-36.2545054892911,
12.));
#78682=CARTESIAN_POINT('Ctrl Pts',(-60.6934044626304,-36.2702345632882,
0.));
#78683=CARTESIAN_POINT('Ctrl Pts',(-60.6934044626304,-36.2702345632882,
12.));
#78684=CARTESIAN_POINT('Ctrl Pts',(-60.7077258593268,-36.2860149033586,
0.));
#78685=CARTESIAN_POINT('Ctrl Pts',(-60.7077258593268,-36.2860149033586,
12.));
#78686=CARTESIAN_POINT('Ctrl Pts',(-60.7220638550396,-36.3018464434204,
0.));
#78687=CARTESIAN_POINT('Ctrl Pts',(-60.7220638550396,-36.3018464434204,
12.));
#78688=CARTESIAN_POINT('Ctrl Pts',(-60.7364182860388,-36.3177291177148,
0.));
#78689=CARTESIAN_POINT('Ctrl Pts',(-60.7364182860388,-36.3177291177148,
12.));
#78690=CARTESIAN_POINT('Ctrl Pts',(-60.7507889896284,-36.3336628607844,
0.));
#78691=CARTESIAN_POINT('Ctrl Pts',(-60.7507889896284,-36.3336628607844,
12.));
#78692=CARTESIAN_POINT('Ctrl Pts',(-60.7651758040792,-36.349647607448,0.));
#78693=CARTESIAN_POINT('Ctrl Pts',(-60.7651758040792,-36.349647607448,12.));
#78694=CARTESIAN_POINT('Ctrl Pts',(-60.7795785685631,-36.3656832927733,
0.));
#78695=CARTESIAN_POINT('Ctrl Pts',(-60.7795785685631,-36.3656832927733,
12.));
#78696=CARTESIAN_POINT('Ctrl Pts',(-60.7939971230781,-36.38176985204,0.));
#78697=CARTESIAN_POINT('Ctrl Pts',(-60.7939971230781,-36.38176985204,12.));
#78698=CARTESIAN_POINT('Ctrl Pts',(-60.8084313084009,-36.3979072207174,
0.));
#78699=CARTESIAN_POINT('Ctrl Pts',(-60.8084313084009,-36.3979072207174,
12.));
#78700=CARTESIAN_POINT('Ctrl Pts',(-60.8228809661179,-36.4140953344869,
0.));
#78701=CARTESIAN_POINT('Ctrl Pts',(-60.8228809661179,-36.4140953344869,
12.));
#78702=CARTESIAN_POINT('Ctrl Pts',(-60.8373459386397,-36.4303341292497,
0.));
#78703=CARTESIAN_POINT('Ctrl Pts',(-60.8373459386397,-36.4303341292497,
12.));
#78704=CARTESIAN_POINT('Ctrl Pts',(-60.851826069218,-36.4466235411353,0.));
#78705=CARTESIAN_POINT('Ctrl Pts',(-60.851826069218,-36.4466235411353,12.));
#78706=CARTESIAN_POINT('Ctrl Pts',(-60.8663212019646,-36.4629635065037,
0.));
#78707=CARTESIAN_POINT('Ctrl Pts',(-60.8663212019646,-36.4629635065037,
12.));
#78708=CARTESIAN_POINT('Ctrl Pts',(-60.8808311818489,-36.4793539619459,
0.));
#78709=CARTESIAN_POINT('Ctrl Pts',(-60.8808311818489,-36.4793539619459,
12.));
#78710=CARTESIAN_POINT('Ctrl Pts',(-60.8953558546791,-36.4957948442832,
0.));
#78711=CARTESIAN_POINT('Ctrl Pts',(-60.8953558546791,-36.4957948442832,
12.));
#78712=CARTESIAN_POINT('Ctrl Pts',(-60.9098950670847,-36.5122860905611,
0.));
#78713=CARTESIAN_POINT('Ctrl Pts',(-60.9098950670847,-36.5122860905611,
12.));
#78714=CARTESIAN_POINT('Ctrl Pts',(-60.924448666499,-36.5288276380417,0.));
#78715=CARTESIAN_POINT('Ctrl Pts',(-60.924448666499,-36.5288276380417,12.));
#78716=CARTESIAN_POINT('Ctrl Pts',(-60.9390165011357,-36.5454194241866,
0.));
#78717=CARTESIAN_POINT('Ctrl Pts',(-60.9390165011357,-36.5454194241866,
12.));
#78718=CARTESIAN_POINT('Ctrl Pts',(-60.9535984199874,-36.5620613866615,
0.));
#78719=CARTESIAN_POINT('Ctrl Pts',(-60.9535984199874,-36.5620613866615,
12.));
#78720=CARTESIAN_POINT('Ctrl Pts',(-60.9681942728237,-36.5787534633416,
0.));
#78721=CARTESIAN_POINT('Ctrl Pts',(-60.9681942728237,-36.5787534633416,
12.));
#78722=CARTESIAN_POINT('Ctrl Pts',(-60.9828039101887,-36.5954955923109,
0.));
#78723=CARTESIAN_POINT('Ctrl Pts',(-60.9828039101887,-36.5954955923109,
12.));
#78724=CARTESIAN_POINT('Ctrl Pts',(-60.9974271833982,-36.6122877118599,
0.));
#78725=CARTESIAN_POINT('Ctrl Pts',(-60.9974271833982,-36.6122877118599,
12.));
#78726=CARTESIAN_POINT('Ctrl Pts',(-61.012063944535,-36.6291297604775,0.));
#78727=CARTESIAN_POINT('Ctrl Pts',(-61.012063944535,-36.6291297604775,12.));
#78728=CARTESIAN_POINT('Ctrl Pts',(-61.0267140464434,-36.6460216768553,
0.));
#78729=CARTESIAN_POINT('Ctrl Pts',(-61.0267140464434,-36.6460216768553,
12.));
#78730=CARTESIAN_POINT('Ctrl Pts',(-61.0413773427204,-36.6629633998885,
0.));
#78731=CARTESIAN_POINT('Ctrl Pts',(-61.0413773427204,-36.6629633998885,
12.));
#78732=CARTESIAN_POINT('Ctrl Pts',(-61.0560536877084,-36.6799548686741,
0.));
#78733=CARTESIAN_POINT('Ctrl Pts',(-61.0560536877084,-36.6799548686741,
12.));
#78734=CARTESIAN_POINT('Ctrl Pts',(-61.0707429364841,-36.6969960225019,
0.));
#78735=CARTESIAN_POINT('Ctrl Pts',(-61.0707429364841,-36.6969960225019,
12.));
#78736=CARTESIAN_POINT('Ctrl Pts',(-61.085444944851,-36.7140868008479,0.));
#78737=CARTESIAN_POINT('Ctrl Pts',(-61.085444944851,-36.7140868008479,12.));
#78738=CARTESIAN_POINT('Ctrl Pts',(-61.1001595693357,-36.7312271433799,
0.));
#78739=CARTESIAN_POINT('Ctrl Pts',(-61.1001595693357,-36.7312271433799,
12.));
#78740=CARTESIAN_POINT('Ctrl Pts',(-61.1148866671821,-36.7484169899591,
0.));
#78741=CARTESIAN_POINT('Ctrl Pts',(-61.1148866671821,-36.7484169899591,
12.));
#78742=CARTESIAN_POINT('Ctrl Pts',(-61.1296260963468,-36.7656562806381,
0.));
#78743=CARTESIAN_POINT('Ctrl Pts',(-61.1296260963468,-36.7656562806381,
12.));
#78744=CARTESIAN_POINT('Ctrl Pts',(-61.1443777154926,-36.782944955654,0.));
#78745=CARTESIAN_POINT('Ctrl Pts',(-61.1443777154926,-36.782944955654,12.));
#78746=CARTESIAN_POINT('Ctrl Pts',(-61.1591413839809,-36.8002829554221,
0.));
#78747=CARTESIAN_POINT('Ctrl Pts',(-61.1591413839809,-36.8002829554221,
12.));
#78748=CARTESIAN_POINT('Ctrl Pts',(-61.1739169618688,-36.8176702205436,
0.));
#78749=CARTESIAN_POINT('Ctrl Pts',(-61.1739169618688,-36.8176702205436,
12.));
#78750=CARTESIAN_POINT('Ctrl Pts',(-61.1887043099026,-36.8351066918043,
0.));
#78751=CARTESIAN_POINT('Ctrl Pts',(-61.1887043099026,-36.8351066918043,
12.));
#78752=CARTESIAN_POINT('Ctrl Pts',(-61.2035032895121,-36.8525923101736,
0.));
#78753=CARTESIAN_POINT('Ctrl Pts',(-61.2035032895121,-36.8525923101736,
12.));
#78754=CARTESIAN_POINT('Ctrl Pts',(-61.2183137628031,-36.8701270167954,
0.));
#78755=CARTESIAN_POINT('Ctrl Pts',(-61.2183137628031,-36.8701270167954,
12.));
#78756=CARTESIAN_POINT('Ctrl Pts',(-61.2331355925513,-36.8877107529844,
0.));
#78757=CARTESIAN_POINT('Ctrl Pts',(-61.2331355925513,-36.8877107529844,
12.));
#78758=CARTESIAN_POINT('Ctrl Pts',(-61.2479686421979,-36.9053434602324,
0.));
#78759=CARTESIAN_POINT('Ctrl Pts',(-61.2479686421979,-36.9053434602324,
12.));
#78760=CARTESIAN_POINT('Ctrl Pts',(-61.2628127758443,-36.9230250802078,
0.));
#78761=CARTESIAN_POINT('Ctrl Pts',(-61.2628127758443,-36.9230250802078,
12.));
#78762=CARTESIAN_POINT('Ctrl Pts',(-61.2776678582474,-36.9407555547542,
0.));
#78763=CARTESIAN_POINT('Ctrl Pts',(-61.2776678582474,-36.9407555547542,
12.));
#78764=CARTESIAN_POINT('Ctrl Pts',(-61.2925337548113,-36.9585348258798,
0.));
#78765=CARTESIAN_POINT('Ctrl Pts',(-61.2925337548113,-36.9585348258798,
12.));
#78766=CARTESIAN_POINT('Ctrl Pts',(-61.3074103315834,-36.976362835757,0.));
#78767=CARTESIAN_POINT('Ctrl Pts',(-61.3074103315834,-36.976362835757,12.));
#78768=CARTESIAN_POINT('Ctrl Pts',(-61.3222974552519,-36.994239526729,0.));
#78769=CARTESIAN_POINT('Ctrl Pts',(-61.3222974552519,-36.994239526729,12.));
#78770=CARTESIAN_POINT('Ctrl Pts',(-61.3371949931397,-37.0121648413088,
0.));
#78771=CARTESIAN_POINT('Ctrl Pts',(-61.3371949931397,-37.0121648413088,
12.));
#78772=CARTESIAN_POINT('Ctrl Pts',(-61.352102813199,-37.0301387221766,0.));
#78773=CARTESIAN_POINT('Ctrl Pts',(-61.352102813199,-37.0301387221766,12.));
#78774=CARTESIAN_POINT('Ctrl Pts',(-61.3670207840041,-37.0481611121698,
0.));
#78775=CARTESIAN_POINT('Ctrl Pts',(-61.3670207840041,-37.0481611121698,
12.));
#78776=CARTESIAN_POINT('Ctrl Pts',(-61.3819487747458,-37.0662319542827,
0.));
#78777=CARTESIAN_POINT('Ctrl Pts',(-61.3819487747458,-37.0662319542827,
12.));
#78778=CARTESIAN_POINT('Ctrl Pts',(-61.3968866552294,-37.0843511916728,
0.));
#78779=CARTESIAN_POINT('Ctrl Pts',(-61.3968866552294,-37.0843511916728,
12.));
#78780=CARTESIAN_POINT('Ctrl Pts',(-61.411834295869,-37.1025187676597,0.));
#78781=CARTESIAN_POINT('Ctrl Pts',(-61.411834295869,-37.1025187676597,12.));
#78782=CARTESIAN_POINT('Ctrl Pts',(-61.4267915676834,-37.1207346257228,
0.));
#78783=CARTESIAN_POINT('Ctrl Pts',(-61.4267915676834,-37.1207346257228,
12.));
#78784=CARTESIAN_POINT('Ctrl Pts',(-61.4417583422888,-37.138998709492,0.));
#78785=CARTESIAN_POINT('Ctrl Pts',(-61.4417583422888,-37.138998709492,12.));
#78786=CARTESIAN_POINT('Ctrl Pts',(-61.4567344918946,-37.157310962747,0.));
#78787=CARTESIAN_POINT('Ctrl Pts',(-61.4567344918946,-37.157310962747,12.));
#78788=CARTESIAN_POINT('Ctrl Pts',(-61.471719889301,-37.1756713294249,0.));
#78789=CARTESIAN_POINT('Ctrl Pts',(-61.471719889301,-37.1756713294249,12.));
#78790=CARTESIAN_POINT('Ctrl Pts',(-61.4867144078939,-37.1940797536182,
0.));
#78791=CARTESIAN_POINT('Ctrl Pts',(-61.4867144078939,-37.1940797536182,
12.));
#78792=CARTESIAN_POINT('Ctrl Pts',(-61.5017179216404,-37.2125361795727,
0.));
#78793=CARTESIAN_POINT('Ctrl Pts',(-61.5017179216404,-37.2125361795727,
12.));
#78794=CARTESIAN_POINT('Ctrl Pts',(-61.5167303050823,-37.2310405516775,
0.));
#78795=CARTESIAN_POINT('Ctrl Pts',(-61.5167303050823,-37.2310405516775,
12.));
#78796=CARTESIAN_POINT('Ctrl Pts',(-61.5317514333319,-37.2495928144661,
0.));
#78797=CARTESIAN_POINT('Ctrl Pts',(-61.5317514333319,-37.2495928144661,
12.));
#78798=CARTESIAN_POINT('Ctrl Pts',(-61.5467811820686,-37.2681929126217,
0.));
#78799=CARTESIAN_POINT('Ctrl Pts',(-61.5467811820686,-37.2681929126217,
12.));
#78800=CARTESIAN_POINT('Ctrl Pts',(-61.5618194275349,-37.286840790977,0.));
#78801=CARTESIAN_POINT('Ctrl Pts',(-61.5618194275349,-37.286840790977,12.));
#78802=CARTESIAN_POINT('Ctrl Pts',(-61.5768660465313,-37.3055363945108,
0.));
#78803=CARTESIAN_POINT('Ctrl Pts',(-61.5768660465313,-37.3055363945108,
12.));
#78804=CARTESIAN_POINT('Ctrl Pts',(-61.591920916412,-37.3242796683395,0.));
#78805=CARTESIAN_POINT('Ctrl Pts',(-61.591920916412,-37.3242796683395,12.));
#78806=CARTESIAN_POINT('Ctrl Pts',(-61.6069839150804,-37.3430705577178,
0.));
#78807=CARTESIAN_POINT('Ctrl Pts',(-61.6069839150804,-37.3430705577178,
12.));
#78808=CARTESIAN_POINT('Ctrl Pts',(-61.6220549209862,-37.3619090080447,
0.));
#78809=CARTESIAN_POINT('Ctrl Pts',(-61.6220549209862,-37.3619090080447,
12.));
#78810=CARTESIAN_POINT('Ctrl Pts',(-61.6371338131208,-37.3807949648622,
0.));
#78811=CARTESIAN_POINT('Ctrl Pts',(-61.6371338131208,-37.3807949648622,
12.));
#78812=CARTESIAN_POINT('Ctrl Pts',(-61.6522204710133,-37.3997283738534,
0.));
#78813=CARTESIAN_POINT('Ctrl Pts',(-61.6522204710133,-37.3997283738534,
12.));
#78814=CARTESIAN_POINT('Ctrl Pts',(-61.667314774725,-37.4187091808324,0.));
#78815=CARTESIAN_POINT('Ctrl Pts',(-61.667314774725,-37.4187091808324,12.));
#78816=CARTESIAN_POINT('Ctrl Pts',(-61.6824166048454,-37.4377373317456,
0.));
#78817=CARTESIAN_POINT('Ctrl Pts',(-61.6824166048454,-37.4377373317456,
12.));
#78818=CARTESIAN_POINT('Ctrl Pts',(-61.69752584249,-37.4568127726776,0.));
#78819=CARTESIAN_POINT('Ctrl Pts',(-61.69752584249,-37.4568127726776,12.));
#78820=CARTESIAN_POINT('Ctrl Pts',(-61.7126423692965,-37.4759354498509,
0.));
#78821=CARTESIAN_POINT('Ctrl Pts',(-61.7126423692965,-37.4759354498509,
12.));
#78822=CARTESIAN_POINT('Ctrl Pts',(-61.7277660674203,-37.4951053096235,
0.));
#78823=CARTESIAN_POINT('Ctrl Pts',(-61.7277660674203,-37.4951053096235,
12.));
#78824=CARTESIAN_POINT('Ctrl Pts',(-61.7428968195296,-37.5143222984794,
0.));
#78825=CARTESIAN_POINT('Ctrl Pts',(-61.7428968195296,-37.5143222984794,
12.));
#78826=CARTESIAN_POINT('Ctrl Pts',(-61.7580345088014,-37.5335863630286,
0.));
#78827=CARTESIAN_POINT('Ctrl Pts',(-61.7580345088014,-37.5335863630286,
12.));
#78828=CARTESIAN_POINT('Ctrl Pts',(-61.7731790189191,-37.5528974500142,
0.));
#78829=CARTESIAN_POINT('Ctrl Pts',(-61.7731790189191,-37.5528974500142,
12.));
#78830=CARTESIAN_POINT('Ctrl Pts',(-61.7883302340689,-37.5722555063112,
0.));
#78831=CARTESIAN_POINT('Ctrl Pts',(-61.7883302340689,-37.5722555063112,
12.));
#78832=CARTESIAN_POINT('Ctrl Pts',(-61.8034880389362,-37.5916604789252,
0.));
#78833=CARTESIAN_POINT('Ctrl Pts',(-61.8034880389362,-37.5916604789252,
12.));
#78834=CARTESIAN_POINT('Ctrl Pts',(-61.8186523187011,-37.6111123149835,
0.));
#78835=CARTESIAN_POINT('Ctrl Pts',(-61.8186523187011,-37.6111123149835,
12.));
#78836=CARTESIAN_POINT('Ctrl Pts',(-61.8338229590345,-37.6306109617341,
0.));
#78837=CARTESIAN_POINT('Ctrl Pts',(-61.8338229590345,-37.6306109617341,
12.));
#78838=CARTESIAN_POINT('Ctrl Pts',(-61.848999846095,-37.6501563665518,0.));
#78839=CARTESIAN_POINT('Ctrl Pts',(-61.848999846095,-37.6501563665518,12.));
#78840=CARTESIAN_POINT('Ctrl Pts',(-61.8641828665257,-37.6697484769389,
0.));
#78841=CARTESIAN_POINT('Ctrl Pts',(-61.8641828665257,-37.6697484769389,
12.));
#78842=CARTESIAN_POINT('Ctrl Pts',(-61.879371907451,-37.6893872405229,0.));
#78843=CARTESIAN_POINT('Ctrl Pts',(-61.879371907451,-37.6893872405229,12.));
#78844=CARTESIAN_POINT('Ctrl Pts',(-61.8945668564714,-37.7090726050488,
0.));
#78845=CARTESIAN_POINT('Ctrl Pts',(-61.8945668564714,-37.7090726050488,
12.));
#78846=CARTESIAN_POINT('Ctrl Pts',(-61.9097676016616,-37.7288045183765,
0.));
#78847=CARTESIAN_POINT('Ctrl Pts',(-61.9097676016616,-37.7288045183765,
12.));
#78848=CARTESIAN_POINT('Ctrl Pts',(-61.9249740315664,-37.748582928488,0.));
#78849=CARTESIAN_POINT('Ctrl Pts',(-61.9249740315664,-37.748582928488,12.));
#78850=CARTESIAN_POINT('Ctrl Pts',(-61.940186035198,-37.7684077834877,0.));
#78851=CARTESIAN_POINT('Ctrl Pts',(-61.940186035198,-37.7684077834877,12.));
#78852=CARTESIAN_POINT('Ctrl Pts',(-61.9554035020335,-37.7882790316012,
0.));
#78853=CARTESIAN_POINT('Ctrl Pts',(-61.9554035020335,-37.7882790316012,
12.));
#78854=CARTESIAN_POINT('Ctrl Pts',(-61.9706263220101,-37.808196621168,0.));
#78855=CARTESIAN_POINT('Ctrl Pts',(-61.9706263220101,-37.808196621168,12.));
#78856=CARTESIAN_POINT('Ctrl Pts',(-61.9858543855221,-37.8281605006371,
0.));
#78857=CARTESIAN_POINT('Ctrl Pts',(-61.9858543855221,-37.8281605006371,
12.));
#78858=CARTESIAN_POINT('Ctrl Pts',(-62.0010875834176,-37.8481706185742,
0.));
#78859=CARTESIAN_POINT('Ctrl Pts',(-62.0010875834176,-37.8481706185742,
12.));
#78860=CARTESIAN_POINT('Ctrl Pts',(-62.0163258069954,-37.8682269236628,
0.));
#78861=CARTESIAN_POINT('Ctrl Pts',(-62.0163258069954,-37.8682269236628,
12.));
#78862=CARTESIAN_POINT('Ctrl Pts',(-62.0315689480022,-37.888329364703,0.));
#78863=CARTESIAN_POINT('Ctrl Pts',(-62.0315689480022,-37.888329364703,12.));
#78864=CARTESIAN_POINT('Ctrl Pts',(-62.0468168986289,-37.9084778906053,
0.));
#78865=CARTESIAN_POINT('Ctrl Pts',(-62.0468168986289,-37.9084778906053,
12.));
#78866=CARTESIAN_POINT('Ctrl Pts',(-62.0620695515072,-37.9286724503849,
0.));
#78867=CARTESIAN_POINT('Ctrl Pts',(-62.0620695515072,-37.9286724503849,
12.));
#78868=CARTESIAN_POINT('Ctrl Pts',(-62.0773267997072,-37.9489129931685,
0.));
#78869=CARTESIAN_POINT('Ctrl Pts',(-62.0773267997072,-37.9489129931685,
12.));
#78870=CARTESIAN_POINT('Ctrl Pts',(-62.0925885367346,-37.9691994681962,
0.));
#78871=CARTESIAN_POINT('Ctrl Pts',(-62.0925885367346,-37.9691994681962,
12.));
#78872=CARTESIAN_POINT('Ctrl Pts',(-62.107854656528,-37.9895318248212,0.));
#78873=CARTESIAN_POINT('Ctrl Pts',(-62.107854656528,-37.9895318248212,12.));
#78874=CARTESIAN_POINT('Ctrl Pts',(-62.1231250534558,-38.0099100125041,
0.));
#78875=CARTESIAN_POINT('Ctrl Pts',(-62.1231250534558,-38.0099100125041,
12.));
#78876=CARTESIAN_POINT('Ctrl Pts',(-62.1383996223136,-38.0303339808059,
0.));
#78877=CARTESIAN_POINT('Ctrl Pts',(-62.1383996223136,-38.0303339808059,
12.));
#78878=CARTESIAN_POINT('Ctrl Pts',(-62.153678258321,-38.0508036793944,0.));
#78879=CARTESIAN_POINT('Ctrl Pts',(-62.153678258321,-38.0508036793944,12.));
#78880=CARTESIAN_POINT('Ctrl Pts',(-62.1689608571182,-38.0713190580466,
0.));
#78881=CARTESIAN_POINT('Ctrl Pts',(-62.1689608571182,-38.0713190580466,
12.));
#78882=CARTESIAN_POINT('Ctrl Pts',(-62.1842473147627,-38.0918800666479,
0.));
#78883=CARTESIAN_POINT('Ctrl Pts',(-62.1842473147627,-38.0918800666479,
12.));
#78884=CARTESIAN_POINT('Ctrl Pts',(-62.1995375277253,-38.1124866551883,
0.));
#78885=CARTESIAN_POINT('Ctrl Pts',(-62.1995375277253,-38.1124866551883,
12.));
#78886=CARTESIAN_POINT('Ctrl Pts',(-62.2148313928859,-38.1331387737528,
0.));
#78887=CARTESIAN_POINT('Ctrl Pts',(-62.2148313928859,-38.1331387737528,
12.));
#78888=CARTESIAN_POINT('Ctrl Pts',(-62.2301288075319,-38.1538363725263,
0.));
#78889=CARTESIAN_POINT('Ctrl Pts',(-62.2301288075319,-38.1538363725263,
12.));
#78890=CARTESIAN_POINT('Ctrl Pts',(-62.2454296693581,-38.1745794017997,
0.));
#78891=CARTESIAN_POINT('Ctrl Pts',(-62.2454296693581,-38.1745794017997,
12.));
#78892=CARTESIAN_POINT('Ctrl Pts',(-62.2607338764655,-38.1953678119692,
0.));
#78893=CARTESIAN_POINT('Ctrl Pts',(-62.2607338764655,-38.1953678119692,
12.));
#78894=CARTESIAN_POINT('Ctrl Pts',(-62.2760413273601,-38.2162015535351,
0.));
#78895=CARTESIAN_POINT('Ctrl Pts',(-62.2760413273601,-38.2162015535351,
12.));
#78896=CARTESIAN_POINT('Ctrl Pts',(-62.2913519209517,-38.2370805770931,
0.));
#78897=CARTESIAN_POINT('Ctrl Pts',(-62.2913519209517,-38.2370805770931,
12.));
#78898=CARTESIAN_POINT('Ctrl Pts',(-62.3066655565497,-38.2580048333356,
0.));
#78899=CARTESIAN_POINT('Ctrl Pts',(-62.3066655565497,-38.2580048333356,
12.));
#78900=CARTESIAN_POINT('Ctrl Pts',(-62.3219821338564,-38.2789742730559,
0.));
#78901=CARTESIAN_POINT('Ctrl Pts',(-62.3219821338564,-38.2789742730559,
12.));
#78902=CARTESIAN_POINT('Ctrl Pts',(-62.337301552961,-38.2999888471474,0.));
#78903=CARTESIAN_POINT('Ctrl Pts',(-62.337301552961,-38.2999888471474,12.));
#78904=CARTESIAN_POINT('Ctrl Pts',(-62.3526237143338,-38.3210485066002,
0.));
#78905=CARTESIAN_POINT('Ctrl Pts',(-62.3526237143338,-38.3210485066002,
12.));
#78906=CARTESIAN_POINT('Ctrl Pts',(-62.3679485188178,-38.3421532024915,
0.));
#78907=CARTESIAN_POINT('Ctrl Pts',(-62.3679485188178,-38.3421532024915,
12.));
#78908=CARTESIAN_POINT('Ctrl Pts',(-62.3832758676281,-38.3633028859835,
0.));
#78909=CARTESIAN_POINT('Ctrl Pts',(-62.3832758676281,-38.3633028859835,
12.));
#78910=CARTESIAN_POINT('Ctrl Pts',(-62.3986056623587,-38.384497508335,0.));
#78911=CARTESIAN_POINT('Ctrl Pts',(-62.3986056623587,-38.384497508335,12.));
#78912=CARTESIAN_POINT('Ctrl Pts',(-62.4139378049891,-38.4057370209054,
0.));
#78913=CARTESIAN_POINT('Ctrl Pts',(-62.4139378049891,-38.4057370209054,
12.));
#78914=CARTESIAN_POINT('Ctrl Pts',(-62.42927219789,-38.4270213751567,0.));
#78915=CARTESIAN_POINT('Ctrl Pts',(-62.42927219789,-38.4270213751567,12.));
#78916=CARTESIAN_POINT('Ctrl Pts',(-62.4446087438304,-38.4483505226511,
0.));
#78917=CARTESIAN_POINT('Ctrl Pts',(-62.4446087438304,-38.4483505226511,
12.));
#78918=CARTESIAN_POINT('Ctrl Pts',(-62.4599473459799,-38.4697244150473,
0.));
#78919=CARTESIAN_POINT('Ctrl Pts',(-62.4599473459799,-38.4697244150473,
12.));
#78920=CARTESIAN_POINT('Ctrl Pts',(-62.4752879078842,-38.4911430040988,
0.));
#78921=CARTESIAN_POINT('Ctrl Pts',(-62.4752879078842,-38.4911430040988,
12.));
#78922=CARTESIAN_POINT('Ctrl Pts',(-62.4906303334435,-38.5126062416495,
0.));
#78923=CARTESIAN_POINT('Ctrl Pts',(-62.4906303334435,-38.5126062416495,
12.));
#78924=CARTESIAN_POINT('Ctrl Pts',(-62.50597452689,-38.5341140796247,0.));
#78925=CARTESIAN_POINT('Ctrl Pts',(-62.50597452689,-38.5341140796247,12.));
#78926=CARTESIAN_POINT('Ctrl Pts',(-62.5213203927672,-38.5556664700201,
0.));
#78927=CARTESIAN_POINT('Ctrl Pts',(-62.5213203927672,-38.5556664700201,
12.));
#78928=CARTESIAN_POINT('Ctrl Pts',(-62.5366678359036,-38.5772633648841,
0.));
#78929=CARTESIAN_POINT('Ctrl Pts',(-62.5366678359036,-38.5772633648841,
12.));
#78930=CARTESIAN_POINT('Ctrl Pts',(-62.5520167614529,-38.5989047163401,
0.));
#78931=CARTESIAN_POINT('Ctrl Pts',(-62.5520167614529,-38.5989047163401,
12.));
#78932=CARTESIAN_POINT('Ctrl Pts',(-62.567367074937,-38.6205904766078,0.));
#78933=CARTESIAN_POINT('Ctrl Pts',(-62.567367074937,-38.6205904766078,12.));
#78934=CARTESIAN_POINT('Ctrl Pts',(-62.5827186822923,-38.6423205980214,
0.));
#78935=CARTESIAN_POINT('Ctrl Pts',(-62.5827186822923,-38.6423205980214,
12.));
#78936=CARTESIAN_POINT('Ctrl Pts',(-62.5980714899048,-38.6640950330418,
0.));
#78937=CARTESIAN_POINT('Ctrl Pts',(-62.5980714899048,-38.6640950330418,
12.));
#78938=CARTESIAN_POINT('Ctrl Pts',(-62.6134254046732,-38.6859137342726,
0.));
#78939=CARTESIAN_POINT('Ctrl Pts',(-62.6134254046732,-38.6859137342726,
12.));
#78940=CARTESIAN_POINT('Ctrl Pts',(-62.6287803339534,-38.7077766544411,
0.));
#78941=CARTESIAN_POINT('Ctrl Pts',(-62.6287803339534,-38.7077766544411,
12.));
#78942=CARTESIAN_POINT('Ctrl Pts',(-62.6441361854406,-38.7296837463605,
0.));
#78943=CARTESIAN_POINT('Ctrl Pts',(-62.6441361854406,-38.7296837463605,
12.));
#78944=CARTESIAN_POINT('Ctrl Pts',(-62.6594928670626,-38.7516349628902,
0.));
#78945=CARTESIAN_POINT('Ctrl Pts',(-62.6594928670626,-38.7516349628902,
12.));
#78946=CARTESIAN_POINT('Ctrl Pts',(-62.6748502868836,-38.7736302568982,
0.));
#78947=CARTESIAN_POINT('Ctrl Pts',(-62.6748502868836,-38.7736302568982,
12.));
#78948=CARTESIAN_POINT('Ctrl Pts',(-62.6902083529698,-38.7956695812032,
0.));
#78949=CARTESIAN_POINT('Ctrl Pts',(-62.6902083529698,-38.7956695812032,
12.));
#78950=CARTESIAN_POINT('Ctrl Pts',(-62.7055669733811,-38.8177528885686,
0.));
#78951=CARTESIAN_POINT('Ctrl Pts',(-62.7055669733811,-38.8177528885686,
12.));
#78952=CARTESIAN_POINT('Ctrl Pts',(-62.7209260564506,-38.8398801318184,
0.));
#78953=CARTESIAN_POINT('Ctrl Pts',(-62.7209260564506,-38.8398801318184,
12.));
#78954=CARTESIAN_POINT('Ctrl Pts',(-62.7362855110052,-38.8620512639239,
0.));
#78955=CARTESIAN_POINT('Ctrl Pts',(-62.7362855110052,-38.8620512639239,
12.));
#78956=CARTESIAN_POINT('Ctrl Pts',(-62.7516452466129,-38.8842662380984,
0.));
#78957=CARTESIAN_POINT('Ctrl Pts',(-62.7516452466129,-38.8842662380984,
12.));
#78958=CARTESIAN_POINT('Ctrl Pts',(-62.7670051738132,-38.9065250078824,
0.));
#78959=CARTESIAN_POINT('Ctrl Pts',(-62.7670051738132,-38.9065250078824,
12.));
#78960=CARTESIAN_POINT('Ctrl Pts',(-62.7823652043677,-38.9288275272319,
0.));
#78961=CARTESIAN_POINT('Ctrl Pts',(-62.7823652043677,-38.9288275272319,
12.));
#78962=CARTESIAN_POINT('Ctrl Pts',(-62.797725250709,-38.9511737503146,0.));
#78963=CARTESIAN_POINT('Ctrl Pts',(-62.797725250709,-38.9511737503146,12.));
#78964=CARTESIAN_POINT('Ctrl Pts',(-62.8130852254004,-38.9735636313073,
0.));
#78965=CARTESIAN_POINT('Ctrl Pts',(-62.8130852254004,-38.9735636313073,
12.));
#78966=CARTESIAN_POINT('Ctrl Pts',(-62.8284450405451,-38.9959971241695,
0.));
#78967=CARTESIAN_POINT('Ctrl Pts',(-62.8284450405451,-38.9959971241695,
12.));
#78968=CARTESIAN_POINT('Ctrl Pts',(-62.8438046073237,-39.0184741824649,
0.));
#78969=CARTESIAN_POINT('Ctrl Pts',(-62.8438046073237,-39.0184741824649,
12.));
#78970=CARTESIAN_POINT('Ctrl Pts',(-62.859163835209,-39.0409947590519,0.));
#78971=CARTESIAN_POINT('Ctrl Pts',(-62.859163835209,-39.0409947590519,12.));
#78972=CARTESIAN_POINT('Ctrl Pts',(-62.8745226326046,-39.0635588063308,
0.));
#78973=CARTESIAN_POINT('Ctrl Pts',(-62.8745226326046,-39.0635588063308,
12.));
#78974=CARTESIAN_POINT('Ctrl Pts',(-62.8898809082659,-39.0861662767964,
0.));
#78975=CARTESIAN_POINT('Ctrl Pts',(-62.8898809082659,-39.0861662767964,
12.));
#78976=CARTESIAN_POINT('Ctrl Pts',(-62.9052385725416,-39.1088171235144,
0.));
#78977=CARTESIAN_POINT('Ctrl Pts',(-62.9052385725416,-39.1088171235144,
12.));
#78978=CARTESIAN_POINT('Ctrl Pts',(-62.9205955385551,-39.1315113005745,
0.));
#78979=CARTESIAN_POINT('Ctrl Pts',(-62.9205955385551,-39.1315113005745,
12.));
#78980=CARTESIAN_POINT('Ctrl Pts',(-62.9359517237352,-39.1542487636708,
0.));
#78981=CARTESIAN_POINT('Ctrl Pts',(-62.9359517237352,-39.1542487636708,
12.));
#78982=CARTESIAN_POINT('Ctrl Pts',(-62.9513070501777,-39.1770294702367,
0.));
#78983=CARTESIAN_POINT('Ctrl Pts',(-62.9513070501777,-39.1770294702367,
12.));
#78984=CARTESIAN_POINT('Ctrl Pts',(-62.9666614412628,-39.199853378159,0.));
#78985=CARTESIAN_POINT('Ctrl Pts',(-62.9666614412628,-39.199853378159,12.));
#78986=CARTESIAN_POINT('Ctrl Pts',(-62.9820148189849,-39.2227204447583,
0.));
#78987=CARTESIAN_POINT('Ctrl Pts',(-62.9820148189849,-39.2227204447583,
12.));
#78988=CARTESIAN_POINT('Ctrl Pts',(-62.9973671008685,-39.2456306256092,
0.));
#78989=CARTESIAN_POINT('Ctrl Pts',(-62.9973671008685,-39.2456306256092,
12.));
#78990=CARTESIAN_POINT('Ctrl Pts',(-63.0127181973703,-39.268583873541,0.));
#78991=CARTESIAN_POINT('Ctrl Pts',(-63.0127181973703,-39.268583873541,12.));
#78992=CARTESIAN_POINT('Ctrl Pts',(-63.0280680082522,-39.2915801372467,
0.));
#78993=CARTESIAN_POINT('Ctrl Pts',(-63.0280680082522,-39.2915801372467,
12.));
#78994=CARTESIAN_POINT('Ctrl Pts',(-63.0434164278221,-39.3146193632546,
0.));
#78995=CARTESIAN_POINT('Ctrl Pts',(-63.0434164278221,-39.3146193632546,
12.));
#78996=CARTESIAN_POINT('Ctrl Pts',(-63.0587633513993,-39.3377014983756,
0.));
#78997=CARTESIAN_POINT('Ctrl Pts',(-63.0587633513993,-39.3377014983756,
12.));
#78998=CARTESIAN_POINT('Ctrl Pts',(-63.0741086815958,-39.3608264920487,
0.));
#78999=CARTESIAN_POINT('Ctrl Pts',(-63.0741086815958,-39.3608264920487,
12.));
#79000=CARTESIAN_POINT('Ctrl Pts',(-63.0894523341238,-39.3839942985688,
0.));
#79001=CARTESIAN_POINT('Ctrl Pts',(-63.0894523341238,-39.3839942985688,
12.));
#79002=CARTESIAN_POINT('Ctrl Pts',(-63.1047942451583,-39.4072048797401,
0.));
#79003=CARTESIAN_POINT('Ctrl Pts',(-63.1047942451583,-39.4072048797401,
12.));
#79004=CARTESIAN_POINT('Ctrl Pts',(-63.1201343730643,-39.4304582059507,
0.));
#79005=CARTESIAN_POINT('Ctrl Pts',(-63.1201343730643,-39.4304582059507,
12.));
#79006=CARTESIAN_POINT('Ctrl Pts',(-63.1354726927781,-39.4537542551852,
0.));
#79007=CARTESIAN_POINT('Ctrl Pts',(-63.1354726927781,-39.4537542551852,
12.));
#79008=CARTESIAN_POINT('Ctrl Pts',(-63.147741892189,-39.4724252610807,0.));
#79009=CARTESIAN_POINT('Ctrl Pts',(-63.147741892189,-39.4724252610807,12.));
#79010=CARTESIAN_POINT('Ctrl Pts',(-63.1569429707564,-39.4864477303613,
0.));
#79011=CARTESIAN_POINT('Ctrl Pts',(-63.1569429707564,-39.4864477303613,
12.));
#79012=CARTESIAN_POINT('Ctrl Pts',(-63.1630766582674,-39.4958045828059,
0.));
#79013=CARTESIAN_POINT('Ctrl Pts',(-63.1630766582674,-39.4958045828059,
12.));
#79014=CARTESIAN_POINT('Ctrl Pts',(-63.1661434108059,-39.5004851439257,
0.));
#79015=CARTESIAN_POINT('Ctrl Pts',(-63.1661434108059,-39.5004851439257,
12.));
#79016=CARTESIAN_POINT('',(-60.1903555511633,-35.7368311217509,0.));
#79017=CARTESIAN_POINT('Ctrl Pts',(-60.1903555511633,-35.7368311217509,
0.));
#79018=CARTESIAN_POINT('Ctrl Pts',(-60.1930746580239,-35.7396040203973,
0.));
#79019=CARTESIAN_POINT('Ctrl Pts',(-60.1985151474406,-35.7451551752456,
0.));
#79020=CARTESIAN_POINT('Ctrl Pts',(-60.2066827086579,-35.7534979801871,
0.));
#79021=CARTESIAN_POINT('Ctrl Pts',(-60.2175864449678,-35.7646538667299,
0.));
#79022=CARTESIAN_POINT('Ctrl Pts',(-60.2312388621286,-35.7786523045782,
0.));
#79023=CARTESIAN_POINT('Ctrl Pts',(-60.2449139865206,-35.7927043145164,
0.));
#79024=CARTESIAN_POINT('Ctrl Pts',(-60.2586117365278,-35.8068098723386,
0.));
#79025=CARTESIAN_POINT('Ctrl Pts',(-60.2723319687507,-35.8209689272574,
0.));
#79026=CARTESIAN_POINT('Ctrl Pts',(-60.2860744798563,-35.8351814020424,
0.));
#79027=CARTESIAN_POINT('Ctrl Pts',(-60.2998390330173,-35.8494472046783,
0.));
#79028=CARTESIAN_POINT('Ctrl Pts',(-60.313625378281,-35.8637662371635,0.));
#79029=CARTESIAN_POINT('Ctrl Pts',(-60.3274332746782,-35.878138405151,0.));
#79030=CARTESIAN_POINT('Ctrl Pts',(-60.3412625135223,-35.8925636280632,
0.));
#79031=CARTESIAN_POINT('Ctrl Pts',(-60.3551129108794,-35.9070418358501,
0.));
#79032=CARTESIAN_POINT('Ctrl Pts',(-60.368984296546,-35.9215729642219,0.));
#79033=CARTESIAN_POINT('Ctrl Pts',(-60.3828765049031,-35.9361569506955,
0.));
#79034=CARTESIAN_POINT('Ctrl Pts',(-60.3967893635487,-35.9507937296726,
0.));
#79035=CARTESIAN_POINT('Ctrl Pts',(-60.4107226875759,-35.9654832299627,
0.));
#79036=CARTESIAN_POINT('Ctrl Pts',(-60.4246762854961,-35.9802253773534,
0.));
#79037=CARTESIAN_POINT('Ctrl Pts',(-60.438649962949,-35.9950200962175,0.));
#79038=CARTESIAN_POINT('Ctrl Pts',(-60.452643526964,-36.0098673113556,0.));
#79039=CARTESIAN_POINT('Ctrl Pts',(-60.4666567908053,-36.0247669500867,
0.));
#79040=CARTESIAN_POINT('Ctrl Pts',(-60.4806895737643,-36.0397189421617,
0.));
#79041=CARTESIAN_POINT('Ctrl Pts',(-60.4947416988396,-36.0547232187681,
0.));
#79042=CARTESIAN_POINT('Ctrl Pts',(-60.5088129911357,-36.0697797118377,
0.));
#79043=CARTESIAN_POINT('Ctrl Pts',(-60.5229032759001,-36.0848883531968,
0.));
#79044=CARTESIAN_POINT('Ctrl Pts',(-60.5370123768841,-36.1000490738532,
0.));
#79045=CARTESIAN_POINT('Ctrl Pts',(-60.5511401172014,-36.1152618043756,
0.));
#79046=CARTESIAN_POINT('Ctrl Pts',(-60.5652863200732,-36.1305264752195,
0.));
#79047=CARTESIAN_POINT('Ctrl Pts',(-60.5794508095555,-36.1458430170425,
0.));
#79048=CARTESIAN_POINT('Ctrl Pts',(-60.5936334114083,-36.1612113610758,
0.));
#79049=CARTESIAN_POINT('Ctrl Pts',(-60.6078339534151,-36.1766314392624,
0.));
#79050=CARTESIAN_POINT('Ctrl Pts',(-60.6220522649129,-36.1921031840617,
0.));
#79051=CARTESIAN_POINT('Ctrl Pts',(-60.6362881765014,-36.2076265283261,
0.));
#79052=CARTESIAN_POINT('Ctrl Pts',(-60.6505415197055,-36.2232014051549,
0.));
#79053=CARTESIAN_POINT('Ctrl Pts',(-60.6648121265908,-36.2388277477225,
0.));
#79054=CARTESIAN_POINT('Ctrl Pts',(-60.6790998297823,-36.2545054892911,
0.));
#79055=CARTESIAN_POINT('Ctrl Pts',(-60.6934044626304,-36.2702345632882,
0.));
#79056=CARTESIAN_POINT('Ctrl Pts',(-60.7077258593268,-36.2860149033586,
0.));
#79057=CARTESIAN_POINT('Ctrl Pts',(-60.7220638550396,-36.3018464434204,
0.));
#79058=CARTESIAN_POINT('Ctrl Pts',(-60.7364182860388,-36.3177291177148,
0.));
#79059=CARTESIAN_POINT('Ctrl Pts',(-60.7507889896284,-36.3336628607844,
0.));
#79060=CARTESIAN_POINT('Ctrl Pts',(-60.7651758040792,-36.349647607448,0.));
#79061=CARTESIAN_POINT('Ctrl Pts',(-60.7795785685631,-36.3656832927733,
0.));
#79062=CARTESIAN_POINT('Ctrl Pts',(-60.7939971230781,-36.38176985204,0.));
#79063=CARTESIAN_POINT('Ctrl Pts',(-60.8084313084009,-36.3979072207174,
0.));
#79064=CARTESIAN_POINT('Ctrl Pts',(-60.8228809661179,-36.4140953344869,
0.));
#79065=CARTESIAN_POINT('Ctrl Pts',(-60.8373459386397,-36.4303341292497,
0.));
#79066=CARTESIAN_POINT('Ctrl Pts',(-60.851826069218,-36.4466235411353,0.));
#79067=CARTESIAN_POINT('Ctrl Pts',(-60.8663212019646,-36.4629635065037,
0.));
#79068=CARTESIAN_POINT('Ctrl Pts',(-60.8808311818489,-36.4793539619459,
0.));
#79069=CARTESIAN_POINT('Ctrl Pts',(-60.8953558546791,-36.4957948442832,
0.));
#79070=CARTESIAN_POINT('Ctrl Pts',(-60.9098950670847,-36.5122860905611,
0.));
#79071=CARTESIAN_POINT('Ctrl Pts',(-60.924448666499,-36.5288276380417,0.));
#79072=CARTESIAN_POINT('Ctrl Pts',(-60.9390165011357,-36.5454194241866,
0.));
#79073=CARTESIAN_POINT('Ctrl Pts',(-60.9535984199874,-36.5620613866615,
0.));
#79074=CARTESIAN_POINT('Ctrl Pts',(-60.9681942728237,-36.5787534633416,
0.));
#79075=CARTESIAN_POINT('Ctrl Pts',(-60.9828039101887,-36.5954955923109,
0.));
#79076=CARTESIAN_POINT('Ctrl Pts',(-60.9974271833982,-36.6122877118599,
0.));
#79077=CARTESIAN_POINT('Ctrl Pts',(-61.012063944535,-36.6291297604775,0.));
#79078=CARTESIAN_POINT('Ctrl Pts',(-61.0267140464434,-36.6460216768553,
0.));
#79079=CARTESIAN_POINT('Ctrl Pts',(-61.0413773427204,-36.6629633998885,
0.));
#79080=CARTESIAN_POINT('Ctrl Pts',(-61.0560536877084,-36.6799548686741,
0.));
#79081=CARTESIAN_POINT('Ctrl Pts',(-61.0707429364841,-36.6969960225019,
0.));
#79082=CARTESIAN_POINT('Ctrl Pts',(-61.085444944851,-36.7140868008479,0.));
#79083=CARTESIAN_POINT('Ctrl Pts',(-61.1001595693357,-36.7312271433799,
0.));
#79084=CARTESIAN_POINT('Ctrl Pts',(-61.1148866671821,-36.7484169899591,
0.));
#79085=CARTESIAN_POINT('Ctrl Pts',(-61.1296260963468,-36.7656562806381,
0.));
#79086=CARTESIAN_POINT('Ctrl Pts',(-61.1443777154926,-36.782944955654,0.));
#79087=CARTESIAN_POINT('Ctrl Pts',(-61.1591413839809,-36.8002829554221,
0.));
#79088=CARTESIAN_POINT('Ctrl Pts',(-61.1739169618688,-36.8176702205436,
0.));
#79089=CARTESIAN_POINT('Ctrl Pts',(-61.1887043099026,-36.8351066918043,
0.));
#79090=CARTESIAN_POINT('Ctrl Pts',(-61.2035032895121,-36.8525923101736,
0.));
#79091=CARTESIAN_POINT('Ctrl Pts',(-61.2183137628031,-36.8701270167954,
0.));
#79092=CARTESIAN_POINT('Ctrl Pts',(-61.2331355925513,-36.8877107529844,
0.));
#79093=CARTESIAN_POINT('Ctrl Pts',(-61.2479686421979,-36.9053434602324,
0.));
#79094=CARTESIAN_POINT('Ctrl Pts',(-61.2628127758443,-36.9230250802078,
0.));
#79095=CARTESIAN_POINT('Ctrl Pts',(-61.2776678582474,-36.9407555547542,
0.));
#79096=CARTESIAN_POINT('Ctrl Pts',(-61.2925337548113,-36.9585348258798,
0.));
#79097=CARTESIAN_POINT('Ctrl Pts',(-61.3074103315834,-36.976362835757,0.));
#79098=CARTESIAN_POINT('Ctrl Pts',(-61.3222974552519,-36.994239526729,0.));
#79099=CARTESIAN_POINT('Ctrl Pts',(-61.3371949931397,-37.0121648413088,
0.));
#79100=CARTESIAN_POINT('Ctrl Pts',(-61.352102813199,-37.0301387221766,0.));
#79101=CARTESIAN_POINT('Ctrl Pts',(-61.3670207840041,-37.0481611121698,
0.));
#79102=CARTESIAN_POINT('Ctrl Pts',(-61.3819487747458,-37.0662319542827,
0.));
#79103=CARTESIAN_POINT('Ctrl Pts',(-61.3968866552294,-37.0843511916728,
0.));
#79104=CARTESIAN_POINT('Ctrl Pts',(-61.411834295869,-37.1025187676597,0.));
#79105=CARTESIAN_POINT('Ctrl Pts',(-61.4267915676834,-37.1207346257228,
0.));
#79106=CARTESIAN_POINT('Ctrl Pts',(-61.4417583422888,-37.138998709492,0.));
#79107=CARTESIAN_POINT('Ctrl Pts',(-61.4567344918946,-37.157310962747,0.));
#79108=CARTESIAN_POINT('Ctrl Pts',(-61.471719889301,-37.1756713294249,0.));
#79109=CARTESIAN_POINT('Ctrl Pts',(-61.4867144078939,-37.1940797536182,
0.));
#79110=CARTESIAN_POINT('Ctrl Pts',(-61.5017179216404,-37.2125361795727,
0.));
#79111=CARTESIAN_POINT('Ctrl Pts',(-61.5167303050823,-37.2310405516775,
0.));
#79112=CARTESIAN_POINT('Ctrl Pts',(-61.5317514333319,-37.2495928144661,
0.));
#79113=CARTESIAN_POINT('Ctrl Pts',(-61.5467811820686,-37.2681929126217,
0.));
#79114=CARTESIAN_POINT('Ctrl Pts',(-61.5618194275349,-37.286840790977,0.));
#79115=CARTESIAN_POINT('Ctrl Pts',(-61.5768660465313,-37.3055363945108,
0.));
#79116=CARTESIAN_POINT('Ctrl Pts',(-61.591920916412,-37.3242796683395,0.));
#79117=CARTESIAN_POINT('Ctrl Pts',(-61.6069839150804,-37.3430705577178,
0.));
#79118=CARTESIAN_POINT('Ctrl Pts',(-61.6220549209862,-37.3619090080447,
0.));
#79119=CARTESIAN_POINT('Ctrl Pts',(-61.6371338131208,-37.3807949648622,
0.));
#79120=CARTESIAN_POINT('Ctrl Pts',(-61.6522204710133,-37.3997283738534,
0.));
#79121=CARTESIAN_POINT('Ctrl Pts',(-61.667314774725,-37.4187091808324,0.));
#79122=CARTESIAN_POINT('Ctrl Pts',(-61.6824166048454,-37.4377373317456,
0.));
#79123=CARTESIAN_POINT('Ctrl Pts',(-61.69752584249,-37.4568127726776,0.));
#79124=CARTESIAN_POINT('Ctrl Pts',(-61.7126423692965,-37.4759354498509,
0.));
#79125=CARTESIAN_POINT('Ctrl Pts',(-61.7277660674203,-37.4951053096235,
0.));
#79126=CARTESIAN_POINT('Ctrl Pts',(-61.7428968195296,-37.5143222984794,
0.));
#79127=CARTESIAN_POINT('Ctrl Pts',(-61.7580345088014,-37.5335863630286,
0.));
#79128=CARTESIAN_POINT('Ctrl Pts',(-61.7731790189191,-37.5528974500142,
0.));
#79129=CARTESIAN_POINT('Ctrl Pts',(-61.7883302340689,-37.5722555063112,
0.));
#79130=CARTESIAN_POINT('Ctrl Pts',(-61.8034880389362,-37.5916604789252,
0.));
#79131=CARTESIAN_POINT('Ctrl Pts',(-61.8186523187011,-37.6111123149835,
0.));
#79132=CARTESIAN_POINT('Ctrl Pts',(-61.8338229590345,-37.6306109617341,
0.));
#79133=CARTESIAN_POINT('Ctrl Pts',(-61.848999846095,-37.6501563665518,0.));
#79134=CARTESIAN_POINT('Ctrl Pts',(-61.8641828665257,-37.6697484769389,
0.));
#79135=CARTESIAN_POINT('Ctrl Pts',(-61.879371907451,-37.6893872405229,0.));
#79136=CARTESIAN_POINT('Ctrl Pts',(-61.8945668564714,-37.7090726050488,
0.));
#79137=CARTESIAN_POINT('Ctrl Pts',(-61.9097676016616,-37.7288045183765,
0.));
#79138=CARTESIAN_POINT('Ctrl Pts',(-61.9249740315664,-37.748582928488,0.));
#79139=CARTESIAN_POINT('Ctrl Pts',(-61.940186035198,-37.7684077834877,0.));
#79140=CARTESIAN_POINT('Ctrl Pts',(-61.9554035020335,-37.7882790316012,
0.));
#79141=CARTESIAN_POINT('Ctrl Pts',(-61.9706263220101,-37.808196621168,0.));
#79142=CARTESIAN_POINT('Ctrl Pts',(-61.9858543855221,-37.8281605006371,
0.));
#79143=CARTESIAN_POINT('Ctrl Pts',(-62.0010875834176,-37.8481706185742,
0.));
#79144=CARTESIAN_POINT('Ctrl Pts',(-62.0163258069954,-37.8682269236628,
0.));
#79145=CARTESIAN_POINT('Ctrl Pts',(-62.0315689480022,-37.888329364703,0.));
#79146=CARTESIAN_POINT('Ctrl Pts',(-62.0468168986289,-37.9084778906053,
0.));
#79147=CARTESIAN_POINT('Ctrl Pts',(-62.0620695515072,-37.9286724503849,
0.));
#79148=CARTESIAN_POINT('Ctrl Pts',(-62.0773267997072,-37.9489129931685,
0.));
#79149=CARTESIAN_POINT('Ctrl Pts',(-62.0925885367346,-37.9691994681962,
0.));
#79150=CARTESIAN_POINT('Ctrl Pts',(-62.107854656528,-37.9895318248212,0.));
#79151=CARTESIAN_POINT('Ctrl Pts',(-62.1231250534558,-38.0099100125041,
0.));
#79152=CARTESIAN_POINT('Ctrl Pts',(-62.1383996223136,-38.0303339808059,
0.));
#79153=CARTESIAN_POINT('Ctrl Pts',(-62.153678258321,-38.0508036793944,0.));
#79154=CARTESIAN_POINT('Ctrl Pts',(-62.1689608571182,-38.0713190580466,
0.));
#79155=CARTESIAN_POINT('Ctrl Pts',(-62.1842473147627,-38.0918800666479,
0.));
#79156=CARTESIAN_POINT('Ctrl Pts',(-62.1995375277253,-38.1124866551883,
0.));
#79157=CARTESIAN_POINT('Ctrl Pts',(-62.2148313928859,-38.1331387737528,
0.));
#79158=CARTESIAN_POINT('Ctrl Pts',(-62.2301288075319,-38.1538363725263,
0.));
#79159=CARTESIAN_POINT('Ctrl Pts',(-62.2454296693581,-38.1745794017997,
0.));
#79160=CARTESIAN_POINT('Ctrl Pts',(-62.2607338764655,-38.1953678119692,
0.));
#79161=CARTESIAN_POINT('Ctrl Pts',(-62.2760413273601,-38.2162015535351,
0.));
#79162=CARTESIAN_POINT('Ctrl Pts',(-62.2913519209517,-38.2370805770931,
0.));
#79163=CARTESIAN_POINT('Ctrl Pts',(-62.3066655565497,-38.2580048333356,
0.));
#79164=CARTESIAN_POINT('Ctrl Pts',(-62.3219821338564,-38.2789742730559,
0.));
#79165=CARTESIAN_POINT('Ctrl Pts',(-62.337301552961,-38.2999888471474,0.));
#79166=CARTESIAN_POINT('Ctrl Pts',(-62.3526237143338,-38.3210485066002,
0.));
#79167=CARTESIAN_POINT('Ctrl Pts',(-62.3679485188178,-38.3421532024915,
0.));
#79168=CARTESIAN_POINT('Ctrl Pts',(-62.3832758676281,-38.3633028859835,
0.));
#79169=CARTESIAN_POINT('Ctrl Pts',(-62.3986056623587,-38.384497508335,0.));
#79170=CARTESIAN_POINT('Ctrl Pts',(-62.4139378049891,-38.4057370209054,
0.));
#79171=CARTESIAN_POINT('Ctrl Pts',(-62.42927219789,-38.4270213751567,0.));
#79172=CARTESIAN_POINT('Ctrl Pts',(-62.4446087438304,-38.4483505226511,
0.));
#79173=CARTESIAN_POINT('Ctrl Pts',(-62.4599473459799,-38.4697244150473,
0.));
#79174=CARTESIAN_POINT('Ctrl Pts',(-62.4752879078842,-38.4911430040988,
0.));
#79175=CARTESIAN_POINT('Ctrl Pts',(-62.4906303334435,-38.5126062416495,
0.));
#79176=CARTESIAN_POINT('Ctrl Pts',(-62.50597452689,-38.5341140796247,0.));
#79177=CARTESIAN_POINT('Ctrl Pts',(-62.5213203927672,-38.5556664700201,
0.));
#79178=CARTESIAN_POINT('Ctrl Pts',(-62.5366678359036,-38.5772633648841,
0.));
#79179=CARTESIAN_POINT('Ctrl Pts',(-62.5520167614529,-38.5989047163401,
0.));
#79180=CARTESIAN_POINT('Ctrl Pts',(-62.567367074937,-38.6205904766078,0.));
#79181=CARTESIAN_POINT('Ctrl Pts',(-62.5827186822923,-38.6423205980214,
0.));
#79182=CARTESIAN_POINT('Ctrl Pts',(-62.5980714899048,-38.6640950330418,
0.));
#79183=CARTESIAN_POINT('Ctrl Pts',(-62.6134254046732,-38.6859137342726,
0.));
#79184=CARTESIAN_POINT('Ctrl Pts',(-62.6287803339534,-38.7077766544411,
0.));
#79185=CARTESIAN_POINT('Ctrl Pts',(-62.6441361854406,-38.7296837463605,
0.));
#79186=CARTESIAN_POINT('Ctrl Pts',(-62.6594928670626,-38.7516349628902,
0.));
#79187=CARTESIAN_POINT('Ctrl Pts',(-62.6748502868836,-38.7736302568982,
0.));
#79188=CARTESIAN_POINT('Ctrl Pts',(-62.6902083529698,-38.7956695812032,
0.));
#79189=CARTESIAN_POINT('Ctrl Pts',(-62.7055669733811,-38.8177528885686,
0.));
#79190=CARTESIAN_POINT('Ctrl Pts',(-62.7209260564506,-38.8398801318184,
0.));
#79191=CARTESIAN_POINT('Ctrl Pts',(-62.7362855110052,-38.8620512639239,
0.));
#79192=CARTESIAN_POINT('Ctrl Pts',(-62.7516452466129,-38.8842662380984,
0.));
#79193=CARTESIAN_POINT('Ctrl Pts',(-62.7670051738132,-38.9065250078824,
0.));
#79194=CARTESIAN_POINT('Ctrl Pts',(-62.7823652043677,-38.9288275272319,
0.));
#79195=CARTESIAN_POINT('Ctrl Pts',(-62.797725250709,-38.9511737503146,0.));
#79196=CARTESIAN_POINT('Ctrl Pts',(-62.8130852254004,-38.9735636313073,
0.));
#79197=CARTESIAN_POINT('Ctrl Pts',(-62.8284450405451,-38.9959971241695,
0.));
#79198=CARTESIAN_POINT('Ctrl Pts',(-62.8438046073237,-39.0184741824649,
0.));
#79199=CARTESIAN_POINT('Ctrl Pts',(-62.859163835209,-39.0409947590519,0.));
#79200=CARTESIAN_POINT('Ctrl Pts',(-62.8745226326046,-39.0635588063308,
0.));
#79201=CARTESIAN_POINT('Ctrl Pts',(-62.8898809082659,-39.0861662767964,
0.));
#79202=CARTESIAN_POINT('Ctrl Pts',(-62.9052385725416,-39.1088171235144,
0.));
#79203=CARTESIAN_POINT('Ctrl Pts',(-62.9205955385551,-39.1315113005745,
0.));
#79204=CARTESIAN_POINT('Ctrl Pts',(-62.9359517237352,-39.1542487636708,
0.));
#79205=CARTESIAN_POINT('Ctrl Pts',(-62.9513070501777,-39.1770294702367,
0.));
#79206=CARTESIAN_POINT('Ctrl Pts',(-62.9644687386693,-39.1965939820802,
0.));
#79207=CARTESIAN_POINT('Ctrl Pts',(-62.9745590018499,-39.2116170128275,
0.));
#79208=CARTESIAN_POINT('Ctrl Pts',(-62.9815782721128,-39.2220794388571,
0.));
#79209=CARTESIAN_POINT('Ctrl Pts',(-62.9855268615901,-39.2279686274717,
0.));
#79210=CARTESIAN_POINT('Ctrl Pts',(-62.9864049293628,-39.2292784191463,
0.));
#79211=CARTESIAN_POINT('',(-60.1903555511633,-35.7368311217509,12.));
#79212=CARTESIAN_POINT('',(-60.1903555511633,-35.7368311217509,0.));
#79213=CARTESIAN_POINT('Ctrl Pts',(-62.9864049293629,-39.2292784191464,
12.));
#79214=CARTESIAN_POINT('Ctrl Pts',(-62.9855268615902,-39.2279686274718,
12.));
#79215=CARTESIAN_POINT('Ctrl Pts',(-62.9815782721128,-39.2220794388572,
12.));
#79216=CARTESIAN_POINT('Ctrl Pts',(-62.9745590018499,-39.2116170128276,
12.));
#79217=CARTESIAN_POINT('Ctrl Pts',(-62.9644687386693,-39.1965939820803,
12.));
#79218=CARTESIAN_POINT('Ctrl Pts',(-62.9513070501777,-39.1770294702367,
12.));
#79219=CARTESIAN_POINT('Ctrl Pts',(-62.9359517237352,-39.1542487636708,
12.));
#79220=CARTESIAN_POINT('Ctrl Pts',(-62.9205955385551,-39.1315113005745,
12.));
#79221=CARTESIAN_POINT('Ctrl Pts',(-62.9052385725416,-39.1088171235144,
12.));
#79222=CARTESIAN_POINT('Ctrl Pts',(-62.8898809082659,-39.0861662767964,
12.));
#79223=CARTESIAN_POINT('Ctrl Pts',(-62.8745226326046,-39.0635588063308,
12.));
#79224=CARTESIAN_POINT('Ctrl Pts',(-62.859163835209,-39.0409947590519,12.));
#79225=CARTESIAN_POINT('Ctrl Pts',(-62.8438046073237,-39.0184741824649,
12.));
#79226=CARTESIAN_POINT('Ctrl Pts',(-62.8284450405451,-38.9959971241695,
12.));
#79227=CARTESIAN_POINT('Ctrl Pts',(-62.8130852254004,-38.9735636313073,
12.));
#79228=CARTESIAN_POINT('Ctrl Pts',(-62.797725250709,-38.9511737503146,12.));
#79229=CARTESIAN_POINT('Ctrl Pts',(-62.7823652043677,-38.9288275272319,
12.));
#79230=CARTESIAN_POINT('Ctrl Pts',(-62.7670051738132,-38.9065250078824,
12.));
#79231=CARTESIAN_POINT('Ctrl Pts',(-62.7516452466129,-38.8842662380984,
12.));
#79232=CARTESIAN_POINT('Ctrl Pts',(-62.7362855110052,-38.8620512639239,
12.));
#79233=CARTESIAN_POINT('Ctrl Pts',(-62.7209260564506,-38.8398801318184,
12.));
#79234=CARTESIAN_POINT('Ctrl Pts',(-62.7055669733811,-38.8177528885686,
12.));
#79235=CARTESIAN_POINT('Ctrl Pts',(-62.6902083529698,-38.7956695812032,
12.));
#79236=CARTESIAN_POINT('Ctrl Pts',(-62.6748502868836,-38.7736302568982,
12.));
#79237=CARTESIAN_POINT('Ctrl Pts',(-62.6594928670626,-38.7516349628902,
12.));
#79238=CARTESIAN_POINT('Ctrl Pts',(-62.6441361854406,-38.7296837463605,
12.));
#79239=CARTESIAN_POINT('Ctrl Pts',(-62.6287803339534,-38.7077766544411,
12.));
#79240=CARTESIAN_POINT('Ctrl Pts',(-62.6134254046732,-38.6859137342726,
12.));
#79241=CARTESIAN_POINT('Ctrl Pts',(-62.5980714899048,-38.6640950330418,
12.));
#79242=CARTESIAN_POINT('Ctrl Pts',(-62.5827186822923,-38.6423205980214,
12.));
#79243=CARTESIAN_POINT('Ctrl Pts',(-62.567367074937,-38.6205904766078,12.));
#79244=CARTESIAN_POINT('Ctrl Pts',(-62.5520167614529,-38.5989047163401,
12.));
#79245=CARTESIAN_POINT('Ctrl Pts',(-62.5366678359036,-38.5772633648841,
12.));
#79246=CARTESIAN_POINT('Ctrl Pts',(-62.5213203927672,-38.5556664700201,
12.));
#79247=CARTESIAN_POINT('Ctrl Pts',(-62.50597452689,-38.5341140796247,12.));
#79248=CARTESIAN_POINT('Ctrl Pts',(-62.4906303334435,-38.5126062416495,
12.));
#79249=CARTESIAN_POINT('Ctrl Pts',(-62.4752879078842,-38.4911430040988,
12.));
#79250=CARTESIAN_POINT('Ctrl Pts',(-62.4599473459799,-38.4697244150473,
12.));
#79251=CARTESIAN_POINT('Ctrl Pts',(-62.4446087438304,-38.4483505226511,
12.));
#79252=CARTESIAN_POINT('Ctrl Pts',(-62.42927219789,-38.4270213751567,12.));
#79253=CARTESIAN_POINT('Ctrl Pts',(-62.4139378049891,-38.4057370209054,
12.));
#79254=CARTESIAN_POINT('Ctrl Pts',(-62.3986056623587,-38.384497508335,12.));
#79255=CARTESIAN_POINT('Ctrl Pts',(-62.3832758676281,-38.3633028859835,
12.));
#79256=CARTESIAN_POINT('Ctrl Pts',(-62.3679485188178,-38.3421532024915,
12.));
#79257=CARTESIAN_POINT('Ctrl Pts',(-62.3526237143338,-38.3210485066002,
12.));
#79258=CARTESIAN_POINT('Ctrl Pts',(-62.337301552961,-38.2999888471474,12.));
#79259=CARTESIAN_POINT('Ctrl Pts',(-62.3219821338564,-38.2789742730559,
12.));
#79260=CARTESIAN_POINT('Ctrl Pts',(-62.3066655565497,-38.2580048333356,
12.));
#79261=CARTESIAN_POINT('Ctrl Pts',(-62.2913519209517,-38.2370805770931,
12.));
#79262=CARTESIAN_POINT('Ctrl Pts',(-62.2760413273601,-38.2162015535351,
12.));
#79263=CARTESIAN_POINT('Ctrl Pts',(-62.2607338764655,-38.1953678119692,
12.));
#79264=CARTESIAN_POINT('Ctrl Pts',(-62.2454296693581,-38.1745794017997,
12.));
#79265=CARTESIAN_POINT('Ctrl Pts',(-62.2301288075319,-38.1538363725263,
12.));
#79266=CARTESIAN_POINT('Ctrl Pts',(-62.2148313928859,-38.1331387737528,
12.));
#79267=CARTESIAN_POINT('Ctrl Pts',(-62.1995375277253,-38.1124866551883,
12.));
#79268=CARTESIAN_POINT('Ctrl Pts',(-62.1842473147627,-38.0918800666479,
12.));
#79269=CARTESIAN_POINT('Ctrl Pts',(-62.1689608571182,-38.0713190580466,
12.));
#79270=CARTESIAN_POINT('Ctrl Pts',(-62.153678258321,-38.0508036793944,12.));
#79271=CARTESIAN_POINT('Ctrl Pts',(-62.1383996223136,-38.0303339808059,
12.));
#79272=CARTESIAN_POINT('Ctrl Pts',(-62.1231250534558,-38.0099100125041,
12.));
#79273=CARTESIAN_POINT('Ctrl Pts',(-62.107854656528,-37.9895318248212,12.));
#79274=CARTESIAN_POINT('Ctrl Pts',(-62.0925885367346,-37.9691994681962,
12.));
#79275=CARTESIAN_POINT('Ctrl Pts',(-62.0773267997072,-37.9489129931685,
12.));
#79276=CARTESIAN_POINT('Ctrl Pts',(-62.0620695515072,-37.9286724503849,
12.));
#79277=CARTESIAN_POINT('Ctrl Pts',(-62.0468168986289,-37.9084778906053,
12.));
#79278=CARTESIAN_POINT('Ctrl Pts',(-62.0315689480022,-37.888329364703,12.));
#79279=CARTESIAN_POINT('Ctrl Pts',(-62.0163258069954,-37.8682269236628,
12.));
#79280=CARTESIAN_POINT('Ctrl Pts',(-62.0010875834176,-37.8481706185742,
12.));
#79281=CARTESIAN_POINT('Ctrl Pts',(-61.9858543855221,-37.8281605006371,
12.));
#79282=CARTESIAN_POINT('Ctrl Pts',(-61.9706263220101,-37.808196621168,12.));
#79283=CARTESIAN_POINT('Ctrl Pts',(-61.9554035020335,-37.7882790316012,
12.));
#79284=CARTESIAN_POINT('Ctrl Pts',(-61.940186035198,-37.7684077834877,12.));
#79285=CARTESIAN_POINT('Ctrl Pts',(-61.9249740315664,-37.748582928488,12.));
#79286=CARTESIAN_POINT('Ctrl Pts',(-61.9097676016616,-37.7288045183765,
12.));
#79287=CARTESIAN_POINT('Ctrl Pts',(-61.8945668564714,-37.7090726050488,
12.));
#79288=CARTESIAN_POINT('Ctrl Pts',(-61.879371907451,-37.6893872405229,12.));
#79289=CARTESIAN_POINT('Ctrl Pts',(-61.8641828665257,-37.6697484769389,
12.));
#79290=CARTESIAN_POINT('Ctrl Pts',(-61.848999846095,-37.6501563665518,12.));
#79291=CARTESIAN_POINT('Ctrl Pts',(-61.8338229590345,-37.6306109617341,
12.));
#79292=CARTESIAN_POINT('Ctrl Pts',(-61.8186523187011,-37.6111123149835,
12.));
#79293=CARTESIAN_POINT('Ctrl Pts',(-61.8034880389362,-37.5916604789252,
12.));
#79294=CARTESIAN_POINT('Ctrl Pts',(-61.7883302340689,-37.5722555063112,
12.));
#79295=CARTESIAN_POINT('Ctrl Pts',(-61.7731790189191,-37.5528974500142,
12.));
#79296=CARTESIAN_POINT('Ctrl Pts',(-61.7580345088014,-37.5335863630286,
12.));
#79297=CARTESIAN_POINT('Ctrl Pts',(-61.7428968195296,-37.5143222984794,
12.));
#79298=CARTESIAN_POINT('Ctrl Pts',(-61.7277660674203,-37.4951053096235,
12.));
#79299=CARTESIAN_POINT('Ctrl Pts',(-61.7126423692965,-37.4759354498509,
12.));
#79300=CARTESIAN_POINT('Ctrl Pts',(-61.69752584249,-37.4568127726776,12.));
#79301=CARTESIAN_POINT('Ctrl Pts',(-61.6824166048454,-37.4377373317456,
12.));
#79302=CARTESIAN_POINT('Ctrl Pts',(-61.667314774725,-37.4187091808324,12.));
#79303=CARTESIAN_POINT('Ctrl Pts',(-61.6522204710133,-37.3997283738534,
12.));
#79304=CARTESIAN_POINT('Ctrl Pts',(-61.6371338131208,-37.3807949648622,
12.));
#79305=CARTESIAN_POINT('Ctrl Pts',(-61.6220549209862,-37.3619090080447,
12.));
#79306=CARTESIAN_POINT('Ctrl Pts',(-61.6069839150804,-37.3430705577178,
12.));
#79307=CARTESIAN_POINT('Ctrl Pts',(-61.591920916412,-37.3242796683395,12.));
#79308=CARTESIAN_POINT('Ctrl Pts',(-61.5768660465313,-37.3055363945108,
12.));
#79309=CARTESIAN_POINT('Ctrl Pts',(-61.5618194275349,-37.286840790977,12.));
#79310=CARTESIAN_POINT('Ctrl Pts',(-61.5467811820686,-37.2681929126217,
12.));
#79311=CARTESIAN_POINT('Ctrl Pts',(-61.5317514333319,-37.2495928144661,
12.));
#79312=CARTESIAN_POINT('Ctrl Pts',(-61.5167303050823,-37.2310405516775,
12.));
#79313=CARTESIAN_POINT('Ctrl Pts',(-61.5017179216404,-37.2125361795727,
12.));
#79314=CARTESIAN_POINT('Ctrl Pts',(-61.4867144078939,-37.1940797536182,
12.));
#79315=CARTESIAN_POINT('Ctrl Pts',(-61.471719889301,-37.1756713294249,12.));
#79316=CARTESIAN_POINT('Ctrl Pts',(-61.4567344918946,-37.157310962747,12.));
#79317=CARTESIAN_POINT('Ctrl Pts',(-61.4417583422888,-37.138998709492,12.));
#79318=CARTESIAN_POINT('Ctrl Pts',(-61.4267915676834,-37.1207346257228,
12.));
#79319=CARTESIAN_POINT('Ctrl Pts',(-61.411834295869,-37.1025187676597,12.));
#79320=CARTESIAN_POINT('Ctrl Pts',(-61.3968866552294,-37.0843511916728,
12.));
#79321=CARTESIAN_POINT('Ctrl Pts',(-61.3819487747458,-37.0662319542827,
12.));
#79322=CARTESIAN_POINT('Ctrl Pts',(-61.3670207840041,-37.0481611121698,
12.));
#79323=CARTESIAN_POINT('Ctrl Pts',(-61.352102813199,-37.0301387221766,12.));
#79324=CARTESIAN_POINT('Ctrl Pts',(-61.3371949931397,-37.0121648413088,
12.));
#79325=CARTESIAN_POINT('Ctrl Pts',(-61.3222974552519,-36.994239526729,12.));
#79326=CARTESIAN_POINT('Ctrl Pts',(-61.3074103315834,-36.976362835757,12.));
#79327=CARTESIAN_POINT('Ctrl Pts',(-61.2925337548113,-36.9585348258798,
12.));
#79328=CARTESIAN_POINT('Ctrl Pts',(-61.2776678582474,-36.9407555547542,
12.));
#79329=CARTESIAN_POINT('Ctrl Pts',(-61.2628127758443,-36.9230250802078,
12.));
#79330=CARTESIAN_POINT('Ctrl Pts',(-61.2479686421979,-36.9053434602324,
12.));
#79331=CARTESIAN_POINT('Ctrl Pts',(-61.2331355925513,-36.8877107529844,
12.));
#79332=CARTESIAN_POINT('Ctrl Pts',(-61.2183137628031,-36.8701270167954,
12.));
#79333=CARTESIAN_POINT('Ctrl Pts',(-61.2035032895121,-36.8525923101736,
12.));
#79334=CARTESIAN_POINT('Ctrl Pts',(-61.1887043099026,-36.8351066918043,
12.));
#79335=CARTESIAN_POINT('Ctrl Pts',(-61.1739169618688,-36.8176702205436,
12.));
#79336=CARTESIAN_POINT('Ctrl Pts',(-61.1591413839809,-36.8002829554221,
12.));
#79337=CARTESIAN_POINT('Ctrl Pts',(-61.1443777154926,-36.782944955654,12.));
#79338=CARTESIAN_POINT('Ctrl Pts',(-61.1296260963468,-36.7656562806381,
12.));
#79339=CARTESIAN_POINT('Ctrl Pts',(-61.1148866671821,-36.7484169899591,
12.));
#79340=CARTESIAN_POINT('Ctrl Pts',(-61.1001595693357,-36.7312271433799,
12.));
#79341=CARTESIAN_POINT('Ctrl Pts',(-61.085444944851,-36.7140868008479,12.));
#79342=CARTESIAN_POINT('Ctrl Pts',(-61.0707429364841,-36.6969960225019,
12.));
#79343=CARTESIAN_POINT('Ctrl Pts',(-61.0560536877084,-36.6799548686741,
12.));
#79344=CARTESIAN_POINT('Ctrl Pts',(-61.0413773427204,-36.6629633998885,
12.));
#79345=CARTESIAN_POINT('Ctrl Pts',(-61.0267140464434,-36.6460216768553,
12.));
#79346=CARTESIAN_POINT('Ctrl Pts',(-61.012063944535,-36.6291297604775,12.));
#79347=CARTESIAN_POINT('Ctrl Pts',(-60.9974271833982,-36.6122877118599,
12.));
#79348=CARTESIAN_POINT('Ctrl Pts',(-60.9828039101887,-36.5954955923109,
12.));
#79349=CARTESIAN_POINT('Ctrl Pts',(-60.9681942728237,-36.5787534633416,
12.));
#79350=CARTESIAN_POINT('Ctrl Pts',(-60.9535984199874,-36.5620613866615,
12.));
#79351=CARTESIAN_POINT('Ctrl Pts',(-60.9390165011357,-36.5454194241866,
12.));
#79352=CARTESIAN_POINT('Ctrl Pts',(-60.924448666499,-36.5288276380417,12.));
#79353=CARTESIAN_POINT('Ctrl Pts',(-60.9098950670847,-36.5122860905611,
12.));
#79354=CARTESIAN_POINT('Ctrl Pts',(-60.8953558546791,-36.4957948442832,
12.));
#79355=CARTESIAN_POINT('Ctrl Pts',(-60.8808311818489,-36.4793539619459,
12.));
#79356=CARTESIAN_POINT('Ctrl Pts',(-60.8663212019646,-36.4629635065037,
12.));
#79357=CARTESIAN_POINT('Ctrl Pts',(-60.851826069218,-36.4466235411353,12.));
#79358=CARTESIAN_POINT('Ctrl Pts',(-60.8373459386397,-36.4303341292497,
12.));
#79359=CARTESIAN_POINT('Ctrl Pts',(-60.8228809661179,-36.4140953344869,
12.));
#79360=CARTESIAN_POINT('Ctrl Pts',(-60.8084313084009,-36.3979072207174,
12.));
#79361=CARTESIAN_POINT('Ctrl Pts',(-60.7939971230781,-36.38176985204,12.));
#79362=CARTESIAN_POINT('Ctrl Pts',(-60.7795785685631,-36.3656832927733,
12.));
#79363=CARTESIAN_POINT('Ctrl Pts',(-60.7651758040792,-36.349647607448,12.));
#79364=CARTESIAN_POINT('Ctrl Pts',(-60.7507889896284,-36.3336628607844,
12.));
#79365=CARTESIAN_POINT('Ctrl Pts',(-60.7364182860388,-36.3177291177148,
12.));
#79366=CARTESIAN_POINT('Ctrl Pts',(-60.7220638550396,-36.3018464434204,
12.));
#79367=CARTESIAN_POINT('Ctrl Pts',(-60.7077258593268,-36.2860149033586,
12.));
#79368=CARTESIAN_POINT('Ctrl Pts',(-60.6934044626304,-36.2702345632882,
12.));
#79369=CARTESIAN_POINT('Ctrl Pts',(-60.6790998297823,-36.2545054892911,
12.));
#79370=CARTESIAN_POINT('Ctrl Pts',(-60.6648121265908,-36.2388277477225,
12.));
#79371=CARTESIAN_POINT('Ctrl Pts',(-60.6505415197055,-36.2232014051549,
12.));
#79372=CARTESIAN_POINT('Ctrl Pts',(-60.6362881765014,-36.2076265283261,
12.));
#79373=CARTESIAN_POINT('Ctrl Pts',(-60.6220522649129,-36.1921031840617,
12.));
#79374=CARTESIAN_POINT('Ctrl Pts',(-60.6078339534151,-36.1766314392624,
12.));
#79375=CARTESIAN_POINT('Ctrl Pts',(-60.5936334114083,-36.1612113610758,
12.));
#79376=CARTESIAN_POINT('Ctrl Pts',(-60.5794508095555,-36.1458430170425,
12.));
#79377=CARTESIAN_POINT('Ctrl Pts',(-60.5652863200732,-36.1305264752195,
12.));
#79378=CARTESIAN_POINT('Ctrl Pts',(-60.5511401172014,-36.1152618043756,
12.));
#79379=CARTESIAN_POINT('Ctrl Pts',(-60.5370123768841,-36.1000490738532,
12.));
#79380=CARTESIAN_POINT('Ctrl Pts',(-60.5229032759001,-36.0848883531968,
12.));
#79381=CARTESIAN_POINT('Ctrl Pts',(-60.5088129911357,-36.0697797118377,
12.));
#79382=CARTESIAN_POINT('Ctrl Pts',(-60.4947416988396,-36.0547232187681,
12.));
#79383=CARTESIAN_POINT('Ctrl Pts',(-60.4806895737643,-36.0397189421617,
12.));
#79384=CARTESIAN_POINT('Ctrl Pts',(-60.4666567908053,-36.0247669500867,
12.));
#79385=CARTESIAN_POINT('Ctrl Pts',(-60.452643526964,-36.0098673113556,12.));
#79386=CARTESIAN_POINT('Ctrl Pts',(-60.438649962949,-35.9950200962175,12.));
#79387=CARTESIAN_POINT('Ctrl Pts',(-60.4246762854961,-35.9802253773534,
12.));
#79388=CARTESIAN_POINT('Ctrl Pts',(-60.4107226875759,-35.9654832299627,
12.));
#79389=CARTESIAN_POINT('Ctrl Pts',(-60.3967893635487,-35.9507937296726,
12.));
#79390=CARTESIAN_POINT('Ctrl Pts',(-60.3828765049031,-35.9361569506955,
12.));
#79391=CARTESIAN_POINT('Ctrl Pts',(-60.368984296546,-35.9215729642219,12.));
#79392=CARTESIAN_POINT('Ctrl Pts',(-60.3551129108794,-35.9070418358501,
12.));
#79393=CARTESIAN_POINT('Ctrl Pts',(-60.3412625135223,-35.8925636280632,
12.));
#79394=CARTESIAN_POINT('Ctrl Pts',(-60.3274332746782,-35.878138405151,12.));
#79395=CARTESIAN_POINT('Ctrl Pts',(-60.313625378281,-35.8637662371635,12.));
#79396=CARTESIAN_POINT('Ctrl Pts',(-60.2998390330173,-35.8494472046783,
12.));
#79397=CARTESIAN_POINT('Ctrl Pts',(-60.2860744798563,-35.8351814020424,
12.));
#79398=CARTESIAN_POINT('Ctrl Pts',(-60.2723319687507,-35.8209689272574,
12.));
#79399=CARTESIAN_POINT('Ctrl Pts',(-60.2586117365278,-35.8068098723386,
12.));
#79400=CARTESIAN_POINT('Ctrl Pts',(-60.2449139865206,-35.7927043145164,
12.));
#79401=CARTESIAN_POINT('Ctrl Pts',(-60.2312388621286,-35.7786523045782,
12.));
#79402=CARTESIAN_POINT('Ctrl Pts',(-60.2175864449678,-35.7646538667299,
12.));
#79403=CARTESIAN_POINT('Ctrl Pts',(-60.2066827086579,-35.7534979801871,
12.));
#79404=CARTESIAN_POINT('Ctrl Pts',(-60.1985151474406,-35.7451551752456,
12.));
#79405=CARTESIAN_POINT('Ctrl Pts',(-60.1930746580239,-35.7396040203973,
12.));
#79406=CARTESIAN_POINT('Ctrl Pts',(-60.1903555511633,-35.7368311217509,
12.));
#79407=CARTESIAN_POINT('Ctrl Pts',(-62.1730054756879,-40.506059810093,0.));
#79408=CARTESIAN_POINT('Ctrl Pts',(-62.1730054756879,-40.506059810093,4.));
#79409=CARTESIAN_POINT('Ctrl Pts',(-62.1730054756879,-40.506059810093,8.));
#79410=CARTESIAN_POINT('Ctrl Pts',(-62.1730054756879,-40.506059810093,12.));
#79411=CARTESIAN_POINT('Ctrl Pts',(-62.2815834512361,-40.5229411493977,
0.));
#79412=CARTESIAN_POINT('Ctrl Pts',(-62.2815834512361,-40.5229411493977,
4.));
#79413=CARTESIAN_POINT('Ctrl Pts',(-62.2815834512362,-40.5229411493977,
8.));
#79414=CARTESIAN_POINT('Ctrl Pts',(-62.2815834512362,-40.5229411493977,
12.));
#79415=CARTESIAN_POINT('Ctrl Pts',(-62.4810961163748,-40.4873422218646,
0.));
#79416=CARTESIAN_POINT('Ctrl Pts',(-62.4810961163748,-40.4873422218646,
4.00000000000001));
#79417=CARTESIAN_POINT('Ctrl Pts',(-62.4810961163749,-40.4873422218646,
7.99999999999999));
#79418=CARTESIAN_POINT('Ctrl Pts',(-62.4810961163749,-40.4873422218646,
12.));
#79419=CARTESIAN_POINT('Ctrl Pts',(-62.6258675056117,-40.3516729626243,
0.));
#79420=CARTESIAN_POINT('Ctrl Pts',(-62.6258675056117,-40.3516729626243,
4.));
#79421=CARTESIAN_POINT('Ctrl Pts',(-62.6258675056118,-40.3516729626244,
8.00000000000001));
#79422=CARTESIAN_POINT('Ctrl Pts',(-62.6258675056118,-40.3516729626244,
12.));
#79423=CARTESIAN_POINT('Ctrl Pts',(-62.6704278106374,-40.2823469776989,
0.));
#79424=CARTESIAN_POINT('Ctrl Pts',(-62.6704278106374,-40.2823469776989,
4.));
#79425=CARTESIAN_POINT('Ctrl Pts',(-62.6704278106375,-40.282346977699,8.));
#79426=CARTESIAN_POINT('Ctrl Pts',(-62.6704278106375,-40.282346977699,12.));
#79427=CARTESIAN_POINT('',(-62.1730054756878,-40.506059810093,0.));
#79428=CARTESIAN_POINT('',(-62.6704278106372,-40.2823469776988,0.));
#79429=CARTESIAN_POINT('Ctrl Pts',(-62.1730054756879,-40.506059810093,2.77555756156289E-16));
#79430=CARTESIAN_POINT('Ctrl Pts',(-62.2815834512361,-40.5229411493977,
2.77555756156289E-16));
#79431=CARTESIAN_POINT('Ctrl Pts',(-62.3955906884582,-40.5025989050931,
2.77555756156289E-16));
#79432=CARTESIAN_POINT('Ctrl Pts',(-62.4917232233451,-40.4495806341085,
2.77555756156289E-16));
#79433=CARTESIAN_POINT('Ctrl Pts',(-62.5638226245102,-40.4098169308702,
2.77555756156289E-16));
#79434=CARTESIAN_POINT('Ctrl Pts',(-62.6258675056117,-40.3516729626243,
2.77555756156289E-16));
#79435=CARTESIAN_POINT('Ctrl Pts',(-62.6704278106374,-40.2823469776989,
2.77555756156289E-16));
#79436=CARTESIAN_POINT('',(-62.6704278106372,-40.2823469776988,12.));
#79437=CARTESIAN_POINT('Ctrl Pts',(-62.6704278106374,-40.2823469776989,
0.));
#79438=CARTESIAN_POINT('Ctrl Pts',(-62.6704278106374,-40.2823469776989,
4.));
#79439=CARTESIAN_POINT('Ctrl Pts',(-62.6704278106375,-40.282346977699,8.));
#79440=CARTESIAN_POINT('Ctrl Pts',(-62.6704278106375,-40.282346977699,12.));
#79441=CARTESIAN_POINT('',(-62.1730054756879,-40.506059810093,12.));
#79442=CARTESIAN_POINT('Ctrl Pts',(-62.6704278106375,-40.282346977699,12.));
#79443=CARTESIAN_POINT('Ctrl Pts',(-62.6258675056118,-40.3516729626244,
12.));
#79444=CARTESIAN_POINT('Ctrl Pts',(-62.5638226245103,-40.4098169308702,
12.));
#79445=CARTESIAN_POINT('Ctrl Pts',(-62.4917232233451,-40.4495806341086,
12.));
#79446=CARTESIAN_POINT('Ctrl Pts',(-62.3955906884583,-40.5025989050931,
12.));
#79447=CARTESIAN_POINT('Ctrl Pts',(-62.2815834512362,-40.5229411493977,
12.));
#79448=CARTESIAN_POINT('Ctrl Pts',(-62.1730054756879,-40.506059810093,12.));
#79449=CARTESIAN_POINT('Ctrl Pts',(-62.1730054756879,-40.506059810093,12.));
#79450=CARTESIAN_POINT('Ctrl Pts',(-62.1730054756879,-40.506059810093,8.));
#79451=CARTESIAN_POINT('Ctrl Pts',(-62.1730054756879,-40.506059810093,4.));
#79452=CARTESIAN_POINT('Ctrl Pts',(-62.1730054756879,-40.506059810093,0.));
#79453=CARTESIAN_POINT('Origin',(-3.16086693261782E-10,-2.01487121870483E-10,
0.));
#79454=CARTESIAN_POINT('Origin',(-3.16086693261782E-10,-2.01487121870483E-10,
12.));
#79455=CARTESIAN_POINT('Origin',(-3.16086693261782E-10,-2.01487121870483E-10,
0.));
#79456=CARTESIAN_POINT('Ctrl Pts',(-66.2207497120638,-34.1330090612036,
0.));
#79457=CARTESIAN_POINT('Ctrl Pts',(-66.2207497120638,-34.1330090612036,
4.));
#79458=CARTESIAN_POINT('Ctrl Pts',(-66.2207497120638,-34.1330090612036,
8.));
#79459=CARTESIAN_POINT('Ctrl Pts',(-66.2207497120638,-34.1330090612036,
12.));
#79460=CARTESIAN_POINT('Ctrl Pts',(-66.2710935941675,-34.0353379297089,
0.));
#79461=CARTESIAN_POINT('Ctrl Pts',(-66.2710935941675,-34.0353379297089,
4.));
#79462=CARTESIAN_POINT('Ctrl Pts',(-66.2710935941675,-34.0353379297089,
8.00000000000001));
#79463=CARTESIAN_POINT('Ctrl Pts',(-66.2710935941675,-34.0353379297089,
12.));
#79464=CARTESIAN_POINT('Ctrl Pts',(-66.3003999311009,-33.8348041971634,
0.));
#79465=CARTESIAN_POINT('Ctrl Pts',(-66.3003999311009,-33.8348041971634,
4.));
#79466=CARTESIAN_POINT('Ctrl Pts',(-66.3003999311009,-33.8348041971634,
7.99999999999999));
#79467=CARTESIAN_POINT('Ctrl Pts',(-66.3003999311009,-33.8348041971634,
12.));
#79468=CARTESIAN_POINT('Ctrl Pts',(-66.2174610329231,-33.6545652280942,
0.));
#79469=CARTESIAN_POINT('Ctrl Pts',(-66.2174610329231,-33.6545652280942,
4.));
#79470=CARTESIAN_POINT('Ctrl Pts',(-66.2174610329231,-33.6545652280942,
8.00000000000001));
#79471=CARTESIAN_POINT('Ctrl Pts',(-66.2174610329231,-33.6545652280942,
12.));
#79472=CARTESIAN_POINT('Ctrl Pts',(-66.165779540567,-33.5903722664959,0.));
#79473=CARTESIAN_POINT('Ctrl Pts',(-66.165779540567,-33.5903722664959,4.));
#79474=CARTESIAN_POINT('Ctrl Pts',(-66.165779540567,-33.5903722664959,8.));
#79475=CARTESIAN_POINT('Ctrl Pts',(-66.165779540567,-33.5903722664959,12.));
#79476=CARTESIAN_POINT('',(-66.2207497120638,-34.1330090612036,0.));
#79477=CARTESIAN_POINT('',(-66.165779540567,-33.5903722664959,0.));
#79478=CARTESIAN_POINT('Ctrl Pts',(-66.2207497120638,-34.1330090612036,
1.38777878078145E-16));
#79479=CARTESIAN_POINT('Ctrl Pts',(-66.2710935941675,-34.0353379297089,
1.38777878078145E-16));
#79480=CARTESIAN_POINT('Ctrl Pts',(-66.2878400724152,-33.9207472253972,
1.38777878078145E-16));
#79481=CARTESIAN_POINT('Ctrl Pts',(-66.2679350453204,-33.8127833826287,
1.38777878078145E-16));
#79482=CARTESIAN_POINT('Ctrl Pts',(-66.2530062749993,-33.7318105005524,
1.38777878078145E-16));
#79483=CARTESIAN_POINT('Ctrl Pts',(-66.2174610329231,-33.6545652280942,
1.38777878078144E-16));
#79484=CARTESIAN_POINT('Ctrl Pts',(-66.165779540567,-33.5903722664959,1.38777878078145E-16));
#79485=CARTESIAN_POINT('',(-66.1657795405671,-33.5903722664959,12.));
#79486=CARTESIAN_POINT('Ctrl Pts',(-66.165779540567,-33.5903722664959,0.));
#79487=CARTESIAN_POINT('Ctrl Pts',(-66.165779540567,-33.5903722664959,4.));
#79488=CARTESIAN_POINT('Ctrl Pts',(-66.165779540567,-33.5903722664959,8.));
#79489=CARTESIAN_POINT('Ctrl Pts',(-66.165779540567,-33.5903722664959,12.));
#79490=CARTESIAN_POINT('',(-66.2207497120638,-34.1330090612036,12.));
#79491=CARTESIAN_POINT('Ctrl Pts',(-66.165779540567,-33.5903722664959,12.));
#79492=CARTESIAN_POINT('Ctrl Pts',(-66.2174610329231,-33.6545652280942,
12.));
#79493=CARTESIAN_POINT('Ctrl Pts',(-66.2530062749993,-33.7318105005524,
12.));
#79494=CARTESIAN_POINT('Ctrl Pts',(-66.2679350453204,-33.8127833826288,
12.));
#79495=CARTESIAN_POINT('Ctrl Pts',(-66.2878400724152,-33.9207472253972,
12.));
#79496=CARTESIAN_POINT('Ctrl Pts',(-66.2710935941675,-34.0353379297089,
12.));
#79497=CARTESIAN_POINT('Ctrl Pts',(-66.2207497120638,-34.1330090612036,
12.));
#79498=CARTESIAN_POINT('Ctrl Pts',(-66.2207497120638,-34.1330090612036,
12.));
#79499=CARTESIAN_POINT('Ctrl Pts',(-66.2207497120638,-34.1330090612036,
8.));
#79500=CARTESIAN_POINT('Ctrl Pts',(-66.2207497120638,-34.1330090612036,
4.));
#79501=CARTESIAN_POINT('Ctrl Pts',(-66.2207497120638,-34.1330090612036,
0.));
#79502=CARTESIAN_POINT('Ctrl Pts',(-63.0759831361898,-30.3549065457811,
0.));
#79503=CARTESIAN_POINT('Ctrl Pts',(-63.0759831361898,-30.3549065457811,
12.));
#79504=CARTESIAN_POINT('Ctrl Pts',(-63.078933570069,-30.3574319069329,0.));
#79505=CARTESIAN_POINT('Ctrl Pts',(-63.078933570069,-30.3574319069329,12.));
#79506=CARTESIAN_POINT('Ctrl Pts',(-63.0848371718048,-30.3624877680651,
0.));
#79507=CARTESIAN_POINT('Ctrl Pts',(-63.0848371718048,-30.3624877680651,
12.));
#79508=CARTESIAN_POINT('Ctrl Pts',(-63.0937007763471,-30.3700869762507,
0.));
#79509=CARTESIAN_POINT('Ctrl Pts',(-63.0937007763471,-30.3700869762507,
12.));
#79510=CARTESIAN_POINT('Ctrl Pts',(-63.105535320226,-30.3802500880403,0.));
#79511=CARTESIAN_POINT('Ctrl Pts',(-63.105535320226,-30.3802500880403,12.));
#79512=CARTESIAN_POINT('Ctrl Pts',(-63.1203558300657,-30.3930053710484,
0.));
#79513=CARTESIAN_POINT('Ctrl Pts',(-63.1203558300657,-30.3930053710484,
12.));
#79514=CARTESIAN_POINT('Ctrl Pts',(-63.135203629844,-30.4058120432228,0.));
#79515=CARTESIAN_POINT('Ctrl Pts',(-63.135203629844,-30.4058120432228,12.));
#79516=CARTESIAN_POINT('Ctrl Pts',(-63.1500786361459,-30.418670087563,0.));
#79517=CARTESIAN_POINT('Ctrl Pts',(-63.1500786361459,-30.418670087563,12.));
#79518=CARTESIAN_POINT('Ctrl Pts',(-63.164980701691,-30.4315794659731,0.));
#79519=CARTESIAN_POINT('Ctrl Pts',(-63.164980701691,-30.4315794659731,12.));
#79520=CARTESIAN_POINT('Ctrl Pts',(-63.179909617189,-30.444540119238,0.));
#79521=CARTESIAN_POINT('Ctrl Pts',(-63.179909617189,-30.444540119238,12.));
#79522=CARTESIAN_POINT('Ctrl Pts',(-63.1948651386942,-30.4575519763337,
0.));
#79523=CARTESIAN_POINT('Ctrl Pts',(-63.1948651386942,-30.4575519763337,
12.));
#79524=CARTESIAN_POINT('Ctrl Pts',(-63.2098470086636,-30.470614961416,0.));
#79525=CARTESIAN_POINT('Ctrl Pts',(-63.2098470086636,-30.470614961416,12.));
#79526=CARTESIAN_POINT('Ctrl Pts',(-63.2248549788221,-30.4837290014989,
0.));
#79527=CARTESIAN_POINT('Ctrl Pts',(-63.2248549788221,-30.4837290014989,
12.));
#79528=CARTESIAN_POINT('Ctrl Pts',(-63.2398888342545,-30.4968940344998,
0.));
#79529=CARTESIAN_POINT('Ctrl Pts',(-63.2398888342545,-30.4968940344998,
12.));
#79530=CARTESIAN_POINT('Ctrl Pts',(-63.2549483856215,-30.5101100066659,
0.));
#79531=CARTESIAN_POINT('Ctrl Pts',(-63.2549483856215,-30.5101100066659,
12.));
#79532=CARTESIAN_POINT('Ctrl Pts',(-63.2700334577639,-30.5233768687865,
0.));
#79533=CARTESIAN_POINT('Ctrl Pts',(-63.2700334577639,-30.5233768687865,
12.));
#79534=CARTESIAN_POINT('Ctrl Pts',(-63.2851438802473,-30.5366945730508,
0.));
#79535=CARTESIAN_POINT('Ctrl Pts',(-63.2851438802473,-30.5366945730508,
12.));
#79536=CARTESIAN_POINT('Ctrl Pts',(-63.3002794756086,-30.5500630691359,
0.));
#79537=CARTESIAN_POINT('Ctrl Pts',(-63.3002794756086,-30.5500630691359,
12.));
#79538=CARTESIAN_POINT('Ctrl Pts',(-63.3154400534397,-30.563482302238,0.));
#79539=CARTESIAN_POINT('Ctrl Pts',(-63.3154400534397,-30.563482302238,12.));
#79540=CARTESIAN_POINT('Ctrl Pts',(-63.3306254165126,-30.5769522151164,
0.));
#79541=CARTESIAN_POINT('Ctrl Pts',(-63.3306254165126,-30.5769522151164,
12.));
#79542=CARTESIAN_POINT('Ctrl Pts',(-63.3458353646154,-30.5904727493711,
0.));
#79543=CARTESIAN_POINT('Ctrl Pts',(-63.3458353646154,-30.5904727493711,
12.));
#79544=CARTESIAN_POINT('Ctrl Pts',(-63.3610696989577,-30.6040438469078,
0.));
#79545=CARTESIAN_POINT('Ctrl Pts',(-63.3610696989577,-30.6040438469078,
12.));
#79546=CARTESIAN_POINT('Ctrl Pts',(-63.3763282271796,-30.6176654515967,
0.));
#79547=CARTESIAN_POINT('Ctrl Pts',(-63.3763282271796,-30.6176654515967,
12.));
#79548=CARTESIAN_POINT('Ctrl Pts',(-63.3916107631376,-30.6313375092062,
0.));
#79549=CARTESIAN_POINT('Ctrl Pts',(-63.3916107631376,-30.6313375092062,
12.));
#79550=CARTESIAN_POINT('Ctrl Pts',(-63.4069171245066,-30.6450599666121,
0.));
#79551=CARTESIAN_POINT('Ctrl Pts',(-63.4069171245066,-30.6450599666121,
12.));
#79552=CARTESIAN_POINT('Ctrl Pts',(-63.4222471311239,-30.6588327712483,
0.));
#79553=CARTESIAN_POINT('Ctrl Pts',(-63.4222471311239,-30.6588327712483,
12.));
#79554=CARTESIAN_POINT('Ctrl Pts',(-63.4376006029604,-30.6726558704315,
0.));
#79555=CARTESIAN_POINT('Ctrl Pts',(-63.4376006029604,-30.6726558704315,
12.));
#79556=CARTESIAN_POINT('Ctrl Pts',(-63.4529773584249,-30.6865292107929,
0.));
#79557=CARTESIAN_POINT('Ctrl Pts',(-63.4529773584249,-30.6865292107929,
12.));
#79558=CARTESIAN_POINT('Ctrl Pts',(-63.4683772152529,-30.7004527385821,
0.));
#79559=CARTESIAN_POINT('Ctrl Pts',(-63.4683772152529,-30.7004527385821,
12.));
#79560=CARTESIAN_POINT('Ctrl Pts',(-63.4837999912771,-30.7144263999265,
0.));
#79561=CARTESIAN_POINT('Ctrl Pts',(-63.4837999912771,-30.7144263999265,
12.));
#79562=CARTESIAN_POINT('Ctrl Pts',(-63.4992455051795,-30.7284501410822,
0.));
#79563=CARTESIAN_POINT('Ctrl Pts',(-63.4992455051795,-30.7284501410822,
12.));
#79564=CARTESIAN_POINT('Ctrl Pts',(-63.5147135773894,-30.7425239087281,
0.));
#79565=CARTESIAN_POINT('Ctrl Pts',(-63.5147135773894,-30.7425239087281,
12.));
#79566=CARTESIAN_POINT('Ctrl Pts',(-63.5302040304142,-30.7566476500757,
0.));
#79567=CARTESIAN_POINT('Ctrl Pts',(-63.5302040304142,-30.7566476500757,
12.));
#79568=CARTESIAN_POINT('Ctrl Pts',(-63.5457166883537,-30.7708213127159,
0.));
#79569=CARTESIAN_POINT('Ctrl Pts',(-63.5457166883537,-30.7708213127159,
12.));
#79570=CARTESIAN_POINT('Ctrl Pts',(-63.5612513766,-30.7850448445205,0.));
#79571=CARTESIAN_POINT('Ctrl Pts',(-63.5612513766,-30.7850448445205,12.));
#79572=CARTESIAN_POINT('Ctrl Pts',(-63.5768079214881,-30.7993181935271,
0.));
#79573=CARTESIAN_POINT('Ctrl Pts',(-63.5768079214881,-30.7993181935271,
12.));
#79574=CARTESIAN_POINT('Ctrl Pts',(-63.5923861498987,-30.813641307801,0.));
#79575=CARTESIAN_POINT('Ctrl Pts',(-63.5923861498987,-30.813641307801,12.));
#79576=CARTESIAN_POINT('Ctrl Pts',(-63.6079858892771,-30.8280141354459,
0.));
#79577=CARTESIAN_POINT('Ctrl Pts',(-63.6079858892771,-30.8280141354459,
12.));
#79578=CARTESIAN_POINT('Ctrl Pts',(-63.6236069678055,-30.8424366246671,
0.));
#79579=CARTESIAN_POINT('Ctrl Pts',(-63.6236069678055,-30.8424366246671,
12.));
#79580=CARTESIAN_POINT('Ctrl Pts',(-63.6392492145233,-30.8569087238131,
0.));
#79581=CARTESIAN_POINT('Ctrl Pts',(-63.6392492145233,-30.8569087238131,
12.));
#79582=CARTESIAN_POINT('Ctrl Pts',(-63.6549124594666,-30.8714303814194,
0.));
#79583=CARTESIAN_POINT('Ctrl Pts',(-63.6549124594666,-30.8714303814194,
12.));
#79584=CARTESIAN_POINT('Ctrl Pts',(-63.6705965337971,-30.8860015462475,
0.));
#79585=CARTESIAN_POINT('Ctrl Pts',(-63.6705965337971,-30.8860015462475,
12.));
#79586=CARTESIAN_POINT('Ctrl Pts',(-63.6863012697328,-30.900622167269,0.));
#79587=CARTESIAN_POINT('Ctrl Pts',(-63.6863012697328,-30.900622167269,12.));
#79588=CARTESIAN_POINT('Ctrl Pts',(-63.7020265004792,-30.9152921936465,
0.));
#79589=CARTESIAN_POINT('Ctrl Pts',(-63.7020265004792,-30.9152921936465,
12.));
#79590=CARTESIAN_POINT('Ctrl Pts',(-63.7177720601609,-30.9300115747115,
0.));
#79591=CARTESIAN_POINT('Ctrl Pts',(-63.7177720601609,-30.9300115747115,
12.));
#79592=CARTESIAN_POINT('Ctrl Pts',(-63.7335377837441,-30.9447802599355,
0.));
#79593=CARTESIAN_POINT('Ctrl Pts',(-63.7335377837441,-30.9447802599355,
12.));
#79594=CARTESIAN_POINT('Ctrl Pts',(-63.749323506987,-30.9595981989103,0.));
#79595=CARTESIAN_POINT('Ctrl Pts',(-63.749323506987,-30.9595981989103,12.));
#79596=CARTESIAN_POINT('Ctrl Pts',(-63.7651290664733,-30.9744653413689,
0.));
#79597=CARTESIAN_POINT('Ctrl Pts',(-63.7651290664733,-30.9744653413689,
12.));
#79598=CARTESIAN_POINT('Ctrl Pts',(-63.7809542996264,-30.989381637191,0.));
#79599=CARTESIAN_POINT('Ctrl Pts',(-63.7809542996264,-30.989381637191,12.));
#79600=CARTESIAN_POINT('Ctrl Pts',(-63.796799044728,-31.0043470364108,0.));
#79601=CARTESIAN_POINT('Ctrl Pts',(-63.796799044728,-31.0043470364108,12.));
#79602=CARTESIAN_POINT('Ctrl Pts',(-63.8126631409364,-31.0193614892171,
0.));
#79603=CARTESIAN_POINT('Ctrl Pts',(-63.8126631409364,-31.0193614892171,
12.));
#79604=CARTESIAN_POINT('Ctrl Pts',(-63.8285464282846,-31.0344249459538,
0.));
#79605=CARTESIAN_POINT('Ctrl Pts',(-63.8285464282846,-31.0344249459538,
12.));
#79606=CARTESIAN_POINT('Ctrl Pts',(-63.8444487476611,-31.0495373571215,
0.));
#79607=CARTESIAN_POINT('Ctrl Pts',(-63.8444487476611,-31.0495373571215,
12.));
#79608=CARTESIAN_POINT('Ctrl Pts',(-63.8603699407922,-31.0646986733723,
0.));
#79609=CARTESIAN_POINT('Ctrl Pts',(-63.8603699407922,-31.0646986733723,
12.));
#79610=CARTESIAN_POINT('Ctrl Pts',(-63.8763098502237,-31.0799088455041,
0.));
#79611=CARTESIAN_POINT('Ctrl Pts',(-63.8763098502237,-31.0799088455041,
12.));
#79612=CARTESIAN_POINT('Ctrl Pts',(-63.8922683192964,-31.0951678244455,
0.));
#79613=CARTESIAN_POINT('Ctrl Pts',(-63.8922683192964,-31.0951678244455,
12.));
#79614=CARTESIAN_POINT('Ctrl Pts',(-63.9082451921448,-31.1104755612607,
0.));
#79615=CARTESIAN_POINT('Ctrl Pts',(-63.9082451921448,-31.1104755612607,
12.));
#79616=CARTESIAN_POINT('Ctrl Pts',(-63.9242403136955,-31.1258320071545,
0.));
#79617=CARTESIAN_POINT('Ctrl Pts',(-63.9242403136955,-31.1258320071545,
12.));
#79618=CARTESIAN_POINT('Ctrl Pts',(-63.940253529665,-31.1412371134727,0.));
#79619=CARTESIAN_POINT('Ctrl Pts',(-63.940253529665,-31.1412371134727,12.));
#79620=CARTESIAN_POINT('Ctrl Pts',(-63.9562846865567,-31.1566908316992,
0.));
#79621=CARTESIAN_POINT('Ctrl Pts',(-63.9562846865567,-31.1566908316992,
12.));
#79622=CARTESIAN_POINT('Ctrl Pts',(-63.9723336316551,-31.1721931134487,
0.));
#79623=CARTESIAN_POINT('Ctrl Pts',(-63.9723336316551,-31.1721931134487,
12.));
#79624=CARTESIAN_POINT('Ctrl Pts',(-63.9884002130211,-31.1877439104717,
0.));
#79625=CARTESIAN_POINT('Ctrl Pts',(-63.9884002130211,-31.1877439104717,
12.));
#79626=CARTESIAN_POINT('Ctrl Pts',(-64.0044842794831,-31.2033431746558,
0.));
#79627=CARTESIAN_POINT('Ctrl Pts',(-64.0044842794831,-31.2033431746558,
12.));
#79628=CARTESIAN_POINT('Ctrl Pts',(-64.02058568063,-31.2189908580245,0.));
#79629=CARTESIAN_POINT('Ctrl Pts',(-64.02058568063,-31.2189908580245,12.));
#79630=CARTESIAN_POINT('Ctrl Pts',(-64.0367042667984,-31.2346869127297,
0.));
#79631=CARTESIAN_POINT('Ctrl Pts',(-64.0367042667984,-31.2346869127297,
12.));
#79632=CARTESIAN_POINT('Ctrl Pts',(-64.0528398890657,-31.2504312910451,
0.));
#79633=CARTESIAN_POINT('Ctrl Pts',(-64.0528398890657,-31.2504312910451,
12.));
#79634=CARTESIAN_POINT('Ctrl Pts',(-64.0689923992461,-31.2662239453728,
0.));
#79635=CARTESIAN_POINT('Ctrl Pts',(-64.0689923992461,-31.2662239453728,
12.));
#79636=CARTESIAN_POINT('Ctrl Pts',(-64.0851616498852,-31.2820648282447,
0.));
#79637=CARTESIAN_POINT('Ctrl Pts',(-64.0851616498852,-31.2820648282447,
12.));
#79638=CARTESIAN_POINT('Ctrl Pts',(-64.1013474942556,-31.2979538923214,
0.));
#79639=CARTESIAN_POINT('Ctrl Pts',(-64.1013474942556,-31.2979538923214,
12.));
#79640=CARTESIAN_POINT('Ctrl Pts',(-64.117549786349,-31.3138910903859,0.));
#79641=CARTESIAN_POINT('Ctrl Pts',(-64.117549786349,-31.3138910903859,12.));
#79642=CARTESIAN_POINT('Ctrl Pts',(-64.133768380869,-31.3298763753377,0.));
#79643=CARTESIAN_POINT('Ctrl Pts',(-64.133768380869,-31.3298763753377,12.));
#79644=CARTESIAN_POINT('Ctrl Pts',(-64.1500031332282,-31.3459097002006,
0.));
#79645=CARTESIAN_POINT('Ctrl Pts',(-64.1500031332282,-31.3459097002006,
12.));
#79646=CARTESIAN_POINT('Ctrl Pts',(-64.166253899542,-31.3619910181228,0.));
#79647=CARTESIAN_POINT('Ctrl Pts',(-64.166253899542,-31.3619910181228,12.));
#79648=CARTESIAN_POINT('Ctrl Pts',(-64.1825205366224,-31.3781202823754,
0.));
#79649=CARTESIAN_POINT('Ctrl Pts',(-64.1825205366224,-31.3781202823754,
12.));
#79650=CARTESIAN_POINT('Ctrl Pts',(-64.1988029019707,-31.3942974463445,
0.));
#79651=CARTESIAN_POINT('Ctrl Pts',(-64.1988029019707,-31.3942974463445,
12.));
#79652=CARTESIAN_POINT('Ctrl Pts',(-64.2151008537697,-31.410522463528,0.));
#79653=CARTESIAN_POINT('Ctrl Pts',(-64.2151008537697,-31.410522463528,12.));
#79654=CARTESIAN_POINT('Ctrl Pts',(-64.231414250881,-31.4267952875423,0.));
#79655=CARTESIAN_POINT('Ctrl Pts',(-64.231414250881,-31.4267952875423,12.));
#79656=CARTESIAN_POINT('Ctrl Pts',(-64.2477429528393,-31.4431158721222,
0.));
#79657=CARTESIAN_POINT('Ctrl Pts',(-64.2477429528393,-31.4431158721222,
12.));
#79658=CARTESIAN_POINT('Ctrl Pts',(-64.2640868198473,-31.4594841711194,
0.));
#79659=CARTESIAN_POINT('Ctrl Pts',(-64.2640868198473,-31.4594841711194,
12.));
#79660=CARTESIAN_POINT('Ctrl Pts',(-64.2804457127671,-31.4759001384941,
0.));
#79661=CARTESIAN_POINT('Ctrl Pts',(-64.2804457127671,-31.4759001384941,
12.));
#79662=CARTESIAN_POINT('Ctrl Pts',(-64.2968194931158,-31.4923637283132,
0.));
#79663=CARTESIAN_POINT('Ctrl Pts',(-64.2968194931158,-31.4923637283132,
12.));
#79664=CARTESIAN_POINT('Ctrl Pts',(-64.3132080230637,-31.5088748947582,
0.));
#79665=CARTESIAN_POINT('Ctrl Pts',(-64.3132080230637,-31.5088748947582,
12.));
#79666=CARTESIAN_POINT('Ctrl Pts',(-64.3296111654283,-31.5254335921245,
0.));
#79667=CARTESIAN_POINT('Ctrl Pts',(-64.3296111654283,-31.5254335921245,
12.));
#79668=CARTESIAN_POINT('Ctrl Pts',(-64.3460287836687,-31.5420397748191,
0.));
#79669=CARTESIAN_POINT('Ctrl Pts',(-64.3460287836687,-31.5420397748191,
12.));
#79670=CARTESIAN_POINT('Ctrl Pts',(-64.3624607418768,-31.5586933973515,
0.));
#79671=CARTESIAN_POINT('Ctrl Pts',(-64.3624607418768,-31.5586933973515,
12.));
#79672=CARTESIAN_POINT('Ctrl Pts',(-64.3789069047733,-31.5753944143336,
0.));
#79673=CARTESIAN_POINT('Ctrl Pts',(-64.3789069047733,-31.5753944143336,
12.));
#79674=CARTESIAN_POINT('Ctrl Pts',(-64.3953671377046,-31.5921427804865,
0.));
#79675=CARTESIAN_POINT('Ctrl Pts',(-64.3953671377046,-31.5921427804865,
12.));
#79676=CARTESIAN_POINT('Ctrl Pts',(-64.4118413066378,-31.6089384506395,
0.));
#79677=CARTESIAN_POINT('Ctrl Pts',(-64.4118413066378,-31.6089384506395,
12.));
#79678=CARTESIAN_POINT('Ctrl Pts',(-64.4283292781565,-31.6257813797287,
0.));
#79679=CARTESIAN_POINT('Ctrl Pts',(-64.4283292781565,-31.6257813797287,
12.));
#79680=CARTESIAN_POINT('Ctrl Pts',(-64.4448309194525,-31.6426715227878,
0.));
#79681=CARTESIAN_POINT('Ctrl Pts',(-64.4448309194525,-31.6426715227878,
12.));
#79682=CARTESIAN_POINT('Ctrl Pts',(-64.4613460983214,-31.6596088349482,
0.));
#79683=CARTESIAN_POINT('Ctrl Pts',(-64.4613460983214,-31.6596088349482,
12.));
#79684=CARTESIAN_POINT('Ctrl Pts',(-64.4778746831614,-31.6765932714464,
0.));
#79685=CARTESIAN_POINT('Ctrl Pts',(-64.4778746831614,-31.6765932714464,
12.));
#79686=CARTESIAN_POINT('Ctrl Pts',(-64.4944165429675,-31.6936247876229,
0.));
#79687=CARTESIAN_POINT('Ctrl Pts',(-64.4944165429675,-31.6936247876229,
12.));
#79688=CARTESIAN_POINT('Ctrl Pts',(-64.510971547327,-31.7107033389201,0.));
#79689=CARTESIAN_POINT('Ctrl Pts',(-64.510971547327,-31.7107033389201,12.));
#79690=CARTESIAN_POINT('Ctrl Pts',(-64.5275395664124,-31.7278288808731,
0.));
#79691=CARTESIAN_POINT('Ctrl Pts',(-64.5275395664124,-31.7278288808731,
12.));
#79692=CARTESIAN_POINT('Ctrl Pts',(-64.544120470977,-31.7450013691112,0.));
#79693=CARTESIAN_POINT('Ctrl Pts',(-64.544120470977,-31.7450013691112,12.));
#79694=CARTESIAN_POINT('Ctrl Pts',(-64.5607141323521,-31.7622207593634,
0.));
#79695=CARTESIAN_POINT('Ctrl Pts',(-64.5607141323521,-31.7622207593634,
12.));
#79696=CARTESIAN_POINT('Ctrl Pts',(-64.5773204224429,-31.7794870074583,
0.));
#79697=CARTESIAN_POINT('Ctrl Pts',(-64.5773204224429,-31.7794870074583,
12.));
#79698=CARTESIAN_POINT('Ctrl Pts',(-64.5939392137235,-31.7968000693218,
0.));
#79699=CARTESIAN_POINT('Ctrl Pts',(-64.5939392137235,-31.7968000693218,
12.));
#79700=CARTESIAN_POINT('Ctrl Pts',(-64.6105703792312,-31.8141599009684,
0.));
#79701=CARTESIAN_POINT('Ctrl Pts',(-64.6105703792312,-31.8141599009684,
12.));
#79702=CARTESIAN_POINT('Ctrl Pts',(-64.6272137925627,-31.8315664585026,
0.));
#79703=CARTESIAN_POINT('Ctrl Pts',(-64.6272137925627,-31.8315664585026,
12.));
#79704=CARTESIAN_POINT('Ctrl Pts',(-64.6438693278714,-31.8490196981248,
0.));
#79705=CARTESIAN_POINT('Ctrl Pts',(-64.6438693278714,-31.8490196981248,
12.));
#79706=CARTESIAN_POINT('Ctrl Pts',(-64.6605368598629,-31.866519576131,0.));
#79707=CARTESIAN_POINT('Ctrl Pts',(-64.6605368598629,-31.866519576131,12.));
#79708=CARTESIAN_POINT('Ctrl Pts',(-64.6772162637907,-31.8840660489107,
0.));
#79709=CARTESIAN_POINT('Ctrl Pts',(-64.6772162637907,-31.8840660489107,
12.));
#79710=CARTESIAN_POINT('Ctrl Pts',(-64.6939074154498,-31.9016590729374,
0.));
#79711=CARTESIAN_POINT('Ctrl Pts',(-64.6939074154498,-31.9016590729374,
12.));
#79712=CARTESIAN_POINT('Ctrl Pts',(-64.7106101911732,-31.9192986047706,
0.));
#79713=CARTESIAN_POINT('Ctrl Pts',(-64.7106101911732,-31.9192986047706,
12.));
#79714=CARTESIAN_POINT('Ctrl Pts',(-64.7273244678297,-31.9369846010615,
0.));
#79715=CARTESIAN_POINT('Ctrl Pts',(-64.7273244678297,-31.9369846010615,
12.));
#79716=CARTESIAN_POINT('Ctrl Pts',(-64.7440501228202,-31.9547170185534,
0.));
#79717=CARTESIAN_POINT('Ctrl Pts',(-64.7440501228202,-31.9547170185534,
12.));
#79718=CARTESIAN_POINT('Ctrl Pts',(-64.7607870340735,-31.9724958140789,
0.));
#79719=CARTESIAN_POINT('Ctrl Pts',(-64.7607870340735,-31.9724958140789,
12.));
#79720=CARTESIAN_POINT('Ctrl Pts',(-64.77753508004,-31.990320944552,0.));
#79721=CARTESIAN_POINT('Ctrl Pts',(-64.77753508004,-31.990320944552,12.));
#79722=CARTESIAN_POINT('Ctrl Pts',(-64.7942941396881,-32.0081923669677,
0.));
#79723=CARTESIAN_POINT('Ctrl Pts',(-64.7942941396881,-32.0081923669677,
12.));
#79724=CARTESIAN_POINT('Ctrl Pts',(-64.8110640925021,-32.0261100384092,
0.));
#79725=CARTESIAN_POINT('Ctrl Pts',(-64.8110640925021,-32.0261100384092,
12.));
#79726=CARTESIAN_POINT('Ctrl Pts',(-64.8278448184786,-32.0440739160477,
0.));
#79727=CARTESIAN_POINT('Ctrl Pts',(-64.8278448184786,-32.0440739160477,
12.));
#79728=CARTESIAN_POINT('Ctrl Pts',(-64.8446361981234,-32.0620839571408,
0.));
#79729=CARTESIAN_POINT('Ctrl Pts',(-64.8446361981234,-32.0620839571408,
12.));
#79730=CARTESIAN_POINT('Ctrl Pts',(-64.861438112445,-32.0801401190241,0.));
#79731=CARTESIAN_POINT('Ctrl Pts',(-64.861438112445,-32.0801401190241,12.));
#79732=CARTESIAN_POINT('Ctrl Pts',(-64.878250442952,-32.0982423591108,0.));
#79733=CARTESIAN_POINT('Ctrl Pts',(-64.878250442952,-32.0982423591108,12.));
#79734=CARTESIAN_POINT('Ctrl Pts',(-64.8950730716493,-32.1163906348979,
0.));
#79735=CARTESIAN_POINT('Ctrl Pts',(-64.8950730716493,-32.1163906348979,
12.));
#79736=CARTESIAN_POINT('Ctrl Pts',(-64.9119058810362,-32.1345849039671,
0.));
#79737=CARTESIAN_POINT('Ctrl Pts',(-64.9119058810362,-32.1345849039671,
12.));
#79738=CARTESIAN_POINT('Ctrl Pts',(-64.9287487541018,-32.1528251239832,
0.));
#79739=CARTESIAN_POINT('Ctrl Pts',(-64.9287487541018,-32.1528251239832,
12.));
#79740=CARTESIAN_POINT('Ctrl Pts',(-64.9456015743203,-32.171111252686,0.));
#79741=CARTESIAN_POINT('Ctrl Pts',(-64.9456015743203,-32.171111252686,12.));
#79742=CARTESIAN_POINT('Ctrl Pts',(-64.9624642256477,-32.1894432478889,
0.));
#79743=CARTESIAN_POINT('Ctrl Pts',(-64.9624642256477,-32.1894432478889,
12.));
#79744=CARTESIAN_POINT('Ctrl Pts',(-64.9793365925194,-32.2078210674857,
0.));
#79745=CARTESIAN_POINT('Ctrl Pts',(-64.9793365925194,-32.2078210674857,
12.));
#79746=CARTESIAN_POINT('Ctrl Pts',(-64.996218559847,-32.2262446694516,0.));
#79747=CARTESIAN_POINT('Ctrl Pts',(-64.996218559847,-32.2262446694516,12.));
#79748=CARTESIAN_POINT('Ctrl Pts',(-65.0131100130155,-32.244714011842,0.));
#79749=CARTESIAN_POINT('Ctrl Pts',(-65.0131100130155,-32.244714011842,12.));
#79750=CARTESIAN_POINT('Ctrl Pts',(-65.0300108378786,-32.2632290527855,
0.));
#79751=CARTESIAN_POINT('Ctrl Pts',(-65.0300108378786,-32.2632290527855,
12.));
#79752=CARTESIAN_POINT('Ctrl Pts',(-65.0469209207548,-32.2817897504799,
0.));
#79753=CARTESIAN_POINT('Ctrl Pts',(-65.0469209207548,-32.2817897504799,
12.));
#79754=CARTESIAN_POINT('Ctrl Pts',(-65.0638401484245,-32.3003960632,0.));
#79755=CARTESIAN_POINT('Ctrl Pts',(-65.0638401484245,-32.3003960632,12.));
#79756=CARTESIAN_POINT('Ctrl Pts',(-65.0807684081278,-32.3190479492985,
0.));
#79757=CARTESIAN_POINT('Ctrl Pts',(-65.0807684081278,-32.3190479492985,
12.));
#79758=CARTESIAN_POINT('Ctrl Pts',(-65.097705587561,-32.3377453672052,0.));
#79759=CARTESIAN_POINT('Ctrl Pts',(-65.097705587561,-32.3377453672052,12.));
#79760=CARTESIAN_POINT('Ctrl Pts',(-65.1146515748723,-32.3564882754212,
0.));
#79761=CARTESIAN_POINT('Ctrl Pts',(-65.1146515748723,-32.3564882754212,
12.));
#79762=CARTESIAN_POINT('Ctrl Pts',(-65.1316062586586,-32.3752766325135,
0.));
#79763=CARTESIAN_POINT('Ctrl Pts',(-65.1316062586586,-32.3752766325135,
12.));
#79764=CARTESIAN_POINT('Ctrl Pts',(-65.1485695279628,-32.3941103971218,
0.));
#79765=CARTESIAN_POINT('Ctrl Pts',(-65.1485695279628,-32.3941103971218,
12.));
#79766=CARTESIAN_POINT('Ctrl Pts',(-65.165541272272,-32.4129895279612,0.));
#79767=CARTESIAN_POINT('Ctrl Pts',(-65.165541272272,-32.4129895279612,12.));
#79768=CARTESIAN_POINT('Ctrl Pts',(-65.182521381514,-32.4319139838212,0.));
#79769=CARTESIAN_POINT('Ctrl Pts',(-65.182521381514,-32.4319139838212,12.));
#79770=CARTESIAN_POINT('Ctrl Pts',(-65.1995097460546,-32.4508837235613,
0.));
#79771=CARTESIAN_POINT('Ctrl Pts',(-65.1995097460546,-32.4508837235613,
12.));
#79772=CARTESIAN_POINT('Ctrl Pts',(-65.2165062566936,-32.4698987061037,
0.));
#79773=CARTESIAN_POINT('Ctrl Pts',(-65.2165062566936,-32.4698987061037,
12.));
#79774=CARTESIAN_POINT('Ctrl Pts',(-65.2335108046625,-32.4889588904397,
0.));
#79775=CARTESIAN_POINT('Ctrl Pts',(-65.2335108046625,-32.4889588904397,
12.));
#79776=CARTESIAN_POINT('Ctrl Pts',(-65.2505232816215,-32.508064235633,0.));
#79777=CARTESIAN_POINT('Ctrl Pts',(-65.2505232816215,-32.508064235633,12.));
#79778=CARTESIAN_POINT('Ctrl Pts',(-65.2675435796558,-32.5272147008191,
0.));
#79779=CARTESIAN_POINT('Ctrl Pts',(-65.2675435796558,-32.5272147008191,
12.));
#79780=CARTESIAN_POINT('Ctrl Pts',(-65.2845715912717,-32.5464102452013,
0.));
#79781=CARTESIAN_POINT('Ctrl Pts',(-65.2845715912717,-32.5464102452013,
12.));
#79782=CARTESIAN_POINT('Ctrl Pts',(-65.3016072093907,-32.565650828042,0.));
#79783=CARTESIAN_POINT('Ctrl Pts',(-65.3016072093907,-32.565650828042,12.));
#79784=CARTESIAN_POINT('Ctrl Pts',(-65.3186503273498,-32.5849364086679,
0.));
#79785=CARTESIAN_POINT('Ctrl Pts',(-65.3186503273498,-32.5849364086679,
12.));
#79786=CARTESIAN_POINT('Ctrl Pts',(-65.3357008389004,-32.6042669464752,
0.));
#79787=CARTESIAN_POINT('Ctrl Pts',(-65.3357008389004,-32.6042669464752,
12.));
#79788=CARTESIAN_POINT('Ctrl Pts',(-65.3527586382082,-32.6236424009302,
0.));
#79789=CARTESIAN_POINT('Ctrl Pts',(-65.3527586382082,-32.6236424009302,
12.));
#79790=CARTESIAN_POINT('Ctrl Pts',(-65.3698236198511,-32.6430627315673,
0.));
#79791=CARTESIAN_POINT('Ctrl Pts',(-65.3698236198511,-32.6430627315673,
12.));
#79792=CARTESIAN_POINT('Ctrl Pts',(-65.3868956788178,-32.6625278979807,
0.));
#79793=CARTESIAN_POINT('Ctrl Pts',(-65.3868956788178,-32.6625278979807,
12.));
#79794=CARTESIAN_POINT('Ctrl Pts',(-65.4039747105033,-32.6820378598262,
0.));
#79795=CARTESIAN_POINT('Ctrl Pts',(-65.4039747105033,-32.6820378598262,
12.));
#79796=CARTESIAN_POINT('Ctrl Pts',(-65.4210606107029,-32.7015925768261,
0.));
#79797=CARTESIAN_POINT('Ctrl Pts',(-65.4210606107029,-32.7015925768261,
12.));
#79798=CARTESIAN_POINT('Ctrl Pts',(-65.4381532756062,-32.7211920087682,
0.));
#79799=CARTESIAN_POINT('Ctrl Pts',(-65.4381532756062,-32.7211920087682,
12.));
#79800=CARTESIAN_POINT('Ctrl Pts',(-65.4552526017907,-32.7408361155038,
0.));
#79801=CARTESIAN_POINT('Ctrl Pts',(-65.4552526017907,-32.7408361155038,
12.));
#79802=CARTESIAN_POINT('Ctrl Pts',(-65.4723584862129,-32.7605248569382,
0.));
#79803=CARTESIAN_POINT('Ctrl Pts',(-65.4723584862129,-32.7605248569382,
12.));
#79804=CARTESIAN_POINT('Ctrl Pts',(-65.4894708262071,-32.7802581930293,
0.));
#79805=CARTESIAN_POINT('Ctrl Pts',(-65.4894708262071,-32.7802581930293,
12.));
#79806=CARTESIAN_POINT('Ctrl Pts',(-65.5065895194938,-32.8000360837981,
0.));
#79807=CARTESIAN_POINT('Ctrl Pts',(-65.5065895194938,-32.8000360837981,
12.));
#79808=CARTESIAN_POINT('Ctrl Pts',(-65.5237144641864,-32.8198584893319,
0.));
#79809=CARTESIAN_POINT('Ctrl Pts',(-65.5237144641864,-32.8198584893319,
12.));
#79810=CARTESIAN_POINT('Ctrl Pts',(-65.5408455587963,-32.8397253697864,
0.));
#79811=CARTESIAN_POINT('Ctrl Pts',(-65.5408455587963,-32.8397253697864,
12.));
#79812=CARTESIAN_POINT('Ctrl Pts',(-65.5579827022412,-32.8596366853826,
0.));
#79813=CARTESIAN_POINT('Ctrl Pts',(-65.5579827022412,-32.8596366853826,
12.));
#79814=CARTESIAN_POINT('Ctrl Pts',(-65.575125793846,-32.8795923964022,0.));
#79815=CARTESIAN_POINT('Ctrl Pts',(-65.575125793846,-32.8795923964022,12.));
#79816=CARTESIAN_POINT('Ctrl Pts',(-65.5922747333181,-32.899592463189,0.));
#79817=CARTESIAN_POINT('Ctrl Pts',(-65.5922747333181,-32.899592463189,12.));
#79818=CARTESIAN_POINT('Ctrl Pts',(-65.6094294207267,-32.9196368461457,
0.));
#79819=CARTESIAN_POINT('Ctrl Pts',(-65.6094294207267,-32.9196368461457,
12.));
#79820=CARTESIAN_POINT('Ctrl Pts',(-65.6265897564782,-32.9397255057273,
0.));
#79821=CARTESIAN_POINT('Ctrl Pts',(-65.6265897564782,-32.9397255057273,
12.));
#79822=CARTESIAN_POINT('Ctrl Pts',(-65.6437556412956,-32.9598584024318,
0.));
#79823=CARTESIAN_POINT('Ctrl Pts',(-65.6437556412956,-32.9598584024318,
12.));
#79824=CARTESIAN_POINT('Ctrl Pts',(-65.6609269761902,-32.9800354967847,
0.));
#79825=CARTESIAN_POINT('Ctrl Pts',(-65.6609269761902,-32.9800354967847,
12.));
#79826=CARTESIAN_POINT('Ctrl Pts',(-65.6781036625041,-33.0002567493581,
0.));
#79827=CARTESIAN_POINT('Ctrl Pts',(-65.6781036625041,-33.0002567493581,
12.));
#79828=CARTESIAN_POINT('Ctrl Pts',(-65.6952856019542,-33.0205221207877,
0.));
#79829=CARTESIAN_POINT('Ctrl Pts',(-65.6952856019542,-33.0205221207877,
12.));
#79830=CARTESIAN_POINT('Ctrl Pts',(-65.7124726966805,-33.0408315717874,
0.));
#79831=CARTESIAN_POINT('Ctrl Pts',(-65.7124726966805,-33.0408315717874,
12.));
#79832=CARTESIAN_POINT('Ctrl Pts',(-65.729664849282,-33.061185063158,0.));
#79833=CARTESIAN_POINT('Ctrl Pts',(-65.729664849282,-33.061185063158,12.));
#79834=CARTESIAN_POINT('Ctrl Pts',(-65.7468619628808,-33.0815825557976,
0.));
#79835=CARTESIAN_POINT('Ctrl Pts',(-65.7468619628808,-33.0815825557976,
12.));
#79836=CARTESIAN_POINT('Ctrl Pts',(-65.7640639410653,-33.102024010688,0.));
#79837=CARTESIAN_POINT('Ctrl Pts',(-65.7640639410653,-33.102024010688,12.));
#79838=CARTESIAN_POINT('Ctrl Pts',(-65.7812706877691,-33.1225093888668,
0.));
#79839=CARTESIAN_POINT('Ctrl Pts',(-65.7812706877691,-33.1225093888668,
12.));
#79840=CARTESIAN_POINT('Ctrl Pts',(-65.7984821071621,-33.1430386513975,
0.));
#79841=CARTESIAN_POINT('Ctrl Pts',(-65.7984821071621,-33.1430386513975,
12.));
#79842=CARTESIAN_POINT('Ctrl Pts',(-65.8156981035504,-33.16361175934,0.));
#79843=CARTESIAN_POINT('Ctrl Pts',(-65.8156981035504,-33.16361175934,12.));
#79844=CARTESIAN_POINT('Ctrl Pts',(-65.8329185812379,-33.1842286737053,
0.));
#79845=CARTESIAN_POINT('Ctrl Pts',(-65.8329185812379,-33.1842286737053,
12.));
#79846=CARTESIAN_POINT('Ctrl Pts',(-65.8501434445174,-33.2048893554496,
0.));
#79847=CARTESIAN_POINT('Ctrl Pts',(-65.8501434445174,-33.2048893554496,
12.));
#79848=CARTESIAN_POINT('Ctrl Pts',(-65.8673725979591,-33.2255937655656,
0.));
#79849=CARTESIAN_POINT('Ctrl Pts',(-65.8673725979591,-33.2255937655656,
12.));
#79850=CARTESIAN_POINT('Ctrl Pts',(-65.8846059466382,-33.2463418651498,
0.));
#79851=CARTESIAN_POINT('Ctrl Pts',(-65.8846059466382,-33.2463418651498,
12.));
#79852=CARTESIAN_POINT('Ctrl Pts',(-65.901843396389,-33.2671336154754,0.));
#79853=CARTESIAN_POINT('Ctrl Pts',(-65.901843396389,-33.2671336154754,12.));
#79854=CARTESIAN_POINT('Ctrl Pts',(-65.9190848540422,-33.2879689780566,
0.));
#79855=CARTESIAN_POINT('Ctrl Pts',(-65.9190848540422,-33.2879689780566,
12.));
#79856=CARTESIAN_POINT('Ctrl Pts',(-65.9363302276822,-33.3088479147151,
0.));
#79857=CARTESIAN_POINT('Ctrl Pts',(-65.9363302276822,-33.3088479147151,
12.));
#79858=CARTESIAN_POINT('Ctrl Pts',(-65.9535794260802,-33.3297703874249,
0.));
#79859=CARTESIAN_POINT('Ctrl Pts',(-65.9535794260802,-33.3297703874249,
12.));
#79860=CARTESIAN_POINT('Ctrl Pts',(-65.9708323581385,-33.3507363581579,
0.));
#79861=CARTESIAN_POINT('Ctrl Pts',(-65.9708323581385,-33.3507363581579,
12.));
#79862=CARTESIAN_POINT('Ctrl Pts',(-65.9880889322822,-33.3717457887095,
0.));
#79863=CARTESIAN_POINT('Ctrl Pts',(-65.9880889322822,-33.3717457887095,
12.));
#79864=CARTESIAN_POINT('Ctrl Pts',(-66.0053490559826,-33.3927986405612,
0.));
#79865=CARTESIAN_POINT('Ctrl Pts',(-66.0053490559826,-33.3927986405612,
12.));
#79866=CARTESIAN_POINT('Ctrl Pts',(-66.0226126349482,-33.4138948746408,
0.));
#79867=CARTESIAN_POINT('Ctrl Pts',(-66.0226126349482,-33.4138948746408,
12.));
#79868=CARTESIAN_POINT('Ctrl Pts',(-66.0398795737827,-33.4350344515128,
0.));
#79869=CARTESIAN_POINT('Ctrl Pts',(-66.0398795737827,-33.4350344515128,
12.));
#79870=CARTESIAN_POINT('Ctrl Pts',(-66.0571497774484,-33.4562173318052,
0.));
#79871=CARTESIAN_POINT('Ctrl Pts',(-66.0571497774484,-33.4562173318052,
12.));
#79872=CARTESIAN_POINT('Ctrl Pts',(-66.0744231525445,-33.4774434765762,
0.));
#79873=CARTESIAN_POINT('Ctrl Pts',(-66.0744231525445,-33.4774434765762,
12.));
#79874=CARTESIAN_POINT('Ctrl Pts',(-66.0916996085237,-33.4987128476618,
0.));
#79875=CARTESIAN_POINT('Ctrl Pts',(-66.0916996085237,-33.4987128476618,
12.));
#79876=CARTESIAN_POINT('Ctrl Pts',(-66.1089790592673,-33.5200254081212,
0.));
#79877=CARTESIAN_POINT('Ctrl Pts',(-66.1089790592673,-33.5200254081212,
12.));
#79878=CARTESIAN_POINT('Ctrl Pts',(-66.1262614234579,-33.5413811223398,
0.));
#79879=CARTESIAN_POINT('Ctrl Pts',(-66.1262614234579,-33.5413811223398,
12.));
#79880=CARTESIAN_POINT('Ctrl Pts',(-66.1435466210966,-33.5627799550422,
0.));
#79881=CARTESIAN_POINT('Ctrl Pts',(-66.1435466210966,-33.5627799550422,
12.));
#79882=CARTESIAN_POINT('Ctrl Pts',(-66.1608345707552,-33.5842218705103,
0.));
#79883=CARTESIAN_POINT('Ctrl Pts',(-66.1608345707552,-33.5842218705103,
12.));
#79884=CARTESIAN_POINT('Ctrl Pts',(-66.1781251863998,-33.6057068316758,
0.));
#79885=CARTESIAN_POINT('Ctrl Pts',(-66.1781251863998,-33.6057068316758,
12.));
#79886=CARTESIAN_POINT('Ctrl Pts',(-66.1954183747167,-33.6272347993519,
0.));
#79887=CARTESIAN_POINT('Ctrl Pts',(-66.1954183747167,-33.6272347993519,
12.));
#79888=CARTESIAN_POINT('Ctrl Pts',(-66.2127140313777,-33.648805731163,0.));
#79889=CARTESIAN_POINT('Ctrl Pts',(-66.2127140313777,-33.648805731163,12.));
#79890=CARTESIAN_POINT('Ctrl Pts',(-66.2300120464323,-33.6704195830526,
0.));
#79891=CARTESIAN_POINT('Ctrl Pts',(-66.2300120464323,-33.6704195830526,
12.));
#79892=CARTESIAN_POINT('Ctrl Pts',(-66.2473123109626,-33.6920763111575,
0.));
#79893=CARTESIAN_POINT('Ctrl Pts',(-66.2473123109626,-33.6920763111575,
12.));
#79894=CARTESIAN_POINT('Ctrl Pts',(-66.2646147235444,-33.713775873597,0.));
#79895=CARTESIAN_POINT('Ctrl Pts',(-66.2646147235444,-33.713775873597,12.));
#79896=CARTESIAN_POINT('Ctrl Pts',(-66.2819191962273,-33.7355182321862,
0.));
#79897=CARTESIAN_POINT('Ctrl Pts',(-66.2819191962273,-33.7355182321862,
12.));
#79898=CARTESIAN_POINT('Ctrl Pts',(-66.2992256621001,-33.7573033544374,
0.));
#79899=CARTESIAN_POINT('Ctrl Pts',(-66.2992256621001,-33.7573033544374,
12.));
#79900=CARTESIAN_POINT('Ctrl Pts',(-66.3165340771053,-33.7791312144798,
0.));
#79901=CARTESIAN_POINT('Ctrl Pts',(-66.3165340771053,-33.7791312144798,
12.));
#79902=CARTESIAN_POINT('Ctrl Pts',(-66.3338444143559,-33.8010017925666,
0.));
#79903=CARTESIAN_POINT('Ctrl Pts',(-66.3338444143559,-33.8010017925666,
12.));
#79904=CARTESIAN_POINT('Ctrl Pts',(-66.3476942111456,-33.8185324184602,
0.));
#79905=CARTESIAN_POINT('Ctrl Pts',(-66.3476942111456,-33.8185324184602,
12.));
#79906=CARTESIAN_POINT('Ctrl Pts',(-66.3580824155565,-33.831699601175,0.));
#79907=CARTESIAN_POINT('Ctrl Pts',(-66.3580824155565,-33.831699601175,12.));
#79908=CARTESIAN_POINT('Ctrl Pts',(-66.3650082659593,-33.8404862618803,
0.));
#79909=CARTESIAN_POINT('Ctrl Pts',(-66.3650082659593,-33.8404862618803,
12.));
#79910=CARTESIAN_POINT('Ctrl Pts',(-66.3684712863594,-33.8448817269567,
0.));
#79911=CARTESIAN_POINT('Ctrl Pts',(-66.3684712863594,-33.8448817269567,
12.));
#79912=CARTESIAN_POINT('',(-63.0759831361898,-30.3549065457811,0.));
#79913=CARTESIAN_POINT('Ctrl Pts',(-63.0759831361898,-30.3549065457811,
0.));
#79914=CARTESIAN_POINT('Ctrl Pts',(-63.078933570069,-30.3574319069329,0.));
#79915=CARTESIAN_POINT('Ctrl Pts',(-63.0848371718048,-30.3624877680651,
0.));
#79916=CARTESIAN_POINT('Ctrl Pts',(-63.0937007763471,-30.3700869762507,
0.));
#79917=CARTESIAN_POINT('Ctrl Pts',(-63.105535320226,-30.3802500880403,0.));
#79918=CARTESIAN_POINT('Ctrl Pts',(-63.1203558300657,-30.3930053710484,
0.));
#79919=CARTESIAN_POINT('Ctrl Pts',(-63.135203629844,-30.4058120432228,0.));
#79920=CARTESIAN_POINT('Ctrl Pts',(-63.1500786361459,-30.418670087563,0.));
#79921=CARTESIAN_POINT('Ctrl Pts',(-63.164980701691,-30.4315794659731,0.));
#79922=CARTESIAN_POINT('Ctrl Pts',(-63.179909617189,-30.444540119238,0.));
#79923=CARTESIAN_POINT('Ctrl Pts',(-63.1948651386942,-30.4575519763337,
0.));
#79924=CARTESIAN_POINT('Ctrl Pts',(-63.2098470086636,-30.470614961416,0.));
#79925=CARTESIAN_POINT('Ctrl Pts',(-63.2248549788221,-30.4837290014989,
0.));
#79926=CARTESIAN_POINT('Ctrl Pts',(-63.2398888342545,-30.4968940344998,
0.));
#79927=CARTESIAN_POINT('Ctrl Pts',(-63.2549483856215,-30.5101100066659,
0.));
#79928=CARTESIAN_POINT('Ctrl Pts',(-63.2700334577639,-30.5233768687865,
0.));
#79929=CARTESIAN_POINT('Ctrl Pts',(-63.2851438802473,-30.5366945730508,
0.));
#79930=CARTESIAN_POINT('Ctrl Pts',(-63.3002794756086,-30.5500630691359,
0.));
#79931=CARTESIAN_POINT('Ctrl Pts',(-63.3154400534397,-30.563482302238,0.));
#79932=CARTESIAN_POINT('Ctrl Pts',(-63.3306254165126,-30.5769522151164,
0.));
#79933=CARTESIAN_POINT('Ctrl Pts',(-63.3458353646154,-30.5904727493711,
0.));
#79934=CARTESIAN_POINT('Ctrl Pts',(-63.3610696989577,-30.6040438469078,
0.));
#79935=CARTESIAN_POINT('Ctrl Pts',(-63.3763282271796,-30.6176654515967,
0.));
#79936=CARTESIAN_POINT('Ctrl Pts',(-63.3916107631376,-30.6313375092062,
0.));
#79937=CARTESIAN_POINT('Ctrl Pts',(-63.4069171245066,-30.6450599666121,
0.));
#79938=CARTESIAN_POINT('Ctrl Pts',(-63.4222471311239,-30.6588327712483,
0.));
#79939=CARTESIAN_POINT('Ctrl Pts',(-63.4376006029604,-30.6726558704315,
0.));
#79940=CARTESIAN_POINT('Ctrl Pts',(-63.4529773584249,-30.6865292107929,
0.));
#79941=CARTESIAN_POINT('Ctrl Pts',(-63.4683772152529,-30.7004527385821,
0.));
#79942=CARTESIAN_POINT('Ctrl Pts',(-63.4837999912771,-30.7144263999265,
0.));
#79943=CARTESIAN_POINT('Ctrl Pts',(-63.4992455051795,-30.7284501410822,
0.));
#79944=CARTESIAN_POINT('Ctrl Pts',(-63.5147135773894,-30.7425239087281,
0.));
#79945=CARTESIAN_POINT('Ctrl Pts',(-63.5302040304142,-30.7566476500757,
0.));
#79946=CARTESIAN_POINT('Ctrl Pts',(-63.5457166883537,-30.7708213127159,
0.));
#79947=CARTESIAN_POINT('Ctrl Pts',(-63.5612513766,-30.7850448445205,0.));
#79948=CARTESIAN_POINT('Ctrl Pts',(-63.5768079214881,-30.7993181935271,
0.));
#79949=CARTESIAN_POINT('Ctrl Pts',(-63.5923861498987,-30.813641307801,0.));
#79950=CARTESIAN_POINT('Ctrl Pts',(-63.6079858892771,-30.8280141354459,
0.));
#79951=CARTESIAN_POINT('Ctrl Pts',(-63.6236069678055,-30.8424366246671,
0.));
#79952=CARTESIAN_POINT('Ctrl Pts',(-63.6392492145233,-30.8569087238131,
0.));
#79953=CARTESIAN_POINT('Ctrl Pts',(-63.6549124594666,-30.8714303814194,
0.));
#79954=CARTESIAN_POINT('Ctrl Pts',(-63.6705965337971,-30.8860015462475,
0.));
#79955=CARTESIAN_POINT('Ctrl Pts',(-63.6863012697328,-30.900622167269,0.));
#79956=CARTESIAN_POINT('Ctrl Pts',(-63.7020265004792,-30.9152921936465,
0.));
#79957=CARTESIAN_POINT('Ctrl Pts',(-63.7177720601609,-30.9300115747115,
0.));
#79958=CARTESIAN_POINT('Ctrl Pts',(-63.7335377837441,-30.9447802599355,
0.));
#79959=CARTESIAN_POINT('Ctrl Pts',(-63.749323506987,-30.9595981989103,0.));
#79960=CARTESIAN_POINT('Ctrl Pts',(-63.7651290664733,-30.9744653413689,
0.));
#79961=CARTESIAN_POINT('Ctrl Pts',(-63.7809542996264,-30.989381637191,0.));
#79962=CARTESIAN_POINT('Ctrl Pts',(-63.796799044728,-31.0043470364108,0.));
#79963=CARTESIAN_POINT('Ctrl Pts',(-63.8126631409364,-31.0193614892171,
0.));
#79964=CARTESIAN_POINT('Ctrl Pts',(-63.8285464282846,-31.0344249459538,
0.));
#79965=CARTESIAN_POINT('Ctrl Pts',(-63.8444487476611,-31.0495373571215,
0.));
#79966=CARTESIAN_POINT('Ctrl Pts',(-63.8603699407922,-31.0646986733723,
0.));
#79967=CARTESIAN_POINT('Ctrl Pts',(-63.8763098502237,-31.0799088455041,
0.));
#79968=CARTESIAN_POINT('Ctrl Pts',(-63.8922683192964,-31.0951678244455,
0.));
#79969=CARTESIAN_POINT('Ctrl Pts',(-63.9082451921448,-31.1104755612607,
0.));
#79970=CARTESIAN_POINT('Ctrl Pts',(-63.9242403136955,-31.1258320071545,
0.));
#79971=CARTESIAN_POINT('Ctrl Pts',(-63.940253529665,-31.1412371134727,0.));
#79972=CARTESIAN_POINT('Ctrl Pts',(-63.9562846865567,-31.1566908316992,
0.));
#79973=CARTESIAN_POINT('Ctrl Pts',(-63.9723336316551,-31.1721931134487,
0.));
#79974=CARTESIAN_POINT('Ctrl Pts',(-63.9884002130211,-31.1877439104717,
0.));
#79975=CARTESIAN_POINT('Ctrl Pts',(-64.0044842794831,-31.2033431746558,
0.));
#79976=CARTESIAN_POINT('Ctrl Pts',(-64.02058568063,-31.2189908580245,0.));
#79977=CARTESIAN_POINT('Ctrl Pts',(-64.0367042667984,-31.2346869127297,
0.));
#79978=CARTESIAN_POINT('Ctrl Pts',(-64.0528398890657,-31.2504312910451,
0.));
#79979=CARTESIAN_POINT('Ctrl Pts',(-64.0689923992461,-31.2662239453728,
0.));
#79980=CARTESIAN_POINT('Ctrl Pts',(-64.0851616498852,-31.2820648282447,
0.));
#79981=CARTESIAN_POINT('Ctrl Pts',(-64.1013474942556,-31.2979538923214,
0.));
#79982=CARTESIAN_POINT('Ctrl Pts',(-64.117549786349,-31.3138910903859,0.));
#79983=CARTESIAN_POINT('Ctrl Pts',(-64.133768380869,-31.3298763753377,0.));
#79984=CARTESIAN_POINT('Ctrl Pts',(-64.1500031332282,-31.3459097002006,
0.));
#79985=CARTESIAN_POINT('Ctrl Pts',(-64.166253899542,-31.3619910181228,0.));
#79986=CARTESIAN_POINT('Ctrl Pts',(-64.1825205366224,-31.3781202823754,
0.));
#79987=CARTESIAN_POINT('Ctrl Pts',(-64.1988029019707,-31.3942974463445,
0.));
#79988=CARTESIAN_POINT('Ctrl Pts',(-64.2151008537697,-31.410522463528,0.));
#79989=CARTESIAN_POINT('Ctrl Pts',(-64.231414250881,-31.4267952875423,0.));
#79990=CARTESIAN_POINT('Ctrl Pts',(-64.2477429528393,-31.4431158721222,
0.));
#79991=CARTESIAN_POINT('Ctrl Pts',(-64.2640868198473,-31.4594841711194,
0.));
#79992=CARTESIAN_POINT('Ctrl Pts',(-64.2804457127671,-31.4759001384941,
0.));
#79993=CARTESIAN_POINT('Ctrl Pts',(-64.2968194931158,-31.4923637283132,
0.));
#79994=CARTESIAN_POINT('Ctrl Pts',(-64.3132080230637,-31.5088748947582,
0.));
#79995=CARTESIAN_POINT('Ctrl Pts',(-64.3296111654283,-31.5254335921245,
0.));
#79996=CARTESIAN_POINT('Ctrl Pts',(-64.3460287836687,-31.5420397748191,
0.));
#79997=CARTESIAN_POINT('Ctrl Pts',(-64.3624607418768,-31.5586933973515,
0.));
#79998=CARTESIAN_POINT('Ctrl Pts',(-64.3789069047733,-31.5753944143336,
0.));
#79999=CARTESIAN_POINT('Ctrl Pts',(-64.3953671377046,-31.5921427804865,
0.));
#80000=CARTESIAN_POINT('Ctrl Pts',(-64.4118413066378,-31.6089384506395,
0.));
#80001=CARTESIAN_POINT('Ctrl Pts',(-64.4283292781565,-31.6257813797287,
0.));
#80002=CARTESIAN_POINT('Ctrl Pts',(-64.4448309194525,-31.6426715227878,
0.));
#80003=CARTESIAN_POINT('Ctrl Pts',(-64.4613460983214,-31.6596088349482,
0.));
#80004=CARTESIAN_POINT('Ctrl Pts',(-64.4778746831614,-31.6765932714464,
0.));
#80005=CARTESIAN_POINT('Ctrl Pts',(-64.4944165429675,-31.6936247876229,
0.));
#80006=CARTESIAN_POINT('Ctrl Pts',(-64.510971547327,-31.7107033389201,0.));
#80007=CARTESIAN_POINT('Ctrl Pts',(-64.5275395664124,-31.7278288808731,
0.));
#80008=CARTESIAN_POINT('Ctrl Pts',(-64.544120470977,-31.7450013691112,0.));
#80009=CARTESIAN_POINT('Ctrl Pts',(-64.5607141323521,-31.7622207593634,
0.));
#80010=CARTESIAN_POINT('Ctrl Pts',(-64.5773204224429,-31.7794870074583,
0.));
#80011=CARTESIAN_POINT('Ctrl Pts',(-64.5939392137235,-31.7968000693218,
0.));
#80012=CARTESIAN_POINT('Ctrl Pts',(-64.6105703792312,-31.8141599009684,
0.));
#80013=CARTESIAN_POINT('Ctrl Pts',(-64.6272137925627,-31.8315664585026,
0.));
#80014=CARTESIAN_POINT('Ctrl Pts',(-64.6438693278714,-31.8490196981248,
0.));
#80015=CARTESIAN_POINT('Ctrl Pts',(-64.6605368598629,-31.866519576131,0.));
#80016=CARTESIAN_POINT('Ctrl Pts',(-64.6772162637907,-31.8840660489107,
0.));
#80017=CARTESIAN_POINT('Ctrl Pts',(-64.6939074154498,-31.9016590729374,
0.));
#80018=CARTESIAN_POINT('Ctrl Pts',(-64.7106101911732,-31.9192986047706,
0.));
#80019=CARTESIAN_POINT('Ctrl Pts',(-64.7273244678297,-31.9369846010615,
0.));
#80020=CARTESIAN_POINT('Ctrl Pts',(-64.7440501228202,-31.9547170185534,
0.));
#80021=CARTESIAN_POINT('Ctrl Pts',(-64.7607870340735,-31.9724958140789,
0.));
#80022=CARTESIAN_POINT('Ctrl Pts',(-64.77753508004,-31.990320944552,0.));
#80023=CARTESIAN_POINT('Ctrl Pts',(-64.7942941396881,-32.0081923669677,
0.));
#80024=CARTESIAN_POINT('Ctrl Pts',(-64.8110640925021,-32.0261100384092,
0.));
#80025=CARTESIAN_POINT('Ctrl Pts',(-64.8278448184786,-32.0440739160477,
0.));
#80026=CARTESIAN_POINT('Ctrl Pts',(-64.8446361981234,-32.0620839571408,
0.));
#80027=CARTESIAN_POINT('Ctrl Pts',(-64.861438112445,-32.0801401190241,0.));
#80028=CARTESIAN_POINT('Ctrl Pts',(-64.878250442952,-32.0982423591108,0.));
#80029=CARTESIAN_POINT('Ctrl Pts',(-64.8950730716493,-32.1163906348979,
0.));
#80030=CARTESIAN_POINT('Ctrl Pts',(-64.9119058810362,-32.1345849039671,
0.));
#80031=CARTESIAN_POINT('Ctrl Pts',(-64.9287487541018,-32.1528251239832,
0.));
#80032=CARTESIAN_POINT('Ctrl Pts',(-64.9456015743203,-32.171111252686,0.));
#80033=CARTESIAN_POINT('Ctrl Pts',(-64.9624642256477,-32.1894432478889,
0.));
#80034=CARTESIAN_POINT('Ctrl Pts',(-64.9793365925194,-32.2078210674857,
0.));
#80035=CARTESIAN_POINT('Ctrl Pts',(-64.996218559847,-32.2262446694516,0.));
#80036=CARTESIAN_POINT('Ctrl Pts',(-65.0131100130155,-32.244714011842,0.));
#80037=CARTESIAN_POINT('Ctrl Pts',(-65.0300108378786,-32.2632290527855,
0.));
#80038=CARTESIAN_POINT('Ctrl Pts',(-65.0469209207548,-32.2817897504799,
0.));
#80039=CARTESIAN_POINT('Ctrl Pts',(-65.0638401484245,-32.3003960632,0.));
#80040=CARTESIAN_POINT('Ctrl Pts',(-65.0807684081278,-32.3190479492985,
0.));
#80041=CARTESIAN_POINT('Ctrl Pts',(-65.097705587561,-32.3377453672052,0.));
#80042=CARTESIAN_POINT('Ctrl Pts',(-65.1146515748723,-32.3564882754212,
0.));
#80043=CARTESIAN_POINT('Ctrl Pts',(-65.1316062586586,-32.3752766325135,
0.));
#80044=CARTESIAN_POINT('Ctrl Pts',(-65.1485695279628,-32.3941103971218,
0.));
#80045=CARTESIAN_POINT('Ctrl Pts',(-65.165541272272,-32.4129895279612,0.));
#80046=CARTESIAN_POINT('Ctrl Pts',(-65.182521381514,-32.4319139838212,0.));
#80047=CARTESIAN_POINT('Ctrl Pts',(-65.1995097460546,-32.4508837235613,
0.));
#80048=CARTESIAN_POINT('Ctrl Pts',(-65.2165062566936,-32.4698987061037,
0.));
#80049=CARTESIAN_POINT('Ctrl Pts',(-65.2335108046625,-32.4889588904397,
0.));
#80050=CARTESIAN_POINT('Ctrl Pts',(-65.2505232816215,-32.508064235633,0.));
#80051=CARTESIAN_POINT('Ctrl Pts',(-65.2675435796558,-32.5272147008191,
0.));
#80052=CARTESIAN_POINT('Ctrl Pts',(-65.2845715912717,-32.5464102452013,
0.));
#80053=CARTESIAN_POINT('Ctrl Pts',(-65.3016072093907,-32.565650828042,0.));
#80054=CARTESIAN_POINT('Ctrl Pts',(-65.3186503273498,-32.5849364086679,
0.));
#80055=CARTESIAN_POINT('Ctrl Pts',(-65.3357008389004,-32.6042669464752,
0.));
#80056=CARTESIAN_POINT('Ctrl Pts',(-65.3527586382082,-32.6236424009302,
0.));
#80057=CARTESIAN_POINT('Ctrl Pts',(-65.3698236198511,-32.6430627315673,
0.));
#80058=CARTESIAN_POINT('Ctrl Pts',(-65.3868956788178,-32.6625278979807,
0.));
#80059=CARTESIAN_POINT('Ctrl Pts',(-65.4039747105033,-32.6820378598262,
0.));
#80060=CARTESIAN_POINT('Ctrl Pts',(-65.4210606107029,-32.7015925768261,
0.));
#80061=CARTESIAN_POINT('Ctrl Pts',(-65.4381532756062,-32.7211920087682,
0.));
#80062=CARTESIAN_POINT('Ctrl Pts',(-65.4552526017907,-32.7408361155038,
0.));
#80063=CARTESIAN_POINT('Ctrl Pts',(-65.4723584862129,-32.7605248569382,
0.));
#80064=CARTESIAN_POINT('Ctrl Pts',(-65.4894708262071,-32.7802581930293,
0.));
#80065=CARTESIAN_POINT('Ctrl Pts',(-65.5065895194938,-32.8000360837981,
0.));
#80066=CARTESIAN_POINT('Ctrl Pts',(-65.5237144641864,-32.8198584893319,
0.));
#80067=CARTESIAN_POINT('Ctrl Pts',(-65.5408455587963,-32.8397253697864,
0.));
#80068=CARTESIAN_POINT('Ctrl Pts',(-65.5579827022412,-32.8596366853826,
0.));
#80069=CARTESIAN_POINT('Ctrl Pts',(-65.575125793846,-32.8795923964022,0.));
#80070=CARTESIAN_POINT('Ctrl Pts',(-65.5922747333181,-32.899592463189,0.));
#80071=CARTESIAN_POINT('Ctrl Pts',(-65.6094294207267,-32.9196368461457,
0.));
#80072=CARTESIAN_POINT('Ctrl Pts',(-65.6265897564782,-32.9397255057273,
0.));
#80073=CARTESIAN_POINT('Ctrl Pts',(-65.6437556412956,-32.9598584024318,
0.));
#80074=CARTESIAN_POINT('Ctrl Pts',(-65.6609269761902,-32.9800354967847,
0.));
#80075=CARTESIAN_POINT('Ctrl Pts',(-65.6781036625041,-33.0002567493581,
0.));
#80076=CARTESIAN_POINT('Ctrl Pts',(-65.6952856019542,-33.0205221207877,
0.));
#80077=CARTESIAN_POINT('Ctrl Pts',(-65.7124726966805,-33.0408315717874,
0.));
#80078=CARTESIAN_POINT('Ctrl Pts',(-65.729664849282,-33.061185063158,0.));
#80079=CARTESIAN_POINT('Ctrl Pts',(-65.7468619628808,-33.0815825557976,
0.));
#80080=CARTESIAN_POINT('Ctrl Pts',(-65.7640639410653,-33.102024010688,0.));
#80081=CARTESIAN_POINT('Ctrl Pts',(-65.7812706877691,-33.1225093888668,
0.));
#80082=CARTESIAN_POINT('Ctrl Pts',(-65.7984821071621,-33.1430386513975,
0.));
#80083=CARTESIAN_POINT('Ctrl Pts',(-65.8156981035504,-33.16361175934,0.));
#80084=CARTESIAN_POINT('Ctrl Pts',(-65.8329185812379,-33.1842286737053,
0.));
#80085=CARTESIAN_POINT('Ctrl Pts',(-65.8501434445174,-33.2048893554496,
0.));
#80086=CARTESIAN_POINT('Ctrl Pts',(-65.8673725979591,-33.2255937655656,
0.));
#80087=CARTESIAN_POINT('Ctrl Pts',(-65.8846059466382,-33.2463418651498,
0.));
#80088=CARTESIAN_POINT('Ctrl Pts',(-65.901843396389,-33.2671336154754,0.));
#80089=CARTESIAN_POINT('Ctrl Pts',(-65.9190848540422,-33.2879689780566,
0.));
#80090=CARTESIAN_POINT('Ctrl Pts',(-65.9363302276822,-33.3088479147151,
0.));
#80091=CARTESIAN_POINT('Ctrl Pts',(-65.9535794260802,-33.3297703874249,
0.));
#80092=CARTESIAN_POINT('Ctrl Pts',(-65.9708323581385,-33.3507363581579,
0.));
#80093=CARTESIAN_POINT('Ctrl Pts',(-65.9880889322822,-33.3717457887095,
0.));
#80094=CARTESIAN_POINT('Ctrl Pts',(-66.0053490559826,-33.3927986405612,
0.));
#80095=CARTESIAN_POINT('Ctrl Pts',(-66.0226126349482,-33.4138948746408,
0.));
#80096=CARTESIAN_POINT('Ctrl Pts',(-66.0398795737827,-33.4350344515128,
0.));
#80097=CARTESIAN_POINT('Ctrl Pts',(-66.0571497774484,-33.4562173318052,
0.));
#80098=CARTESIAN_POINT('Ctrl Pts',(-66.0744231525445,-33.4774434765762,
0.));
#80099=CARTESIAN_POINT('Ctrl Pts',(-66.0916996085237,-33.4987128476618,
0.));
#80100=CARTESIAN_POINT('Ctrl Pts',(-66.1089790592673,-33.5200254081212,
0.));
#80101=CARTESIAN_POINT('Ctrl Pts',(-66.1262614234579,-33.5413811223398,
0.));
#80102=CARTESIAN_POINT('Ctrl Pts',(-66.1410781873125,-33.5597240685729,
0.));
#80103=CARTESIAN_POINT('Ctrl Pts',(-66.1524393973986,-33.5738105077707,
0.));
#80104=CARTESIAN_POINT('Ctrl Pts',(-66.1603438177306,-33.5836213513974,
0.));
#80105=CARTESIAN_POINT('Ctrl Pts',(-66.1647906582409,-33.5891439876228,
0.));
#80106=CARTESIAN_POINT('Ctrl Pts',(-66.165779540567,-33.5903722664958,0.));
#80107=CARTESIAN_POINT('',(-63.0759831361898,-30.3549065457811,12.));
#80108=CARTESIAN_POINT('',(-63.0759831361898,-30.3549065457811,0.));
#80109=CARTESIAN_POINT('Ctrl Pts',(-66.165779540567,-33.5903722664958,12.));
#80110=CARTESIAN_POINT('Ctrl Pts',(-66.1647906582409,-33.5891439876228,
12.));
#80111=CARTESIAN_POINT('Ctrl Pts',(-66.1603438177306,-33.5836213513974,
12.));
#80112=CARTESIAN_POINT('Ctrl Pts',(-66.1524393973986,-33.5738105077707,
12.));
#80113=CARTESIAN_POINT('Ctrl Pts',(-66.1410781873125,-33.5597240685729,
12.));
#80114=CARTESIAN_POINT('Ctrl Pts',(-66.1262614234579,-33.5413811223398,
12.));
#80115=CARTESIAN_POINT('Ctrl Pts',(-66.1089790592673,-33.5200254081212,
12.));
#80116=CARTESIAN_POINT('Ctrl Pts',(-66.0916996085237,-33.4987128476618,
12.));
#80117=CARTESIAN_POINT('Ctrl Pts',(-66.0744231525445,-33.4774434765762,
12.));
#80118=CARTESIAN_POINT('Ctrl Pts',(-66.0571497774484,-33.4562173318052,
12.));
#80119=CARTESIAN_POINT('Ctrl Pts',(-66.0398795737827,-33.4350344515128,
12.));
#80120=CARTESIAN_POINT('Ctrl Pts',(-66.0226126349482,-33.4138948746408,
12.));
#80121=CARTESIAN_POINT('Ctrl Pts',(-66.0053490559826,-33.3927986405612,
12.));
#80122=CARTESIAN_POINT('Ctrl Pts',(-65.9880889322822,-33.3717457887095,
12.));
#80123=CARTESIAN_POINT('Ctrl Pts',(-65.9708323581385,-33.3507363581579,
12.));
#80124=CARTESIAN_POINT('Ctrl Pts',(-65.9535794260802,-33.3297703874249,
12.));
#80125=CARTESIAN_POINT('Ctrl Pts',(-65.9363302276822,-33.3088479147151,
12.));
#80126=CARTESIAN_POINT('Ctrl Pts',(-65.9190848540422,-33.2879689780566,
12.));
#80127=CARTESIAN_POINT('Ctrl Pts',(-65.901843396389,-33.2671336154754,12.));
#80128=CARTESIAN_POINT('Ctrl Pts',(-65.8846059466382,-33.2463418651498,
12.));
#80129=CARTESIAN_POINT('Ctrl Pts',(-65.8673725979591,-33.2255937655656,
12.));
#80130=CARTESIAN_POINT('Ctrl Pts',(-65.8501434445174,-33.2048893554496,
12.));
#80131=CARTESIAN_POINT('Ctrl Pts',(-65.8329185812379,-33.1842286737053,
12.));
#80132=CARTESIAN_POINT('Ctrl Pts',(-65.8156981035504,-33.16361175934,12.));
#80133=CARTESIAN_POINT('Ctrl Pts',(-65.7984821071621,-33.1430386513975,
12.));
#80134=CARTESIAN_POINT('Ctrl Pts',(-65.7812706877691,-33.1225093888668,
12.));
#80135=CARTESIAN_POINT('Ctrl Pts',(-65.7640639410653,-33.102024010688,12.));
#80136=CARTESIAN_POINT('Ctrl Pts',(-65.7468619628808,-33.0815825557976,
12.));
#80137=CARTESIAN_POINT('Ctrl Pts',(-65.729664849282,-33.061185063158,12.));
#80138=CARTESIAN_POINT('Ctrl Pts',(-65.7124726966805,-33.0408315717874,
12.));
#80139=CARTESIAN_POINT('Ctrl Pts',(-65.6952856019542,-33.0205221207877,
12.));
#80140=CARTESIAN_POINT('Ctrl Pts',(-65.6781036625041,-33.0002567493581,
12.));
#80141=CARTESIAN_POINT('Ctrl Pts',(-65.6609269761902,-32.9800354967847,
12.));
#80142=CARTESIAN_POINT('Ctrl Pts',(-65.6437556412956,-32.9598584024318,
12.));
#80143=CARTESIAN_POINT('Ctrl Pts',(-65.6265897564782,-32.9397255057273,
12.));
#80144=CARTESIAN_POINT('Ctrl Pts',(-65.6094294207267,-32.9196368461457,
12.));
#80145=CARTESIAN_POINT('Ctrl Pts',(-65.5922747333181,-32.899592463189,12.));
#80146=CARTESIAN_POINT('Ctrl Pts',(-65.575125793846,-32.8795923964022,12.));
#80147=CARTESIAN_POINT('Ctrl Pts',(-65.5579827022412,-32.8596366853826,
12.));
#80148=CARTESIAN_POINT('Ctrl Pts',(-65.5408455587963,-32.8397253697864,
12.));
#80149=CARTESIAN_POINT('Ctrl Pts',(-65.5237144641864,-32.8198584893319,
12.));
#80150=CARTESIAN_POINT('Ctrl Pts',(-65.5065895194938,-32.8000360837981,
12.));
#80151=CARTESIAN_POINT('Ctrl Pts',(-65.4894708262071,-32.7802581930293,
12.));
#80152=CARTESIAN_POINT('Ctrl Pts',(-65.4723584862129,-32.7605248569382,
12.));
#80153=CARTESIAN_POINT('Ctrl Pts',(-65.4552526017907,-32.7408361155038,
12.));
#80154=CARTESIAN_POINT('Ctrl Pts',(-65.4381532756062,-32.7211920087682,
12.));
#80155=CARTESIAN_POINT('Ctrl Pts',(-65.4210606107029,-32.7015925768261,
12.));
#80156=CARTESIAN_POINT('Ctrl Pts',(-65.4039747105033,-32.6820378598262,
12.));
#80157=CARTESIAN_POINT('Ctrl Pts',(-65.3868956788178,-32.6625278979807,
12.));
#80158=CARTESIAN_POINT('Ctrl Pts',(-65.3698236198511,-32.6430627315673,
12.));
#80159=CARTESIAN_POINT('Ctrl Pts',(-65.3527586382082,-32.6236424009302,
12.));
#80160=CARTESIAN_POINT('Ctrl Pts',(-65.3357008389004,-32.6042669464752,
12.));
#80161=CARTESIAN_POINT('Ctrl Pts',(-65.3186503273498,-32.5849364086679,
12.));
#80162=CARTESIAN_POINT('Ctrl Pts',(-65.3016072093907,-32.565650828042,12.));
#80163=CARTESIAN_POINT('Ctrl Pts',(-65.2845715912717,-32.5464102452013,
12.));
#80164=CARTESIAN_POINT('Ctrl Pts',(-65.2675435796558,-32.5272147008191,
12.));
#80165=CARTESIAN_POINT('Ctrl Pts',(-65.2505232816215,-32.508064235633,12.));
#80166=CARTESIAN_POINT('Ctrl Pts',(-65.2335108046625,-32.4889588904397,
12.));
#80167=CARTESIAN_POINT('Ctrl Pts',(-65.2165062566936,-32.4698987061037,
12.));
#80168=CARTESIAN_POINT('Ctrl Pts',(-65.1995097460546,-32.4508837235613,
12.));
#80169=CARTESIAN_POINT('Ctrl Pts',(-65.182521381514,-32.4319139838212,12.));
#80170=CARTESIAN_POINT('Ctrl Pts',(-65.165541272272,-32.4129895279612,12.));
#80171=CARTESIAN_POINT('Ctrl Pts',(-65.1485695279628,-32.3941103971218,
12.));
#80172=CARTESIAN_POINT('Ctrl Pts',(-65.1316062586586,-32.3752766325135,
12.));
#80173=CARTESIAN_POINT('Ctrl Pts',(-65.1146515748723,-32.3564882754212,
12.));
#80174=CARTESIAN_POINT('Ctrl Pts',(-65.097705587561,-32.3377453672052,12.));
#80175=CARTESIAN_POINT('Ctrl Pts',(-65.0807684081278,-32.3190479492985,
12.));
#80176=CARTESIAN_POINT('Ctrl Pts',(-65.0638401484245,-32.3003960632,12.));
#80177=CARTESIAN_POINT('Ctrl Pts',(-65.0469209207548,-32.2817897504799,
12.));
#80178=CARTESIAN_POINT('Ctrl Pts',(-65.0300108378786,-32.2632290527855,
12.));
#80179=CARTESIAN_POINT('Ctrl Pts',(-65.0131100130155,-32.244714011842,12.));
#80180=CARTESIAN_POINT('Ctrl Pts',(-64.996218559847,-32.2262446694516,12.));
#80181=CARTESIAN_POINT('Ctrl Pts',(-64.9793365925194,-32.2078210674857,
12.));
#80182=CARTESIAN_POINT('Ctrl Pts',(-64.9624642256477,-32.1894432478889,
12.));
#80183=CARTESIAN_POINT('Ctrl Pts',(-64.9456015743203,-32.171111252686,12.));
#80184=CARTESIAN_POINT('Ctrl Pts',(-64.9287487541018,-32.1528251239832,
12.));
#80185=CARTESIAN_POINT('Ctrl Pts',(-64.9119058810362,-32.1345849039671,
12.));
#80186=CARTESIAN_POINT('Ctrl Pts',(-64.8950730716493,-32.1163906348979,
12.));
#80187=CARTESIAN_POINT('Ctrl Pts',(-64.878250442952,-32.0982423591108,12.));
#80188=CARTESIAN_POINT('Ctrl Pts',(-64.861438112445,-32.0801401190241,12.));
#80189=CARTESIAN_POINT('Ctrl Pts',(-64.8446361981234,-32.0620839571408,
12.));
#80190=CARTESIAN_POINT('Ctrl Pts',(-64.8278448184786,-32.0440739160477,
12.));
#80191=CARTESIAN_POINT('Ctrl Pts',(-64.8110640925021,-32.0261100384092,
12.));
#80192=CARTESIAN_POINT('Ctrl Pts',(-64.7942941396881,-32.0081923669677,
12.));
#80193=CARTESIAN_POINT('Ctrl Pts',(-64.77753508004,-31.990320944552,12.));
#80194=CARTESIAN_POINT('Ctrl Pts',(-64.7607870340735,-31.9724958140789,
12.));
#80195=CARTESIAN_POINT('Ctrl Pts',(-64.7440501228202,-31.9547170185534,
12.));
#80196=CARTESIAN_POINT('Ctrl Pts',(-64.7273244678297,-31.9369846010615,
12.));
#80197=CARTESIAN_POINT('Ctrl Pts',(-64.7106101911732,-31.9192986047706,
12.));
#80198=CARTESIAN_POINT('Ctrl Pts',(-64.6939074154498,-31.9016590729374,
12.));
#80199=CARTESIAN_POINT('Ctrl Pts',(-64.6772162637907,-31.8840660489107,
12.));
#80200=CARTESIAN_POINT('Ctrl Pts',(-64.6605368598629,-31.866519576131,12.));
#80201=CARTESIAN_POINT('Ctrl Pts',(-64.6438693278714,-31.8490196981248,
12.));
#80202=CARTESIAN_POINT('Ctrl Pts',(-64.6272137925627,-31.8315664585026,
12.));
#80203=CARTESIAN_POINT('Ctrl Pts',(-64.6105703792312,-31.8141599009684,
12.));
#80204=CARTESIAN_POINT('Ctrl Pts',(-64.5939392137235,-31.7968000693218,
12.));
#80205=CARTESIAN_POINT('Ctrl Pts',(-64.5773204224429,-31.7794870074583,
12.));
#80206=CARTESIAN_POINT('Ctrl Pts',(-64.5607141323521,-31.7622207593634,
12.));
#80207=CARTESIAN_POINT('Ctrl Pts',(-64.544120470977,-31.7450013691112,12.));
#80208=CARTESIAN_POINT('Ctrl Pts',(-64.5275395664124,-31.7278288808731,
12.));
#80209=CARTESIAN_POINT('Ctrl Pts',(-64.510971547327,-31.7107033389201,12.));
#80210=CARTESIAN_POINT('Ctrl Pts',(-64.4944165429675,-31.6936247876229,
12.));
#80211=CARTESIAN_POINT('Ctrl Pts',(-64.4778746831614,-31.6765932714464,
12.));
#80212=CARTESIAN_POINT('Ctrl Pts',(-64.4613460983214,-31.6596088349482,
12.));
#80213=CARTESIAN_POINT('Ctrl Pts',(-64.4448309194525,-31.6426715227878,
12.));
#80214=CARTESIAN_POINT('Ctrl Pts',(-64.4283292781565,-31.6257813797287,
12.));
#80215=CARTESIAN_POINT('Ctrl Pts',(-64.4118413066378,-31.6089384506395,
12.));
#80216=CARTESIAN_POINT('Ctrl Pts',(-64.3953671377046,-31.5921427804865,
12.));
#80217=CARTESIAN_POINT('Ctrl Pts',(-64.3789069047733,-31.5753944143336,
12.));
#80218=CARTESIAN_POINT('Ctrl Pts',(-64.3624607418768,-31.5586933973515,
12.));
#80219=CARTESIAN_POINT('Ctrl Pts',(-64.3460287836687,-31.5420397748191,
12.));
#80220=CARTESIAN_POINT('Ctrl Pts',(-64.3296111654283,-31.5254335921245,
12.));
#80221=CARTESIAN_POINT('Ctrl Pts',(-64.3132080230637,-31.5088748947582,
12.));
#80222=CARTESIAN_POINT('Ctrl Pts',(-64.2968194931158,-31.4923637283132,
12.));
#80223=CARTESIAN_POINT('Ctrl Pts',(-64.2804457127671,-31.4759001384941,
12.));
#80224=CARTESIAN_POINT('Ctrl Pts',(-64.2640868198473,-31.4594841711194,
12.));
#80225=CARTESIAN_POINT('Ctrl Pts',(-64.2477429528393,-31.4431158721222,
12.));
#80226=CARTESIAN_POINT('Ctrl Pts',(-64.231414250881,-31.4267952875423,12.));
#80227=CARTESIAN_POINT('Ctrl Pts',(-64.2151008537697,-31.410522463528,12.));
#80228=CARTESIAN_POINT('Ctrl Pts',(-64.1988029019707,-31.3942974463445,
12.));
#80229=CARTESIAN_POINT('Ctrl Pts',(-64.1825205366224,-31.3781202823754,
12.));
#80230=CARTESIAN_POINT('Ctrl Pts',(-64.166253899542,-31.3619910181228,12.));
#80231=CARTESIAN_POINT('Ctrl Pts',(-64.1500031332282,-31.3459097002006,
12.));
#80232=CARTESIAN_POINT('Ctrl Pts',(-64.133768380869,-31.3298763753377,12.));
#80233=CARTESIAN_POINT('Ctrl Pts',(-64.117549786349,-31.3138910903859,12.));
#80234=CARTESIAN_POINT('Ctrl Pts',(-64.1013474942556,-31.2979538923214,
12.));
#80235=CARTESIAN_POINT('Ctrl Pts',(-64.0851616498852,-31.2820648282447,
12.));
#80236=CARTESIAN_POINT('Ctrl Pts',(-64.0689923992461,-31.2662239453728,
12.));
#80237=CARTESIAN_POINT('Ctrl Pts',(-64.0528398890657,-31.2504312910451,
12.));
#80238=CARTESIAN_POINT('Ctrl Pts',(-64.0367042667984,-31.2346869127297,
12.));
#80239=CARTESIAN_POINT('Ctrl Pts',(-64.02058568063,-31.2189908580245,12.));
#80240=CARTESIAN_POINT('Ctrl Pts',(-64.0044842794831,-31.2033431746558,
12.));
#80241=CARTESIAN_POINT('Ctrl Pts',(-63.9884002130211,-31.1877439104717,
12.));
#80242=CARTESIAN_POINT('Ctrl Pts',(-63.9723336316551,-31.1721931134487,
12.));
#80243=CARTESIAN_POINT('Ctrl Pts',(-63.9562846865567,-31.1566908316992,
12.));
#80244=CARTESIAN_POINT('Ctrl Pts',(-63.940253529665,-31.1412371134727,12.));
#80245=CARTESIAN_POINT('Ctrl Pts',(-63.9242403136955,-31.1258320071545,
12.));
#80246=CARTESIAN_POINT('Ctrl Pts',(-63.9082451921448,-31.1104755612607,
12.));
#80247=CARTESIAN_POINT('Ctrl Pts',(-63.8922683192964,-31.0951678244455,
12.));
#80248=CARTESIAN_POINT('Ctrl Pts',(-63.8763098502237,-31.0799088455041,
12.));
#80249=CARTESIAN_POINT('Ctrl Pts',(-63.8603699407922,-31.0646986733723,
12.));
#80250=CARTESIAN_POINT('Ctrl Pts',(-63.8444487476611,-31.0495373571215,
12.));
#80251=CARTESIAN_POINT('Ctrl Pts',(-63.8285464282846,-31.0344249459538,
12.));
#80252=CARTESIAN_POINT('Ctrl Pts',(-63.8126631409364,-31.0193614892171,
12.));
#80253=CARTESIAN_POINT('Ctrl Pts',(-63.796799044728,-31.0043470364108,12.));
#80254=CARTESIAN_POINT('Ctrl Pts',(-63.7809542996264,-30.989381637191,12.));
#80255=CARTESIAN_POINT('Ctrl Pts',(-63.7651290664733,-30.9744653413689,
12.));
#80256=CARTESIAN_POINT('Ctrl Pts',(-63.749323506987,-30.9595981989103,12.));
#80257=CARTESIAN_POINT('Ctrl Pts',(-63.7335377837441,-30.9447802599355,
12.));
#80258=CARTESIAN_POINT('Ctrl Pts',(-63.7177720601609,-30.9300115747115,
12.));
#80259=CARTESIAN_POINT('Ctrl Pts',(-63.7020265004792,-30.9152921936465,
12.));
#80260=CARTESIAN_POINT('Ctrl Pts',(-63.6863012697328,-30.900622167269,12.));
#80261=CARTESIAN_POINT('Ctrl Pts',(-63.6705965337971,-30.8860015462475,
12.));
#80262=CARTESIAN_POINT('Ctrl Pts',(-63.6549124594666,-30.8714303814194,
12.));
#80263=CARTESIAN_POINT('Ctrl Pts',(-63.6392492145233,-30.8569087238131,
12.));
#80264=CARTESIAN_POINT('Ctrl Pts',(-63.6236069678055,-30.8424366246671,
12.));
#80265=CARTESIAN_POINT('Ctrl Pts',(-63.6079858892771,-30.8280141354459,
12.));
#80266=CARTESIAN_POINT('Ctrl Pts',(-63.5923861498987,-30.813641307801,12.));
#80267=CARTESIAN_POINT('Ctrl Pts',(-63.5768079214881,-30.7993181935271,
12.));
#80268=CARTESIAN_POINT('Ctrl Pts',(-63.5612513766,-30.7850448445205,12.));
#80269=CARTESIAN_POINT('Ctrl Pts',(-63.5457166883537,-30.7708213127159,
12.));
#80270=CARTESIAN_POINT('Ctrl Pts',(-63.5302040304142,-30.7566476500757,
12.));
#80271=CARTESIAN_POINT('Ctrl Pts',(-63.5147135773894,-30.7425239087281,
12.));
#80272=CARTESIAN_POINT('Ctrl Pts',(-63.4992455051795,-30.7284501410822,
12.));
#80273=CARTESIAN_POINT('Ctrl Pts',(-63.4837999912771,-30.7144263999265,
12.));
#80274=CARTESIAN_POINT('Ctrl Pts',(-63.4683772152529,-30.7004527385821,
12.));
#80275=CARTESIAN_POINT('Ctrl Pts',(-63.4529773584249,-30.6865292107929,
12.));
#80276=CARTESIAN_POINT('Ctrl Pts',(-63.4376006029604,-30.6726558704315,
12.));
#80277=CARTESIAN_POINT('Ctrl Pts',(-63.4222471311239,-30.6588327712483,
12.));
#80278=CARTESIAN_POINT('Ctrl Pts',(-63.4069171245066,-30.6450599666121,
12.));
#80279=CARTESIAN_POINT('Ctrl Pts',(-63.3916107631376,-30.6313375092062,
12.));
#80280=CARTESIAN_POINT('Ctrl Pts',(-63.3763282271796,-30.6176654515967,
12.));
#80281=CARTESIAN_POINT('Ctrl Pts',(-63.3610696989577,-30.6040438469078,
12.));
#80282=CARTESIAN_POINT('Ctrl Pts',(-63.3458353646154,-30.5904727493711,
12.));
#80283=CARTESIAN_POINT('Ctrl Pts',(-63.3306254165126,-30.5769522151164,
12.));
#80284=CARTESIAN_POINT('Ctrl Pts',(-63.3154400534397,-30.563482302238,12.));
#80285=CARTESIAN_POINT('Ctrl Pts',(-63.3002794756086,-30.5500630691359,
12.));
#80286=CARTESIAN_POINT('Ctrl Pts',(-63.2851438802473,-30.5366945730508,
12.));
#80287=CARTESIAN_POINT('Ctrl Pts',(-63.2700334577639,-30.5233768687865,
12.));
#80288=CARTESIAN_POINT('Ctrl Pts',(-63.2549483856215,-30.5101100066659,
12.));
#80289=CARTESIAN_POINT('Ctrl Pts',(-63.2398888342545,-30.4968940344998,
12.));
#80290=CARTESIAN_POINT('Ctrl Pts',(-63.2248549788221,-30.4837290014989,
12.));
#80291=CARTESIAN_POINT('Ctrl Pts',(-63.2098470086636,-30.470614961416,12.));
#80292=CARTESIAN_POINT('Ctrl Pts',(-63.1948651386942,-30.4575519763337,
12.));
#80293=CARTESIAN_POINT('Ctrl Pts',(-63.179909617189,-30.444540119238,12.));
#80294=CARTESIAN_POINT('Ctrl Pts',(-63.164980701691,-30.4315794659731,12.));
#80295=CARTESIAN_POINT('Ctrl Pts',(-63.1500786361459,-30.418670087563,12.));
#80296=CARTESIAN_POINT('Ctrl Pts',(-63.135203629844,-30.4058120432228,12.));
#80297=CARTESIAN_POINT('Ctrl Pts',(-63.1203558300657,-30.3930053710484,
12.));
#80298=CARTESIAN_POINT('Ctrl Pts',(-63.105535320226,-30.3802500880403,12.));
#80299=CARTESIAN_POINT('Ctrl Pts',(-63.0937007763471,-30.3700869762507,
12.));
#80300=CARTESIAN_POINT('Ctrl Pts',(-63.0848371718048,-30.3624877680651,
12.));
#80301=CARTESIAN_POINT('Ctrl Pts',(-63.078933570069,-30.3574319069329,12.));
#80302=CARTESIAN_POINT('Ctrl Pts',(-63.0759831361898,-30.3549065457811,
12.));
#80303=CARTESIAN_POINT('Ctrl Pts',(-65.4667541478385,-34.933187552314,-5.55111512312578E-16));
#80304=CARTESIAN_POINT('Ctrl Pts',(-65.4667541478385,-34.933187552314,4.));
#80305=CARTESIAN_POINT('Ctrl Pts',(-65.4667541478385,-34.933187552314,8.));
#80306=CARTESIAN_POINT('Ctrl Pts',(-65.4667541478385,-34.933187552314,12.));
#80307=CARTESIAN_POINT('Ctrl Pts',(-65.5763902570748,-34.940541458921,-5.55111512312578E-16));
#80308=CARTESIAN_POINT('Ctrl Pts',(-65.5763902570748,-34.940541458921,4.));
#80309=CARTESIAN_POINT('Ctrl Pts',(-65.5763902570748,-34.940541458921,8.));
#80310=CARTESIAN_POINT('Ctrl Pts',(-65.5763902570748,-34.940541458921,12.));
#80311=CARTESIAN_POINT('Ctrl Pts',(-65.7720412680588,-34.8876896346299,
-5.55111512312578E-16));
#80312=CARTESIAN_POINT('Ctrl Pts',(-65.7720412680588,-34.8876896346299,
4.00000000000001));
#80313=CARTESIAN_POINT('Ctrl Pts',(-65.7720412680588,-34.8876896346299,
7.99999999999999));
#80314=CARTESIAN_POINT('Ctrl Pts',(-65.7720412680588,-34.8876896346299,
12.));
#80315=CARTESIAN_POINT('Ctrl Pts',(-65.9044372006542,-34.7399186668304,
-5.55111512312578E-16));
#80316=CARTESIAN_POINT('Ctrl Pts',(-65.9044372006542,-34.7399186668304,
3.99999999999999));
#80317=CARTESIAN_POINT('Ctrl Pts',(-65.9044372006542,-34.7399186668304,
8.00000000000001));
#80318=CARTESIAN_POINT('Ctrl Pts',(-65.9044372006542,-34.7399186668304,
12.));
#80319=CARTESIAN_POINT('Ctrl Pts',(-65.9427857825584,-34.6669728017261,
-5.55111512312578E-16));
#80320=CARTESIAN_POINT('Ctrl Pts',(-65.9427857825584,-34.6669728017261,
4.));
#80321=CARTESIAN_POINT('Ctrl Pts',(-65.9427857825584,-34.6669728017261,
8.));
#80322=CARTESIAN_POINT('Ctrl Pts',(-65.9427857825584,-34.6669728017261,
12.));
#80323=CARTESIAN_POINT('',(-65.4667541478385,-34.933187552314,0.));
#80324=CARTESIAN_POINT('',(-65.9427857825584,-34.6669728017261,2.77555756156289E-16));
#80325=CARTESIAN_POINT('Ctrl Pts',(-65.4667541478385,-34.933187552314,8.50995567916391E-16));
#80326=CARTESIAN_POINT('Ctrl Pts',(-65.5763902570748,-34.940541458921,8.50995567916389E-16));
#80327=CARTESIAN_POINT('Ctrl Pts',(-65.6881908347799,-34.910340416469,8.50995567916392E-16));
#80328=CARTESIAN_POINT('Ctrl Pts',(-65.7793366930113,-34.8491453679733,
8.50995567916391E-16));
#80329=CARTESIAN_POINT('Ctrl Pts',(-65.8476960866847,-34.8032490816016,
8.50995567916391E-16));
#80330=CARTESIAN_POINT('Ctrl Pts',(-65.9044372006542,-34.7399186668304,
8.50995567916389E-16));
#80331=CARTESIAN_POINT('Ctrl Pts',(-65.9427857825584,-34.6669728017261,
8.50995567916391E-16));
#80332=CARTESIAN_POINT('',(-65.9427857825584,-34.6669728017261,12.));
#80333=CARTESIAN_POINT('Ctrl Pts',(-65.9427857825584,-34.6669728017261,
-5.55111512312578E-16));
#80334=CARTESIAN_POINT('Ctrl Pts',(-65.9427857825584,-34.6669728017261,
4.));
#80335=CARTESIAN_POINT('Ctrl Pts',(-65.9427857825584,-34.6669728017261,
8.));
#80336=CARTESIAN_POINT('Ctrl Pts',(-65.9427857825584,-34.6669728017261,
12.));
#80337=CARTESIAN_POINT('',(-65.4667541478385,-34.933187552314,12.));
#80338=CARTESIAN_POINT('Ctrl Pts',(-65.9427857825584,-34.6669728017261,
12.));
#80339=CARTESIAN_POINT('Ctrl Pts',(-65.9044372006542,-34.7399186668304,
12.));
#80340=CARTESIAN_POINT('Ctrl Pts',(-65.8476960866847,-34.8032490816016,
12.));
#80341=CARTESIAN_POINT('Ctrl Pts',(-65.7793366930113,-34.8491453679733,
12.));
#80342=CARTESIAN_POINT('Ctrl Pts',(-65.68819083478,-34.910340416469,12.));
#80343=CARTESIAN_POINT('Ctrl Pts',(-65.5763902570748,-34.940541458921,12.));
#80344=CARTESIAN_POINT('Ctrl Pts',(-65.4667541478385,-34.933187552314,12.));
#80345=CARTESIAN_POINT('Ctrl Pts',(-65.4667541478385,-34.933187552314,12.));
#80346=CARTESIAN_POINT('Ctrl Pts',(-65.4667541478385,-34.933187552314,8.));
#80347=CARTESIAN_POINT('Ctrl Pts',(-65.4667541478385,-34.933187552314,4.));
#80348=CARTESIAN_POINT('Ctrl Pts',(-65.4667541478385,-34.933187552314,-5.55111512312578E-16));
#80349=CARTESIAN_POINT('Origin',(-3.32444647725448E-10,-1.73171632017259E-10,
0.));
#80350=CARTESIAN_POINT('Origin',(-3.32444647725448E-10,-1.73171632017259E-10,
12.));
#80351=CARTESIAN_POINT('Origin',(-3.32444647725448E-10,-1.73171632017259E-10,
0.));
#80352=CARTESIAN_POINT('Ctrl Pts',(-68.9436475237602,-28.2316040302268,
0.));
#80353=CARTESIAN_POINT('Ctrl Pts',(-68.9436475237602,-28.2316040302268,
4.));
#80354=CARTESIAN_POINT('Ctrl Pts',(-68.9436475237602,-28.2316040302268,
8.));
#80355=CARTESIAN_POINT('Ctrl Pts',(-68.9436475237602,-28.2316040302268,
12.));
#80356=CARTESIAN_POINT('Ctrl Pts',(-68.9852872321829,-28.1299168084375,
0.));
#80357=CARTESIAN_POINT('Ctrl Pts',(-68.9852872321829,-28.1299168084375,
4.));
#80358=CARTESIAN_POINT('Ctrl Pts',(-68.9852872321829,-28.1299168084375,
8.));
#80359=CARTESIAN_POINT('Ctrl Pts',(-68.9852872321829,-28.1299168084375,
12.));
#80360=CARTESIAN_POINT('Ctrl Pts',(-68.9970049015576,-27.9275918177424,
0.));
#80361=CARTESIAN_POINT('Ctrl Pts',(-68.9970049015576,-27.9275918177424,
4.));
#80362=CARTESIAN_POINT('Ctrl Pts',(-68.9970049015576,-27.9275918177424,
8.));
#80363=CARTESIAN_POINT('Ctrl Pts',(-68.9970049015576,-27.9275918177424,
12.));
#80364=CARTESIAN_POINT('Ctrl Pts',(-68.8986722313985,-27.7552674476211,
0.));
#80365=CARTESIAN_POINT('Ctrl Pts',(-68.8986722313985,-27.7552674476211,
4.));
#80366=CARTESIAN_POINT('Ctrl Pts',(-68.8986722313985,-27.7552674476211,
8.));
#80367=CARTESIAN_POINT('Ctrl Pts',(-68.8986722313985,-27.7552674476211,
12.));
#80368=CARTESIAN_POINT('Ctrl Pts',(-68.8415926174766,-27.6958230984747,
0.));
#80369=CARTESIAN_POINT('Ctrl Pts',(-68.8415926174766,-27.6958230984747,
4.));
#80370=CARTESIAN_POINT('Ctrl Pts',(-68.8415926174766,-27.6958230984747,
8.));
#80371=CARTESIAN_POINT('Ctrl Pts',(-68.8415926174766,-27.6958230984747,
12.));
#80372=CARTESIAN_POINT('',(-68.9436475237602,-28.2316040302268,0.));
#80373=CARTESIAN_POINT('',(-68.8415926174765,-27.6958230984748,0.));
#80374=CARTESIAN_POINT('Ctrl Pts',(-68.9436475237602,-28.2316040302268,
1.8809784878858E-35));
#80375=CARTESIAN_POINT('Ctrl Pts',(-68.9852872321829,-28.1299168084375,
1.88097848788579E-35));
#80376=CARTESIAN_POINT('Ctrl Pts',(-68.9919830432542,-28.0143025280403,
1.8809784878858E-35));
#80377=CARTESIAN_POINT('Ctrl Pts',(-68.9627440495797,-27.9084843686468,
1.8809784878858E-35));
#80378=CARTESIAN_POINT('Ctrl Pts',(-68.9408148043239,-27.8291207491017,
1.8809784878858E-35));
#80379=CARTESIAN_POINT('Ctrl Pts',(-68.8986722313985,-27.7552674476211,
1.88097848788579E-35));
#80380=CARTESIAN_POINT('Ctrl Pts',(-68.8415926174766,-27.6958230984747,
1.8809784878858E-35));
#80381=CARTESIAN_POINT('',(-68.8415926174765,-27.6958230984748,12.));
#80382=CARTESIAN_POINT('Ctrl Pts',(-68.8415926174766,-27.6958230984747,
0.));
#80383=CARTESIAN_POINT('Ctrl Pts',(-68.8415926174766,-27.6958230984747,
4.));
#80384=CARTESIAN_POINT('Ctrl Pts',(-68.8415926174766,-27.6958230984747,
8.));
#80385=CARTESIAN_POINT('Ctrl Pts',(-68.8415926174766,-27.6958230984747,
12.));
#80386=CARTESIAN_POINT('',(-68.9436475237602,-28.2316040302268,12.));
#80387=CARTESIAN_POINT('Ctrl Pts',(-68.8415926174766,-27.6958230984747,
12.));
#80388=CARTESIAN_POINT('Ctrl Pts',(-68.8986722313985,-27.7552674476211,
12.));
#80389=CARTESIAN_POINT('Ctrl Pts',(-68.9408148043239,-27.8291207491017,
12.));
#80390=CARTESIAN_POINT('Ctrl Pts',(-68.9627440495797,-27.9084843686468,
12.));
#80391=CARTESIAN_POINT('Ctrl Pts',(-68.9919830432542,-28.0143025280403,
12.));
#80392=CARTESIAN_POINT('Ctrl Pts',(-68.9852872321829,-28.1299168084375,
12.));
#80393=CARTESIAN_POINT('Ctrl Pts',(-68.9436475237602,-28.2316040302268,
12.));
#80394=CARTESIAN_POINT('Ctrl Pts',(-68.9436475237602,-28.2316040302268,
12.));
#80395=CARTESIAN_POINT('Ctrl Pts',(-68.9436475237602,-28.2316040302268,
8.));
#80396=CARTESIAN_POINT('Ctrl Pts',(-68.9436475237602,-28.2316040302268,
4.));
#80397=CARTESIAN_POINT('Ctrl Pts',(-68.9436475237602,-28.2316040302268,
0.));
#80398=CARTESIAN_POINT('Ctrl Pts',(-65.4815644032299,-24.7419628022042,
0.));
#80399=CARTESIAN_POINT('Ctrl Pts',(-65.4815644032299,-24.7419628022042,
12.));
#80400=CARTESIAN_POINT('Ctrl Pts',(-65.4847237095443,-24.7442214063382,
0.));
#80401=CARTESIAN_POINT('Ctrl Pts',(-65.4847237095443,-24.7442214063382,
12.));
#80402=CARTESIAN_POINT('Ctrl Pts',(-65.4910454936254,-24.7487434955982,
0.));
#80403=CARTESIAN_POINT('Ctrl Pts',(-65.4910454936254,-24.7487434955982,
12.));
#80404=CARTESIAN_POINT('Ctrl Pts',(-65.5005376841101,-24.7555412724651,
0.));
#80405=CARTESIAN_POINT('Ctrl Pts',(-65.5005376841101,-24.7555412724651,
12.));
#80406=CARTESIAN_POINT('Ctrl Pts',(-65.5132129675333,-24.7646342620841,
0.));
#80407=CARTESIAN_POINT('Ctrl Pts',(-65.5132129675333,-24.7646342620841,
12.));
#80408=CARTESIAN_POINT('Ctrl Pts',(-65.5290887770232,-24.7760493148465,
0.));
#80409=CARTESIAN_POINT('Ctrl Pts',(-65.5290887770232,-24.7760493148465,
12.));
#80410=CARTESIAN_POINT('Ctrl Pts',(-65.5449962514661,-24.787513182749,0.));
#80411=CARTESIAN_POINT('Ctrl Pts',(-65.5449962514661,-24.787513182749,12.));
#80412=CARTESIAN_POINT('Ctrl Pts',(-65.5609353062829,-24.799025856126,0.));
#80413=CARTESIAN_POINT('Ctrl Pts',(-65.5609353062829,-24.799025856126,12.));
#80414=CARTESIAN_POINT('Ctrl Pts',(-65.5769057914333,-24.8105873098626,
0.));
#80415=CARTESIAN_POINT('Ctrl Pts',(-65.5769057914333,-24.8105873098626,
12.));
#80416=CARTESIAN_POINT('Ctrl Pts',(-65.5929074932624,-24.8221975032104,
0.));
#80417=CARTESIAN_POINT('Ctrl Pts',(-65.5929074932624,-24.8221975032104,
12.));
#80418=CARTESIAN_POINT('Ctrl Pts',(-65.6089401625628,-24.8338563866764,
0.));
#80419=CARTESIAN_POINT('Ctrl Pts',(-65.6089401625628,-24.8338563866764,
12.));
#80420=CARTESIAN_POINT('Ctrl Pts',(-65.6250035361612,-24.8455639071517,
0.));
#80421=CARTESIAN_POINT('Ctrl Pts',(-65.6250035361612,-24.8455639071517,
12.));
#80422=CARTESIAN_POINT('Ctrl Pts',(-65.6410973603661,-24.8573200135666,
0.));
#80423=CARTESIAN_POINT('Ctrl Pts',(-65.6410973603661,-24.8573200135666,
12.));
#80424=CARTESIAN_POINT('Ctrl Pts',(-65.6572214156692,-24.8691246628057,
0.));
#80425=CARTESIAN_POINT('Ctrl Pts',(-65.6572214156692,-24.8691246628057,
12.));
#80426=CARTESIAN_POINT('Ctrl Pts',(-65.6733755087669,-24.8809778178229,
0.));
#80427=CARTESIAN_POINT('Ctrl Pts',(-65.6733755087669,-24.8809778178229,
12.));
#80428=CARTESIAN_POINT('Ctrl Pts',(-65.6895594608775,-24.8928794448607,
0.));
#80429=CARTESIAN_POINT('Ctrl Pts',(-65.6895594608775,-24.8928794448607,
12.));
#80430=CARTESIAN_POINT('Ctrl Pts',(-65.7057730980483,-24.9048295111448,
0.));
#80431=CARTESIAN_POINT('Ctrl Pts',(-65.7057730980483,-24.9048295111448,
12.));
#80432=CARTESIAN_POINT('Ctrl Pts',(-65.7220162391054,-24.9168279820106,
0.));
#80433=CARTESIAN_POINT('Ctrl Pts',(-65.7220162391054,-24.9168279820106,
12.));
#80434=CARTESIAN_POINT('Ctrl Pts',(-65.7382886895888,-24.928874819458,0.));
#80435=CARTESIAN_POINT('Ctrl Pts',(-65.7382886895888,-24.928874819458,12.));
#80436=CARTESIAN_POINT('Ctrl Pts',(-65.7545902480323,-24.9409699836537,
0.));
#80437=CARTESIAN_POINT('Ctrl Pts',(-65.7545902480323,-24.9409699836537,
12.));
#80438=CARTESIAN_POINT('Ctrl Pts',(-65.7709207098959,-24.9531134338696,
0.));
#80439=CARTESIAN_POINT('Ctrl Pts',(-65.7709207098959,-24.9531134338696,
12.));
#80440=CARTESIAN_POINT('Ctrl Pts',(-65.7872798720823,-24.9653051295581,
0.));
#80441=CARTESIAN_POINT('Ctrl Pts',(-65.7872798720823,-24.9653051295581,
12.));
#80442=CARTESIAN_POINT('Ctrl Pts',(-65.8036675380718,-24.9775450315682,
0.));
#80443=CARTESIAN_POINT('Ctrl Pts',(-65.8036675380718,-24.9775450315682,
12.));
#80444=CARTESIAN_POINT('Ctrl Pts',(-65.8200835177024,-24.9898331020983,
0.));
#80445=CARTESIAN_POINT('Ctrl Pts',(-65.8200835177024,-24.9898331020983,
12.));
#80446=CARTESIAN_POINT('Ctrl Pts',(-65.8365276247128,-25.002169304117,0.));
#80447=CARTESIAN_POINT('Ctrl Pts',(-65.8365276247128,-25.002169304117,12.));
#80448=CARTESIAN_POINT('Ctrl Pts',(-65.8529996750445,-25.0145536009604,
0.));
#80449=CARTESIAN_POINT('Ctrl Pts',(-65.8529996750445,-25.0145536009604,
12.));
#80450=CARTESIAN_POINT('Ctrl Pts',(-65.8694994847616,-25.0269859558362,
0.));
#80451=CARTESIAN_POINT('Ctrl Pts',(-65.8694994847616,-25.0269859558362,
12.));
#80452=CARTESIAN_POINT('Ctrl Pts',(-65.8860268683128,-25.0394663314055,
0.));
#80453=CARTESIAN_POINT('Ctrl Pts',(-65.8860268683128,-25.0394663314055,
12.));
#80454=CARTESIAN_POINT('Ctrl Pts',(-65.9025816394424,-25.0519946900078,
0.));
#80455=CARTESIAN_POINT('Ctrl Pts',(-65.9025816394424,-25.0519946900078,
12.));
#80456=CARTESIAN_POINT('Ctrl Pts',(-65.919163611981,-25.0645709938524,0.));
#80457=CARTESIAN_POINT('Ctrl Pts',(-65.919163611981,-25.0645709938524,12.));
#80458=CARTESIAN_POINT('Ctrl Pts',(-65.9357726006163,-25.0771952052028,
0.));
#80459=CARTESIAN_POINT('Ctrl Pts',(-65.9357726006163,-25.0771952052028,
12.));
#80460=CARTESIAN_POINT('Ctrl Pts',(-65.9524084218139,-25.0898672865915,
0.));
#80461=CARTESIAN_POINT('Ctrl Pts',(-65.9524084218139,-25.0898672865915,
12.));
#80462=CARTESIAN_POINT('Ctrl Pts',(-65.9690708941558,-25.1025872009004,
0.));
#80463=CARTESIAN_POINT('Ctrl Pts',(-65.9690708941558,-25.1025872009004,
12.));
#80464=CARTESIAN_POINT('Ctrl Pts',(-65.9857598378433,-25.1153549112503,
0.));
#80465=CARTESIAN_POINT('Ctrl Pts',(-65.9857598378433,-25.1153549112503,
12.));
#80466=CARTESIAN_POINT('Ctrl Pts',(-66.0024750743897,-25.1281703809297,
0.));
#80467=CARTESIAN_POINT('Ctrl Pts',(-66.0024750743897,-25.1281703809297,
12.));
#80468=CARTESIAN_POINT('Ctrl Pts',(-66.0192164262621,-25.1410335733099,
0.));
#80469=CARTESIAN_POINT('Ctrl Pts',(-66.0192164262621,-25.1410335733099,
12.));
#80470=CARTESIAN_POINT('Ctrl Pts',(-66.0359837164734,-25.1539444517419,
0.));
#80471=CARTESIAN_POINT('Ctrl Pts',(-66.0359837164734,-25.1539444517419,
12.));
#80472=CARTESIAN_POINT('Ctrl Pts',(-66.0527767686025,-25.1669029795661,
0.));
#80473=CARTESIAN_POINT('Ctrl Pts',(-66.0527767686025,-25.1669029795661,
12.));
#80474=CARTESIAN_POINT('Ctrl Pts',(-66.0695954069713,-25.1799091201599,
0.));
#80475=CARTESIAN_POINT('Ctrl Pts',(-66.0695954069713,-25.1799091201599,
12.));
#80476=CARTESIAN_POINT('Ctrl Pts',(-66.086439456768,-25.1929628369685,0.));
#80477=CARTESIAN_POINT('Ctrl Pts',(-66.086439456768,-25.1929628369685,12.));
#80478=CARTESIAN_POINT('Ctrl Pts',(-66.10330874419,-25.2060640935365,0.));
#80479=CARTESIAN_POINT('Ctrl Pts',(-66.10330874419,-25.2060640935365,12.));
#80480=CARTESIAN_POINT('Ctrl Pts',(-66.1202030965758,-25.2192128535357,
0.));
#80481=CARTESIAN_POINT('Ctrl Pts',(-66.1202030965758,-25.2192128535357,
12.));
#80482=CARTESIAN_POINT('Ctrl Pts',(-66.1371223423345,-25.232409080755,0.));
#80483=CARTESIAN_POINT('Ctrl Pts',(-66.1371223423345,-25.232409080755,12.));
#80484=CARTESIAN_POINT('Ctrl Pts',(-66.1540663108754,-25.2456527390875,
0.));
#80485=CARTESIAN_POINT('Ctrl Pts',(-66.1540663108754,-25.2456527390875,
12.));
#80486=CARTESIAN_POINT('Ctrl Pts',(-66.1710348325384,-25.2589437925147,
0.));
#80487=CARTESIAN_POINT('Ctrl Pts',(-66.1710348325384,-25.2589437925147,
12.));
#80488=CARTESIAN_POINT('Ctrl Pts',(-66.1880277385136,-25.2722822050837,
0.));
#80489=CARTESIAN_POINT('Ctrl Pts',(-66.1880277385136,-25.2722822050837,
12.));
#80490=CARTESIAN_POINT('Ctrl Pts',(-66.2050448607911,-25.285667940893,0.));
#80491=CARTESIAN_POINT('Ctrl Pts',(-66.2050448607911,-25.285667940893,12.));
#80492=CARTESIAN_POINT('Ctrl Pts',(-66.2220860321952,-25.2991009641094,
0.));
#80493=CARTESIAN_POINT('Ctrl Pts',(-66.2220860321952,-25.2991009641094,
12.));
#80494=CARTESIAN_POINT('Ctrl Pts',(-66.2391510863998,-25.312581238973,0.));
#80495=CARTESIAN_POINT('Ctrl Pts',(-66.2391510863998,-25.312581238973,12.));
#80496=CARTESIAN_POINT('Ctrl Pts',(-66.2562398579471,-25.3261087298026,
0.));
#80497=CARTESIAN_POINT('Ctrl Pts',(-66.2562398579471,-25.3261087298026,
12.));
#80498=CARTESIAN_POINT('Ctrl Pts',(-66.2733521822662,-25.3396834009949,
0.));
#80499=CARTESIAN_POINT('Ctrl Pts',(-66.2733521822662,-25.3396834009949,
12.));
#80500=CARTESIAN_POINT('Ctrl Pts',(-66.290487895671,-25.3533052170249,0.));
#80501=CARTESIAN_POINT('Ctrl Pts',(-66.290487895671,-25.3533052170249,12.));
#80502=CARTESIAN_POINT('Ctrl Pts',(-66.3076468353412,-25.3669741424488,
0.));
#80503=CARTESIAN_POINT('Ctrl Pts',(-66.3076468353412,-25.3669741424488,
12.));
#80504=CARTESIAN_POINT('Ctrl Pts',(-66.3248288393046,-25.3806901419012,
0.));
#80505=CARTESIAN_POINT('Ctrl Pts',(-66.3248288393046,-25.3806901419012,
12.));
#80506=CARTESIAN_POINT('Ctrl Pts',(-66.3420337464178,-25.3944531800901,
0.));
#80507=CARTESIAN_POINT('Ctrl Pts',(-66.3420337464178,-25.3944531800901,
12.));
#80508=CARTESIAN_POINT('Ctrl Pts',(-66.359261396341,-25.4082632217847,0.));
#80509=CARTESIAN_POINT('Ctrl Pts',(-66.359261396341,-25.4082632217847,12.));
#80510=CARTESIAN_POINT('Ctrl Pts',(-66.3765116295364,-25.4221202318199,
0.));
#80511=CARTESIAN_POINT('Ctrl Pts',(-66.3765116295364,-25.4221202318199,
12.));
#80512=CARTESIAN_POINT('Ctrl Pts',(-66.3937842872685,-25.4360241751018,
0.));
#80513=CARTESIAN_POINT('Ctrl Pts',(-66.3937842872685,-25.4360241751018,
12.));
#80514=CARTESIAN_POINT('Ctrl Pts',(-66.4110792116,-25.4499750166079,0.));
#80515=CARTESIAN_POINT('Ctrl Pts',(-66.4110792116,-25.4499750166079,12.));
#80516=CARTESIAN_POINT('Ctrl Pts',(-66.4283962453899,-25.4639727213849,
0.));
#80517=CARTESIAN_POINT('Ctrl Pts',(-66.4283962453899,-25.4639727213849,
12.));
#80518=CARTESIAN_POINT('Ctrl Pts',(-66.4457352322871,-25.4780172545417,
0.));
#80519=CARTESIAN_POINT('Ctrl Pts',(-66.4457352322871,-25.4780172545417,
12.));
#80520=CARTESIAN_POINT('Ctrl Pts',(-66.4630960167252,-25.4921085812547,
0.));
#80521=CARTESIAN_POINT('Ctrl Pts',(-66.4630960167252,-25.4921085812547,
12.));
#80522=CARTESIAN_POINT('Ctrl Pts',(-66.4804784439148,-25.5062466667702,
0.));
#80523=CARTESIAN_POINT('Ctrl Pts',(-66.4804784439148,-25.5062466667702,
12.));
#80524=CARTESIAN_POINT('Ctrl Pts',(-66.4978823598354,-25.5204314764033,
0.));
#80525=CARTESIAN_POINT('Ctrl Pts',(-66.4978823598354,-25.5204314764033,
12.));
#80526=CARTESIAN_POINT('Ctrl Pts',(-66.5153076112231,-25.534662975532,0.));
#80527=CARTESIAN_POINT('Ctrl Pts',(-66.5153076112231,-25.534662975532,12.));
#80528=CARTESIAN_POINT('Ctrl Pts',(-66.5327540455624,-25.5489411295912,
0.));
#80529=CARTESIAN_POINT('Ctrl Pts',(-66.5327540455624,-25.5489411295912,
12.));
#80530=CARTESIAN_POINT('Ctrl Pts',(-66.5502215110829,-25.5632659040792,
0.));
#80531=CARTESIAN_POINT('Ctrl Pts',(-66.5502215110829,-25.5632659040792,
12.));
#80532=CARTESIAN_POINT('Ctrl Pts',(-66.5677098567542,-25.5776372645601,
0.));
#80533=CARTESIAN_POINT('Ctrl Pts',(-66.5677098567542,-25.5776372645601,
12.));
#80534=CARTESIAN_POINT('Ctrl Pts',(-66.5852189322813,-25.5920551766629,
0.));
#80535=CARTESIAN_POINT('Ctrl Pts',(-66.5852189322813,-25.5920551766629,
12.));
#80536=CARTESIAN_POINT('Ctrl Pts',(-66.6027485880963,-25.6065196060756,
0.));
#80537=CARTESIAN_POINT('Ctrl Pts',(-66.6027485880963,-25.6065196060756,
12.));
#80538=CARTESIAN_POINT('Ctrl Pts',(-66.6202986753506,-25.6210305185403,
0.));
#80539=CARTESIAN_POINT('Ctrl Pts',(-66.6202986753506,-25.6210305185403,
12.));
#80540=CARTESIAN_POINT('Ctrl Pts',(-66.6378690459129,-25.6355878798614,
0.));
#80541=CARTESIAN_POINT('Ctrl Pts',(-66.6378690459129,-25.6355878798614,
12.));
#80542=CARTESIAN_POINT('Ctrl Pts',(-66.6554595523624,-25.6501916559055,
0.));
#80543=CARTESIAN_POINT('Ctrl Pts',(-66.6554595523624,-25.6501916559055,
12.));
#80544=CARTESIAN_POINT('Ctrl Pts',(-66.6730700479837,-25.6648418126013,
0.));
#80545=CARTESIAN_POINT('Ctrl Pts',(-66.6730700479837,-25.6648418126013,
12.));
#80546=CARTESIAN_POINT('Ctrl Pts',(-66.6907003867572,-25.6795383159319,
0.));
#80547=CARTESIAN_POINT('Ctrl Pts',(-66.6907003867572,-25.6795383159319,
12.));
#80548=CARTESIAN_POINT('Ctrl Pts',(-66.7083504233529,-25.6942811319322,
0.));
#80549=CARTESIAN_POINT('Ctrl Pts',(-66.7083504233529,-25.6942811319322,
12.));
#80550=CARTESIAN_POINT('Ctrl Pts',(-66.7260200131266,-25.7090702266963,
0.));
#80551=CARTESIAN_POINT('Ctrl Pts',(-66.7260200131266,-25.7090702266963,
12.));
#80552=CARTESIAN_POINT('Ctrl Pts',(-66.7437090121153,-25.7239055663772,
0.));
#80553=CARTESIAN_POINT('Ctrl Pts',(-66.7437090121153,-25.7239055663772,
12.));
#80554=CARTESIAN_POINT('Ctrl Pts',(-66.7614172770316,-25.7387871171866,
0.));
#80555=CARTESIAN_POINT('Ctrl Pts',(-66.7614172770316,-25.7387871171866,
12.));
#80556=CARTESIAN_POINT('Ctrl Pts',(-66.7791446652545,-25.7537148453864,
0.));
#80557=CARTESIAN_POINT('Ctrl Pts',(-66.7791446652545,-25.7537148453864,
12.));
#80558=CARTESIAN_POINT('Ctrl Pts',(-66.7968910348245,-25.7686887172878,
0.));
#80559=CARTESIAN_POINT('Ctrl Pts',(-66.7968910348245,-25.7686887172878,
12.));
#80560=CARTESIAN_POINT('Ctrl Pts',(-66.8146562444433,-25.7837086992595,
0.));
#80561=CARTESIAN_POINT('Ctrl Pts',(-66.8146562444433,-25.7837086992595,
12.));
#80562=CARTESIAN_POINT('Ctrl Pts',(-66.8324401534668,-25.7987747577269,
0.));
#80563=CARTESIAN_POINT('Ctrl Pts',(-66.8324401534668,-25.7987747577269,
12.));
#80564=CARTESIAN_POINT('Ctrl Pts',(-66.8502426219001,-25.8138868591709,
0.));
#80565=CARTESIAN_POINT('Ctrl Pts',(-66.8502426219001,-25.8138868591709,
12.));
#80566=CARTESIAN_POINT('Ctrl Pts',(-66.8680635103876,-25.8290449701193,
0.));
#80567=CARTESIAN_POINT('Ctrl Pts',(-66.8680635103876,-25.8290449701193,
12.));
#80568=CARTESIAN_POINT('Ctrl Pts',(-66.8859026802088,-25.844249057147,0.));
#80569=CARTESIAN_POINT('Ctrl Pts',(-66.8859026802088,-25.844249057147,12.));
#80570=CARTESIAN_POINT('Ctrl Pts',(-66.9037599932761,-25.8594990868833,
0.));
#80571=CARTESIAN_POINT('Ctrl Pts',(-66.9037599932761,-25.8594990868833,
12.));
#80572=CARTESIAN_POINT('Ctrl Pts',(-66.92163531213,-25.8747950260111,0.));
#80573=CARTESIAN_POINT('Ctrl Pts',(-66.92163531213,-25.8747950260111,12.));
#80574=CARTESIAN_POINT('Ctrl Pts',(-66.939528499934,-25.890136841266,0.));
#80575=CARTESIAN_POINT('Ctrl Pts',(-66.939528499934,-25.890136841266,12.));
#80576=CARTESIAN_POINT('Ctrl Pts',(-66.9574394204663,-25.9055244994277,
0.));
#80577=CARTESIAN_POINT('Ctrl Pts',(-66.9574394204663,-25.9055244994277,
12.));
#80578=CARTESIAN_POINT('Ctrl Pts',(-66.975367938115,-25.9209579673209,0.));
#80579=CARTESIAN_POINT('Ctrl Pts',(-66.975367938115,-25.9209579673209,12.));
#80580=CARTESIAN_POINT('Ctrl Pts',(-66.9933139178778,-25.9364372118222,
0.));
#80581=CARTESIAN_POINT('Ctrl Pts',(-66.9933139178778,-25.9364372118222,
12.));
#80582=CARTESIAN_POINT('Ctrl Pts',(-67.0112772253556,-25.9519621998598,
0.));
#80583=CARTESIAN_POINT('Ctrl Pts',(-67.0112772253556,-25.9519621998598,
12.));
#80584=CARTESIAN_POINT('Ctrl Pts',(-67.0292577267489,-25.967532898412,0.));
#80585=CARTESIAN_POINT('Ctrl Pts',(-67.0292577267489,-25.967532898412,12.));
#80586=CARTESIAN_POINT('Ctrl Pts',(-67.0472552888485,-25.9831492744984,
0.));
#80587=CARTESIAN_POINT('Ctrl Pts',(-67.0472552888485,-25.9831492744984,
12.));
#80588=CARTESIAN_POINT('Ctrl Pts',(-67.0652697790325,-25.9988112951814,
0.));
#80589=CARTESIAN_POINT('Ctrl Pts',(-67.0652697790325,-25.9988112951814,
12.));
#80590=CARTESIAN_POINT('Ctrl Pts',(-67.0833010652634,-26.014518927573,0.));
#80591=CARTESIAN_POINT('Ctrl Pts',(-67.0833010652634,-26.014518927573,12.));
#80592=CARTESIAN_POINT('Ctrl Pts',(-67.101349016084,-26.030272138834,0.));
#80593=CARTESIAN_POINT('Ctrl Pts',(-67.101349016084,-26.030272138834,12.));
#80594=CARTESIAN_POINT('Ctrl Pts',(-67.1194135006124,-26.0460708961725,
0.));
#80595=CARTESIAN_POINT('Ctrl Pts',(-67.1194135006124,-26.0460708961725,
12.));
#80596=CARTESIAN_POINT('Ctrl Pts',(-67.1374943885354,-26.061915166836,0.));
#80597=CARTESIAN_POINT('Ctrl Pts',(-67.1374943885354,-26.061915166836,12.));
#80598=CARTESIAN_POINT('Ctrl Pts',(-67.1555915501049,-26.0778049181128,
0.));
#80599=CARTESIAN_POINT('Ctrl Pts',(-67.1555915501049,-26.0778049181128,
12.));
#80600=CARTESIAN_POINT('Ctrl Pts',(-67.173704856136,-26.0937401173383,0.));
#80601=CARTESIAN_POINT('Ctrl Pts',(-67.173704856136,-26.0937401173383,12.));
#80602=CARTESIAN_POINT('Ctrl Pts',(-67.1918341780018,-26.1097207318949,
0.));
#80603=CARTESIAN_POINT('Ctrl Pts',(-67.1918341780018,-26.1097207318949,
12.));
#80604=CARTESIAN_POINT('Ctrl Pts',(-67.2099793876297,-26.1257467292102,
0.));
#80605=CARTESIAN_POINT('Ctrl Pts',(-67.2099793876297,-26.1257467292102,
12.));
#80606=CARTESIAN_POINT('Ctrl Pts',(-67.2281403574938,-26.1418180767489,
0.));
#80607=CARTESIAN_POINT('Ctrl Pts',(-67.2281403574938,-26.1418180767489,
12.));
#80608=CARTESIAN_POINT('Ctrl Pts',(-67.2463169606115,-26.1579347420138,
0.));
#80609=CARTESIAN_POINT('Ctrl Pts',(-67.2463169606115,-26.1579347420138,
12.));
#80610=CARTESIAN_POINT('Ctrl Pts',(-67.2645090705421,-26.1740966925529,
0.));
#80611=CARTESIAN_POINT('Ctrl Pts',(-67.2645090705421,-26.1740966925529,
12.));
#80612=CARTESIAN_POINT('Ctrl Pts',(-67.282716561383,-26.1903038959589,0.));
#80613=CARTESIAN_POINT('Ctrl Pts',(-67.282716561383,-26.1903038959589,12.));
#80614=CARTESIAN_POINT('Ctrl Pts',(-67.3009393077651,-26.2065563198683,
0.));
#80615=CARTESIAN_POINT('Ctrl Pts',(-67.3009393077651,-26.2065563198683,
12.));
#80616=CARTESIAN_POINT('Ctrl Pts',(-67.3191771848463,-26.2228539319526,
0.));
#80617=CARTESIAN_POINT('Ctrl Pts',(-67.3191771848463,-26.2228539319526,
12.));
#80618=CARTESIAN_POINT('Ctrl Pts',(-67.3374300683073,-26.2391966999191,
0.));
#80619=CARTESIAN_POINT('Ctrl Pts',(-67.3374300683073,-26.2391966999191,
12.));
#80620=CARTESIAN_POINT('Ctrl Pts',(-67.3556978343507,-26.255584591518,0.));
#80621=CARTESIAN_POINT('Ctrl Pts',(-67.3556978343507,-26.255584591518,12.));
#80622=CARTESIAN_POINT('Ctrl Pts',(-67.3739803596969,-26.2720175745423,
0.));
#80623=CARTESIAN_POINT('Ctrl Pts',(-67.3739803596969,-26.2720175745423,
12.));
#80624=CARTESIAN_POINT('Ctrl Pts',(-67.392277521581,-26.288495616827,0.));
#80625=CARTESIAN_POINT('Ctrl Pts',(-67.392277521581,-26.288495616827,12.));
#80626=CARTESIAN_POINT('Ctrl Pts',(-67.4105891977461,-26.3050186862407,
0.));
#80627=CARTESIAN_POINT('Ctrl Pts',(-67.4105891977461,-26.3050186862407,
12.));
#80628=CARTESIAN_POINT('Ctrl Pts',(-67.4289152664398,-26.321586750686,0.));
#80629=CARTESIAN_POINT('Ctrl Pts',(-67.4289152664398,-26.321586750686,12.));
#80630=CARTESIAN_POINT('Ctrl Pts',(-67.4472556064119,-26.3381997781055,
0.));
#80631=CARTESIAN_POINT('Ctrl Pts',(-67.4472556064119,-26.3381997781055,
12.));
#80632=CARTESIAN_POINT('Ctrl Pts',(-67.4656100969116,-26.3548577364833,
0.));
#80633=CARTESIAN_POINT('Ctrl Pts',(-67.4656100969116,-26.3548577364833,
12.));
#80634=CARTESIAN_POINT('Ctrl Pts',(-67.4839786176836,-26.3715605938433,
0.));
#80635=CARTESIAN_POINT('Ctrl Pts',(-67.4839786176836,-26.3715605938433,
12.));
#80636=CARTESIAN_POINT('Ctrl Pts',(-67.5023610489622,-26.3883083182421,
0.));
#80637=CARTESIAN_POINT('Ctrl Pts',(-67.5023610489622,-26.3883083182421,
12.));
#80638=CARTESIAN_POINT('Ctrl Pts',(-67.5207572714683,-26.4051008777675,
0.));
#80639=CARTESIAN_POINT('Ctrl Pts',(-67.5207572714683,-26.4051008777675,
12.));
#80640=CARTESIAN_POINT('Ctrl Pts',(-67.5391671664072,-26.4219382405458,
0.));
#80641=CARTESIAN_POINT('Ctrl Pts',(-67.5391671664072,-26.4219382405458,
12.));
#80642=CARTESIAN_POINT('Ctrl Pts',(-67.5575906154657,-26.4388203747425,
0.));
#80643=CARTESIAN_POINT('Ctrl Pts',(-67.5575906154657,-26.4388203747425,
12.));
#80644=CARTESIAN_POINT('Ctrl Pts',(-67.5760275008093,-26.4557472485621,
0.));
#80645=CARTESIAN_POINT('Ctrl Pts',(-67.5760275008093,-26.4557472485621,
12.));
#80646=CARTESIAN_POINT('Ctrl Pts',(-67.5944777050768,-26.4727188302409,
0.));
#80647=CARTESIAN_POINT('Ctrl Pts',(-67.5944777050768,-26.4727188302409,
12.));
#80648=CARTESIAN_POINT('Ctrl Pts',(-67.6129411113757,-26.489735088044,0.));
#80649=CARTESIAN_POINT('Ctrl Pts',(-67.6129411113757,-26.489735088044,12.));
#80650=CARTESIAN_POINT('Ctrl Pts',(-67.6314176032811,-26.5067959902725,
0.));
#80651=CARTESIAN_POINT('Ctrl Pts',(-67.6314176032811,-26.5067959902725,
12.));
#80652=CARTESIAN_POINT('Ctrl Pts',(-67.649907064832,-26.5239015052654,0.));
#80653=CARTESIAN_POINT('Ctrl Pts',(-67.649907064832,-26.5239015052654,12.));
#80654=CARTESIAN_POINT('Ctrl Pts',(-67.6684093805291,-26.5410516013985,
0.));
#80655=CARTESIAN_POINT('Ctrl Pts',(-67.6684093805291,-26.5410516013985,
12.));
#80656=CARTESIAN_POINT('Ctrl Pts',(-67.6869244353294,-26.5582462470794,
0.));
#80657=CARTESIAN_POINT('Ctrl Pts',(-67.6869244353294,-26.5582462470794,
12.));
#80658=CARTESIAN_POINT('Ctrl Pts',(-67.7054521146424,-26.5754854107421,
0.));
#80659=CARTESIAN_POINT('Ctrl Pts',(-67.7054521146424,-26.5754854107421,
12.));
#80660=CARTESIAN_POINT('Ctrl Pts',(-67.7239923043288,-26.5927690608544,
0.));
#80661=CARTESIAN_POINT('Ctrl Pts',(-67.7239923043288,-26.5927690608544,
12.));
#80662=CARTESIAN_POINT('Ctrl Pts',(-67.7425448906977,-26.6100971659202,
0.));
#80663=CARTESIAN_POINT('Ctrl Pts',(-67.7425448906977,-26.6100971659202,
12.));
#80664=CARTESIAN_POINT('Ctrl Pts',(-67.7611097605042,-26.6274696944793,
0.));
#80665=CARTESIAN_POINT('Ctrl Pts',(-67.7611097605042,-26.6274696944793,
12.));
#80666=CARTESIAN_POINT('Ctrl Pts',(-67.7796868009455,-26.6448866151029,
0.));
#80667=CARTESIAN_POINT('Ctrl Pts',(-67.7796868009455,-26.6448866151029,
12.));
#80668=CARTESIAN_POINT('Ctrl Pts',(-67.798275899657,-26.6623478963871,0.));
#80669=CARTESIAN_POINT('Ctrl Pts',(-67.798275899657,-26.6623478963871,12.));
#80670=CARTESIAN_POINT('Ctrl Pts',(-67.8168769447098,-26.6798535069589,
0.));
#80671=CARTESIAN_POINT('Ctrl Pts',(-67.8168769447098,-26.6798535069589,
12.));
#80672=CARTESIAN_POINT('Ctrl Pts',(-67.8354898246086,-26.6974034154804,
0.));
#80673=CARTESIAN_POINT('Ctrl Pts',(-67.8354898246086,-26.6974034154804,
12.));
#80674=CARTESIAN_POINT('Ctrl Pts',(-67.8541144282875,-26.7149975906478,
0.));
#80675=CARTESIAN_POINT('Ctrl Pts',(-67.8541144282875,-26.7149975906478,
12.));
#80676=CARTESIAN_POINT('Ctrl Pts',(-67.8727506451063,-26.7326360011885,
0.));
#80677=CARTESIAN_POINT('Ctrl Pts',(-67.8727506451063,-26.7326360011885,
12.));
#80678=CARTESIAN_POINT('Ctrl Pts',(-67.8913983648436,-26.7503186158522,
0.));
#80679=CARTESIAN_POINT('Ctrl Pts',(-67.8913983648436,-26.7503186158522,
12.));
#80680=CARTESIAN_POINT('Ctrl Pts',(-67.9100574776972,-26.7680454034169,
0.));
#80681=CARTESIAN_POINT('Ctrl Pts',(-67.9100574776972,-26.7680454034169,
12.));
#80682=CARTESIAN_POINT('Ctrl Pts',(-67.928727874284,-26.7858163326934,0.));
#80683=CARTESIAN_POINT('Ctrl Pts',(-67.928727874284,-26.7858163326934,12.));
#80684=CARTESIAN_POINT('Ctrl Pts',(-67.9474094456396,-26.8036313725262,
0.));
#80685=CARTESIAN_POINT('Ctrl Pts',(-67.9474094456396,-26.8036313725262,
12.));
#80686=CARTESIAN_POINT('Ctrl Pts',(-67.9661020832164,-26.821490491792,0.));
#80687=CARTESIAN_POINT('Ctrl Pts',(-67.9661020832164,-26.821490491792,12.));
#80688=CARTESIAN_POINT('Ctrl Pts',(-67.9848056788809,-26.8393936593911,
0.));
#80689=CARTESIAN_POINT('Ctrl Pts',(-67.9848056788809,-26.8393936593911,
12.));
#80690=CARTESIAN_POINT('Ctrl Pts',(-68.0035201249102,-26.8573408442496,
0.));
#80691=CARTESIAN_POINT('Ctrl Pts',(-68.0035201249102,-26.8573408442496,
12.));
#80692=CARTESIAN_POINT('Ctrl Pts',(-68.0222453139856,-26.8753320153252,
0.));
#80693=CARTESIAN_POINT('Ctrl Pts',(-68.0222453139856,-26.8753320153252,
12.));
#80694=CARTESIAN_POINT('Ctrl Pts',(-68.0409811391869,-26.8933671416063,
0.));
#80695=CARTESIAN_POINT('Ctrl Pts',(-68.0409811391869,-26.8933671416063,
12.));
#80696=CARTESIAN_POINT('Ctrl Pts',(-68.0597274939859,-26.911446192111,0.));
#80697=CARTESIAN_POINT('Ctrl Pts',(-68.0597274939859,-26.911446192111,12.));
#80698=CARTESIAN_POINT('Ctrl Pts',(-68.0784842722369,-26.9295691358779,
0.));
#80699=CARTESIAN_POINT('Ctrl Pts',(-68.0784842722369,-26.9295691358779,
12.));
#80700=CARTESIAN_POINT('Ctrl Pts',(-68.0972513681751,-26.9477359419652,
0.));
#80701=CARTESIAN_POINT('Ctrl Pts',(-68.0972513681751,-26.9477359419652,
12.));
#80702=CARTESIAN_POINT('Ctrl Pts',(-68.1160286764255,-26.9659465794601,
0.));
#80703=CARTESIAN_POINT('Ctrl Pts',(-68.1160286764255,-26.9659465794601,
12.));
#80704=CARTESIAN_POINT('Ctrl Pts',(-68.1348160920106,-26.9842010174822,
0.));
#80705=CARTESIAN_POINT('Ctrl Pts',(-68.1348160920106,-26.9842010174822,
12.));
#80706=CARTESIAN_POINT('Ctrl Pts',(-68.1536135103557,-27.0024992251838,
0.));
#80707=CARTESIAN_POINT('Ctrl Pts',(-68.1536135103557,-27.0024992251838,
12.));
#80708=CARTESIAN_POINT('Ctrl Pts',(-68.1724208272958,-27.0208411717472,
0.));
#80709=CARTESIAN_POINT('Ctrl Pts',(-68.1724208272958,-27.0208411717472,
12.));
#80710=CARTESIAN_POINT('Ctrl Pts',(-68.1912379390773,-27.0392268263798,
0.));
#80711=CARTESIAN_POINT('Ctrl Pts',(-68.1912379390773,-27.0392268263798,
12.));
#80712=CARTESIAN_POINT('Ctrl Pts',(-68.2100647423332,-27.0576561583172,
0.));
#80713=CARTESIAN_POINT('Ctrl Pts',(-68.2100647423332,-27.0576561583172,
12.));
#80714=CARTESIAN_POINT('Ctrl Pts',(-68.2289011340615,-27.0761291368226,
0.));
#80715=CARTESIAN_POINT('Ctrl Pts',(-68.2289011340615,-27.0761291368226,
12.));
#80716=CARTESIAN_POINT('Ctrl Pts',(-68.2477470116012,-27.0946457311813,
0.));
#80717=CARTESIAN_POINT('Ctrl Pts',(-68.2477470116012,-27.0946457311813,
12.));
#80718=CARTESIAN_POINT('Ctrl Pts',(-68.2666022726104,-27.1132059106943,
0.));
#80719=CARTESIAN_POINT('Ctrl Pts',(-68.2666022726104,-27.1132059106943,
12.));
#80720=CARTESIAN_POINT('Ctrl Pts',(-68.2854668150364,-27.1318096446649,
0.));
#80721=CARTESIAN_POINT('Ctrl Pts',(-68.2854668150364,-27.1318096446649,
12.));
#80722=CARTESIAN_POINT('Ctrl Pts',(-68.3043405371603,-27.1504569024136,
0.));
#80723=CARTESIAN_POINT('Ctrl Pts',(-68.3043405371603,-27.1504569024136,
12.));
#80724=CARTESIAN_POINT('Ctrl Pts',(-68.3232233376425,-27.1691476532921,
0.));
#80725=CARTESIAN_POINT('Ctrl Pts',(-68.3232233376425,-27.1691476532921,
12.));
#80726=CARTESIAN_POINT('Ctrl Pts',(-68.3421151155711,-27.1878818666926,
0.));
#80727=CARTESIAN_POINT('Ctrl Pts',(-68.3421151155711,-27.1878818666926,
12.));
#80728=CARTESIAN_POINT('Ctrl Pts',(-68.3610157704994,-27.2066595120542,
0.));
#80729=CARTESIAN_POINT('Ctrl Pts',(-68.3610157704994,-27.2066595120542,
12.));
#80730=CARTESIAN_POINT('Ctrl Pts',(-68.3799252025102,-27.2254805588673,
0.));
#80731=CARTESIAN_POINT('Ctrl Pts',(-68.3799252025102,-27.2254805588673,
12.));
#80732=CARTESIAN_POINT('Ctrl Pts',(-68.3988433121581,-27.244344976665,0.));
#80733=CARTESIAN_POINT('Ctrl Pts',(-68.3988433121581,-27.244344976665,12.));
#80734=CARTESIAN_POINT('Ctrl Pts',(-68.4177700003465,-27.263252735006,0.));
#80735=CARTESIAN_POINT('Ctrl Pts',(-68.4177700003465,-27.263252735006,12.));
#80736=CARTESIAN_POINT('Ctrl Pts',(-68.4367051682164,-27.2822038034538,
0.));
#80737=CARTESIAN_POINT('Ctrl Pts',(-68.4367051682164,-27.2822038034538,
12.));
#80738=CARTESIAN_POINT('Ctrl Pts',(-68.4556487170441,-27.301198151557,0.));
#80739=CARTESIAN_POINT('Ctrl Pts',(-68.4556487170441,-27.301198151557,12.));
#80740=CARTESIAN_POINT('Ctrl Pts',(-68.4746005480997,-27.3202357488154,
0.));
#80741=CARTESIAN_POINT('Ctrl Pts',(-68.4746005480997,-27.3202357488154,
12.));
#80742=CARTESIAN_POINT('Ctrl Pts',(-68.4935605626372,-27.3393165646752,
0.));
#80743=CARTESIAN_POINT('Ctrl Pts',(-68.4935605626372,-27.3393165646752,
12.));
#80744=CARTESIAN_POINT('Ctrl Pts',(-68.5125286621902,-27.3584405685947,
0.));
#80745=CARTESIAN_POINT('Ctrl Pts',(-68.5125286621902,-27.3584405685947,
12.));
#80746=CARTESIAN_POINT('Ctrl Pts',(-68.5315047488046,-27.3776077300918,
0.));
#80747=CARTESIAN_POINT('Ctrl Pts',(-68.5315047488046,-27.3776077300918,
12.));
#80748=CARTESIAN_POINT('Ctrl Pts',(-68.5504887252976,-27.3968180187941,
0.));
#80749=CARTESIAN_POINT('Ctrl Pts',(-68.5504887252976,-27.3968180187941,
12.));
#80750=CARTESIAN_POINT('Ctrl Pts',(-68.5694804955002,-27.4160714044825,
0.));
#80751=CARTESIAN_POINT('Ctrl Pts',(-68.5694804955002,-27.4160714044825,
12.));
#80752=CARTESIAN_POINT('Ctrl Pts',(-68.5884799645193,-27.4353678571349,
0.));
#80753=CARTESIAN_POINT('Ctrl Pts',(-68.5884799645193,-27.4353678571349,
12.));
#80754=CARTESIAN_POINT('Ctrl Pts',(-68.6074870381588,-27.4547073468213,
0.));
#80755=CARTESIAN_POINT('Ctrl Pts',(-68.6074870381588,-27.4547073468213,
12.));
#80756=CARTESIAN_POINT('Ctrl Pts',(-68.6265016223536,-27.4740898435977,
0.));
#80757=CARTESIAN_POINT('Ctrl Pts',(-68.6265016223536,-27.4740898435977,
12.));
#80758=CARTESIAN_POINT('Ctrl Pts',(-68.6455236225471,-27.4935153173863,
0.));
#80759=CARTESIAN_POINT('Ctrl Pts',(-68.6455236225471,-27.4935153173863,
12.));
#80760=CARTESIAN_POINT('Ctrl Pts',(-68.6645529432059,-27.5129837378797,
0.));
#80761=CARTESIAN_POINT('Ctrl Pts',(-68.6645529432059,-27.5129837378797,
12.));
#80762=CARTESIAN_POINT('Ctrl Pts',(-68.683589486992,-27.5324950743723,0.));
#80763=CARTESIAN_POINT('Ctrl Pts',(-68.683589486992,-27.5324950743723,12.));
#80764=CARTESIAN_POINT('Ctrl Pts',(-68.7026331554348,-27.552049295893,0.));
#80765=CARTESIAN_POINT('Ctrl Pts',(-68.7026331554348,-27.552049295893,12.));
#80766=CARTESIAN_POINT('Ctrl Pts',(-68.721683850427,-27.5716463715027,0.));
#80767=CARTESIAN_POINT('Ctrl Pts',(-68.721683850427,-27.5716463715027,12.));
#80768=CARTESIAN_POINT('Ctrl Pts',(-68.7407414755291,-27.5912862705482,
0.));
#80769=CARTESIAN_POINT('Ctrl Pts',(-68.7407414755291,-27.5912862705482,
12.));
#80770=CARTESIAN_POINT('Ctrl Pts',(-68.7598059372121,-27.6109689629025,
0.));
#80771=CARTESIAN_POINT('Ctrl Pts',(-68.7598059372121,-27.6109689629025,
12.));
#80772=CARTESIAN_POINT('Ctrl Pts',(-68.7788771464655,-27.6306944192711,
0.));
#80773=CARTESIAN_POINT('Ctrl Pts',(-68.7788771464655,-27.6306944192711,
12.));
#80774=CARTESIAN_POINT('Ctrl Pts',(-68.7979550191773,-27.6504626112621,
0.));
#80775=CARTESIAN_POINT('Ctrl Pts',(-68.7979550191773,-27.6504626112621,
12.));
#80776=CARTESIAN_POINT('Ctrl Pts',(-68.8170394725786,-27.670273510707,0.));
#80777=CARTESIAN_POINT('Ctrl Pts',(-68.8170394725786,-27.670273510707,12.));
#80778=CARTESIAN_POINT('Ctrl Pts',(-68.8361304224378,-27.6901270891201,
0.));
#80779=CARTESIAN_POINT('Ctrl Pts',(-68.8361304224378,-27.6901270891201,
12.));
#80780=CARTESIAN_POINT('Ctrl Pts',(-68.855227779818,-27.7100233170728,0.));
#80781=CARTESIAN_POINT('Ctrl Pts',(-68.855227779818,-27.7100233170728,12.));
#80782=CARTESIAN_POINT('Ctrl Pts',(-68.8743314483451,-27.7299621636602,
0.));
#80783=CARTESIAN_POINT('Ctrl Pts',(-68.8743314483451,-27.7299621636602,
12.));
#80784=CARTESIAN_POINT('Ctrl Pts',(-68.8934413203945,-27.7499435957608,
0.));
#80785=CARTESIAN_POINT('Ctrl Pts',(-68.8934413203945,-27.7499435957608,
12.));
#80786=CARTESIAN_POINT('Ctrl Pts',(-68.9125572825946,-27.7699675790683,
0.));
#80787=CARTESIAN_POINT('Ctrl Pts',(-68.9125572825946,-27.7699675790683,
12.));
#80788=CARTESIAN_POINT('Ctrl Pts',(-68.9316792226187,-27.7900340793796,
0.));
#80789=CARTESIAN_POINT('Ctrl Pts',(-68.9316792226187,-27.7900340793796,
12.));
#80790=CARTESIAN_POINT('Ctrl Pts',(-68.9508070357786,-27.8101430638128,
0.));
#80791=CARTESIAN_POINT('Ctrl Pts',(-68.9508070357786,-27.8101430638128,
12.));
#80792=CARTESIAN_POINT('Ctrl Pts',(-68.9699406311305,-27.8302945019939,
0.));
#80793=CARTESIAN_POINT('Ctrl Pts',(-68.9699406311305,-27.8302945019939,
12.));
#80794=CARTESIAN_POINT('Ctrl Pts',(-68.9890799391863,-27.8504883673903,
0.));
#80795=CARTESIAN_POINT('Ctrl Pts',(-68.9890799391863,-27.8504883673903,
12.));
#80796=CARTESIAN_POINT('Ctrl Pts',(-69.0082249138015,-27.8707246380697,
0.));
#80797=CARTESIAN_POINT('Ctrl Pts',(-69.0082249138015,-27.8707246380697,
12.));
#80798=CARTESIAN_POINT('Ctrl Pts',(-69.0273755264702,-27.8910032967037,
0.));
#80799=CARTESIAN_POINT('Ctrl Pts',(-69.0273755264702,-27.8910032967037,
12.));
#80800=CARTESIAN_POINT('Ctrl Pts',(-69.0427005153223,-27.9072601239469,
0.));
#80801=CARTESIAN_POINT('Ctrl Pts',(-69.0427005153223,-27.9072601239469,
12.));
#80802=CARTESIAN_POINT('Ctrl Pts',(-69.0541967850685,-27.9194718098851,
0.));
#80803=CARTESIAN_POINT('Ctrl Pts',(-69.0541967850685,-27.9194718098851,
12.));
#80804=CARTESIAN_POINT('Ctrl Pts',(-69.0618620884596,-27.9276214070576,
0.));
#80805=CARTESIAN_POINT('Ctrl Pts',(-69.0618620884596,-27.9276214070576,
12.));
#80806=CARTESIAN_POINT('Ctrl Pts',(-69.065695021045,-27.9316983239472,0.));
#80807=CARTESIAN_POINT('Ctrl Pts',(-69.065695021045,-27.9316983239472,12.));
#80808=CARTESIAN_POINT('',(-65.4815644032299,-24.7419628022042,0.));
#80809=CARTESIAN_POINT('Ctrl Pts',(-65.4815644032299,-24.7419628022042,
0.));
#80810=CARTESIAN_POINT('Ctrl Pts',(-65.4847237095443,-24.7442214063382,
0.));
#80811=CARTESIAN_POINT('Ctrl Pts',(-65.4910454936254,-24.7487434955982,
0.));
#80812=CARTESIAN_POINT('Ctrl Pts',(-65.5005376841101,-24.7555412724651,
0.));
#80813=CARTESIAN_POINT('Ctrl Pts',(-65.5132129675333,-24.7646342620841,
0.));
#80814=CARTESIAN_POINT('Ctrl Pts',(-65.5290887770232,-24.7760493148465,
0.));
#80815=CARTESIAN_POINT('Ctrl Pts',(-65.5449962514661,-24.787513182749,0.));
#80816=CARTESIAN_POINT('Ctrl Pts',(-65.5609353062829,-24.799025856126,0.));
#80817=CARTESIAN_POINT('Ctrl Pts',(-65.5769057914333,-24.8105873098626,
0.));
#80818=CARTESIAN_POINT('Ctrl Pts',(-65.5929074932624,-24.8221975032104,
0.));
#80819=CARTESIAN_POINT('Ctrl Pts',(-65.6089401625628,-24.8338563866764,
0.));
#80820=CARTESIAN_POINT('Ctrl Pts',(-65.6250035361612,-24.8455639071517,
0.));
#80821=CARTESIAN_POINT('Ctrl Pts',(-65.6410973603661,-24.8573200135666,
0.));
#80822=CARTESIAN_POINT('Ctrl Pts',(-65.6572214156692,-24.8691246628057,
0.));
#80823=CARTESIAN_POINT('Ctrl Pts',(-65.6733755087669,-24.8809778178229,
0.));
#80824=CARTESIAN_POINT('Ctrl Pts',(-65.6895594608775,-24.8928794448607,
0.));
#80825=CARTESIAN_POINT('Ctrl Pts',(-65.7057730980483,-24.9048295111448,
0.));
#80826=CARTESIAN_POINT('Ctrl Pts',(-65.7220162391054,-24.9168279820106,
0.));
#80827=CARTESIAN_POINT('Ctrl Pts',(-65.7382886895888,-24.928874819458,0.));
#80828=CARTESIAN_POINT('Ctrl Pts',(-65.7545902480323,-24.9409699836537,
0.));
#80829=CARTESIAN_POINT('Ctrl Pts',(-65.7709207098959,-24.9531134338696,
0.));
#80830=CARTESIAN_POINT('Ctrl Pts',(-65.7872798720823,-24.9653051295581,
0.));
#80831=CARTESIAN_POINT('Ctrl Pts',(-65.8036675380718,-24.9775450315682,
0.));
#80832=CARTESIAN_POINT('Ctrl Pts',(-65.8200835177024,-24.9898331020983,
0.));
#80833=CARTESIAN_POINT('Ctrl Pts',(-65.8365276247128,-25.002169304117,0.));
#80834=CARTESIAN_POINT('Ctrl Pts',(-65.8529996750445,-25.0145536009604,
0.));
#80835=CARTESIAN_POINT('Ctrl Pts',(-65.8694994847616,-25.0269859558362,
0.));
#80836=CARTESIAN_POINT('Ctrl Pts',(-65.8860268683128,-25.0394663314055,
0.));
#80837=CARTESIAN_POINT('Ctrl Pts',(-65.9025816394424,-25.0519946900078,
0.));
#80838=CARTESIAN_POINT('Ctrl Pts',(-65.919163611981,-25.0645709938524,0.));
#80839=CARTESIAN_POINT('Ctrl Pts',(-65.9357726006163,-25.0771952052028,
0.));
#80840=CARTESIAN_POINT('Ctrl Pts',(-65.9524084218139,-25.0898672865915,
0.));
#80841=CARTESIAN_POINT('Ctrl Pts',(-65.9690708941558,-25.1025872009004,
0.));
#80842=CARTESIAN_POINT('Ctrl Pts',(-65.9857598378433,-25.1153549112503,
0.));
#80843=CARTESIAN_POINT('Ctrl Pts',(-66.0024750743897,-25.1281703809297,
0.));
#80844=CARTESIAN_POINT('Ctrl Pts',(-66.0192164262621,-25.1410335733099,
0.));
#80845=CARTESIAN_POINT('Ctrl Pts',(-66.0359837164734,-25.1539444517419,
0.));
#80846=CARTESIAN_POINT('Ctrl Pts',(-66.0527767686025,-25.1669029795661,
0.));
#80847=CARTESIAN_POINT('Ctrl Pts',(-66.0695954069713,-25.1799091201599,
0.));
#80848=CARTESIAN_POINT('Ctrl Pts',(-66.086439456768,-25.1929628369685,0.));
#80849=CARTESIAN_POINT('Ctrl Pts',(-66.10330874419,-25.2060640935365,0.));
#80850=CARTESIAN_POINT('Ctrl Pts',(-66.1202030965758,-25.2192128535357,
0.));
#80851=CARTESIAN_POINT('Ctrl Pts',(-66.1371223423345,-25.232409080755,0.));
#80852=CARTESIAN_POINT('Ctrl Pts',(-66.1540663108754,-25.2456527390875,
0.));
#80853=CARTESIAN_POINT('Ctrl Pts',(-66.1710348325384,-25.2589437925147,
0.));
#80854=CARTESIAN_POINT('Ctrl Pts',(-66.1880277385136,-25.2722822050837,
0.));
#80855=CARTESIAN_POINT('Ctrl Pts',(-66.2050448607911,-25.285667940893,0.));
#80856=CARTESIAN_POINT('Ctrl Pts',(-66.2220860321952,-25.2991009641094,
0.));
#80857=CARTESIAN_POINT('Ctrl Pts',(-66.2391510863998,-25.312581238973,0.));
#80858=CARTESIAN_POINT('Ctrl Pts',(-66.2562398579471,-25.3261087298026,
0.));
#80859=CARTESIAN_POINT('Ctrl Pts',(-66.2733521822662,-25.3396834009949,
0.));
#80860=CARTESIAN_POINT('Ctrl Pts',(-66.290487895671,-25.3533052170249,0.));
#80861=CARTESIAN_POINT('Ctrl Pts',(-66.3076468353412,-25.3669741424488,
0.));
#80862=CARTESIAN_POINT('Ctrl Pts',(-66.3248288393046,-25.3806901419012,
0.));
#80863=CARTESIAN_POINT('Ctrl Pts',(-66.3420337464178,-25.3944531800901,
0.));
#80864=CARTESIAN_POINT('Ctrl Pts',(-66.359261396341,-25.4082632217847,0.));
#80865=CARTESIAN_POINT('Ctrl Pts',(-66.3765116295364,-25.4221202318199,
0.));
#80866=CARTESIAN_POINT('Ctrl Pts',(-66.3937842872685,-25.4360241751018,
0.));
#80867=CARTESIAN_POINT('Ctrl Pts',(-66.4110792116,-25.4499750166079,0.));
#80868=CARTESIAN_POINT('Ctrl Pts',(-66.4283962453899,-25.4639727213849,
0.));
#80869=CARTESIAN_POINT('Ctrl Pts',(-66.4457352322871,-25.4780172545417,
0.));
#80870=CARTESIAN_POINT('Ctrl Pts',(-66.4630960167252,-25.4921085812547,
0.));
#80871=CARTESIAN_POINT('Ctrl Pts',(-66.4804784439148,-25.5062466667702,
0.));
#80872=CARTESIAN_POINT('Ctrl Pts',(-66.4978823598354,-25.5204314764033,
0.));
#80873=CARTESIAN_POINT('Ctrl Pts',(-66.5153076112231,-25.534662975532,0.));
#80874=CARTESIAN_POINT('Ctrl Pts',(-66.5327540455624,-25.5489411295912,
0.));
#80875=CARTESIAN_POINT('Ctrl Pts',(-66.5502215110829,-25.5632659040792,
0.));
#80876=CARTESIAN_POINT('Ctrl Pts',(-66.5677098567542,-25.5776372645601,
0.));
#80877=CARTESIAN_POINT('Ctrl Pts',(-66.5852189322813,-25.5920551766629,
0.));
#80878=CARTESIAN_POINT('Ctrl Pts',(-66.6027485880963,-25.6065196060756,
0.));
#80879=CARTESIAN_POINT('Ctrl Pts',(-66.6202986753506,-25.6210305185403,
0.));
#80880=CARTESIAN_POINT('Ctrl Pts',(-66.6378690459129,-25.6355878798614,
0.));
#80881=CARTESIAN_POINT('Ctrl Pts',(-66.6554595523624,-25.6501916559055,
0.));
#80882=CARTESIAN_POINT('Ctrl Pts',(-66.6730700479837,-25.6648418126013,
0.));
#80883=CARTESIAN_POINT('Ctrl Pts',(-66.6907003867572,-25.6795383159319,
0.));
#80884=CARTESIAN_POINT('Ctrl Pts',(-66.7083504233529,-25.6942811319322,
0.));
#80885=CARTESIAN_POINT('Ctrl Pts',(-66.7260200131266,-25.7090702266963,
0.));
#80886=CARTESIAN_POINT('Ctrl Pts',(-66.7437090121153,-25.7239055663772,
0.));
#80887=CARTESIAN_POINT('Ctrl Pts',(-66.7614172770316,-25.7387871171866,
0.));
#80888=CARTESIAN_POINT('Ctrl Pts',(-66.7791446652545,-25.7537148453864,
0.));
#80889=CARTESIAN_POINT('Ctrl Pts',(-66.7968910348245,-25.7686887172878,
0.));
#80890=CARTESIAN_POINT('Ctrl Pts',(-66.8146562444433,-25.7837086992595,
0.));
#80891=CARTESIAN_POINT('Ctrl Pts',(-66.8324401534668,-25.7987747577269,
0.));
#80892=CARTESIAN_POINT('Ctrl Pts',(-66.8502426219001,-25.8138868591709,
0.));
#80893=CARTESIAN_POINT('Ctrl Pts',(-66.8680635103876,-25.8290449701193,
0.));
#80894=CARTESIAN_POINT('Ctrl Pts',(-66.8859026802088,-25.844249057147,0.));
#80895=CARTESIAN_POINT('Ctrl Pts',(-66.9037599932761,-25.8594990868833,
0.));
#80896=CARTESIAN_POINT('Ctrl Pts',(-66.92163531213,-25.8747950260111,0.));
#80897=CARTESIAN_POINT('Ctrl Pts',(-66.939528499934,-25.890136841266,0.));
#80898=CARTESIAN_POINT('Ctrl Pts',(-66.9574394204663,-25.9055244994277,
0.));
#80899=CARTESIAN_POINT('Ctrl Pts',(-66.975367938115,-25.9209579673209,0.));
#80900=CARTESIAN_POINT('Ctrl Pts',(-66.9933139178778,-25.9364372118222,
0.));
#80901=CARTESIAN_POINT('Ctrl Pts',(-67.0112772253556,-25.9519621998598,
0.));
#80902=CARTESIAN_POINT('Ctrl Pts',(-67.0292577267489,-25.967532898412,0.));
#80903=CARTESIAN_POINT('Ctrl Pts',(-67.0472552888485,-25.9831492744984,
0.));
#80904=CARTESIAN_POINT('Ctrl Pts',(-67.0652697790325,-25.9988112951814,
0.));
#80905=CARTESIAN_POINT('Ctrl Pts',(-67.0833010652634,-26.014518927573,0.));
#80906=CARTESIAN_POINT('Ctrl Pts',(-67.101349016084,-26.030272138834,0.));
#80907=CARTESIAN_POINT('Ctrl Pts',(-67.1194135006124,-26.0460708961725,
0.));
#80908=CARTESIAN_POINT('Ctrl Pts',(-67.1374943885354,-26.061915166836,0.));
#80909=CARTESIAN_POINT('Ctrl Pts',(-67.1555915501049,-26.0778049181128,
0.));
#80910=CARTESIAN_POINT('Ctrl Pts',(-67.173704856136,-26.0937401173383,0.));
#80911=CARTESIAN_POINT('Ctrl Pts',(-67.1918341780018,-26.1097207318949,
0.));
#80912=CARTESIAN_POINT('Ctrl Pts',(-67.2099793876297,-26.1257467292102,
0.));
#80913=CARTESIAN_POINT('Ctrl Pts',(-67.2281403574938,-26.1418180767489,
0.));
#80914=CARTESIAN_POINT('Ctrl Pts',(-67.2463169606115,-26.1579347420138,
0.));
#80915=CARTESIAN_POINT('Ctrl Pts',(-67.2645090705421,-26.1740966925529,
0.));
#80916=CARTESIAN_POINT('Ctrl Pts',(-67.282716561383,-26.1903038959589,0.));
#80917=CARTESIAN_POINT('Ctrl Pts',(-67.3009393077651,-26.2065563198683,
0.));
#80918=CARTESIAN_POINT('Ctrl Pts',(-67.3191771848463,-26.2228539319526,
0.));
#80919=CARTESIAN_POINT('Ctrl Pts',(-67.3374300683073,-26.2391966999191,
0.));
#80920=CARTESIAN_POINT('Ctrl Pts',(-67.3556978343507,-26.255584591518,0.));
#80921=CARTESIAN_POINT('Ctrl Pts',(-67.3739803596969,-26.2720175745423,
0.));
#80922=CARTESIAN_POINT('Ctrl Pts',(-67.392277521581,-26.288495616827,0.));
#80923=CARTESIAN_POINT('Ctrl Pts',(-67.4105891977461,-26.3050186862407,
0.));
#80924=CARTESIAN_POINT('Ctrl Pts',(-67.4289152664398,-26.321586750686,0.));
#80925=CARTESIAN_POINT('Ctrl Pts',(-67.4472556064119,-26.3381997781055,
0.));
#80926=CARTESIAN_POINT('Ctrl Pts',(-67.4656100969116,-26.3548577364833,
0.));
#80927=CARTESIAN_POINT('Ctrl Pts',(-67.4839786176836,-26.3715605938433,
0.));
#80928=CARTESIAN_POINT('Ctrl Pts',(-67.5023610489622,-26.3883083182421,
0.));
#80929=CARTESIAN_POINT('Ctrl Pts',(-67.5207572714683,-26.4051008777675,
0.));
#80930=CARTESIAN_POINT('Ctrl Pts',(-67.5391671664072,-26.4219382405458,
0.));
#80931=CARTESIAN_POINT('Ctrl Pts',(-67.5575906154657,-26.4388203747425,
0.));
#80932=CARTESIAN_POINT('Ctrl Pts',(-67.5760275008093,-26.4557472485621,
0.));
#80933=CARTESIAN_POINT('Ctrl Pts',(-67.5944777050768,-26.4727188302409,
0.));
#80934=CARTESIAN_POINT('Ctrl Pts',(-67.6129411113757,-26.489735088044,0.));
#80935=CARTESIAN_POINT('Ctrl Pts',(-67.6314176032811,-26.5067959902725,
0.));
#80936=CARTESIAN_POINT('Ctrl Pts',(-67.649907064832,-26.5239015052654,0.));
#80937=CARTESIAN_POINT('Ctrl Pts',(-67.6684093805291,-26.5410516013985,
0.));
#80938=CARTESIAN_POINT('Ctrl Pts',(-67.6869244353294,-26.5582462470794,
0.));
#80939=CARTESIAN_POINT('Ctrl Pts',(-67.7054521146424,-26.5754854107421,
0.));
#80940=CARTESIAN_POINT('Ctrl Pts',(-67.7239923043288,-26.5927690608544,
0.));
#80941=CARTESIAN_POINT('Ctrl Pts',(-67.7425448906977,-26.6100971659202,
0.));
#80942=CARTESIAN_POINT('Ctrl Pts',(-67.7611097605042,-26.6274696944793,
0.));
#80943=CARTESIAN_POINT('Ctrl Pts',(-67.7796868009455,-26.6448866151029,
0.));
#80944=CARTESIAN_POINT('Ctrl Pts',(-67.798275899657,-26.6623478963871,0.));
#80945=CARTESIAN_POINT('Ctrl Pts',(-67.8168769447098,-26.6798535069589,
0.));
#80946=CARTESIAN_POINT('Ctrl Pts',(-67.8354898246086,-26.6974034154804,
0.));
#80947=CARTESIAN_POINT('Ctrl Pts',(-67.8541144282875,-26.7149975906478,
0.));
#80948=CARTESIAN_POINT('Ctrl Pts',(-67.8727506451063,-26.7326360011885,
0.));
#80949=CARTESIAN_POINT('Ctrl Pts',(-67.8913983648436,-26.7503186158522,
0.));
#80950=CARTESIAN_POINT('Ctrl Pts',(-67.9100574776972,-26.7680454034169,
0.));
#80951=CARTESIAN_POINT('Ctrl Pts',(-67.928727874284,-26.7858163326934,0.));
#80952=CARTESIAN_POINT('Ctrl Pts',(-67.9474094456396,-26.8036313725262,
0.));
#80953=CARTESIAN_POINT('Ctrl Pts',(-67.9661020832164,-26.821490491792,0.));
#80954=CARTESIAN_POINT('Ctrl Pts',(-67.9848056788809,-26.8393936593911,
0.));
#80955=CARTESIAN_POINT('Ctrl Pts',(-68.0035201249102,-26.8573408442496,
0.));
#80956=CARTESIAN_POINT('Ctrl Pts',(-68.0222453139856,-26.8753320153252,
0.));
#80957=CARTESIAN_POINT('Ctrl Pts',(-68.0409811391869,-26.8933671416063,
0.));
#80958=CARTESIAN_POINT('Ctrl Pts',(-68.0597274939859,-26.911446192111,0.));
#80959=CARTESIAN_POINT('Ctrl Pts',(-68.0784842722369,-26.9295691358779,
0.));
#80960=CARTESIAN_POINT('Ctrl Pts',(-68.0972513681751,-26.9477359419652,
0.));
#80961=CARTESIAN_POINT('Ctrl Pts',(-68.1160286764255,-26.9659465794601,
0.));
#80962=CARTESIAN_POINT('Ctrl Pts',(-68.1348160920106,-26.9842010174822,
0.));
#80963=CARTESIAN_POINT('Ctrl Pts',(-68.1536135103557,-27.0024992251838,
0.));
#80964=CARTESIAN_POINT('Ctrl Pts',(-68.1724208272958,-27.0208411717472,
0.));
#80965=CARTESIAN_POINT('Ctrl Pts',(-68.1912379390773,-27.0392268263798,
0.));
#80966=CARTESIAN_POINT('Ctrl Pts',(-68.2100647423332,-27.0576561583172,
0.));
#80967=CARTESIAN_POINT('Ctrl Pts',(-68.2289011340615,-27.0761291368226,
0.));
#80968=CARTESIAN_POINT('Ctrl Pts',(-68.2477470116012,-27.0946457311813,
0.));
#80969=CARTESIAN_POINT('Ctrl Pts',(-68.2666022726104,-27.1132059106943,
0.));
#80970=CARTESIAN_POINT('Ctrl Pts',(-68.2854668150364,-27.1318096446649,
0.));
#80971=CARTESIAN_POINT('Ctrl Pts',(-68.3043405371603,-27.1504569024136,
0.));
#80972=CARTESIAN_POINT('Ctrl Pts',(-68.3232233376425,-27.1691476532921,
0.));
#80973=CARTESIAN_POINT('Ctrl Pts',(-68.3421151155711,-27.1878818666926,
0.));
#80974=CARTESIAN_POINT('Ctrl Pts',(-68.3610157704994,-27.2066595120542,
0.));
#80975=CARTESIAN_POINT('Ctrl Pts',(-68.3799252025102,-27.2254805588673,
0.));
#80976=CARTESIAN_POINT('Ctrl Pts',(-68.3988433121581,-27.244344976665,0.));
#80977=CARTESIAN_POINT('Ctrl Pts',(-68.4177700003465,-27.263252735006,0.));
#80978=CARTESIAN_POINT('Ctrl Pts',(-68.4367051682164,-27.2822038034538,
0.));
#80979=CARTESIAN_POINT('Ctrl Pts',(-68.4556487170441,-27.301198151557,0.));
#80980=CARTESIAN_POINT('Ctrl Pts',(-68.4746005480997,-27.3202357488154,
0.));
#80981=CARTESIAN_POINT('Ctrl Pts',(-68.4935605626372,-27.3393165646752,
0.));
#80982=CARTESIAN_POINT('Ctrl Pts',(-68.5125286621902,-27.3584405685947,
0.));
#80983=CARTESIAN_POINT('Ctrl Pts',(-68.5315047488046,-27.3776077300918,
0.));
#80984=CARTESIAN_POINT('Ctrl Pts',(-68.5504887252976,-27.3968180187941,
0.));
#80985=CARTESIAN_POINT('Ctrl Pts',(-68.5694804955002,-27.4160714044825,
0.));
#80986=CARTESIAN_POINT('Ctrl Pts',(-68.5884799645193,-27.4353678571349,
0.));
#80987=CARTESIAN_POINT('Ctrl Pts',(-68.6074870381588,-27.4547073468213,
0.));
#80988=CARTESIAN_POINT('Ctrl Pts',(-68.6265016223536,-27.4740898435977,
0.));
#80989=CARTESIAN_POINT('Ctrl Pts',(-68.6455236225471,-27.4935153173863,
0.));
#80990=CARTESIAN_POINT('Ctrl Pts',(-68.6645529432059,-27.5129837378797,
0.));
#80991=CARTESIAN_POINT('Ctrl Pts',(-68.683589486992,-27.5324950743723,0.));
#80992=CARTESIAN_POINT('Ctrl Pts',(-68.7026331554348,-27.552049295893,0.));
#80993=CARTESIAN_POINT('Ctrl Pts',(-68.721683850427,-27.5716463715027,0.));
#80994=CARTESIAN_POINT('Ctrl Pts',(-68.7407414755291,-27.5912862705482,
0.));
#80995=CARTESIAN_POINT('Ctrl Pts',(-68.7598059372121,-27.6109689629025,
0.));
#80996=CARTESIAN_POINT('Ctrl Pts',(-68.7788771464655,-27.6306944192711,
0.));
#80997=CARTESIAN_POINT('Ctrl Pts',(-68.7979550191773,-27.6504626112621,
0.));
#80998=CARTESIAN_POINT('Ctrl Pts',(-68.8143140938751,-27.667444390988,0.));
#80999=CARTESIAN_POINT('Ctrl Pts',(-68.8268597851977,-27.6804870323282,
0.));
#81000=CARTESIAN_POINT('Ctrl Pts',(-68.8355891981871,-27.6895716271078,
0.));
#81001=CARTESIAN_POINT('Ctrl Pts',(-68.8405004465887,-27.6946856803474,
0.));
#81002=CARTESIAN_POINT('Ctrl Pts',(-68.8415926174765,-27.6958230984748,
0.));
#81003=CARTESIAN_POINT('',(-65.4815644032299,-24.7419628022042,12.));
#81004=CARTESIAN_POINT('',(-65.4815644032299,-24.7419628022042,0.));
#81005=CARTESIAN_POINT('Ctrl Pts',(-68.8415926174765,-27.6958230984748,
12.));
#81006=CARTESIAN_POINT('Ctrl Pts',(-68.8405004465887,-27.6946856803474,
12.));
#81007=CARTESIAN_POINT('Ctrl Pts',(-68.8355891981871,-27.6895716271078,
12.));
#81008=CARTESIAN_POINT('Ctrl Pts',(-68.8268597851977,-27.6804870323282,
12.));
#81009=CARTESIAN_POINT('Ctrl Pts',(-68.8143140938751,-27.667444390988,12.));
#81010=CARTESIAN_POINT('Ctrl Pts',(-68.7979550191773,-27.6504626112621,
12.));
#81011=CARTESIAN_POINT('Ctrl Pts',(-68.7788771464655,-27.6306944192711,
12.));
#81012=CARTESIAN_POINT('Ctrl Pts',(-68.7598059372121,-27.6109689629025,
12.));
#81013=CARTESIAN_POINT('Ctrl Pts',(-68.7407414755291,-27.5912862705482,
12.));
#81014=CARTESIAN_POINT('Ctrl Pts',(-68.721683850427,-27.5716463715027,12.));
#81015=CARTESIAN_POINT('Ctrl Pts',(-68.7026331554348,-27.552049295893,12.));
#81016=CARTESIAN_POINT('Ctrl Pts',(-68.683589486992,-27.5324950743723,12.));
#81017=CARTESIAN_POINT('Ctrl Pts',(-68.6645529432059,-27.5129837378797,
12.));
#81018=CARTESIAN_POINT('Ctrl Pts',(-68.6455236225471,-27.4935153173863,
12.));
#81019=CARTESIAN_POINT('Ctrl Pts',(-68.6265016223536,-27.4740898435977,
12.));
#81020=CARTESIAN_POINT('Ctrl Pts',(-68.6074870381588,-27.4547073468213,
12.));
#81021=CARTESIAN_POINT('Ctrl Pts',(-68.5884799645193,-27.4353678571349,
12.));
#81022=CARTESIAN_POINT('Ctrl Pts',(-68.5694804955002,-27.4160714044825,
12.));
#81023=CARTESIAN_POINT('Ctrl Pts',(-68.5504887252976,-27.3968180187941,
12.));
#81024=CARTESIAN_POINT('Ctrl Pts',(-68.5315047488046,-27.3776077300918,
12.));
#81025=CARTESIAN_POINT('Ctrl Pts',(-68.5125286621902,-27.3584405685947,
12.));
#81026=CARTESIAN_POINT('Ctrl Pts',(-68.4935605626372,-27.3393165646752,
12.));
#81027=CARTESIAN_POINT('Ctrl Pts',(-68.4746005480997,-27.3202357488154,
12.));
#81028=CARTESIAN_POINT('Ctrl Pts',(-68.4556487170441,-27.301198151557,12.));
#81029=CARTESIAN_POINT('Ctrl Pts',(-68.4367051682164,-27.2822038034538,
12.));
#81030=CARTESIAN_POINT('Ctrl Pts',(-68.4177700003465,-27.263252735006,12.));
#81031=CARTESIAN_POINT('Ctrl Pts',(-68.3988433121581,-27.244344976665,12.));
#81032=CARTESIAN_POINT('Ctrl Pts',(-68.3799252025102,-27.2254805588673,
12.));
#81033=CARTESIAN_POINT('Ctrl Pts',(-68.3610157704994,-27.2066595120542,
12.));
#81034=CARTESIAN_POINT('Ctrl Pts',(-68.3421151155711,-27.1878818666926,
12.));
#81035=CARTESIAN_POINT('Ctrl Pts',(-68.3232233376425,-27.1691476532921,
12.));
#81036=CARTESIAN_POINT('Ctrl Pts',(-68.3043405371603,-27.1504569024136,
12.));
#81037=CARTESIAN_POINT('Ctrl Pts',(-68.2854668150364,-27.1318096446649,
12.));
#81038=CARTESIAN_POINT('Ctrl Pts',(-68.2666022726104,-27.1132059106943,
12.));
#81039=CARTESIAN_POINT('Ctrl Pts',(-68.2477470116012,-27.0946457311813,
12.));
#81040=CARTESIAN_POINT('Ctrl Pts',(-68.2289011340615,-27.0761291368226,
12.));
#81041=CARTESIAN_POINT('Ctrl Pts',(-68.2100647423332,-27.0576561583172,
12.));
#81042=CARTESIAN_POINT('Ctrl Pts',(-68.1912379390773,-27.0392268263798,
12.));
#81043=CARTESIAN_POINT('Ctrl Pts',(-68.1724208272958,-27.0208411717472,
12.));
#81044=CARTESIAN_POINT('Ctrl Pts',(-68.1536135103557,-27.0024992251838,
12.));
#81045=CARTESIAN_POINT('Ctrl Pts',(-68.1348160920106,-26.9842010174822,
12.));
#81046=CARTESIAN_POINT('Ctrl Pts',(-68.1160286764255,-26.9659465794601,
12.));
#81047=CARTESIAN_POINT('Ctrl Pts',(-68.0972513681751,-26.9477359419652,
12.));
#81048=CARTESIAN_POINT('Ctrl Pts',(-68.0784842722369,-26.9295691358779,
12.));
#81049=CARTESIAN_POINT('Ctrl Pts',(-68.0597274939859,-26.911446192111,12.));
#81050=CARTESIAN_POINT('Ctrl Pts',(-68.0409811391869,-26.8933671416063,
12.));
#81051=CARTESIAN_POINT('Ctrl Pts',(-68.0222453139856,-26.8753320153252,
12.));
#81052=CARTESIAN_POINT('Ctrl Pts',(-68.0035201249102,-26.8573408442496,
12.));
#81053=CARTESIAN_POINT('Ctrl Pts',(-67.9848056788809,-26.8393936593911,
12.));
#81054=CARTESIAN_POINT('Ctrl Pts',(-67.9661020832164,-26.821490491792,12.));
#81055=CARTESIAN_POINT('Ctrl Pts',(-67.9474094456396,-26.8036313725262,
12.));
#81056=CARTESIAN_POINT('Ctrl Pts',(-67.928727874284,-26.7858163326934,12.));
#81057=CARTESIAN_POINT('Ctrl Pts',(-67.9100574776972,-26.7680454034169,
12.));
#81058=CARTESIAN_POINT('Ctrl Pts',(-67.8913983648436,-26.7503186158522,
12.));
#81059=CARTESIAN_POINT('Ctrl Pts',(-67.8727506451063,-26.7326360011885,
12.));
#81060=CARTESIAN_POINT('Ctrl Pts',(-67.8541144282875,-26.7149975906478,
12.));
#81061=CARTESIAN_POINT('Ctrl Pts',(-67.8354898246086,-26.6974034154804,
12.));
#81062=CARTESIAN_POINT('Ctrl Pts',(-67.8168769447098,-26.6798535069589,
12.));
#81063=CARTESIAN_POINT('Ctrl Pts',(-67.798275899657,-26.6623478963871,12.));
#81064=CARTESIAN_POINT('Ctrl Pts',(-67.7796868009455,-26.6448866151029,
12.));
#81065=CARTESIAN_POINT('Ctrl Pts',(-67.7611097605042,-26.6274696944793,
12.));
#81066=CARTESIAN_POINT('Ctrl Pts',(-67.7425448906977,-26.6100971659202,
12.));
#81067=CARTESIAN_POINT('Ctrl Pts',(-67.7239923043288,-26.5927690608544,
12.));
#81068=CARTESIAN_POINT('Ctrl Pts',(-67.7054521146424,-26.5754854107421,
12.));
#81069=CARTESIAN_POINT('Ctrl Pts',(-67.6869244353294,-26.5582462470794,
12.));
#81070=CARTESIAN_POINT('Ctrl Pts',(-67.6684093805291,-26.5410516013985,
12.));
#81071=CARTESIAN_POINT('Ctrl Pts',(-67.649907064832,-26.5239015052654,12.));
#81072=CARTESIAN_POINT('Ctrl Pts',(-67.6314176032811,-26.5067959902725,
12.));
#81073=CARTESIAN_POINT('Ctrl Pts',(-67.6129411113757,-26.489735088044,12.));
#81074=CARTESIAN_POINT('Ctrl Pts',(-67.5944777050768,-26.4727188302409,
12.));
#81075=CARTESIAN_POINT('Ctrl Pts',(-67.5760275008093,-26.4557472485621,
12.));
#81076=CARTESIAN_POINT('Ctrl Pts',(-67.5575906154657,-26.4388203747425,
12.));
#81077=CARTESIAN_POINT('Ctrl Pts',(-67.5391671664072,-26.4219382405458,
12.));
#81078=CARTESIAN_POINT('Ctrl Pts',(-67.5207572714683,-26.4051008777675,
12.));
#81079=CARTESIAN_POINT('Ctrl Pts',(-67.5023610489622,-26.3883083182421,
12.));
#81080=CARTESIAN_POINT('Ctrl Pts',(-67.4839786176836,-26.3715605938433,
12.));
#81081=CARTESIAN_POINT('Ctrl Pts',(-67.4656100969116,-26.3548577364833,
12.));
#81082=CARTESIAN_POINT('Ctrl Pts',(-67.4472556064119,-26.3381997781055,
12.));
#81083=CARTESIAN_POINT('Ctrl Pts',(-67.4289152664398,-26.321586750686,12.));
#81084=CARTESIAN_POINT('Ctrl Pts',(-67.4105891977461,-26.3050186862407,
12.));
#81085=CARTESIAN_POINT('Ctrl Pts',(-67.392277521581,-26.288495616827,12.));
#81086=CARTESIAN_POINT('Ctrl Pts',(-67.3739803596969,-26.2720175745423,
12.));
#81087=CARTESIAN_POINT('Ctrl Pts',(-67.3556978343507,-26.255584591518,12.));
#81088=CARTESIAN_POINT('Ctrl Pts',(-67.3374300683073,-26.2391966999191,
12.));
#81089=CARTESIAN_POINT('Ctrl Pts',(-67.3191771848463,-26.2228539319526,
12.));
#81090=CARTESIAN_POINT('Ctrl Pts',(-67.3009393077651,-26.2065563198683,
12.));
#81091=CARTESIAN_POINT('Ctrl Pts',(-67.282716561383,-26.1903038959589,12.));
#81092=CARTESIAN_POINT('Ctrl Pts',(-67.2645090705421,-26.1740966925529,
12.));
#81093=CARTESIAN_POINT('Ctrl Pts',(-67.2463169606115,-26.1579347420138,
12.));
#81094=CARTESIAN_POINT('Ctrl Pts',(-67.2281403574938,-26.1418180767489,
12.));
#81095=CARTESIAN_POINT('Ctrl Pts',(-67.2099793876297,-26.1257467292102,
12.));
#81096=CARTESIAN_POINT('Ctrl Pts',(-67.1918341780018,-26.1097207318949,
12.));
#81097=CARTESIAN_POINT('Ctrl Pts',(-67.173704856136,-26.0937401173383,12.));
#81098=CARTESIAN_POINT('Ctrl Pts',(-67.1555915501049,-26.0778049181128,
12.));
#81099=CARTESIAN_POINT('Ctrl Pts',(-67.1374943885354,-26.061915166836,12.));
#81100=CARTESIAN_POINT('Ctrl Pts',(-67.1194135006124,-26.0460708961725,
12.));
#81101=CARTESIAN_POINT('Ctrl Pts',(-67.101349016084,-26.030272138834,12.));
#81102=CARTESIAN_POINT('Ctrl Pts',(-67.0833010652634,-26.014518927573,12.));
#81103=CARTESIAN_POINT('Ctrl Pts',(-67.0652697790325,-25.9988112951814,
12.));
#81104=CARTESIAN_POINT('Ctrl Pts',(-67.0472552888485,-25.9831492744984,
12.));
#81105=CARTESIAN_POINT('Ctrl Pts',(-67.0292577267489,-25.967532898412,12.));
#81106=CARTESIAN_POINT('Ctrl Pts',(-67.0112772253556,-25.9519621998598,
12.));
#81107=CARTESIAN_POINT('Ctrl Pts',(-66.9933139178778,-25.9364372118222,
12.));
#81108=CARTESIAN_POINT('Ctrl Pts',(-66.975367938115,-25.9209579673209,12.));
#81109=CARTESIAN_POINT('Ctrl Pts',(-66.9574394204663,-25.9055244994277,
12.));
#81110=CARTESIAN_POINT('Ctrl Pts',(-66.939528499934,-25.890136841266,12.));
#81111=CARTESIAN_POINT('Ctrl Pts',(-66.92163531213,-25.8747950260111,12.));
#81112=CARTESIAN_POINT('Ctrl Pts',(-66.9037599932761,-25.8594990868833,
12.));
#81113=CARTESIAN_POINT('Ctrl Pts',(-66.8859026802088,-25.844249057147,12.));
#81114=CARTESIAN_POINT('Ctrl Pts',(-66.8680635103876,-25.8290449701193,
12.));
#81115=CARTESIAN_POINT('Ctrl Pts',(-66.8502426219001,-25.8138868591709,
12.));
#81116=CARTESIAN_POINT('Ctrl Pts',(-66.8324401534668,-25.7987747577269,
12.));
#81117=CARTESIAN_POINT('Ctrl Pts',(-66.8146562444433,-25.7837086992595,
12.));
#81118=CARTESIAN_POINT('Ctrl Pts',(-66.7968910348245,-25.7686887172878,
12.));
#81119=CARTESIAN_POINT('Ctrl Pts',(-66.7791446652545,-25.7537148453864,
12.));
#81120=CARTESIAN_POINT('Ctrl Pts',(-66.7614172770316,-25.7387871171866,
12.));
#81121=CARTESIAN_POINT('Ctrl Pts',(-66.7437090121153,-25.7239055663772,
12.));
#81122=CARTESIAN_POINT('Ctrl Pts',(-66.7260200131266,-25.7090702266963,
12.));
#81123=CARTESIAN_POINT('Ctrl Pts',(-66.7083504233529,-25.6942811319322,
12.));
#81124=CARTESIAN_POINT('Ctrl Pts',(-66.6907003867572,-25.6795383159319,
12.));
#81125=CARTESIAN_POINT('Ctrl Pts',(-66.6730700479837,-25.6648418126013,
12.));
#81126=CARTESIAN_POINT('Ctrl Pts',(-66.6554595523624,-25.6501916559055,
12.));
#81127=CARTESIAN_POINT('Ctrl Pts',(-66.6378690459129,-25.6355878798614,
12.));
#81128=CARTESIAN_POINT('Ctrl Pts',(-66.6202986753506,-25.6210305185403,
12.));
#81129=CARTESIAN_POINT('Ctrl Pts',(-66.6027485880963,-25.6065196060756,
12.));
#81130=CARTESIAN_POINT('Ctrl Pts',(-66.5852189322813,-25.5920551766629,
12.));
#81131=CARTESIAN_POINT('Ctrl Pts',(-66.5677098567542,-25.5776372645601,
12.));
#81132=CARTESIAN_POINT('Ctrl Pts',(-66.5502215110829,-25.5632659040792,
12.));
#81133=CARTESIAN_POINT('Ctrl Pts',(-66.5327540455624,-25.5489411295912,
12.));
#81134=CARTESIAN_POINT('Ctrl Pts',(-66.5153076112231,-25.534662975532,12.));
#81135=CARTESIAN_POINT('Ctrl Pts',(-66.4978823598354,-25.5204314764033,
12.));
#81136=CARTESIAN_POINT('Ctrl Pts',(-66.4804784439148,-25.5062466667702,
12.));
#81137=CARTESIAN_POINT('Ctrl Pts',(-66.4630960167252,-25.4921085812547,
12.));
#81138=CARTESIAN_POINT('Ctrl Pts',(-66.4457352322871,-25.4780172545417,
12.));
#81139=CARTESIAN_POINT('Ctrl Pts',(-66.4283962453899,-25.4639727213849,
12.));
#81140=CARTESIAN_POINT('Ctrl Pts',(-66.4110792116,-25.4499750166079,12.));
#81141=CARTESIAN_POINT('Ctrl Pts',(-66.3937842872685,-25.4360241751018,
12.));
#81142=CARTESIAN_POINT('Ctrl Pts',(-66.3765116295364,-25.4221202318199,
12.));
#81143=CARTESIAN_POINT('Ctrl Pts',(-66.359261396341,-25.4082632217847,12.));
#81144=CARTESIAN_POINT('Ctrl Pts',(-66.3420337464178,-25.3944531800901,
12.));
#81145=CARTESIAN_POINT('Ctrl Pts',(-66.3248288393046,-25.3806901419012,
12.));
#81146=CARTESIAN_POINT('Ctrl Pts',(-66.3076468353412,-25.3669741424488,
12.));
#81147=CARTESIAN_POINT('Ctrl Pts',(-66.290487895671,-25.3533052170249,12.));
#81148=CARTESIAN_POINT('Ctrl Pts',(-66.2733521822662,-25.3396834009949,
12.));
#81149=CARTESIAN_POINT('Ctrl Pts',(-66.2562398579471,-25.3261087298026,
12.));
#81150=CARTESIAN_POINT('Ctrl Pts',(-66.2391510863998,-25.312581238973,12.));
#81151=CARTESIAN_POINT('Ctrl Pts',(-66.2220860321952,-25.2991009641094,
12.));
#81152=CARTESIAN_POINT('Ctrl Pts',(-66.2050448607911,-25.285667940893,12.));
#81153=CARTESIAN_POINT('Ctrl Pts',(-66.1880277385136,-25.2722822050837,
12.));
#81154=CARTESIAN_POINT('Ctrl Pts',(-66.1710348325384,-25.2589437925147,
12.));
#81155=CARTESIAN_POINT('Ctrl Pts',(-66.1540663108754,-25.2456527390875,
12.));
#81156=CARTESIAN_POINT('Ctrl Pts',(-66.1371223423345,-25.232409080755,12.));
#81157=CARTESIAN_POINT('Ctrl Pts',(-66.1202030965758,-25.2192128535357,
12.));
#81158=CARTESIAN_POINT('Ctrl Pts',(-66.10330874419,-25.2060640935365,12.));
#81159=CARTESIAN_POINT('Ctrl Pts',(-66.086439456768,-25.1929628369685,12.));
#81160=CARTESIAN_POINT('Ctrl Pts',(-66.0695954069713,-25.1799091201599,
12.));
#81161=CARTESIAN_POINT('Ctrl Pts',(-66.0527767686025,-25.1669029795661,
12.));
#81162=CARTESIAN_POINT('Ctrl Pts',(-66.0359837164734,-25.1539444517419,
12.));
#81163=CARTESIAN_POINT('Ctrl Pts',(-66.0192164262621,-25.1410335733099,
12.));
#81164=CARTESIAN_POINT('Ctrl Pts',(-66.0024750743897,-25.1281703809297,
12.));
#81165=CARTESIAN_POINT('Ctrl Pts',(-65.9857598378433,-25.1153549112503,
12.));
#81166=CARTESIAN_POINT('Ctrl Pts',(-65.9690708941558,-25.1025872009004,
12.));
#81167=CARTESIAN_POINT('Ctrl Pts',(-65.9524084218139,-25.0898672865915,
12.));
#81168=CARTESIAN_POINT('Ctrl Pts',(-65.9357726006163,-25.0771952052028,
12.));
#81169=CARTESIAN_POINT('Ctrl Pts',(-65.919163611981,-25.0645709938524,12.));
#81170=CARTESIAN_POINT('Ctrl Pts',(-65.9025816394424,-25.0519946900078,
12.));
#81171=CARTESIAN_POINT('Ctrl Pts',(-65.8860268683128,-25.0394663314055,
12.));
#81172=CARTESIAN_POINT('Ctrl Pts',(-65.8694994847616,-25.0269859558362,
12.));
#81173=CARTESIAN_POINT('Ctrl Pts',(-65.8529996750445,-25.0145536009604,
12.));
#81174=CARTESIAN_POINT('Ctrl Pts',(-65.8365276247128,-25.002169304117,12.));
#81175=CARTESIAN_POINT('Ctrl Pts',(-65.8200835177024,-24.9898331020983,
12.));
#81176=CARTESIAN_POINT('Ctrl Pts',(-65.8036675380718,-24.9775450315682,
12.));
#81177=CARTESIAN_POINT('Ctrl Pts',(-65.7872798720823,-24.9653051295581,
12.));
#81178=CARTESIAN_POINT('Ctrl Pts',(-65.7709207098959,-24.9531134338696,
12.));
#81179=CARTESIAN_POINT('Ctrl Pts',(-65.7545902480323,-24.9409699836537,
12.));
#81180=CARTESIAN_POINT('Ctrl Pts',(-65.7382886895888,-24.928874819458,12.));
#81181=CARTESIAN_POINT('Ctrl Pts',(-65.7220162391054,-24.9168279820106,
12.));
#81182=CARTESIAN_POINT('Ctrl Pts',(-65.7057730980483,-24.9048295111448,
12.));
#81183=CARTESIAN_POINT('Ctrl Pts',(-65.6895594608775,-24.8928794448607,
12.));
#81184=CARTESIAN_POINT('Ctrl Pts',(-65.6733755087669,-24.8809778178229,
12.));
#81185=CARTESIAN_POINT('Ctrl Pts',(-65.6572214156692,-24.8691246628057,
12.));
#81186=CARTESIAN_POINT('Ctrl Pts',(-65.6410973603661,-24.8573200135666,
12.));
#81187=CARTESIAN_POINT('Ctrl Pts',(-65.6250035361612,-24.8455639071517,
12.));
#81188=CARTESIAN_POINT('Ctrl Pts',(-65.6089401625628,-24.8338563866764,
12.));
#81189=CARTESIAN_POINT('Ctrl Pts',(-65.5929074932624,-24.8221975032104,
12.));
#81190=CARTESIAN_POINT('Ctrl Pts',(-65.5769057914333,-24.8105873098626,
12.));
#81191=CARTESIAN_POINT('Ctrl Pts',(-65.5609353062829,-24.799025856126,12.));
#81192=CARTESIAN_POINT('Ctrl Pts',(-65.5449962514661,-24.787513182749,12.));
#81193=CARTESIAN_POINT('Ctrl Pts',(-65.5290887770232,-24.7760493148465,
12.));
#81194=CARTESIAN_POINT('Ctrl Pts',(-65.5132129675333,-24.7646342620841,
12.));
#81195=CARTESIAN_POINT('Ctrl Pts',(-65.5005376841101,-24.7555412724651,
12.));
#81196=CARTESIAN_POINT('Ctrl Pts',(-65.4910454936254,-24.7487434955982,
12.));
#81197=CARTESIAN_POINT('Ctrl Pts',(-65.4847237095443,-24.7442214063382,
12.));
#81198=CARTESIAN_POINT('Ctrl Pts',(-65.4815644032299,-24.7419628022042,
12.));
#81199=CARTESIAN_POINT('Ctrl Pts',(-68.2622612910177,-29.0944526440266,
-5.55111512312578E-16));
#81200=CARTESIAN_POINT('Ctrl Pts',(-68.2622612910177,-29.0944526440266,
4.));
#81201=CARTESIAN_POINT('Ctrl Pts',(-68.2622612910177,-29.0944526440266,
8.));
#81202=CARTESIAN_POINT('Ctrl Pts',(-68.2622612910177,-29.0944526440266,
12.));
#81203=CARTESIAN_POINT('Ctrl Pts',(-68.3721211369509,-29.0922231502664,
-5.55111512312578E-16));
#81204=CARTESIAN_POINT('Ctrl Pts',(-68.3721211369509,-29.0922231502664,
3.99999999999999));
#81205=CARTESIAN_POINT('Ctrl Pts',(-68.3721211369508,-29.0922231502664,
8.));
#81206=CARTESIAN_POINT('Ctrl Pts',(-68.3721211369508,-29.0922231502664,
12.));
#81207=CARTESIAN_POINT('Ctrl Pts',(-68.5624216146675,-29.0225207419381,
-5.55111512312578E-16));
#81208=CARTESIAN_POINT('Ctrl Pts',(-68.5624216146675,-29.0225207419381,
4.00000000000001));
#81209=CARTESIAN_POINT('Ctrl Pts',(-68.5624216146675,-29.0225207419382,
7.99999999999999));
#81210=CARTESIAN_POINT('Ctrl Pts',(-68.5624216146675,-29.0225207419382,
12.));
#81211=CARTESIAN_POINT('Ctrl Pts',(-68.6814343344132,-28.8637726134455,
-5.55111512312578E-16));
#81212=CARTESIAN_POINT('Ctrl Pts',(-68.6814343344132,-28.8637726134455,
3.99999999999999));
#81213=CARTESIAN_POINT('Ctrl Pts',(-68.6814343344132,-28.8637726134455,
8.00000000000001));
#81214=CARTESIAN_POINT('Ctrl Pts',(-68.6814343344132,-28.8637726134455,
12.));
#81215=CARTESIAN_POINT('Ctrl Pts',(-68.7132793373319,-28.7877620302417,
-5.55111512312578E-16));
#81216=CARTESIAN_POINT('Ctrl Pts',(-68.7132793373319,-28.7877620302417,
4.));
#81217=CARTESIAN_POINT('Ctrl Pts',(-68.7132793373319,-28.7877620302417,
8.));
#81218=CARTESIAN_POINT('Ctrl Pts',(-68.7132793373319,-28.7877620302417,
12.));
#81219=CARTESIAN_POINT('',(-68.2622612910177,-29.0944526440266,0.));
#81220=CARTESIAN_POINT('',(-68.7132793373317,-28.7877620302417,0.));
#81221=CARTESIAN_POINT('Ctrl Pts',(-68.2622612910177,-29.0944526440266,
2.77555756156289E-16));
#81222=CARTESIAN_POINT('Ctrl Pts',(-68.3721211369509,-29.0922231502664,
2.77555756156288E-16));
#81223=CARTESIAN_POINT('Ctrl Pts',(-68.4808642670747,-29.0523932026502,
2.7755575615629E-16));
#81224=CARTESIAN_POINT('Ctrl Pts',(-68.5663297619426,-28.983487101511,2.77555756156289E-16));
#81225=CARTESIAN_POINT('Ctrl Pts',(-68.6304288830936,-28.9318075256566,
2.77555756156289E-16));
#81226=CARTESIAN_POINT('Ctrl Pts',(-68.6814343344132,-28.8637726134455,
2.77555756156288E-16));
#81227=CARTESIAN_POINT('Ctrl Pts',(-68.7132793373319,-28.7877620302417,
2.77555756156289E-16));
#81228=CARTESIAN_POINT('',(-68.7132793373317,-28.7877620302417,12.));
#81229=CARTESIAN_POINT('Ctrl Pts',(-68.7132793373319,-28.7877620302417,
-5.55111512312578E-16));
#81230=CARTESIAN_POINT('Ctrl Pts',(-68.7132793373319,-28.7877620302417,
4.));
#81231=CARTESIAN_POINT('Ctrl Pts',(-68.7132793373319,-28.7877620302417,
8.));
#81232=CARTESIAN_POINT('Ctrl Pts',(-68.7132793373319,-28.7877620302417,
12.));
#81233=CARTESIAN_POINT('',(-68.2622612910177,-29.0944526440266,12.));
#81234=CARTESIAN_POINT('Ctrl Pts',(-68.7132793373319,-28.7877620302417,
12.));
#81235=CARTESIAN_POINT('Ctrl Pts',(-68.6814343344132,-28.8637726134455,
12.));
#81236=CARTESIAN_POINT('Ctrl Pts',(-68.6304288830936,-28.9318075256567,
12.));
#81237=CARTESIAN_POINT('Ctrl Pts',(-68.5663297619426,-28.983487101511,12.));
#81238=CARTESIAN_POINT('Ctrl Pts',(-68.4808642670747,-29.0523932026502,
12.));
#81239=CARTESIAN_POINT('Ctrl Pts',(-68.3721211369508,-29.0922231502664,
12.));
#81240=CARTESIAN_POINT('Ctrl Pts',(-68.2622612910177,-29.0944526440266,
12.));
#81241=CARTESIAN_POINT('Ctrl Pts',(-68.2622612910177,-29.0944526440266,
12.));
#81242=CARTESIAN_POINT('Ctrl Pts',(-68.2622612910177,-29.0944526440266,
8.));
#81243=CARTESIAN_POINT('Ctrl Pts',(-68.2622612910177,-29.0944526440266,
4.));
#81244=CARTESIAN_POINT('Ctrl Pts',(-68.2622612910177,-29.0944526440266,
-5.55111512312578E-16));
#81245=CARTESIAN_POINT('Origin',(-3.46272497684358E-10,-1.43538201480493E-10,
0.));
#81246=CARTESIAN_POINT('Origin',(-3.46272497684358E-10,-1.43538201480493E-10,
12.));
#81247=CARTESIAN_POINT('Origin',(-3.46272497684358E-10,-1.43538201480493E-10,
0.));
#81248=CARTESIAN_POINT('Ctrl Pts',(-71.1418425484881,-22.1153394458716,
0.));
#81249=CARTESIAN_POINT('Ctrl Pts',(-71.1418425484881,-22.1153394458716,
4.));
#81250=CARTESIAN_POINT('Ctrl Pts',(-71.1418425484881,-22.1153394458716,
8.));
#81251=CARTESIAN_POINT('Ctrl Pts',(-71.1418425484881,-22.1153394458716,
12.));
#81252=CARTESIAN_POINT('Ctrl Pts',(-71.1744611799059,-22.0104100349462,
0.));
#81253=CARTESIAN_POINT('Ctrl Pts',(-71.1744611799059,-22.0104100349462,
4.));
#81254=CARTESIAN_POINT('Ctrl Pts',(-71.1744611799059,-22.0104100349463,
8.));
#81255=CARTESIAN_POINT('Ctrl Pts',(-71.1744611799059,-22.0104100349463,
12.));
#81256=CARTESIAN_POINT('Ctrl Pts',(-71.168501135194,-21.8078334561032,0.));
#81257=CARTESIAN_POINT('Ctrl Pts',(-71.168501135194,-21.8078334561032,4.));
#81258=CARTESIAN_POINT('Ctrl Pts',(-71.168501135194,-21.8078334561032,7.99999999999999));
#81259=CARTESIAN_POINT('Ctrl Pts',(-71.168501135194,-21.8078334561032,12.));
#81260=CARTESIAN_POINT('Ctrl Pts',(-71.0555229320378,-21.6447353227845,
0.));
#81261=CARTESIAN_POINT('Ctrl Pts',(-71.0555229320378,-21.6447353227845,
4.));
#81262=CARTESIAN_POINT('Ctrl Pts',(-71.0555229320377,-21.6447353227846,
8.00000000000001));
#81263=CARTESIAN_POINT('Ctrl Pts',(-71.0555229320377,-21.6447353227846,
12.));
#81264=CARTESIAN_POINT('Ctrl Pts',(-70.9934796068778,-21.5904919934805,
0.));
#81265=CARTESIAN_POINT('Ctrl Pts',(-70.9934796068778,-21.5904919934805,
4.));
#81266=CARTESIAN_POINT('Ctrl Pts',(-70.9934796068777,-21.5904919934805,
8.));
#81267=CARTESIAN_POINT('Ctrl Pts',(-70.9934796068777,-21.5904919934805,
12.));
#81268=CARTESIAN_POINT('',(-71.1418425484881,-22.1153394458716,0.));
#81269=CARTESIAN_POINT('',(-70.993479606878,-21.5904919934802,0.));
#81270=CARTESIAN_POINT('Ctrl Pts',(-71.1418425484881,-22.1153394458716,
0.));
#81271=CARTESIAN_POINT('Ctrl Pts',(-71.1744611799059,-22.0104100349462,
0.));
#81272=CARTESIAN_POINT('Ctrl Pts',(-71.1710554400705,-21.894651989893,0.));
#81273=CARTESIAN_POINT('Ctrl Pts',(-71.132704995437,-21.7917848658274,0.));
#81274=CARTESIAN_POINT('Ctrl Pts',(-71.1039421619619,-21.7146345227782,
0.));
#81275=CARTESIAN_POINT('Ctrl Pts',(-71.0555229320378,-21.6447353227845,
0.));
#81276=CARTESIAN_POINT('Ctrl Pts',(-70.9934796068778,-21.5904919934805,
0.));
#81277=CARTESIAN_POINT('',(-70.993479606878,-21.5904919934802,12.));
#81278=CARTESIAN_POINT('Ctrl Pts',(-70.9934796068778,-21.5904919934805,
0.));
#81279=CARTESIAN_POINT('Ctrl Pts',(-70.9934796068778,-21.5904919934805,
4.));
#81280=CARTESIAN_POINT('Ctrl Pts',(-70.9934796068777,-21.5904919934805,
8.));
#81281=CARTESIAN_POINT('Ctrl Pts',(-70.9934796068777,-21.5904919934805,
12.));
#81282=CARTESIAN_POINT('',(-71.1418425484881,-22.1153394458716,12.));
#81283=CARTESIAN_POINT('Ctrl Pts',(-70.9934796068777,-21.5904919934805,
12.));
#81284=CARTESIAN_POINT('Ctrl Pts',(-71.0555229320377,-21.6447353227846,
12.));
#81285=CARTESIAN_POINT('Ctrl Pts',(-71.1039421619619,-21.7146345227783,
12.));
#81286=CARTESIAN_POINT('Ctrl Pts',(-71.132704995437,-21.7917848658275,12.));
#81287=CARTESIAN_POINT('Ctrl Pts',(-71.1710554400705,-21.8946519898931,
12.));
#81288=CARTESIAN_POINT('Ctrl Pts',(-71.1744611799059,-22.0104100349463,
12.));
#81289=CARTESIAN_POINT('Ctrl Pts',(-71.1418425484881,-22.1153394458716,
12.));
#81290=CARTESIAN_POINT('Ctrl Pts',(-71.1418425484881,-22.1153394458716,
12.));
#81291=CARTESIAN_POINT('Ctrl Pts',(-71.1418425484881,-22.1153394458716,
8.));
#81292=CARTESIAN_POINT('Ctrl Pts',(-71.1418425484881,-22.1153394458716,
4.));
#81293=CARTESIAN_POINT('Ctrl Pts',(-71.1418425484881,-22.1153394458716,
0.));
#81294=CARTESIAN_POINT('Ctrl Pts',(-67.3887914263118,-18.9407177820969,
0.));
#81295=CARTESIAN_POINT('Ctrl Pts',(-67.3887914263118,-18.9407177820969,
12.));
#81296=CARTESIAN_POINT('Ctrl Pts',(-67.3921355608328,-18.9426924398719,
0.));
#81297=CARTESIAN_POINT('Ctrl Pts',(-67.3921355608328,-18.9426924398719,
12.));
#81298=CARTESIAN_POINT('Ctrl Pts',(-67.3988274146651,-18.9466463414299,
0.));
#81299=CARTESIAN_POINT('Ctrl Pts',(-67.3988274146651,-18.9466463414299,
12.));
#81300=CARTESIAN_POINT('Ctrl Pts',(-67.4088759497911,-18.9525909517915,
0.));
#81301=CARTESIAN_POINT('Ctrl Pts',(-67.4088759497911,-18.9525909517915,
12.));
#81302=CARTESIAN_POINT('Ctrl Pts',(-67.4222955061981,-18.9605446160985,
0.));
#81303=CARTESIAN_POINT('Ctrl Pts',(-67.4222955061981,-18.9605446160985,
12.));
#81304=CARTESIAN_POINT('Ctrl Pts',(-67.4391057908418,-18.9705325631711,
0.));
#81305=CARTESIAN_POINT('Ctrl Pts',(-67.4391057908418,-18.9705325631711,
12.));
#81306=CARTESIAN_POINT('Ctrl Pts',(-67.4559518744638,-18.9805663798449,
0.));
#81307=CARTESIAN_POINT('Ctrl Pts',(-67.4559518744638,-18.9805663798449,
12.));
#81308=CARTESIAN_POINT('Ctrl Pts',(-67.472833671964,-18.9906460638625,0.));
#81309=CARTESIAN_POINT('Ctrl Pts',(-67.472833671964,-18.9906460638625,12.));
#81310=CARTESIAN_POINT('Ctrl Pts',(-67.4897510316844,-19.0007716032819,
0.));
#81311=CARTESIAN_POINT('Ctrl Pts',(-67.4897510316844,-19.0007716032819,
12.));
#81312=CARTESIAN_POINT('Ctrl Pts',(-67.5067037372317,-19.0109429761306,
0.));
#81313=CARTESIAN_POINT('Ctrl Pts',(-67.5067037372317,-19.0109429761306,
12.));
#81314=CARTESIAN_POINT('Ctrl Pts',(-67.5236915360331,-19.021160154824,0.));
#81315=CARTESIAN_POINT('Ctrl Pts',(-67.5236915360331,-19.021160154824,12.));
#81316=CARTESIAN_POINT('Ctrl Pts',(-67.540714161288,-19.0314231093923,0.));
#81317=CARTESIAN_POINT('Ctrl Pts',(-67.540714161288,-19.0314231093923,12.));
#81318=CARTESIAN_POINT('Ctrl Pts',(-67.5577713558194,-19.0417318110708,
0.));
#81319=CARTESIAN_POINT('Ctrl Pts',(-67.5577713558194,-19.0417318110708,
12.));
#81320=CARTESIAN_POINT('Ctrl Pts',(-67.5748628971964,-19.0520862360396,
0.));
#81321=CARTESIAN_POINT('Ctrl Pts',(-67.5748628971964,-19.0520862360396,
12.));
#81322=CARTESIAN_POINT('Ctrl Pts',(-67.5919885896222,-19.062486364241,0.));
#81323=CARTESIAN_POINT('Ctrl Pts',(-67.5919885896222,-19.062486364241,12.));
#81324=CARTESIAN_POINT('Ctrl Pts',(-67.6091482520534,-19.072932177628,0.));
#81325=CARTESIAN_POINT('Ctrl Pts',(-67.6091482520534,-19.072932177628,12.));
#81326=CARTESIAN_POINT('Ctrl Pts',(-67.6263417083426,-19.0834236587118,
0.));
#81327=CARTESIAN_POINT('Ctrl Pts',(-67.6263417083426,-19.0834236587118,
12.));
#81328=CARTESIAN_POINT('Ctrl Pts',(-67.6435687749841,-19.0939607887502,
0.));
#81329=CARTESIAN_POINT('Ctrl Pts',(-67.6435687749841,-19.0939607887502,
12.));
#81330=CARTESIAN_POINT('Ctrl Pts',(-67.6608292549462,-19.1045435468358,
0.));
#81331=CARTESIAN_POINT('Ctrl Pts',(-67.6608292549462,-19.1045435468358,
12.));
#81332=CARTESIAN_POINT('Ctrl Pts',(-67.6781229440573,-19.115171910846,0.));
#81333=CARTESIAN_POINT('Ctrl Pts',(-67.6781229440573,-19.115171910846,12.));
#81334=CARTESIAN_POINT('Ctrl Pts',(-67.6954496350063,-19.1258458580345,
0.));
#81335=CARTESIAN_POINT('Ctrl Pts',(-67.6954496350063,-19.1258458580345,
12.));
#81336=CARTESIAN_POINT('Ctrl Pts',(-67.7128091219348,-19.136565365709,0.));
#81337=CARTESIAN_POINT('Ctrl Pts',(-67.7128091219348,-19.136565365709,12.));
#81338=CARTESIAN_POINT('Ctrl Pts',(-67.7302012056584,-19.1473304119955,
0.));
#81339=CARTESIAN_POINT('Ctrl Pts',(-67.7302012056584,-19.1473304119955,
12.));
#81340=CARTESIAN_POINT('Ctrl Pts',(-67.7476256934444,-19.1581409758097,
0.));
#81341=CARTESIAN_POINT('Ctrl Pts',(-67.7476256934444,-19.1581409758097,
12.));
#81342=CARTESIAN_POINT('Ctrl Pts',(-67.7650823965127,-19.168997036495,0.));
#81343=CARTESIAN_POINT('Ctrl Pts',(-67.7650823965127,-19.168997036495,12.));
#81344=CARTESIAN_POINT('Ctrl Pts',(-67.7825711283096,-19.1798985735688,
0.));
#81345=CARTESIAN_POINT('Ctrl Pts',(-67.7825711283096,-19.1798985735688,
12.));
#81346=CARTESIAN_POINT('Ctrl Pts',(-67.8000917023926,-19.1908455664098,
0.));
#81347=CARTESIAN_POINT('Ctrl Pts',(-67.8000917023926,-19.1908455664098,
12.));
#81348=CARTESIAN_POINT('Ctrl Pts',(-67.8176439306621,-19.201837993993,0.));
#81349=CARTESIAN_POINT('Ctrl Pts',(-67.8176439306621,-19.201837993993,12.));
#81350=CARTESIAN_POINT('Ctrl Pts',(-67.835227624289,-19.2128758350346,0.));
#81351=CARTESIAN_POINT('Ctrl Pts',(-67.835227624289,-19.2128758350346,12.));
#81352=CARTESIAN_POINT('Ctrl Pts',(-67.8528425945184,-19.2239590681133,
0.));
#81353=CARTESIAN_POINT('Ctrl Pts',(-67.8528425945184,-19.2239590681133,
12.));
#81354=CARTESIAN_POINT('Ctrl Pts',(-67.8704886534544,-19.2350876717874,
0.));
#81355=CARTESIAN_POINT('Ctrl Pts',(-67.8704886534544,-19.2350876717874,
12.));
#81356=CARTESIAN_POINT('Ctrl Pts',(-67.8881656149955,-19.2462616247279,
0.));
#81357=CARTESIAN_POINT('Ctrl Pts',(-67.8881656149955,-19.2462616247279,
12.));
#81358=CARTESIAN_POINT('Ctrl Pts',(-67.9058732951788,-19.2574809057696,
0.));
#81359=CARTESIAN_POINT('Ctrl Pts',(-67.9058732951788,-19.2574809057696,
12.));
#81360=CARTESIAN_POINT('Ctrl Pts',(-67.9236115116758,-19.2687454938442,
0.));
#81361=CARTESIAN_POINT('Ctrl Pts',(-67.9236115116758,-19.2687454938442,
12.));
#81362=CARTESIAN_POINT('Ctrl Pts',(-67.9413800834793,-19.280055367936,0.));
#81363=CARTESIAN_POINT('Ctrl Pts',(-67.9413800834793,-19.280055367936,12.));
#81364=CARTESIAN_POINT('Ctrl Pts',(-67.9591788305394,-19.2914105070286,
0.));
#81365=CARTESIAN_POINT('Ctrl Pts',(-67.9591788305394,-19.2914105070286,
12.));
#81366=CARTESIAN_POINT('Ctrl Pts',(-67.9770075733485,-19.302810890038,0.));
#81367=CARTESIAN_POINT('Ctrl Pts',(-67.9770075733485,-19.302810890038,12.));
#81368=CARTESIAN_POINT('Ctrl Pts',(-67.9948661329617,-19.3142564958203,
0.));
#81369=CARTESIAN_POINT('Ctrl Pts',(-67.9948661329617,-19.3142564958203,
12.));
#81370=CARTESIAN_POINT('Ctrl Pts',(-68.0127543311776,-19.3257473032035,
0.));
#81371=CARTESIAN_POINT('Ctrl Pts',(-68.0127543311776,-19.3257473032035,
12.));
#81372=CARTESIAN_POINT('Ctrl Pts',(-68.0306719906636,-19.3372832910076,
0.));
#81373=CARTESIAN_POINT('Ctrl Pts',(-68.0306719906636,-19.3372832910076,
12.));
#81374=CARTESIAN_POINT('Ctrl Pts',(-68.0486189351011,-19.3488644380641,
0.));
#81375=CARTESIAN_POINT('Ctrl Pts',(-68.0486189351011,-19.3488644380641,
12.));
#81376=CARTESIAN_POINT('Ctrl Pts',(-68.0665949893195,-19.3604907232314,
0.));
#81377=CARTESIAN_POINT('Ctrl Pts',(-68.0665949893195,-19.3604907232314,
12.));
#81378=CARTESIAN_POINT('Ctrl Pts',(-68.0845999792247,-19.3721621253912,
0.));
#81379=CARTESIAN_POINT('Ctrl Pts',(-68.0845999792247,-19.3721621253912,
12.));
#81380=CARTESIAN_POINT('Ctrl Pts',(-68.1026337317285,-19.3838786234421,
0.));
#81381=CARTESIAN_POINT('Ctrl Pts',(-68.1026337317285,-19.3838786234421,
12.));
#81382=CARTESIAN_POINT('Ctrl Pts',(-68.1206960746769,-19.3956401962895,
0.));
#81383=CARTESIAN_POINT('Ctrl Pts',(-68.1206960746769,-19.3956401962895,
12.));
#81384=CARTESIAN_POINT('Ctrl Pts',(-68.1387868367691,-19.40744682283,0.));
#81385=CARTESIAN_POINT('Ctrl Pts',(-68.1387868367691,-19.40744682283,12.));
#81386=CARTESIAN_POINT('Ctrl Pts',(-68.1569058475054,-19.4192984819418,
0.));
#81387=CARTESIAN_POINT('Ctrl Pts',(-68.1569058475054,-19.4192984819418,
12.));
#81388=CARTESIAN_POINT('Ctrl Pts',(-68.1750529372232,-19.4311951524983,
0.));
#81389=CARTESIAN_POINT('Ctrl Pts',(-68.1750529372232,-19.4311951524983,
12.));
#81390=CARTESIAN_POINT('Ctrl Pts',(-68.1932279371127,-19.4431368133719,
0.));
#81391=CARTESIAN_POINT('Ctrl Pts',(-68.1932279371127,-19.4431368133719,
12.));
#81392=CARTESIAN_POINT('Ctrl Pts',(-68.2114306792358,-19.4551234434381,
0.));
#81393=CARTESIAN_POINT('Ctrl Pts',(-68.2114306792358,-19.4551234434381,
12.));
#81394=CARTESIAN_POINT('Ctrl Pts',(-68.2296609965448,-19.467155021572,0.));
#81395=CARTESIAN_POINT('Ctrl Pts',(-68.2296609965448,-19.467155021572,12.));
#81396=CARTESIAN_POINT('Ctrl Pts',(-68.2479187228803,-19.4792315266501,
0.));
#81397=CARTESIAN_POINT('Ctrl Pts',(-68.2479187228803,-19.4792315266501,
12.));
#81398=CARTESIAN_POINT('Ctrl Pts',(-68.2662036929526,-19.4913529375543,
0.));
#81399=CARTESIAN_POINT('Ctrl Pts',(-68.2662036929526,-19.4913529375543,
12.));
#81400=CARTESIAN_POINT('Ctrl Pts',(-68.2845157423233,-19.5035192331705,
0.));
#81401=CARTESIAN_POINT('Ctrl Pts',(-68.2845157423233,-19.5035192331705,
12.));
#81402=CARTESIAN_POINT('Ctrl Pts',(-68.3028547073864,-19.5157303923856,
0.));
#81403=CARTESIAN_POINT('Ctrl Pts',(-68.3028547073864,-19.5157303923856,
12.));
#81404=CARTESIAN_POINT('Ctrl Pts',(-68.3212204253417,-19.5279863940773,
0.));
#81405=CARTESIAN_POINT('Ctrl Pts',(-68.3212204253417,-19.5279863940773,
12.));
#81406=CARTESIAN_POINT('Ctrl Pts',(-68.3396127341938,-19.5402872171191,
0.));
#81407=CARTESIAN_POINT('Ctrl Pts',(-68.3396127341938,-19.5402872171191,
12.));
#81408=CARTESIAN_POINT('Ctrl Pts',(-68.3580314727523,-19.5526328403852,
0.));
#81409=CARTESIAN_POINT('Ctrl Pts',(-68.3580314727523,-19.5526328403852,
12.));
#81410=CARTESIAN_POINT('Ctrl Pts',(-68.3764764806287,-19.5650232427516,
0.));
#81411=CARTESIAN_POINT('Ctrl Pts',(-68.3764764806287,-19.5650232427516,
12.));
#81412=CARTESIAN_POINT('Ctrl Pts',(-68.3949475982335,-19.5774584030938,
0.));
#81413=CARTESIAN_POINT('Ctrl Pts',(-68.3949475982335,-19.5774584030938,
12.));
#81414=CARTESIAN_POINT('Ctrl Pts',(-68.4134446667696,-19.5899383002803,
0.));
#81415=CARTESIAN_POINT('Ctrl Pts',(-68.4134446667696,-19.5899383002803,
12.));
#81416=CARTESIAN_POINT('Ctrl Pts',(-68.4319675282275,-19.6024629131785,
0.));
#81417=CARTESIAN_POINT('Ctrl Pts',(-68.4319675282275,-19.6024629131785,
12.));
#81418=CARTESIAN_POINT('Ctrl Pts',(-68.4505160253778,-19.6150322206577,
0.));
#81419=CARTESIAN_POINT('Ctrl Pts',(-68.4505160253778,-19.6150322206577,
12.));
#81420=CARTESIAN_POINT('Ctrl Pts',(-68.4690900017632,-19.6276462015888,
0.));
#81421=CARTESIAN_POINT('Ctrl Pts',(-68.4690900017632,-19.6276462015888,
12.));
#81422=CARTESIAN_POINT('Ctrl Pts',(-68.4876893016856,-19.6403048348395,
0.));
#81423=CARTESIAN_POINT('Ctrl Pts',(-68.4876893016856,-19.6403048348395,
12.));
#81424=CARTESIAN_POINT('Ctrl Pts',(-68.5063137701971,-19.6530080992686,
0.));
#81425=CARTESIAN_POINT('Ctrl Pts',(-68.5063137701971,-19.6530080992686,
12.));
#81426=CARTESIAN_POINT('Ctrl Pts',(-68.5249632530979,-19.6657559737336,
0.));
#81427=CARTESIAN_POINT('Ctrl Pts',(-68.5249632530979,-19.6657559737336,
12.));
#81428=CARTESIAN_POINT('Ctrl Pts',(-68.5436375969311,-19.6785484370927,
0.));
#81429=CARTESIAN_POINT('Ctrl Pts',(-68.5436375969311,-19.6785484370927,
12.));
#81430=CARTESIAN_POINT('Ctrl Pts',(-68.5623366489779,-19.6913854682046,
0.));
#81431=CARTESIAN_POINT('Ctrl Pts',(-68.5623366489779,-19.6913854682046,
12.));
#81432=CARTESIAN_POINT('Ctrl Pts',(-68.581060257249,-19.7042670459237,0.));
#81433=CARTESIAN_POINT('Ctrl Pts',(-68.581060257249,-19.7042670459237,12.));
#81434=CARTESIAN_POINT('Ctrl Pts',(-68.5998082704766,-19.7171931490956,
0.));
#81435=CARTESIAN_POINT('Ctrl Pts',(-68.5998082704766,-19.7171931490956,
12.));
#81436=CARTESIAN_POINT('Ctrl Pts',(-68.6185805381126,-19.7301637565652,
0.));
#81437=CARTESIAN_POINT('Ctrl Pts',(-68.6185805381126,-19.7301637565652,
12.));
#81438=CARTESIAN_POINT('Ctrl Pts',(-68.6373769103224,-19.7431788471776,
0.));
#81439=CARTESIAN_POINT('Ctrl Pts',(-68.6373769103224,-19.7431788471776,
12.));
#81440=CARTESIAN_POINT('Ctrl Pts',(-68.6561972379793,-19.7562383997781,
0.));
#81441=CARTESIAN_POINT('Ctrl Pts',(-68.6561972379793,-19.7562383997781,
12.));
#81442=CARTESIAN_POINT('Ctrl Pts',(-68.6750413726547,-19.7693423932058,
0.));
#81443=CARTESIAN_POINT('Ctrl Pts',(-68.6750413726547,-19.7693423932058,
12.));
#81444=CARTESIAN_POINT('Ctrl Pts',(-68.6939091666111,-19.7824908062913,
0.));
#81445=CARTESIAN_POINT('Ctrl Pts',(-68.6939091666111,-19.7824908062913,
12.));
#81446=CARTESIAN_POINT('Ctrl Pts',(-68.7128004727998,-19.795683617864,0.));
#81447=CARTESIAN_POINT('Ctrl Pts',(-68.7128004727998,-19.795683617864,12.));
#81448=CARTESIAN_POINT('Ctrl Pts',(-68.7317151448557,-19.8089208067532,
0.));
#81449=CARTESIAN_POINT('Ctrl Pts',(-68.7317151448557,-19.8089208067532,
12.));
#81450=CARTESIAN_POINT('Ctrl Pts',(-68.7506530370918,-19.8222023517874,
0.));
#81451=CARTESIAN_POINT('Ctrl Pts',(-68.7506530370918,-19.8222023517874,
12.));
#81452=CARTESIAN_POINT('Ctrl Pts',(-68.7696140044892,-19.835528231787,0.));
#81453=CARTESIAN_POINT('Ctrl Pts',(-68.7696140044892,-19.835528231787,12.));
#81454=CARTESIAN_POINT('Ctrl Pts',(-68.7885979026927,-19.8488984255642,
0.));
#81455=CARTESIAN_POINT('Ctrl Pts',(-68.7885979026927,-19.8488984255642,
12.));
#81456=CARTESIAN_POINT('Ctrl Pts',(-68.8076045880102,-19.8623129119304,
0.));
#81457=CARTESIAN_POINT('Ctrl Pts',(-68.8076045880102,-19.8623129119304,
12.));
#81458=CARTESIAN_POINT('Ctrl Pts',(-68.8266339174068,-19.8757716696969,
0.));
#81459=CARTESIAN_POINT('Ctrl Pts',(-68.8266339174068,-19.8757716696969,
12.));
#81460=CARTESIAN_POINT('Ctrl Pts',(-68.8456857484988,-19.8892746776734,
0.));
#81461=CARTESIAN_POINT('Ctrl Pts',(-68.8456857484988,-19.8892746776734,
12.));
#81462=CARTESIAN_POINT('Ctrl Pts',(-68.8647599395437,-19.9028219146607,
0.));
#81463=CARTESIAN_POINT('Ctrl Pts',(-68.8647599395437,-19.9028219146607,
12.));
#81464=CARTESIAN_POINT('Ctrl Pts',(-68.8838563494356,-19.9164133594513,
0.));
#81465=CARTESIAN_POINT('Ctrl Pts',(-68.8838563494356,-19.9164133594513,
12.));
#81466=CARTESIAN_POINT('Ctrl Pts',(-68.902974837704,-19.9300489908364,0.));
#81467=CARTESIAN_POINT('Ctrl Pts',(-68.902974837704,-19.9300489908364,12.));
#81468=CARTESIAN_POINT('Ctrl Pts',(-68.9221152645086,-19.9437287876063,
0.));
#81469=CARTESIAN_POINT('Ctrl Pts',(-68.9221152645086,-19.9437287876063,
12.));
#81470=CARTESIAN_POINT('Ctrl Pts',(-68.9412774906346,-19.9574527285492,
0.));
#81471=CARTESIAN_POINT('Ctrl Pts',(-68.9412774906346,-19.9574527285492,
12.));
#81472=CARTESIAN_POINT('Ctrl Pts',(-68.960461377483,-19.9712207924437,0.));
#81473=CARTESIAN_POINT('Ctrl Pts',(-68.960461377483,-19.9712207924437,12.));
#81474=CARTESIAN_POINT('Ctrl Pts',(-68.9796667870667,-19.98503295806,0.));
#81475=CARTESIAN_POINT('Ctrl Pts',(-68.9796667870667,-19.98503295806,12.));
#81476=CARTESIAN_POINT('Ctrl Pts',(-68.9988935820101,-19.9988892041671,
0.));
#81477=CARTESIAN_POINT('Ctrl Pts',(-68.9988935820101,-19.9988892041671,
12.));
#81478=CARTESIAN_POINT('Ctrl Pts',(-69.0181416255433,-20.0127895095327,
0.));
#81479=CARTESIAN_POINT('Ctrl Pts',(-69.0181416255433,-20.0127895095327,
12.));
#81480=CARTESIAN_POINT('Ctrl Pts',(-69.0374107814977,-20.0267338529221,
0.));
#81481=CARTESIAN_POINT('Ctrl Pts',(-69.0374107814977,-20.0267338529221,
12.));
#81482=CARTESIAN_POINT('Ctrl Pts',(-69.0567009142968,-20.0407222130902,
0.));
#81483=CARTESIAN_POINT('Ctrl Pts',(-69.0567009142968,-20.0407222130902,
12.));
#81484=CARTESIAN_POINT('Ctrl Pts',(-69.0760118889525,-20.0547545687839,
0.));
#81485=CARTESIAN_POINT('Ctrl Pts',(-69.0760118889525,-20.0547545687839,
12.));
#81486=CARTESIAN_POINT('Ctrl Pts',(-69.0953435710634,-20.0688308987478,
0.));
#81487=CARTESIAN_POINT('Ctrl Pts',(-69.0953435710634,-20.0688308987478,
12.));
#81488=CARTESIAN_POINT('Ctrl Pts',(-69.1146958268104,-20.0829511817251,
0.));
#81489=CARTESIAN_POINT('Ctrl Pts',(-69.1146958268104,-20.0829511817251,
12.));
#81490=CARTESIAN_POINT('Ctrl Pts',(-69.1340685229516,-20.0971153964557,
0.));
#81491=CARTESIAN_POINT('Ctrl Pts',(-69.1340685229516,-20.0971153964557,
12.));
#81492=CARTESIAN_POINT('Ctrl Pts',(-69.1534615268153,-20.1113235216694,
0.));
#81493=CARTESIAN_POINT('Ctrl Pts',(-69.1534615268153,-20.1113235216694,
12.));
#81494=CARTESIAN_POINT('Ctrl Pts',(-69.172874706296,-20.1255755360871,0.));
#81495=CARTESIAN_POINT('Ctrl Pts',(-69.172874706296,-20.1255755360871,12.));
#81496=CARTESIAN_POINT('Ctrl Pts',(-69.1923079298534,-20.1398714184278,
0.));
#81497=CARTESIAN_POINT('Ctrl Pts',(-69.1923079298534,-20.1398714184278,
12.));
#81498=CARTESIAN_POINT('Ctrl Pts',(-69.2117610665073,-20.1542111474086,
0.));
#81499=CARTESIAN_POINT('Ctrl Pts',(-69.2117610665073,-20.1542111474086,
12.));
#81500=CARTESIAN_POINT('Ctrl Pts',(-69.2312339858337,-20.1685947017433,
0.));
#81501=CARTESIAN_POINT('Ctrl Pts',(-69.2312339858337,-20.1685947017433,
12.));
#81502=CARTESIAN_POINT('Ctrl Pts',(-69.2507265579562,-20.183022060135,0.));
#81503=CARTESIAN_POINT('Ctrl Pts',(-69.2507265579562,-20.183022060135,12.));
#81504=CARTESIAN_POINT('Ctrl Pts',(-69.2702386535432,-20.1974932012775,
0.));
#81505=CARTESIAN_POINT('Ctrl Pts',(-69.2702386535432,-20.1974932012775,
12.));
#81506=CARTESIAN_POINT('Ctrl Pts',(-69.2897701438066,-20.2120081038622,
0.));
#81507=CARTESIAN_POINT('Ctrl Pts',(-69.2897701438066,-20.2120081038622,
12.));
#81508=CARTESIAN_POINT('Ctrl Pts',(-69.3093209004986,-20.2265667465784,
0.));
#81509=CARTESIAN_POINT('Ctrl Pts',(-69.3093209004986,-20.2265667465784,
12.));
#81510=CARTESIAN_POINT('Ctrl Pts',(-69.3288907959065,-20.2411691081122,
0.));
#81511=CARTESIAN_POINT('Ctrl Pts',(-69.3288907959065,-20.2411691081122,
12.));
#81512=CARTESIAN_POINT('Ctrl Pts',(-69.3484797028454,-20.255815167139,0.));
#81513=CARTESIAN_POINT('Ctrl Pts',(-69.3484797028454,-20.255815167139,12.));
#81514=CARTESIAN_POINT('Ctrl Pts',(-69.3680874946548,-20.2705049023241,
0.));
#81515=CARTESIAN_POINT('Ctrl Pts',(-69.3680874946548,-20.2705049023241,
12.));
#81516=CARTESIAN_POINT('Ctrl Pts',(-69.3877140451975,-20.2852382923299,
0.));
#81517=CARTESIAN_POINT('Ctrl Pts',(-69.3877140451975,-20.2852382923299,
12.));
#81518=CARTESIAN_POINT('Ctrl Pts',(-69.4073592288562,-20.3000153158167,
0.));
#81519=CARTESIAN_POINT('Ctrl Pts',(-69.4073592288562,-20.3000153158167,
12.));
#81520=CARTESIAN_POINT('Ctrl Pts',(-69.4270229205296,-20.3148359514414,
0.));
#81521=CARTESIAN_POINT('Ctrl Pts',(-69.4270229205296,-20.3148359514414,
12.));
#81522=CARTESIAN_POINT('Ctrl Pts',(-69.4467049956257,-20.3297001778505,
0.));
#81523=CARTESIAN_POINT('Ctrl Pts',(-69.4467049956257,-20.3297001778505,
12.));
#81524=CARTESIAN_POINT('Ctrl Pts',(-69.4664053300579,-20.3446079736799,
0.));
#81525=CARTESIAN_POINT('Ctrl Pts',(-69.4664053300579,-20.3446079736799,
12.));
#81526=CARTESIAN_POINT('Ctrl Pts',(-69.4861238002433,-20.359559317562,0.));
#81527=CARTESIAN_POINT('Ctrl Pts',(-69.4861238002433,-20.359559317562,12.));
#81528=CARTESIAN_POINT('Ctrl Pts',(-69.5058602831004,-20.3745541881267,
0.));
#81529=CARTESIAN_POINT('Ctrl Pts',(-69.5058602831004,-20.3745541881267,
12.));
#81530=CARTESIAN_POINT('Ctrl Pts',(-69.5256146560444,-20.3895925640006,
0.));
#81531=CARTESIAN_POINT('Ctrl Pts',(-69.5256146560444,-20.3895925640006,
12.));
#81532=CARTESIAN_POINT('Ctrl Pts',(-69.5453867969815,-20.4046744238002,
0.));
#81533=CARTESIAN_POINT('Ctrl Pts',(-69.5453867969815,-20.4046744238002,
12.));
#81534=CARTESIAN_POINT('Ctrl Pts',(-69.565176584305,-20.4197997461306,0.));
#81535=CARTESIAN_POINT('Ctrl Pts',(-69.565176584305,-20.4197997461306,12.));
#81536=CARTESIAN_POINT('Ctrl Pts',(-69.5849838968944,-20.4349685095928,
0.));
#81537=CARTESIAN_POINT('Ctrl Pts',(-69.5849838968944,-20.4349685095928,
12.));
#81538=CARTESIAN_POINT('Ctrl Pts',(-69.6048086141122,-20.4501806927854,
0.));
#81539=CARTESIAN_POINT('Ctrl Pts',(-69.6048086141122,-20.4501806927854,
12.));
#81540=CARTESIAN_POINT('Ctrl Pts',(-69.6246506158009,-20.4654362743036,
0.));
#81541=CARTESIAN_POINT('Ctrl Pts',(-69.6246506158009,-20.4654362743036,
12.));
#81542=CARTESIAN_POINT('Ctrl Pts',(-69.6445097822778,-20.4807352327335,
0.));
#81543=CARTESIAN_POINT('Ctrl Pts',(-69.6445097822778,-20.4807352327335,
12.));
#81544=CARTESIAN_POINT('Ctrl Pts',(-69.6643859943291,-20.4960775466487,
0.));
#81545=CARTESIAN_POINT('Ctrl Pts',(-69.6643859943291,-20.4960775466487,
12.));
#81546=CARTESIAN_POINT('Ctrl Pts',(-69.6842791332102,-20.511463194618,0.));
#81547=CARTESIAN_POINT('Ctrl Pts',(-69.6842791332102,-20.511463194618,12.));
#81548=CARTESIAN_POINT('Ctrl Pts',(-69.7041890806421,-20.5268921552076,
0.));
#81549=CARTESIAN_POINT('Ctrl Pts',(-69.7041890806421,-20.5268921552076,
12.));
#81550=CARTESIAN_POINT('Ctrl Pts',(-69.7241157188086,-20.54236440698,0.));
#81551=CARTESIAN_POINT('Ctrl Pts',(-69.7241157188086,-20.54236440698,12.));
#81552=CARTESIAN_POINT('Ctrl Pts',(-69.7440589303511,-20.5578799284898,
0.));
#81553=CARTESIAN_POINT('Ctrl Pts',(-69.7440589303511,-20.5578799284898,
12.));
#81554=CARTESIAN_POINT('Ctrl Pts',(-69.7640185983641,-20.5734386982782,
0.));
#81555=CARTESIAN_POINT('Ctrl Pts',(-69.7640185983641,-20.5734386982782,
12.));
#81556=CARTESIAN_POINT('Ctrl Pts',(-69.7839946063942,-20.5890406948809,
0.));
#81557=CARTESIAN_POINT('Ctrl Pts',(-69.7839946063942,-20.5890406948809,
12.));
#81558=CARTESIAN_POINT('Ctrl Pts',(-69.8039868384382,-20.6046858968305,
0.));
#81559=CARTESIAN_POINT('Ctrl Pts',(-69.8039868384382,-20.6046858968305,
12.));
#81560=CARTESIAN_POINT('Ctrl Pts',(-69.8239951789402,-20.6203742826566,
0.));
#81561=CARTESIAN_POINT('Ctrl Pts',(-69.8239951789402,-20.6203742826566,
12.));
#81562=CARTESIAN_POINT('Ctrl Pts',(-69.8440195127874,-20.6361058308812,
0.));
#81563=CARTESIAN_POINT('Ctrl Pts',(-69.8440195127874,-20.6361058308812,
12.));
#81564=CARTESIAN_POINT('Ctrl Pts',(-69.8640597253058,-20.6518805200132,
0.));
#81565=CARTESIAN_POINT('Ctrl Pts',(-69.8640597253058,-20.6518805200132,
12.));
#81566=CARTESIAN_POINT('Ctrl Pts',(-69.884115702258,-20.6676983285542,0.));
#81567=CARTESIAN_POINT('Ctrl Pts',(-69.884115702258,-20.6676983285542,12.));
#81568=CARTESIAN_POINT('Ctrl Pts',(-69.9041873298416,-20.6835592350031,
0.));
#81569=CARTESIAN_POINT('Ctrl Pts',(-69.9041873298416,-20.6835592350031,
12.));
#81570=CARTESIAN_POINT('Ctrl Pts',(-69.9242744946854,-20.6994632178551,
0.));
#81571=CARTESIAN_POINT('Ctrl Pts',(-69.9242744946854,-20.6994632178551,
12.));
#81572=CARTESIAN_POINT('Ctrl Pts',(-69.9443770838444,-20.7154102555996,
0.));
#81573=CARTESIAN_POINT('Ctrl Pts',(-69.9443770838444,-20.7154102555996,
12.));
#81574=CARTESIAN_POINT('Ctrl Pts',(-69.9644949847929,-20.7314003267118,
0.));
#81575=CARTESIAN_POINT('Ctrl Pts',(-69.9644949847929,-20.7314003267118,
12.));
#81576=CARTESIAN_POINT('Ctrl Pts',(-69.9846280854254,-20.7474334096582,
0.));
#81577=CARTESIAN_POINT('Ctrl Pts',(-69.9846280854254,-20.7474334096582,
12.));
#81578=CARTESIAN_POINT('Ctrl Pts',(-70.0047762740569,-20.7635094829017,
0.));
#81579=CARTESIAN_POINT('Ctrl Pts',(-70.0047762740569,-20.7635094829017,
12.));
#81580=CARTESIAN_POINT('Ctrl Pts',(-70.0249394394221,-20.7796285249023,
0.));
#81581=CARTESIAN_POINT('Ctrl Pts',(-70.0249394394221,-20.7796285249023,
12.));
#81582=CARTESIAN_POINT('Ctrl Pts',(-70.0451174706739,-20.7957905141155,
0.));
#81583=CARTESIAN_POINT('Ctrl Pts',(-70.0451174706739,-20.7957905141155,
12.));
#81584=CARTESIAN_POINT('Ctrl Pts',(-70.0653102573798,-20.8119954289846,
0.));
#81585=CARTESIAN_POINT('Ctrl Pts',(-70.0653102573798,-20.8119954289846,
12.));
#81586=CARTESIAN_POINT('Ctrl Pts',(-70.0855176895185,-20.8282432479425,
0.));
#81587=CARTESIAN_POINT('Ctrl Pts',(-70.0855176895185,-20.8282432479425,
12.));
#81588=CARTESIAN_POINT('Ctrl Pts',(-70.1057396574741,-20.8445339494185,
0.));
#81589=CARTESIAN_POINT('Ctrl Pts',(-70.1057396574741,-20.8445339494185,
12.));
#81590=CARTESIAN_POINT('Ctrl Pts',(-70.1259760520306,-20.8608675118377,
0.));
#81591=CARTESIAN_POINT('Ctrl Pts',(-70.1259760520306,-20.8608675118377,
12.));
#81592=CARTESIAN_POINT('Ctrl Pts',(-70.1462267643649,-20.8772439136207,
0.));
#81593=CARTESIAN_POINT('Ctrl Pts',(-70.1462267643649,-20.8772439136207,
12.));
#81594=CARTESIAN_POINT('Ctrl Pts',(-70.1664916860366,-20.8936631331751,
0.));
#81595=CARTESIAN_POINT('Ctrl Pts',(-70.1664916860366,-20.8936631331751,
12.));
#81596=CARTESIAN_POINT('Ctrl Pts',(-70.1867707089866,-20.9101251488948,
0.));
#81597=CARTESIAN_POINT('Ctrl Pts',(-70.1867707089866,-20.9101251488948,
12.));
#81598=CARTESIAN_POINT('Ctrl Pts',(-70.2070637255469,-20.9266299391688,
0.));
#81599=CARTESIAN_POINT('Ctrl Pts',(-70.2070637255469,-20.9266299391688,
12.));
#81600=CARTESIAN_POINT('Ctrl Pts',(-70.2273706284479,-20.9431774823833,
0.));
#81601=CARTESIAN_POINT('Ctrl Pts',(-70.2273706284479,-20.9431774823833,
12.));
#81602=CARTESIAN_POINT('Ctrl Pts',(-70.2476913108242,-20.9597677569227,
0.));
#81603=CARTESIAN_POINT('Ctrl Pts',(-70.2476913108242,-20.9597677569227,
12.));
#81604=CARTESIAN_POINT('Ctrl Pts',(-70.2680256662215,-20.9764007411649,
0.));
#81605=CARTESIAN_POINT('Ctrl Pts',(-70.2680256662215,-20.9764007411649,
12.));
#81606=CARTESIAN_POINT('Ctrl Pts',(-70.288373588597,-20.9930764134771,0.));
#81607=CARTESIAN_POINT('Ctrl Pts',(-70.288373588597,-20.9930764134771,12.));
#81608=CARTESIAN_POINT('Ctrl Pts',(-70.3087349722959,-21.0097947522212,
0.));
#81609=CARTESIAN_POINT('Ctrl Pts',(-70.3087349722959,-21.0097947522212,
12.));
#81610=CARTESIAN_POINT('Ctrl Pts',(-70.3291097120293,-21.0265557357544,
0.));
#81611=CARTESIAN_POINT('Ctrl Pts',(-70.3291097120293,-21.0265557357544,
12.));
#81612=CARTESIAN_POINT('Ctrl Pts',(-70.3494977028497,-21.0433593424266,
0.));
#81613=CARTESIAN_POINT('Ctrl Pts',(-70.3494977028497,-21.0433593424266,
12.));
#81614=CARTESIAN_POINT('Ctrl Pts',(-70.3698988401291,-21.0602055505751,
0.));
#81615=CARTESIAN_POINT('Ctrl Pts',(-70.3698988401291,-21.0602055505751,
12.));
#81616=CARTESIAN_POINT('Ctrl Pts',(-70.3903130195279,-21.0770943385146,
0.));
#81617=CARTESIAN_POINT('Ctrl Pts',(-70.3903130195279,-21.0770943385146,
12.));
#81618=CARTESIAN_POINT('Ctrl Pts',(-70.4107401370403,-21.0940256845477,
0.));
#81619=CARTESIAN_POINT('Ctrl Pts',(-70.4107401370403,-21.0940256845477,
12.));
#81620=CARTESIAN_POINT('Ctrl Pts',(-70.4311800890411,-21.110999566975,0.));
#81621=CARTESIAN_POINT('Ctrl Pts',(-70.4311800890411,-21.110999566975,12.));
#81622=CARTESIAN_POINT('Ctrl Pts',(-70.4516327723349,-21.1280159641003,
0.));
#81623=CARTESIAN_POINT('Ctrl Pts',(-70.4516327723349,-21.1280159641003,
12.));
#81624=CARTESIAN_POINT('Ctrl Pts',(-70.4720980841934,-21.1450748542335,
0.));
#81625=CARTESIAN_POINT('Ctrl Pts',(-70.4720980841934,-21.1450748542335,
12.));
#81626=CARTESIAN_POINT('Ctrl Pts',(-70.4925759224208,-21.1621762156894,
0.));
#81627=CARTESIAN_POINT('Ctrl Pts',(-70.4925759224208,-21.1621762156894,
12.));
#81628=CARTESIAN_POINT('Ctrl Pts',(-70.5130661852946,-21.1793200267844,
0.));
#81629=CARTESIAN_POINT('Ctrl Pts',(-70.5130661852946,-21.1793200267844,
12.));
#81630=CARTESIAN_POINT('Ctrl Pts',(-70.5335687714422,-21.1965062658296,
0.));
#81631=CARTESIAN_POINT('Ctrl Pts',(-70.5335687714422,-21.1965062658296,
12.));
#81632=CARTESIAN_POINT('Ctrl Pts',(-70.5540835797281,-21.2137349111207,
0.));
#81633=CARTESIAN_POINT('Ctrl Pts',(-70.5540835797281,-21.2137349111207,
12.));
#81634=CARTESIAN_POINT('Ctrl Pts',(-70.5746105091503,-21.2310059409265,
0.));
#81635=CARTESIAN_POINT('Ctrl Pts',(-70.5746105091503,-21.2310059409265,
12.));
#81636=CARTESIAN_POINT('Ctrl Pts',(-70.5951494586961,-21.2483193334677,
0.));
#81637=CARTESIAN_POINT('Ctrl Pts',(-70.5951494586961,-21.2483193334677,
12.));
#81638=CARTESIAN_POINT('Ctrl Pts',(-70.6157003273326,-21.2656750669129,
0.));
#81639=CARTESIAN_POINT('Ctrl Pts',(-70.6157003273326,-21.2656750669129,
12.));
#81640=CARTESIAN_POINT('Ctrl Pts',(-70.6362630143062,-21.2830731194188,
0.));
#81641=CARTESIAN_POINT('Ctrl Pts',(-70.6362630143062,-21.2830731194188,
12.));
#81642=CARTESIAN_POINT('Ctrl Pts',(-70.6568374193786,-21.3005134691563,
0.));
#81643=CARTESIAN_POINT('Ctrl Pts',(-70.6568374193786,-21.3005134691563,
12.));
#81644=CARTESIAN_POINT('Ctrl Pts',(-70.6774234430899,-21.3179960943389,
0.));
#81645=CARTESIAN_POINT('Ctrl Pts',(-70.6774234430899,-21.3179960943389,
12.));
#81646=CARTESIAN_POINT('Ctrl Pts',(-70.6980209870032,-21.3355209732438,
0.));
#81647=CARTESIAN_POINT('Ctrl Pts',(-70.6980209870032,-21.3355209732438,
12.));
#81648=CARTESIAN_POINT('Ctrl Pts',(-70.7186299539698,-21.353088084234,0.));
#81649=CARTESIAN_POINT('Ctrl Pts',(-70.7186299539698,-21.353088084234,12.));
#81650=CARTESIAN_POINT('Ctrl Pts',(-70.7392502475437,-21.3706974057028,
0.));
#81651=CARTESIAN_POINT('Ctrl Pts',(-70.7392502475437,-21.3706974057028,
12.));
#81652=CARTESIAN_POINT('Ctrl Pts',(-70.7598817714078,-21.3883489160187,
0.));
#81653=CARTESIAN_POINT('Ctrl Pts',(-70.7598817714078,-21.3883489160187,
12.));
#81654=CARTESIAN_POINT('Ctrl Pts',(-70.780524428744,-21.4060425934595,0.));
#81655=CARTESIAN_POINT('Ctrl Pts',(-70.780524428744,-21.4060425934595,12.));
#81656=CARTESIAN_POINT('Ctrl Pts',(-70.8011781217409,-21.4237784161592,
0.));
#81657=CARTESIAN_POINT('Ctrl Pts',(-70.8011781217409,-21.4237784161592,
12.));
#81658=CARTESIAN_POINT('Ctrl Pts',(-70.8218427507545,-21.4415563620127,
0.));
#81659=CARTESIAN_POINT('Ctrl Pts',(-70.8218427507545,-21.4415563620127,
12.));
#81660=CARTESIAN_POINT('Ctrl Pts',(-70.84251821499,-21.4593764087492,0.));
#81661=CARTESIAN_POINT('Ctrl Pts',(-70.84251821499,-21.4593764087492,12.));
#81662=CARTESIAN_POINT('Ctrl Pts',(-70.8632044140166,-21.4772385340978,
0.));
#81663=CARTESIAN_POINT('Ctrl Pts',(-70.8632044140166,-21.4772385340978,
12.));
#81664=CARTESIAN_POINT('Ctrl Pts',(-70.8839012490903,-21.4951427159272,
0.));
#81665=CARTESIAN_POINT('Ctrl Pts',(-70.8839012490903,-21.4951427159272,
12.));
#81666=CARTESIAN_POINT('Ctrl Pts',(-70.9046086244123,-21.5130889323767,
0.));
#81667=CARTESIAN_POINT('Ctrl Pts',(-70.9046086244123,-21.5130889323767,
12.));
#81668=CARTESIAN_POINT('Ctrl Pts',(-70.9253264487576,-21.5310771620209,
0.));
#81669=CARTESIAN_POINT('Ctrl Pts',(-70.9253264487576,-21.5310771620209,
12.));
#81670=CARTESIAN_POINT('Ctrl Pts',(-70.9460546358597,-21.549107383907,0.));
#81671=CARTESIAN_POINT('Ctrl Pts',(-70.9460546358597,-21.549107383907,12.));
#81672=CARTESIAN_POINT('Ctrl Pts',(-70.9667931008097,-21.5671795771873,
0.));
#81673=CARTESIAN_POINT('Ctrl Pts',(-70.9667931008097,-21.5671795771873,
12.));
#81674=CARTESIAN_POINT('Ctrl Pts',(-70.9875417572138,-21.5852937208258,
0.));
#81675=CARTESIAN_POINT('Ctrl Pts',(-70.9875417572138,-21.5852937208258,
12.));
#81676=CARTESIAN_POINT('Ctrl Pts',(-71.0083005139086,-21.6034497932574,
0.));
#81677=CARTESIAN_POINT('Ctrl Pts',(-71.0083005139086,-21.6034497932574,
12.));
#81678=CARTESIAN_POINT('Ctrl Pts',(-71.0290692721932,-21.6216477720941,
0.));
#81679=CARTESIAN_POINT('Ctrl Pts',(-71.0290692721932,-21.6216477720941,
12.));
#81680=CARTESIAN_POINT('Ctrl Pts',(-71.0498479219659,-21.6398876337207,
0.));
#81681=CARTESIAN_POINT('Ctrl Pts',(-71.0498479219659,-21.6398876337207,
12.));
#81682=CARTESIAN_POINT('Ctrl Pts',(-71.0706363472965,-21.6581693538424,
0.));
#81683=CARTESIAN_POINT('Ctrl Pts',(-71.0706363472965,-21.6581693538424,
12.));
#81684=CARTESIAN_POINT('Ctrl Pts',(-71.0914344333048,-21.6764929081763,
0.));
#81685=CARTESIAN_POINT('Ctrl Pts',(-71.0914344333048,-21.6764929081763,
12.));
#81686=CARTESIAN_POINT('Ctrl Pts',(-71.1122420728349,-21.6948582730895,
0.));
#81687=CARTESIAN_POINT('Ctrl Pts',(-71.1122420728349,-21.6948582730895,
12.));
#81688=CARTESIAN_POINT('Ctrl Pts',(-71.133059172642,-21.7132654262501,0.));
#81689=CARTESIAN_POINT('Ctrl Pts',(-71.133059172642,-21.7132654262501,12.));
#81690=CARTESIAN_POINT('Ctrl Pts',(-71.1538856611899,-21.7317143472827,
0.));
#81691=CARTESIAN_POINT('Ctrl Pts',(-71.1538856611899,-21.7317143472827,
12.));
#81692=CARTESIAN_POINT('Ctrl Pts',(-71.1747214905981,-21.7502050183602,
0.));
#81693=CARTESIAN_POINT('Ctrl Pts',(-71.1747214905981,-21.7502050183602,
12.));
#81694=CARTESIAN_POINT('Ctrl Pts',(-71.1955666309591,-21.7687374247046,
0.));
#81695=CARTESIAN_POINT('Ctrl Pts',(-71.1955666309591,-21.7687374247046,
12.));
#81696=CARTESIAN_POINT('Ctrl Pts',(-71.212250179455,-21.7835967290261,0.));
#81697=CARTESIAN_POINT('Ctrl Pts',(-71.212250179455,-21.7835967290261,12.));
#81698=CARTESIAN_POINT('Ctrl Pts',(-71.2247670209821,-21.7947599798839,
0.));
#81699=CARTESIAN_POINT('Ctrl Pts',(-71.2247670209821,-21.7947599798839,
12.));
#81700=CARTESIAN_POINT('Ctrl Pts',(-71.2331134397743,-21.8022104901682,
0.));
#81701=CARTESIAN_POINT('Ctrl Pts',(-71.2331134397743,-21.8022104901682,
12.));
#81702=CARTESIAN_POINT('Ctrl Pts',(-71.2372871136137,-21.8059378310719,
0.));
#81703=CARTESIAN_POINT('Ctrl Pts',(-71.2372871136137,-21.8059378310719,
12.));
#81704=CARTESIAN_POINT('',(-67.3887914263118,-18.9407177820969,0.));
#81705=CARTESIAN_POINT('Ctrl Pts',(-67.3887914263118,-18.9407177820969,
0.));
#81706=CARTESIAN_POINT('Ctrl Pts',(-67.3921355608328,-18.9426924398719,
0.));
#81707=CARTESIAN_POINT('Ctrl Pts',(-67.3988274146651,-18.9466463414299,
0.));
#81708=CARTESIAN_POINT('Ctrl Pts',(-67.4088759497911,-18.9525909517915,
0.));
#81709=CARTESIAN_POINT('Ctrl Pts',(-67.4222955061981,-18.9605446160985,
0.));
#81710=CARTESIAN_POINT('Ctrl Pts',(-67.4391057908418,-18.9705325631711,
0.));
#81711=CARTESIAN_POINT('Ctrl Pts',(-67.4559518744638,-18.9805663798449,
0.));
#81712=CARTESIAN_POINT('Ctrl Pts',(-67.472833671964,-18.9906460638625,0.));
#81713=CARTESIAN_POINT('Ctrl Pts',(-67.4897510316844,-19.0007716032819,
0.));
#81714=CARTESIAN_POINT('Ctrl Pts',(-67.5067037372317,-19.0109429761306,
0.));
#81715=CARTESIAN_POINT('Ctrl Pts',(-67.5236915360331,-19.021160154824,0.));
#81716=CARTESIAN_POINT('Ctrl Pts',(-67.540714161288,-19.0314231093923,0.));
#81717=CARTESIAN_POINT('Ctrl Pts',(-67.5577713558194,-19.0417318110708,
0.));
#81718=CARTESIAN_POINT('Ctrl Pts',(-67.5748628971964,-19.0520862360396,
0.));
#81719=CARTESIAN_POINT('Ctrl Pts',(-67.5919885896222,-19.062486364241,0.));
#81720=CARTESIAN_POINT('Ctrl Pts',(-67.6091482520534,-19.072932177628,0.));
#81721=CARTESIAN_POINT('Ctrl Pts',(-67.6263417083426,-19.0834236587118,
0.));
#81722=CARTESIAN_POINT('Ctrl Pts',(-67.6435687749841,-19.0939607887502,
0.));
#81723=CARTESIAN_POINT('Ctrl Pts',(-67.6608292549462,-19.1045435468358,
0.));
#81724=CARTESIAN_POINT('Ctrl Pts',(-67.6781229440573,-19.115171910846,0.));
#81725=CARTESIAN_POINT('Ctrl Pts',(-67.6954496350063,-19.1258458580345,
0.));
#81726=CARTESIAN_POINT('Ctrl Pts',(-67.7128091219348,-19.136565365709,0.));
#81727=CARTESIAN_POINT('Ctrl Pts',(-67.7302012056584,-19.1473304119955,
0.));
#81728=CARTESIAN_POINT('Ctrl Pts',(-67.7476256934444,-19.1581409758097,
0.));
#81729=CARTESIAN_POINT('Ctrl Pts',(-67.7650823965127,-19.168997036495,0.));
#81730=CARTESIAN_POINT('Ctrl Pts',(-67.7825711283096,-19.1798985735688,
0.));
#81731=CARTESIAN_POINT('Ctrl Pts',(-67.8000917023926,-19.1908455664098,
0.));
#81732=CARTESIAN_POINT('Ctrl Pts',(-67.8176439306621,-19.201837993993,0.));
#81733=CARTESIAN_POINT('Ctrl Pts',(-67.835227624289,-19.2128758350346,0.));
#81734=CARTESIAN_POINT('Ctrl Pts',(-67.8528425945184,-19.2239590681133,
0.));
#81735=CARTESIAN_POINT('Ctrl Pts',(-67.8704886534544,-19.2350876717874,
0.));
#81736=CARTESIAN_POINT('Ctrl Pts',(-67.8881656149955,-19.2462616247279,
0.));
#81737=CARTESIAN_POINT('Ctrl Pts',(-67.9058732951788,-19.2574809057696,
0.));
#81738=CARTESIAN_POINT('Ctrl Pts',(-67.9236115116758,-19.2687454938442,
0.));
#81739=CARTESIAN_POINT('Ctrl Pts',(-67.9413800834793,-19.280055367936,0.));
#81740=CARTESIAN_POINT('Ctrl Pts',(-67.9591788305394,-19.2914105070286,
0.));
#81741=CARTESIAN_POINT('Ctrl Pts',(-67.9770075733485,-19.302810890038,0.));
#81742=CARTESIAN_POINT('Ctrl Pts',(-67.9948661329617,-19.3142564958203,
0.));
#81743=CARTESIAN_POINT('Ctrl Pts',(-68.0127543311776,-19.3257473032035,
0.));
#81744=CARTESIAN_POINT('Ctrl Pts',(-68.0306719906636,-19.3372832910076,
0.));
#81745=CARTESIAN_POINT('Ctrl Pts',(-68.0486189351011,-19.3488644380641,
0.));
#81746=CARTESIAN_POINT('Ctrl Pts',(-68.0665949893195,-19.3604907232314,
0.));
#81747=CARTESIAN_POINT('Ctrl Pts',(-68.0845999792247,-19.3721621253912,
0.));
#81748=CARTESIAN_POINT('Ctrl Pts',(-68.1026337317285,-19.3838786234421,
0.));
#81749=CARTESIAN_POINT('Ctrl Pts',(-68.1206960746769,-19.3956401962895,
0.));
#81750=CARTESIAN_POINT('Ctrl Pts',(-68.1387868367691,-19.40744682283,0.));
#81751=CARTESIAN_POINT('Ctrl Pts',(-68.1569058475054,-19.4192984819418,
0.));
#81752=CARTESIAN_POINT('Ctrl Pts',(-68.1750529372232,-19.4311951524983,
0.));
#81753=CARTESIAN_POINT('Ctrl Pts',(-68.1932279371127,-19.4431368133719,
0.));
#81754=CARTESIAN_POINT('Ctrl Pts',(-68.2114306792358,-19.4551234434381,
0.));
#81755=CARTESIAN_POINT('Ctrl Pts',(-68.2296609965448,-19.467155021572,0.));
#81756=CARTESIAN_POINT('Ctrl Pts',(-68.2479187228803,-19.4792315266501,
0.));
#81757=CARTESIAN_POINT('Ctrl Pts',(-68.2662036929526,-19.4913529375543,
0.));
#81758=CARTESIAN_POINT('Ctrl Pts',(-68.2845157423233,-19.5035192331705,
0.));
#81759=CARTESIAN_POINT('Ctrl Pts',(-68.3028547073864,-19.5157303923856,
0.));
#81760=CARTESIAN_POINT('Ctrl Pts',(-68.3212204253417,-19.5279863940773,
0.));
#81761=CARTESIAN_POINT('Ctrl Pts',(-68.3396127341938,-19.5402872171191,
0.));
#81762=CARTESIAN_POINT('Ctrl Pts',(-68.3580314727523,-19.5526328403852,
0.));
#81763=CARTESIAN_POINT('Ctrl Pts',(-68.3764764806287,-19.5650232427516,
0.));
#81764=CARTESIAN_POINT('Ctrl Pts',(-68.3949475982335,-19.5774584030938,
0.));
#81765=CARTESIAN_POINT('Ctrl Pts',(-68.4134446667696,-19.5899383002803,
0.));
#81766=CARTESIAN_POINT('Ctrl Pts',(-68.4319675282275,-19.6024629131785,
0.));
#81767=CARTESIAN_POINT('Ctrl Pts',(-68.4505160253778,-19.6150322206577,
0.));
#81768=CARTESIAN_POINT('Ctrl Pts',(-68.4690900017632,-19.6276462015888,
0.));
#81769=CARTESIAN_POINT('Ctrl Pts',(-68.4876893016856,-19.6403048348395,
0.));
#81770=CARTESIAN_POINT('Ctrl Pts',(-68.5063137701971,-19.6530080992686,
0.));
#81771=CARTESIAN_POINT('Ctrl Pts',(-68.5249632530979,-19.6657559737336,
0.));
#81772=CARTESIAN_POINT('Ctrl Pts',(-68.5436375969311,-19.6785484370927,
0.));
#81773=CARTESIAN_POINT('Ctrl Pts',(-68.5623366489779,-19.6913854682046,
0.));
#81774=CARTESIAN_POINT('Ctrl Pts',(-68.581060257249,-19.7042670459237,0.));
#81775=CARTESIAN_POINT('Ctrl Pts',(-68.5998082704766,-19.7171931490956,
0.));
#81776=CARTESIAN_POINT('Ctrl Pts',(-68.6185805381126,-19.7301637565652,
0.));
#81777=CARTESIAN_POINT('Ctrl Pts',(-68.6373769103224,-19.7431788471776,
0.));
#81778=CARTESIAN_POINT('Ctrl Pts',(-68.6561972379793,-19.7562383997781,
0.));
#81779=CARTESIAN_POINT('Ctrl Pts',(-68.6750413726547,-19.7693423932058,
0.));
#81780=CARTESIAN_POINT('Ctrl Pts',(-68.6939091666111,-19.7824908062913,
0.));
#81781=CARTESIAN_POINT('Ctrl Pts',(-68.7128004727998,-19.795683617864,0.));
#81782=CARTESIAN_POINT('Ctrl Pts',(-68.7317151448557,-19.8089208067532,
0.));
#81783=CARTESIAN_POINT('Ctrl Pts',(-68.7506530370918,-19.8222023517874,
0.));
#81784=CARTESIAN_POINT('Ctrl Pts',(-68.7696140044892,-19.835528231787,0.));
#81785=CARTESIAN_POINT('Ctrl Pts',(-68.7885979026927,-19.8488984255642,
0.));
#81786=CARTESIAN_POINT('Ctrl Pts',(-68.8076045880102,-19.8623129119304,
0.));
#81787=CARTESIAN_POINT('Ctrl Pts',(-68.8266339174068,-19.8757716696969,
0.));
#81788=CARTESIAN_POINT('Ctrl Pts',(-68.8456857484988,-19.8892746776734,
0.));
#81789=CARTESIAN_POINT('Ctrl Pts',(-68.8647599395437,-19.9028219146607,
0.));
#81790=CARTESIAN_POINT('Ctrl Pts',(-68.8838563494356,-19.9164133594513,
0.));
#81791=CARTESIAN_POINT('Ctrl Pts',(-68.902974837704,-19.9300489908364,0.));
#81792=CARTESIAN_POINT('Ctrl Pts',(-68.9221152645086,-19.9437287876063,
0.));
#81793=CARTESIAN_POINT('Ctrl Pts',(-68.9412774906346,-19.9574527285492,
0.));
#81794=CARTESIAN_POINT('Ctrl Pts',(-68.960461377483,-19.9712207924437,0.));
#81795=CARTESIAN_POINT('Ctrl Pts',(-68.9796667870667,-19.98503295806,0.));
#81796=CARTESIAN_POINT('Ctrl Pts',(-68.9988935820101,-19.9988892041671,
0.));
#81797=CARTESIAN_POINT('Ctrl Pts',(-69.0181416255433,-20.0127895095327,
0.));
#81798=CARTESIAN_POINT('Ctrl Pts',(-69.0374107814977,-20.0267338529221,
0.));
#81799=CARTESIAN_POINT('Ctrl Pts',(-69.0567009142968,-20.0407222130902,
0.));
#81800=CARTESIAN_POINT('Ctrl Pts',(-69.0760118889525,-20.0547545687839,
0.));
#81801=CARTESIAN_POINT('Ctrl Pts',(-69.0953435710634,-20.0688308987478,
0.));
#81802=CARTESIAN_POINT('Ctrl Pts',(-69.1146958268104,-20.0829511817251,
0.));
#81803=CARTESIAN_POINT('Ctrl Pts',(-69.1340685229516,-20.0971153964557,
0.));
#81804=CARTESIAN_POINT('Ctrl Pts',(-69.1534615268153,-20.1113235216694,
0.));
#81805=CARTESIAN_POINT('Ctrl Pts',(-69.172874706296,-20.1255755360871,0.));
#81806=CARTESIAN_POINT('Ctrl Pts',(-69.1923079298534,-20.1398714184278,
0.));
#81807=CARTESIAN_POINT('Ctrl Pts',(-69.2117610665073,-20.1542111474086,
0.));
#81808=CARTESIAN_POINT('Ctrl Pts',(-69.2312339858337,-20.1685947017433,
0.));
#81809=CARTESIAN_POINT('Ctrl Pts',(-69.2507265579562,-20.183022060135,0.));
#81810=CARTESIAN_POINT('Ctrl Pts',(-69.2702386535432,-20.1974932012775,
0.));
#81811=CARTESIAN_POINT('Ctrl Pts',(-69.2897701438066,-20.2120081038622,
0.));
#81812=CARTESIAN_POINT('Ctrl Pts',(-69.3093209004986,-20.2265667465784,
0.));
#81813=CARTESIAN_POINT('Ctrl Pts',(-69.3288907959065,-20.2411691081122,
0.));
#81814=CARTESIAN_POINT('Ctrl Pts',(-69.3484797028454,-20.255815167139,0.));
#81815=CARTESIAN_POINT('Ctrl Pts',(-69.3680874946548,-20.2705049023241,
0.));
#81816=CARTESIAN_POINT('Ctrl Pts',(-69.3877140451975,-20.2852382923299,
0.));
#81817=CARTESIAN_POINT('Ctrl Pts',(-69.4073592288562,-20.3000153158167,
0.));
#81818=CARTESIAN_POINT('Ctrl Pts',(-69.4270229205296,-20.3148359514414,
0.));
#81819=CARTESIAN_POINT('Ctrl Pts',(-69.4467049956257,-20.3297001778505,
0.));
#81820=CARTESIAN_POINT('Ctrl Pts',(-69.4664053300579,-20.3446079736799,
0.));
#81821=CARTESIAN_POINT('Ctrl Pts',(-69.4861238002433,-20.359559317562,0.));
#81822=CARTESIAN_POINT('Ctrl Pts',(-69.5058602831004,-20.3745541881267,
0.));
#81823=CARTESIAN_POINT('Ctrl Pts',(-69.5256146560444,-20.3895925640006,
0.));
#81824=CARTESIAN_POINT('Ctrl Pts',(-69.5453867969815,-20.4046744238002,
0.));
#81825=CARTESIAN_POINT('Ctrl Pts',(-69.565176584305,-20.4197997461306,0.));
#81826=CARTESIAN_POINT('Ctrl Pts',(-69.5849838968944,-20.4349685095928,
0.));
#81827=CARTESIAN_POINT('Ctrl Pts',(-69.6048086141122,-20.4501806927854,
0.));
#81828=CARTESIAN_POINT('Ctrl Pts',(-69.6246506158009,-20.4654362743036,
0.));
#81829=CARTESIAN_POINT('Ctrl Pts',(-69.6445097822778,-20.4807352327335,
0.));
#81830=CARTESIAN_POINT('Ctrl Pts',(-69.6643859943291,-20.4960775466487,
0.));
#81831=CARTESIAN_POINT('Ctrl Pts',(-69.6842791332102,-20.511463194618,0.));
#81832=CARTESIAN_POINT('Ctrl Pts',(-69.7041890806421,-20.5268921552076,
0.));
#81833=CARTESIAN_POINT('Ctrl Pts',(-69.7241157188086,-20.54236440698,0.));
#81834=CARTESIAN_POINT('Ctrl Pts',(-69.7440589303511,-20.5578799284898,
0.));
#81835=CARTESIAN_POINT('Ctrl Pts',(-69.7640185983641,-20.5734386982782,
0.));
#81836=CARTESIAN_POINT('Ctrl Pts',(-69.7839946063942,-20.5890406948809,
0.));
#81837=CARTESIAN_POINT('Ctrl Pts',(-69.8039868384382,-20.6046858968305,
0.));
#81838=CARTESIAN_POINT('Ctrl Pts',(-69.8239951789402,-20.6203742826566,
0.));
#81839=CARTESIAN_POINT('Ctrl Pts',(-69.8440195127874,-20.6361058308812,
0.));
#81840=CARTESIAN_POINT('Ctrl Pts',(-69.8640597253058,-20.6518805200132,
0.));
#81841=CARTESIAN_POINT('Ctrl Pts',(-69.884115702258,-20.6676983285542,0.));
#81842=CARTESIAN_POINT('Ctrl Pts',(-69.9041873298416,-20.6835592350031,
0.));
#81843=CARTESIAN_POINT('Ctrl Pts',(-69.9242744946854,-20.6994632178551,
0.));
#81844=CARTESIAN_POINT('Ctrl Pts',(-69.9443770838444,-20.7154102555996,
0.));
#81845=CARTESIAN_POINT('Ctrl Pts',(-69.9644949847929,-20.7314003267118,
0.));
#81846=CARTESIAN_POINT('Ctrl Pts',(-69.9846280854254,-20.7474334096582,
0.));
#81847=CARTESIAN_POINT('Ctrl Pts',(-70.0047762740569,-20.7635094829017,
0.));
#81848=CARTESIAN_POINT('Ctrl Pts',(-70.0249394394221,-20.7796285249023,
0.));
#81849=CARTESIAN_POINT('Ctrl Pts',(-70.0451174706739,-20.7957905141155,
0.));
#81850=CARTESIAN_POINT('Ctrl Pts',(-70.0653102573798,-20.8119954289846,
0.));
#81851=CARTESIAN_POINT('Ctrl Pts',(-70.0855176895185,-20.8282432479425,
0.));
#81852=CARTESIAN_POINT('Ctrl Pts',(-70.1057396574741,-20.8445339494185,
0.));
#81853=CARTESIAN_POINT('Ctrl Pts',(-70.1259760520306,-20.8608675118377,
0.));
#81854=CARTESIAN_POINT('Ctrl Pts',(-70.1462267643649,-20.8772439136207,
0.));
#81855=CARTESIAN_POINT('Ctrl Pts',(-70.1664916860366,-20.8936631331751,
0.));
#81856=CARTESIAN_POINT('Ctrl Pts',(-70.1867707089866,-20.9101251488948,
0.));
#81857=CARTESIAN_POINT('Ctrl Pts',(-70.2070637255469,-20.9266299391688,
0.));
#81858=CARTESIAN_POINT('Ctrl Pts',(-70.2273706284479,-20.9431774823833,
0.));
#81859=CARTESIAN_POINT('Ctrl Pts',(-70.2476913108242,-20.9597677569227,
0.));
#81860=CARTESIAN_POINT('Ctrl Pts',(-70.2680256662215,-20.9764007411649,
0.));
#81861=CARTESIAN_POINT('Ctrl Pts',(-70.288373588597,-20.9930764134771,0.));
#81862=CARTESIAN_POINT('Ctrl Pts',(-70.3087349722959,-21.0097947522212,
0.));
#81863=CARTESIAN_POINT('Ctrl Pts',(-70.3291097120293,-21.0265557357544,
0.));
#81864=CARTESIAN_POINT('Ctrl Pts',(-70.3494977028497,-21.0433593424266,
0.));
#81865=CARTESIAN_POINT('Ctrl Pts',(-70.3698988401291,-21.0602055505751,
0.));
#81866=CARTESIAN_POINT('Ctrl Pts',(-70.3903130195279,-21.0770943385146,
0.));
#81867=CARTESIAN_POINT('Ctrl Pts',(-70.4107401370403,-21.0940256845477,
0.));
#81868=CARTESIAN_POINT('Ctrl Pts',(-70.4311800890411,-21.110999566975,0.));
#81869=CARTESIAN_POINT('Ctrl Pts',(-70.4516327723349,-21.1280159641003,
0.));
#81870=CARTESIAN_POINT('Ctrl Pts',(-70.4720980841934,-21.1450748542335,
0.));
#81871=CARTESIAN_POINT('Ctrl Pts',(-70.4925759224208,-21.1621762156894,
0.));
#81872=CARTESIAN_POINT('Ctrl Pts',(-70.5130661852946,-21.1793200267844,
0.));
#81873=CARTESIAN_POINT('Ctrl Pts',(-70.5335687714422,-21.1965062658296,
0.));
#81874=CARTESIAN_POINT('Ctrl Pts',(-70.5540835797281,-21.2137349111207,
0.));
#81875=CARTESIAN_POINT('Ctrl Pts',(-70.5746105091503,-21.2310059409265,
0.));
#81876=CARTESIAN_POINT('Ctrl Pts',(-70.5951494586961,-21.2483193334677,
0.));
#81877=CARTESIAN_POINT('Ctrl Pts',(-70.6157003273326,-21.2656750669129,
0.));
#81878=CARTESIAN_POINT('Ctrl Pts',(-70.6362630143062,-21.2830731194188,
0.));
#81879=CARTESIAN_POINT('Ctrl Pts',(-70.6568374193786,-21.3005134691563,
0.));
#81880=CARTESIAN_POINT('Ctrl Pts',(-70.6774234430899,-21.3179960943389,
0.));
#81881=CARTESIAN_POINT('Ctrl Pts',(-70.6980209870032,-21.3355209732438,
0.));
#81882=CARTESIAN_POINT('Ctrl Pts',(-70.7186299539698,-21.353088084234,0.));
#81883=CARTESIAN_POINT('Ctrl Pts',(-70.7392502475437,-21.3706974057028,
0.));
#81884=CARTESIAN_POINT('Ctrl Pts',(-70.7598817714078,-21.3883489160187,
0.));
#81885=CARTESIAN_POINT('Ctrl Pts',(-70.780524428744,-21.4060425934595,0.));
#81886=CARTESIAN_POINT('Ctrl Pts',(-70.8011781217409,-21.4237784161592,
0.));
#81887=CARTESIAN_POINT('Ctrl Pts',(-70.8218427507545,-21.4415563620127,
0.));
#81888=CARTESIAN_POINT('Ctrl Pts',(-70.84251821499,-21.4593764087492,0.));
#81889=CARTESIAN_POINT('Ctrl Pts',(-70.8632044140166,-21.4772385340978,
0.));
#81890=CARTESIAN_POINT('Ctrl Pts',(-70.8839012490903,-21.4951427159272,
0.));
#81891=CARTESIAN_POINT('Ctrl Pts',(-70.9046086244123,-21.5130889323767,
0.));
#81892=CARTESIAN_POINT('Ctrl Pts',(-70.9253264487576,-21.5310771620209,
0.));
#81893=CARTESIAN_POINT('Ctrl Pts',(-70.9460546358597,-21.549107383907,0.));
#81894=CARTESIAN_POINT('Ctrl Pts',(-70.9638315189647,-21.5645987555282,
0.));
#81895=CARTESIAN_POINT('Ctrl Pts',(-70.9774662112376,-21.5764983366351,
0.));
#81896=CARTESIAN_POINT('Ctrl Pts',(-70.9869541807809,-21.5847875433161,
0.));
#81897=CARTESIAN_POINT('Ctrl Pts',(-70.9922924595083,-21.589454092537,0.));
#81898=CARTESIAN_POINT('Ctrl Pts',(-70.993479606878,-21.5904919934802,0.));
#81899=CARTESIAN_POINT('',(-67.3887914263118,-18.9407177820969,12.));
#81900=CARTESIAN_POINT('',(-67.3887914263118,-18.9407177820969,0.));
#81901=CARTESIAN_POINT('Ctrl Pts',(-70.993479606878,-21.5904919934802,12.));
#81902=CARTESIAN_POINT('Ctrl Pts',(-70.9922924595083,-21.589454092537,12.));
#81903=CARTESIAN_POINT('Ctrl Pts',(-70.9869541807809,-21.5847875433161,
12.));
#81904=CARTESIAN_POINT('Ctrl Pts',(-70.9774662112376,-21.5764983366351,
12.));
#81905=CARTESIAN_POINT('Ctrl Pts',(-70.9638315189647,-21.5645987555282,
12.));
#81906=CARTESIAN_POINT('Ctrl Pts',(-70.9460546358597,-21.549107383907,12.));
#81907=CARTESIAN_POINT('Ctrl Pts',(-70.9253264487576,-21.5310771620209,
12.));
#81908=CARTESIAN_POINT('Ctrl Pts',(-70.9046086244123,-21.5130889323767,
12.));
#81909=CARTESIAN_POINT('Ctrl Pts',(-70.8839012490903,-21.4951427159272,
12.));
#81910=CARTESIAN_POINT('Ctrl Pts',(-70.8632044140166,-21.4772385340978,
12.));
#81911=CARTESIAN_POINT('Ctrl Pts',(-70.84251821499,-21.4593764087492,12.));
#81912=CARTESIAN_POINT('Ctrl Pts',(-70.8218427507545,-21.4415563620127,
12.));
#81913=CARTESIAN_POINT('Ctrl Pts',(-70.8011781217409,-21.4237784161592,
12.));
#81914=CARTESIAN_POINT('Ctrl Pts',(-70.780524428744,-21.4060425934595,12.));
#81915=CARTESIAN_POINT('Ctrl Pts',(-70.7598817714078,-21.3883489160187,
12.));
#81916=CARTESIAN_POINT('Ctrl Pts',(-70.7392502475437,-21.3706974057028,
12.));
#81917=CARTESIAN_POINT('Ctrl Pts',(-70.7186299539698,-21.353088084234,12.));
#81918=CARTESIAN_POINT('Ctrl Pts',(-70.6980209870032,-21.3355209732438,
12.));
#81919=CARTESIAN_POINT('Ctrl Pts',(-70.6774234430899,-21.3179960943389,
12.));
#81920=CARTESIAN_POINT('Ctrl Pts',(-70.6568374193786,-21.3005134691563,
12.));
#81921=CARTESIAN_POINT('Ctrl Pts',(-70.6362630143062,-21.2830731194188,
12.));
#81922=CARTESIAN_POINT('Ctrl Pts',(-70.6157003273326,-21.2656750669129,
12.));
#81923=CARTESIAN_POINT('Ctrl Pts',(-70.5951494586961,-21.2483193334677,
12.));
#81924=CARTESIAN_POINT('Ctrl Pts',(-70.5746105091503,-21.2310059409265,
12.));
#81925=CARTESIAN_POINT('Ctrl Pts',(-70.5540835797281,-21.2137349111207,
12.));
#81926=CARTESIAN_POINT('Ctrl Pts',(-70.5335687714422,-21.1965062658296,
12.));
#81927=CARTESIAN_POINT('Ctrl Pts',(-70.5130661852946,-21.1793200267844,
12.));
#81928=CARTESIAN_POINT('Ctrl Pts',(-70.4925759224208,-21.1621762156894,
12.));
#81929=CARTESIAN_POINT('Ctrl Pts',(-70.4720980841934,-21.1450748542335,
12.));
#81930=CARTESIAN_POINT('Ctrl Pts',(-70.4516327723349,-21.1280159641003,
12.));
#81931=CARTESIAN_POINT('Ctrl Pts',(-70.4311800890411,-21.110999566975,12.));
#81932=CARTESIAN_POINT('Ctrl Pts',(-70.4107401370403,-21.0940256845477,
12.));
#81933=CARTESIAN_POINT('Ctrl Pts',(-70.3903130195279,-21.0770943385146,
12.));
#81934=CARTESIAN_POINT('Ctrl Pts',(-70.3698988401291,-21.0602055505751,
12.));
#81935=CARTESIAN_POINT('Ctrl Pts',(-70.3494977028497,-21.0433593424266,
12.));
#81936=CARTESIAN_POINT('Ctrl Pts',(-70.3291097120293,-21.0265557357544,
12.));
#81937=CARTESIAN_POINT('Ctrl Pts',(-70.3087349722959,-21.0097947522212,
12.));
#81938=CARTESIAN_POINT('Ctrl Pts',(-70.288373588597,-20.9930764134771,12.));
#81939=CARTESIAN_POINT('Ctrl Pts',(-70.2680256662215,-20.9764007411649,
12.));
#81940=CARTESIAN_POINT('Ctrl Pts',(-70.2476913108242,-20.9597677569227,
12.));
#81941=CARTESIAN_POINT('Ctrl Pts',(-70.2273706284479,-20.9431774823833,
12.));
#81942=CARTESIAN_POINT('Ctrl Pts',(-70.2070637255469,-20.9266299391688,
12.));
#81943=CARTESIAN_POINT('Ctrl Pts',(-70.1867707089866,-20.9101251488948,
12.));
#81944=CARTESIAN_POINT('Ctrl Pts',(-70.1664916860366,-20.8936631331751,
12.));
#81945=CARTESIAN_POINT('Ctrl Pts',(-70.1462267643649,-20.8772439136207,
12.));
#81946=CARTESIAN_POINT('Ctrl Pts',(-70.1259760520306,-20.8608675118377,
12.));
#81947=CARTESIAN_POINT('Ctrl Pts',(-70.1057396574741,-20.8445339494185,
12.));
#81948=CARTESIAN_POINT('Ctrl Pts',(-70.0855176895185,-20.8282432479425,
12.));
#81949=CARTESIAN_POINT('Ctrl Pts',(-70.0653102573798,-20.8119954289846,
12.));
#81950=CARTESIAN_POINT('Ctrl Pts',(-70.0451174706739,-20.7957905141155,
12.));
#81951=CARTESIAN_POINT('Ctrl Pts',(-70.0249394394221,-20.7796285249023,
12.));
#81952=CARTESIAN_POINT('Ctrl Pts',(-70.0047762740569,-20.7635094829017,
12.));
#81953=CARTESIAN_POINT('Ctrl Pts',(-69.9846280854254,-20.7474334096582,
12.));
#81954=CARTESIAN_POINT('Ctrl Pts',(-69.9644949847929,-20.7314003267118,
12.));
#81955=CARTESIAN_POINT('Ctrl Pts',(-69.9443770838444,-20.7154102555996,
12.));
#81956=CARTESIAN_POINT('Ctrl Pts',(-69.9242744946854,-20.6994632178551,
12.));
#81957=CARTESIAN_POINT('Ctrl Pts',(-69.9041873298416,-20.6835592350031,
12.));
#81958=CARTESIAN_POINT('Ctrl Pts',(-69.884115702258,-20.6676983285542,12.));
#81959=CARTESIAN_POINT('Ctrl Pts',(-69.8640597253058,-20.6518805200132,
12.));
#81960=CARTESIAN_POINT('Ctrl Pts',(-69.8440195127874,-20.6361058308812,
12.));
#81961=CARTESIAN_POINT('Ctrl Pts',(-69.8239951789402,-20.6203742826566,
12.));
#81962=CARTESIAN_POINT('Ctrl Pts',(-69.8039868384382,-20.6046858968305,
12.));
#81963=CARTESIAN_POINT('Ctrl Pts',(-69.7839946063942,-20.5890406948809,
12.));
#81964=CARTESIAN_POINT('Ctrl Pts',(-69.7640185983641,-20.5734386982782,
12.));
#81965=CARTESIAN_POINT('Ctrl Pts',(-69.7440589303511,-20.5578799284898,
12.));
#81966=CARTESIAN_POINT('Ctrl Pts',(-69.7241157188086,-20.54236440698,12.));
#81967=CARTESIAN_POINT('Ctrl Pts',(-69.7041890806421,-20.5268921552076,
12.));
#81968=CARTESIAN_POINT('Ctrl Pts',(-69.6842791332102,-20.511463194618,12.));
#81969=CARTESIAN_POINT('Ctrl Pts',(-69.6643859943291,-20.4960775466487,
12.));
#81970=CARTESIAN_POINT('Ctrl Pts',(-69.6445097822778,-20.4807352327335,
12.));
#81971=CARTESIAN_POINT('Ctrl Pts',(-69.6246506158009,-20.4654362743036,
12.));
#81972=CARTESIAN_POINT('Ctrl Pts',(-69.6048086141122,-20.4501806927854,
12.));
#81973=CARTESIAN_POINT('Ctrl Pts',(-69.5849838968944,-20.4349685095928,
12.));
#81974=CARTESIAN_POINT('Ctrl Pts',(-69.565176584305,-20.4197997461306,12.));
#81975=CARTESIAN_POINT('Ctrl Pts',(-69.5453867969815,-20.4046744238002,
12.));
#81976=CARTESIAN_POINT('Ctrl Pts',(-69.5256146560444,-20.3895925640006,
12.));
#81977=CARTESIAN_POINT('Ctrl Pts',(-69.5058602831004,-20.3745541881267,
12.));
#81978=CARTESIAN_POINT('Ctrl Pts',(-69.4861238002433,-20.359559317562,12.));
#81979=CARTESIAN_POINT('Ctrl Pts',(-69.4664053300579,-20.3446079736799,
12.));
#81980=CARTESIAN_POINT('Ctrl Pts',(-69.4467049956257,-20.3297001778505,
12.));
#81981=CARTESIAN_POINT('Ctrl Pts',(-69.4270229205296,-20.3148359514414,
12.));
#81982=CARTESIAN_POINT('Ctrl Pts',(-69.4073592288562,-20.3000153158167,
12.));
#81983=CARTESIAN_POINT('Ctrl Pts',(-69.3877140451975,-20.2852382923299,
12.));
#81984=CARTESIAN_POINT('Ctrl Pts',(-69.3680874946548,-20.2705049023241,
12.));
#81985=CARTESIAN_POINT('Ctrl Pts',(-69.3484797028454,-20.255815167139,12.));
#81986=CARTESIAN_POINT('Ctrl Pts',(-69.3288907959065,-20.2411691081122,
12.));
#81987=CARTESIAN_POINT('Ctrl Pts',(-69.3093209004986,-20.2265667465784,
12.));
#81988=CARTESIAN_POINT('Ctrl Pts',(-69.2897701438066,-20.2120081038622,
12.));
#81989=CARTESIAN_POINT('Ctrl Pts',(-69.2702386535432,-20.1974932012775,
12.));
#81990=CARTESIAN_POINT('Ctrl Pts',(-69.2507265579562,-20.183022060135,12.));
#81991=CARTESIAN_POINT('Ctrl Pts',(-69.2312339858337,-20.1685947017433,
12.));
#81992=CARTESIAN_POINT('Ctrl Pts',(-69.2117610665073,-20.1542111474086,
12.));
#81993=CARTESIAN_POINT('Ctrl Pts',(-69.1923079298534,-20.1398714184278,
12.));
#81994=CARTESIAN_POINT('Ctrl Pts',(-69.172874706296,-20.1255755360871,12.));
#81995=CARTESIAN_POINT('Ctrl Pts',(-69.1534615268153,-20.1113235216694,
12.));
#81996=CARTESIAN_POINT('Ctrl Pts',(-69.1340685229516,-20.0971153964557,
12.));
#81997=CARTESIAN_POINT('Ctrl Pts',(-69.1146958268104,-20.0829511817251,
12.));
#81998=CARTESIAN_POINT('Ctrl Pts',(-69.0953435710634,-20.0688308987478,
12.));
#81999=CARTESIAN_POINT('Ctrl Pts',(-69.0760118889525,-20.0547545687839,
12.));
#82000=CARTESIAN_POINT('Ctrl Pts',(-69.0567009142968,-20.0407222130902,
12.));
#82001=CARTESIAN_POINT('Ctrl Pts',(-69.0374107814977,-20.0267338529221,
12.));
#82002=CARTESIAN_POINT('Ctrl Pts',(-69.0181416255433,-20.0127895095327,
12.));
#82003=CARTESIAN_POINT('Ctrl Pts',(-68.9988935820101,-19.9988892041671,
12.));
#82004=CARTESIAN_POINT('Ctrl Pts',(-68.9796667870667,-19.98503295806,12.));
#82005=CARTESIAN_POINT('Ctrl Pts',(-68.960461377483,-19.9712207924437,12.));
#82006=CARTESIAN_POINT('Ctrl Pts',(-68.9412774906346,-19.9574527285492,
12.));
#82007=CARTESIAN_POINT('Ctrl Pts',(-68.9221152645086,-19.9437287876063,
12.));
#82008=CARTESIAN_POINT('Ctrl Pts',(-68.902974837704,-19.9300489908364,12.));
#82009=CARTESIAN_POINT('Ctrl Pts',(-68.8838563494356,-19.9164133594513,
12.));
#82010=CARTESIAN_POINT('Ctrl Pts',(-68.8647599395437,-19.9028219146607,
12.));
#82011=CARTESIAN_POINT('Ctrl Pts',(-68.8456857484988,-19.8892746776734,
12.));
#82012=CARTESIAN_POINT('Ctrl Pts',(-68.8266339174068,-19.8757716696969,
12.));
#82013=CARTESIAN_POINT('Ctrl Pts',(-68.8076045880102,-19.8623129119304,
12.));
#82014=CARTESIAN_POINT('Ctrl Pts',(-68.7885979026927,-19.8488984255642,
12.));
#82015=CARTESIAN_POINT('Ctrl Pts',(-68.7696140044892,-19.835528231787,12.));
#82016=CARTESIAN_POINT('Ctrl Pts',(-68.7506530370918,-19.8222023517874,
12.));
#82017=CARTESIAN_POINT('Ctrl Pts',(-68.7317151448557,-19.8089208067532,
12.));
#82018=CARTESIAN_POINT('Ctrl Pts',(-68.7128004727998,-19.795683617864,12.));
#82019=CARTESIAN_POINT('Ctrl Pts',(-68.6939091666111,-19.7824908062913,
12.));
#82020=CARTESIAN_POINT('Ctrl Pts',(-68.6750413726547,-19.7693423932058,
12.));
#82021=CARTESIAN_POINT('Ctrl Pts',(-68.6561972379793,-19.7562383997781,
12.));
#82022=CARTESIAN_POINT('Ctrl Pts',(-68.6373769103224,-19.7431788471776,
12.));
#82023=CARTESIAN_POINT('Ctrl Pts',(-68.6185805381126,-19.7301637565652,
12.));
#82024=CARTESIAN_POINT('Ctrl Pts',(-68.5998082704766,-19.7171931490956,
12.));
#82025=CARTESIAN_POINT('Ctrl Pts',(-68.581060257249,-19.7042670459237,12.));
#82026=CARTESIAN_POINT('Ctrl Pts',(-68.5623366489779,-19.6913854682046,
12.));
#82027=CARTESIAN_POINT('Ctrl Pts',(-68.5436375969311,-19.6785484370927,
12.));
#82028=CARTESIAN_POINT('Ctrl Pts',(-68.5249632530979,-19.6657559737336,
12.));
#82029=CARTESIAN_POINT('Ctrl Pts',(-68.5063137701971,-19.6530080992686,
12.));
#82030=CARTESIAN_POINT('Ctrl Pts',(-68.4876893016856,-19.6403048348395,
12.));
#82031=CARTESIAN_POINT('Ctrl Pts',(-68.4690900017632,-19.6276462015888,
12.));
#82032=CARTESIAN_POINT('Ctrl Pts',(-68.4505160253778,-19.6150322206577,
12.));
#82033=CARTESIAN_POINT('Ctrl Pts',(-68.4319675282275,-19.6024629131785,
12.));
#82034=CARTESIAN_POINT('Ctrl Pts',(-68.4134446667696,-19.5899383002803,
12.));
#82035=CARTESIAN_POINT('Ctrl Pts',(-68.3949475982335,-19.5774584030938,
12.));
#82036=CARTESIAN_POINT('Ctrl Pts',(-68.3764764806287,-19.5650232427516,
12.));
#82037=CARTESIAN_POINT('Ctrl Pts',(-68.3580314727523,-19.5526328403852,
12.));
#82038=CARTESIAN_POINT('Ctrl Pts',(-68.3396127341938,-19.5402872171191,
12.));
#82039=CARTESIAN_POINT('Ctrl Pts',(-68.3212204253417,-19.5279863940773,
12.));
#82040=CARTESIAN_POINT('Ctrl Pts',(-68.3028547073864,-19.5157303923856,
12.));
#82041=CARTESIAN_POINT('Ctrl Pts',(-68.2845157423233,-19.5035192331705,
12.));
#82042=CARTESIAN_POINT('Ctrl Pts',(-68.2662036929526,-19.4913529375543,
12.));
#82043=CARTESIAN_POINT('Ctrl Pts',(-68.2479187228803,-19.4792315266501,
12.));
#82044=CARTESIAN_POINT('Ctrl Pts',(-68.2296609965448,-19.467155021572,12.));
#82045=CARTESIAN_POINT('Ctrl Pts',(-68.2114306792358,-19.4551234434381,
12.));
#82046=CARTESIAN_POINT('Ctrl Pts',(-68.1932279371127,-19.4431368133719,
12.));
#82047=CARTESIAN_POINT('Ctrl Pts',(-68.1750529372232,-19.4311951524983,
12.));
#82048=CARTESIAN_POINT('Ctrl Pts',(-68.1569058475054,-19.4192984819418,
12.));
#82049=CARTESIAN_POINT('Ctrl Pts',(-68.1387868367691,-19.40744682283,12.));
#82050=CARTESIAN_POINT('Ctrl Pts',(-68.1206960746769,-19.3956401962895,
12.));
#82051=CARTESIAN_POINT('Ctrl Pts',(-68.1026337317285,-19.3838786234421,
12.));
#82052=CARTESIAN_POINT('Ctrl Pts',(-68.0845999792247,-19.3721621253912,
12.));
#82053=CARTESIAN_POINT('Ctrl Pts',(-68.0665949893195,-19.3604907232314,
12.));
#82054=CARTESIAN_POINT('Ctrl Pts',(-68.0486189351011,-19.3488644380641,
12.));
#82055=CARTESIAN_POINT('Ctrl Pts',(-68.0306719906636,-19.3372832910076,
12.));
#82056=CARTESIAN_POINT('Ctrl Pts',(-68.0127543311776,-19.3257473032035,
12.));
#82057=CARTESIAN_POINT('Ctrl Pts',(-67.9948661329617,-19.3142564958203,
12.));
#82058=CARTESIAN_POINT('Ctrl Pts',(-67.9770075733485,-19.302810890038,12.));
#82059=CARTESIAN_POINT('Ctrl Pts',(-67.9591788305394,-19.2914105070286,
12.));
#82060=CARTESIAN_POINT('Ctrl Pts',(-67.9413800834793,-19.280055367936,12.));
#82061=CARTESIAN_POINT('Ctrl Pts',(-67.9236115116758,-19.2687454938442,
12.));
#82062=CARTESIAN_POINT('Ctrl Pts',(-67.9058732951788,-19.2574809057696,
12.));
#82063=CARTESIAN_POINT('Ctrl Pts',(-67.8881656149955,-19.2462616247279,
12.));
#82064=CARTESIAN_POINT('Ctrl Pts',(-67.8704886534544,-19.2350876717874,
12.));
#82065=CARTESIAN_POINT('Ctrl Pts',(-67.8528425945184,-19.2239590681133,
12.));
#82066=CARTESIAN_POINT('Ctrl Pts',(-67.835227624289,-19.2128758350346,12.));
#82067=CARTESIAN_POINT('Ctrl Pts',(-67.8176439306621,-19.201837993993,12.));
#82068=CARTESIAN_POINT('Ctrl Pts',(-67.8000917023926,-19.1908455664098,
12.));
#82069=CARTESIAN_POINT('Ctrl Pts',(-67.7825711283096,-19.1798985735688,
12.));
#82070=CARTESIAN_POINT('Ctrl Pts',(-67.7650823965127,-19.168997036495,12.));
#82071=CARTESIAN_POINT('Ctrl Pts',(-67.7476256934444,-19.1581409758097,
12.));
#82072=CARTESIAN_POINT('Ctrl Pts',(-67.7302012056584,-19.1473304119955,
12.));
#82073=CARTESIAN_POINT('Ctrl Pts',(-67.7128091219348,-19.136565365709,12.));
#82074=CARTESIAN_POINT('Ctrl Pts',(-67.6954496350063,-19.1258458580345,
12.));
#82075=CARTESIAN_POINT('Ctrl Pts',(-67.6781229440573,-19.115171910846,12.));
#82076=CARTESIAN_POINT('Ctrl Pts',(-67.6608292549462,-19.1045435468358,
12.));
#82077=CARTESIAN_POINT('Ctrl Pts',(-67.6435687749841,-19.0939607887502,
12.));
#82078=CARTESIAN_POINT('Ctrl Pts',(-67.6263417083426,-19.0834236587118,
12.));
#82079=CARTESIAN_POINT('Ctrl Pts',(-67.6091482520534,-19.072932177628,12.));
#82080=CARTESIAN_POINT('Ctrl Pts',(-67.5919885896222,-19.062486364241,12.));
#82081=CARTESIAN_POINT('Ctrl Pts',(-67.5748628971964,-19.0520862360396,
12.));
#82082=CARTESIAN_POINT('Ctrl Pts',(-67.5577713558194,-19.0417318110708,
12.));
#82083=CARTESIAN_POINT('Ctrl Pts',(-67.540714161288,-19.0314231093923,12.));
#82084=CARTESIAN_POINT('Ctrl Pts',(-67.5236915360331,-19.021160154824,12.));
#82085=CARTESIAN_POINT('Ctrl Pts',(-67.5067037372317,-19.0109429761306,
12.));
#82086=CARTESIAN_POINT('Ctrl Pts',(-67.4897510316844,-19.0007716032819,
12.));
#82087=CARTESIAN_POINT('Ctrl Pts',(-67.472833671964,-18.9906460638625,12.));
#82088=CARTESIAN_POINT('Ctrl Pts',(-67.4559518744638,-18.9805663798449,
12.));
#82089=CARTESIAN_POINT('Ctrl Pts',(-67.4391057908418,-18.9705325631711,
12.));
#82090=CARTESIAN_POINT('Ctrl Pts',(-67.4222955061981,-18.9605446160985,
12.));
#82091=CARTESIAN_POINT('Ctrl Pts',(-67.4088759497911,-18.9525909517915,
12.));
#82092=CARTESIAN_POINT('Ctrl Pts',(-67.3988274146651,-18.9466463414299,
12.));
#82093=CARTESIAN_POINT('Ctrl Pts',(-67.3921355608328,-18.9426924398719,
12.));
#82094=CARTESIAN_POINT('Ctrl Pts',(-67.3887914263118,-18.9407177820969,
12.));
#82095=CARTESIAN_POINT('Ctrl Pts',(-70.538251407892,-23.0342913834073,-1.11022302462516E-15));
#82096=CARTESIAN_POINT('Ctrl Pts',(-70.538251407892,-23.0342913834073,4.));
#82097=CARTESIAN_POINT('Ctrl Pts',(-70.538251407892,-23.0342913834073,8.));
#82098=CARTESIAN_POINT('Ctrl Pts',(-70.538251407892,-23.0342913834073,12.));
#82099=CARTESIAN_POINT('Ctrl Pts',(-70.6474988907591,-23.0224954570734,
-1.11022302462516E-15));
#82100=CARTESIAN_POINT('Ctrl Pts',(-70.6474988907591,-23.0224954570734,
4.));
#82101=CARTESIAN_POINT('Ctrl Pts',(-70.6474988907591,-23.0224954570734,
8.00000000000001));
#82102=CARTESIAN_POINT('Ctrl Pts',(-70.6474988907591,-23.0224954570734,
12.));
#82103=CARTESIAN_POINT('Ctrl Pts',(-70.83100071469,-22.9364730048789,-1.11022302462516E-15));
#82104=CARTESIAN_POINT('Ctrl Pts',(-70.83100071469,-22.9364730048789,4.));
#82105=CARTESIAN_POINT('Ctrl Pts',(-70.83100071469,-22.936473004879,7.99999999999999));
#82106=CARTESIAN_POINT('Ctrl Pts',(-70.83100071469,-22.936473004879,12.));
#82107=CARTESIAN_POINT('Ctrl Pts',(-70.9357242819029,-22.7679558220498,
-1.11022302462516E-15));
#82108=CARTESIAN_POINT('Ctrl Pts',(-70.9357242819029,-22.7679558220498,
4.));
#82109=CARTESIAN_POINT('Ctrl Pts',(-70.935724281903,-22.7679558220499,8.00000000000001));
#82110=CARTESIAN_POINT('Ctrl Pts',(-70.935724281903,-22.7679558220499,12.));
#82111=CARTESIAN_POINT('Ctrl Pts',(-70.9608233461354,-22.6894590071812,
-1.11022302462516E-15));
#82112=CARTESIAN_POINT('Ctrl Pts',(-70.9608233461354,-22.6894590071812,
4.));
#82113=CARTESIAN_POINT('Ctrl Pts',(-70.9608233461355,-22.6894590071812,
8.));
#82114=CARTESIAN_POINT('Ctrl Pts',(-70.9608233461355,-22.6894590071812,
12.));
#82115=CARTESIAN_POINT('',(-70.538251407892,-23.0342913834073,0.));
#82116=CARTESIAN_POINT('',(-70.9608233461355,-22.6894590071813,2.77555756156289E-16));
#82117=CARTESIAN_POINT('Ctrl Pts',(-70.538251407892,-23.0342913834073,0.));
#82118=CARTESIAN_POINT('Ctrl Pts',(-70.6474988907591,-23.0224954570734,
-3.08148791101957E-31));
#82119=CARTESIAN_POINT('Ctrl Pts',(-70.7523570758625,-22.9733397701051,
4.3140830754274E-31));
#82120=CARTESIAN_POINT('Ctrl Pts',(-70.8314917485681,-22.8972470282358,
0.));
#82121=CARTESIAN_POINT('Ctrl Pts',(-70.8908427530974,-22.8401774718337,
-1.54074395550979E-31));
#82122=CARTESIAN_POINT('Ctrl Pts',(-70.9357242819029,-22.7679558220498,
-9.24446373305873E-31));
#82123=CARTESIAN_POINT('Ctrl Pts',(-70.9608233461354,-22.6894590071812,
3.28429327576129E-46));
#82124=CARTESIAN_POINT('',(-70.9608233461355,-22.6894590071812,12.));
#82125=CARTESIAN_POINT('Ctrl Pts',(-70.9608233461354,-22.6894590071812,
-1.11022302462516E-15));
#82126=CARTESIAN_POINT('Ctrl Pts',(-70.9608233461354,-22.6894590071812,
4.));
#82127=CARTESIAN_POINT('Ctrl Pts',(-70.9608233461355,-22.6894590071812,
8.));
#82128=CARTESIAN_POINT('Ctrl Pts',(-70.9608233461355,-22.6894590071812,
12.));
#82129=CARTESIAN_POINT('',(-70.538251407892,-23.0342913834073,12.));
#82130=CARTESIAN_POINT('Ctrl Pts',(-70.9608233461355,-22.6894590071812,
12.));
#82131=CARTESIAN_POINT('Ctrl Pts',(-70.935724281903,-22.7679558220499,12.));
#82132=CARTESIAN_POINT('Ctrl Pts',(-70.8908427530974,-22.8401774718338,
12.));
#82133=CARTESIAN_POINT('Ctrl Pts',(-70.8314917485682,-22.8972470282358,
12.));
#82134=CARTESIAN_POINT('Ctrl Pts',(-70.7523570758625,-22.9733397701052,
12.));
#82135=CARTESIAN_POINT('Ctrl Pts',(-70.6474988907591,-23.0224954570734,
12.));
#82136=CARTESIAN_POINT('Ctrl Pts',(-70.538251407892,-23.0342913834073,12.));
#82137=CARTESIAN_POINT('Ctrl Pts',(-70.538251407892,-23.0342913834073,12.));
#82138=CARTESIAN_POINT('Ctrl Pts',(-70.538251407892,-23.0342913834073,8.));
#82139=CARTESIAN_POINT('Ctrl Pts',(-70.538251407892,-23.0342913834073,4.));
#82140=CARTESIAN_POINT('Ctrl Pts',(-70.538251407892,-23.0342913834073,-1.11022302462516E-15));
#82141=CARTESIAN_POINT('Origin',(-3.57465004850839E-10,-1.12812358559725E-10,
0.));
#82142=CARTESIAN_POINT('Origin',(-3.57465004850839E-10,-1.12812358559725E-10,
12.));
#82143=CARTESIAN_POINT('Origin',(-3.57465004850839E-10,-1.12812358559725E-10,
0.));
#82144=CARTESIAN_POINT('Ctrl Pts',(-72.7986051948032,-15.8307637747259,
-1.11022302462516E-15));
#82145=CARTESIAN_POINT('Ctrl Pts',(-72.7986051948032,-15.8307637747259,
4.));
#82146=CARTESIAN_POINT('Ctrl Pts',(-72.7986051948032,-15.8307637747259,
8.));
#82147=CARTESIAN_POINT('Ctrl Pts',(-72.7986051948032,-15.8307637747259,
12.));
#82148=CARTESIAN_POINT('Ctrl Pts',(-72.8219545017353,-15.7233907508395,
-1.11022302462516E-15));
#82149=CARTESIAN_POINT('Ctrl Pts',(-72.8219545017353,-15.7233907508395,
3.99999999999999));
#82150=CARTESIAN_POINT('Ctrl Pts',(-72.8219545017353,-15.7233907508395,
8.));
#82151=CARTESIAN_POINT('Ctrl Pts',(-72.8219545017353,-15.7233907508395,
12.));
#82152=CARTESIAN_POINT('Ctrl Pts',(-72.7983622347338,-15.5221041200722,
-1.0371419571966E-15));
#82153=CARTESIAN_POINT('Ctrl Pts',(-72.7983622347338,-15.5221041200722,
4.00000000000001));
#82154=CARTESIAN_POINT('Ctrl Pts',(-72.7983622347338,-15.5221041200722,
8.));
#82155=CARTESIAN_POINT('Ctrl Pts',(-72.7983622347338,-15.5221041200722,
12.));
#82156=CARTESIAN_POINT('Ctrl Pts',(-72.6715981986666,-15.3694736926919,
-8.63611844393267E-16));
#82157=CARTESIAN_POINT('Ctrl Pts',(-72.6715981986666,-15.3694736926919,
3.99999999999999));
#82158=CARTESIAN_POINT('Ctrl Pts',(-72.6715981986666,-15.3694736926919,
8.));
#82159=CARTESIAN_POINT('Ctrl Pts',(-72.6715981986666,-15.3694736926919,
12.));
#82160=CARTESIAN_POINT('Ctrl Pts',(-72.6050633494357,-15.3208442077191,
-7.79957864156004E-16));
#82161=CARTESIAN_POINT('Ctrl Pts',(-72.6050633494357,-15.3208442077191,
4.));
#82162=CARTESIAN_POINT('Ctrl Pts',(-72.6050633494357,-15.3208442077191,
8.));
#82163=CARTESIAN_POINT('Ctrl Pts',(-72.6050633494357,-15.3208442077191,
12.));
#82164=CARTESIAN_POINT('',(-72.7986051948032,-15.8307637747259,0.));
#82165=CARTESIAN_POINT('',(-72.6050633494356,-15.3208442077192,0.));
#82166=CARTESIAN_POINT('Ctrl Pts',(-72.7986051948032,-15.8307637747259,
-1.38777878078144E-16));
#82167=CARTESIAN_POINT('Ctrl Pts',(-72.8219545017353,-15.7233907508395,
-1.38777878078146E-16));
#82168=CARTESIAN_POINT('Ctrl Pts',(-72.8084732063058,-15.6083698189725,
-9.70172681189663E-17));
#82169=CARTESIAN_POINT('Ctrl Pts',(-72.761303169957,-15.5092366269869,-2.24569698741506E-17));
#82170=CARTESIAN_POINT('Ctrl Pts',(-72.7259256426954,-15.4348867329977,
3.34632538094614E-17));
#82171=CARTESIAN_POINT('Ctrl Pts',(-72.6715981986666,-15.3694736926919,
1.07833302153744E-16));
#82172=CARTESIAN_POINT('Ctrl Pts',(-72.6050633494357,-15.3208442077191,
1.91487282391008E-16));
#82173=CARTESIAN_POINT('',(-72.6050633494356,-15.3208442077192,12.));
#82174=CARTESIAN_POINT('Ctrl Pts',(-72.6050633494357,-15.3208442077191,
-7.79957864156004E-16));
#82175=CARTESIAN_POINT('Ctrl Pts',(-72.6050633494357,-15.3208442077191,
4.));
#82176=CARTESIAN_POINT('Ctrl Pts',(-72.6050633494357,-15.3208442077191,
8.));
#82177=CARTESIAN_POINT('Ctrl Pts',(-72.6050633494357,-15.3208442077191,
12.));
#82178=CARTESIAN_POINT('',(-72.7986051948032,-15.8307637747259,12.));
#82179=CARTESIAN_POINT('Ctrl Pts',(-72.6050633494357,-15.3208442077191,
12.));
#82180=CARTESIAN_POINT('Ctrl Pts',(-72.6715981986666,-15.3694736926919,
12.));
#82181=CARTESIAN_POINT('Ctrl Pts',(-72.7259256426954,-15.4348867329977,
12.));
#82182=CARTESIAN_POINT('Ctrl Pts',(-72.761303169957,-15.5092366269869,12.));
#82183=CARTESIAN_POINT('Ctrl Pts',(-72.8084732063058,-15.6083698189725,
12.));
#82184=CARTESIAN_POINT('Ctrl Pts',(-72.8219545017353,-15.7233907508395,
12.));
#82185=CARTESIAN_POINT('Ctrl Pts',(-72.7986051948032,-15.8307637747259,
12.));
#82186=CARTESIAN_POINT('Ctrl Pts',(-72.7986051948032,-15.8307637747259,
12.));
#82187=CARTESIAN_POINT('Ctrl Pts',(-72.7986051948032,-15.8307637747259,
8.));
#82188=CARTESIAN_POINT('Ctrl Pts',(-72.7986051948032,-15.8307637747259,
4.));
#82189=CARTESIAN_POINT('Ctrl Pts',(-72.7986051948032,-15.8307637747259,
-1.11022302462516E-15));
#82190=CARTESIAN_POINT('Ctrl Pts',(-68.7831490561748,-12.9953224629497,
0.));
#82191=CARTESIAN_POINT('Ctrl Pts',(-68.7831490561748,-12.9953224629497,
12.));
#82192=CARTESIAN_POINT('Ctrl Pts',(-68.7866525680193,-12.9969981460277,
0.));
#82193=CARTESIAN_POINT('Ctrl Pts',(-68.7866525680193,-12.9969981460277,
12.));
#82194=CARTESIAN_POINT('Ctrl Pts',(-68.7936635625545,-13.0003537683054,
0.));
#82195=CARTESIAN_POINT('Ctrl Pts',(-68.7936635625545,-13.0003537683054,
12.));
#82196=CARTESIAN_POINT('Ctrl Pts',(-68.804191966902,-13.0053999700875,0.));
#82197=CARTESIAN_POINT('Ctrl Pts',(-68.804191966902,-13.0053999700875,12.));
#82198=CARTESIAN_POINT('Ctrl Pts',(-68.8182536653656,-13.0121537768945,
0.));
#82199=CARTESIAN_POINT('Ctrl Pts',(-68.8182536653656,-13.0121537768945,
12.));
#82200=CARTESIAN_POINT('Ctrl Pts',(-68.8358704887468,-13.0206386039691,
0.));
#82201=CARTESIAN_POINT('Ctrl Pts',(-68.8358704887468,-13.0206386039691,
12.));
#82202=CARTESIAN_POINT('Ctrl Pts',(-68.8535269726793,-13.0291660060107,
0.));
#82203=CARTESIAN_POINT('Ctrl Pts',(-68.8535269726793,-13.0291660060107,
12.));
#82204=CARTESIAN_POINT('Ctrl Pts',(-68.8712230321906,-13.0377359881875,
0.));
#82205=CARTESIAN_POINT('Ctrl Pts',(-68.8712230321906,-13.0377359881875,
12.));
#82206=CARTESIAN_POINT('Ctrl Pts',(-68.8889585151585,-13.0463485518206,
0.));
#82207=CARTESIAN_POINT('Ctrl Pts',(-68.8889585151585,-13.0463485518206,
12.));
#82208=CARTESIAN_POINT('Ctrl Pts',(-68.9067332040985,-13.0550036938813,
0.));
#82209=CARTESIAN_POINT('Ctrl Pts',(-68.9067332040985,-13.0550036938813,
12.));
#82210=CARTESIAN_POINT('Ctrl Pts',(-68.9245468449945,-13.0637014089029,
0.));
#82211=CARTESIAN_POINT('Ctrl Pts',(-68.9245468449945,-13.0637014089029,
12.));
#82212=CARTESIAN_POINT('Ctrl Pts',(-68.9423991694492,-13.072441690283,0.));
#82213=CARTESIAN_POINT('Ctrl Pts',(-68.9423991694492,-13.072441690283,12.));
#82214=CARTESIAN_POINT('Ctrl Pts',(-68.9602899187573,-13.0812245317807,
0.));
#82215=CARTESIAN_POINT('Ctrl Pts',(-68.9602899187573,-13.0812245317807,
12.));
#82216=CARTESIAN_POINT('Ctrl Pts',(-68.9782188692581,-13.090049929053,0.));
#82217=CARTESIAN_POINT('Ctrl Pts',(-68.9782188692581,-13.090049929053,12.));
#82218=CARTESIAN_POINT('Ctrl Pts',(-68.9961858241519,-13.0989178791833,
0.));
#82219=CARTESIAN_POINT('Ctrl Pts',(-68.9961858241519,-13.0989178791833,
12.));
#82220=CARTESIAN_POINT('Ctrl Pts',(-69.0141906015113,-13.1078283799722,
0.));
#82221=CARTESIAN_POINT('Ctrl Pts',(-69.0141906015113,-13.1078283799722,
12.));
#82222=CARTESIAN_POINT('Ctrl Pts',(-69.0322330243348,-13.1167814293497,
0.));
#82223=CARTESIAN_POINT('Ctrl Pts',(-69.0322330243348,-13.1167814293497,
12.));
#82224=CARTESIAN_POINT('Ctrl Pts',(-69.0503129081817,-13.1257770246385,
0.));
#82225=CARTESIAN_POINT('Ctrl Pts',(-69.0503129081817,-13.1257770246385,
12.));
#82226=CARTESIAN_POINT('Ctrl Pts',(-69.0684300549477,-13.1348151621834,
0.));
#82227=CARTESIAN_POINT('Ctrl Pts',(-69.0684300549477,-13.1348151621834,
12.));
#82228=CARTESIAN_POINT('Ctrl Pts',(-69.0865842593102,-13.1438958377404,
0.));
#82229=CARTESIAN_POINT('Ctrl Pts',(-69.0865842593102,-13.1438958377404,
12.));
#82230=CARTESIAN_POINT('Ctrl Pts',(-69.1047753127643,-13.1530190467183,
0.));
#82231=CARTESIAN_POINT('Ctrl Pts',(-69.1047753127643,-13.1530190467183,
12.));
#82232=CARTESIAN_POINT('Ctrl Pts',(-69.1230030082573,-13.1621847844528,
0.));
#82233=CARTESIAN_POINT('Ctrl Pts',(-69.1230030082573,-13.1621847844528,
12.));
#82234=CARTESIAN_POINT('Ctrl Pts',(-69.1412671454564,-13.1713930465132,
0.));
#82235=CARTESIAN_POINT('Ctrl Pts',(-69.1412671454564,-13.1713930465132,
12.));
#82236=CARTESIAN_POINT('Ctrl Pts',(-69.1595675305245,-13.1806438286934,
0.));
#82237=CARTESIAN_POINT('Ctrl Pts',(-69.1595675305245,-13.1806438286934,
12.));
#82238=CARTESIAN_POINT('Ctrl Pts',(-69.1779039735996,-13.1899371268683,
0.));
#82239=CARTESIAN_POINT('Ctrl Pts',(-69.1779039735996,-13.1899371268683,
12.));
#82240=CARTESIAN_POINT('Ctrl Pts',(-69.1962762870527,-13.1992729368928,
0.));
#82241=CARTESIAN_POINT('Ctrl Pts',(-69.1962762870527,-13.1992729368928,
12.));
#82242=CARTESIAN_POINT('Ctrl Pts',(-69.2146842833537,-13.2086512544735,
0.));
#82243=CARTESIAN_POINT('Ctrl Pts',(-69.2146842833537,-13.2086512544735,
12.));
#82244=CARTESIAN_POINT('Ctrl Pts',(-69.2331277732861,-13.2180720750594,
0.));
#82245=CARTESIAN_POINT('Ctrl Pts',(-69.2331277732861,-13.2180720750594,
12.));
#82246=CARTESIAN_POINT('Ctrl Pts',(-69.2516065668844,-13.2275353939051,
0.));
#82247=CARTESIAN_POINT('Ctrl Pts',(-69.2516065668844,-13.2275353939051,
12.));
#82248=CARTESIAN_POINT('Ctrl Pts',(-69.2701204742449,-13.237041206122,0.));
#82249=CARTESIAN_POINT('Ctrl Pts',(-69.2701204742449,-13.237041206122,12.));
#82250=CARTESIAN_POINT('Ctrl Pts',(-69.2886693063182,-13.2465895067262,
0.));
#82251=CARTESIAN_POINT('Ctrl Pts',(-69.2886693063182,-13.2465895067262,
12.));
#82252=CARTESIAN_POINT('Ctrl Pts',(-69.3072528758518,-13.2561802906896,
0.));
#82253=CARTESIAN_POINT('Ctrl Pts',(-69.3072528758518,-13.2561802906896,
12.));
#82254=CARTESIAN_POINT('Ctrl Pts',(-69.3258709977382,-13.265813552961,0.));
#82255=CARTESIAN_POINT('Ctrl Pts',(-69.3258709977382,-13.265813552961,12.));
#82256=CARTESIAN_POINT('Ctrl Pts',(-69.3445234885065,-13.2754892884433,
0.));
#82257=CARTESIAN_POINT('Ctrl Pts',(-69.3445234885065,-13.2754892884433,
12.));
#82258=CARTESIAN_POINT('Ctrl Pts',(-69.3632101660066,-13.2852074919765,
0.));
#82259=CARTESIAN_POINT('Ctrl Pts',(-69.3632101660066,-13.2852074919765,
12.));
#82260=CARTESIAN_POINT('Ctrl Pts',(-69.3819308490422,-13.2949681583167,
0.));
#82261=CARTESIAN_POINT('Ctrl Pts',(-69.3819308490422,-13.2949681583167,
12.));
#82262=CARTESIAN_POINT('Ctrl Pts',(-69.4006853569511,-13.3047712821051,
0.));
#82263=CARTESIAN_POINT('Ctrl Pts',(-69.4006853569511,-13.3047712821051,
12.));
#82264=CARTESIAN_POINT('Ctrl Pts',(-69.4194735096265,-13.3146168578743,
0.));
#82265=CARTESIAN_POINT('Ctrl Pts',(-69.4194735096265,-13.3146168578743,
12.));
#82266=CARTESIAN_POINT('Ctrl Pts',(-69.4382951276998,-13.3245048800643,
0.));
#82267=CARTESIAN_POINT('Ctrl Pts',(-69.4382951276998,-13.3245048800643,
12.));
#82268=CARTESIAN_POINT('Ctrl Pts',(-69.4571500326673,-13.3344353430313,
0.));
#82269=CARTESIAN_POINT('Ctrl Pts',(-69.4571500326673,-13.3344353430313,
12.));
#82270=CARTESIAN_POINT('Ctrl Pts',(-69.4760380470365,-13.3444082410543,
0.));
#82271=CARTESIAN_POINT('Ctrl Pts',(-69.4760380470365,-13.3444082410543,
12.));
#82272=CARTESIAN_POINT('Ctrl Pts',(-69.4949589944606,-13.3544235683393,
0.));
#82273=CARTESIAN_POINT('Ctrl Pts',(-69.4949589944606,-13.3544235683393,
12.));
#82274=CARTESIAN_POINT('Ctrl Pts',(-69.5139126996675,-13.3644813190219,
0.));
#82275=CARTESIAN_POINT('Ctrl Pts',(-69.5139126996675,-13.3644813190219,
12.));
#82276=CARTESIAN_POINT('Ctrl Pts',(-69.5328989883885,-13.3745814871664,
0.));
#82277=CARTESIAN_POINT('Ctrl Pts',(-69.5328989883885,-13.3745814871664,
12.));
#82278=CARTESIAN_POINT('Ctrl Pts',(-69.5519176872862,-13.3847240667627,
0.));
#82279=CARTESIAN_POINT('Ctrl Pts',(-69.5519176872862,-13.3847240667627,
12.));
#82280=CARTESIAN_POINT('Ctrl Pts',(-69.5709686238724,-13.3949090517177,
0.));
#82281=CARTESIAN_POINT('Ctrl Pts',(-69.5709686238724,-13.3949090517177,
12.));
#82282=CARTESIAN_POINT('Ctrl Pts',(-69.5900516264553,-13.40513643585,0.));
#82283=CARTESIAN_POINT('Ctrl Pts',(-69.5900516264553,-13.40513643585,12.));
#82284=CARTESIAN_POINT('Ctrl Pts',(-69.6091665241765,-13.4154062129002,
0.));
#82285=CARTESIAN_POINT('Ctrl Pts',(-69.6091665241765,-13.4154062129002,
12.));
#82286=CARTESIAN_POINT('Ctrl Pts',(-69.6283131470273,-13.4257183765341,
0.));
#82287=CARTESIAN_POINT('Ctrl Pts',(-69.6283131470273,-13.4257183765341,
12.));
#82288=CARTESIAN_POINT('Ctrl Pts',(-69.6474913258675,-13.4360729203442,
0.));
#82289=CARTESIAN_POINT('Ctrl Pts',(-69.6474913258675,-13.4360729203442,
12.));
#82290=CARTESIAN_POINT('Ctrl Pts',(-69.666700892444,-13.4464698378453,0.));
#82291=CARTESIAN_POINT('Ctrl Pts',(-69.666700892444,-13.4464698378453,12.));
#82292=CARTESIAN_POINT('Ctrl Pts',(-69.6859416793886,-13.456909122476,0.));
#82293=CARTESIAN_POINT('Ctrl Pts',(-69.6859416793886,-13.456909122476,12.));
#82294=CARTESIAN_POINT('Ctrl Pts',(-69.7052135201998,-13.4673907676044,
0.));
#82295=CARTESIAN_POINT('Ctrl Pts',(-69.7052135201998,-13.4673907676044,
12.));
#82296=CARTESIAN_POINT('Ctrl Pts',(-69.724516249225,-13.4779147665285,0.));
#82297=CARTESIAN_POINT('Ctrl Pts',(-69.724516249225,-13.4779147665285,12.));
#82298=CARTESIAN_POINT('Ctrl Pts',(-69.7438497016406,-13.4884811124748,
0.));
#82299=CARTESIAN_POINT('Ctrl Pts',(-69.7438497016406,-13.4884811124748,
12.));
#82300=CARTESIAN_POINT('Ctrl Pts',(-69.7632137134249,-13.4990897985904,
0.));
#82301=CARTESIAN_POINT('Ctrl Pts',(-69.7632137134249,-13.4990897985904,
12.));
#82302=CARTESIAN_POINT('Ctrl Pts',(-69.7826081213576,-13.5097408179479,
0.));
#82303=CARTESIAN_POINT('Ctrl Pts',(-69.7826081213576,-13.5097408179479,
12.));
#82304=CARTESIAN_POINT('Ctrl Pts',(-69.8020327630205,-13.5204341635507,
0.));
#82305=CARTESIAN_POINT('Ctrl Pts',(-69.8020327630205,-13.5204341635507,
12.));
#82306=CARTESIAN_POINT('Ctrl Pts',(-69.8214874767944,-13.5311698283339,
0.));
#82307=CARTESIAN_POINT('Ctrl Pts',(-69.8214874767944,-13.5311698283339,
12.));
#82308=CARTESIAN_POINT('Ctrl Pts',(-69.840972101856,-13.5419478051625,0.));
#82309=CARTESIAN_POINT('Ctrl Pts',(-69.840972101856,-13.5419478051625,12.));
#82310=CARTESIAN_POINT('Ctrl Pts',(-69.8604864781706,-13.5527680868255,
0.));
#82311=CARTESIAN_POINT('Ctrl Pts',(-69.8604864781706,-13.5527680868255,
12.));
#82312=CARTESIAN_POINT('Ctrl Pts',(-69.8800304464882,-13.5636306660421,
0.));
#82313=CARTESIAN_POINT('Ctrl Pts',(-69.8800304464882,-13.5636306660421,
12.));
#82314=CARTESIAN_POINT('Ctrl Pts',(-69.8996038483361,-13.5745355354656,
0.));
#82315=CARTESIAN_POINT('Ctrl Pts',(-69.8996038483361,-13.5745355354656,
12.));
#82316=CARTESIAN_POINT('Ctrl Pts',(-69.9192065260108,-13.5854826876834,
0.));
#82317=CARTESIAN_POINT('Ctrl Pts',(-69.9192065260108,-13.5854826876834,
12.));
#82318=CARTESIAN_POINT('Ctrl Pts',(-69.9388383225648,-13.5964721152135,
0.));
#82319=CARTESIAN_POINT('Ctrl Pts',(-69.9388383225648,-13.5964721152135,
12.));
#82320=CARTESIAN_POINT('Ctrl Pts',(-69.9584990817974,-13.6075038104998,
0.));
#82321=CARTESIAN_POINT('Ctrl Pts',(-69.9584990817974,-13.6075038104998,
12.));
#82322=CARTESIAN_POINT('Ctrl Pts',(-69.9781886482527,-13.6185777659198,
0.));
#82323=CARTESIAN_POINT('Ctrl Pts',(-69.9781886482527,-13.6185777659198,
12.));
#82324=CARTESIAN_POINT('Ctrl Pts',(-69.9979068672153,-13.6296939737865,
0.));
#82325=CARTESIAN_POINT('Ctrl Pts',(-69.9979068672153,-13.6296939737865,
12.));
#82326=CARTESIAN_POINT('Ctrl Pts',(-70.0176535847049,-13.6408524263496,
0.));
#82327=CARTESIAN_POINT('Ctrl Pts',(-70.0176535847049,-13.6408524263496,
12.));
#82328=CARTESIAN_POINT('Ctrl Pts',(-70.0374286474677,-13.6520531157907,
0.));
#82329=CARTESIAN_POINT('Ctrl Pts',(-70.0374286474677,-13.6520531157907,
12.));
#82330=CARTESIAN_POINT('Ctrl Pts',(-70.0572319029676,-13.6632960342196,
0.));
#82331=CARTESIAN_POINT('Ctrl Pts',(-70.0572319029676,-13.6632960342196,
12.));
#82332=CARTESIAN_POINT('Ctrl Pts',(-70.0770631993856,-13.6745811736829,
0.));
#82333=CARTESIAN_POINT('Ctrl Pts',(-70.0770631993856,-13.6745811736829,
12.));
#82334=CARTESIAN_POINT('Ctrl Pts',(-70.0969223856136,-13.6859085261653,
0.));
#82335=CARTESIAN_POINT('Ctrl Pts',(-70.0969223856136,-13.6859085261653,
12.));
#82336=CARTESIAN_POINT('Ctrl Pts',(-70.1168093112486,-13.6972780835897,
0.));
#82337=CARTESIAN_POINT('Ctrl Pts',(-70.1168093112486,-13.6972780835897,
12.));
#82338=CARTESIAN_POINT('Ctrl Pts',(-70.1367238265825,-13.7086898378121,
0.));
#82339=CARTESIAN_POINT('Ctrl Pts',(-70.1367238265825,-13.7086898378121,
12.));
#82340=CARTESIAN_POINT('Ctrl Pts',(-70.156665782595,-13.7201437806199,0.));
#82341=CARTESIAN_POINT('Ctrl Pts',(-70.156665782595,-13.7201437806199,12.));
#82342=CARTESIAN_POINT('Ctrl Pts',(-70.1766350309518,-13.7316399037392,
0.));
#82343=CARTESIAN_POINT('Ctrl Pts',(-70.1766350309518,-13.7316399037392,
12.));
#82344=CARTESIAN_POINT('Ctrl Pts',(-70.1966314239995,-13.7431781988364,
0.));
#82345=CARTESIAN_POINT('Ctrl Pts',(-70.1966314239995,-13.7431781988364,
12.));
#82346=CARTESIAN_POINT('Ctrl Pts',(-70.2166548147604,-13.754758657518,0.));
#82347=CARTESIAN_POINT('Ctrl Pts',(-70.2166548147604,-13.754758657518,12.));
#82348=CARTESIAN_POINT('Ctrl Pts',(-70.2367050569215,-13.7663812713243,
0.));
#82349=CARTESIAN_POINT('Ctrl Pts',(-70.2367050569215,-13.7663812713243,
12.));
#82350=CARTESIAN_POINT('Ctrl Pts',(-70.2567820048303,-13.7780460317294,
0.));
#82351=CARTESIAN_POINT('Ctrl Pts',(-70.2567820048303,-13.7780460317294,
12.));
#82352=CARTESIAN_POINT('Ctrl Pts',(-70.2768855134947,-13.7897529301491,
0.));
#82353=CARTESIAN_POINT('Ctrl Pts',(-70.2768855134947,-13.7897529301491,
12.));
#82354=CARTESIAN_POINT('Ctrl Pts',(-70.2970154385774,-13.8015019579414,
0.));
#82355=CARTESIAN_POINT('Ctrl Pts',(-70.2970154385774,-13.8015019579414,
12.));
#82356=CARTESIAN_POINT('Ctrl Pts',(-70.3171716363897,-13.8132931064063,
0.));
#82357=CARTESIAN_POINT('Ctrl Pts',(-70.3171716363897,-13.8132931064063,
12.));
#82358=CARTESIAN_POINT('Ctrl Pts',(-70.3373539638809,-13.825126366779,0.));
#82359=CARTESIAN_POINT('Ctrl Pts',(-70.3373539638809,-13.825126366779,12.));
#82360=CARTESIAN_POINT('Ctrl Pts',(-70.3575622786335,-13.8370017302309,
0.));
#82361=CARTESIAN_POINT('Ctrl Pts',(-70.3575622786335,-13.8370017302309,
12.));
#82362=CARTESIAN_POINT('Ctrl Pts',(-70.3777964388632,-13.8489191878767,
0.));
#82363=CARTESIAN_POINT('Ctrl Pts',(-70.3777964388632,-13.8489191878767,
12.));
#82364=CARTESIAN_POINT('Ctrl Pts',(-70.3980563034133,-13.8608787307751,
0.));
#82365=CARTESIAN_POINT('Ctrl Pts',(-70.3980563034133,-13.8608787307751,
12.));
#82366=CARTESIAN_POINT('Ctrl Pts',(-70.4183417317499,-13.8728803499287,
0.));
#82367=CARTESIAN_POINT('Ctrl Pts',(-70.4183417317499,-13.8728803499287,
12.));
#82368=CARTESIAN_POINT('Ctrl Pts',(-70.4386525839521,-13.8849240362763,
0.));
#82369=CARTESIAN_POINT('Ctrl Pts',(-70.4386525839521,-13.8849240362763,
12.));
#82370=CARTESIAN_POINT('Ctrl Pts',(-70.4589887207073,-13.8970097806953,
0.));
#82371=CARTESIAN_POINT('Ctrl Pts',(-70.4589887207073,-13.8970097806953,
12.));
#82372=CARTESIAN_POINT('Ctrl Pts',(-70.4793500033124,-13.9091375740088,
0.));
#82373=CARTESIAN_POINT('Ctrl Pts',(-70.4793500033124,-13.9091375740088,
12.));
#82374=CARTESIAN_POINT('Ctrl Pts',(-70.4997362936673,-13.9213074069852,
0.));
#82375=CARTESIAN_POINT('Ctrl Pts',(-70.4997362936673,-13.9213074069852,
12.));
#82376=CARTESIAN_POINT('Ctrl Pts',(-70.520147454271,-13.9335192703388,0.));
#82377=CARTESIAN_POINT('Ctrl Pts',(-70.520147454271,-13.9335192703388,12.));
#82378=CARTESIAN_POINT('Ctrl Pts',(-70.5405833482112,-13.9457731547215,
0.));
#82379=CARTESIAN_POINT('Ctrl Pts',(-70.5405833482112,-13.9457731547215,
12.));
#82380=CARTESIAN_POINT('Ctrl Pts',(-70.5610438391612,-13.958069050726,0.));
#82381=CARTESIAN_POINT('Ctrl Pts',(-70.5610438391612,-13.958069050726,12.));
#82382=CARTESIAN_POINT('Ctrl Pts',(-70.5815287913784,-13.9704069488917,
0.));
#82383=CARTESIAN_POINT('Ctrl Pts',(-70.5815287913784,-13.9704069488917,
12.));
#82384=CARTESIAN_POINT('Ctrl Pts',(-70.6020380697004,-13.9827868397057,
0.));
#82385=CARTESIAN_POINT('Ctrl Pts',(-70.6020380697004,-13.9827868397057,
12.));
#82386=CARTESIAN_POINT('Ctrl Pts',(-70.6225715395394,-13.9952087136018,
0.));
#82387=CARTESIAN_POINT('Ctrl Pts',(-70.6225715395394,-13.9952087136018,
12.));
#82388=CARTESIAN_POINT('Ctrl Pts',(-70.6431290668745,-14.0076725609536,
0.));
#82389=CARTESIAN_POINT('Ctrl Pts',(-70.6431290668745,-14.0076725609536,
12.));
#82390=CARTESIAN_POINT('Ctrl Pts',(-70.6637105182484,-14.0201783720769,
0.));
#82391=CARTESIAN_POINT('Ctrl Pts',(-70.6637105182484,-14.0201783720769,
12.));
#82392=CARTESIAN_POINT('Ctrl Pts',(-70.6843157607668,-14.0327261372362,
0.));
#82393=CARTESIAN_POINT('Ctrl Pts',(-70.6843157607668,-14.0327261372362,
12.));
#82394=CARTESIAN_POINT('Ctrl Pts',(-70.7049446620928,-14.0453158466451,
0.));
#82395=CARTESIAN_POINT('Ctrl Pts',(-70.7049446620928,-14.0453158466451,
12.));
#82396=CARTESIAN_POINT('Ctrl Pts',(-70.7255970904436,-14.0579474904657,
0.));
#82397=CARTESIAN_POINT('Ctrl Pts',(-70.7255970904436,-14.0579474904657,
12.));
#82398=CARTESIAN_POINT('Ctrl Pts',(-70.7462729145807,-14.0706210588016,
0.));
#82399=CARTESIAN_POINT('Ctrl Pts',(-70.7462729145807,-14.0706210588016,
12.));
#82400=CARTESIAN_POINT('Ctrl Pts',(-70.7669720038077,-14.0833365416996,
0.));
#82401=CARTESIAN_POINT('Ctrl Pts',(-70.7669720038077,-14.0833365416996,
12.));
#82402=CARTESIAN_POINT('Ctrl Pts',(-70.7876942279697,-14.0960939291569,
0.));
#82403=CARTESIAN_POINT('Ctrl Pts',(-70.7876942279697,-14.0960939291569,
12.));
#82404=CARTESIAN_POINT('Ctrl Pts',(-70.8084394574493,-14.1088932111214,
0.));
#82405=CARTESIAN_POINT('Ctrl Pts',(-70.8084394574493,-14.1088932111214,
12.));
#82406=CARTESIAN_POINT('Ctrl Pts',(-70.8292075631621,-14.1217343774913,
0.));
#82407=CARTESIAN_POINT('Ctrl Pts',(-70.8292075631621,-14.1217343774913,
12.));
#82408=CARTESIAN_POINT('Ctrl Pts',(-70.8499984165489,-14.1346174181078,
0.));
#82409=CARTESIAN_POINT('Ctrl Pts',(-70.8499984165489,-14.1346174181078,
12.));
#82410=CARTESIAN_POINT('Ctrl Pts',(-70.8708118895715,-14.1475423227568,
0.));
#82411=CARTESIAN_POINT('Ctrl Pts',(-70.8708118895715,-14.1475423227568,
12.));
#82412=CARTESIAN_POINT('Ctrl Pts',(-70.8916478547132,-14.1605090811754,
0.));
#82413=CARTESIAN_POINT('Ctrl Pts',(-70.8916478547132,-14.1605090811754,
12.));
#82414=CARTESIAN_POINT('Ctrl Pts',(-70.9125061849745,-14.1735176830533,
0.));
#82415=CARTESIAN_POINT('Ctrl Pts',(-70.9125061849745,-14.1735176830533,
12.));
#82416=CARTESIAN_POINT('Ctrl Pts',(-70.9333867538704,-14.186568118032,0.));
#82417=CARTESIAN_POINT('Ctrl Pts',(-70.9333867538704,-14.186568118032,12.));
#82418=CARTESIAN_POINT('Ctrl Pts',(-70.9542894354216,-14.1996603756982,
0.));
#82419=CARTESIAN_POINT('Ctrl Pts',(-70.9542894354216,-14.1996603756982,
12.));
#82420=CARTESIAN_POINT('Ctrl Pts',(-70.9752141041518,-14.2127944455838,
0.));
#82421=CARTESIAN_POINT('Ctrl Pts',(-70.9752141041518,-14.2127944455838,
12.));
#82422=CARTESIAN_POINT('Ctrl Pts',(-70.9961606350861,-14.2259703171737,
0.));
#82423=CARTESIAN_POINT('Ctrl Pts',(-70.9961606350861,-14.2259703171737,
12.));
#82424=CARTESIAN_POINT('Ctrl Pts',(-71.0171289037488,-14.2391879799061,
0.));
#82425=CARTESIAN_POINT('Ctrl Pts',(-71.0171289037488,-14.2391879799061,
12.));
#82426=CARTESIAN_POINT('Ctrl Pts',(-71.0381187861588,-14.2524474231732,
0.));
#82427=CARTESIAN_POINT('Ctrl Pts',(-71.0381187861588,-14.2524474231732,
12.));
#82428=CARTESIAN_POINT('Ctrl Pts',(-71.0591301588231,-14.2657486363139,
0.));
#82429=CARTESIAN_POINT('Ctrl Pts',(-71.0591301588231,-14.2657486363139,
12.));
#82430=CARTESIAN_POINT('Ctrl Pts',(-71.0801628987332,-14.2790916086133,
0.));
#82431=CARTESIAN_POINT('Ctrl Pts',(-71.0801628987332,-14.2790916086133,
12.));
#82432=CARTESIAN_POINT('Ctrl Pts',(-71.1012168833643,-14.2924763293105,
0.));
#82433=CARTESIAN_POINT('Ctrl Pts',(-71.1012168833643,-14.2924763293105,
12.));
#82434=CARTESIAN_POINT('Ctrl Pts',(-71.1222919906727,-14.3059027875994,
0.));
#82435=CARTESIAN_POINT('Ctrl Pts',(-71.1222919906727,-14.3059027875994,
12.));
#82436=CARTESIAN_POINT('Ctrl Pts',(-71.1433880990929,-14.3193709726294,
0.));
#82437=CARTESIAN_POINT('Ctrl Pts',(-71.1433880990929,-14.3193709726294,
12.));
#82438=CARTESIAN_POINT('Ctrl Pts',(-71.1645050875308,-14.3328808734989,
0.));
#82439=CARTESIAN_POINT('Ctrl Pts',(-71.1645050875308,-14.3328808734989,
12.));
#82440=CARTESIAN_POINT('Ctrl Pts',(-71.1856428353593,-14.3464324792533,
0.));
#82441=CARTESIAN_POINT('Ctrl Pts',(-71.1856428353593,-14.3464324792533,
12.));
#82442=CARTESIAN_POINT('Ctrl Pts',(-71.2068012224174,-14.3600257788924,
0.));
#82443=CARTESIAN_POINT('Ctrl Pts',(-71.2068012224174,-14.3600257788924,
12.));
#82444=CARTESIAN_POINT('Ctrl Pts',(-71.2279801290084,-14.3736607613722,
0.));
#82445=CARTESIAN_POINT('Ctrl Pts',(-71.2279801290084,-14.3736607613722,
12.));
#82446=CARTESIAN_POINT('Ctrl Pts',(-71.2491794358958,-14.3873374156056,
0.));
#82447=CARTESIAN_POINT('Ctrl Pts',(-71.2491794358958,-14.3873374156056,
12.));
#82448=CARTESIAN_POINT('Ctrl Pts',(-71.2703990242988,-14.401055730457,0.));
#82449=CARTESIAN_POINT('Ctrl Pts',(-71.2703990242988,-14.401055730457,12.));
#82450=CARTESIAN_POINT('Ctrl Pts',(-71.2916387758861,-14.4148156947384,
0.));
#82451=CARTESIAN_POINT('Ctrl Pts',(-71.2916387758861,-14.4148156947384,
12.));
#82452=CARTESIAN_POINT('Ctrl Pts',(-71.312898572777,-14.4286172972166,0.));
#82453=CARTESIAN_POINT('Ctrl Pts',(-71.312898572777,-14.4286172972166,12.));
#82454=CARTESIAN_POINT('Ctrl Pts',(-71.3341782975386,-14.4424605266165,
0.));
#82455=CARTESIAN_POINT('Ctrl Pts',(-71.3341782975386,-14.4424605266165,
12.));
#82456=CARTESIAN_POINT('Ctrl Pts',(-71.3554778331835,-14.4563453716204,
0.));
#82457=CARTESIAN_POINT('Ctrl Pts',(-71.3554778331835,-14.4563453716204,
12.));
#82458=CARTESIAN_POINT('Ctrl Pts',(-71.376797063165,-14.4702718208651,0.));
#82459=CARTESIAN_POINT('Ctrl Pts',(-71.376797063165,-14.4702718208651,12.));
#82460=CARTESIAN_POINT('Ctrl Pts',(-71.3981358713723,-14.4842398629355,
0.));
#82461=CARTESIAN_POINT('Ctrl Pts',(-71.3981358713723,-14.4842398629355,
12.));
#82462=CARTESIAN_POINT('Ctrl Pts',(-71.4194941421292,-14.4982494863718,
0.));
#82463=CARTESIAN_POINT('Ctrl Pts',(-71.4194941421292,-14.4982494863718,
12.));
#82464=CARTESIAN_POINT('Ctrl Pts',(-71.4408717601923,-14.5123006796728,
0.));
#82465=CARTESIAN_POINT('Ctrl Pts',(-71.4408717601923,-14.5123006796728,
12.));
#82466=CARTESIAN_POINT('Ctrl Pts',(-71.4622686107475,-14.5263934312969,
0.));
#82467=CARTESIAN_POINT('Ctrl Pts',(-71.4622686107475,-14.5263934312969,
12.));
#82468=CARTESIAN_POINT('Ctrl Pts',(-71.4836845794048,-14.540527729659,0.));
#82469=CARTESIAN_POINT('Ctrl Pts',(-71.4836845794048,-14.540527729659,12.));
#82470=CARTESIAN_POINT('Ctrl Pts',(-71.5051195521909,-14.5547035631233,
0.));
#82471=CARTESIAN_POINT('Ctrl Pts',(-71.5051195521909,-14.5547035631233,
12.));
#82472=CARTESIAN_POINT('Ctrl Pts',(-71.5265734155498,-14.5689209200091,
0.));
#82473=CARTESIAN_POINT('Ctrl Pts',(-71.5265734155498,-14.5689209200091,
12.));
#82474=CARTESIAN_POINT('Ctrl Pts',(-71.5480460563447,-14.5831797885952,
0.));
#82475=CARTESIAN_POINT('Ctrl Pts',(-71.5480460563447,-14.5831797885952,
12.));
#82476=CARTESIAN_POINT('Ctrl Pts',(-71.5695373618562,-14.597480157121,0.));
#82477=CARTESIAN_POINT('Ctrl Pts',(-71.5695373618562,-14.597480157121,12.));
#82478=CARTESIAN_POINT('Ctrl Pts',(-71.5910472197813,-14.6118220137849,
0.));
#82479=CARTESIAN_POINT('Ctrl Pts',(-71.5910472197813,-14.6118220137849,
12.));
#82480=CARTESIAN_POINT('Ctrl Pts',(-71.612575518229,-14.626205346737,0.));
#82481=CARTESIAN_POINT('Ctrl Pts',(-71.612575518229,-14.626205346737,12.));
#82482=CARTESIAN_POINT('Ctrl Pts',(-71.6341221457168,-14.6406301440814,
0.));
#82483=CARTESIAN_POINT('Ctrl Pts',(-71.6341221457168,-14.6406301440814,
12.));
#82484=CARTESIAN_POINT('Ctrl Pts',(-71.6556869911662,-14.6550963938829,
0.));
#82485=CARTESIAN_POINT('Ctrl Pts',(-71.6556869911662,-14.6550963938829,
12.));
#82486=CARTESIAN_POINT('Ctrl Pts',(-71.6772699438963,-14.6696040841678,
0.));
#82487=CARTESIAN_POINT('Ctrl Pts',(-71.6772699438963,-14.6696040841678,
12.));
#82488=CARTESIAN_POINT('Ctrl Pts',(-71.6988708936172,-14.6841532029232,
0.));
#82489=CARTESIAN_POINT('Ctrl Pts',(-71.6988708936172,-14.6841532029232,
12.));
#82490=CARTESIAN_POINT('Ctrl Pts',(-71.7204897304194,-14.69874373809,0.));
#82491=CARTESIAN_POINT('Ctrl Pts',(-71.7204897304194,-14.69874373809,12.));
#82492=CARTESIAN_POINT('Ctrl Pts',(-71.7421263447719,-14.7133756775625,
0.));
#82493=CARTESIAN_POINT('Ctrl Pts',(-71.7421263447719,-14.7133756775625,
12.));
#82494=CARTESIAN_POINT('Ctrl Pts',(-71.7637806275328,-14.7280490091957,
0.));
#82495=CARTESIAN_POINT('Ctrl Pts',(-71.7637806275328,-14.7280490091957,
12.));
#82496=CARTESIAN_POINT('Ctrl Pts',(-71.7854524699569,-14.7427637208072,
0.));
#82497=CARTESIAN_POINT('Ctrl Pts',(-71.7854524699569,-14.7427637208072,
12.));
#82498=CARTESIAN_POINT('Ctrl Pts',(-71.8071417637017,-14.7575198001776,
0.));
#82499=CARTESIAN_POINT('Ctrl Pts',(-71.8071417637017,-14.7575198001776,
12.));
#82500=CARTESIAN_POINT('Ctrl Pts',(-71.8288484008333,-14.7723172350451,
0.));
#82501=CARTESIAN_POINT('Ctrl Pts',(-71.8288484008333,-14.7723172350451,
12.));
#82502=CARTESIAN_POINT('Ctrl Pts',(-71.8505722738272,-14.7871560131016,
0.));
#82503=CARTESIAN_POINT('Ctrl Pts',(-71.8505722738272,-14.7871560131016,
12.));
#82504=CARTESIAN_POINT('Ctrl Pts',(-71.8723132755446,-14.8020361219998,
0.));
#82505=CARTESIAN_POINT('Ctrl Pts',(-71.8723132755446,-14.8020361219998,
12.));
#82506=CARTESIAN_POINT('Ctrl Pts',(-71.8940712992109,-14.8169575493557,
0.));
#82507=CARTESIAN_POINT('Ctrl Pts',(-71.8940712992109,-14.8169575493557,
12.));
#82508=CARTESIAN_POINT('Ctrl Pts',(-71.9158462383914,-14.8319202827482,
0.));
#82509=CARTESIAN_POINT('Ctrl Pts',(-71.9158462383914,-14.8319202827482,
12.));
#82510=CARTESIAN_POINT('Ctrl Pts',(-71.9376379869678,-14.8469243097162,
0.));
#82511=CARTESIAN_POINT('Ctrl Pts',(-71.9376379869678,-14.8469243097162,
12.));
#82512=CARTESIAN_POINT('Ctrl Pts',(-71.9594464391078,-14.8619696177506,
0.));
#82513=CARTESIAN_POINT('Ctrl Pts',(-71.9594464391078,-14.8619696177506,
12.));
#82514=CARTESIAN_POINT('Ctrl Pts',(-71.9812714893102,-14.8770561943014,
0.));
#82515=CARTESIAN_POINT('Ctrl Pts',(-71.9812714893102,-14.8770561943014,
12.));
#82516=CARTESIAN_POINT('Ctrl Pts',(-72.0031130324529,-14.8921840267832,
0.));
#82517=CARTESIAN_POINT('Ctrl Pts',(-72.0031130324529,-14.8921840267832,
12.));
#82518=CARTESIAN_POINT('Ctrl Pts',(-72.0249709638422,-14.9073531025764,
0.));
#82519=CARTESIAN_POINT('Ctrl Pts',(-72.0249709638422,-14.9073531025764,
12.));
#82520=CARTESIAN_POINT('Ctrl Pts',(-72.0468451792505,-14.9225634090268,
0.));
#82521=CARTESIAN_POINT('Ctrl Pts',(-72.0468451792505,-14.9225634090268,
12.));
#82522=CARTESIAN_POINT('Ctrl Pts',(-72.0687355749806,-14.9378149334388,
0.));
#82523=CARTESIAN_POINT('Ctrl Pts',(-72.0687355749806,-14.9378149334388,
12.));
#82524=CARTESIAN_POINT('Ctrl Pts',(-72.0906420478076,-14.9531076630767,
0.));
#82525=CARTESIAN_POINT('Ctrl Pts',(-72.0906420478076,-14.9531076630767,
12.));
#82526=CARTESIAN_POINT('Ctrl Pts',(-72.112564494854,-14.9684415851698,0.));
#82527=CARTESIAN_POINT('Ctrl Pts',(-72.112564494854,-14.9684415851698,12.));
#82528=CARTESIAN_POINT('Ctrl Pts',(-72.1345028134777,-14.9838166869107,
0.));
#82529=CARTESIAN_POINT('Ctrl Pts',(-72.1345028134777,-14.9838166869107,
12.));
#82530=CARTESIAN_POINT('Ctrl Pts',(-72.1564569011669,-14.9992329554537,
0.));
#82531=CARTESIAN_POINT('Ctrl Pts',(-72.1564569011669,-14.9992329554537,
12.));
#82532=CARTESIAN_POINT('Ctrl Pts',(-72.1784266553953,-15.0146903779062,
0.));
#82533=CARTESIAN_POINT('Ctrl Pts',(-72.1784266553953,-15.0146903779062,
12.));
#82534=CARTESIAN_POINT('Ctrl Pts',(-72.2004119736115,-15.0301889413257,
0.));
#82535=CARTESIAN_POINT('Ctrl Pts',(-72.2004119736115,-15.0301889413257,
12.));
#82536=CARTESIAN_POINT('Ctrl Pts',(-72.2224127535415,-15.0457286327331,
0.));
#82537=CARTESIAN_POINT('Ctrl Pts',(-72.2224127535415,-15.0457286327331,
12.));
#82538=CARTESIAN_POINT('Ctrl Pts',(-72.2444288934262,-15.0613094391189,
0.));
#82539=CARTESIAN_POINT('Ctrl Pts',(-72.2444288934262,-15.0613094391189,
12.));
#82540=CARTESIAN_POINT('Ctrl Pts',(-72.2664602922852,-15.0769313474476,
0.));
#82541=CARTESIAN_POINT('Ctrl Pts',(-72.2664602922852,-15.0769313474476,
12.));
#82542=CARTESIAN_POINT('Ctrl Pts',(-72.2885068501628,-15.0925943446589,
0.));
#82543=CARTESIAN_POINT('Ctrl Pts',(-72.2885068501628,-15.0925943446589,
12.));
#82544=CARTESIAN_POINT('Ctrl Pts',(-72.3105684683944,-15.1082984176649,
0.));
#82545=CARTESIAN_POINT('Ctrl Pts',(-72.3105684683944,-15.1082984176649,
12.));
#82546=CARTESIAN_POINT('Ctrl Pts',(-72.3326450490177,-15.124043553347,0.));
#82547=CARTESIAN_POINT('Ctrl Pts',(-72.3326450490177,-15.124043553347,12.));
#82548=CARTESIAN_POINT('Ctrl Pts',(-72.3547364941969,-15.1398297385506,
0.));
#82549=CARTESIAN_POINT('Ctrl Pts',(-72.3547364941969,-15.1398297385506,
12.));
#82550=CARTESIAN_POINT('Ctrl Pts',(-72.376842705589,-15.1556569600744,0.));
#82551=CARTESIAN_POINT('Ctrl Pts',(-72.376842705589,-15.1556569600744,12.));
#82552=CARTESIAN_POINT('Ctrl Pts',(-72.3989635838492,-15.1715252046606,
0.));
#82553=CARTESIAN_POINT('Ctrl Pts',(-72.3989635838492,-15.1715252046606,
12.));
#82554=CARTESIAN_POINT('Ctrl Pts',(-72.421099027786,-15.1874344589725,0.));
#82555=CARTESIAN_POINT('Ctrl Pts',(-72.421099027786,-15.1874344589725,12.));
#82556=CARTESIAN_POINT('Ctrl Pts',(-72.4432489350471,-15.2033847096091,
0.));
#82557=CARTESIAN_POINT('Ctrl Pts',(-72.4432489350471,-15.2033847096091,
12.));
#82558=CARTESIAN_POINT('Ctrl Pts',(-72.4654132036428,-15.2193759431372,
0.));
#82559=CARTESIAN_POINT('Ctrl Pts',(-72.4654132036428,-15.2193759431372,
12.));
#82560=CARTESIAN_POINT('Ctrl Pts',(-72.4875917332761,-15.235408146116,0.));
#82561=CARTESIAN_POINT('Ctrl Pts',(-72.4875917332761,-15.235408146116,12.));
#82562=CARTESIAN_POINT('Ctrl Pts',(-72.5097844266075,-15.2514813051172,
0.));
#82563=CARTESIAN_POINT('Ctrl Pts',(-72.5097844266075,-15.2514813051172,
12.));
#82564=CARTESIAN_POINT('Ctrl Pts',(-72.5319911908917,-15.2675954067479,
0.));
#82565=CARTESIAN_POINT('Ctrl Pts',(-72.5319911908917,-15.2675954067479,
12.));
#82566=CARTESIAN_POINT('Ctrl Pts',(-72.5542119383642,-15.2837504376535,
0.));
#82567=CARTESIAN_POINT('Ctrl Pts',(-72.5542119383642,-15.2837504376535,
12.));
#82568=CARTESIAN_POINT('Ctrl Pts',(-72.5764465826224,-15.299946384466,0.));
#82569=CARTESIAN_POINT('Ctrl Pts',(-72.5764465826224,-15.299946384466,12.));
#82570=CARTESIAN_POINT('Ctrl Pts',(-72.5986950357677,-15.3161832337594,
0.));
#82571=CARTESIAN_POINT('Ctrl Pts',(-72.5986950357677,-15.3161832337594,
12.));
#82572=CARTESIAN_POINT('Ctrl Pts',(-72.6209572051042,-15.3324609719955,
0.));
#82573=CARTESIAN_POINT('Ctrl Pts',(-72.6209572051042,-15.3324609719955,
12.));
#82574=CARTESIAN_POINT('Ctrl Pts',(-72.6432329903553,-15.3487795854745,
0.));
#82575=CARTESIAN_POINT('Ctrl Pts',(-72.6432329903553,-15.3487795854745,
12.));
#82576=CARTESIAN_POINT('Ctrl Pts',(-72.6655222797801,-15.3651390602665,
0.));
#82577=CARTESIAN_POINT('Ctrl Pts',(-72.6655222797801,-15.3651390602665,
12.));
#82578=CARTESIAN_POINT('Ctrl Pts',(-72.687824955772,-15.3815393822736,0.));
#82579=CARTESIAN_POINT('Ctrl Pts',(-72.687824955772,-15.3815393822736,12.));
#82580=CARTESIAN_POINT('Ctrl Pts',(-72.7101409017716,-15.3979805373174,
0.));
#82581=CARTESIAN_POINT('Ctrl Pts',(-72.7101409017716,-15.3979805373174,
12.));
#82582=CARTESIAN_POINT('Ctrl Pts',(-72.7324700089712,-15.4144625111944,
0.));
#82583=CARTESIAN_POINT('Ctrl Pts',(-72.7324700089712,-15.4144625111944,
12.));
#82584=CARTESIAN_POINT('Ctrl Pts',(-72.7548121825342,-15.4309852897844,
0.));
#82585=CARTESIAN_POINT('Ctrl Pts',(-72.7548121825342,-15.4309852897844,
12.));
#82586=CARTESIAN_POINT('Ctrl Pts',(-72.777167349421,-15.4475488590243,0.));
#82587=CARTESIAN_POINT('Ctrl Pts',(-72.777167349421,-15.4475488590243,12.));
#82588=CARTESIAN_POINT('Ctrl Pts',(-72.7995354603795,-15.4641532053281,
0.));
#82589=CARTESIAN_POINT('Ctrl Pts',(-72.7995354603795,-15.4641532053281,
12.));
#82590=CARTESIAN_POINT('Ctrl Pts',(-72.8219164843279,-15.4807983165804,
0.));
#82591=CARTESIAN_POINT('Ctrl Pts',(-72.8219164843279,-15.4807983165804,
12.));
#82592=CARTESIAN_POINT('Ctrl Pts',(-72.8398316205897,-15.494147009702,0.));
#82593=CARTESIAN_POINT('Ctrl Pts',(-72.8398316205897,-15.494147009702,12.));
#82594=CARTESIAN_POINT('Ctrl Pts',(-72.8532737731759,-15.5041768663998,
0.));
#82595=CARTESIAN_POINT('Ctrl Pts',(-72.8532737731759,-15.5041768663998,
12.));
#82596=CARTESIAN_POINT('Ctrl Pts',(-72.8622377860824,-15.5108715869141,
0.));
#82597=CARTESIAN_POINT('Ctrl Pts',(-72.8622377860824,-15.5108715869141,
12.));
#82598=CARTESIAN_POINT('Ctrl Pts',(-72.8667204369977,-15.5142209845168,
0.));
#82599=CARTESIAN_POINT('Ctrl Pts',(-72.8667204369977,-15.5142209845168,
12.));
#82600=CARTESIAN_POINT('',(-68.7831490561748,-12.9953224629497,0.));
#82601=CARTESIAN_POINT('Ctrl Pts',(-68.7831490561748,-12.9953224629497,
0.));
#82602=CARTESIAN_POINT('Ctrl Pts',(-68.7866525680193,-12.9969981460277,
0.));
#82603=CARTESIAN_POINT('Ctrl Pts',(-68.7936635625545,-13.0003537683054,
0.));
#82604=CARTESIAN_POINT('Ctrl Pts',(-68.804191966902,-13.0053999700875,0.));
#82605=CARTESIAN_POINT('Ctrl Pts',(-68.8182536653656,-13.0121537768945,
0.));
#82606=CARTESIAN_POINT('Ctrl Pts',(-68.8358704887468,-13.0206386039691,
0.));
#82607=CARTESIAN_POINT('Ctrl Pts',(-68.8535269726793,-13.0291660060107,
0.));
#82608=CARTESIAN_POINT('Ctrl Pts',(-68.8712230321906,-13.0377359881875,
0.));
#82609=CARTESIAN_POINT('Ctrl Pts',(-68.8889585151585,-13.0463485518206,
0.));
#82610=CARTESIAN_POINT('Ctrl Pts',(-68.9067332040985,-13.0550036938813,
0.));
#82611=CARTESIAN_POINT('Ctrl Pts',(-68.9245468449945,-13.0637014089029,
0.));
#82612=CARTESIAN_POINT('Ctrl Pts',(-68.9423991694492,-13.072441690283,0.));
#82613=CARTESIAN_POINT('Ctrl Pts',(-68.9602899187573,-13.0812245317807,
0.));
#82614=CARTESIAN_POINT('Ctrl Pts',(-68.9782188692581,-13.090049929053,0.));
#82615=CARTESIAN_POINT('Ctrl Pts',(-68.9961858241519,-13.0989178791833,
0.));
#82616=CARTESIAN_POINT('Ctrl Pts',(-69.0141906015113,-13.1078283799722,
0.));
#82617=CARTESIAN_POINT('Ctrl Pts',(-69.0322330243348,-13.1167814293497,
0.));
#82618=CARTESIAN_POINT('Ctrl Pts',(-69.0503129081817,-13.1257770246385,
0.));
#82619=CARTESIAN_POINT('Ctrl Pts',(-69.0684300549477,-13.1348151621834,
0.));
#82620=CARTESIAN_POINT('Ctrl Pts',(-69.0865842593102,-13.1438958377404,
0.));
#82621=CARTESIAN_POINT('Ctrl Pts',(-69.1047753127643,-13.1530190467183,
0.));
#82622=CARTESIAN_POINT('Ctrl Pts',(-69.1230030082573,-13.1621847844528,
0.));
#82623=CARTESIAN_POINT('Ctrl Pts',(-69.1412671454564,-13.1713930465132,
0.));
#82624=CARTESIAN_POINT('Ctrl Pts',(-69.1595675305245,-13.1806438286934,
0.));
#82625=CARTESIAN_POINT('Ctrl Pts',(-69.1779039735996,-13.1899371268683,
0.));
#82626=CARTESIAN_POINT('Ctrl Pts',(-69.1962762870527,-13.1992729368928,
0.));
#82627=CARTESIAN_POINT('Ctrl Pts',(-69.2146842833537,-13.2086512544735,
0.));
#82628=CARTESIAN_POINT('Ctrl Pts',(-69.2331277732861,-13.2180720750594,
0.));
#82629=CARTESIAN_POINT('Ctrl Pts',(-69.2516065668844,-13.2275353939051,
0.));
#82630=CARTESIAN_POINT('Ctrl Pts',(-69.2701204742449,-13.237041206122,0.));
#82631=CARTESIAN_POINT('Ctrl Pts',(-69.2886693063182,-13.2465895067262,
0.));
#82632=CARTESIAN_POINT('Ctrl Pts',(-69.3072528758518,-13.2561802906896,
0.));
#82633=CARTESIAN_POINT('Ctrl Pts',(-69.3258709977382,-13.265813552961,0.));
#82634=CARTESIAN_POINT('Ctrl Pts',(-69.3445234885065,-13.2754892884433,
0.));
#82635=CARTESIAN_POINT('Ctrl Pts',(-69.3632101660066,-13.2852074919765,
0.));
#82636=CARTESIAN_POINT('Ctrl Pts',(-69.3819308490422,-13.2949681583167,
0.));
#82637=CARTESIAN_POINT('Ctrl Pts',(-69.4006853569511,-13.3047712821051,
0.));
#82638=CARTESIAN_POINT('Ctrl Pts',(-69.4194735096265,-13.3146168578743,
0.));
#82639=CARTESIAN_POINT('Ctrl Pts',(-69.4382951276998,-13.3245048800643,
0.));
#82640=CARTESIAN_POINT('Ctrl Pts',(-69.4571500326673,-13.3344353430313,
0.));
#82641=CARTESIAN_POINT('Ctrl Pts',(-69.4760380470365,-13.3444082410543,
0.));
#82642=CARTESIAN_POINT('Ctrl Pts',(-69.4949589944606,-13.3544235683393,
0.));
#82643=CARTESIAN_POINT('Ctrl Pts',(-69.5139126996675,-13.3644813190219,
0.));
#82644=CARTESIAN_POINT('Ctrl Pts',(-69.5328989883885,-13.3745814871664,
0.));
#82645=CARTESIAN_POINT('Ctrl Pts',(-69.5519176872862,-13.3847240667627,
0.));
#82646=CARTESIAN_POINT('Ctrl Pts',(-69.5709686238724,-13.3949090517177,
0.));
#82647=CARTESIAN_POINT('Ctrl Pts',(-69.5900516264553,-13.40513643585,0.));
#82648=CARTESIAN_POINT('Ctrl Pts',(-69.6091665241765,-13.4154062129002,
0.));
#82649=CARTESIAN_POINT('Ctrl Pts',(-69.6283131470273,-13.4257183765341,
0.));
#82650=CARTESIAN_POINT('Ctrl Pts',(-69.6474913258675,-13.4360729203442,
0.));
#82651=CARTESIAN_POINT('Ctrl Pts',(-69.666700892444,-13.4464698378453,0.));
#82652=CARTESIAN_POINT('Ctrl Pts',(-69.6859416793886,-13.456909122476,0.));
#82653=CARTESIAN_POINT('Ctrl Pts',(-69.7052135201998,-13.4673907676044,
0.));
#82654=CARTESIAN_POINT('Ctrl Pts',(-69.724516249225,-13.4779147665285,0.));
#82655=CARTESIAN_POINT('Ctrl Pts',(-69.7438497016406,-13.4884811124748,
0.));
#82656=CARTESIAN_POINT('Ctrl Pts',(-69.7632137134249,-13.4990897985904,
0.));
#82657=CARTESIAN_POINT('Ctrl Pts',(-69.7826081213576,-13.5097408179479,
0.));
#82658=CARTESIAN_POINT('Ctrl Pts',(-69.8020327630205,-13.5204341635507,
0.));
#82659=CARTESIAN_POINT('Ctrl Pts',(-69.8214874767944,-13.5311698283339,
0.));
#82660=CARTESIAN_POINT('Ctrl Pts',(-69.840972101856,-13.5419478051625,0.));
#82661=CARTESIAN_POINT('Ctrl Pts',(-69.8604864781706,-13.5527680868255,
0.));
#82662=CARTESIAN_POINT('Ctrl Pts',(-69.8800304464882,-13.5636306660421,
0.));
#82663=CARTESIAN_POINT('Ctrl Pts',(-69.8996038483361,-13.5745355354656,
0.));
#82664=CARTESIAN_POINT('Ctrl Pts',(-69.9192065260108,-13.5854826876834,
0.));
#82665=CARTESIAN_POINT('Ctrl Pts',(-69.9388383225648,-13.5964721152135,
0.));
#82666=CARTESIAN_POINT('Ctrl Pts',(-69.9584990817974,-13.6075038104998,
0.));
#82667=CARTESIAN_POINT('Ctrl Pts',(-69.9781886482527,-13.6185777659198,
0.));
#82668=CARTESIAN_POINT('Ctrl Pts',(-69.9979068672153,-13.6296939737865,
0.));
#82669=CARTESIAN_POINT('Ctrl Pts',(-70.0176535847049,-13.6408524263496,
0.));
#82670=CARTESIAN_POINT('Ctrl Pts',(-70.0374286474677,-13.6520531157907,
0.));
#82671=CARTESIAN_POINT('Ctrl Pts',(-70.0572319029676,-13.6632960342196,
0.));
#82672=CARTESIAN_POINT('Ctrl Pts',(-70.0770631993856,-13.6745811736829,
0.));
#82673=CARTESIAN_POINT('Ctrl Pts',(-70.0969223856136,-13.6859085261653,
0.));
#82674=CARTESIAN_POINT('Ctrl Pts',(-70.1168093112486,-13.6972780835897,
0.));
#82675=CARTESIAN_POINT('Ctrl Pts',(-70.1367238265825,-13.7086898378121,
0.));
#82676=CARTESIAN_POINT('Ctrl Pts',(-70.156665782595,-13.7201437806199,0.));
#82677=CARTESIAN_POINT('Ctrl Pts',(-70.1766350309518,-13.7316399037392,
0.));
#82678=CARTESIAN_POINT('Ctrl Pts',(-70.1966314239995,-13.7431781988364,
0.));
#82679=CARTESIAN_POINT('Ctrl Pts',(-70.2166548147604,-13.754758657518,0.));
#82680=CARTESIAN_POINT('Ctrl Pts',(-70.2367050569215,-13.7663812713243,
0.));
#82681=CARTESIAN_POINT('Ctrl Pts',(-70.2567820048303,-13.7780460317294,
0.));
#82682=CARTESIAN_POINT('Ctrl Pts',(-70.2768855134947,-13.7897529301491,
0.));
#82683=CARTESIAN_POINT('Ctrl Pts',(-70.2970154385774,-13.8015019579414,
0.));
#82684=CARTESIAN_POINT('Ctrl Pts',(-70.3171716363897,-13.8132931064063,
0.));
#82685=CARTESIAN_POINT('Ctrl Pts',(-70.3373539638809,-13.825126366779,0.));
#82686=CARTESIAN_POINT('Ctrl Pts',(-70.3575622786335,-13.8370017302309,
0.));
#82687=CARTESIAN_POINT('Ctrl Pts',(-70.3777964388632,-13.8489191878767,
0.));
#82688=CARTESIAN_POINT('Ctrl Pts',(-70.3980563034133,-13.8608787307751,
0.));
#82689=CARTESIAN_POINT('Ctrl Pts',(-70.4183417317499,-13.8728803499287,
0.));
#82690=CARTESIAN_POINT('Ctrl Pts',(-70.4386525839521,-13.8849240362763,
0.));
#82691=CARTESIAN_POINT('Ctrl Pts',(-70.4589887207073,-13.8970097806953,
0.));
#82692=CARTESIAN_POINT('Ctrl Pts',(-70.4793500033124,-13.9091375740088,
0.));
#82693=CARTESIAN_POINT('Ctrl Pts',(-70.4997362936673,-13.9213074069852,
0.));
#82694=CARTESIAN_POINT('Ctrl Pts',(-70.520147454271,-13.9335192703388,0.));
#82695=CARTESIAN_POINT('Ctrl Pts',(-70.5405833482112,-13.9457731547215,
0.));
#82696=CARTESIAN_POINT('Ctrl Pts',(-70.5610438391612,-13.958069050726,0.));
#82697=CARTESIAN_POINT('Ctrl Pts',(-70.5815287913784,-13.9704069488917,
0.));
#82698=CARTESIAN_POINT('Ctrl Pts',(-70.6020380697004,-13.9827868397057,
0.));
#82699=CARTESIAN_POINT('Ctrl Pts',(-70.6225715395394,-13.9952087136018,
0.));
#82700=CARTESIAN_POINT('Ctrl Pts',(-70.6431290668745,-14.0076725609536,
0.));
#82701=CARTESIAN_POINT('Ctrl Pts',(-70.6637105182484,-14.0201783720769,
0.));
#82702=CARTESIAN_POINT('Ctrl Pts',(-70.6843157607668,-14.0327261372362,
0.));
#82703=CARTESIAN_POINT('Ctrl Pts',(-70.7049446620928,-14.0453158466451,
0.));
#82704=CARTESIAN_POINT('Ctrl Pts',(-70.7255970904436,-14.0579474904657,
0.));
#82705=CARTESIAN_POINT('Ctrl Pts',(-70.7462729145807,-14.0706210588016,
0.));
#82706=CARTESIAN_POINT('Ctrl Pts',(-70.7669720038077,-14.0833365416996,
0.));
#82707=CARTESIAN_POINT('Ctrl Pts',(-70.7876942279697,-14.0960939291569,
0.));
#82708=CARTESIAN_POINT('Ctrl Pts',(-70.8084394574493,-14.1088932111214,
0.));
#82709=CARTESIAN_POINT('Ctrl Pts',(-70.8292075631621,-14.1217343774913,
0.));
#82710=CARTESIAN_POINT('Ctrl Pts',(-70.8499984165489,-14.1346174181078,
0.));
#82711=CARTESIAN_POINT('Ctrl Pts',(-70.8708118895715,-14.1475423227568,
0.));
#82712=CARTESIAN_POINT('Ctrl Pts',(-70.8916478547132,-14.1605090811754,
0.));
#82713=CARTESIAN_POINT('Ctrl Pts',(-70.9125061849745,-14.1735176830533,
0.));
#82714=CARTESIAN_POINT('Ctrl Pts',(-70.9333867538704,-14.186568118032,0.));
#82715=CARTESIAN_POINT('Ctrl Pts',(-70.9542894354216,-14.1996603756982,
0.));
#82716=CARTESIAN_POINT('Ctrl Pts',(-70.9752141041518,-14.2127944455838,
0.));
#82717=CARTESIAN_POINT('Ctrl Pts',(-70.9961606350861,-14.2259703171737,
0.));
#82718=CARTESIAN_POINT('Ctrl Pts',(-71.0171289037488,-14.2391879799061,
0.));
#82719=CARTESIAN_POINT('Ctrl Pts',(-71.0381187861588,-14.2524474231732,
0.));
#82720=CARTESIAN_POINT('Ctrl Pts',(-71.0591301588231,-14.2657486363139,
0.));
#82721=CARTESIAN_POINT('Ctrl Pts',(-71.0801628987332,-14.2790916086133,
0.));
#82722=CARTESIAN_POINT('Ctrl Pts',(-71.1012168833643,-14.2924763293105,
0.));
#82723=CARTESIAN_POINT('Ctrl Pts',(-71.1222919906727,-14.3059027875994,
0.));
#82724=CARTESIAN_POINT('Ctrl Pts',(-71.1433880990929,-14.3193709726294,
0.));
#82725=CARTESIAN_POINT('Ctrl Pts',(-71.1645050875308,-14.3328808734989,
0.));
#82726=CARTESIAN_POINT('Ctrl Pts',(-71.1856428353593,-14.3464324792533,
0.));
#82727=CARTESIAN_POINT('Ctrl Pts',(-71.2068012224174,-14.3600257788924,
0.));
#82728=CARTESIAN_POINT('Ctrl Pts',(-71.2279801290084,-14.3736607613722,
0.));
#82729=CARTESIAN_POINT('Ctrl Pts',(-71.2491794358958,-14.3873374156056,
0.));
#82730=CARTESIAN_POINT('Ctrl Pts',(-71.2703990242988,-14.401055730457,0.));
#82731=CARTESIAN_POINT('Ctrl Pts',(-71.2916387758861,-14.4148156947384,
0.));
#82732=CARTESIAN_POINT('Ctrl Pts',(-71.312898572777,-14.4286172972166,0.));
#82733=CARTESIAN_POINT('Ctrl Pts',(-71.3341782975386,-14.4424605266165,
0.));
#82734=CARTESIAN_POINT('Ctrl Pts',(-71.3554778331835,-14.4563453716204,
0.));
#82735=CARTESIAN_POINT('Ctrl Pts',(-71.376797063165,-14.4702718208651,0.));
#82736=CARTESIAN_POINT('Ctrl Pts',(-71.3981358713723,-14.4842398629355,
0.));
#82737=CARTESIAN_POINT('Ctrl Pts',(-71.4194941421292,-14.4982494863718,
0.));
#82738=CARTESIAN_POINT('Ctrl Pts',(-71.4408717601923,-14.5123006796728,
0.));
#82739=CARTESIAN_POINT('Ctrl Pts',(-71.4622686107475,-14.5263934312969,
0.));
#82740=CARTESIAN_POINT('Ctrl Pts',(-71.4836845794048,-14.540527729659,0.));
#82741=CARTESIAN_POINT('Ctrl Pts',(-71.5051195521909,-14.5547035631233,
0.));
#82742=CARTESIAN_POINT('Ctrl Pts',(-71.5265734155498,-14.5689209200091,
0.));
#82743=CARTESIAN_POINT('Ctrl Pts',(-71.5480460563447,-14.5831797885952,
0.));
#82744=CARTESIAN_POINT('Ctrl Pts',(-71.5695373618562,-14.597480157121,0.));
#82745=CARTESIAN_POINT('Ctrl Pts',(-71.5910472197813,-14.6118220137849,
0.));
#82746=CARTESIAN_POINT('Ctrl Pts',(-71.612575518229,-14.626205346737,0.));
#82747=CARTESIAN_POINT('Ctrl Pts',(-71.6341221457168,-14.6406301440814,
0.));
#82748=CARTESIAN_POINT('Ctrl Pts',(-71.6556869911662,-14.6550963938829,
0.));
#82749=CARTESIAN_POINT('Ctrl Pts',(-71.6772699438963,-14.6696040841678,
0.));
#82750=CARTESIAN_POINT('Ctrl Pts',(-71.6988708936172,-14.6841532029232,
0.));
#82751=CARTESIAN_POINT('Ctrl Pts',(-71.7204897304194,-14.69874373809,0.));
#82752=CARTESIAN_POINT('Ctrl Pts',(-71.7421263447719,-14.7133756775625,
0.));
#82753=CARTESIAN_POINT('Ctrl Pts',(-71.7637806275328,-14.7280490091957,
0.));
#82754=CARTESIAN_POINT('Ctrl Pts',(-71.7854524699569,-14.7427637208072,
0.));
#82755=CARTESIAN_POINT('Ctrl Pts',(-71.8071417637017,-14.7575198001776,
0.));
#82756=CARTESIAN_POINT('Ctrl Pts',(-71.8288484008333,-14.7723172350451,
0.));
#82757=CARTESIAN_POINT('Ctrl Pts',(-71.8505722738272,-14.7871560131016,
0.));
#82758=CARTESIAN_POINT('Ctrl Pts',(-71.8723132755446,-14.8020361219998,
0.));
#82759=CARTESIAN_POINT('Ctrl Pts',(-71.8940712992109,-14.8169575493557,
0.));
#82760=CARTESIAN_POINT('Ctrl Pts',(-71.9158462383914,-14.8319202827482,
0.));
#82761=CARTESIAN_POINT('Ctrl Pts',(-71.9376379869678,-14.8469243097162,
0.));
#82762=CARTESIAN_POINT('Ctrl Pts',(-71.9594464391078,-14.8619696177506,
0.));
#82763=CARTESIAN_POINT('Ctrl Pts',(-71.9812714893102,-14.8770561943014,
0.));
#82764=CARTESIAN_POINT('Ctrl Pts',(-72.0031130324529,-14.8921840267832,
0.));
#82765=CARTESIAN_POINT('Ctrl Pts',(-72.0249709638422,-14.9073531025764,
0.));
#82766=CARTESIAN_POINT('Ctrl Pts',(-72.0468451792505,-14.9225634090268,
0.));
#82767=CARTESIAN_POINT('Ctrl Pts',(-72.0687355749806,-14.9378149334388,
0.));
#82768=CARTESIAN_POINT('Ctrl Pts',(-72.0906420478076,-14.9531076630767,
0.));
#82769=CARTESIAN_POINT('Ctrl Pts',(-72.112564494854,-14.9684415851698,0.));
#82770=CARTESIAN_POINT('Ctrl Pts',(-72.1345028134777,-14.9838166869107,
0.));
#82771=CARTESIAN_POINT('Ctrl Pts',(-72.1564569011669,-14.9992329554537,
0.));
#82772=CARTESIAN_POINT('Ctrl Pts',(-72.1784266553953,-15.0146903779062,
0.));
#82773=CARTESIAN_POINT('Ctrl Pts',(-72.2004119736115,-15.0301889413257,
0.));
#82774=CARTESIAN_POINT('Ctrl Pts',(-72.2224127535415,-15.0457286327331,
0.));
#82775=CARTESIAN_POINT('Ctrl Pts',(-72.2444288934262,-15.0613094391189,
0.));
#82776=CARTESIAN_POINT('Ctrl Pts',(-72.2664602922852,-15.0769313474476,
0.));
#82777=CARTESIAN_POINT('Ctrl Pts',(-72.2885068501628,-15.0925943446589,
0.));
#82778=CARTESIAN_POINT('Ctrl Pts',(-72.3105684683944,-15.1082984176649,
0.));
#82779=CARTESIAN_POINT('Ctrl Pts',(-72.3326450490177,-15.124043553347,0.));
#82780=CARTESIAN_POINT('Ctrl Pts',(-72.3547364941969,-15.1398297385506,
0.));
#82781=CARTESIAN_POINT('Ctrl Pts',(-72.376842705589,-15.1556569600744,0.));
#82782=CARTESIAN_POINT('Ctrl Pts',(-72.3989635838492,-15.1715252046606,
0.));
#82783=CARTESIAN_POINT('Ctrl Pts',(-72.421099027786,-15.1874344589725,0.));
#82784=CARTESIAN_POINT('Ctrl Pts',(-72.4432489350471,-15.2033847096091,
0.));
#82785=CARTESIAN_POINT('Ctrl Pts',(-72.4654132036428,-15.2193759431372,
0.));
#82786=CARTESIAN_POINT('Ctrl Pts',(-72.4875917332761,-15.235408146116,0.));
#82787=CARTESIAN_POINT('Ctrl Pts',(-72.5097844266075,-15.2514813051172,
0.));
#82788=CARTESIAN_POINT('Ctrl Pts',(-72.5319911908917,-15.2675954067479,
0.));
#82789=CARTESIAN_POINT('Ctrl Pts',(-72.5542119383642,-15.2837504376535,
0.));
#82790=CARTESIAN_POINT('Ctrl Pts',(-72.5732713370619,-15.297633502478,0.));
#82791=CARTESIAN_POINT('Ctrl Pts',(-72.5878912620441,-15.308299460354,0.));
#82792=CARTESIAN_POINT('Ctrl Pts',(-72.5980655789638,-15.3157301930684,
0.));
#82793=CARTESIAN_POINT('Ctrl Pts',(-72.6037902604925,-15.3199137230132,
0.));
#82794=CARTESIAN_POINT('Ctrl Pts',(-72.6050633494356,-15.3208442077192,
0.));
#82795=CARTESIAN_POINT('',(-68.7831490561748,-12.9953224629497,12.));
#82796=CARTESIAN_POINT('',(-68.7831490561748,-12.9953224629497,0.));
#82797=CARTESIAN_POINT('Ctrl Pts',(-72.6050633494356,-15.3208442077192,
12.));
#82798=CARTESIAN_POINT('Ctrl Pts',(-72.6037902604925,-15.3199137230132,
12.));
#82799=CARTESIAN_POINT('Ctrl Pts',(-72.5980655789638,-15.3157301930684,
12.));
#82800=CARTESIAN_POINT('Ctrl Pts',(-72.5878912620441,-15.308299460354,12.));
#82801=CARTESIAN_POINT('Ctrl Pts',(-72.5732713370619,-15.297633502478,12.));
#82802=CARTESIAN_POINT('Ctrl Pts',(-72.5542119383642,-15.2837504376535,
12.));
#82803=CARTESIAN_POINT('Ctrl Pts',(-72.5319911908917,-15.2675954067479,
12.));
#82804=CARTESIAN_POINT('Ctrl Pts',(-72.5097844266075,-15.2514813051172,
12.));
#82805=CARTESIAN_POINT('Ctrl Pts',(-72.4875917332761,-15.235408146116,12.));
#82806=CARTESIAN_POINT('Ctrl Pts',(-72.4654132036428,-15.2193759431372,
12.));
#82807=CARTESIAN_POINT('Ctrl Pts',(-72.4432489350471,-15.2033847096091,
12.));
#82808=CARTESIAN_POINT('Ctrl Pts',(-72.421099027786,-15.1874344589725,12.));
#82809=CARTESIAN_POINT('Ctrl Pts',(-72.3989635838492,-15.1715252046606,
12.));
#82810=CARTESIAN_POINT('Ctrl Pts',(-72.376842705589,-15.1556569600744,12.));
#82811=CARTESIAN_POINT('Ctrl Pts',(-72.3547364941969,-15.1398297385506,
12.));
#82812=CARTESIAN_POINT('Ctrl Pts',(-72.3326450490177,-15.124043553347,12.));
#82813=CARTESIAN_POINT('Ctrl Pts',(-72.3105684683944,-15.1082984176649,
12.));
#82814=CARTESIAN_POINT('Ctrl Pts',(-72.2885068501628,-15.0925943446589,
12.));
#82815=CARTESIAN_POINT('Ctrl Pts',(-72.2664602922852,-15.0769313474476,
12.));
#82816=CARTESIAN_POINT('Ctrl Pts',(-72.2444288934262,-15.0613094391189,
12.));
#82817=CARTESIAN_POINT('Ctrl Pts',(-72.2224127535415,-15.0457286327331,
12.));
#82818=CARTESIAN_POINT('Ctrl Pts',(-72.2004119736115,-15.0301889413257,
12.));
#82819=CARTESIAN_POINT('Ctrl Pts',(-72.1784266553953,-15.0146903779062,
12.));
#82820=CARTESIAN_POINT('Ctrl Pts',(-72.1564569011669,-14.9992329554537,
12.));
#82821=CARTESIAN_POINT('Ctrl Pts',(-72.1345028134777,-14.9838166869107,
12.));
#82822=CARTESIAN_POINT('Ctrl Pts',(-72.112564494854,-14.9684415851698,12.));
#82823=CARTESIAN_POINT('Ctrl Pts',(-72.0906420478076,-14.9531076630767,
12.));
#82824=CARTESIAN_POINT('Ctrl Pts',(-72.0687355749806,-14.9378149334388,
12.));
#82825=CARTESIAN_POINT('Ctrl Pts',(-72.0468451792505,-14.9225634090268,
12.));
#82826=CARTESIAN_POINT('Ctrl Pts',(-72.0249709638422,-14.9073531025764,
12.));
#82827=CARTESIAN_POINT('Ctrl Pts',(-72.0031130324529,-14.8921840267832,
12.));
#82828=CARTESIAN_POINT('Ctrl Pts',(-71.9812714893102,-14.8770561943014,
12.));
#82829=CARTESIAN_POINT('Ctrl Pts',(-71.9594464391078,-14.8619696177506,
12.));
#82830=CARTESIAN_POINT('Ctrl Pts',(-71.9376379869678,-14.8469243097162,
12.));
#82831=CARTESIAN_POINT('Ctrl Pts',(-71.9158462383914,-14.8319202827482,
12.));
#82832=CARTESIAN_POINT('Ctrl Pts',(-71.8940712992109,-14.8169575493557,
12.));
#82833=CARTESIAN_POINT('Ctrl Pts',(-71.8723132755446,-14.8020361219998,
12.));
#82834=CARTESIAN_POINT('Ctrl Pts',(-71.8505722738272,-14.7871560131016,
12.));
#82835=CARTESIAN_POINT('Ctrl Pts',(-71.8288484008333,-14.7723172350451,
12.));
#82836=CARTESIAN_POINT('Ctrl Pts',(-71.8071417637017,-14.7575198001776,
12.));
#82837=CARTESIAN_POINT('Ctrl Pts',(-71.7854524699569,-14.7427637208072,
12.));
#82838=CARTESIAN_POINT('Ctrl Pts',(-71.7637806275328,-14.7280490091957,
12.));
#82839=CARTESIAN_POINT('Ctrl Pts',(-71.7421263447719,-14.7133756775625,
12.));
#82840=CARTESIAN_POINT('Ctrl Pts',(-71.7204897304194,-14.69874373809,12.));
#82841=CARTESIAN_POINT('Ctrl Pts',(-71.6988708936172,-14.6841532029232,
12.));
#82842=CARTESIAN_POINT('Ctrl Pts',(-71.6772699438963,-14.6696040841678,
12.));
#82843=CARTESIAN_POINT('Ctrl Pts',(-71.6556869911662,-14.6550963938829,
12.));
#82844=CARTESIAN_POINT('Ctrl Pts',(-71.6341221457168,-14.6406301440814,
12.));
#82845=CARTESIAN_POINT('Ctrl Pts',(-71.612575518229,-14.626205346737,12.));
#82846=CARTESIAN_POINT('Ctrl Pts',(-71.5910472197813,-14.6118220137849,
12.));
#82847=CARTESIAN_POINT('Ctrl Pts',(-71.5695373618562,-14.597480157121,12.));
#82848=CARTESIAN_POINT('Ctrl Pts',(-71.5480460563447,-14.5831797885952,
12.));
#82849=CARTESIAN_POINT('Ctrl Pts',(-71.5265734155498,-14.5689209200091,
12.));
#82850=CARTESIAN_POINT('Ctrl Pts',(-71.5051195521909,-14.5547035631233,
12.));
#82851=CARTESIAN_POINT('Ctrl Pts',(-71.4836845794048,-14.540527729659,12.));
#82852=CARTESIAN_POINT('Ctrl Pts',(-71.4622686107475,-14.5263934312969,
12.));
#82853=CARTESIAN_POINT('Ctrl Pts',(-71.4408717601923,-14.5123006796728,
12.));
#82854=CARTESIAN_POINT('Ctrl Pts',(-71.4194941421292,-14.4982494863718,
12.));
#82855=CARTESIAN_POINT('Ctrl Pts',(-71.3981358713723,-14.4842398629355,
12.));
#82856=CARTESIAN_POINT('Ctrl Pts',(-71.376797063165,-14.4702718208651,12.));
#82857=CARTESIAN_POINT('Ctrl Pts',(-71.3554778331835,-14.4563453716204,
12.));
#82858=CARTESIAN_POINT('Ctrl Pts',(-71.3341782975386,-14.4424605266165,
12.));
#82859=CARTESIAN_POINT('Ctrl Pts',(-71.312898572777,-14.4286172972166,12.));
#82860=CARTESIAN_POINT('Ctrl Pts',(-71.2916387758861,-14.4148156947384,
12.));
#82861=CARTESIAN_POINT('Ctrl Pts',(-71.2703990242988,-14.401055730457,12.));
#82862=CARTESIAN_POINT('Ctrl Pts',(-71.2491794358958,-14.3873374156056,
12.));
#82863=CARTESIAN_POINT('Ctrl Pts',(-71.2279801290084,-14.3736607613722,
12.));
#82864=CARTESIAN_POINT('Ctrl Pts',(-71.2068012224174,-14.3600257788924,
12.));
#82865=CARTESIAN_POINT('Ctrl Pts',(-71.1856428353593,-14.3464324792533,
12.));
#82866=CARTESIAN_POINT('Ctrl Pts',(-71.1645050875308,-14.3328808734989,
12.));
#82867=CARTESIAN_POINT('Ctrl Pts',(-71.1433880990929,-14.3193709726294,
12.));
#82868=CARTESIAN_POINT('Ctrl Pts',(-71.1222919906727,-14.3059027875994,
12.));
#82869=CARTESIAN_POINT('Ctrl Pts',(-71.1012168833643,-14.2924763293105,
12.));
#82870=CARTESIAN_POINT('Ctrl Pts',(-71.0801628987332,-14.2790916086133,
12.));
#82871=CARTESIAN_POINT('Ctrl Pts',(-71.0591301588231,-14.2657486363139,
12.));
#82872=CARTESIAN_POINT('Ctrl Pts',(-71.0381187861588,-14.2524474231732,
12.));
#82873=CARTESIAN_POINT('Ctrl Pts',(-71.0171289037488,-14.2391879799061,
12.));
#82874=CARTESIAN_POINT('Ctrl Pts',(-70.9961606350861,-14.2259703171737,
12.));
#82875=CARTESIAN_POINT('Ctrl Pts',(-70.9752141041518,-14.2127944455838,
12.));
#82876=CARTESIAN_POINT('Ctrl Pts',(-70.9542894354216,-14.1996603756982,
12.));
#82877=CARTESIAN_POINT('Ctrl Pts',(-70.9333867538704,-14.186568118032,12.));
#82878=CARTESIAN_POINT('Ctrl Pts',(-70.9125061849745,-14.1735176830533,
12.));
#82879=CARTESIAN_POINT('Ctrl Pts',(-70.8916478547132,-14.1605090811754,
12.));
#82880=CARTESIAN_POINT('Ctrl Pts',(-70.8708118895715,-14.1475423227568,
12.));
#82881=CARTESIAN_POINT('Ctrl Pts',(-70.8499984165489,-14.1346174181078,
12.));
#82882=CARTESIAN_POINT('Ctrl Pts',(-70.8292075631621,-14.1217343774913,
12.));
#82883=CARTESIAN_POINT('Ctrl Pts',(-70.8084394574493,-14.1088932111214,
12.));
#82884=CARTESIAN_POINT('Ctrl Pts',(-70.7876942279697,-14.0960939291569,
12.));
#82885=CARTESIAN_POINT('Ctrl Pts',(-70.7669720038077,-14.0833365416996,
12.));
#82886=CARTESIAN_POINT('Ctrl Pts',(-70.7462729145807,-14.0706210588016,
12.));
#82887=CARTESIAN_POINT('Ctrl Pts',(-70.7255970904436,-14.0579474904657,
12.));
#82888=CARTESIAN_POINT('Ctrl Pts',(-70.7049446620928,-14.0453158466451,
12.));
#82889=CARTESIAN_POINT('Ctrl Pts',(-70.6843157607668,-14.0327261372362,
12.));
#82890=CARTESIAN_POINT('Ctrl Pts',(-70.6637105182484,-14.0201783720769,
12.));
#82891=CARTESIAN_POINT('Ctrl Pts',(-70.6431290668745,-14.0076725609536,
12.));
#82892=CARTESIAN_POINT('Ctrl Pts',(-70.6225715395394,-13.9952087136018,
12.));
#82893=CARTESIAN_POINT('Ctrl Pts',(-70.6020380697004,-13.9827868397057,
12.));
#82894=CARTESIAN_POINT('Ctrl Pts',(-70.5815287913784,-13.9704069488917,
12.));
#82895=CARTESIAN_POINT('Ctrl Pts',(-70.5610438391612,-13.958069050726,12.));
#82896=CARTESIAN_POINT('Ctrl Pts',(-70.5405833482112,-13.9457731547215,
12.));
#82897=CARTESIAN_POINT('Ctrl Pts',(-70.520147454271,-13.9335192703388,12.));
#82898=CARTESIAN_POINT('Ctrl Pts',(-70.4997362936673,-13.9213074069852,
12.));
#82899=CARTESIAN_POINT('Ctrl Pts',(-70.4793500033124,-13.9091375740088,
12.));
#82900=CARTESIAN_POINT('Ctrl Pts',(-70.4589887207073,-13.8970097806953,
12.));
#82901=CARTESIAN_POINT('Ctrl Pts',(-70.4386525839521,-13.8849240362763,
12.));
#82902=CARTESIAN_POINT('Ctrl Pts',(-70.4183417317499,-13.8728803499287,
12.));
#82903=CARTESIAN_POINT('Ctrl Pts',(-70.3980563034133,-13.8608787307751,
12.));
#82904=CARTESIAN_POINT('Ctrl Pts',(-70.3777964388632,-13.8489191878767,
12.));
#82905=CARTESIAN_POINT('Ctrl Pts',(-70.3575622786335,-13.8370017302309,
12.));
#82906=CARTESIAN_POINT('Ctrl Pts',(-70.3373539638809,-13.825126366779,12.));
#82907=CARTESIAN_POINT('Ctrl Pts',(-70.3171716363897,-13.8132931064063,
12.));
#82908=CARTESIAN_POINT('Ctrl Pts',(-70.2970154385774,-13.8015019579414,
12.));
#82909=CARTESIAN_POINT('Ctrl Pts',(-70.2768855134947,-13.7897529301491,
12.));
#82910=CARTESIAN_POINT('Ctrl Pts',(-70.2567820048303,-13.7780460317294,
12.));
#82911=CARTESIAN_POINT('Ctrl Pts',(-70.2367050569215,-13.7663812713243,
12.));
#82912=CARTESIAN_POINT('Ctrl Pts',(-70.2166548147604,-13.754758657518,12.));
#82913=CARTESIAN_POINT('Ctrl Pts',(-70.1966314239995,-13.7431781988364,
12.));
#82914=CARTESIAN_POINT('Ctrl Pts',(-70.1766350309518,-13.7316399037392,
12.));
#82915=CARTESIAN_POINT('Ctrl Pts',(-70.156665782595,-13.7201437806199,12.));
#82916=CARTESIAN_POINT('Ctrl Pts',(-70.1367238265825,-13.7086898378121,
12.));
#82917=CARTESIAN_POINT('Ctrl Pts',(-70.1168093112486,-13.6972780835897,
12.));
#82918=CARTESIAN_POINT('Ctrl Pts',(-70.0969223856136,-13.6859085261653,
12.));
#82919=CARTESIAN_POINT('Ctrl Pts',(-70.0770631993856,-13.6745811736829,
12.));
#82920=CARTESIAN_POINT('Ctrl Pts',(-70.0572319029676,-13.6632960342196,
12.));
#82921=CARTESIAN_POINT('Ctrl Pts',(-70.0374286474677,-13.6520531157907,
12.));
#82922=CARTESIAN_POINT('Ctrl Pts',(-70.0176535847049,-13.6408524263496,
12.));
#82923=CARTESIAN_POINT('Ctrl Pts',(-69.9979068672153,-13.6296939737865,
12.));
#82924=CARTESIAN_POINT('Ctrl Pts',(-69.9781886482527,-13.6185777659198,
12.));
#82925=CARTESIAN_POINT('Ctrl Pts',(-69.9584990817974,-13.6075038104998,
12.));
#82926=CARTESIAN_POINT('Ctrl Pts',(-69.9388383225648,-13.5964721152135,
12.));
#82927=CARTESIAN_POINT('Ctrl Pts',(-69.9192065260108,-13.5854826876834,
12.));
#82928=CARTESIAN_POINT('Ctrl Pts',(-69.8996038483361,-13.5745355354656,
12.));
#82929=CARTESIAN_POINT('Ctrl Pts',(-69.8800304464882,-13.5636306660421,
12.));
#82930=CARTESIAN_POINT('Ctrl Pts',(-69.8604864781706,-13.5527680868255,
12.));
#82931=CARTESIAN_POINT('Ctrl Pts',(-69.840972101856,-13.5419478051625,12.));
#82932=CARTESIAN_POINT('Ctrl Pts',(-69.8214874767944,-13.5311698283339,
12.));
#82933=CARTESIAN_POINT('Ctrl Pts',(-69.8020327630205,-13.5204341635507,
12.));
#82934=CARTESIAN_POINT('Ctrl Pts',(-69.7826081213576,-13.5097408179479,
12.));
#82935=CARTESIAN_POINT('Ctrl Pts',(-69.7632137134249,-13.4990897985904,
12.));
#82936=CARTESIAN_POINT('Ctrl Pts',(-69.7438497016406,-13.4884811124748,
12.));
#82937=CARTESIAN_POINT('Ctrl Pts',(-69.724516249225,-13.4779147665285,12.));
#82938=CARTESIAN_POINT('Ctrl Pts',(-69.7052135201998,-13.4673907676044,
12.));
#82939=CARTESIAN_POINT('Ctrl Pts',(-69.6859416793886,-13.456909122476,12.));
#82940=CARTESIAN_POINT('Ctrl Pts',(-69.666700892444,-13.4464698378453,12.));
#82941=CARTESIAN_POINT('Ctrl Pts',(-69.6474913258675,-13.4360729203442,
12.));
#82942=CARTESIAN_POINT('Ctrl Pts',(-69.6283131470273,-13.4257183765341,
12.));
#82943=CARTESIAN_POINT('Ctrl Pts',(-69.6091665241765,-13.4154062129002,
12.));
#82944=CARTESIAN_POINT('Ctrl Pts',(-69.5900516264553,-13.40513643585,12.));
#82945=CARTESIAN_POINT('Ctrl Pts',(-69.5709686238724,-13.3949090517177,
12.));
#82946=CARTESIAN_POINT('Ctrl Pts',(-69.5519176872862,-13.3847240667627,
12.));
#82947=CARTESIAN_POINT('Ctrl Pts',(-69.5328989883885,-13.3745814871664,
12.));
#82948=CARTESIAN_POINT('Ctrl Pts',(-69.5139126996675,-13.3644813190219,
12.));
#82949=CARTESIAN_POINT('Ctrl Pts',(-69.4949589944606,-13.3544235683393,
12.));
#82950=CARTESIAN_POINT('Ctrl Pts',(-69.4760380470365,-13.3444082410543,
12.));
#82951=CARTESIAN_POINT('Ctrl Pts',(-69.4571500326673,-13.3344353430313,
12.));
#82952=CARTESIAN_POINT('Ctrl Pts',(-69.4382951276998,-13.3245048800643,
12.));
#82953=CARTESIAN_POINT('Ctrl Pts',(-69.4194735096265,-13.3146168578743,
12.));
#82954=CARTESIAN_POINT('Ctrl Pts',(-69.4006853569511,-13.3047712821051,
12.));
#82955=CARTESIAN_POINT('Ctrl Pts',(-69.3819308490422,-13.2949681583167,
12.));
#82956=CARTESIAN_POINT('Ctrl Pts',(-69.3632101660066,-13.2852074919765,
12.));
#82957=CARTESIAN_POINT('Ctrl Pts',(-69.3445234885065,-13.2754892884433,
12.));
#82958=CARTESIAN_POINT('Ctrl Pts',(-69.3258709977382,-13.265813552961,12.));
#82959=CARTESIAN_POINT('Ctrl Pts',(-69.3072528758518,-13.2561802906896,
12.));
#82960=CARTESIAN_POINT('Ctrl Pts',(-69.2886693063182,-13.2465895067262,
12.));
#82961=CARTESIAN_POINT('Ctrl Pts',(-69.2701204742449,-13.237041206122,12.));
#82962=CARTESIAN_POINT('Ctrl Pts',(-69.2516065668844,-13.2275353939051,
12.));
#82963=CARTESIAN_POINT('Ctrl Pts',(-69.2331277732861,-13.2180720750594,
12.));
#82964=CARTESIAN_POINT('Ctrl Pts',(-69.2146842833537,-13.2086512544735,
12.));
#82965=CARTESIAN_POINT('Ctrl Pts',(-69.1962762870527,-13.1992729368928,
12.));
#82966=CARTESIAN_POINT('Ctrl Pts',(-69.1779039735996,-13.1899371268683,
12.));
#82967=CARTESIAN_POINT('Ctrl Pts',(-69.1595675305245,-13.1806438286934,
12.));
#82968=CARTESIAN_POINT('Ctrl Pts',(-69.1412671454564,-13.1713930465132,
12.));
#82969=CARTESIAN_POINT('Ctrl Pts',(-69.1230030082573,-13.1621847844528,
12.));
#82970=CARTESIAN_POINT('Ctrl Pts',(-69.1047753127643,-13.1530190467183,
12.));
#82971=CARTESIAN_POINT('Ctrl Pts',(-69.0865842593102,-13.1438958377404,
12.));
#82972=CARTESIAN_POINT('Ctrl Pts',(-69.0684300549477,-13.1348151621834,
12.));
#82973=CARTESIAN_POINT('Ctrl Pts',(-69.0503129081817,-13.1257770246385,
12.));
#82974=CARTESIAN_POINT('Ctrl Pts',(-69.0322330243348,-13.1167814293497,
12.));
#82975=CARTESIAN_POINT('Ctrl Pts',(-69.0141906015113,-13.1078283799722,
12.));
#82976=CARTESIAN_POINT('Ctrl Pts',(-68.9961858241519,-13.0989178791833,
12.));
#82977=CARTESIAN_POINT('Ctrl Pts',(-68.9782188692581,-13.090049929053,12.));
#82978=CARTESIAN_POINT('Ctrl Pts',(-68.9602899187573,-13.0812245317807,
12.));
#82979=CARTESIAN_POINT('Ctrl Pts',(-68.9423991694492,-13.072441690283,12.));
#82980=CARTESIAN_POINT('Ctrl Pts',(-68.9245468449945,-13.0637014089029,
12.));
#82981=CARTESIAN_POINT('Ctrl Pts',(-68.9067332040985,-13.0550036938813,
12.));
#82982=CARTESIAN_POINT('Ctrl Pts',(-68.8889585151585,-13.0463485518206,
12.));
#82983=CARTESIAN_POINT('Ctrl Pts',(-68.8712230321906,-13.0377359881875,
12.));
#82984=CARTESIAN_POINT('Ctrl Pts',(-68.8535269726793,-13.0291660060107,
12.));
#82985=CARTESIAN_POINT('Ctrl Pts',(-68.8358704887468,-13.0206386039691,
12.));
#82986=CARTESIAN_POINT('Ctrl Pts',(-68.8182536653656,-13.0121537768945,
12.));
#82987=CARTESIAN_POINT('Ctrl Pts',(-68.804191966902,-13.0053999700875,12.));
#82988=CARTESIAN_POINT('Ctrl Pts',(-68.7936635625545,-13.0003537683054,
12.));
#82989=CARTESIAN_POINT('Ctrl Pts',(-68.7866525680193,-12.9969981460277,
12.));
#82990=CARTESIAN_POINT('Ctrl Pts',(-68.7831490561748,-12.9953224629497,
12.));
#82991=CARTESIAN_POINT('Ctrl Pts',(-72.277402839391,-16.7988252568749,0.));
#82992=CARTESIAN_POINT('Ctrl Pts',(-72.277402839391,-16.7988252568749,4.));
#82993=CARTESIAN_POINT('Ctrl Pts',(-72.2774028393911,-16.7988252568749,
8.));
#82994=CARTESIAN_POINT('Ctrl Pts',(-72.2774028393911,-16.7988252568749,
12.));
#82995=CARTESIAN_POINT('Ctrl Pts',(-72.3852065198821,-16.7775526720895,
0.));
#82996=CARTESIAN_POINT('Ctrl Pts',(-72.3852065198821,-16.7775526720895,
4.));
#82997=CARTESIAN_POINT('Ctrl Pts',(-72.3852065198822,-16.7775526720895,
8.00000000000001));
#82998=CARTESIAN_POINT('Ctrl Pts',(-72.3852065198822,-16.7775526720895,
12.));
#82999=CARTESIAN_POINT('Ctrl Pts',(-72.5605133546287,-16.675864902556,0.));
#83000=CARTESIAN_POINT('Ctrl Pts',(-72.5605133546287,-16.675864902556,4.));
#83001=CARTESIAN_POINT('Ctrl Pts',(-72.5605133546287,-16.675864902556,7.99999999999999));
#83002=CARTESIAN_POINT('Ctrl Pts',(-72.5605133546287,-16.675864902556,12.));
#83003=CARTESIAN_POINT('Ctrl Pts',(-72.650150535446,-16.4988611391809,0.));
#83004=CARTESIAN_POINT('Ctrl Pts',(-72.650150535446,-16.4988611391809,4.));
#83005=CARTESIAN_POINT('Ctrl Pts',(-72.6501505354461,-16.4988611391808,
8.00000000000001));
#83006=CARTESIAN_POINT('Ctrl Pts',(-72.6501505354461,-16.4988611391808,
12.));
#83007=CARTESIAN_POINT('Ctrl Pts',(-72.6683126419583,-16.4184755008062,
0.));
#83008=CARTESIAN_POINT('Ctrl Pts',(-72.6683126419583,-16.4184755008062,
4.));
#83009=CARTESIAN_POINT('Ctrl Pts',(-72.6683126419584,-16.4184755008061,
8.));
#83010=CARTESIAN_POINT('Ctrl Pts',(-72.6683126419584,-16.4184755008061,
12.));
#83011=CARTESIAN_POINT('',(-72.277402839391,-16.7988252568749,0.));
#83012=CARTESIAN_POINT('',(-72.6683126419585,-16.4184755008062,0.));
#83013=CARTESIAN_POINT('Ctrl Pts',(-72.277402839391,-16.7988252568749,2.77555756156289E-16));
#83014=CARTESIAN_POINT('Ctrl Pts',(-72.3852065198821,-16.7775526720895,
2.77555756156289E-16));
#83015=CARTESIAN_POINT('Ctrl Pts',(-72.485381854023,-16.7194453752132,2.77555756156289E-16));
#83016=CARTESIAN_POINT('Ctrl Pts',(-72.5575834236156,-16.636745100756,2.77555756156289E-16));
#83017=CARTESIAN_POINT('Ctrl Pts',(-72.61173460081,-16.574719894913,2.77555756156289E-16));
#83018=CARTESIAN_POINT('Ctrl Pts',(-72.650150535446,-16.4988611391809,2.77555756156289E-16));
#83019=CARTESIAN_POINT('Ctrl Pts',(-72.6683126419583,-16.4184755008062,
2.77555756156289E-16));
#83020=CARTESIAN_POINT('',(-72.6683126419585,-16.4184755008062,12.));
#83021=CARTESIAN_POINT('Ctrl Pts',(-72.6683126419583,-16.4184755008062,
0.));
#83022=CARTESIAN_POINT('Ctrl Pts',(-72.6683126419583,-16.4184755008062,
4.));
#83023=CARTESIAN_POINT('Ctrl Pts',(-72.6683126419584,-16.4184755008061,
8.));
#83024=CARTESIAN_POINT('Ctrl Pts',(-72.6683126419584,-16.4184755008061,
12.));
#83025=CARTESIAN_POINT('',(-72.2774028393911,-16.7988252568749,12.));
#83026=CARTESIAN_POINT('Ctrl Pts',(-72.6683126419584,-16.4184755008061,
12.));
#83027=CARTESIAN_POINT('Ctrl Pts',(-72.6501505354461,-16.4988611391808,
12.));
#83028=CARTESIAN_POINT('Ctrl Pts',(-72.6117346008101,-16.574719894913,12.));
#83029=CARTESIAN_POINT('Ctrl Pts',(-72.5575834236157,-16.6367451007559,
12.));
#83030=CARTESIAN_POINT('Ctrl Pts',(-72.4853818540231,-16.7194453752132,
12.));
#83031=CARTESIAN_POINT('Ctrl Pts',(-72.3852065198822,-16.7775526720895,
12.));
#83032=CARTESIAN_POINT('Ctrl Pts',(-72.2774028393911,-16.7988252568749,
12.));
#83033=CARTESIAN_POINT('Ctrl Pts',(-72.2774028393911,-16.7988252568749,
12.));
#83034=CARTESIAN_POINT('Ctrl Pts',(-72.2774028393911,-16.7988252568749,
8.));
#83035=CARTESIAN_POINT('Ctrl Pts',(-72.277402839391,-16.7988252568749,4.));
#83036=CARTESIAN_POINT('Ctrl Pts',(-72.277402839391,-16.7988252568749,0.));
#83037=CARTESIAN_POINT('Origin',(-3.65936987487134E-10,-8.12279454723525E-11,
0.));
#83038=CARTESIAN_POINT('Origin',(-3.65936987487134E-10,-8.12279454723525E-11,
12.));
#83039=CARTESIAN_POINT('Origin',(-3.65936987487134E-10,-8.12279454723525E-11,
0.));
#83040=CARTESIAN_POINT('Ctrl Pts',(-73.9013264985861,-9.42570643237816,
0.));
#83041=CARTESIAN_POINT('Ctrl Pts',(-73.9013264985861,-9.42570643237816,
4.));
#83042=CARTESIAN_POINT('Ctrl Pts',(-73.9013264985861,-9.42570643237813,
8.));
#83043=CARTESIAN_POINT('Ctrl Pts',(-73.9013264985861,-9.42570643237813,
12.));
#83044=CARTESIAN_POINT('Ctrl Pts',(-73.9152287787081,-9.31670696907602,
0.));
#83045=CARTESIAN_POINT('Ctrl Pts',(-73.9152287787081,-9.31670696907602,
4.));
#83046=CARTESIAN_POINT('Ctrl Pts',(-73.9152287787081,-9.31670696907599,
8.00000000000001));
#83047=CARTESIAN_POINT('Ctrl Pts',(-73.9152287787081,-9.31670696907599,
12.));
#83048=CARTESIAN_POINT('Ctrl Pts',(-73.8741839722667,-9.11824194722532,
0.));
#83049=CARTESIAN_POINT('Ctrl Pts',(-73.8741839722667,-9.11824194722532,
4.));
#83050=CARTESIAN_POINT('Ctrl Pts',(-73.8741839722668,-9.1182419472253,7.99999999999999));
#83051=CARTESIAN_POINT('Ctrl Pts',(-73.8741839722668,-9.1182419472253,12.));
#83052=CARTESIAN_POINT('Ctrl Pts',(-73.7345987226919,-8.97724108745549,
0.));
#83053=CARTESIAN_POINT('Ctrl Pts',(-73.7345987226919,-8.97724108745549,
4.));
#83054=CARTESIAN_POINT('Ctrl Pts',(-73.7345987226919,-8.97724108745545,
8.00000000000001));
#83055=CARTESIAN_POINT('Ctrl Pts',(-73.7345987226919,-8.97724108745545,
12.));
#83056=CARTESIAN_POINT('Ctrl Pts',(-73.6640787197673,-8.93459554655806,
0.));
#83057=CARTESIAN_POINT('Ctrl Pts',(-73.6640787197673,-8.93459554655806,
4.));
#83058=CARTESIAN_POINT('Ctrl Pts',(-73.6640787197673,-8.93459554655801,
8.));
#83059=CARTESIAN_POINT('Ctrl Pts',(-73.6640787197673,-8.93459554655801,
12.));
#83060=CARTESIAN_POINT('',(-73.9013264985861,-9.42570643237816,0.));
#83061=CARTESIAN_POINT('',(-73.6640787197672,-8.93459554655821,0.));
#83062=CARTESIAN_POINT('Ctrl Pts',(-73.9013264985861,-9.42570643237816,
0.));
#83063=CARTESIAN_POINT('Ctrl Pts',(-73.9152287787081,-9.31670696907602,
0.));
#83064=CARTESIAN_POINT('Ctrl Pts',(-73.8917746035988,-9.20329838516133,
0.));
#83065=CARTESIAN_POINT('Ctrl Pts',(-73.8361439572621,-9.10865360927305,
0.));
#83066=CARTESIAN_POINT('Ctrl Pts',(-73.7944209725097,-9.03767002735684,
0.));
#83067=CARTESIAN_POINT('Ctrl Pts',(-73.7345987226919,-8.97724108745549,
0.));
#83068=CARTESIAN_POINT('Ctrl Pts',(-73.6640787197673,-8.93459554655806,
0.));
#83069=CARTESIAN_POINT('',(-73.6640787197672,-8.93459554655823,12.));
#83070=CARTESIAN_POINT('Ctrl Pts',(-73.6640787197673,-8.93459554655806,
0.));
#83071=CARTESIAN_POINT('Ctrl Pts',(-73.6640787197673,-8.93459554655806,
4.));
#83072=CARTESIAN_POINT('Ctrl Pts',(-73.6640787197673,-8.93459554655801,
8.));
#83073=CARTESIAN_POINT('Ctrl Pts',(-73.6640787197673,-8.93459554655801,
12.));
#83074=CARTESIAN_POINT('',(-73.9013264985861,-9.42570643237813,12.));
#83075=CARTESIAN_POINT('Ctrl Pts',(-73.6640787197673,-8.93459554655801,
12.));
#83076=CARTESIAN_POINT('Ctrl Pts',(-73.7345987226919,-8.97724108745545,
12.));
#83077=CARTESIAN_POINT('Ctrl Pts',(-73.7944209725097,-9.03767002735682,
12.));
#83078=CARTESIAN_POINT('Ctrl Pts',(-73.8361439572622,-9.10865360927303,
12.));
#83079=CARTESIAN_POINT('Ctrl Pts',(-73.8917746035988,-9.20329838516131,
12.));
#83080=CARTESIAN_POINT('Ctrl Pts',(-73.9152287787081,-9.31670696907599,
12.));
#83081=CARTESIAN_POINT('Ctrl Pts',(-73.9013264985861,-9.42570643237813,
12.));
#83082=CARTESIAN_POINT('Ctrl Pts',(-73.9013264985861,-9.42570643237813,
12.));
#83083=CARTESIAN_POINT('Ctrl Pts',(-73.9013264985861,-9.42570643237813,
8.));
#83084=CARTESIAN_POINT('Ctrl Pts',(-73.9013264985861,-9.42570643237816,
4.));
#83085=CARTESIAN_POINT('Ctrl Pts',(-73.9013264985861,-9.42570643237816,
0.));
#83086=CARTESIAN_POINT('Ctrl Pts',(-69.6540253893192,-6.95102489306925,
0.));
#83087=CARTESIAN_POINT('Ctrl Pts',(-69.6540253893192,-6.95102489306925,
12.));
#83088=CARTESIAN_POINT('Ctrl Pts',(-69.6576616146467,-6.95238884849025,
0.));
#83089=CARTESIAN_POINT('Ctrl Pts',(-69.6576616146467,-6.95238884849025,
12.));
#83090=CARTESIAN_POINT('Ctrl Pts',(-69.664938391983,-6.95512065317599,0.));
#83091=CARTESIAN_POINT('Ctrl Pts',(-69.664938391983,-6.95512065317599,12.));
#83092=CARTESIAN_POINT('Ctrl Pts',(-69.6758665380378,-6.95923004173591,
0.));
#83093=CARTESIAN_POINT('Ctrl Pts',(-69.6758665380378,-6.95923004173591,
12.));
#83094=CARTESIAN_POINT('Ctrl Pts',(-69.6904633605421,-6.96473259049513,
0.));
#83095=CARTESIAN_POINT('Ctrl Pts',(-69.6904633605421,-6.96473259049513,
12.));
#83096=CARTESIAN_POINT('Ctrl Pts',(-69.7087526479973,-6.97164972291439,
0.));
#83097=CARTESIAN_POINT('Ctrl Pts',(-69.7087526479973,-6.97164972291439,
12.));
#83098=CARTESIAN_POINT('Ctrl Pts',(-69.7270851557366,-6.97860581164527,
0.));
#83099=CARTESIAN_POINT('Ctrl Pts',(-69.7270851557366,-6.97860581164527,
12.));
#83100=CARTESIAN_POINT('Ctrl Pts',(-69.7454607995607,-6.98560086924214,
0.));
#83101=CARTESIAN_POINT('Ctrl Pts',(-69.7454607995607,-6.98560086924214,
12.));
#83102=CARTESIAN_POINT('Ctrl Pts',(-69.7638794280419,-6.9926349102794,0.));
#83103=CARTESIAN_POINT('Ctrl Pts',(-69.7638794280419,-6.9926349102794,12.));
#83104=CARTESIAN_POINT('Ctrl Pts',(-69.782340824259,-6.99970795069476,0.));
#83105=CARTESIAN_POINT('Ctrl Pts',(-69.782340824259,-6.99970795069476,12.));
#83106=CARTESIAN_POINT('Ctrl Pts',(-69.8008447346863,-7.0068200071815,0.));
#83107=CARTESIAN_POINT('Ctrl Pts',(-69.8008447346863,-7.0068200071815,12.));
#83108=CARTESIAN_POINT('Ctrl Pts',(-69.8193908913722,-7.01397109655454,
0.));
#83109=CARTESIAN_POINT('Ctrl Pts',(-69.8193908913722,-7.01397109655454,
12.));
#83110=CARTESIAN_POINT('Ctrl Pts',(-69.8379790360518,-7.02116123514451,
0.));
#83111=CARTESIAN_POINT('Ctrl Pts',(-69.8379790360518,-7.02116123514451,
12.));
#83112=CARTESIAN_POINT('Ctrl Pts',(-69.8566089455375,-7.02839043811812,
0.));
#83113=CARTESIAN_POINT('Ctrl Pts',(-69.8566089455375,-7.02839043811812,
12.));
#83114=CARTESIAN_POINT('Ctrl Pts',(-69.8752804235238,-7.03565871972221,
0.));
#83115=CARTESIAN_POINT('Ctrl Pts',(-69.8752804235238,-7.03565871972221,
12.));
#83116=CARTESIAN_POINT('Ctrl Pts',(-69.8939932885841,-7.04296609362165,
0.));
#83117=CARTESIAN_POINT('Ctrl Pts',(-69.8939932885841,-7.04296609362165,
12.));
#83118=CARTESIAN_POINT('Ctrl Pts',(-69.9127473642099,-7.05031257318115,
0.));
#83119=CARTESIAN_POINT('Ctrl Pts',(-69.9127473642099,-7.05031257318115,
12.));
#83120=CARTESIAN_POINT('Ctrl Pts',(-69.9315424664291,-7.05769817180857,
0.));
#83121=CARTESIAN_POINT('Ctrl Pts',(-69.9315424664291,-7.05769817180857,
12.));
#83122=CARTESIAN_POINT('Ctrl Pts',(-69.9503783975727,-7.06512290312849,
0.));
#83123=CARTESIAN_POINT('Ctrl Pts',(-69.9503783975727,-7.06512290312849,
12.));
#83124=CARTESIAN_POINT('Ctrl Pts',(-69.9692549527296,-7.07258678080831,
0.));
#83125=CARTESIAN_POINT('Ctrl Pts',(-69.9692549527296,-7.07258678080831,
12.));
#83126=CARTESIAN_POINT('Ctrl Pts',(-69.988171923788,-7.08008981844652,0.));
#83127=CARTESIAN_POINT('Ctrl Pts',(-69.988171923788,-7.08008981844652,12.));
#83128=CARTESIAN_POINT('Ctrl Pts',(-70.0071291040766,-7.08763202944246,
0.));
#83129=CARTESIAN_POINT('Ctrl Pts',(-70.0071291040766,-7.08763202944246,
12.));
#83130=CARTESIAN_POINT('Ctrl Pts',(-70.0261262936388,-7.09521342684248,
0.));
#83131=CARTESIAN_POINT('Ctrl Pts',(-70.0261262936388,-7.09521342684248,
12.));
#83132=CARTESIAN_POINT('Ctrl Pts',(-70.0451632990086,-7.10283402335034,
0.));
#83133=CARTESIAN_POINT('Ctrl Pts',(-70.0451632990086,-7.10283402335034,
12.));
#83134=CARTESIAN_POINT('Ctrl Pts',(-70.0642399306869,-7.11049383140445,
0.));
#83135=CARTESIAN_POINT('Ctrl Pts',(-70.0642399306869,-7.11049383140445,
12.));
#83136=CARTESIAN_POINT('Ctrl Pts',(-70.0833560013975,-7.11819286322826,
0.));
#83137=CARTESIAN_POINT('Ctrl Pts',(-70.0833560013975,-7.11819286322826,
12.));
#83138=CARTESIAN_POINT('Ctrl Pts',(-70.1025113239495,-7.12593113088903,
0.));
#83139=CARTESIAN_POINT('Ctrl Pts',(-70.1025113239495,-7.12593113088903,
12.));
#83140=CARTESIAN_POINT('Ctrl Pts',(-70.1217057094499,-7.13370864634442,
0.));
#83141=CARTESIAN_POINT('Ctrl Pts',(-70.1217057094499,-7.13370864634442,
12.));
#83142=CARTESIAN_POINT('Ctrl Pts',(-70.1409389682424,-7.14152542142373,
0.));
#83143=CARTESIAN_POINT('Ctrl Pts',(-70.1409389682424,-7.14152542142373,
12.));
#83144=CARTESIAN_POINT('Ctrl Pts',(-70.1602109107202,-7.14938146780813,
0.));
#83145=CARTESIAN_POINT('Ctrl Pts',(-70.1602109107202,-7.14938146780813,
12.));
#83146=CARTESIAN_POINT('Ctrl Pts',(-70.1795213481185,-7.15727679700933,
0.));
#83147=CARTESIAN_POINT('Ctrl Pts',(-70.1795213481185,-7.15727679700933,
12.));
#83148=CARTESIAN_POINT('Ctrl Pts',(-70.1988700934593,-7.16521142033863,
0.));
#83149=CARTESIAN_POINT('Ctrl Pts',(-70.1988700934593,-7.16521142033863,
12.));
#83150=CARTESIAN_POINT('Ctrl Pts',(-70.2182569618994,-7.17318534889715,
0.));
#83151=CARTESIAN_POINT('Ctrl Pts',(-70.2182569618994,-7.17318534889715,
12.));
#83152=CARTESIAN_POINT('Ctrl Pts',(-70.2376817702215,-7.18119859359777,
0.));
#83153=CARTESIAN_POINT('Ctrl Pts',(-70.2376817702215,-7.18119859359777,
12.));
#83154=CARTESIAN_POINT('Ctrl Pts',(-70.2571443365192,-7.18925116517555,
0.));
#83155=CARTESIAN_POINT('Ctrl Pts',(-70.2571443365192,-7.18925116517555,
12.));
#83156=CARTESIAN_POINT('Ctrl Pts',(-70.2766444798285,-7.19734307419873,
0.));
#83157=CARTESIAN_POINT('Ctrl Pts',(-70.2766444798285,-7.19734307419873,
12.));
#83158=CARTESIAN_POINT('Ctrl Pts',(-70.2961820197077,-7.20547433107482,
0.));
#83159=CARTESIAN_POINT('Ctrl Pts',(-70.2961820197077,-7.20547433107482,
12.));
#83160=CARTESIAN_POINT('Ctrl Pts',(-70.3157567762588,-7.21364494605449,
0.));
#83161=CARTESIAN_POINT('Ctrl Pts',(-70.3157567762588,-7.21364494605449,
12.));
#83162=CARTESIAN_POINT('Ctrl Pts',(-70.3353685703112,-7.22185492923191,
0.));
#83163=CARTESIAN_POINT('Ctrl Pts',(-70.3353685703112,-7.22185492923191,
12.));
#83164=CARTESIAN_POINT('Ctrl Pts',(-70.3550172235486,-7.23010429054229,
0.));
#83165=CARTESIAN_POINT('Ctrl Pts',(-70.3550172235486,-7.23010429054229,
12.));
#83166=CARTESIAN_POINT('Ctrl Pts',(-70.3747025586552,-7.23839303975606,
0.));
#83167=CARTESIAN_POINT('Ctrl Pts',(-70.3747025586552,-7.23839303975606,
12.));
#83168=CARTESIAN_POINT('Ctrl Pts',(-70.3944243994504,-7.24672118647084,
0.));
#83169=CARTESIAN_POINT('Ctrl Pts',(-70.3944243994504,-7.24672118647084,
12.));
#83170=CARTESIAN_POINT('Ctrl Pts',(-70.4141825708178,-7.25508874012043,
0.));
#83171=CARTESIAN_POINT('Ctrl Pts',(-70.4141825708178,-7.25508874012043,
12.));
#83172=CARTESIAN_POINT('Ctrl Pts',(-70.4339768986346,-7.26349570998032,
0.));
#83173=CARTESIAN_POINT('Ctrl Pts',(-70.4339768986346,-7.26349570998032,
12.));
#83174=CARTESIAN_POINT('Ctrl Pts',(-70.4538072096992,-7.27194210517062,
0.));
#83175=CARTESIAN_POINT('Ctrl Pts',(-70.4538072096992,-7.27194210517062,
12.));
#83176=CARTESIAN_POINT('Ctrl Pts',(-70.4736733316487,-7.2804279346547,0.));
#83177=CARTESIAN_POINT('Ctrl Pts',(-70.4736733316487,-7.2804279346547,12.));
#83178=CARTESIAN_POINT('Ctrl Pts',(-70.4935750929058,-7.28895320723862,
0.));
#83179=CARTESIAN_POINT('Ctrl Pts',(-70.4935750929058,-7.28895320723862,
12.));
#83180=CARTESIAN_POINT('Ctrl Pts',(-70.5135123227169,-7.29751793157822,
0.));
#83181=CARTESIAN_POINT('Ctrl Pts',(-70.5135123227169,-7.29751793157822,
12.));
#83182=CARTESIAN_POINT('Ctrl Pts',(-70.5334848511681,-7.30612211618053,
0.));
#83183=CARTESIAN_POINT('Ctrl Pts',(-70.5334848511681,-7.30612211618053,
12.));
#83184=CARTESIAN_POINT('Ctrl Pts',(-70.5534925092043,-7.31476576940391,
0.));
#83185=CARTESIAN_POINT('Ctrl Pts',(-70.5534925092043,-7.31476576940391,
12.));
#83186=CARTESIAN_POINT('Ctrl Pts',(-70.5735351286476,-7.32344889945219,
0.));
#83187=CARTESIAN_POINT('Ctrl Pts',(-70.5735351286476,-7.32344889945219,
12.));
#83188=CARTESIAN_POINT('Ctrl Pts',(-70.5936125421946,-7.3321715143759,0.));
#83189=CARTESIAN_POINT('Ctrl Pts',(-70.5936125421946,-7.3321715143759,12.));
#83190=CARTESIAN_POINT('Ctrl Pts',(-70.6137245833996,-7.34093362208007,
0.));
#83191=CARTESIAN_POINT('Ctrl Pts',(-70.6137245833996,-7.34093362208007,
12.));
#83192=CARTESIAN_POINT('Ctrl Pts',(-70.6338710866562,-7.34973523032577,
0.));
#83193=CARTESIAN_POINT('Ctrl Pts',(-70.6338710866562,-7.34973523032577,
12.));
#83194=CARTESIAN_POINT('Ctrl Pts',(-70.6540518871775,-7.35857634673054,
0.));
#83195=CARTESIAN_POINT('Ctrl Pts',(-70.6540518871775,-7.35857634673054,
12.));
#83196=CARTESIAN_POINT('Ctrl Pts',(-70.6742668209687,-7.367456978763,0.));
#83197=CARTESIAN_POINT('Ctrl Pts',(-70.6742668209687,-7.367456978763,12.));
#83198=CARTESIAN_POINT('Ctrl Pts',(-70.694515724827,-7.37637713374767,0.));
#83199=CARTESIAN_POINT('Ctrl Pts',(-70.694515724827,-7.37637713374767,12.));
#83200=CARTESIAN_POINT('Ctrl Pts',(-70.7147984363424,-7.38533681887032,
0.));
#83201=CARTESIAN_POINT('Ctrl Pts',(-70.7147984363424,-7.38533681887032,
12.));
#83202=CARTESIAN_POINT('Ctrl Pts',(-70.735114793895,-7.3943360411789,0.));
#83203=CARTESIAN_POINT('Ctrl Pts',(-70.735114793895,-7.3943360411789,12.));
#83204=CARTESIAN_POINT('Ctrl Pts',(-70.7554646366514,-7.4033748075823,0.));
#83205=CARTESIAN_POINT('Ctrl Pts',(-70.7554646366514,-7.4033748075823,12.));
#83206=CARTESIAN_POINT('Ctrl Pts',(-70.7758478045576,-7.41245312484487,
0.));
#83207=CARTESIAN_POINT('Ctrl Pts',(-70.7758478045576,-7.41245312484487,
12.));
#83208=CARTESIAN_POINT('Ctrl Pts',(-70.7962641383351,-7.42157099959316,
0.));
#83209=CARTESIAN_POINT('Ctrl Pts',(-70.7962641383351,-7.42157099959316,
12.));
#83210=CARTESIAN_POINT('Ctrl Pts',(-70.8167134794738,-7.43072843832008,
0.));
#83211=CARTESIAN_POINT('Ctrl Pts',(-70.8167134794738,-7.43072843832008,
12.));
#83212=CARTESIAN_POINT('Ctrl Pts',(-70.8371956702242,-7.43992544738606,
0.));
#83213=CARTESIAN_POINT('Ctrl Pts',(-70.8371956702242,-7.43992544738606,
12.));
#83214=CARTESIAN_POINT('Ctrl Pts',(-70.8577105535841,-7.44916203301645,
0.));
#83215=CARTESIAN_POINT('Ctrl Pts',(-70.8577105535841,-7.44916203301645,
12.));
#83216=CARTESIAN_POINT('Ctrl Pts',(-70.8782579732885,-7.45843820129776,
0.));
#83217=CARTESIAN_POINT('Ctrl Pts',(-70.8782579732885,-7.45843820129776,
12.));
#83218=CARTESIAN_POINT('Ctrl Pts',(-70.8988377738088,-7.46775395818518,
0.));
#83219=CARTESIAN_POINT('Ctrl Pts',(-70.8988377738088,-7.46775395818518,
12.));
#83220=CARTESIAN_POINT('Ctrl Pts',(-70.9194498003483,-7.47710930950554,
0.));
#83221=CARTESIAN_POINT('Ctrl Pts',(-70.9194498003483,-7.47710930950554,
12.));
#83222=CARTESIAN_POINT('Ctrl Pts',(-70.9400938988373,-7.48650426095823,
0.));
#83223=CARTESIAN_POINT('Ctrl Pts',(-70.9400938988373,-7.48650426095823,
12.));
#83224=CARTESIAN_POINT('Ctrl Pts',(-70.9607699159234,-7.49593881811141,
0.));
#83225=CARTESIAN_POINT('Ctrl Pts',(-70.9607699159234,-7.49593881811141,
12.));
#83226=CARTESIAN_POINT('Ctrl Pts',(-70.9814776989637,-7.50541298639948,
0.));
#83227=CARTESIAN_POINT('Ctrl Pts',(-70.9814776989637,-7.50541298639948,
12.));
#83228=CARTESIAN_POINT('Ctrl Pts',(-71.0022170960235,-7.51492677113111,
0.));
#83229=CARTESIAN_POINT('Ctrl Pts',(-71.0022170960235,-7.51492677113111,
12.));
#83230=CARTESIAN_POINT('Ctrl Pts',(-71.0229879558713,-7.52448017749136,
0.));
#83231=CARTESIAN_POINT('Ctrl Pts',(-71.0229879558713,-7.52448017749136,
12.));
#83232=CARTESIAN_POINT('Ctrl Pts',(-71.0437901279722,-7.53407321054253,
0.));
#83233=CARTESIAN_POINT('Ctrl Pts',(-71.0437901279722,-7.53407321054253,
12.));
#83234=CARTESIAN_POINT('Ctrl Pts',(-71.0646234624783,-7.54370587521948,
0.));
#83235=CARTESIAN_POINT('Ctrl Pts',(-71.0646234624783,-7.54370587521948,
12.));
#83236=CARTESIAN_POINT('Ctrl Pts',(-71.0854878102203,-7.55337817632872,
0.));
#83237=CARTESIAN_POINT('Ctrl Pts',(-71.0854878102203,-7.55337817632872,
12.));
#83238=CARTESIAN_POINT('Ctrl Pts',(-71.1063830227074,-7.56309011855616,
0.));
#83239=CARTESIAN_POINT('Ctrl Pts',(-71.1063830227074,-7.56309011855616,
12.));
#83240=CARTESIAN_POINT('Ctrl Pts',(-71.1273089521218,-7.57284170646866,
0.));
#83241=CARTESIAN_POINT('Ctrl Pts',(-71.1273089521218,-7.57284170646866,
12.));
#83242=CARTESIAN_POINT('Ctrl Pts',(-71.1482654513133,-7.58263294451465,
0.));
#83243=CARTESIAN_POINT('Ctrl Pts',(-71.1482654513133,-7.58263294451465,
12.));
#83244=CARTESIAN_POINT('Ctrl Pts',(-71.1692523737887,-7.5924638370186,0.));
#83245=CARTESIAN_POINT('Ctrl Pts',(-71.1692523737887,-7.5924638370186,12.));
#83246=CARTESIAN_POINT('Ctrl Pts',(-71.1902695737063,-7.60233438818156,
0.));
#83247=CARTESIAN_POINT('Ctrl Pts',(-71.1902695737063,-7.60233438818156,
12.));
#83248=CARTESIAN_POINT('Ctrl Pts',(-71.2113169058778,-7.61224460208886,
0.));
#83249=CARTESIAN_POINT('Ctrl Pts',(-71.2113169058778,-7.61224460208886,
12.));
#83250=CARTESIAN_POINT('Ctrl Pts',(-71.232394225762,-7.62219448271124,0.));
#83251=CARTESIAN_POINT('Ctrl Pts',(-71.232394225762,-7.62219448271124,12.));
#83252=CARTESIAN_POINT('Ctrl Pts',(-71.2535013894587,-7.63218403390514,
0.));
#83253=CARTESIAN_POINT('Ctrl Pts',(-71.2535013894587,-7.63218403390514,
12.));
#83254=CARTESIAN_POINT('Ctrl Pts',(-71.2746382536974,-7.64221325940671,
0.));
#83255=CARTESIAN_POINT('Ctrl Pts',(-71.2746382536974,-7.64221325940671,
12.));
#83256=CARTESIAN_POINT('Ctrl Pts',(-71.2958046758334,-7.65228216283342,
0.));
#83257=CARTESIAN_POINT('Ctrl Pts',(-71.2958046758334,-7.65228216283342,
12.));
#83258=CARTESIAN_POINT('Ctrl Pts',(-71.3170005138474,-7.66239074769119,
0.));
#83259=CARTESIAN_POINT('Ctrl Pts',(-71.3170005138474,-7.66239074769119,
12.));
#83260=CARTESIAN_POINT('Ctrl Pts',(-71.3382256263405,-7.67253901737539,
0.));
#83261=CARTESIAN_POINT('Ctrl Pts',(-71.3382256263405,-7.67253901737539,
12.));
#83262=CARTESIAN_POINT('Ctrl Pts',(-71.3594798725294,-7.68272697517103,
0.));
#83263=CARTESIAN_POINT('Ctrl Pts',(-71.3594798725294,-7.68272697517103,
12.));
#83264=CARTESIAN_POINT('Ctrl Pts',(-71.380763112236,-7.69295462424647,0.));
#83265=CARTESIAN_POINT('Ctrl Pts',(-71.380763112236,-7.69295462424647,12.));
#83266=CARTESIAN_POINT('Ctrl Pts',(-71.4020752058827,-7.70322196765572,
0.));
#83267=CARTESIAN_POINT('Ctrl Pts',(-71.4020752058827,-7.70322196765572,
12.));
#83268=CARTESIAN_POINT('Ctrl Pts',(-71.4234160144943,-7.71352900834537,
0.));
#83269=CARTESIAN_POINT('Ctrl Pts',(-71.4234160144943,-7.71352900834537,
12.));
#83270=CARTESIAN_POINT('Ctrl Pts',(-71.4447853996919,-7.72387574915544,
0.));
#83271=CARTESIAN_POINT('Ctrl Pts',(-71.4447853996919,-7.72387574915544,
12.));
#83272=CARTESIAN_POINT('Ctrl Pts',(-71.4661832236881,-7.73426219281931,
0.));
#83273=CARTESIAN_POINT('Ctrl Pts',(-71.4661832236881,-7.73426219281931,
12.));
#83274=CARTESIAN_POINT('Ctrl Pts',(-71.487609349277,-7.74468834195734,0.));
#83275=CARTESIAN_POINT('Ctrl Pts',(-71.487609349277,-7.74468834195734,12.));
#83276=CARTESIAN_POINT('Ctrl Pts',(-71.5090636398307,-7.75515419907955,
0.));
#83277=CARTESIAN_POINT('Ctrl Pts',(-71.5090636398307,-7.75515419907955,
12.));
#83278=CARTESIAN_POINT('Ctrl Pts',(-71.5305459592987,-7.76565976659218,
0.));
#83279=CARTESIAN_POINT('Ctrl Pts',(-71.5305459592987,-7.76565976659218,
12.));
#83280=CARTESIAN_POINT('Ctrl Pts',(-71.5520561722039,-7.77620504679868,
0.));
#83281=CARTESIAN_POINT('Ctrl Pts',(-71.5520561722039,-7.77620504679868,
12.));
#83282=CARTESIAN_POINT('Ctrl Pts',(-71.5735941436366,-7.78679004189935,
0.));
#83283=CARTESIAN_POINT('Ctrl Pts',(-71.5735941436366,-7.78679004189935,
12.));
#83284=CARTESIAN_POINT('Ctrl Pts',(-71.5951597392471,-7.79741475398511,
0.));
#83285=CARTESIAN_POINT('Ctrl Pts',(-71.5951597392471,-7.79741475398511,
12.));
#83286=CARTESIAN_POINT('Ctrl Pts',(-71.616752825242,-7.80807918504017,0.));
#83287=CARTESIAN_POINT('Ctrl Pts',(-71.616752825242,-7.80807918504017,12.));
#83288=CARTESIAN_POINT('Ctrl Pts',(-71.638373268384,-7.81878333694856,0.));
#83289=CARTESIAN_POINT('Ctrl Pts',(-71.638373268384,-7.81878333694856,12.));
#83290=CARTESIAN_POINT('Ctrl Pts',(-71.6600209359869,-7.82952721149504,
0.));
#83291=CARTESIAN_POINT('Ctrl Pts',(-71.6600209359869,-7.82952721149504,
12.));
#83292=CARTESIAN_POINT('Ctrl Pts',(-71.681695695912,-7.84031081036488,0.));
#83293=CARTESIAN_POINT('Ctrl Pts',(-71.681695695912,-7.84031081036488,12.));
#83294=CARTESIAN_POINT('Ctrl Pts',(-71.7033974165576,-7.85113413513739,
0.));
#83295=CARTESIAN_POINT('Ctrl Pts',(-71.7033974165576,-7.85113413513739,
12.));
#83296=CARTESIAN_POINT('Ctrl Pts',(-71.7251259668573,-7.86199718728829,
0.));
#83297=CARTESIAN_POINT('Ctrl Pts',(-71.7251259668573,-7.86199718728829,
12.));
#83298=CARTESIAN_POINT('Ctrl Pts',(-71.7468812162795,-7.87289996819654,
0.));
#83299=CARTESIAN_POINT('Ctrl Pts',(-71.7468812162795,-7.87289996819654,
12.));
#83300=CARTESIAN_POINT('Ctrl Pts',(-71.768663034824,-7.88384247914521,0.));
#83301=CARTESIAN_POINT('Ctrl Pts',(-71.768663034824,-7.88384247914521,12.));
#83302=CARTESIAN_POINT('Ctrl Pts',(-71.7904712930172,-7.89482472132135,
0.));
#83303=CARTESIAN_POINT('Ctrl Pts',(-71.7904712930172,-7.89482472132135,
12.));
#83304=CARTESIAN_POINT('Ctrl Pts',(-71.8123058619038,-7.90584669580955,
0.));
#83305=CARTESIAN_POINT('Ctrl Pts',(-71.8123058619038,-7.90584669580955,
12.));
#83306=CARTESIAN_POINT('Ctrl Pts',(-71.8341666130424,-7.9169084035937,0.));
#83307=CARTESIAN_POINT('Ctrl Pts',(-71.8341666130424,-7.9169084035937,12.));
#83308=CARTESIAN_POINT('Ctrl Pts',(-71.8560534185071,-7.928009845564,0.));
#83309=CARTESIAN_POINT('Ctrl Pts',(-71.8560534185071,-7.928009845564,12.));
#83310=CARTESIAN_POINT('Ctrl Pts',(-71.8779661508833,-7.93915102251796,
0.));
#83311=CARTESIAN_POINT('Ctrl Pts',(-71.8779661508833,-7.93915102251796,
12.));
#83312=CARTESIAN_POINT('Ctrl Pts',(-71.8999046832642,-7.95033193516046,
0.));
#83313=CARTESIAN_POINT('Ctrl Pts',(-71.8999046832642,-7.95033193516046,
12.));
#83314=CARTESIAN_POINT('Ctrl Pts',(-71.9218688892426,-7.96155258409751,
0.));
#83315=CARTESIAN_POINT('Ctrl Pts',(-71.9218688892426,-7.96155258409751,
12.));
#83316=CARTESIAN_POINT('Ctrl Pts',(-71.9438586429072,-7.97281296983702,
0.));
#83317=CARTESIAN_POINT('Ctrl Pts',(-71.9438586429072,-7.97281296983702,
12.));
#83318=CARTESIAN_POINT('Ctrl Pts',(-71.9658738188421,-7.98411309279597,
0.));
#83319=CARTESIAN_POINT('Ctrl Pts',(-71.9658738188421,-7.98411309279597,
12.));
#83320=CARTESIAN_POINT('Ctrl Pts',(-71.9879142921248,-7.99545295330182,
0.));
#83321=CARTESIAN_POINT('Ctrl Pts',(-71.9879142921248,-7.99545295330182,
12.));
#83322=CARTESIAN_POINT('Ctrl Pts',(-72.0099799383216,-8.0068325515925,0.));
#83323=CARTESIAN_POINT('Ctrl Pts',(-72.0099799383216,-8.0068325515925,12.));
#83324=CARTESIAN_POINT('Ctrl Pts',(-72.0320706334802,-8.0182518878107,0.));
#83325=CARTESIAN_POINT('Ctrl Pts',(-72.0320706334802,-8.0182518878107,12.));
#83326=CARTESIAN_POINT('Ctrl Pts',(-72.0541862541262,-8.02971096200328,
0.));
#83327=CARTESIAN_POINT('Ctrl Pts',(-72.0541862541262,-8.02971096200328,
12.));
#83328=CARTESIAN_POINT('Ctrl Pts',(-72.0763266772632,-8.04120977412891,
0.));
#83329=CARTESIAN_POINT('Ctrl Pts',(-72.0763266772632,-8.04120977412891,
12.));
#83330=CARTESIAN_POINT('Ctrl Pts',(-72.0984917803702,-8.05274832405957,
0.));
#83331=CARTESIAN_POINT('Ctrl Pts',(-72.0984917803702,-8.05274832405957,
12.));
#83332=CARTESIAN_POINT('Ctrl Pts',(-72.1206814413985,-8.06432661158089,
0.));
#83333=CARTESIAN_POINT('Ctrl Pts',(-72.1206814413985,-8.06432661158089,
12.));
#83334=CARTESIAN_POINT('Ctrl Pts',(-72.1428955387648,-8.07594463638699,
0.));
#83335=CARTESIAN_POINT('Ctrl Pts',(-72.1428955387648,-8.07594463638699,
12.));
#83336=CARTESIAN_POINT('Ctrl Pts',(-72.165133951346,-8.08760239807815,0.));
#83337=CARTESIAN_POINT('Ctrl Pts',(-72.165133951346,-8.08760239807815,12.));
#83338=CARTESIAN_POINT('Ctrl Pts',(-72.18739655848,-8.09929989616873,0.));
#83339=CARTESIAN_POINT('Ctrl Pts',(-72.18739655848,-8.09929989616873,12.));
#83340=CARTESIAN_POINT('Ctrl Pts',(-72.2096832399626,-8.11103713008922,
0.));
#83341=CARTESIAN_POINT('Ctrl Pts',(-72.2096832399626,-8.11103713008922,
12.));
#83342=CARTESIAN_POINT('Ctrl Pts',(-72.2319938760451,-8.12281409918661,
0.));
#83343=CARTESIAN_POINT('Ctrl Pts',(-72.2319938760451,-8.12281409918661,
12.));
#83344=CARTESIAN_POINT('Ctrl Pts',(-72.2543283474279,-8.13463080272029,
0.));
#83345=CARTESIAN_POINT('Ctrl Pts',(-72.2543283474279,-8.13463080272029,
12.));
#83346=CARTESIAN_POINT('Ctrl Pts',(-72.2766865352552,-8.14648723985793,
0.));
#83347=CARTESIAN_POINT('Ctrl Pts',(-72.2766865352552,-8.14648723985793,
12.));
#83348=CARTESIAN_POINT('Ctrl Pts',(-72.2990683211155,-8.15838340968327,
0.));
#83349=CARTESIAN_POINT('Ctrl Pts',(-72.2990683211155,-8.15838340968327,
12.));
#83350=CARTESIAN_POINT('Ctrl Pts',(-72.3214735870402,-8.17031931119882,
0.));
#83351=CARTESIAN_POINT('Ctrl Pts',(-72.3214735870402,-8.17031931119882,
12.));
#83352=CARTESIAN_POINT('Ctrl Pts',(-72.3439022155007,-8.18229494332622,
0.));
#83353=CARTESIAN_POINT('Ctrl Pts',(-72.3439022155007,-8.18229494332622,
12.));
#83354=CARTESIAN_POINT('Ctrl Pts',(-72.3663540894034,-8.19431030490319,
0.));
#83355=CARTESIAN_POINT('Ctrl Pts',(-72.3663540894034,-8.19431030490319,
12.));
#83356=CARTESIAN_POINT('Ctrl Pts',(-72.3888290920845,-8.20636539467781,
0.));
#83357=CARTESIAN_POINT('Ctrl Pts',(-72.3888290920845,-8.20636539467781,
12.));
#83358=CARTESIAN_POINT('Ctrl Pts',(-72.4113271073091,-8.21846021131563,
0.));
#83359=CARTESIAN_POINT('Ctrl Pts',(-72.4113271073091,-8.21846021131563,
12.));
#83360=CARTESIAN_POINT('Ctrl Pts',(-72.4338480192701,-8.23059475340354,
0.));
#83361=CARTESIAN_POINT('Ctrl Pts',(-72.4338480192701,-8.23059475340354,
12.));
#83362=CARTESIAN_POINT('Ctrl Pts',(-72.4563917125842,-8.24276901945036,
0.));
#83363=CARTESIAN_POINT('Ctrl Pts',(-72.4563917125842,-8.24276901945036,
12.));
#83364=CARTESIAN_POINT('Ctrl Pts',(-72.4789580722871,-8.25498300788493,
0.));
#83365=CARTESIAN_POINT('Ctrl Pts',(-72.4789580722871,-8.25498300788493,
12.));
#83366=CARTESIAN_POINT('Ctrl Pts',(-72.501546983825,-8.26723671704923,0.));
#83367=CARTESIAN_POINT('Ctrl Pts',(-72.501546983825,-8.26723671704923,12.));
#83368=CARTESIAN_POINT('Ctrl Pts',(-72.524158333056,-8.27953014520385,0.));
#83369=CARTESIAN_POINT('Ctrl Pts',(-72.524158333056,-8.27953014520385,12.));
#83370=CARTESIAN_POINT('Ctrl Pts',(-72.5467920062522,-8.29186329053288,
0.));
#83371=CARTESIAN_POINT('Ctrl Pts',(-72.5467920062522,-8.29186329053288,
12.));
#83372=CARTESIAN_POINT('Ctrl Pts',(-72.5694478900983,-8.30423615114455,
0.));
#83373=CARTESIAN_POINT('Ctrl Pts',(-72.5694478900983,-8.30423615114455,
12.));
#83374=CARTESIAN_POINT('Ctrl Pts',(-72.5921258716899,-8.31664872507008,
0.));
#83375=CARTESIAN_POINT('Ctrl Pts',(-72.5921258716899,-8.31664872507008,
12.));
#83376=CARTESIAN_POINT('Ctrl Pts',(-72.614825838529,-8.32910101025652,0.));
#83377=CARTESIAN_POINT('Ctrl Pts',(-72.614825838529,-8.32910101025652,12.));
#83378=CARTESIAN_POINT('Ctrl Pts',(-72.6375476785208,-8.34159300456965,
0.));
#83379=CARTESIAN_POINT('Ctrl Pts',(-72.6375476785208,-8.34159300456965,
12.));
#83380=CARTESIAN_POINT('Ctrl Pts',(-72.6602912799689,-8.35412470580083,
0.));
#83381=CARTESIAN_POINT('Ctrl Pts',(-72.6602912799689,-8.35412470580083,
12.));
#83382=CARTESIAN_POINT('Ctrl Pts',(-72.68305653157,-8.36669611166833,0.));
#83383=CARTESIAN_POINT('Ctrl Pts',(-72.68305653157,-8.36669611166833,12.));
#83384=CARTESIAN_POINT('Ctrl Pts',(-72.7058433224072,-8.37930721981734,
0.));
#83385=CARTESIAN_POINT('Ctrl Pts',(-72.7058433224072,-8.37930721981734,
12.));
#83386=CARTESIAN_POINT('Ctrl Pts',(-72.728651541938,-8.39195802781406,0.));
#83387=CARTESIAN_POINT('Ctrl Pts',(-72.728651541938,-8.39195802781406,12.));
#83388=CARTESIAN_POINT('Ctrl Pts',(-72.7514810799932,-8.40464853314493,
0.));
#83389=CARTESIAN_POINT('Ctrl Pts',(-72.7514810799932,-8.40464853314493,
12.));
#83390=CARTESIAN_POINT('Ctrl Pts',(-72.7743318267876,-8.41737873322352,
0.));
#83391=CARTESIAN_POINT('Ctrl Pts',(-72.7743318267876,-8.41737873322352,
12.));
#83392=CARTESIAN_POINT('Ctrl Pts',(-72.7972036729283,-8.4301486253917,0.));
#83393=CARTESIAN_POINT('Ctrl Pts',(-72.7972036729283,-8.4301486253917,12.));
#83394=CARTESIAN_POINT('Ctrl Pts',(-72.8200965094197,-8.44295820691906,
0.));
#83395=CARTESIAN_POINT('Ctrl Pts',(-72.8200965094197,-8.44295820691906,
12.));
#83396=CARTESIAN_POINT('Ctrl Pts',(-72.8430102276703,-8.4558074749977,0.));
#83397=CARTESIAN_POINT('Ctrl Pts',(-72.8430102276703,-8.4558074749977,12.));
#83398=CARTESIAN_POINT('Ctrl Pts',(-72.8659447194918,-8.46869642673763,
0.));
#83399=CARTESIAN_POINT('Ctrl Pts',(-72.8659447194918,-8.46869642673763,
12.));
#83400=CARTESIAN_POINT('Ctrl Pts',(-72.888899877077,-8.48162505917627,0.));
#83401=CARTESIAN_POINT('Ctrl Pts',(-72.888899877077,-8.48162505917627,12.));
#83402=CARTESIAN_POINT('Ctrl Pts',(-72.9118755929785,-8.49459336928275,
0.));
#83403=CARTESIAN_POINT('Ctrl Pts',(-72.9118755929785,-8.49459336928275,
12.));
#83404=CARTESIAN_POINT('Ctrl Pts',(-72.9348717600837,-8.50760135395979,
0.));
#83405=CARTESIAN_POINT('Ctrl Pts',(-72.9348717600837,-8.50760135395979,
12.));
#83406=CARTESIAN_POINT('Ctrl Pts',(-72.9578882715923,-8.52064901004243,
0.));
#83407=CARTESIAN_POINT('Ctrl Pts',(-72.9578882715923,-8.52064901004243,
12.));
#83408=CARTESIAN_POINT('Ctrl Pts',(-72.9809250209843,-8.53373633429303,
0.));
#83409=CARTESIAN_POINT('Ctrl Pts',(-72.9809250209843,-8.53373633429303,
12.));
#83410=CARTESIAN_POINT('Ctrl Pts',(-73.0039819020663,-8.54686332340438,
0.));
#83411=CARTESIAN_POINT('Ctrl Pts',(-73.0039819020663,-8.54686332340438,
12.));
#83412=CARTESIAN_POINT('Ctrl Pts',(-73.0270588090193,-8.56002997400096,
0.));
#83413=CARTESIAN_POINT('Ctrl Pts',(-73.0270588090193,-8.56002997400096,
12.));
#83414=CARTESIAN_POINT('Ctrl Pts',(-73.0501556364482,-8.57323628263595,
0.));
#83415=CARTESIAN_POINT('Ctrl Pts',(-73.0501556364482,-8.57323628263595,
12.));
#83416=CARTESIAN_POINT('Ctrl Pts',(-73.073272279419,-8.58648224578723,0.));
#83417=CARTESIAN_POINT('Ctrl Pts',(-73.073272279419,-8.58648224578723,12.));
#83418=CARTESIAN_POINT('Ctrl Pts',(-73.0964086335226,-8.59976785984538,
0.));
#83419=CARTESIAN_POINT('Ctrl Pts',(-73.0964086335226,-8.59976785984538,
12.));
#83420=CARTESIAN_POINT('Ctrl Pts',(-73.1195645948169,-8.61309312111988,
0.));
#83421=CARTESIAN_POINT('Ctrl Pts',(-73.1195645948169,-8.61309312111988,
12.));
#83422=CARTESIAN_POINT('Ctrl Pts',(-73.142740059703,-8.62645802585474,0.));
#83423=CARTESIAN_POINT('Ctrl Pts',(-73.142740059703,-8.62645802585474,12.));
#83424=CARTESIAN_POINT('Ctrl Pts',(-73.165934924813,-8.63986257023735,0.));
#83425=CARTESIAN_POINT('Ctrl Pts',(-73.165934924813,-8.63986257023735,12.));
#83426=CARTESIAN_POINT('Ctrl Pts',(-73.1891490869057,-8.65330675040535,
0.));
#83427=CARTESIAN_POINT('Ctrl Pts',(-73.1891490869057,-8.65330675040535,
12.));
#83428=CARTESIAN_POINT('Ctrl Pts',(-73.2123824427212,-8.66679056245095,
0.));
#83429=CARTESIAN_POINT('Ctrl Pts',(-73.2123824427212,-8.66679056245095,
12.));
#83430=CARTESIAN_POINT('Ctrl Pts',(-73.2356348889704,-8.68031400241883,
0.));
#83431=CARTESIAN_POINT('Ctrl Pts',(-73.2356348889704,-8.68031400241883,
12.));
#83432=CARTESIAN_POINT('Ctrl Pts',(-73.2589063226373,-8.69387706629304,
0.));
#83433=CARTESIAN_POINT('Ctrl Pts',(-73.2589063226373,-8.69387706629304,
12.));
#83434=CARTESIAN_POINT('Ctrl Pts',(-73.282196641216,-8.70747974998244,0.));
#83435=CARTESIAN_POINT('Ctrl Pts',(-73.282196641216,-8.70747974998244,12.));
#83436=CARTESIAN_POINT('Ctrl Pts',(-73.3055057429744,-8.72112204930232,
0.));
#83437=CARTESIAN_POINT('Ctrl Pts',(-73.3055057429744,-8.72112204930232,
12.));
#83438=CARTESIAN_POINT('Ctrl Pts',(-73.3288335271989,-8.73480395995359,
0.));
#83439=CARTESIAN_POINT('Ctrl Pts',(-73.3288335271989,-8.73480395995359,
12.));
#83440=CARTESIAN_POINT('Ctrl Pts',(-73.3521798944595,-8.74852547749736,
0.));
#83441=CARTESIAN_POINT('Ctrl Pts',(-73.3521798944595,-8.74852547749736,
12.));
#83442=CARTESIAN_POINT('Ctrl Pts',(-73.3755447460235,-8.76228659740304,
0.));
#83443=CARTESIAN_POINT('Ctrl Pts',(-73.3755447460235,-8.76228659740304,
12.));
#83444=CARTESIAN_POINT('Ctrl Pts',(-73.3989279832808,-8.77608731509303,
0.));
#83445=CARTESIAN_POINT('Ctrl Pts',(-73.3989279832808,-8.77608731509303,
12.));
#83446=CARTESIAN_POINT('Ctrl Pts',(-73.422329507112,-8.78992762598738,0.));
#83447=CARTESIAN_POINT('Ctrl Pts',(-73.422329507112,-8.78992762598738,12.));
#83448=CARTESIAN_POINT('Ctrl Pts',(-73.4457492173949,-8.80380752553714,
0.));
#83449=CARTESIAN_POINT('Ctrl Pts',(-73.4457492173949,-8.80380752553714,
12.));
#83450=CARTESIAN_POINT('Ctrl Pts',(-73.4691870121608,-8.81772700927593,
0.));
#83451=CARTESIAN_POINT('Ctrl Pts',(-73.4691870121608,-8.81772700927593,
12.));
#83452=CARTESIAN_POINT('Ctrl Pts',(-73.4926427882787,-8.83168607277414,
0.));
#83453=CARTESIAN_POINT('Ctrl Pts',(-73.4926427882787,-8.83168607277414,
12.));
#83454=CARTESIAN_POINT('Ctrl Pts',(-73.5161164429765,-8.84568471153893,
0.));
#83455=CARTESIAN_POINT('Ctrl Pts',(-73.5161164429765,-8.84568471153893,
12.));
#83456=CARTESIAN_POINT('Ctrl Pts',(-73.5396078751672,-8.85972292092182,
0.));
#83457=CARTESIAN_POINT('Ctrl Pts',(-73.5396078751672,-8.85972292092182,
12.));
#83458=CARTESIAN_POINT('Ctrl Pts',(-73.5631169867113,-8.87380069602954,
0.));
#83459=CARTESIAN_POINT('Ctrl Pts',(-73.5631169867113,-8.87380069602954,
12.));
#83460=CARTESIAN_POINT('Ctrl Pts',(-73.5866436840493,-8.8879180316034,0.));
#83461=CARTESIAN_POINT('Ctrl Pts',(-73.5866436840493,-8.8879180316034,12.));
#83462=CARTESIAN_POINT('Ctrl Pts',(-73.6101878785868,-8.90207492198871,
0.));
#83463=CARTESIAN_POINT('Ctrl Pts',(-73.6101878785868,-8.90207492198871,
12.));
#83464=CARTESIAN_POINT('Ctrl Pts',(-73.6337494830846,-8.91627136139886,
0.));
#83465=CARTESIAN_POINT('Ctrl Pts',(-73.6337494830846,-8.91627136139886,
12.));
#83466=CARTESIAN_POINT('Ctrl Pts',(-73.6573284088088,-8.9305073441197,0.));
#83467=CARTESIAN_POINT('Ctrl Pts',(-73.6573284088088,-8.9305073441197,12.));
#83468=CARTESIAN_POINT('Ctrl Pts',(-73.6809245622361,-8.94478286474383,
0.));
#83469=CARTESIAN_POINT('Ctrl Pts',(-73.6809245622361,-8.94478286474383,
12.));
#83470=CARTESIAN_POINT('Ctrl Pts',(-73.7045378422775,-8.9590979183629,0.));
#83471=CARTESIAN_POINT('Ctrl Pts',(-73.7045378422775,-8.9590979183629,12.));
#83472=CARTESIAN_POINT('Ctrl Pts',(-73.7281681364031,-8.97345250083917,
0.));
#83473=CARTESIAN_POINT('Ctrl Pts',(-73.7281681364031,-8.97345250083917,
12.));
#83474=CARTESIAN_POINT('Ctrl Pts',(-73.7518153262253,-8.98784660837827,
0.));
#83475=CARTESIAN_POINT('Ctrl Pts',(-73.7518153262253,-8.98784660837827,
12.));
#83476=CARTESIAN_POINT('Ctrl Pts',(-73.7754792943925,-9.00228023701466,
0.));
#83477=CARTESIAN_POINT('Ctrl Pts',(-73.7754792943925,-9.00228023701466,
12.));
#83478=CARTESIAN_POINT('Ctrl Pts',(-73.7991599312731,-9.01675338208221,
0.));
#83479=CARTESIAN_POINT('Ctrl Pts',(-73.7991599312731,-9.01675338208221,
12.));
#83480=CARTESIAN_POINT('Ctrl Pts',(-73.8228571411607,-9.0312660377798,0.));
#83481=CARTESIAN_POINT('Ctrl Pts',(-73.8228571411607,-9.0312660377798,12.));
#83482=CARTESIAN_POINT('Ctrl Pts',(-73.8465708500679,-9.04581819646384,
0.));
#83483=CARTESIAN_POINT('Ctrl Pts',(-73.8465708500679,-9.04581819646384,
12.));
#83484=CARTESIAN_POINT('Ctrl Pts',(-73.870301007746,-9.06040984889249,0.));
#83485=CARTESIAN_POINT('Ctrl Pts',(-73.870301007746,-9.06040984889249,12.));
#83486=CARTESIAN_POINT('Ctrl Pts',(-73.8940475821756,-9.07504098570547,
0.));
#83487=CARTESIAN_POINT('Ctrl Pts',(-73.8940475821756,-9.07504098570547,
12.));
#83488=CARTESIAN_POINT('Ctrl Pts',(-73.9130579611989,-9.08677747601237,
0.));
#83489=CARTESIAN_POINT('Ctrl Pts',(-73.9130579611989,-9.08677747601237,
12.));
#83490=CARTESIAN_POINT('Ctrl Pts',(-73.9273231219464,-9.09559760528458,
0.));
#83491=CARTESIAN_POINT('Ctrl Pts',(-73.9273231219464,-9.09559760528458,
12.));
#83492=CARTESIAN_POINT('Ctrl Pts',(-73.9368365074164,-9.10148558516323,
0.));
#83493=CARTESIAN_POINT('Ctrl Pts',(-73.9368365074164,-9.10148558516323,
12.));
#83494=CARTESIAN_POINT('Ctrl Pts',(-73.9415940197274,-9.10443154852686,
0.));
#83495=CARTESIAN_POINT('Ctrl Pts',(-73.9415940197274,-9.10443154852686,
12.));
#83496=CARTESIAN_POINT('',(-69.6540253893192,-6.95102489306925,0.));
#83497=CARTESIAN_POINT('Ctrl Pts',(-69.6540253893192,-6.95102489306925,
0.));
#83498=CARTESIAN_POINT('Ctrl Pts',(-69.6576616146467,-6.95238884849025,
0.));
#83499=CARTESIAN_POINT('Ctrl Pts',(-69.664938391983,-6.95512065317599,0.));
#83500=CARTESIAN_POINT('Ctrl Pts',(-69.6758665380378,-6.95923004173591,
0.));
#83501=CARTESIAN_POINT('Ctrl Pts',(-69.6904633605421,-6.96473259049513,
0.));
#83502=CARTESIAN_POINT('Ctrl Pts',(-69.7087526479973,-6.97164972291439,
0.));
#83503=CARTESIAN_POINT('Ctrl Pts',(-69.7270851557366,-6.97860581164527,
0.));
#83504=CARTESIAN_POINT('Ctrl Pts',(-69.7454607995607,-6.98560086924214,
0.));
#83505=CARTESIAN_POINT('Ctrl Pts',(-69.7638794280419,-6.9926349102794,0.));
#83506=CARTESIAN_POINT('Ctrl Pts',(-69.782340824259,-6.99970795069476,0.));
#83507=CARTESIAN_POINT('Ctrl Pts',(-69.8008447346863,-7.0068200071815,0.));
#83508=CARTESIAN_POINT('Ctrl Pts',(-69.8193908913722,-7.01397109655454,
0.));
#83509=CARTESIAN_POINT('Ctrl Pts',(-69.8379790360518,-7.02116123514451,
0.));
#83510=CARTESIAN_POINT('Ctrl Pts',(-69.8566089455375,-7.02839043811812,
0.));
#83511=CARTESIAN_POINT('Ctrl Pts',(-69.8752804235238,-7.03565871972221,
0.));
#83512=CARTESIAN_POINT('Ctrl Pts',(-69.8939932885841,-7.04296609362165,
0.));
#83513=CARTESIAN_POINT('Ctrl Pts',(-69.9127473642099,-7.05031257318115,
0.));
#83514=CARTESIAN_POINT('Ctrl Pts',(-69.9315424664291,-7.05769817180857,
0.));
#83515=CARTESIAN_POINT('Ctrl Pts',(-69.9503783975727,-7.06512290312849,
0.));
#83516=CARTESIAN_POINT('Ctrl Pts',(-69.9692549527296,-7.07258678080831,
0.));
#83517=CARTESIAN_POINT('Ctrl Pts',(-69.988171923788,-7.08008981844652,0.));
#83518=CARTESIAN_POINT('Ctrl Pts',(-70.0071291040766,-7.08763202944246,
0.));
#83519=CARTESIAN_POINT('Ctrl Pts',(-70.0261262936388,-7.09521342684248,
0.));
#83520=CARTESIAN_POINT('Ctrl Pts',(-70.0451632990086,-7.10283402335034,
0.));
#83521=CARTESIAN_POINT('Ctrl Pts',(-70.0642399306869,-7.11049383140445,
0.));
#83522=CARTESIAN_POINT('Ctrl Pts',(-70.0833560013975,-7.11819286322826,
0.));
#83523=CARTESIAN_POINT('Ctrl Pts',(-70.1025113239495,-7.12593113088903,
0.));
#83524=CARTESIAN_POINT('Ctrl Pts',(-70.1217057094499,-7.13370864634442,
0.));
#83525=CARTESIAN_POINT('Ctrl Pts',(-70.1409389682424,-7.14152542142373,
0.));
#83526=CARTESIAN_POINT('Ctrl Pts',(-70.1602109107202,-7.14938146780813,
0.));
#83527=CARTESIAN_POINT('Ctrl Pts',(-70.1795213481185,-7.15727679700933,
0.));
#83528=CARTESIAN_POINT('Ctrl Pts',(-70.1988700934593,-7.16521142033863,
0.));
#83529=CARTESIAN_POINT('Ctrl Pts',(-70.2182569618994,-7.17318534889715,
0.));
#83530=CARTESIAN_POINT('Ctrl Pts',(-70.2376817702215,-7.18119859359777,
0.));
#83531=CARTESIAN_POINT('Ctrl Pts',(-70.2571443365192,-7.18925116517555,
0.));
#83532=CARTESIAN_POINT('Ctrl Pts',(-70.2766444798285,-7.19734307419873,
0.));
#83533=CARTESIAN_POINT('Ctrl Pts',(-70.2961820197077,-7.20547433107482,
0.));
#83534=CARTESIAN_POINT('Ctrl Pts',(-70.3157567762588,-7.21364494605449,
0.));
#83535=CARTESIAN_POINT('Ctrl Pts',(-70.3353685703112,-7.22185492923191,
0.));
#83536=CARTESIAN_POINT('Ctrl Pts',(-70.3550172235486,-7.23010429054229,
0.));
#83537=CARTESIAN_POINT('Ctrl Pts',(-70.3747025586552,-7.23839303975606,
0.));
#83538=CARTESIAN_POINT('Ctrl Pts',(-70.3944243994504,-7.24672118647084,
0.));
#83539=CARTESIAN_POINT('Ctrl Pts',(-70.4141825708178,-7.25508874012043,
0.));
#83540=CARTESIAN_POINT('Ctrl Pts',(-70.4339768986346,-7.26349570998032,
0.));
#83541=CARTESIAN_POINT('Ctrl Pts',(-70.4538072096992,-7.27194210517062,
0.));
#83542=CARTESIAN_POINT('Ctrl Pts',(-70.4736733316487,-7.2804279346547,0.));
#83543=CARTESIAN_POINT('Ctrl Pts',(-70.4935750929058,-7.28895320723862,
0.));
#83544=CARTESIAN_POINT('Ctrl Pts',(-70.5135123227169,-7.29751793157822,
0.));
#83545=CARTESIAN_POINT('Ctrl Pts',(-70.5334848511681,-7.30612211618053,
0.));
#83546=CARTESIAN_POINT('Ctrl Pts',(-70.5534925092043,-7.31476576940391,
0.));
#83547=CARTESIAN_POINT('Ctrl Pts',(-70.5735351286476,-7.32344889945219,
0.));
#83548=CARTESIAN_POINT('Ctrl Pts',(-70.5936125421946,-7.3321715143759,0.));
#83549=CARTESIAN_POINT('Ctrl Pts',(-70.6137245833996,-7.34093362208007,
0.));
#83550=CARTESIAN_POINT('Ctrl Pts',(-70.6338710866562,-7.34973523032577,
0.));
#83551=CARTESIAN_POINT('Ctrl Pts',(-70.6540518871775,-7.35857634673054,
0.));
#83552=CARTESIAN_POINT('Ctrl Pts',(-70.6742668209687,-7.367456978763,0.));
#83553=CARTESIAN_POINT('Ctrl Pts',(-70.694515724827,-7.37637713374767,0.));
#83554=CARTESIAN_POINT('Ctrl Pts',(-70.7147984363424,-7.38533681887032,
0.));
#83555=CARTESIAN_POINT('Ctrl Pts',(-70.735114793895,-7.3943360411789,0.));
#83556=CARTESIAN_POINT('Ctrl Pts',(-70.7554646366514,-7.4033748075823,0.));
#83557=CARTESIAN_POINT('Ctrl Pts',(-70.7758478045576,-7.41245312484487,
0.));
#83558=CARTESIAN_POINT('Ctrl Pts',(-70.7962641383351,-7.42157099959316,
0.));
#83559=CARTESIAN_POINT('Ctrl Pts',(-70.8167134794738,-7.43072843832008,
0.));
#83560=CARTESIAN_POINT('Ctrl Pts',(-70.8371956702242,-7.43992544738606,
0.));
#83561=CARTESIAN_POINT('Ctrl Pts',(-70.8577105535841,-7.44916203301645,
0.));
#83562=CARTESIAN_POINT('Ctrl Pts',(-70.8782579732885,-7.45843820129776,
0.));
#83563=CARTESIAN_POINT('Ctrl Pts',(-70.8988377738088,-7.46775395818518,
0.));
#83564=CARTESIAN_POINT('Ctrl Pts',(-70.9194498003483,-7.47710930950554,
0.));
#83565=CARTESIAN_POINT('Ctrl Pts',(-70.9400938988373,-7.48650426095823,
0.));
#83566=CARTESIAN_POINT('Ctrl Pts',(-70.9607699159234,-7.49593881811141,
0.));
#83567=CARTESIAN_POINT('Ctrl Pts',(-70.9814776989637,-7.50541298639948,
0.));
#83568=CARTESIAN_POINT('Ctrl Pts',(-71.0022170960235,-7.51492677113111,
0.));
#83569=CARTESIAN_POINT('Ctrl Pts',(-71.0229879558713,-7.52448017749136,
0.));
#83570=CARTESIAN_POINT('Ctrl Pts',(-71.0437901279722,-7.53407321054253,
0.));
#83571=CARTESIAN_POINT('Ctrl Pts',(-71.0646234624783,-7.54370587521948,
0.));
#83572=CARTESIAN_POINT('Ctrl Pts',(-71.0854878102203,-7.55337817632872,
0.));
#83573=CARTESIAN_POINT('Ctrl Pts',(-71.1063830227074,-7.56309011855616,
0.));
#83574=CARTESIAN_POINT('Ctrl Pts',(-71.1273089521218,-7.57284170646866,
0.));
#83575=CARTESIAN_POINT('Ctrl Pts',(-71.1482654513133,-7.58263294451465,
0.));
#83576=CARTESIAN_POINT('Ctrl Pts',(-71.1692523737887,-7.5924638370186,0.));
#83577=CARTESIAN_POINT('Ctrl Pts',(-71.1902695737063,-7.60233438818156,
0.));
#83578=CARTESIAN_POINT('Ctrl Pts',(-71.2113169058778,-7.61224460208886,
0.));
#83579=CARTESIAN_POINT('Ctrl Pts',(-71.232394225762,-7.62219448271124,0.));
#83580=CARTESIAN_POINT('Ctrl Pts',(-71.2535013894587,-7.63218403390514,
0.));
#83581=CARTESIAN_POINT('Ctrl Pts',(-71.2746382536974,-7.64221325940671,
0.));
#83582=CARTESIAN_POINT('Ctrl Pts',(-71.2958046758334,-7.65228216283342,
0.));
#83583=CARTESIAN_POINT('Ctrl Pts',(-71.3170005138474,-7.66239074769119,
0.));
#83584=CARTESIAN_POINT('Ctrl Pts',(-71.3382256263405,-7.67253901737539,
0.));
#83585=CARTESIAN_POINT('Ctrl Pts',(-71.3594798725294,-7.68272697517103,
0.));
#83586=CARTESIAN_POINT('Ctrl Pts',(-71.380763112236,-7.69295462424647,0.));
#83587=CARTESIAN_POINT('Ctrl Pts',(-71.4020752058827,-7.70322196765572,
0.));
#83588=CARTESIAN_POINT('Ctrl Pts',(-71.4234160144943,-7.71352900834537,
0.));
#83589=CARTESIAN_POINT('Ctrl Pts',(-71.4447853996919,-7.72387574915544,
0.));
#83590=CARTESIAN_POINT('Ctrl Pts',(-71.4661832236881,-7.73426219281931,
0.));
#83591=CARTESIAN_POINT('Ctrl Pts',(-71.487609349277,-7.74468834195734,0.));
#83592=CARTESIAN_POINT('Ctrl Pts',(-71.5090636398307,-7.75515419907955,
0.));
#83593=CARTESIAN_POINT('Ctrl Pts',(-71.5305459592987,-7.76565976659218,
0.));
#83594=CARTESIAN_POINT('Ctrl Pts',(-71.5520561722039,-7.77620504679868,
0.));
#83595=CARTESIAN_POINT('Ctrl Pts',(-71.5735941436366,-7.78679004189935,
0.));
#83596=CARTESIAN_POINT('Ctrl Pts',(-71.5951597392471,-7.79741475398511,
0.));
#83597=CARTESIAN_POINT('Ctrl Pts',(-71.616752825242,-7.80807918504017,0.));
#83598=CARTESIAN_POINT('Ctrl Pts',(-71.638373268384,-7.81878333694856,0.));
#83599=CARTESIAN_POINT('Ctrl Pts',(-71.6600209359869,-7.82952721149504,
0.));
#83600=CARTESIAN_POINT('Ctrl Pts',(-71.681695695912,-7.84031081036488,0.));
#83601=CARTESIAN_POINT('Ctrl Pts',(-71.7033974165576,-7.85113413513739,
0.));
#83602=CARTESIAN_POINT('Ctrl Pts',(-71.7251259668573,-7.86199718728829,
0.));
#83603=CARTESIAN_POINT('Ctrl Pts',(-71.7468812162795,-7.87289996819654,
0.));
#83604=CARTESIAN_POINT('Ctrl Pts',(-71.768663034824,-7.88384247914521,0.));
#83605=CARTESIAN_POINT('Ctrl Pts',(-71.7904712930172,-7.89482472132135,
0.));
#83606=CARTESIAN_POINT('Ctrl Pts',(-71.8123058619038,-7.90584669580955,
0.));
#83607=CARTESIAN_POINT('Ctrl Pts',(-71.8341666130424,-7.9169084035937,0.));
#83608=CARTESIAN_POINT('Ctrl Pts',(-71.8560534185071,-7.928009845564,0.));
#83609=CARTESIAN_POINT('Ctrl Pts',(-71.8779661508833,-7.93915102251796,
0.));
#83610=CARTESIAN_POINT('Ctrl Pts',(-71.8999046832642,-7.95033193516046,
0.));
#83611=CARTESIAN_POINT('Ctrl Pts',(-71.9218688892426,-7.96155258409751,
0.));
#83612=CARTESIAN_POINT('Ctrl Pts',(-71.9438586429072,-7.97281296983702,
0.));
#83613=CARTESIAN_POINT('Ctrl Pts',(-71.9658738188421,-7.98411309279597,
0.));
#83614=CARTESIAN_POINT('Ctrl Pts',(-71.9879142921248,-7.99545295330182,
0.));
#83615=CARTESIAN_POINT('Ctrl Pts',(-72.0099799383216,-8.0068325515925,0.));
#83616=CARTESIAN_POINT('Ctrl Pts',(-72.0320706334802,-8.0182518878107,0.));
#83617=CARTESIAN_POINT('Ctrl Pts',(-72.0541862541262,-8.02971096200328,
0.));
#83618=CARTESIAN_POINT('Ctrl Pts',(-72.0763266772632,-8.04120977412891,
0.));
#83619=CARTESIAN_POINT('Ctrl Pts',(-72.0984917803702,-8.05274832405957,
0.));
#83620=CARTESIAN_POINT('Ctrl Pts',(-72.1206814413985,-8.06432661158089,
0.));
#83621=CARTESIAN_POINT('Ctrl Pts',(-72.1428955387648,-8.07594463638699,
0.));
#83622=CARTESIAN_POINT('Ctrl Pts',(-72.165133951346,-8.08760239807815,0.));
#83623=CARTESIAN_POINT('Ctrl Pts',(-72.18739655848,-8.09929989616873,0.));
#83624=CARTESIAN_POINT('Ctrl Pts',(-72.2096832399626,-8.11103713008922,
0.));
#83625=CARTESIAN_POINT('Ctrl Pts',(-72.2319938760451,-8.12281409918661,
0.));
#83626=CARTESIAN_POINT('Ctrl Pts',(-72.2543283474279,-8.13463080272029,
0.));
#83627=CARTESIAN_POINT('Ctrl Pts',(-72.2766865352552,-8.14648723985793,
0.));
#83628=CARTESIAN_POINT('Ctrl Pts',(-72.2990683211155,-8.15838340968327,
0.));
#83629=CARTESIAN_POINT('Ctrl Pts',(-72.3214735870402,-8.17031931119882,
0.));
#83630=CARTESIAN_POINT('Ctrl Pts',(-72.3439022155007,-8.18229494332622,
0.));
#83631=CARTESIAN_POINT('Ctrl Pts',(-72.3663540894034,-8.19431030490319,
0.));
#83632=CARTESIAN_POINT('Ctrl Pts',(-72.3888290920845,-8.20636539467781,
0.));
#83633=CARTESIAN_POINT('Ctrl Pts',(-72.4113271073091,-8.21846021131563,
0.));
#83634=CARTESIAN_POINT('Ctrl Pts',(-72.4338480192701,-8.23059475340354,
0.));
#83635=CARTESIAN_POINT('Ctrl Pts',(-72.4563917125842,-8.24276901945036,
0.));
#83636=CARTESIAN_POINT('Ctrl Pts',(-72.4789580722871,-8.25498300788493,
0.));
#83637=CARTESIAN_POINT('Ctrl Pts',(-72.501546983825,-8.26723671704923,0.));
#83638=CARTESIAN_POINT('Ctrl Pts',(-72.524158333056,-8.27953014520385,0.));
#83639=CARTESIAN_POINT('Ctrl Pts',(-72.5467920062522,-8.29186329053288,
0.));
#83640=CARTESIAN_POINT('Ctrl Pts',(-72.5694478900983,-8.30423615114455,
0.));
#83641=CARTESIAN_POINT('Ctrl Pts',(-72.5921258716899,-8.31664872507008,
0.));
#83642=CARTESIAN_POINT('Ctrl Pts',(-72.614825838529,-8.32910101025652,0.));
#83643=CARTESIAN_POINT('Ctrl Pts',(-72.6375476785208,-8.34159300456965,
0.));
#83644=CARTESIAN_POINT('Ctrl Pts',(-72.6602912799689,-8.35412470580083,
0.));
#83645=CARTESIAN_POINT('Ctrl Pts',(-72.68305653157,-8.36669611166833,0.));
#83646=CARTESIAN_POINT('Ctrl Pts',(-72.7058433224072,-8.37930721981734,
0.));
#83647=CARTESIAN_POINT('Ctrl Pts',(-72.728651541938,-8.39195802781406,0.));
#83648=CARTESIAN_POINT('Ctrl Pts',(-72.7514810799932,-8.40464853314493,
0.));
#83649=CARTESIAN_POINT('Ctrl Pts',(-72.7743318267876,-8.41737873322352,
0.));
#83650=CARTESIAN_POINT('Ctrl Pts',(-72.7972036729283,-8.4301486253917,0.));
#83651=CARTESIAN_POINT('Ctrl Pts',(-72.8200965094197,-8.44295820691906,
0.));
#83652=CARTESIAN_POINT('Ctrl Pts',(-72.8430102276703,-8.4558074749977,0.));
#83653=CARTESIAN_POINT('Ctrl Pts',(-72.8659447194918,-8.46869642673763,
0.));
#83654=CARTESIAN_POINT('Ctrl Pts',(-72.888899877077,-8.48162505917627,0.));
#83655=CARTESIAN_POINT('Ctrl Pts',(-72.9118755929785,-8.49459336928275,
0.));
#83656=CARTESIAN_POINT('Ctrl Pts',(-72.9348717600837,-8.50760135395979,
0.));
#83657=CARTESIAN_POINT('Ctrl Pts',(-72.9578882715923,-8.52064901004243,
0.));
#83658=CARTESIAN_POINT('Ctrl Pts',(-72.9809250209843,-8.53373633429303,
0.));
#83659=CARTESIAN_POINT('Ctrl Pts',(-73.0039819020663,-8.54686332340438,
0.));
#83660=CARTESIAN_POINT('Ctrl Pts',(-73.0270588090193,-8.56002997400096,
0.));
#83661=CARTESIAN_POINT('Ctrl Pts',(-73.0501556364482,-8.57323628263595,
0.));
#83662=CARTESIAN_POINT('Ctrl Pts',(-73.073272279419,-8.58648224578723,0.));
#83663=CARTESIAN_POINT('Ctrl Pts',(-73.0964086335226,-8.59976785984538,
0.));
#83664=CARTESIAN_POINT('Ctrl Pts',(-73.1195645948169,-8.61309312111988,
0.));
#83665=CARTESIAN_POINT('Ctrl Pts',(-73.142740059703,-8.62645802585474,0.));
#83666=CARTESIAN_POINT('Ctrl Pts',(-73.165934924813,-8.63986257023735,0.));
#83667=CARTESIAN_POINT('Ctrl Pts',(-73.1891490869057,-8.65330675040535,
0.));
#83668=CARTESIAN_POINT('Ctrl Pts',(-73.2123824427212,-8.66679056245095,
0.));
#83669=CARTESIAN_POINT('Ctrl Pts',(-73.2356348889704,-8.68031400241883,
0.));
#83670=CARTESIAN_POINT('Ctrl Pts',(-73.2589063226373,-8.69387706629304,
0.));
#83671=CARTESIAN_POINT('Ctrl Pts',(-73.282196641216,-8.70747974998244,0.));
#83672=CARTESIAN_POINT('Ctrl Pts',(-73.3055057429744,-8.72112204930232,
0.));
#83673=CARTESIAN_POINT('Ctrl Pts',(-73.3288335271989,-8.73480395995359,
0.));
#83674=CARTESIAN_POINT('Ctrl Pts',(-73.3521798944595,-8.74852547749736,
0.));
#83675=CARTESIAN_POINT('Ctrl Pts',(-73.3755447460235,-8.76228659740304,
0.));
#83676=CARTESIAN_POINT('Ctrl Pts',(-73.3989279832808,-8.77608731509303,
0.));
#83677=CARTESIAN_POINT('Ctrl Pts',(-73.422329507112,-8.78992762598738,0.));
#83678=CARTESIAN_POINT('Ctrl Pts',(-73.4457492173949,-8.80380752553714,
0.));
#83679=CARTESIAN_POINT('Ctrl Pts',(-73.4691870121608,-8.81772700927593,
0.));
#83680=CARTESIAN_POINT('Ctrl Pts',(-73.4926427882787,-8.83168607277414,
0.));
#83681=CARTESIAN_POINT('Ctrl Pts',(-73.5161164429765,-8.84568471153893,
0.));
#83682=CARTESIAN_POINT('Ctrl Pts',(-73.5396078751672,-8.85972292092182,
0.));
#83683=CARTESIAN_POINT('Ctrl Pts',(-73.5631169867113,-8.87380069602954,
0.));
#83684=CARTESIAN_POINT('Ctrl Pts',(-73.5866436840493,-8.8879180316034,0.));
#83685=CARTESIAN_POINT('Ctrl Pts',(-73.6101878785868,-8.90207492198871,
0.));
#83686=CARTESIAN_POINT('Ctrl Pts',(-73.6303847393444,-8.91424402151024,
0.));
#83687=CARTESIAN_POINT('Ctrl Pts',(-73.6458786305788,-8.92359518177555,
0.));
#83688=CARTESIAN_POINT('Ctrl Pts',(-73.6566618621797,-8.9301108881603,0.));
#83689=CARTESIAN_POINT('Ctrl Pts',(-73.6627293782263,-8.9337795596399,0.));
#83690=CARTESIAN_POINT('Ctrl Pts',(-73.6640787197672,-8.9345955465582,0.));
#83691=CARTESIAN_POINT('',(-69.6540253893192,-6.95102489306925,12.));
#83692=CARTESIAN_POINT('',(-69.6540253893192,-6.95102489306925,0.));
#83693=CARTESIAN_POINT('Ctrl Pts',(-73.6640787197672,-8.93459554655823,
12.));
#83694=CARTESIAN_POINT('Ctrl Pts',(-73.6627293782263,-8.93377955963992,
12.));
#83695=CARTESIAN_POINT('Ctrl Pts',(-73.6566618621798,-8.93011088816032,
12.));
#83696=CARTESIAN_POINT('Ctrl Pts',(-73.6458786305789,-8.92359518177556,
12.));
#83697=CARTESIAN_POINT('Ctrl Pts',(-73.6303847393445,-8.91424402151025,
12.));
#83698=CARTESIAN_POINT('Ctrl Pts',(-73.6101878785868,-8.90207492198871,
12.));
#83699=CARTESIAN_POINT('Ctrl Pts',(-73.5866436840493,-8.8879180316034,12.));
#83700=CARTESIAN_POINT('Ctrl Pts',(-73.5631169867113,-8.87380069602954,
12.));
#83701=CARTESIAN_POINT('Ctrl Pts',(-73.5396078751672,-8.85972292092182,
12.));
#83702=CARTESIAN_POINT('Ctrl Pts',(-73.5161164429765,-8.84568471153893,
12.));
#83703=CARTESIAN_POINT('Ctrl Pts',(-73.4926427882787,-8.83168607277414,
12.));
#83704=CARTESIAN_POINT('Ctrl Pts',(-73.4691870121608,-8.81772700927593,
12.));
#83705=CARTESIAN_POINT('Ctrl Pts',(-73.4457492173949,-8.80380752553714,
12.));
#83706=CARTESIAN_POINT('Ctrl Pts',(-73.422329507112,-8.78992762598738,12.));
#83707=CARTESIAN_POINT('Ctrl Pts',(-73.3989279832808,-8.77608731509303,
12.));
#83708=CARTESIAN_POINT('Ctrl Pts',(-73.3755447460235,-8.76228659740304,
12.));
#83709=CARTESIAN_POINT('Ctrl Pts',(-73.3521798944595,-8.74852547749736,
12.));
#83710=CARTESIAN_POINT('Ctrl Pts',(-73.3288335271989,-8.73480395995359,
12.));
#83711=CARTESIAN_POINT('Ctrl Pts',(-73.3055057429744,-8.72112204930232,
12.));
#83712=CARTESIAN_POINT('Ctrl Pts',(-73.282196641216,-8.70747974998244,12.));
#83713=CARTESIAN_POINT('Ctrl Pts',(-73.2589063226373,-8.69387706629304,
12.));
#83714=CARTESIAN_POINT('Ctrl Pts',(-73.2356348889704,-8.68031400241883,
12.));
#83715=CARTESIAN_POINT('Ctrl Pts',(-73.2123824427212,-8.66679056245095,
12.));
#83716=CARTESIAN_POINT('Ctrl Pts',(-73.1891490869057,-8.65330675040535,
12.));
#83717=CARTESIAN_POINT('Ctrl Pts',(-73.165934924813,-8.63986257023735,12.));
#83718=CARTESIAN_POINT('Ctrl Pts',(-73.142740059703,-8.62645802585474,12.));
#83719=CARTESIAN_POINT('Ctrl Pts',(-73.1195645948169,-8.61309312111988,
12.));
#83720=CARTESIAN_POINT('Ctrl Pts',(-73.0964086335226,-8.59976785984538,
12.));
#83721=CARTESIAN_POINT('Ctrl Pts',(-73.073272279419,-8.58648224578723,12.));
#83722=CARTESIAN_POINT('Ctrl Pts',(-73.0501556364482,-8.57323628263595,
12.));
#83723=CARTESIAN_POINT('Ctrl Pts',(-73.0270588090193,-8.56002997400096,
12.));
#83724=CARTESIAN_POINT('Ctrl Pts',(-73.0039819020663,-8.54686332340438,
12.));
#83725=CARTESIAN_POINT('Ctrl Pts',(-72.9809250209843,-8.53373633429303,
12.));
#83726=CARTESIAN_POINT('Ctrl Pts',(-72.9578882715923,-8.52064901004243,
12.));
#83727=CARTESIAN_POINT('Ctrl Pts',(-72.9348717600837,-8.50760135395979,
12.));
#83728=CARTESIAN_POINT('Ctrl Pts',(-72.9118755929785,-8.49459336928275,
12.));
#83729=CARTESIAN_POINT('Ctrl Pts',(-72.888899877077,-8.48162505917627,12.));
#83730=CARTESIAN_POINT('Ctrl Pts',(-72.8659447194918,-8.46869642673763,
12.));
#83731=CARTESIAN_POINT('Ctrl Pts',(-72.8430102276703,-8.4558074749977,12.));
#83732=CARTESIAN_POINT('Ctrl Pts',(-72.8200965094197,-8.44295820691906,
12.));
#83733=CARTESIAN_POINT('Ctrl Pts',(-72.7972036729283,-8.4301486253917,12.));
#83734=CARTESIAN_POINT('Ctrl Pts',(-72.7743318267876,-8.41737873322352,
12.));
#83735=CARTESIAN_POINT('Ctrl Pts',(-72.7514810799932,-8.40464853314493,
12.));
#83736=CARTESIAN_POINT('Ctrl Pts',(-72.728651541938,-8.39195802781406,12.));
#83737=CARTESIAN_POINT('Ctrl Pts',(-72.7058433224072,-8.37930721981734,
12.));
#83738=CARTESIAN_POINT('Ctrl Pts',(-72.68305653157,-8.36669611166833,12.));
#83739=CARTESIAN_POINT('Ctrl Pts',(-72.6602912799689,-8.35412470580083,
12.));
#83740=CARTESIAN_POINT('Ctrl Pts',(-72.6375476785208,-8.34159300456965,
12.));
#83741=CARTESIAN_POINT('Ctrl Pts',(-72.614825838529,-8.32910101025652,12.));
#83742=CARTESIAN_POINT('Ctrl Pts',(-72.5921258716899,-8.31664872507008,
12.));
#83743=CARTESIAN_POINT('Ctrl Pts',(-72.5694478900983,-8.30423615114455,
12.));
#83744=CARTESIAN_POINT('Ctrl Pts',(-72.5467920062522,-8.29186329053288,
12.));
#83745=CARTESIAN_POINT('Ctrl Pts',(-72.524158333056,-8.27953014520385,12.));
#83746=CARTESIAN_POINT('Ctrl Pts',(-72.501546983825,-8.26723671704923,12.));
#83747=CARTESIAN_POINT('Ctrl Pts',(-72.4789580722871,-8.25498300788493,
12.));
#83748=CARTESIAN_POINT('Ctrl Pts',(-72.4563917125842,-8.24276901945036,
12.));
#83749=CARTESIAN_POINT('Ctrl Pts',(-72.4338480192701,-8.23059475340354,
12.));
#83750=CARTESIAN_POINT('Ctrl Pts',(-72.4113271073091,-8.21846021131563,
12.));
#83751=CARTESIAN_POINT('Ctrl Pts',(-72.3888290920845,-8.20636539467781,
12.));
#83752=CARTESIAN_POINT('Ctrl Pts',(-72.3663540894034,-8.19431030490319,
12.));
#83753=CARTESIAN_POINT('Ctrl Pts',(-72.3439022155007,-8.18229494332622,
12.));
#83754=CARTESIAN_POINT('Ctrl Pts',(-72.3214735870402,-8.17031931119882,
12.));
#83755=CARTESIAN_POINT('Ctrl Pts',(-72.2990683211155,-8.15838340968327,
12.));
#83756=CARTESIAN_POINT('Ctrl Pts',(-72.2766865352552,-8.14648723985793,
12.));
#83757=CARTESIAN_POINT('Ctrl Pts',(-72.2543283474279,-8.13463080272029,
12.));
#83758=CARTESIAN_POINT('Ctrl Pts',(-72.2319938760451,-8.12281409918661,
12.));
#83759=CARTESIAN_POINT('Ctrl Pts',(-72.2096832399626,-8.11103713008922,
12.));
#83760=CARTESIAN_POINT('Ctrl Pts',(-72.18739655848,-8.09929989616873,12.));
#83761=CARTESIAN_POINT('Ctrl Pts',(-72.165133951346,-8.08760239807815,12.));
#83762=CARTESIAN_POINT('Ctrl Pts',(-72.1428955387648,-8.07594463638699,
12.));
#83763=CARTESIAN_POINT('Ctrl Pts',(-72.1206814413985,-8.06432661158089,
12.));
#83764=CARTESIAN_POINT('Ctrl Pts',(-72.0984917803702,-8.05274832405957,
12.));
#83765=CARTESIAN_POINT('Ctrl Pts',(-72.0763266772632,-8.04120977412891,
12.));
#83766=CARTESIAN_POINT('Ctrl Pts',(-72.0541862541262,-8.02971096200328,
12.));
#83767=CARTESIAN_POINT('Ctrl Pts',(-72.0320706334802,-8.0182518878107,12.));
#83768=CARTESIAN_POINT('Ctrl Pts',(-72.0099799383216,-8.0068325515925,12.));
#83769=CARTESIAN_POINT('Ctrl Pts',(-71.9879142921248,-7.99545295330182,
12.));
#83770=CARTESIAN_POINT('Ctrl Pts',(-71.9658738188421,-7.98411309279597,
12.));
#83771=CARTESIAN_POINT('Ctrl Pts',(-71.9438586429072,-7.97281296983702,
12.));
#83772=CARTESIAN_POINT('Ctrl Pts',(-71.9218688892426,-7.96155258409751,
12.));
#83773=CARTESIAN_POINT('Ctrl Pts',(-71.8999046832642,-7.95033193516046,
12.));
#83774=CARTESIAN_POINT('Ctrl Pts',(-71.8779661508833,-7.93915102251796,
12.));
#83775=CARTESIAN_POINT('Ctrl Pts',(-71.8560534185071,-7.928009845564,12.));
#83776=CARTESIAN_POINT('Ctrl Pts',(-71.8341666130424,-7.9169084035937,12.));
#83777=CARTESIAN_POINT('Ctrl Pts',(-71.8123058619038,-7.90584669580955,
12.));
#83778=CARTESIAN_POINT('Ctrl Pts',(-71.7904712930172,-7.89482472132135,
12.));
#83779=CARTESIAN_POINT('Ctrl Pts',(-71.768663034824,-7.88384247914521,12.));
#83780=CARTESIAN_POINT('Ctrl Pts',(-71.7468812162795,-7.87289996819654,
12.));
#83781=CARTESIAN_POINT('Ctrl Pts',(-71.7251259668573,-7.86199718728829,
12.));
#83782=CARTESIAN_POINT('Ctrl Pts',(-71.7033974165576,-7.85113413513739,
12.));
#83783=CARTESIAN_POINT('Ctrl Pts',(-71.681695695912,-7.84031081036488,12.));
#83784=CARTESIAN_POINT('Ctrl Pts',(-71.6600209359869,-7.82952721149504,
12.));
#83785=CARTESIAN_POINT('Ctrl Pts',(-71.638373268384,-7.81878333694856,12.));
#83786=CARTESIAN_POINT('Ctrl Pts',(-71.616752825242,-7.80807918504017,12.));
#83787=CARTESIAN_POINT('Ctrl Pts',(-71.5951597392471,-7.79741475398511,
12.));
#83788=CARTESIAN_POINT('Ctrl Pts',(-71.5735941436366,-7.78679004189935,
12.));
#83789=CARTESIAN_POINT('Ctrl Pts',(-71.5520561722039,-7.77620504679868,
12.));
#83790=CARTESIAN_POINT('Ctrl Pts',(-71.5305459592987,-7.76565976659218,
12.));
#83791=CARTESIAN_POINT('Ctrl Pts',(-71.5090636398307,-7.75515419907955,
12.));
#83792=CARTESIAN_POINT('Ctrl Pts',(-71.487609349277,-7.74468834195734,12.));
#83793=CARTESIAN_POINT('Ctrl Pts',(-71.4661832236881,-7.73426219281931,
12.));
#83794=CARTESIAN_POINT('Ctrl Pts',(-71.4447853996919,-7.72387574915544,
12.));
#83795=CARTESIAN_POINT('Ctrl Pts',(-71.4234160144943,-7.71352900834537,
12.));
#83796=CARTESIAN_POINT('Ctrl Pts',(-71.4020752058827,-7.70322196765572,
12.));
#83797=CARTESIAN_POINT('Ctrl Pts',(-71.380763112236,-7.69295462424647,12.));
#83798=CARTESIAN_POINT('Ctrl Pts',(-71.3594798725294,-7.68272697517103,
12.));
#83799=CARTESIAN_POINT('Ctrl Pts',(-71.3382256263405,-7.67253901737539,
12.));
#83800=CARTESIAN_POINT('Ctrl Pts',(-71.3170005138474,-7.66239074769119,
12.));
#83801=CARTESIAN_POINT('Ctrl Pts',(-71.2958046758334,-7.65228216283342,
12.));
#83802=CARTESIAN_POINT('Ctrl Pts',(-71.2746382536974,-7.64221325940671,
12.));
#83803=CARTESIAN_POINT('Ctrl Pts',(-71.2535013894587,-7.63218403390514,
12.));
#83804=CARTESIAN_POINT('Ctrl Pts',(-71.232394225762,-7.62219448271124,12.));
#83805=CARTESIAN_POINT('Ctrl Pts',(-71.2113169058778,-7.61224460208886,
12.));
#83806=CARTESIAN_POINT('Ctrl Pts',(-71.1902695737063,-7.60233438818156,
12.));
#83807=CARTESIAN_POINT('Ctrl Pts',(-71.1692523737887,-7.5924638370186,12.));
#83808=CARTESIAN_POINT('Ctrl Pts',(-71.1482654513133,-7.58263294451465,
12.));
#83809=CARTESIAN_POINT('Ctrl Pts',(-71.1273089521218,-7.57284170646866,
12.));
#83810=CARTESIAN_POINT('Ctrl Pts',(-71.1063830227074,-7.56309011855616,
12.));
#83811=CARTESIAN_POINT('Ctrl Pts',(-71.0854878102203,-7.55337817632872,
12.));
#83812=CARTESIAN_POINT('Ctrl Pts',(-71.0646234624783,-7.54370587521948,
12.));
#83813=CARTESIAN_POINT('Ctrl Pts',(-71.0437901279722,-7.53407321054253,
12.));
#83814=CARTESIAN_POINT('Ctrl Pts',(-71.0229879558713,-7.52448017749136,
12.));
#83815=CARTESIAN_POINT('Ctrl Pts',(-71.0022170960235,-7.51492677113111,
12.));
#83816=CARTESIAN_POINT('Ctrl Pts',(-70.9814776989637,-7.50541298639948,
12.));
#83817=CARTESIAN_POINT('Ctrl Pts',(-70.9607699159234,-7.49593881811141,
12.));
#83818=CARTESIAN_POINT('Ctrl Pts',(-70.9400938988373,-7.48650426095823,
12.));
#83819=CARTESIAN_POINT('Ctrl Pts',(-70.9194498003483,-7.47710930950554,
12.));
#83820=CARTESIAN_POINT('Ctrl Pts',(-70.8988377738088,-7.46775395818518,
12.));
#83821=CARTESIAN_POINT('Ctrl Pts',(-70.8782579732885,-7.45843820129776,
12.));
#83822=CARTESIAN_POINT('Ctrl Pts',(-70.8577105535841,-7.44916203301645,
12.));
#83823=CARTESIAN_POINT('Ctrl Pts',(-70.8371956702242,-7.43992544738606,
12.));
#83824=CARTESIAN_POINT('Ctrl Pts',(-70.8167134794738,-7.43072843832008,
12.));
#83825=CARTESIAN_POINT('Ctrl Pts',(-70.7962641383351,-7.42157099959316,
12.));
#83826=CARTESIAN_POINT('Ctrl Pts',(-70.7758478045576,-7.41245312484487,
12.));
#83827=CARTESIAN_POINT('Ctrl Pts',(-70.7554646366514,-7.4033748075823,12.));
#83828=CARTESIAN_POINT('Ctrl Pts',(-70.735114793895,-7.3943360411789,12.));
#83829=CARTESIAN_POINT('Ctrl Pts',(-70.7147984363424,-7.38533681887032,
12.));
#83830=CARTESIAN_POINT('Ctrl Pts',(-70.694515724827,-7.37637713374767,12.));
#83831=CARTESIAN_POINT('Ctrl Pts',(-70.6742668209687,-7.367456978763,12.));
#83832=CARTESIAN_POINT('Ctrl Pts',(-70.6540518871775,-7.35857634673054,
12.));
#83833=CARTESIAN_POINT('Ctrl Pts',(-70.6338710866562,-7.34973523032577,
12.));
#83834=CARTESIAN_POINT('Ctrl Pts',(-70.6137245833996,-7.34093362208007,
12.));
#83835=CARTESIAN_POINT('Ctrl Pts',(-70.5936125421946,-7.3321715143759,12.));
#83836=CARTESIAN_POINT('Ctrl Pts',(-70.5735351286476,-7.32344889945219,
12.));
#83837=CARTESIAN_POINT('Ctrl Pts',(-70.5534925092043,-7.31476576940391,
12.));
#83838=CARTESIAN_POINT('Ctrl Pts',(-70.5334848511681,-7.30612211618053,
12.));
#83839=CARTESIAN_POINT('Ctrl Pts',(-70.5135123227169,-7.29751793157822,
12.));
#83840=CARTESIAN_POINT('Ctrl Pts',(-70.4935750929058,-7.28895320723862,
12.));
#83841=CARTESIAN_POINT('Ctrl Pts',(-70.4736733316487,-7.2804279346547,12.));
#83842=CARTESIAN_POINT('Ctrl Pts',(-70.4538072096992,-7.27194210517062,
12.));
#83843=CARTESIAN_POINT('Ctrl Pts',(-70.4339768986346,-7.26349570998032,
12.));
#83844=CARTESIAN_POINT('Ctrl Pts',(-70.4141825708178,-7.25508874012043,
12.));
#83845=CARTESIAN_POINT('Ctrl Pts',(-70.3944243994504,-7.24672118647084,
12.));
#83846=CARTESIAN_POINT('Ctrl Pts',(-70.3747025586552,-7.23839303975606,
12.));
#83847=CARTESIAN_POINT('Ctrl Pts',(-70.3550172235486,-7.23010429054229,
12.));
#83848=CARTESIAN_POINT('Ctrl Pts',(-70.3353685703112,-7.22185492923191,
12.));
#83849=CARTESIAN_POINT('Ctrl Pts',(-70.3157567762588,-7.21364494605449,
12.));
#83850=CARTESIAN_POINT('Ctrl Pts',(-70.2961820197077,-7.20547433107482,
12.));
#83851=CARTESIAN_POINT('Ctrl Pts',(-70.2766444798285,-7.19734307419873,
12.));
#83852=CARTESIAN_POINT('Ctrl Pts',(-70.2571443365192,-7.18925116517555,
12.));
#83853=CARTESIAN_POINT('Ctrl Pts',(-70.2376817702215,-7.18119859359777,
12.));
#83854=CARTESIAN_POINT('Ctrl Pts',(-70.2182569618994,-7.17318534889715,
12.));
#83855=CARTESIAN_POINT('Ctrl Pts',(-70.1988700934593,-7.16521142033863,
12.));
#83856=CARTESIAN_POINT('Ctrl Pts',(-70.1795213481185,-7.15727679700933,
12.));
#83857=CARTESIAN_POINT('Ctrl Pts',(-70.1602109107202,-7.14938146780813,
12.));
#83858=CARTESIAN_POINT('Ctrl Pts',(-70.1409389682424,-7.14152542142373,
12.));
#83859=CARTESIAN_POINT('Ctrl Pts',(-70.1217057094499,-7.13370864634442,
12.));
#83860=CARTESIAN_POINT('Ctrl Pts',(-70.1025113239495,-7.12593113088903,
12.));
#83861=CARTESIAN_POINT('Ctrl Pts',(-70.0833560013975,-7.11819286322826,
12.));
#83862=CARTESIAN_POINT('Ctrl Pts',(-70.0642399306869,-7.11049383140445,
12.));
#83863=CARTESIAN_POINT('Ctrl Pts',(-70.0451632990086,-7.10283402335034,
12.));
#83864=CARTESIAN_POINT('Ctrl Pts',(-70.0261262936388,-7.09521342684248,
12.));
#83865=CARTESIAN_POINT('Ctrl Pts',(-70.0071291040766,-7.08763202944246,
12.));
#83866=CARTESIAN_POINT('Ctrl Pts',(-69.988171923788,-7.08008981844652,12.));
#83867=CARTESIAN_POINT('Ctrl Pts',(-69.9692549527296,-7.07258678080831,
12.));
#83868=CARTESIAN_POINT('Ctrl Pts',(-69.9503783975727,-7.06512290312849,
12.));
#83869=CARTESIAN_POINT('Ctrl Pts',(-69.9315424664291,-7.05769817180857,
12.));
#83870=CARTESIAN_POINT('Ctrl Pts',(-69.9127473642099,-7.05031257318115,
12.));
#83871=CARTESIAN_POINT('Ctrl Pts',(-69.8939932885841,-7.04296609362165,
12.));
#83872=CARTESIAN_POINT('Ctrl Pts',(-69.8752804235238,-7.03565871972221,
12.));
#83873=CARTESIAN_POINT('Ctrl Pts',(-69.8566089455375,-7.02839043811812,
12.));
#83874=CARTESIAN_POINT('Ctrl Pts',(-69.8379790360518,-7.02116123514451,
12.));
#83875=CARTESIAN_POINT('Ctrl Pts',(-69.8193908913722,-7.01397109655454,
12.));
#83876=CARTESIAN_POINT('Ctrl Pts',(-69.8008447346863,-7.0068200071815,12.));
#83877=CARTESIAN_POINT('Ctrl Pts',(-69.782340824259,-6.99970795069476,12.));
#83878=CARTESIAN_POINT('Ctrl Pts',(-69.7638794280419,-6.9926349102794,12.));
#83879=CARTESIAN_POINT('Ctrl Pts',(-69.7454607995607,-6.98560086924214,
12.));
#83880=CARTESIAN_POINT('Ctrl Pts',(-69.7270851557366,-6.97860581164527,
12.));
#83881=CARTESIAN_POINT('Ctrl Pts',(-69.7087526479973,-6.97164972291439,
12.));
#83882=CARTESIAN_POINT('Ctrl Pts',(-69.6904633605421,-6.96473259049513,
12.));
#83883=CARTESIAN_POINT('Ctrl Pts',(-69.6758665380378,-6.95923004173591,
12.));
#83884=CARTESIAN_POINT('Ctrl Pts',(-69.664938391983,-6.95512065317599,12.));
#83885=CARTESIAN_POINT('Ctrl Pts',(-69.6576616146467,-6.95238884849025,
12.));
#83886=CARTESIAN_POINT('Ctrl Pts',(-69.6540253893192,-6.95102489306925,
12.));
#83887=CARTESIAN_POINT('Ctrl Pts',(-73.4664795929942,-10.4355099267295,
-5.55111512312578E-16));
#83888=CARTESIAN_POINT('Ctrl Pts',(-73.4664795929942,-10.4355099267295,
4.));
#83889=CARTESIAN_POINT('Ctrl Pts',(-73.4664795929942,-10.4355099267295,
8.));
#83890=CARTESIAN_POINT('Ctrl Pts',(-73.4664795929942,-10.4355099267295,
12.));
#83891=CARTESIAN_POINT('Ctrl Pts',(-73.572019020007,-10.4049225807074,-5.55111512312578E-16));
#83892=CARTESIAN_POINT('Ctrl Pts',(-73.572019020007,-10.4049225807074,4.));
#83893=CARTESIAN_POINT('Ctrl Pts',(-73.572019020007,-10.4049225807074,8.00000000000001));
#83894=CARTESIAN_POINT('Ctrl Pts',(-73.572019020007,-10.4049225807074,12.));
#83895=CARTESIAN_POINT('Ctrl Pts',(-73.7377969500798,-10.2883434191781,
-5.55111512312578E-16));
#83896=CARTESIAN_POINT('Ctrl Pts',(-73.7377969500798,-10.2883434191781,
4.));
#83897=CARTESIAN_POINT('Ctrl Pts',(-73.7377969500798,-10.2883434191781,
7.99999999999999));
#83898=CARTESIAN_POINT('Ctrl Pts',(-73.7377969500798,-10.2883434191781,
12.));
#83899=CARTESIAN_POINT('Ctrl Pts',(-73.8116652760545,-10.1042001607578,
-5.55111512312578E-16));
#83900=CARTESIAN_POINT('Ctrl Pts',(-73.8116652760545,-10.1042001607578,
4.));
#83901=CARTESIAN_POINT('Ctrl Pts',(-73.8116652760545,-10.1042001607578,
8.00000000000001));
#83902=CARTESIAN_POINT('Ctrl Pts',(-73.8116652760545,-10.1042001607578,
12.));
#83903=CARTESIAN_POINT('Ctrl Pts',(-73.8227522002494,-10.0225374821233,
-5.55111512312578E-16));
#83904=CARTESIAN_POINT('Ctrl Pts',(-73.8227522002494,-10.0225374821233,
4.));
#83905=CARTESIAN_POINT('Ctrl Pts',(-73.8227522002494,-10.0225374821233,
8.));
#83906=CARTESIAN_POINT('Ctrl Pts',(-73.8227522002494,-10.0225374821233,
12.));
#83907=CARTESIAN_POINT('',(-73.4664795929942,-10.4355099267295,2.77555756156289E-16));
#83908=CARTESIAN_POINT('',(-73.8227522002494,-10.0225374821234,0.));
#83909=CARTESIAN_POINT('Ctrl Pts',(-73.4664795929942,-10.4355099267295,
4.16333634234434E-16));
#83910=CARTESIAN_POINT('Ctrl Pts',(-73.572019020007,-10.4049225807074,4.16333634234433E-16));
#83911=CARTESIAN_POINT('Ctrl Pts',(-73.6667492657629,-10.3383059169764,
4.16333634234434E-16));
#83912=CARTESIAN_POINT('Ctrl Pts',(-73.7314682122214,-10.2496275073218,
4.16333634234434E-16));
#83913=CARTESIAN_POINT('Ctrl Pts',(-73.7800074220654,-10.1831187000808,
4.16333634234434E-16));
#83914=CARTESIAN_POINT('Ctrl Pts',(-73.8116652760545,-10.1042001607578,
4.16333634234433E-16));
#83915=CARTESIAN_POINT('Ctrl Pts',(-73.8227522002494,-10.0225374821233,
4.16333634234434E-16));
#83916=CARTESIAN_POINT('',(-73.8227522002494,-10.0225374821234,12.));
#83917=CARTESIAN_POINT('Ctrl Pts',(-73.8227522002494,-10.0225374821233,
-5.55111512312578E-16));
#83918=CARTESIAN_POINT('Ctrl Pts',(-73.8227522002494,-10.0225374821233,
4.));
#83919=CARTESIAN_POINT('Ctrl Pts',(-73.8227522002494,-10.0225374821233,
8.));
#83920=CARTESIAN_POINT('Ctrl Pts',(-73.8227522002494,-10.0225374821233,
12.));
#83921=CARTESIAN_POINT('',(-73.4664795929942,-10.4355099267295,12.));
#83922=CARTESIAN_POINT('Ctrl Pts',(-73.8227522002494,-10.0225374821233,
12.));
#83923=CARTESIAN_POINT('Ctrl Pts',(-73.8116652760545,-10.1042001607578,
12.));
#83924=CARTESIAN_POINT('Ctrl Pts',(-73.7800074220654,-10.1831187000808,
12.));
#83925=CARTESIAN_POINT('Ctrl Pts',(-73.7314682122214,-10.2496275073218,
12.));
#83926=CARTESIAN_POINT('Ctrl Pts',(-73.6667492657629,-10.3383059169764,
12.));
#83927=CARTESIAN_POINT('Ctrl Pts',(-73.572019020007,-10.4049225807074,12.));
#83928=CARTESIAN_POINT('Ctrl Pts',(-73.4664795929942,-10.4355099267295,
12.));
#83929=CARTESIAN_POINT('Ctrl Pts',(-73.4664795929942,-10.4355099267295,
12.));
#83930=CARTESIAN_POINT('Ctrl Pts',(-73.4664795929942,-10.4355099267295,
8.));
#83931=CARTESIAN_POINT('Ctrl Pts',(-73.4664795929942,-10.4355099267295,
4.));
#83932=CARTESIAN_POINT('Ctrl Pts',(-73.4664795929942,-10.4355099267295,
-5.55111512312578E-16));
#83933=CARTESIAN_POINT('Origin',(-3.71623968689858E-10,-4.90253386731613E-11,
0.));
#83934=CARTESIAN_POINT('Origin',(-3.71623968689858E-10,-4.90253386731613E-11,
12.));
#83935=CARTESIAN_POINT('Origin',(-3.71623968689858E-10,-4.90253386731613E-11,
0.));
#83936=CARTESIAN_POINT('Ctrl Pts',(-74.4416140848738,-2.94891377268286,
0.));
#83937=CARTESIAN_POINT('Ctrl Pts',(-74.4416140848738,-2.94891377268286,
4.));
#83938=CARTESIAN_POINT('Ctrl Pts',(-74.4416140848738,-2.94891377268283,
8.));
#83939=CARTESIAN_POINT('Ctrl Pts',(-74.4416140848738,-2.94891377268283,
12.));
#83940=CARTESIAN_POINT('Ctrl Pts',(-74.4459635334396,-2.83911742169655,
0.));
#83941=CARTESIAN_POINT('Ctrl Pts',(-74.4459635334396,-2.83911742169655,
4.));
#83942=CARTESIAN_POINT('Ctrl Pts',(-74.4459635334396,-2.83911742169652,
8.00000000000001));
#83943=CARTESIAN_POINT('Ctrl Pts',(-74.4459635334396,-2.83911742169652,
12.));
#83944=CARTESIAN_POINT('Ctrl Pts',(-74.3877786926473,-2.64498412359339,
0.));
#83945=CARTESIAN_POINT('Ctrl Pts',(-74.3877786926473,-2.64498412359339,
4.));
#83946=CARTESIAN_POINT('Ctrl Pts',(-74.3877786926473,-2.64498412359335,
7.99999999999999));
#83947=CARTESIAN_POINT('Ctrl Pts',(-74.3877786926473,-2.64498412359335,
12.));
#83948=CARTESIAN_POINT('Ctrl Pts',(-74.2364344282703,-2.51668625693784,
0.));
#83949=CARTESIAN_POINT('Ctrl Pts',(-74.2364344282703,-2.51668625693784,
4.));
#83950=CARTESIAN_POINT('Ctrl Pts',(-74.2364344282703,-2.51668625693778,
8.00000000000001));
#83951=CARTESIAN_POINT('Ctrl Pts',(-74.2364344282703,-2.51668625693778,
12.));
#83952=CARTESIAN_POINT('Ctrl Pts',(-74.1624659714557,-2.48034921843197,
0.));
#83953=CARTESIAN_POINT('Ctrl Pts',(-74.1624659714557,-2.48034921843197,
4.));
#83954=CARTESIAN_POINT('Ctrl Pts',(-74.1624659714557,-2.48034921843191,
8.));
#83955=CARTESIAN_POINT('Ctrl Pts',(-74.1624659714557,-2.48034921843191,
12.));
#83956=CARTESIAN_POINT('',(-74.4416140848738,-2.94891377268286,0.));
#83957=CARTESIAN_POINT('',(-74.1624659714555,-2.48034921843229,0.));
#83958=CARTESIAN_POINT('Ctrl Pts',(-74.4416140848738,-2.94891377268286,
0.));
#83959=CARTESIAN_POINT('Ctrl Pts',(-74.4459635334396,-2.83911742169655,
0.));
#83960=CARTESIAN_POINT('Ctrl Pts',(-74.4127150529868,-2.72818410849474,
0.));
#83961=CARTESIAN_POINT('Ctrl Pts',(-74.3490471689146,-2.63874807903093,
0.));
#83962=CARTESIAN_POINT('Ctrl Pts',(-74.3012962558604,-2.57167105693308,
0.));
#83963=CARTESIAN_POINT('Ctrl Pts',(-74.2364344282703,-2.51668625693784,
0.));
#83964=CARTESIAN_POINT('Ctrl Pts',(-74.1624659714557,-2.48034921843197,
0.));
#83965=CARTESIAN_POINT('',(-74.1624659714555,-2.48034921843228,12.));
#83966=CARTESIAN_POINT('Ctrl Pts',(-74.1624659714557,-2.48034921843197,
0.));
#83967=CARTESIAN_POINT('Ctrl Pts',(-74.1624659714557,-2.48034921843197,
4.));
#83968=CARTESIAN_POINT('Ctrl Pts',(-74.1624659714557,-2.48034921843191,
8.));
#83969=CARTESIAN_POINT('Ctrl Pts',(-74.1624659714557,-2.48034921843191,
12.));
#83970=CARTESIAN_POINT('',(-74.4416140848738,-2.94891377268283,12.));
#83971=CARTESIAN_POINT('Ctrl Pts',(-74.1624659714557,-2.48034921843191,
12.));
#83972=CARTESIAN_POINT('Ctrl Pts',(-74.2364344282703,-2.51668625693778,
12.));
#83973=CARTESIAN_POINT('Ctrl Pts',(-74.3012962558604,-2.57167105693303,
12.));
#83974=CARTESIAN_POINT('Ctrl Pts',(-74.3490471689146,-2.63874807903089,
12.));
#83975=CARTESIAN_POINT('Ctrl Pts',(-74.4127150529868,-2.72818410849471,
12.));
#83976=CARTESIAN_POINT('Ctrl Pts',(-74.4459635334396,-2.83911742169652,
12.));
#83977=CARTESIAN_POINT('Ctrl Pts',(-74.4416140848738,-2.94891377268283,
12.));
#83978=CARTESIAN_POINT('Ctrl Pts',(-74.4416140848738,-2.94891377268283,
12.));
#83979=CARTESIAN_POINT('Ctrl Pts',(-74.4416140848738,-2.94891377268283,
8.));
#83980=CARTESIAN_POINT('Ctrl Pts',(-74.4416140848738,-2.94891377268286,
4.));
#83981=CARTESIAN_POINT('Ctrl Pts',(-74.4416140848738,-2.94891377268286,
0.));
#83982=CARTESIAN_POINT('Ctrl Pts',(-69.9947925310006,-0.85382582660898,
0.));
#83983=CARTESIAN_POINT('Ctrl Pts',(-69.9947925310006,-0.85382582660898,
12.));
#83984=CARTESIAN_POINT('Ctrl Pts',(-69.9985337959407,-0.854867673848592,
0.));
#83985=CARTESIAN_POINT('Ctrl Pts',(-69.9985337959407,-0.854867673848592,
12.));
#83986=CARTESIAN_POINT('Ctrl Pts',(-70.0060209754087,-0.856954870259201,
0.));
#83987=CARTESIAN_POINT('Ctrl Pts',(-70.0060209754087,-0.856954870259201,
12.));
#83988=CARTESIAN_POINT('Ctrl Pts',(-70.0172656933806,-0.860096170668732,
0.));
#83989=CARTESIAN_POINT('Ctrl Pts',(-70.0172656933806,-0.860096170668732,
12.));
#83990=CARTESIAN_POINT('Ctrl Pts',(-70.0322865492925,-0.864305583661541,
0.));
#83991=CARTESIAN_POINT('Ctrl Pts',(-70.0322865492925,-0.864305583661541,
12.));
#83992=CARTESIAN_POINT('Ctrl Pts',(-70.051109108301,-0.86960237787112,0.));
#83993=CARTESIAN_POINT('Ctrl Pts',(-70.051109108301,-0.86960237787112,12.));
#83994=CARTESIAN_POINT('Ctrl Pts',(-70.0699781183935,-0.874934213255836,
0.));
#83995=CARTESIAN_POINT('Ctrl Pts',(-70.0699781183935,-0.874934213255836,
12.));
#83996=CARTESIAN_POINT('Ctrl Pts',(-70.0888934967855,-0.880301109660725,
0.));
#83997=CARTESIAN_POINT('Ctrl Pts',(-70.0888934967855,-0.880301109660725,
12.));
#83998=CARTESIAN_POINT('Ctrl Pts',(-70.1078550938958,-0.885703094802532,
0.));
#83999=CARTESIAN_POINT('Ctrl Pts',(-70.1078550938958,-0.885703094802532,
12.));
#84000=CARTESIAN_POINT('Ctrl Pts',(-70.1268626950175,-0.891140203464239,
0.));
#84001=CARTESIAN_POINT('Ctrl Pts',(-70.1268626950175,-0.891140203464239,
12.));
#84002=CARTESIAN_POINT('Ctrl Pts',(-70.1459160490446,-0.89661247437184,
0.));
#84003=CARTESIAN_POINT('Ctrl Pts',(-70.1459160490446,-0.89661247437184,
12.));
#84004=CARTESIAN_POINT('Ctrl Pts',(-70.1650148905109,-0.902119947629767,
0.));
#84005=CARTESIAN_POINT('Ctrl Pts',(-70.1650148905109,-0.902119947629767,
12.));
#84006=CARTESIAN_POINT('Ctrl Pts',(-70.1841589635574,-0.907662662015781,
0.));
#84007=CARTESIAN_POINT('Ctrl Pts',(-70.1841589635574,-0.907662662015781,
12.));
#84008=CARTESIAN_POINT('Ctrl Pts',(-70.2033480471676,-0.913240652090975,
0.));
#84009=CARTESIAN_POINT('Ctrl Pts',(-70.2033480471676,-0.913240652090975,
12.));
#84010=CARTESIAN_POINT('Ctrl Pts',(-70.2225819470248,-0.918853949157115,
0.));
#84011=CARTESIAN_POINT('Ctrl Pts',(-70.2225819470248,-0.918853949157115,
12.));
#84012=CARTESIAN_POINT('Ctrl Pts',(-70.2418604835837,-0.924502582639452,
0.));
#84013=CARTESIAN_POINT('Ctrl Pts',(-70.2418604835837,-0.924502582639452,
12.));
#84014=CARTESIAN_POINT('Ctrl Pts',(-70.2611834821724,-0.930186581235545,
0.));
#84015=CARTESIAN_POINT('Ctrl Pts',(-70.2611834821724,-0.930186581235545,
12.));
#84016=CARTESIAN_POINT('Ctrl Pts',(-70.2805507606872,-0.935905974336476,
0.));
#84017=CARTESIAN_POINT('Ctrl Pts',(-70.2805507606872,-0.935905974336476,
12.));
#84018=CARTESIAN_POINT('Ctrl Pts',(-70.299962123399,-0.941660792742975,
0.));
#84019=CARTESIAN_POINT('Ctrl Pts',(-70.299962123399,-0.941660792742975,
12.));
#84020=CARTESIAN_POINT('Ctrl Pts',(-70.3194173673674,-0.9474510679296,0.));
#84021=CARTESIAN_POINT('Ctrl Pts',(-70.3194173673674,-0.9474510679296,12.));
#84022=CARTESIAN_POINT('Ctrl Pts',(-70.338916286458,-0.953276831581238,
0.));
#84023=CARTESIAN_POINT('Ctrl Pts',(-70.338916286458,-0.953276831581238,
12.));
#84024=CARTESIAN_POINT('Ctrl Pts',(-70.3584586759536,-0.959138115058827,
0.));
#84025=CARTESIAN_POINT('Ctrl Pts',(-70.3584586759536,-0.959138115058827,
12.));
#84026=CARTESIAN_POINT('Ctrl Pts',(-70.3780443377956,-0.965034948786444,
0.));
#84027=CARTESIAN_POINT('Ctrl Pts',(-70.3780443377956,-0.965034948786444,
12.));
#84028=CARTESIAN_POINT('Ctrl Pts',(-70.3976730803614,-0.970967362281171,
0.));
#84029=CARTESIAN_POINT('Ctrl Pts',(-70.3976730803614,-0.970967362281171,
12.));
#84030=CARTESIAN_POINT('Ctrl Pts',(-70.417344715957,-0.976935384450037,
0.));
#84031=CARTESIAN_POINT('Ctrl Pts',(-70.417344715957,-0.976935384450037,
12.));
#84032=CARTESIAN_POINT('Ctrl Pts',(-70.4370590590842,-0.982939043792151,
0.));
#84033=CARTESIAN_POINT('Ctrl Pts',(-70.4370590590842,-0.982939043792151,
12.));
#84034=CARTESIAN_POINT('Ctrl Pts',(-70.4568159243163,-0.988978368643646,
0.));
#84035=CARTESIAN_POINT('Ctrl Pts',(-70.4568159243163,-0.988978368643646,
12.));
#84036=CARTESIAN_POINT('Ctrl Pts',(-70.4766151245212,-0.995053387379752,
0.));
#84037=CARTESIAN_POINT('Ctrl Pts',(-70.4766151245212,-0.995053387379752,
12.));
#84038=CARTESIAN_POINT('Ctrl Pts',(-70.4964564717953,-1.00116412831442,
0.));
#84039=CARTESIAN_POINT('Ctrl Pts',(-70.4964564717953,-1.00116412831442,
12.));
#84040=CARTESIAN_POINT('Ctrl Pts',(-70.5163397782713,-1.00731061960968,
0.));
#84041=CARTESIAN_POINT('Ctrl Pts',(-70.5163397782713,-1.00731061960968,
12.));
#84042=CARTESIAN_POINT('Ctrl Pts',(-70.5362648569061,-1.01349288918537,
0.));
#84043=CARTESIAN_POINT('Ctrl Pts',(-70.5362648569061,-1.01349288918537,
12.));
#84044=CARTESIAN_POINT('Ctrl Pts',(-70.556231522419,-1.01971096460597,0.));
#84045=CARTESIAN_POINT('Ctrl Pts',(-70.556231522419,-1.01971096460597,12.));
#84046=CARTESIAN_POINT('Ctrl Pts',(-70.5762395916377,-1.02596487304048,
0.));
#84047=CARTESIAN_POINT('Ctrl Pts',(-70.5762395916377,-1.02596487304048,
12.));
#84048=CARTESIAN_POINT('Ctrl Pts',(-70.5962888829934,-1.0322546413287,0.));
#84049=CARTESIAN_POINT('Ctrl Pts',(-70.5962888829934,-1.0322546413287,12.));
#84050=CARTESIAN_POINT('Ctrl Pts',(-70.6163792162073,-1.03858029601903,
0.));
#84051=CARTESIAN_POINT('Ctrl Pts',(-70.6163792162073,-1.03858029601903,
12.));
#84052=CARTESIAN_POINT('Ctrl Pts',(-70.6365104119252,-1.04494186341156,
0.));
#84053=CARTESIAN_POINT('Ctrl Pts',(-70.6365104119252,-1.04494186341156,
12.));
#84054=CARTESIAN_POINT('Ctrl Pts',(-70.6566822912991,-1.05133936960071,
0.));
#84055=CARTESIAN_POINT('Ctrl Pts',(-70.6566822912991,-1.05133936960071,
12.));
#84056=CARTESIAN_POINT('Ctrl Pts',(-70.676894676009,-1.0577728404773,0.));
#84057=CARTESIAN_POINT('Ctrl Pts',(-70.676894676009,-1.0577728404773,12.));
#84058=CARTESIAN_POINT('Ctrl Pts',(-70.6971473884459,-1.0642423017128,0.));
#84059=CARTESIAN_POINT('Ctrl Pts',(-70.6971473884459,-1.0642423017128,12.));
#84060=CARTESIAN_POINT('Ctrl Pts',(-70.7174402518378,-1.07074777874595,
0.));
#84061=CARTESIAN_POINT('Ctrl Pts',(-70.7174402518378,-1.07074777874595,
12.));
#84062=CARTESIAN_POINT('Ctrl Pts',(-70.7377730903953,-1.07728929676408,
0.));
#84063=CARTESIAN_POINT('Ctrl Pts',(-70.7377730903953,-1.07728929676408,
12.));
#84064=CARTESIAN_POINT('Ctrl Pts',(-70.7581457294447,-1.08386688068342,
0.));
#84065=CARTESIAN_POINT('Ctrl Pts',(-70.7581457294447,-1.08386688068342,
12.));
#84066=CARTESIAN_POINT('Ctrl Pts',(-70.7785579953583,-1.09048055516426,
0.));
#84067=CARTESIAN_POINT('Ctrl Pts',(-70.7785579953583,-1.09048055516426,
12.));
#84068=CARTESIAN_POINT('Ctrl Pts',(-70.799009715484,-1.09713034462265,0.));
#84069=CARTESIAN_POINT('Ctrl Pts',(-70.799009715484,-1.09713034462265,12.));
#84070=CARTESIAN_POINT('Ctrl Pts',(-70.8195007180745,-1.10381627323946,
0.));
#84071=CARTESIAN_POINT('Ctrl Pts',(-70.8195007180745,-1.10381627323946,
12.));
#84072=CARTESIAN_POINT('Ctrl Pts',(-70.8400308322037,-1.11053836496639,
0.));
#84073=CARTESIAN_POINT('Ctrl Pts',(-70.8400308322037,-1.11053836496639,
12.));
#84074=CARTESIAN_POINT('Ctrl Pts',(-70.8605998877149,-1.11729664352992,
0.));
#84075=CARTESIAN_POINT('Ctrl Pts',(-70.8605998877149,-1.11729664352992,
12.));
#84076=CARTESIAN_POINT('Ctrl Pts',(-70.8812077152586,-1.12409113243513,
0.));
#84077=CARTESIAN_POINT('Ctrl Pts',(-70.8812077152586,-1.12409113243513,
12.));
#84078=CARTESIAN_POINT('Ctrl Pts',(-70.9018541463089,-1.13092185496564,
0.));
#84079=CARTESIAN_POINT('Ctrl Pts',(-70.9018541463089,-1.13092185496564,
12.));
#84080=CARTESIAN_POINT('Ctrl Pts',(-70.9225390131826,-1.13778883418213,
0.));
#84081=CARTESIAN_POINT('Ctrl Pts',(-70.9225390131826,-1.13778883418213,
12.));
#84082=CARTESIAN_POINT('Ctrl Pts',(-70.9432621490566,-1.14469209291488,
0.));
#84083=CARTESIAN_POINT('Ctrl Pts',(-70.9432621490566,-1.14469209291488,
12.));
#84084=CARTESIAN_POINT('Ctrl Pts',(-70.9640233879659,-1.15163165376524,
0.));
#84085=CARTESIAN_POINT('Ctrl Pts',(-70.9640233879659,-1.15163165376524,
12.));
#84086=CARTESIAN_POINT('Ctrl Pts',(-70.9848225647871,-1.15860753911485,
0.));
#84087=CARTESIAN_POINT('Ctrl Pts',(-70.9848225647871,-1.15860753911485,
12.));
#84088=CARTESIAN_POINT('Ctrl Pts',(-71.0056595152204,-1.1656197711288,0.));
#84089=CARTESIAN_POINT('Ctrl Pts',(-71.0056595152204,-1.1656197711288,12.));
#84090=CARTESIAN_POINT('Ctrl Pts',(-71.0265340757699,-1.17266837175777,
0.));
#84091=CARTESIAN_POINT('Ctrl Pts',(-71.0265340757699,-1.17266837175777,
12.));
#84092=CARTESIAN_POINT('Ctrl Pts',(-71.0474460837159,-1.17975336273504,
0.));
#84093=CARTESIAN_POINT('Ctrl Pts',(-71.0474460837159,-1.17975336273504,
12.));
#84094=CARTESIAN_POINT('Ctrl Pts',(-71.0683953771149,-1.18687476558133,
0.));
#84095=CARTESIAN_POINT('Ctrl Pts',(-71.0683953771149,-1.18687476558133,
12.));
#84096=CARTESIAN_POINT('Ctrl Pts',(-71.089381794801,-1.19403260161002,0.));
#84097=CARTESIAN_POINT('Ctrl Pts',(-71.089381794801,-1.19403260161002,12.));
#84098=CARTESIAN_POINT('Ctrl Pts',(-71.1104051763839,-1.20122689192836,
0.));
#84099=CARTESIAN_POINT('Ctrl Pts',(-71.1104051763839,-1.20122689192836,
12.));
#84100=CARTESIAN_POINT('Ctrl Pts',(-71.1314653622442,-1.20845765743647,
0.));
#84101=CARTESIAN_POINT('Ctrl Pts',(-71.1314653622442,-1.20845765743647,
12.));
#84102=CARTESIAN_POINT('Ctrl Pts',(-71.1525621935267,-1.21572491882262,
0.));
#84103=CARTESIAN_POINT('Ctrl Pts',(-71.1525621935267,-1.21572491882262,
12.));
#84104=CARTESIAN_POINT('Ctrl Pts',(-71.1736955121362,-1.22302869657017,
0.));
#84105=CARTESIAN_POINT('Ctrl Pts',(-71.1736955121362,-1.22302869657017,
12.));
#84106=CARTESIAN_POINT('Ctrl Pts',(-71.194865160732,-1.23036901096239,0.));
#84107=CARTESIAN_POINT('Ctrl Pts',(-71.194865160732,-1.23036901096239,12.));
#84108=CARTESIAN_POINT('Ctrl Pts',(-71.2160709827191,-1.23774588208427,
0.));
#84109=CARTESIAN_POINT('Ctrl Pts',(-71.2160709827191,-1.23774588208427,
12.));
#84110=CARTESIAN_POINT('Ctrl Pts',(-71.2373128222352,-1.24515932982112,
0.));
#84111=CARTESIAN_POINT('Ctrl Pts',(-71.2373128222352,-1.24515932982112,
12.));
#84112=CARTESIAN_POINT('Ctrl Pts',(-71.2585905241406,-1.25260937385568,
0.));
#84113=CARTESIAN_POINT('Ctrl Pts',(-71.2585905241406,-1.25260937385568,
12.));
#84114=CARTESIAN_POINT('Ctrl Pts',(-71.2799039340175,-1.2600960336757,0.));
#84115=CARTESIAN_POINT('Ctrl Pts',(-71.2799039340175,-1.2600960336757,12.));
#84116=CARTESIAN_POINT('Ctrl Pts',(-71.3012528981661,-1.26761932857724,
0.));
#84117=CARTESIAN_POINT('Ctrl Pts',(-71.3012528981661,-1.26761932857724,
12.));
#84118=CARTESIAN_POINT('Ctrl Pts',(-71.3226372635996,-1.27517927766608,
0.));
#84119=CARTESIAN_POINT('Ctrl Pts',(-71.3226372635996,-1.27517927766608,
12.));
#84120=CARTESIAN_POINT('Ctrl Pts',(-71.3440568780347,-1.28277589985471,
0.));
#84121=CARTESIAN_POINT('Ctrl Pts',(-71.3440568780347,-1.28277589985471,
12.));
#84122=CARTESIAN_POINT('Ctrl Pts',(-71.3655115898827,-1.29040921386059,
0.));
#84123=CARTESIAN_POINT('Ctrl Pts',(-71.3655115898827,-1.29040921386059,
12.));
#84124=CARTESIAN_POINT('Ctrl Pts',(-71.3870012482499,-1.29807923821413,
0.));
#84125=CARTESIAN_POINT('Ctrl Pts',(-71.3870012482499,-1.29807923821413,
12.));
#84126=CARTESIAN_POINT('Ctrl Pts',(-71.4085257029322,-1.30578599126139,
0.));
#84127=CARTESIAN_POINT('Ctrl Pts',(-71.4085257029322,-1.30578599126139,
12.));
#84128=CARTESIAN_POINT('Ctrl Pts',(-71.4300848044087,-1.31352949116537,
0.));
#84129=CARTESIAN_POINT('Ctrl Pts',(-71.4300848044087,-1.31352949116537,
12.));
#84130=CARTESIAN_POINT('Ctrl Pts',(-71.4516784038317,-1.32130975590226,
0.));
#84131=CARTESIAN_POINT('Ctrl Pts',(-71.4516784038317,-1.32130975590226,
12.));
#84132=CARTESIAN_POINT('Ctrl Pts',(-71.4733063530187,-1.32912680326123,
0.));
#84133=CARTESIAN_POINT('Ctrl Pts',(-71.4733063530187,-1.32912680326123,
12.));
#84134=CARTESIAN_POINT('Ctrl Pts',(-71.4949685044522,-1.33698065085219,
0.));
#84135=CARTESIAN_POINT('Ctrl Pts',(-71.4949685044522,-1.33698065085219,
12.));
#84136=CARTESIAN_POINT('Ctrl Pts',(-71.516664711275,-1.3448713161078,0.));
#84137=CARTESIAN_POINT('Ctrl Pts',(-71.516664711275,-1.3448713161078,12.));
#84138=CARTESIAN_POINT('Ctrl Pts',(-71.5383948272845,-1.35279881628455,
0.));
#84139=CARTESIAN_POINT('Ctrl Pts',(-71.5383948272845,-1.35279881628455,
12.));
#84140=CARTESIAN_POINT('Ctrl Pts',(-71.5601587069217,-1.36076316845816,
0.));
#84141=CARTESIAN_POINT('Ctrl Pts',(-71.5601587069217,-1.36076316845816,
12.));
#84142=CARTESIAN_POINT('Ctrl Pts',(-71.5819562052663,-1.36876438952465,
0.));
#84143=CARTESIAN_POINT('Ctrl Pts',(-71.5819562052663,-1.36876438952465,
12.));
#84144=CARTESIAN_POINT('Ctrl Pts',(-71.6037871780385,-1.37680249620779,
0.));
#84145=CARTESIAN_POINT('Ctrl Pts',(-71.6037871780385,-1.37680249620779,
12.));
#84146=CARTESIAN_POINT('Ctrl Pts',(-71.625651481593,-1.38487750506082,0.));
#84147=CARTESIAN_POINT('Ctrl Pts',(-71.625651481593,-1.38487750506082,12.));
#84148=CARTESIAN_POINT('Ctrl Pts',(-71.6475489729134,-1.39298943246722,
0.));
#84149=CARTESIAN_POINT('Ctrl Pts',(-71.6475489729134,-1.39298943246722,
12.));
#84150=CARTESIAN_POINT('Ctrl Pts',(-71.6694795096001,-1.40113829463576,
0.));
#84151=CARTESIAN_POINT('Ctrl Pts',(-71.6694795096001,-1.40113829463576,
12.));
#84152=CARTESIAN_POINT('Ctrl Pts',(-71.6914429498663,-1.40932410760248,
0.));
#84153=CARTESIAN_POINT('Ctrl Pts',(-71.6914429498663,-1.40932410760248,
12.));
#84154=CARTESIAN_POINT('Ctrl Pts',(-71.7134391525389,-1.41754688723773,
0.));
#84155=CARTESIAN_POINT('Ctrl Pts',(-71.7134391525389,-1.41754688723773,
12.));
#84156=CARTESIAN_POINT('Ctrl Pts',(-71.7354679770528,-1.42580664924769,
0.));
#84157=CARTESIAN_POINT('Ctrl Pts',(-71.7354679770528,-1.42580664924769,
12.));
#84158=CARTESIAN_POINT('Ctrl Pts',(-71.7575292834469,-1.43410340917495,
0.));
#84159=CARTESIAN_POINT('Ctrl Pts',(-71.7575292834469,-1.43410340917495,
12.));
#84160=CARTESIAN_POINT('Ctrl Pts',(-71.7796229323526,-1.44243718239315,
0.));
#84161=CARTESIAN_POINT('Ctrl Pts',(-71.7796229323526,-1.44243718239315,
12.));
#84162=CARTESIAN_POINT('Ctrl Pts',(-71.8017487849895,-1.45080798410965,
0.));
#84163=CARTESIAN_POINT('Ctrl Pts',(-71.8017487849895,-1.45080798410965,
12.));
#84164=CARTESIAN_POINT('Ctrl Pts',(-71.8239067031683,-1.45921582937231,
0.));
#84165=CARTESIAN_POINT('Ctrl Pts',(-71.8239067031683,-1.45921582937231,
12.));
#84166=CARTESIAN_POINT('Ctrl Pts',(-71.8460965492839,-1.46766073307088,
0.));
#84167=CARTESIAN_POINT('Ctrl Pts',(-71.8460965492839,-1.46766073307088,
12.));
#84168=CARTESIAN_POINT('Ctrl Pts',(-71.8683181863116,-1.47614270993728,
0.));
#84169=CARTESIAN_POINT('Ctrl Pts',(-71.8683181863116,-1.47614270993728,
12.));
#84170=CARTESIAN_POINT('Ctrl Pts',(-71.8905714777961,-1.48466177454019,
0.));
#84171=CARTESIAN_POINT('Ctrl Pts',(-71.8905714777961,-1.48466177454019,
12.));
#84172=CARTESIAN_POINT('Ctrl Pts',(-71.912856287848,-1.49321794128798,0.));
#84173=CARTESIAN_POINT('Ctrl Pts',(-71.912856287848,-1.49321794128798,12.));
#84174=CARTESIAN_POINT('Ctrl Pts',(-71.9351724811443,-1.50181122443534,
0.));
#84175=CARTESIAN_POINT('Ctrl Pts',(-71.9351724811443,-1.50181122443534,
12.));
#84176=CARTESIAN_POINT('Ctrl Pts',(-71.9575199229241,-1.51044163808453,
0.));
#84177=CARTESIAN_POINT('Ctrl Pts',(-71.9575199229241,-1.51044163808453,
12.));
#84178=CARTESIAN_POINT('Ctrl Pts',(-71.979898478983,-1.51910919618566,0.));
#84179=CARTESIAN_POINT('Ctrl Pts',(-71.979898478983,-1.51910919618566,12.));
#84180=CARTESIAN_POINT('Ctrl Pts',(-72.0023080156647,-1.52781391253102,
0.));
#84181=CARTESIAN_POINT('Ctrl Pts',(-72.0023080156647,-1.52781391253102,
12.));
#84182=CARTESIAN_POINT('Ctrl Pts',(-72.0247483998579,-1.53655580075812,
0.));
#84183=CARTESIAN_POINT('Ctrl Pts',(-72.0247483998579,-1.53655580075812,
12.));
#84184=CARTESIAN_POINT('Ctrl Pts',(-72.0472194989963,-1.54533487435626,
0.));
#84185=CARTESIAN_POINT('Ctrl Pts',(-72.0472194989963,-1.54533487435626,
12.));
#84186=CARTESIAN_POINT('Ctrl Pts',(-72.0697211810545,-1.55415114666773,
0.));
#84187=CARTESIAN_POINT('Ctrl Pts',(-72.0697211810545,-1.55415114666773,
12.));
#84188=CARTESIAN_POINT('Ctrl Pts',(-72.0922533145433,-1.56300463088808,
0.));
#84189=CARTESIAN_POINT('Ctrl Pts',(-72.0922533145433,-1.56300463088808,
12.));
#84190=CARTESIAN_POINT('Ctrl Pts',(-72.1148157684995,-1.5718953400604,0.));
#84191=CARTESIAN_POINT('Ctrl Pts',(-72.1148157684995,-1.5718953400604,12.));
#84192=CARTESIAN_POINT('Ctrl Pts',(-72.1374084124839,-1.58082328707803,
0.));
#84193=CARTESIAN_POINT('Ctrl Pts',(-72.1374084124839,-1.58082328707803,
12.));
#84194=CARTESIAN_POINT('Ctrl Pts',(-72.1600311165821,-1.58978848469123,
0.));
#84195=CARTESIAN_POINT('Ctrl Pts',(-72.1600311165821,-1.58978848469123,
12.));
#84196=CARTESIAN_POINT('Ctrl Pts',(-72.1826837514001,-1.59879094550847,
0.));
#84197=CARTESIAN_POINT('Ctrl Pts',(-72.1826837514001,-1.59879094550847,
12.));
#84198=CARTESIAN_POINT('Ctrl Pts',(-72.2053661880608,-1.60783068199663,
0.));
#84199=CARTESIAN_POINT('Ctrl Pts',(-72.2053661880608,-1.60783068199663,
12.));
#84200=CARTESIAN_POINT('Ctrl Pts',(-72.2280782981937,-1.6169077064754,0.));
#84201=CARTESIAN_POINT('Ctrl Pts',(-72.2280782981937,-1.6169077064754,12.));
#84202=CARTESIAN_POINT('Ctrl Pts',(-72.2508199539323,-1.6260220311193,0.));
#84203=CARTESIAN_POINT('Ctrl Pts',(-72.2508199539323,-1.6260220311193,12.));
#84204=CARTESIAN_POINT('Ctrl Pts',(-72.2735910279149,-1.63517366796463,
0.));
#84205=CARTESIAN_POINT('Ctrl Pts',(-72.2735910279149,-1.63517366796463,
12.));
#84206=CARTESIAN_POINT('Ctrl Pts',(-72.2963913932813,-1.64436262891079,
0.));
#84207=CARTESIAN_POINT('Ctrl Pts',(-72.2963913932813,-1.64436262891079,
12.));
#84208=CARTESIAN_POINT('Ctrl Pts',(-72.319220923669,-1.65358892572062,0.));
#84209=CARTESIAN_POINT('Ctrl Pts',(-72.319220923669,-1.65358892572062,12.));
#84210=CARTESIAN_POINT('Ctrl Pts',(-72.3420794932047,-1.66285257001496,
0.));
#84211=CARTESIAN_POINT('Ctrl Pts',(-72.3420794932047,-1.66285257001496,
12.));
#84212=CARTESIAN_POINT('Ctrl Pts',(-72.3649669765004,-1.67215357327365,
0.));
#84213=CARTESIAN_POINT('Ctrl Pts',(-72.3649669765004,-1.67215357327365,
12.));
#84214=CARTESIAN_POINT('Ctrl Pts',(-72.387883248654,-1.68149194684281,0.));
#84215=CARTESIAN_POINT('Ctrl Pts',(-72.387883248654,-1.68149194684281,12.));
#84216=CARTESIAN_POINT('Ctrl Pts',(-72.4108281852467,-1.69086770193637,
0.));
#84217=CARTESIAN_POINT('Ctrl Pts',(-72.4108281852467,-1.69086770193637,
12.));
#84218=CARTESIAN_POINT('Ctrl Pts',(-72.4338016623391,-1.70028084963647,
0.));
#84219=CARTESIAN_POINT('Ctrl Pts',(-72.4338016623391,-1.70028084963647,
12.));
#84220=CARTESIAN_POINT('Ctrl Pts',(-72.456803556463,-1.70973140088841,0.));
#84221=CARTESIAN_POINT('Ctrl Pts',(-72.456803556463,-1.70973140088841,12.));
#84222=CARTESIAN_POINT('Ctrl Pts',(-72.479833744618,-1.71921936650038,0.));
#84223=CARTESIAN_POINT('Ctrl Pts',(-72.479833744618,-1.71921936650038,12.));
#84224=CARTESIAN_POINT('Ctrl Pts',(-72.5028921042721,-1.72874475715103,
0.));
#84225=CARTESIAN_POINT('Ctrl Pts',(-72.5028921042721,-1.72874475715103,
12.));
#84226=CARTESIAN_POINT('Ctrl Pts',(-72.5259785133595,-1.73830758339125,
0.));
#84227=CARTESIAN_POINT('Ctrl Pts',(-72.5259785133595,-1.73830758339125,
12.));
#84228=CARTESIAN_POINT('Ctrl Pts',(-72.5490928502769,-1.74790785564473,
0.));
#84229=CARTESIAN_POINT('Ctrl Pts',(-72.5490928502769,-1.74790785564473,
12.));
#84230=CARTESIAN_POINT('Ctrl Pts',(-72.5722349938774,-1.75754558420344,
0.));
#84231=CARTESIAN_POINT('Ctrl Pts',(-72.5722349938774,-1.75754558420344,
12.));
#84232=CARTESIAN_POINT('Ctrl Pts',(-72.5954048234638,-1.76722077922574,
0.));
#84233=CARTESIAN_POINT('Ctrl Pts',(-72.5954048234638,-1.76722077922574,
12.));
#84234=CARTESIAN_POINT('Ctrl Pts',(-72.6186022187907,-1.77693345074426,
0.));
#84235=CARTESIAN_POINT('Ctrl Pts',(-72.6186022187907,-1.77693345074426,
12.));
#84236=CARTESIAN_POINT('Ctrl Pts',(-72.6418270600619,-1.78668360866811,
0.));
#84237=CARTESIAN_POINT('Ctrl Pts',(-72.6418270600619,-1.78668360866811,
12.));
#84238=CARTESIAN_POINT('Ctrl Pts',(-72.6650792279274,-1.79647126278358,
0.));
#84239=CARTESIAN_POINT('Ctrl Pts',(-72.6650792279274,-1.79647126278358,
12.));
#84240=CARTESIAN_POINT('Ctrl Pts',(-72.6883586034769,-1.8062964227505,0.));
#84241=CARTESIAN_POINT('Ctrl Pts',(-72.6883586034769,-1.8062964227505,12.));
#84242=CARTESIAN_POINT('Ctrl Pts',(-72.7116650682344,-1.81615909809871,
0.));
#84243=CARTESIAN_POINT('Ctrl Pts',(-72.7116650682344,-1.81615909809871,
12.));
#84244=CARTESIAN_POINT('Ctrl Pts',(-72.7349985041592,-1.82605929823564,
0.));
#84245=CARTESIAN_POINT('Ctrl Pts',(-72.7349985041592,-1.82605929823564,
12.));
#84246=CARTESIAN_POINT('Ctrl Pts',(-72.7583587936447,-1.83599703244924,
0.));
#84247=CARTESIAN_POINT('Ctrl Pts',(-72.7583587936447,-1.83599703244924,
12.));
#84248=CARTESIAN_POINT('Ctrl Pts',(-72.7817458195155,-1.84597230990857,
0.));
#84249=CARTESIAN_POINT('Ctrl Pts',(-72.7817458195155,-1.84597230990857,
12.));
#84250=CARTESIAN_POINT('Ctrl Pts',(-72.8051594650222,-1.85598513966113,
0.));
#84251=CARTESIAN_POINT('Ctrl Pts',(-72.8051594650222,-1.85598513966113,
12.));
#84252=CARTESIAN_POINT('Ctrl Pts',(-72.8285996138359,-1.86603553062771,
0.));
#84253=CARTESIAN_POINT('Ctrl Pts',(-72.8285996138359,-1.86603553062771,
12.));
#84254=CARTESIAN_POINT('Ctrl Pts',(-72.8520661500477,-1.87612349160944,
0.));
#84255=CARTESIAN_POINT('Ctrl Pts',(-72.8520661500477,-1.87612349160944,
12.));
#84256=CARTESIAN_POINT('Ctrl Pts',(-72.875558958168,-1.88624903129188,0.));
#84257=CARTESIAN_POINT('Ctrl Pts',(-72.875558958168,-1.88624903129188,12.));
#84258=CARTESIAN_POINT('Ctrl Pts',(-72.8990779231226,-1.89641215824582,
0.));
#84259=CARTESIAN_POINT('Ctrl Pts',(-72.8990779231226,-1.89641215824582,
12.));
#84260=CARTESIAN_POINT('Ctrl Pts',(-72.9226229302478,-1.90661288092587,
0.));
#84261=CARTESIAN_POINT('Ctrl Pts',(-72.9226229302478,-1.90661288092587,
12.));
#84262=CARTESIAN_POINT('Ctrl Pts',(-72.9461938652811,-1.91685120766436,
0.));
#84263=CARTESIAN_POINT('Ctrl Pts',(-72.9461938652811,-1.91685120766436,
12.));
#84264=CARTESIAN_POINT('Ctrl Pts',(-72.9697906143636,-1.9271271466766,0.));
#84265=CARTESIAN_POINT('Ctrl Pts',(-72.9697906143636,-1.9271271466766,12.));
#84266=CARTESIAN_POINT('Ctrl Pts',(-72.9934130640415,-1.93744070606566,
0.));
#84267=CARTESIAN_POINT('Ctrl Pts',(-72.9934130640415,-1.93744070606566,
12.));
#84268=CARTESIAN_POINT('Ctrl Pts',(-73.0170611012661,-1.94779189382302,
0.));
#84269=CARTESIAN_POINT('Ctrl Pts',(-73.0170611012661,-1.94779189382302,
12.));
#84270=CARTESIAN_POINT('Ctrl Pts',(-73.040734613391,-1.95818071782767,0.));
#84271=CARTESIAN_POINT('Ctrl Pts',(-73.040734613391,-1.95818071782767,12.));
#84272=CARTESIAN_POINT('Ctrl Pts',(-73.0644334881673,-1.96860718583932,
0.));
#84273=CARTESIAN_POINT('Ctrl Pts',(-73.0644334881673,-1.96860718583932,
12.));
#84274=CARTESIAN_POINT('Ctrl Pts',(-73.0881576137407,-1.97907130550157,
0.));
#84275=CARTESIAN_POINT('Ctrl Pts',(-73.0881576137407,-1.97907130550157,
12.));
#84276=CARTESIAN_POINT('Ctrl Pts',(-73.1119068786475,-1.98957308434918,
0.));
#84277=CARTESIAN_POINT('Ctrl Pts',(-73.1119068786475,-1.98957308434918,
12.));
#84278=CARTESIAN_POINT('Ctrl Pts',(-73.1356811718091,-2.00011252980981,
0.));
#84279=CARTESIAN_POINT('Ctrl Pts',(-73.1356811718091,-2.00011252980981,
12.));
#84280=CARTESIAN_POINT('Ctrl Pts',(-73.1594803825252,-2.01068964920467,
0.));
#84281=CARTESIAN_POINT('Ctrl Pts',(-73.1594803825252,-2.01068964920467,
12.));
#84282=CARTESIAN_POINT('Ctrl Pts',(-73.183304400462,-2.02130444974362,0.));
#84283=CARTESIAN_POINT('Ctrl Pts',(-73.183304400462,-2.02130444974362,12.));
#84284=CARTESIAN_POINT('Ctrl Pts',(-73.2071531156504,-2.03195693852454,
0.));
#84285=CARTESIAN_POINT('Ctrl Pts',(-73.2071531156504,-2.03195693852454,
12.));
#84286=CARTESIAN_POINT('Ctrl Pts',(-73.2310264184976,-2.04264712253928,
0.));
#84287=CARTESIAN_POINT('Ctrl Pts',(-73.2310264184976,-2.04264712253928,
12.));
#84288=CARTESIAN_POINT('Ctrl Pts',(-73.2549241997953,-2.05337500867403,
0.));
#84289=CARTESIAN_POINT('Ctrl Pts',(-73.2549241997953,-2.05337500867403,
12.));
#84290=CARTESIAN_POINT('Ctrl Pts',(-73.2788463507246,-2.06414060370834,
0.));
#84291=CARTESIAN_POINT('Ctrl Pts',(-73.2788463507246,-2.06414060370834,
12.));
#84292=CARTESIAN_POINT('Ctrl Pts',(-73.3027927628626,-2.07494391430941,
0.));
#84293=CARTESIAN_POINT('Ctrl Pts',(-73.3027927628626,-2.07494391430941,
12.));
#84294=CARTESIAN_POINT('Ctrl Pts',(-73.3267633281807,-2.08578494702743,
0.));
#84295=CARTESIAN_POINT('Ctrl Pts',(-73.3267633281807,-2.08578494702743,
12.));
#84296=CARTESIAN_POINT('Ctrl Pts',(-73.3507579390239,-2.09666370830716,
0.));
#84297=CARTESIAN_POINT('Ctrl Pts',(-73.3507579390239,-2.09666370830716,
12.));
#84298=CARTESIAN_POINT('Ctrl Pts',(-73.3747764880893,-2.1075802044939,0.));
#84299=CARTESIAN_POINT('Ctrl Pts',(-73.3747764880893,-2.1075802044939,12.));
#84300=CARTESIAN_POINT('Ctrl Pts',(-73.3988188684021,-2.11853444183761,
0.));
#84301=CARTESIAN_POINT('Ctrl Pts',(-73.3988188684021,-2.11853444183761,
12.));
#84302=CARTESIAN_POINT('Ctrl Pts',(-73.4228849732925,-2.12952642649367,
0.));
#84303=CARTESIAN_POINT('Ctrl Pts',(-73.4228849732925,-2.12952642649367,
12.));
#84304=CARTESIAN_POINT('Ctrl Pts',(-73.4469746963637,-2.14055616452057,
0.));
#84305=CARTESIAN_POINT('Ctrl Pts',(-73.4469746963637,-2.14055616452057,
12.));
#84306=CARTESIAN_POINT('Ctrl Pts',(-73.4710879315382,-2.15162366187906,
0.));
#84307=CARTESIAN_POINT('Ctrl Pts',(-73.4710879315382,-2.15162366187906,
12.));
#84308=CARTESIAN_POINT('Ctrl Pts',(-73.4952245731054,-2.16272892442919,
0.));
#84309=CARTESIAN_POINT('Ctrl Pts',(-73.4952245731054,-2.16272892442919,
12.));
#84310=CARTESIAN_POINT('Ctrl Pts',(-73.5193845157708,-2.17387195792306,
0.));
#84311=CARTESIAN_POINT('Ctrl Pts',(-73.5193845157708,-2.17387195792306,
12.));
#84312=CARTESIAN_POINT('Ctrl Pts',(-73.5435676546929,-2.18505276799753,
0.));
#84313=CARTESIAN_POINT('Ctrl Pts',(-73.5435676546929,-2.18505276799753,
12.));
#84314=CARTESIAN_POINT('Ctrl Pts',(-73.5677738855452,-2.19627136015678,
0.));
#84315=CARTESIAN_POINT('Ctrl Pts',(-73.5677738855452,-2.19627136015678,
12.));
#84316=CARTESIAN_POINT('Ctrl Pts',(-73.5920031044595,-2.20752773978348,
0.));
#84317=CARTESIAN_POINT('Ctrl Pts',(-73.5920031044595,-2.20752773978348,
12.));
#84318=CARTESIAN_POINT('Ctrl Pts',(-73.6162552079038,-2.21882191216518,
0.));
#84319=CARTESIAN_POINT('Ctrl Pts',(-73.6162552079038,-2.21882191216518,
12.));
#84320=CARTESIAN_POINT('Ctrl Pts',(-73.6405300925712,-2.23015388251287,
0.));
#84321=CARTESIAN_POINT('Ctrl Pts',(-73.6405300925712,-2.23015388251287,
12.));
#84322=CARTESIAN_POINT('Ctrl Pts',(-73.6648276552767,-2.24152365597697,
0.));
#84323=CARTESIAN_POINT('Ctrl Pts',(-73.6648276552767,-2.24152365597697,
12.));
#84324=CARTESIAN_POINT('Ctrl Pts',(-73.6891477928129,-2.25293123766425,
0.));
#84325=CARTESIAN_POINT('Ctrl Pts',(-73.6891477928129,-2.25293123766425,
12.));
#84326=CARTESIAN_POINT('Ctrl Pts',(-73.7134904019389,-2.26437663263667,
0.));
#84327=CARTESIAN_POINT('Ctrl Pts',(-73.7134904019389,-2.26437663263667,
12.));
#84328=CARTESIAN_POINT('Ctrl Pts',(-73.7378553796807,-2.27585984587198,
0.));
#84329=CARTESIAN_POINT('Ctrl Pts',(-73.7378553796807,-2.27585984587198,
12.));
#84330=CARTESIAN_POINT('Ctrl Pts',(-73.762242623566,-2.28738088222863,0.));
#84331=CARTESIAN_POINT('Ctrl Pts',(-73.762242623566,-2.28738088222863,12.));
#84332=CARTESIAN_POINT('Ctrl Pts',(-73.786652031885,-2.29893974640434,0.));
#84333=CARTESIAN_POINT('Ctrl Pts',(-73.786652031885,-2.29893974640434,12.));
#84334=CARTESIAN_POINT('Ctrl Pts',(-73.8110835039327,-2.31053644289416,
0.));
#84335=CARTESIAN_POINT('Ctrl Pts',(-73.8110835039327,-2.31053644289416,
12.));
#84336=CARTESIAN_POINT('Ctrl Pts',(-73.8355369402706,-2.32217097594197,
0.));
#84337=CARTESIAN_POINT('Ctrl Pts',(-73.8355369402706,-2.32217097594197,
12.));
#84338=CARTESIAN_POINT('Ctrl Pts',(-73.8600122421468,-2.33384334963957,
0.));
#84339=CARTESIAN_POINT('Ctrl Pts',(-73.8600122421468,-2.33384334963957,
12.));
#84340=CARTESIAN_POINT('Ctrl Pts',(-73.8845093109274,-2.3455535680212,0.));
#84341=CARTESIAN_POINT('Ctrl Pts',(-73.8845093109274,-2.3455535680212,12.));
#84342=CARTESIAN_POINT('Ctrl Pts',(-73.9090280474712,-2.35730163516315,
0.));
#84343=CARTESIAN_POINT('Ctrl Pts',(-73.9090280474712,-2.35730163516315,
12.));
#84344=CARTESIAN_POINT('Ctrl Pts',(-73.9335683516404,-2.36908755526003,
0.));
#84345=CARTESIAN_POINT('Ctrl Pts',(-73.9335683516404,-2.36908755526003,
12.));
#84346=CARTESIAN_POINT('Ctrl Pts',(-73.958130121465,-2.3809113327496,0.));
#84347=CARTESIAN_POINT('Ctrl Pts',(-73.958130121465,-2.3809113327496,12.));
#84348=CARTESIAN_POINT('Ctrl Pts',(-73.9827132538206,-2.39277297220756,
0.));
#84349=CARTESIAN_POINT('Ctrl Pts',(-73.9827132538206,-2.39277297220756,
12.));
#84350=CARTESIAN_POINT('Ctrl Pts',(-74.0073176459344,-2.40467247811536,
0.));
#84351=CARTESIAN_POINT('Ctrl Pts',(-74.0073176459344,-2.40467247811536,
12.));
#84352=CARTESIAN_POINT('Ctrl Pts',(-74.0319431966989,-2.41660985465251,
0.));
#84353=CARTESIAN_POINT('Ctrl Pts',(-74.0319431966989,-2.41660985465251,
12.));
#84354=CARTESIAN_POINT('Ctrl Pts',(-74.0565898079218,-2.42858510549778,
0.));
#84355=CARTESIAN_POINT('Ctrl Pts',(-74.0565898079218,-2.42858510549778,
12.));
#84356=CARTESIAN_POINT('Ctrl Pts',(-74.0812573859411,-2.44059823356675,
0.));
#84357=CARTESIAN_POINT('Ctrl Pts',(-74.0812573859411,-2.44059823356675,
12.));
#84358=CARTESIAN_POINT('Ctrl Pts',(-74.1059458420067,-2.45264924094775,
0.));
#84359=CARTESIAN_POINT('Ctrl Pts',(-74.1059458420067,-2.45264924094775,
12.));
#84360=CARTESIAN_POINT('Ctrl Pts',(-74.1306550887071,-2.46473812947959,
0.));
#84361=CARTESIAN_POINT('Ctrl Pts',(-74.1306550887071,-2.46473812947959,
12.));
#84362=CARTESIAN_POINT('Ctrl Pts',(-74.155385037148,-2.47686490120354,0.));
#84363=CARTESIAN_POINT('Ctrl Pts',(-74.155385037148,-2.47686490120354,12.));
#84364=CARTESIAN_POINT('Ctrl Pts',(-74.1801355936907,-2.48902955888384,
0.));
#84365=CARTESIAN_POINT('Ctrl Pts',(-74.1801355936907,-2.48902955888384,
12.));
#84366=CARTESIAN_POINT('Ctrl Pts',(-74.2049066572031,-2.50123210644135,
0.));
#84367=CARTESIAN_POINT('Ctrl Pts',(-74.2049066572031,-2.50123210644135,
12.));
#84368=CARTESIAN_POINT('Ctrl Pts',(-74.229698115223,-2.51347254956167,0.));
#84369=CARTESIAN_POINT('Ctrl Pts',(-74.229698115223,-2.51347254956167,12.));
#84370=CARTESIAN_POINT('Ctrl Pts',(-74.2545098494824,-2.52575089478303,
0.));
#84371=CARTESIAN_POINT('Ctrl Pts',(-74.2545098494824,-2.52575089478303,
12.));
#84372=CARTESIAN_POINT('Ctrl Pts',(-74.2793417427308,-2.53806714838286,
0.));
#84373=CARTESIAN_POINT('Ctrl Pts',(-74.2793417427308,-2.53806714838286,
12.));
#84374=CARTESIAN_POINT('Ctrl Pts',(-74.3041936853468,-2.5504213152678,0.));
#84375=CARTESIAN_POINT('Ctrl Pts',(-74.3041936853468,-2.5504213152678,12.));
#84376=CARTESIAN_POINT('Ctrl Pts',(-74.3290655814831,-2.56281339800017,
0.));
#84377=CARTESIAN_POINT('Ctrl Pts',(-74.3290655814831,-2.56281339800017,
12.));
#84378=CARTESIAN_POINT('Ctrl Pts',(-74.3539573567672,-2.57524339541389,
0.));
#84379=CARTESIAN_POINT('Ctrl Pts',(-74.3539573567672,-2.57524339541389,
12.));
#84380=CARTESIAN_POINT('Ctrl Pts',(-74.3788689603363,-2.58771130268175,
0.));
#84381=CARTESIAN_POINT('Ctrl Pts',(-74.3788689603363,-2.58771130268175,
12.));
#84382=CARTESIAN_POINT('Ctrl Pts',(-74.4038003594771,-2.60021711326977,
0.));
#84383=CARTESIAN_POINT('Ctrl Pts',(-74.4038003594771,-2.60021711326977,
12.));
#84384=CARTESIAN_POINT('Ctrl Pts',(-74.4237613007988,-2.61025207898403,
0.));
#84385=CARTESIAN_POINT('Ctrl Pts',(-74.4237613007988,-2.61025207898403,
12.));
#84386=CARTESIAN_POINT('Ctrl Pts',(-74.4387409032207,-2.61779535432112,
0.));
#84387=CARTESIAN_POINT('Ctrl Pts',(-74.4387409032207,-2.61779535432112,
12.));
#84388=CARTESIAN_POINT('Ctrl Pts',(-74.4487312586464,-2.62283178248202,
0.));
#84389=CARTESIAN_POINT('Ctrl Pts',(-74.4487312586464,-2.62283178248202,
12.));
#84390=CARTESIAN_POINT('Ctrl Pts',(-74.4537274248118,-2.62535189104655,
0.));
#84391=CARTESIAN_POINT('Ctrl Pts',(-74.4537274248118,-2.62535189104655,
12.));
#84392=CARTESIAN_POINT('',(-69.9947925310006,-0.85382582660898,0.));
#84393=CARTESIAN_POINT('Ctrl Pts',(-69.9947925310006,-0.85382582660898,
0.));
#84394=CARTESIAN_POINT('Ctrl Pts',(-69.9985337959407,-0.854867673848592,
0.));
#84395=CARTESIAN_POINT('Ctrl Pts',(-70.0060209754087,-0.856954870259201,
0.));
#84396=CARTESIAN_POINT('Ctrl Pts',(-70.0172656933806,-0.860096170668732,
0.));
#84397=CARTESIAN_POINT('Ctrl Pts',(-70.0322865492925,-0.864305583661541,
0.));
#84398=CARTESIAN_POINT('Ctrl Pts',(-70.051109108301,-0.86960237787112,0.));
#84399=CARTESIAN_POINT('Ctrl Pts',(-70.0699781183935,-0.874934213255836,
0.));
#84400=CARTESIAN_POINT('Ctrl Pts',(-70.0888934967855,-0.880301109660725,
0.));
#84401=CARTESIAN_POINT('Ctrl Pts',(-70.1078550938958,-0.885703094802532,
0.));
#84402=CARTESIAN_POINT('Ctrl Pts',(-70.1268626950175,-0.891140203464239,
0.));
#84403=CARTESIAN_POINT('Ctrl Pts',(-70.1459160490446,-0.89661247437184,
0.));
#84404=CARTESIAN_POINT('Ctrl Pts',(-70.1650148905109,-0.902119947629767,
0.));
#84405=CARTESIAN_POINT('Ctrl Pts',(-70.1841589635574,-0.907662662015781,
0.));
#84406=CARTESIAN_POINT('Ctrl Pts',(-70.2033480471676,-0.913240652090975,
0.));
#84407=CARTESIAN_POINT('Ctrl Pts',(-70.2225819470248,-0.918853949157115,
0.));
#84408=CARTESIAN_POINT('Ctrl Pts',(-70.2418604835837,-0.924502582639452,
0.));
#84409=CARTESIAN_POINT('Ctrl Pts',(-70.2611834821724,-0.930186581235545,
0.));
#84410=CARTESIAN_POINT('Ctrl Pts',(-70.2805507606872,-0.935905974336476,
0.));
#84411=CARTESIAN_POINT('Ctrl Pts',(-70.299962123399,-0.941660792742975,
0.));
#84412=CARTESIAN_POINT('Ctrl Pts',(-70.3194173673674,-0.9474510679296,0.));
#84413=CARTESIAN_POINT('Ctrl Pts',(-70.338916286458,-0.953276831581238,
0.));
#84414=CARTESIAN_POINT('Ctrl Pts',(-70.3584586759536,-0.959138115058827,
0.));
#84415=CARTESIAN_POINT('Ctrl Pts',(-70.3780443377956,-0.965034948786444,
0.));
#84416=CARTESIAN_POINT('Ctrl Pts',(-70.3976730803614,-0.970967362281171,
0.));
#84417=CARTESIAN_POINT('Ctrl Pts',(-70.417344715957,-0.976935384450037,
0.));
#84418=CARTESIAN_POINT('Ctrl Pts',(-70.4370590590842,-0.982939043792151,
0.));
#84419=CARTESIAN_POINT('Ctrl Pts',(-70.4568159243163,-0.988978368643646,
0.));
#84420=CARTESIAN_POINT('Ctrl Pts',(-70.4766151245212,-0.995053387379752,
0.));
#84421=CARTESIAN_POINT('Ctrl Pts',(-70.4964564717953,-1.00116412831442,
0.));
#84422=CARTESIAN_POINT('Ctrl Pts',(-70.5163397782713,-1.00731061960968,
0.));
#84423=CARTESIAN_POINT('Ctrl Pts',(-70.5362648569061,-1.01349288918537,
0.));
#84424=CARTESIAN_POINT('Ctrl Pts',(-70.556231522419,-1.01971096460597,0.));
#84425=CARTESIAN_POINT('Ctrl Pts',(-70.5762395916377,-1.02596487304048,
0.));
#84426=CARTESIAN_POINT('Ctrl Pts',(-70.5962888829934,-1.0322546413287,0.));
#84427=CARTESIAN_POINT('Ctrl Pts',(-70.6163792162073,-1.03858029601903,
0.));
#84428=CARTESIAN_POINT('Ctrl Pts',(-70.6365104119252,-1.04494186341156,
0.));
#84429=CARTESIAN_POINT('Ctrl Pts',(-70.6566822912991,-1.05133936960071,
0.));
#84430=CARTESIAN_POINT('Ctrl Pts',(-70.676894676009,-1.0577728404773,0.));
#84431=CARTESIAN_POINT('Ctrl Pts',(-70.6971473884459,-1.0642423017128,0.));
#84432=CARTESIAN_POINT('Ctrl Pts',(-70.7174402518378,-1.07074777874595,
0.));
#84433=CARTESIAN_POINT('Ctrl Pts',(-70.7377730903953,-1.07728929676408,
0.));
#84434=CARTESIAN_POINT('Ctrl Pts',(-70.7581457294447,-1.08386688068342,
0.));
#84435=CARTESIAN_POINT('Ctrl Pts',(-70.7785579953583,-1.09048055516426,
0.));
#84436=CARTESIAN_POINT('Ctrl Pts',(-70.799009715484,-1.09713034462265,0.));
#84437=CARTESIAN_POINT('Ctrl Pts',(-70.8195007180745,-1.10381627323946,
0.));
#84438=CARTESIAN_POINT('Ctrl Pts',(-70.8400308322037,-1.11053836496639,
0.));
#84439=CARTESIAN_POINT('Ctrl Pts',(-70.8605998877149,-1.11729664352992,
0.));
#84440=CARTESIAN_POINT('Ctrl Pts',(-70.8812077152586,-1.12409113243513,
0.));
#84441=CARTESIAN_POINT('Ctrl Pts',(-70.9018541463089,-1.13092185496564,
0.));
#84442=CARTESIAN_POINT('Ctrl Pts',(-70.9225390131826,-1.13778883418213,
0.));
#84443=CARTESIAN_POINT('Ctrl Pts',(-70.9432621490566,-1.14469209291488,
0.));
#84444=CARTESIAN_POINT('Ctrl Pts',(-70.9640233879659,-1.15163165376524,
0.));
#84445=CARTESIAN_POINT('Ctrl Pts',(-70.9848225647871,-1.15860753911485,
0.));
#84446=CARTESIAN_POINT('Ctrl Pts',(-71.0056595152204,-1.1656197711288,0.));
#84447=CARTESIAN_POINT('Ctrl Pts',(-71.0265340757699,-1.17266837175777,
0.));
#84448=CARTESIAN_POINT('Ctrl Pts',(-71.0474460837159,-1.17975336273504,
0.));
#84449=CARTESIAN_POINT('Ctrl Pts',(-71.0683953771149,-1.18687476558133,
0.));
#84450=CARTESIAN_POINT('Ctrl Pts',(-71.089381794801,-1.19403260161002,0.));
#84451=CARTESIAN_POINT('Ctrl Pts',(-71.1104051763839,-1.20122689192836,
0.));
#84452=CARTESIAN_POINT('Ctrl Pts',(-71.1314653622442,-1.20845765743647,
0.));
#84453=CARTESIAN_POINT('Ctrl Pts',(-71.1525621935267,-1.21572491882262,
0.));
#84454=CARTESIAN_POINT('Ctrl Pts',(-71.1736955121362,-1.22302869657017,
0.));
#84455=CARTESIAN_POINT('Ctrl Pts',(-71.194865160732,-1.23036901096239,0.));
#84456=CARTESIAN_POINT('Ctrl Pts',(-71.2160709827191,-1.23774588208427,
0.));
#84457=CARTESIAN_POINT('Ctrl Pts',(-71.2373128222352,-1.24515932982112,
0.));
#84458=CARTESIAN_POINT('Ctrl Pts',(-71.2585905241406,-1.25260937385568,
0.));
#84459=CARTESIAN_POINT('Ctrl Pts',(-71.2799039340175,-1.2600960336757,0.));
#84460=CARTESIAN_POINT('Ctrl Pts',(-71.3012528981661,-1.26761932857724,
0.));
#84461=CARTESIAN_POINT('Ctrl Pts',(-71.3226372635996,-1.27517927766608,
0.));
#84462=CARTESIAN_POINT('Ctrl Pts',(-71.3440568780347,-1.28277589985471,
0.));
#84463=CARTESIAN_POINT('Ctrl Pts',(-71.3655115898827,-1.29040921386059,
0.));
#84464=CARTESIAN_POINT('Ctrl Pts',(-71.3870012482499,-1.29807923821413,
0.));
#84465=CARTESIAN_POINT('Ctrl Pts',(-71.4085257029322,-1.30578599126139,
0.));
#84466=CARTESIAN_POINT('Ctrl Pts',(-71.4300848044087,-1.31352949116537,
0.));
#84467=CARTESIAN_POINT('Ctrl Pts',(-71.4516784038317,-1.32130975590226,
0.));
#84468=CARTESIAN_POINT('Ctrl Pts',(-71.4733063530187,-1.32912680326123,
0.));
#84469=CARTESIAN_POINT('Ctrl Pts',(-71.4949685044522,-1.33698065085219,
0.));
#84470=CARTESIAN_POINT('Ctrl Pts',(-71.516664711275,-1.3448713161078,0.));
#84471=CARTESIAN_POINT('Ctrl Pts',(-71.5383948272845,-1.35279881628455,
0.));
#84472=CARTESIAN_POINT('Ctrl Pts',(-71.5601587069217,-1.36076316845816,
0.));
#84473=CARTESIAN_POINT('Ctrl Pts',(-71.5819562052663,-1.36876438952465,
0.));
#84474=CARTESIAN_POINT('Ctrl Pts',(-71.6037871780385,-1.37680249620779,
0.));
#84475=CARTESIAN_POINT('Ctrl Pts',(-71.625651481593,-1.38487750506082,0.));
#84476=CARTESIAN_POINT('Ctrl Pts',(-71.6475489729134,-1.39298943246722,
0.));
#84477=CARTESIAN_POINT('Ctrl Pts',(-71.6694795096001,-1.40113829463576,
0.));
#84478=CARTESIAN_POINT('Ctrl Pts',(-71.6914429498663,-1.40932410760248,
0.));
#84479=CARTESIAN_POINT('Ctrl Pts',(-71.7134391525389,-1.41754688723773,
0.));
#84480=CARTESIAN_POINT('Ctrl Pts',(-71.7354679770528,-1.42580664924769,
0.));
#84481=CARTESIAN_POINT('Ctrl Pts',(-71.7575292834469,-1.43410340917495,
0.));
#84482=CARTESIAN_POINT('Ctrl Pts',(-71.7796229323526,-1.44243718239315,
0.));
#84483=CARTESIAN_POINT('Ctrl Pts',(-71.8017487849895,-1.45080798410965,
0.));
#84484=CARTESIAN_POINT('Ctrl Pts',(-71.8239067031683,-1.45921582937231,
0.));
#84485=CARTESIAN_POINT('Ctrl Pts',(-71.8460965492839,-1.46766073307088,
0.));
#84486=CARTESIAN_POINT('Ctrl Pts',(-71.8683181863116,-1.47614270993728,
0.));
#84487=CARTESIAN_POINT('Ctrl Pts',(-71.8905714777961,-1.48466177454019,
0.));
#84488=CARTESIAN_POINT('Ctrl Pts',(-71.912856287848,-1.49321794128798,0.));
#84489=CARTESIAN_POINT('Ctrl Pts',(-71.9351724811443,-1.50181122443534,
0.));
#84490=CARTESIAN_POINT('Ctrl Pts',(-71.9575199229241,-1.51044163808453,
0.));
#84491=CARTESIAN_POINT('Ctrl Pts',(-71.979898478983,-1.51910919618566,0.));
#84492=CARTESIAN_POINT('Ctrl Pts',(-72.0023080156647,-1.52781391253102,
0.));
#84493=CARTESIAN_POINT('Ctrl Pts',(-72.0247483998579,-1.53655580075812,
0.));
#84494=CARTESIAN_POINT('Ctrl Pts',(-72.0472194989963,-1.54533487435626,
0.));
#84495=CARTESIAN_POINT('Ctrl Pts',(-72.0697211810545,-1.55415114666773,
0.));
#84496=CARTESIAN_POINT('Ctrl Pts',(-72.0922533145433,-1.56300463088808,
0.));
#84497=CARTESIAN_POINT('Ctrl Pts',(-72.1148157684995,-1.5718953400604,0.));
#84498=CARTESIAN_POINT('Ctrl Pts',(-72.1374084124839,-1.58082328707803,
0.));
#84499=CARTESIAN_POINT('Ctrl Pts',(-72.1600311165821,-1.58978848469123,
0.));
#84500=CARTESIAN_POINT('Ctrl Pts',(-72.1826837514001,-1.59879094550847,
0.));
#84501=CARTESIAN_POINT('Ctrl Pts',(-72.2053661880608,-1.60783068199663,
0.));
#84502=CARTESIAN_POINT('Ctrl Pts',(-72.2280782981937,-1.6169077064754,0.));
#84503=CARTESIAN_POINT('Ctrl Pts',(-72.2508199539323,-1.6260220311193,0.));
#84504=CARTESIAN_POINT('Ctrl Pts',(-72.2735910279149,-1.63517366796463,
0.));
#84505=CARTESIAN_POINT('Ctrl Pts',(-72.2963913932813,-1.64436262891079,
0.));
#84506=CARTESIAN_POINT('Ctrl Pts',(-72.319220923669,-1.65358892572062,0.));
#84507=CARTESIAN_POINT('Ctrl Pts',(-72.3420794932047,-1.66285257001496,
0.));
#84508=CARTESIAN_POINT('Ctrl Pts',(-72.3649669765004,-1.67215357327365,
0.));
#84509=CARTESIAN_POINT('Ctrl Pts',(-72.387883248654,-1.68149194684281,0.));
#84510=CARTESIAN_POINT('Ctrl Pts',(-72.4108281852467,-1.69086770193637,
0.));
#84511=CARTESIAN_POINT('Ctrl Pts',(-72.4338016623391,-1.70028084963647,
0.));
#84512=CARTESIAN_POINT('Ctrl Pts',(-72.456803556463,-1.70973140088841,0.));
#84513=CARTESIAN_POINT('Ctrl Pts',(-72.479833744618,-1.71921936650038,0.));
#84514=CARTESIAN_POINT('Ctrl Pts',(-72.5028921042721,-1.72874475715103,
0.));
#84515=CARTESIAN_POINT('Ctrl Pts',(-72.5259785133595,-1.73830758339125,
0.));
#84516=CARTESIAN_POINT('Ctrl Pts',(-72.5490928502769,-1.74790785564473,
0.));
#84517=CARTESIAN_POINT('Ctrl Pts',(-72.5722349938774,-1.75754558420344,
0.));
#84518=CARTESIAN_POINT('Ctrl Pts',(-72.5954048234638,-1.76722077922574,
0.));
#84519=CARTESIAN_POINT('Ctrl Pts',(-72.6186022187907,-1.77693345074426,
0.));
#84520=CARTESIAN_POINT('Ctrl Pts',(-72.6418270600619,-1.78668360866811,
0.));
#84521=CARTESIAN_POINT('Ctrl Pts',(-72.6650792279274,-1.79647126278358,
0.));
#84522=CARTESIAN_POINT('Ctrl Pts',(-72.6883586034769,-1.8062964227505,0.));
#84523=CARTESIAN_POINT('Ctrl Pts',(-72.7116650682344,-1.81615909809871,
0.));
#84524=CARTESIAN_POINT('Ctrl Pts',(-72.7349985041592,-1.82605929823564,
0.));
#84525=CARTESIAN_POINT('Ctrl Pts',(-72.7583587936447,-1.83599703244924,
0.));
#84526=CARTESIAN_POINT('Ctrl Pts',(-72.7817458195155,-1.84597230990857,
0.));
#84527=CARTESIAN_POINT('Ctrl Pts',(-72.8051594650222,-1.85598513966113,
0.));
#84528=CARTESIAN_POINT('Ctrl Pts',(-72.8285996138359,-1.86603553062771,
0.));
#84529=CARTESIAN_POINT('Ctrl Pts',(-72.8520661500477,-1.87612349160944,
0.));
#84530=CARTESIAN_POINT('Ctrl Pts',(-72.875558958168,-1.88624903129188,0.));
#84531=CARTESIAN_POINT('Ctrl Pts',(-72.8990779231226,-1.89641215824582,
0.));
#84532=CARTESIAN_POINT('Ctrl Pts',(-72.9226229302478,-1.90661288092587,
0.));
#84533=CARTESIAN_POINT('Ctrl Pts',(-72.9461938652811,-1.91685120766436,
0.));
#84534=CARTESIAN_POINT('Ctrl Pts',(-72.9697906143636,-1.9271271466766,0.));
#84535=CARTESIAN_POINT('Ctrl Pts',(-72.9934130640415,-1.93744070606566,
0.));
#84536=CARTESIAN_POINT('Ctrl Pts',(-73.0170611012661,-1.94779189382302,
0.));
#84537=CARTESIAN_POINT('Ctrl Pts',(-73.040734613391,-1.95818071782767,0.));
#84538=CARTESIAN_POINT('Ctrl Pts',(-73.0644334881673,-1.96860718583932,
0.));
#84539=CARTESIAN_POINT('Ctrl Pts',(-73.0881576137407,-1.97907130550157,
0.));
#84540=CARTESIAN_POINT('Ctrl Pts',(-73.1119068786475,-1.98957308434918,
0.));
#84541=CARTESIAN_POINT('Ctrl Pts',(-73.1356811718091,-2.00011252980981,
0.));
#84542=CARTESIAN_POINT('Ctrl Pts',(-73.1594803825252,-2.01068964920467,
0.));
#84543=CARTESIAN_POINT('Ctrl Pts',(-73.183304400462,-2.02130444974362,0.));
#84544=CARTESIAN_POINT('Ctrl Pts',(-73.2071531156504,-2.03195693852454,
0.));
#84545=CARTESIAN_POINT('Ctrl Pts',(-73.2310264184976,-2.04264712253928,
0.));
#84546=CARTESIAN_POINT('Ctrl Pts',(-73.2549241997953,-2.05337500867403,
0.));
#84547=CARTESIAN_POINT('Ctrl Pts',(-73.2788463507246,-2.06414060370834,
0.));
#84548=CARTESIAN_POINT('Ctrl Pts',(-73.3027927628626,-2.07494391430941,
0.));
#84549=CARTESIAN_POINT('Ctrl Pts',(-73.3267633281807,-2.08578494702743,
0.));
#84550=CARTESIAN_POINT('Ctrl Pts',(-73.3507579390239,-2.09666370830716,
0.));
#84551=CARTESIAN_POINT('Ctrl Pts',(-73.3747764880893,-2.1075802044939,0.));
#84552=CARTESIAN_POINT('Ctrl Pts',(-73.3988188684021,-2.11853444183761,
0.));
#84553=CARTESIAN_POINT('Ctrl Pts',(-73.4228849732925,-2.12952642649367,
0.));
#84554=CARTESIAN_POINT('Ctrl Pts',(-73.4469746963637,-2.14055616452057,
0.));
#84555=CARTESIAN_POINT('Ctrl Pts',(-73.4710879315382,-2.15162366187906,
0.));
#84556=CARTESIAN_POINT('Ctrl Pts',(-73.4952245731054,-2.16272892442919,
0.));
#84557=CARTESIAN_POINT('Ctrl Pts',(-73.5193845157708,-2.17387195792306,
0.));
#84558=CARTESIAN_POINT('Ctrl Pts',(-73.5435676546929,-2.18505276799753,
0.));
#84559=CARTESIAN_POINT('Ctrl Pts',(-73.5677738855452,-2.19627136015678,
0.));
#84560=CARTESIAN_POINT('Ctrl Pts',(-73.5920031044595,-2.20752773978348,
0.));
#84561=CARTESIAN_POINT('Ctrl Pts',(-73.6162552079038,-2.21882191216518,
0.));
#84562=CARTESIAN_POINT('Ctrl Pts',(-73.6405300925712,-2.23015388251287,
0.));
#84563=CARTESIAN_POINT('Ctrl Pts',(-73.6648276552767,-2.24152365597697,
0.));
#84564=CARTESIAN_POINT('Ctrl Pts',(-73.6891477928129,-2.25293123766425,
0.));
#84565=CARTESIAN_POINT('Ctrl Pts',(-73.7134904019389,-2.26437663263667,
0.));
#84566=CARTESIAN_POINT('Ctrl Pts',(-73.7378553796807,-2.27585984587198,
0.));
#84567=CARTESIAN_POINT('Ctrl Pts',(-73.762242623566,-2.28738088222863,0.));
#84568=CARTESIAN_POINT('Ctrl Pts',(-73.786652031885,-2.29893974640434,0.));
#84569=CARTESIAN_POINT('Ctrl Pts',(-73.8110835039327,-2.31053644289416,
0.));
#84570=CARTESIAN_POINT('Ctrl Pts',(-73.8355369402706,-2.32217097594197,
0.));
#84571=CARTESIAN_POINT('Ctrl Pts',(-73.8600122421468,-2.33384334963957,
0.));
#84572=CARTESIAN_POINT('Ctrl Pts',(-73.8845093109274,-2.3455535680212,0.));
#84573=CARTESIAN_POINT('Ctrl Pts',(-73.9090280474712,-2.35730163516315,
0.));
#84574=CARTESIAN_POINT('Ctrl Pts',(-73.9335683516404,-2.36908755526003,
0.));
#84575=CARTESIAN_POINT('Ctrl Pts',(-73.958130121465,-2.3809113327496,0.));
#84576=CARTESIAN_POINT('Ctrl Pts',(-73.9827132538206,-2.39277297220756,
0.));
#84577=CARTESIAN_POINT('Ctrl Pts',(-74.0073176459344,-2.40467247811536,
0.));
#84578=CARTESIAN_POINT('Ctrl Pts',(-74.0319431966989,-2.41660985465251,
0.));
#84579=CARTESIAN_POINT('Ctrl Pts',(-74.0565898079218,-2.42858510549778,
0.));
#84580=CARTESIAN_POINT('Ctrl Pts',(-74.0812573859411,-2.44059823356675,
0.));
#84581=CARTESIAN_POINT('Ctrl Pts',(-74.1059458420067,-2.45264924094775,
0.));
#84582=CARTESIAN_POINT('Ctrl Pts',(-74.127126454519,-2.46301176097118,0.));
#84583=CARTESIAN_POINT('Ctrl Pts',(-74.143376394138,-2.47097695564993,0.));
#84584=CARTESIAN_POINT('Ctrl Pts',(-74.1546864735166,-2.47652804724537,
0.));
#84585=CARTESIAN_POINT('Ctrl Pts',(-74.1610506466206,-2.47965393945475,
0.));
#84586=CARTESIAN_POINT('Ctrl Pts',(-74.1624659714555,-2.48034921843229,
0.));
#84587=CARTESIAN_POINT('',(-69.9947925310006,-0.85382582660898,12.));
#84588=CARTESIAN_POINT('',(-69.9947925310006,-0.85382582660898,0.));
#84589=CARTESIAN_POINT('Ctrl Pts',(-74.1624659714555,-2.48034921843227,
12.));
#84590=CARTESIAN_POINT('Ctrl Pts',(-74.1610506466206,-2.47965393945474,
12.));
#84591=CARTESIAN_POINT('Ctrl Pts',(-74.1546864735166,-2.47652804724537,
12.));
#84592=CARTESIAN_POINT('Ctrl Pts',(-74.143376394138,-2.47097695564992,12.));
#84593=CARTESIAN_POINT('Ctrl Pts',(-74.127126454519,-2.46301176097117,12.));
#84594=CARTESIAN_POINT('Ctrl Pts',(-74.1059458420067,-2.45264924094775,
12.));
#84595=CARTESIAN_POINT('Ctrl Pts',(-74.0812573859411,-2.44059823356675,
12.));
#84596=CARTESIAN_POINT('Ctrl Pts',(-74.0565898079218,-2.42858510549778,
12.));
#84597=CARTESIAN_POINT('Ctrl Pts',(-74.0319431966989,-2.41660985465251,
12.));
#84598=CARTESIAN_POINT('Ctrl Pts',(-74.0073176459344,-2.40467247811536,
12.));
#84599=CARTESIAN_POINT('Ctrl Pts',(-73.9827132538206,-2.39277297220756,
12.));
#84600=CARTESIAN_POINT('Ctrl Pts',(-73.958130121465,-2.3809113327496,12.));
#84601=CARTESIAN_POINT('Ctrl Pts',(-73.9335683516404,-2.36908755526003,
12.));
#84602=CARTESIAN_POINT('Ctrl Pts',(-73.9090280474712,-2.35730163516315,
12.));
#84603=CARTESIAN_POINT('Ctrl Pts',(-73.8845093109274,-2.3455535680212,12.));
#84604=CARTESIAN_POINT('Ctrl Pts',(-73.8600122421468,-2.33384334963957,
12.));
#84605=CARTESIAN_POINT('Ctrl Pts',(-73.8355369402706,-2.32217097594197,
12.));
#84606=CARTESIAN_POINT('Ctrl Pts',(-73.8110835039327,-2.31053644289416,
12.));
#84607=CARTESIAN_POINT('Ctrl Pts',(-73.786652031885,-2.29893974640434,12.));
#84608=CARTESIAN_POINT('Ctrl Pts',(-73.762242623566,-2.28738088222863,12.));
#84609=CARTESIAN_POINT('Ctrl Pts',(-73.7378553796807,-2.27585984587198,
12.));
#84610=CARTESIAN_POINT('Ctrl Pts',(-73.7134904019389,-2.26437663263667,
12.));
#84611=CARTESIAN_POINT('Ctrl Pts',(-73.6891477928129,-2.25293123766425,
12.));
#84612=CARTESIAN_POINT('Ctrl Pts',(-73.6648276552767,-2.24152365597697,
12.));
#84613=CARTESIAN_POINT('Ctrl Pts',(-73.6405300925712,-2.23015388251287,
12.));
#84614=CARTESIAN_POINT('Ctrl Pts',(-73.6162552079038,-2.21882191216518,
12.));
#84615=CARTESIAN_POINT('Ctrl Pts',(-73.5920031044595,-2.20752773978348,
12.));
#84616=CARTESIAN_POINT('Ctrl Pts',(-73.5677738855452,-2.19627136015678,
12.));
#84617=CARTESIAN_POINT('Ctrl Pts',(-73.5435676546929,-2.18505276799753,
12.));
#84618=CARTESIAN_POINT('Ctrl Pts',(-73.5193845157708,-2.17387195792306,
12.));
#84619=CARTESIAN_POINT('Ctrl Pts',(-73.4952245731054,-2.16272892442919,
12.));
#84620=CARTESIAN_POINT('Ctrl Pts',(-73.4710879315382,-2.15162366187906,
12.));
#84621=CARTESIAN_POINT('Ctrl Pts',(-73.4469746963637,-2.14055616452057,
12.));
#84622=CARTESIAN_POINT('Ctrl Pts',(-73.4228849732925,-2.12952642649367,
12.));
#84623=CARTESIAN_POINT('Ctrl Pts',(-73.3988188684021,-2.11853444183761,
12.));
#84624=CARTESIAN_POINT('Ctrl Pts',(-73.3747764880893,-2.1075802044939,12.));
#84625=CARTESIAN_POINT('Ctrl Pts',(-73.3507579390239,-2.09666370830716,
12.));
#84626=CARTESIAN_POINT('Ctrl Pts',(-73.3267633281807,-2.08578494702743,
12.));
#84627=CARTESIAN_POINT('Ctrl Pts',(-73.3027927628626,-2.07494391430941,
12.));
#84628=CARTESIAN_POINT('Ctrl Pts',(-73.2788463507246,-2.06414060370834,
12.));
#84629=CARTESIAN_POINT('Ctrl Pts',(-73.2549241997953,-2.05337500867403,
12.));
#84630=CARTESIAN_POINT('Ctrl Pts',(-73.2310264184976,-2.04264712253928,
12.));
#84631=CARTESIAN_POINT('Ctrl Pts',(-73.2071531156504,-2.03195693852454,
12.));
#84632=CARTESIAN_POINT('Ctrl Pts',(-73.183304400462,-2.02130444974362,12.));
#84633=CARTESIAN_POINT('Ctrl Pts',(-73.1594803825252,-2.01068964920467,
12.));
#84634=CARTESIAN_POINT('Ctrl Pts',(-73.1356811718091,-2.00011252980981,
12.));
#84635=CARTESIAN_POINT('Ctrl Pts',(-73.1119068786475,-1.98957308434918,
12.));
#84636=CARTESIAN_POINT('Ctrl Pts',(-73.0881576137407,-1.97907130550157,
12.));
#84637=CARTESIAN_POINT('Ctrl Pts',(-73.0644334881673,-1.96860718583932,
12.));
#84638=CARTESIAN_POINT('Ctrl Pts',(-73.040734613391,-1.95818071782767,12.));
#84639=CARTESIAN_POINT('Ctrl Pts',(-73.0170611012661,-1.94779189382302,
12.));
#84640=CARTESIAN_POINT('Ctrl Pts',(-72.9934130640415,-1.93744070606566,
12.));
#84641=CARTESIAN_POINT('Ctrl Pts',(-72.9697906143636,-1.9271271466766,12.));
#84642=CARTESIAN_POINT('Ctrl Pts',(-72.9461938652811,-1.91685120766436,
12.));
#84643=CARTESIAN_POINT('Ctrl Pts',(-72.9226229302478,-1.90661288092587,
12.));
#84644=CARTESIAN_POINT('Ctrl Pts',(-72.8990779231226,-1.89641215824582,
12.));
#84645=CARTESIAN_POINT('Ctrl Pts',(-72.875558958168,-1.88624903129188,12.));
#84646=CARTESIAN_POINT('Ctrl Pts',(-72.8520661500477,-1.87612349160944,
12.));
#84647=CARTESIAN_POINT('Ctrl Pts',(-72.8285996138359,-1.86603553062771,
12.));
#84648=CARTESIAN_POINT('Ctrl Pts',(-72.8051594650222,-1.85598513966113,
12.));
#84649=CARTESIAN_POINT('Ctrl Pts',(-72.7817458195155,-1.84597230990857,
12.));
#84650=CARTESIAN_POINT('Ctrl Pts',(-72.7583587936447,-1.83599703244924,
12.));
#84651=CARTESIAN_POINT('Ctrl Pts',(-72.7349985041592,-1.82605929823564,
12.));
#84652=CARTESIAN_POINT('Ctrl Pts',(-72.7116650682344,-1.81615909809871,
12.));
#84653=CARTESIAN_POINT('Ctrl Pts',(-72.6883586034769,-1.8062964227505,12.));
#84654=CARTESIAN_POINT('Ctrl Pts',(-72.6650792279274,-1.79647126278358,
12.));
#84655=CARTESIAN_POINT('Ctrl Pts',(-72.6418270600619,-1.78668360866811,
12.));
#84656=CARTESIAN_POINT('Ctrl Pts',(-72.6186022187907,-1.77693345074426,
12.));
#84657=CARTESIAN_POINT('Ctrl Pts',(-72.5954048234638,-1.76722077922574,
12.));
#84658=CARTESIAN_POINT('Ctrl Pts',(-72.5722349938774,-1.75754558420344,
12.));
#84659=CARTESIAN_POINT('Ctrl Pts',(-72.5490928502769,-1.74790785564473,
12.));
#84660=CARTESIAN_POINT('Ctrl Pts',(-72.5259785133595,-1.73830758339125,
12.));
#84661=CARTESIAN_POINT('Ctrl Pts',(-72.5028921042721,-1.72874475715103,
12.));
#84662=CARTESIAN_POINT('Ctrl Pts',(-72.479833744618,-1.71921936650038,12.));
#84663=CARTESIAN_POINT('Ctrl Pts',(-72.456803556463,-1.70973140088841,12.));
#84664=CARTESIAN_POINT('Ctrl Pts',(-72.4338016623391,-1.70028084963647,
12.));
#84665=CARTESIAN_POINT('Ctrl Pts',(-72.4108281852467,-1.69086770193637,
12.));
#84666=CARTESIAN_POINT('Ctrl Pts',(-72.387883248654,-1.68149194684281,12.));
#84667=CARTESIAN_POINT('Ctrl Pts',(-72.3649669765004,-1.67215357327365,
12.));
#84668=CARTESIAN_POINT('Ctrl Pts',(-72.3420794932047,-1.66285257001496,
12.));
#84669=CARTESIAN_POINT('Ctrl Pts',(-72.319220923669,-1.65358892572062,12.));
#84670=CARTESIAN_POINT('Ctrl Pts',(-72.2963913932813,-1.64436262891079,
12.));
#84671=CARTESIAN_POINT('Ctrl Pts',(-72.2735910279149,-1.63517366796463,
12.));
#84672=CARTESIAN_POINT('Ctrl Pts',(-72.2508199539323,-1.6260220311193,12.));
#84673=CARTESIAN_POINT('Ctrl Pts',(-72.2280782981937,-1.6169077064754,12.));
#84674=CARTESIAN_POINT('Ctrl Pts',(-72.2053661880608,-1.60783068199663,
12.));
#84675=CARTESIAN_POINT('Ctrl Pts',(-72.1826837514001,-1.59879094550847,
12.));
#84676=CARTESIAN_POINT('Ctrl Pts',(-72.1600311165821,-1.58978848469123,
12.));
#84677=CARTESIAN_POINT('Ctrl Pts',(-72.1374084124839,-1.58082328707803,
12.));
#84678=CARTESIAN_POINT('Ctrl Pts',(-72.1148157684995,-1.5718953400604,12.));
#84679=CARTESIAN_POINT('Ctrl Pts',(-72.0922533145433,-1.56300463088808,
12.));
#84680=CARTESIAN_POINT('Ctrl Pts',(-72.0697211810545,-1.55415114666773,
12.));
#84681=CARTESIAN_POINT('Ctrl Pts',(-72.0472194989963,-1.54533487435626,
12.));
#84682=CARTESIAN_POINT('Ctrl Pts',(-72.0247483998579,-1.53655580075812,
12.));
#84683=CARTESIAN_POINT('Ctrl Pts',(-72.0023080156647,-1.52781391253102,
12.));
#84684=CARTESIAN_POINT('Ctrl Pts',(-71.979898478983,-1.51910919618566,12.));
#84685=CARTESIAN_POINT('Ctrl Pts',(-71.9575199229241,-1.51044163808453,
12.));
#84686=CARTESIAN_POINT('Ctrl Pts',(-71.9351724811443,-1.50181122443534,
12.));
#84687=CARTESIAN_POINT('Ctrl Pts',(-71.912856287848,-1.49321794128798,12.));
#84688=CARTESIAN_POINT('Ctrl Pts',(-71.8905714777961,-1.48466177454019,
12.));
#84689=CARTESIAN_POINT('Ctrl Pts',(-71.8683181863116,-1.47614270993728,
12.));
#84690=CARTESIAN_POINT('Ctrl Pts',(-71.8460965492839,-1.46766073307088,
12.));
#84691=CARTESIAN_POINT('Ctrl Pts',(-71.8239067031683,-1.45921582937231,
12.));
#84692=CARTESIAN_POINT('Ctrl Pts',(-71.8017487849895,-1.45080798410965,
12.));
#84693=CARTESIAN_POINT('Ctrl Pts',(-71.7796229323526,-1.44243718239315,
12.));
#84694=CARTESIAN_POINT('Ctrl Pts',(-71.7575292834469,-1.43410340917495,
12.));
#84695=CARTESIAN_POINT('Ctrl Pts',(-71.7354679770528,-1.42580664924769,
12.));
#84696=CARTESIAN_POINT('Ctrl Pts',(-71.7134391525389,-1.41754688723773,
12.));
#84697=CARTESIAN_POINT('Ctrl Pts',(-71.6914429498663,-1.40932410760248,
12.));
#84698=CARTESIAN_POINT('Ctrl Pts',(-71.6694795096001,-1.40113829463576,
12.));
#84699=CARTESIAN_POINT('Ctrl Pts',(-71.6475489729134,-1.39298943246722,
12.));
#84700=CARTESIAN_POINT('Ctrl Pts',(-71.625651481593,-1.38487750506082,12.));
#84701=CARTESIAN_POINT('Ctrl Pts',(-71.6037871780385,-1.37680249620779,
12.));
#84702=CARTESIAN_POINT('Ctrl Pts',(-71.5819562052663,-1.36876438952465,
12.));
#84703=CARTESIAN_POINT('Ctrl Pts',(-71.5601587069217,-1.36076316845816,
12.));
#84704=CARTESIAN_POINT('Ctrl Pts',(-71.5383948272845,-1.35279881628455,
12.));
#84705=CARTESIAN_POINT('Ctrl Pts',(-71.516664711275,-1.3448713161078,12.));
#84706=CARTESIAN_POINT('Ctrl Pts',(-71.4949685044522,-1.33698065085219,
12.));
#84707=CARTESIAN_POINT('Ctrl Pts',(-71.4733063530187,-1.32912680326123,
12.));
#84708=CARTESIAN_POINT('Ctrl Pts',(-71.4516784038317,-1.32130975590226,
12.));
#84709=CARTESIAN_POINT('Ctrl Pts',(-71.4300848044087,-1.31352949116537,
12.));
#84710=CARTESIAN_POINT('Ctrl Pts',(-71.4085257029322,-1.30578599126139,
12.));
#84711=CARTESIAN_POINT('Ctrl Pts',(-71.3870012482499,-1.29807923821413,
12.));
#84712=CARTESIAN_POINT('Ctrl Pts',(-71.3655115898827,-1.29040921386059,
12.));
#84713=CARTESIAN_POINT('Ctrl Pts',(-71.3440568780347,-1.28277589985471,
12.));
#84714=CARTESIAN_POINT('Ctrl Pts',(-71.3226372635996,-1.27517927766608,
12.));
#84715=CARTESIAN_POINT('Ctrl Pts',(-71.3012528981661,-1.26761932857724,
12.));
#84716=CARTESIAN_POINT('Ctrl Pts',(-71.2799039340175,-1.2600960336757,12.));
#84717=CARTESIAN_POINT('Ctrl Pts',(-71.2585905241406,-1.25260937385568,
12.));
#84718=CARTESIAN_POINT('Ctrl Pts',(-71.2373128222352,-1.24515932982112,
12.));
#84719=CARTESIAN_POINT('Ctrl Pts',(-71.2160709827191,-1.23774588208427,
12.));
#84720=CARTESIAN_POINT('Ctrl Pts',(-71.194865160732,-1.23036901096239,12.));
#84721=CARTESIAN_POINT('Ctrl Pts',(-71.1736955121362,-1.22302869657017,
12.));
#84722=CARTESIAN_POINT('Ctrl Pts',(-71.1525621935267,-1.21572491882262,
12.));
#84723=CARTESIAN_POINT('Ctrl Pts',(-71.1314653622442,-1.20845765743647,
12.));
#84724=CARTESIAN_POINT('Ctrl Pts',(-71.1104051763839,-1.20122689192836,
12.));
#84725=CARTESIAN_POINT('Ctrl Pts',(-71.089381794801,-1.19403260161002,12.));
#84726=CARTESIAN_POINT('Ctrl Pts',(-71.0683953771149,-1.18687476558133,
12.));
#84727=CARTESIAN_POINT('Ctrl Pts',(-71.0474460837159,-1.17975336273504,
12.));
#84728=CARTESIAN_POINT('Ctrl Pts',(-71.0265340757699,-1.17266837175777,
12.));
#84729=CARTESIAN_POINT('Ctrl Pts',(-71.0056595152204,-1.1656197711288,12.));
#84730=CARTESIAN_POINT('Ctrl Pts',(-70.9848225647871,-1.15860753911485,
12.));
#84731=CARTESIAN_POINT('Ctrl Pts',(-70.9640233879659,-1.15163165376524,
12.));
#84732=CARTESIAN_POINT('Ctrl Pts',(-70.9432621490566,-1.14469209291488,
12.));
#84733=CARTESIAN_POINT('Ctrl Pts',(-70.9225390131826,-1.13778883418213,
12.));
#84734=CARTESIAN_POINT('Ctrl Pts',(-70.9018541463089,-1.13092185496564,
12.));
#84735=CARTESIAN_POINT('Ctrl Pts',(-70.8812077152586,-1.12409113243513,
12.));
#84736=CARTESIAN_POINT('Ctrl Pts',(-70.8605998877149,-1.11729664352992,
12.));
#84737=CARTESIAN_POINT('Ctrl Pts',(-70.8400308322037,-1.11053836496639,
12.));
#84738=CARTESIAN_POINT('Ctrl Pts',(-70.8195007180745,-1.10381627323946,
12.));
#84739=CARTESIAN_POINT('Ctrl Pts',(-70.799009715484,-1.09713034462265,12.));
#84740=CARTESIAN_POINT('Ctrl Pts',(-70.7785579953583,-1.09048055516426,
12.));
#84741=CARTESIAN_POINT('Ctrl Pts',(-70.7581457294447,-1.08386688068342,
12.));
#84742=CARTESIAN_POINT('Ctrl Pts',(-70.7377730903953,-1.07728929676408,
12.));
#84743=CARTESIAN_POINT('Ctrl Pts',(-70.7174402518378,-1.07074777874595,
12.));
#84744=CARTESIAN_POINT('Ctrl Pts',(-70.6971473884459,-1.0642423017128,12.));
#84745=CARTESIAN_POINT('Ctrl Pts',(-70.676894676009,-1.0577728404773,12.));
#84746=CARTESIAN_POINT('Ctrl Pts',(-70.6566822912991,-1.05133936960071,
12.));
#84747=CARTESIAN_POINT('Ctrl Pts',(-70.6365104119252,-1.04494186341156,
12.));
#84748=CARTESIAN_POINT('Ctrl Pts',(-70.6163792162073,-1.03858029601903,
12.));
#84749=CARTESIAN_POINT('Ctrl Pts',(-70.5962888829934,-1.0322546413287,12.));
#84750=CARTESIAN_POINT('Ctrl Pts',(-70.5762395916377,-1.02596487304048,
12.));
#84751=CARTESIAN_POINT('Ctrl Pts',(-70.556231522419,-1.01971096460597,12.));
#84752=CARTESIAN_POINT('Ctrl Pts',(-70.5362648569061,-1.01349288918537,
12.));
#84753=CARTESIAN_POINT('Ctrl Pts',(-70.5163397782713,-1.00731061960968,
12.));
#84754=CARTESIAN_POINT('Ctrl Pts',(-70.4964564717953,-1.00116412831442,
12.));
#84755=CARTESIAN_POINT('Ctrl Pts',(-70.4766151245212,-0.995053387379752,
12.));
#84756=CARTESIAN_POINT('Ctrl Pts',(-70.4568159243163,-0.988978368643646,
12.));
#84757=CARTESIAN_POINT('Ctrl Pts',(-70.4370590590842,-0.982939043792151,
12.));
#84758=CARTESIAN_POINT('Ctrl Pts',(-70.417344715957,-0.976935384450037,
12.));
#84759=CARTESIAN_POINT('Ctrl Pts',(-70.3976730803614,-0.970967362281171,
12.));
#84760=CARTESIAN_POINT('Ctrl Pts',(-70.3780443377956,-0.965034948786444,
12.));
#84761=CARTESIAN_POINT('Ctrl Pts',(-70.3584586759536,-0.959138115058827,
12.));
#84762=CARTESIAN_POINT('Ctrl Pts',(-70.338916286458,-0.953276831581238,
12.));
#84763=CARTESIAN_POINT('Ctrl Pts',(-70.3194173673674,-0.9474510679296,12.));
#84764=CARTESIAN_POINT('Ctrl Pts',(-70.299962123399,-0.941660792742975,
12.));
#84765=CARTESIAN_POINT('Ctrl Pts',(-70.2805507606872,-0.935905974336476,
12.));
#84766=CARTESIAN_POINT('Ctrl Pts',(-70.2611834821724,-0.930186581235545,
12.));
#84767=CARTESIAN_POINT('Ctrl Pts',(-70.2418604835837,-0.924502582639452,
12.));
#84768=CARTESIAN_POINT('Ctrl Pts',(-70.2225819470248,-0.918853949157115,
12.));
#84769=CARTESIAN_POINT('Ctrl Pts',(-70.2033480471676,-0.913240652090975,
12.));
#84770=CARTESIAN_POINT('Ctrl Pts',(-70.1841589635574,-0.907662662015781,
12.));
#84771=CARTESIAN_POINT('Ctrl Pts',(-70.1650148905109,-0.902119947629767,
12.));
#84772=CARTESIAN_POINT('Ctrl Pts',(-70.1459160490446,-0.89661247437184,
12.));
#84773=CARTESIAN_POINT('Ctrl Pts',(-70.1268626950175,-0.891140203464239,
12.));
#84774=CARTESIAN_POINT('Ctrl Pts',(-70.1078550938958,-0.885703094802532,
12.));
#84775=CARTESIAN_POINT('Ctrl Pts',(-70.0888934967855,-0.880301109660725,
12.));
#84776=CARTESIAN_POINT('Ctrl Pts',(-70.0699781183935,-0.874934213255836,
12.));
#84777=CARTESIAN_POINT('Ctrl Pts',(-70.051109108301,-0.86960237787112,12.));
#84778=CARTESIAN_POINT('Ctrl Pts',(-70.0322865492925,-0.864305583661541,
12.));
#84779=CARTESIAN_POINT('Ctrl Pts',(-70.0172656933806,-0.860096170668732,
12.));
#84780=CARTESIAN_POINT('Ctrl Pts',(-70.0060209754087,-0.856954870259201,
12.));
#84781=CARTESIAN_POINT('Ctrl Pts',(-69.9985337959407,-0.854867673848592,
12.));
#84782=CARTESIAN_POINT('Ctrl Pts',(-69.9947925310006,-0.85382582660898,
12.));
#84783=CARTESIAN_POINT('Ctrl Pts',(-74.0964320766209,-3.99277406490865,
-5.55111512312578E-16));
#84784=CARTESIAN_POINT('Ctrl Pts',(-74.0964320766209,-3.99277406490865,
4.));
#84785=CARTESIAN_POINT('Ctrl Pts',(-74.0964320766209,-3.99277406490865,
8.));
#84786=CARTESIAN_POINT('Ctrl Pts',(-74.0964320766209,-3.99277406490865,
12.));
#84787=CARTESIAN_POINT('Ctrl Pts',(-74.1989040313894,-3.95310474582224,
-5.55111512312578E-16));
#84788=CARTESIAN_POINT('Ctrl Pts',(-74.1989040313894,-3.95310474582224,
3.99999999999999));
#84789=CARTESIAN_POINT('Ctrl Pts',(-74.1989040313895,-3.95310474582224,
8.));
#84790=CARTESIAN_POINT('Ctrl Pts',(-74.1989040313895,-3.95310474582224,
12.));
#84791=CARTESIAN_POINT('Ctrl Pts',(-74.3538917248567,-3.82252142018526,
-5.55111512312578E-16));
#84792=CARTESIAN_POINT('Ctrl Pts',(-74.3538917248567,-3.82252142018526,
4.00000000000001));
#84793=CARTESIAN_POINT('Ctrl Pts',(-74.3538917248567,-3.82252142018526,
7.99999999999998));
#84794=CARTESIAN_POINT('Ctrl Pts',(-74.3538917248567,-3.82252142018526,
12.));
#84795=CARTESIAN_POINT('Ctrl Pts',(-74.41142867521,-3.63264011802866,-5.55111512312578E-16));
#84796=CARTESIAN_POINT('Ctrl Pts',(-74.41142867521,-3.63264011802866,3.99999999999999));
#84797=CARTESIAN_POINT('Ctrl Pts',(-74.41142867521,-3.63264011802866,8.00000000000001));
#84798=CARTESIAN_POINT('Ctrl Pts',(-74.41142867521,-3.63264011802866,12.));
#84799=CARTESIAN_POINT('Ctrl Pts',(-74.4153560388999,-3.55032190142802,
-5.55111512312578E-16));
#84800=CARTESIAN_POINT('Ctrl Pts',(-74.4153560388999,-3.55032190142802,
4.));
#84801=CARTESIAN_POINT('Ctrl Pts',(-74.4153560388999,-3.55032190142802,
8.));
#84802=CARTESIAN_POINT('Ctrl Pts',(-74.4153560388999,-3.55032190142802,
12.));
#84803=CARTESIAN_POINT('',(-74.0964320766209,-3.99277406490865,0.));
#84804=CARTESIAN_POINT('',(-74.4153560388999,-3.55032190142802,-2.77555756156289E-16));
#84805=CARTESIAN_POINT('Ctrl Pts',(-74.0964320766209,-3.99277406490865,
-1.23259516440783E-31));
#84806=CARTESIAN_POINT('Ctrl Pts',(-74.1989040313894,-3.95310474582224,
-8.16594296420187E-31));
#84807=CARTESIAN_POINT('Ctrl Pts',(-74.2874684276565,-3.87848570260111,
3.85185988877447E-31));
#84808=CARTESIAN_POINT('Ctrl Pts',(-74.3442121731107,-3.78450405480215,
1.54074395550979E-31));
#84809=CARTESIAN_POINT('Ctrl Pts',(-74.3867699822014,-3.71401781895292,
-3.08148791101957E-32));
#84810=CARTESIAN_POINT('Ctrl Pts',(-74.41142867521,-3.63264011802866,-1.07852076885685E-30));
#84811=CARTESIAN_POINT('Ctrl Pts',(-74.4153560388999,-3.55032190142802,
-7.70371977754892E-32));
#84812=CARTESIAN_POINT('',(-74.4153560388999,-3.55032190142802,12.));
#84813=CARTESIAN_POINT('Ctrl Pts',(-74.4153560388999,-3.55032190142802,
-5.55111512312578E-16));
#84814=CARTESIAN_POINT('Ctrl Pts',(-74.4153560388999,-3.55032190142802,
4.));
#84815=CARTESIAN_POINT('Ctrl Pts',(-74.4153560388999,-3.55032190142802,
8.));
#84816=CARTESIAN_POINT('Ctrl Pts',(-74.4153560388999,-3.55032190142802,
12.));
#84817=CARTESIAN_POINT('',(-74.0964320766209,-3.99277406490864,12.));
#84818=CARTESIAN_POINT('Ctrl Pts',(-74.4153560388999,-3.55032190142802,
12.));
#84819=CARTESIAN_POINT('Ctrl Pts',(-74.41142867521,-3.63264011802866,12.));
#84820=CARTESIAN_POINT('Ctrl Pts',(-74.3867699822014,-3.71401781895292,
12.));
#84821=CARTESIAN_POINT('Ctrl Pts',(-74.3442121731107,-3.78450405480214,
12.));
#84822=CARTESIAN_POINT('Ctrl Pts',(-74.2874684276565,-3.87848570260111,
12.));
#84823=CARTESIAN_POINT('Ctrl Pts',(-74.1989040313895,-3.95310474582224,
12.));
#84824=CARTESIAN_POINT('Ctrl Pts',(-74.0964320766209,-3.99277406490865,
12.));
#84825=CARTESIAN_POINT('Ctrl Pts',(-74.0964320766209,-3.99277406490865,
12.));
#84826=CARTESIAN_POINT('Ctrl Pts',(-74.0964320766209,-3.99277406490865,
8.));
#84827=CARTESIAN_POINT('Ctrl Pts',(-74.0964320766209,-3.99277406490865,
4.));
#84828=CARTESIAN_POINT('Ctrl Pts',(-74.0964320766209,-3.99277406490865,
-5.55111512312578E-16));
#84829=CARTESIAN_POINT('Origin',(-3.74482667098164E-10,-1.64496194443586E-11,
0.));
#84830=CARTESIAN_POINT('Origin',(-3.74482667098164E-10,-1.64496194443586E-11,
12.));
#84831=CARTESIAN_POINT('Origin',(-3.74482667098164E-10,-1.64496194443586E-11,
0.));
#84832=CARTESIAN_POINT('Ctrl Pts',(-74.4153560389001,3.55032190142523,0.));
#84833=CARTESIAN_POINT('Ctrl Pts',(-74.4153560389001,3.55032190142523,4.));
#84834=CARTESIAN_POINT('Ctrl Pts',(-74.4153560389001,3.55032190142524,8.));
#84835=CARTESIAN_POINT('Ctrl Pts',(-74.4153560389001,3.55032190142524,12.));
#84836=CARTESIAN_POINT('Ctrl Pts',(-74.4101195539797,3.66007952356786,0.));
#84837=CARTESIAN_POINT('Ctrl Pts',(-74.4101195539797,3.66007952356786,4.));
#84838=CARTESIAN_POINT('Ctrl Pts',(-74.4101195539797,3.66007952356787,8.00000000000001));
#84839=CARTESIAN_POINT('Ctrl Pts',(-74.4101195539797,3.66007952356787,12.));
#84840=CARTESIAN_POINT('Ctrl Pts',(-74.3352361483148,3.84840282419241,-7.30790067565468E-17));
#84841=CARTESIAN_POINT('Ctrl Pts',(-74.3352361483148,3.84840282419241,4.));
#84842=CARTESIAN_POINT('Ctrl Pts',(-74.3352361483148,3.84840282419244,7.99999999999999));
#84843=CARTESIAN_POINT('Ctrl Pts',(-74.3352361483148,3.84840282419244,12.));
#84844=CARTESIAN_POINT('Ctrl Pts',(-74.1732860426647,3.96302207561163,-2.46611180232189E-16));
#84845=CARTESIAN_POINT('Ctrl Pts',(-74.1732860426647,3.96302207561163,4.));
#84846=CARTESIAN_POINT('Ctrl Pts',(-74.1732860426647,3.96302207561166,8.00000000000001));
#84847=CARTESIAN_POINT('Ctrl Pts',(-74.1732860426647,3.96302207561166,12.));
#84848=CARTESIAN_POINT('Ctrl Pts',(-74.0964320765798,3.99277406492194,-3.30265160469534E-16));
#84849=CARTESIAN_POINT('Ctrl Pts',(-74.0964320765798,3.99277406492194,4.));
#84850=CARTESIAN_POINT('Ctrl Pts',(-74.0964320765798,3.99277406492197,8.));
#84851=CARTESIAN_POINT('Ctrl Pts',(-74.0964320765798,3.99277406492197,12.));
#84852=CARTESIAN_POINT('',(-74.4153560389001,3.55032190142523,0.));
#84853=CARTESIAN_POINT('',(-74.0964320765797,3.9927740649218,0.));
#84854=CARTESIAN_POINT('Ctrl Pts',(-74.4153560389001,3.55032190142523,2.74425517504379E-17));
#84855=CARTESIAN_POINT('Ctrl Pts',(-74.4101195539797,3.66007952356786,2.74425517504379E-17));
#84856=CARTESIAN_POINT('Ctrl Pts',(-74.3673290364569,3.76769283821046,-1.43168806818745E-17));
#84857=CARTESIAN_POINT('Ctrl Pts',(-74.2961085760818,3.85123952454111,-8.88773471449119E-17));
#84858=CARTESIAN_POINT('Ctrl Pts',(-74.2426932308005,3.91389953928911,-1.4479769699219E-16));
#84859=CARTESIAN_POINT('Ctrl Pts',(-74.1732860426647,3.96302207561163,-2.19168628481751E-16));
#84860=CARTESIAN_POINT('Ctrl Pts',(-74.0964320765798,3.99277406492194,-3.02822608719096E-16));
#84861=CARTESIAN_POINT('',(-74.0964320765797,3.99277406492181,12.));
#84862=CARTESIAN_POINT('Ctrl Pts',(-74.0964320765798,3.99277406492194,-3.30265160469534E-16));
#84863=CARTESIAN_POINT('Ctrl Pts',(-74.0964320765798,3.99277406492194,4.));
#84864=CARTESIAN_POINT('Ctrl Pts',(-74.0964320765798,3.99277406492197,8.));
#84865=CARTESIAN_POINT('Ctrl Pts',(-74.0964320765798,3.99277406492197,12.));
#84866=CARTESIAN_POINT('',(-74.4153560389001,3.55032190142524,12.));
#84867=CARTESIAN_POINT('Ctrl Pts',(-74.0964320765798,3.99277406492197,12.));
#84868=CARTESIAN_POINT('Ctrl Pts',(-74.1732860426647,3.96302207561166,12.));
#84869=CARTESIAN_POINT('Ctrl Pts',(-74.2426932308005,3.91389953928914,12.));
#84870=CARTESIAN_POINT('Ctrl Pts',(-74.2961085760818,3.85123952454114,12.));
#84871=CARTESIAN_POINT('Ctrl Pts',(-74.3673290364569,3.76769283821048,12.));
#84872=CARTESIAN_POINT('Ctrl Pts',(-74.4101195539797,3.66007952356787,12.));
#84873=CARTESIAN_POINT('Ctrl Pts',(-74.4153560389001,3.55032190142524,12.));
#84874=CARTESIAN_POINT('Ctrl Pts',(-74.4153560389001,3.55032190142524,12.));
#84875=CARTESIAN_POINT('Ctrl Pts',(-74.4153560389001,3.55032190142524,8.));
#84876=CARTESIAN_POINT('Ctrl Pts',(-74.4153560389001,3.55032190142523,4.));
#84877=CARTESIAN_POINT('Ctrl Pts',(-74.4153560389001,3.55032190142523,0.));
#84878=CARTESIAN_POINT('Ctrl Pts',(-69.8028570375097,5.24987136994592,0.));
#84879=CARTESIAN_POINT('Ctrl Pts',(-69.8028570375097,5.24987136994592,12.));
#84880=CARTESIAN_POINT('Ctrl Pts',(-69.8066748687772,5.24915955997427,0.));
#84881=CARTESIAN_POINT('Ctrl Pts',(-69.8066748687772,5.24915955997427,12.));
#84882=CARTESIAN_POINT('Ctrl Pts',(-69.8143154684204,5.24773285666376,0.));
#84883=CARTESIAN_POINT('Ctrl Pts',(-69.8143154684204,5.24773285666376,12.));
#84884=CARTESIAN_POINT('Ctrl Pts',(-69.8257911792159,5.2455835515975,0.));
#84885=CARTESIAN_POINT('Ctrl Pts',(-69.8257911792159,5.2455835515975,12.));
#84886=CARTESIAN_POINT('Ctrl Pts',(-69.841121750752,5.24269931054569,0.));
#84887=CARTESIAN_POINT('Ctrl Pts',(-69.841121750752,5.24269931054569,12.));
#84888=CARTESIAN_POINT('Ctrl Pts',(-69.8603343302743,5.23906316634802,0.));
#84889=CARTESIAN_POINT('Ctrl Pts',(-69.8603343302743,5.23906316634802,12.));
#84890=CARTESIAN_POINT('Ctrl Pts',(-69.8795962381599,5.2353961627962,0.));
#84891=CARTESIAN_POINT('Ctrl Pts',(-69.8795962381599,5.2353961627962,12.));
#84892=CARTESIAN_POINT('Ctrl Pts',(-69.8989073936688,5.23169827290555,0.));
#84893=CARTESIAN_POINT('Ctrl Pts',(-69.8989073936688,5.23169827290555,12.));
#84894=CARTESIAN_POINT('Ctrl Pts',(-69.9182676502048,5.22796945602793,0.));
#84895=CARTESIAN_POINT('Ctrl Pts',(-69.9182676502048,5.22796945602793,12.));
#84896=CARTESIAN_POINT('Ctrl Pts',(-69.9376767969095,5.22420965879981,0.));
#84897=CARTESIAN_POINT('Ctrl Pts',(-69.9376767969095,5.22420965879981,12.));
#84898=CARTESIAN_POINT('Ctrl Pts',(-69.9571345870076,5.2204188207572,0.));
#84899=CARTESIAN_POINT('Ctrl Pts',(-69.9571345870076,5.2204188207572,12.));
#84900=CARTESIAN_POINT('Ctrl Pts',(-69.9766407595385,5.21659687881139,0.));
#84901=CARTESIAN_POINT('Ctrl Pts',(-69.9766407595385,5.21659687881139,12.));
#84902=CARTESIAN_POINT('Ctrl Pts',(-69.9961950629965,5.21274377203259,0.));
#84903=CARTESIAN_POINT('Ctrl Pts',(-69.9961950629965,5.21274377203259,12.));
#84904=CARTESIAN_POINT('Ctrl Pts',(-70.0157972802182,5.20885944672836,0.));
#84905=CARTESIAN_POINT('Ctrl Pts',(-70.0157972802182,5.20885944672836,12.));
#84906=CARTESIAN_POINT('Ctrl Pts',(-70.0354472203546,5.20494385478025,0.));
#84907=CARTESIAN_POINT('Ctrl Pts',(-70.0354472203546,5.20494385478025,12.));
#84908=CARTESIAN_POINT('Ctrl Pts',(-70.0551447071082,5.20099695122656,0.));
#84909=CARTESIAN_POINT('Ctrl Pts',(-70.0551447071082,5.20099695122656,12.));
#84910=CARTESIAN_POINT('Ctrl Pts',(-70.0748895689729,5.19701869225528,0.));
#84911=CARTESIAN_POINT('Ctrl Pts',(-70.0748895689729,5.19701869225528,12.));
#84912=CARTESIAN_POINT('Ctrl Pts',(-70.0946816270997,5.19300903271579,0.));
#84913=CARTESIAN_POINT('Ctrl Pts',(-70.0946816270997,5.19300903271579,12.));
#84914=CARTESIAN_POINT('Ctrl Pts',(-70.1145206891885,5.18896792486565,0.));
#84915=CARTESIAN_POINT('Ctrl Pts',(-70.1145206891885,5.18896792486565,12.));
#84916=CARTESIAN_POINT('Ctrl Pts',(-70.1344065558145,5.18489531966264,0.));
#84917=CARTESIAN_POINT('Ctrl Pts',(-70.1344065558145,5.18489531966264,12.));
#84918=CARTESIAN_POINT('Ctrl Pts',(-70.1543390243892,5.18079116757666,0.));
#84919=CARTESIAN_POINT('Ctrl Pts',(-70.1543390243892,5.18079116757666,12.));
#84920=CARTESIAN_POINT('Ctrl Pts',(-70.1743178937077,5.17665541952382,0.));
#84921=CARTESIAN_POINT('Ctrl Pts',(-70.1743178937077,5.17665541952382,12.));
#84922=CARTESIAN_POINT('Ctrl Pts',(-70.1943429691167,5.17248802793389,0.));
#84923=CARTESIAN_POINT('Ctrl Pts',(-70.1943429691167,5.17248802793389,12.));
#84924=CARTESIAN_POINT('Ctrl Pts',(-70.2144140622953,5.16828894670108,0.));
#84925=CARTESIAN_POINT('Ctrl Pts',(-70.2144140622953,5.16828894670108,12.));
#84926=CARTESIAN_POINT('Ctrl Pts',(-70.2345309887833,5.16405813066976,0.));
#84927=CARTESIAN_POINT('Ctrl Pts',(-70.2345309887833,5.16405813066976,12.));
#84928=CARTESIAN_POINT('Ctrl Pts',(-70.2546935662722,5.15979553528203,0.));
#84929=CARTESIAN_POINT('Ctrl Pts',(-70.2546935662722,5.15979553528203,12.));
#84930=CARTESIAN_POINT('Ctrl Pts',(-70.2749016125105,5.15550111614859,0.));
#84931=CARTESIAN_POINT('Ctrl Pts',(-70.2749016125105,5.15550111614859,12.));
#84932=CARTESIAN_POINT('Ctrl Pts',(-70.2951549435512,5.15117482869254,0.));
#84933=CARTESIAN_POINT('Ctrl Pts',(-70.2951549435512,5.15117482869254,12.));
#84934=CARTESIAN_POINT('Ctrl Pts',(-70.3154533746736,5.1468166283308,0.));
#84935=CARTESIAN_POINT('Ctrl Pts',(-70.3154533746736,5.1468166283308,12.));
#84936=CARTESIAN_POINT('Ctrl Pts',(-70.3357967211796,5.14242647063479,0.));
#84937=CARTESIAN_POINT('Ctrl Pts',(-70.3357967211796,5.14242647063479,12.));
#84938=CARTESIAN_POINT('Ctrl Pts',(-70.3561847991714,5.13800431148903,0.));
#84939=CARTESIAN_POINT('Ctrl Pts',(-70.3561847991714,5.13800431148903,12.));
#84940=CARTESIAN_POINT('Ctrl Pts',(-70.3766174264757,5.13355010728567,0.));
#84941=CARTESIAN_POINT('Ctrl Pts',(-70.3766174264757,5.13355010728567,12.));
#84942=CARTESIAN_POINT('Ctrl Pts',(-70.3970944229851,5.12906381499456,0.));
#84943=CARTESIAN_POINT('Ctrl Pts',(-70.3970944229851,5.12906381499456,12.));
#84944=CARTESIAN_POINT('Ctrl Pts',(-70.417615610161,5.12454539205328,0.));
#84945=CARTESIAN_POINT('Ctrl Pts',(-70.417615610161,5.12454539205328,12.));
#84946=CARTESIAN_POINT('Ctrl Pts',(-70.4381808107245,5.11999479630211,0.));
#84947=CARTESIAN_POINT('Ctrl Pts',(-70.4381808107245,5.11999479630211,12.));
#84948=CARTESIAN_POINT('Ctrl Pts',(-70.458789848296,5.11541198590932,0.));
#84949=CARTESIAN_POINT('Ctrl Pts',(-70.458789848296,5.11541198590932,12.));
#84950=CARTESIAN_POINT('Ctrl Pts',(-70.4794425469825,5.11079691929213,0.));
#84951=CARTESIAN_POINT('Ctrl Pts',(-70.4794425469825,5.11079691929213,12.));
#84952=CARTESIAN_POINT('Ctrl Pts',(-70.500138731399,5.10614955511663,0.));
#84953=CARTESIAN_POINT('Ctrl Pts',(-70.500138731399,5.10614955511663,12.));
#84954=CARTESIAN_POINT('Ctrl Pts',(-70.5208782268497,5.1014698523294,0.));
#84955=CARTESIAN_POINT('Ctrl Pts',(-70.5208782268497,5.1014698523294,12.));
#84956=CARTESIAN_POINT('Ctrl Pts',(-70.5416608594526,5.09675777018182,0.));
#84957=CARTESIAN_POINT('Ctrl Pts',(-70.5416608594526,5.09675777018182,12.));
#84958=CARTESIAN_POINT('Ctrl Pts',(-70.5624864562824,5.09201326826134,0.));
#84959=CARTESIAN_POINT('Ctrl Pts',(-70.5624864562824,5.09201326826134,12.));
#84960=CARTESIAN_POINT('Ctrl Pts',(-70.5833548455014,5.08723630652272,0.));
#84961=CARTESIAN_POINT('Ctrl Pts',(-70.5833548455014,5.08723630652272,12.));
#84962=CARTESIAN_POINT('Ctrl Pts',(-70.6042658562923,5.08242684526686,0.));
#84963=CARTESIAN_POINT('Ctrl Pts',(-70.6042658562923,5.08242684526686,12.));
#84964=CARTESIAN_POINT('Ctrl Pts',(-70.6252193187878,5.07758484512302,0.));
#84965=CARTESIAN_POINT('Ctrl Pts',(-70.6252193187878,5.07758484512302,12.));
#84966=CARTESIAN_POINT('Ctrl Pts',(-70.6462150640015,5.07271026703354,0.));
#84967=CARTESIAN_POINT('Ctrl Pts',(-70.6462150640015,5.07271026703354,12.));
#84968=CARTESIAN_POINT('Ctrl Pts',(-70.6672529237455,5.06780307224071,0.));
#84969=CARTESIAN_POINT('Ctrl Pts',(-70.6672529237455,5.06780307224071,12.));
#84970=CARTESIAN_POINT('Ctrl Pts',(-70.6883327305784,5.06286322227819,0.));
#84971=CARTESIAN_POINT('Ctrl Pts',(-70.6883327305784,5.06286322227819,12.));
#84972=CARTESIAN_POINT('Ctrl Pts',(-70.7094543178438,5.05789067897057,0.));
#84973=CARTESIAN_POINT('Ctrl Pts',(-70.7094543178438,5.05789067897057,12.));
#84974=CARTESIAN_POINT('Ctrl Pts',(-70.7306175196863,5.05288540443482,0.));
#84975=CARTESIAN_POINT('Ctrl Pts',(-70.7306175196863,5.05288540443482,12.));
#84976=CARTESIAN_POINT('Ctrl Pts',(-70.7518221710706,5.04784736108346,0.));
#84977=CARTESIAN_POINT('Ctrl Pts',(-70.7518221710706,5.04784736108346,12.));
#84978=CARTESIAN_POINT('Ctrl Pts',(-70.7730681077983,5.04277651163349,0.));
#84979=CARTESIAN_POINT('Ctrl Pts',(-70.7730681077983,5.04277651163349,12.));
#84980=CARTESIAN_POINT('Ctrl Pts',(-70.7943551665059,5.03767281910479,0.));
#84981=CARTESIAN_POINT('Ctrl Pts',(-70.7943551665059,5.03767281910479,12.));
#84982=CARTESIAN_POINT('Ctrl Pts',(-70.8156831846488,5.0325362468094,0.));
#84983=CARTESIAN_POINT('Ctrl Pts',(-70.8156831846488,5.0325362468094,12.));
#84984=CARTESIAN_POINT('Ctrl Pts',(-70.8370520004843,5.02736675834692,0.));
#84985=CARTESIAN_POINT('Ctrl Pts',(-70.8370520004843,5.02736675834692,12.));
#84986=CARTESIAN_POINT('Ctrl Pts',(-70.8584614530519,5.0221643176006,0.));
#84987=CARTESIAN_POINT('Ctrl Pts',(-70.8584614530519,5.0221643176006,12.));
#84988=CARTESIAN_POINT('Ctrl Pts',(-70.8799113821452,5.0169288887379,0.));
#84989=CARTESIAN_POINT('Ctrl Pts',(-70.8799113821452,5.0169288887379,12.));
#84990=CARTESIAN_POINT('Ctrl Pts',(-70.9014016283124,5.01166043620567,0.));
#84991=CARTESIAN_POINT('Ctrl Pts',(-70.9014016283124,5.01166043620567,12.));
#84992=CARTESIAN_POINT('Ctrl Pts',(-70.9229320328589,5.00635892472513,0.));
#84993=CARTESIAN_POINT('Ctrl Pts',(-70.9229320328589,5.00635892472513,12.));
#84994=CARTESIAN_POINT('Ctrl Pts',(-70.9445024378439,5.00102431929039,0.));
#84995=CARTESIAN_POINT('Ctrl Pts',(-70.9445024378439,5.00102431929039,12.));
#84996=CARTESIAN_POINT('Ctrl Pts',(-70.9661126860773,4.99565658516913,0.));
#84997=CARTESIAN_POINT('Ctrl Pts',(-70.9661126860773,4.99565658516913,12.));
#84998=CARTESIAN_POINT('Ctrl Pts',(-70.9877626211113,4.99025568790664,0.));
#84999=CARTESIAN_POINT('Ctrl Pts',(-70.9877626211113,4.99025568790664,12.));
#85000=CARTESIAN_POINT('Ctrl Pts',(-71.0094520872377,4.98482159331863,0.));
#85001=CARTESIAN_POINT('Ctrl Pts',(-71.0094520872377,4.98482159331863,12.));
#85002=CARTESIAN_POINT('Ctrl Pts',(-71.0311809294821,4.97935426748584,0.));
#85003=CARTESIAN_POINT('Ctrl Pts',(-71.0311809294821,4.97935426748584,12.));
#85004=CARTESIAN_POINT('Ctrl Pts',(-71.0529489935961,4.97385367675158,0.));
#85005=CARTESIAN_POINT('Ctrl Pts',(-71.0529489935961,4.97385367675158,12.));
#85006=CARTESIAN_POINT('Ctrl Pts',(-71.0747561260436,4.9683197877219,0.));
#85007=CARTESIAN_POINT('Ctrl Pts',(-71.0747561260436,4.9683197877219,12.));
#85008=CARTESIAN_POINT('Ctrl Pts',(-71.0966021739907,4.96275256726765,0.));
#85009=CARTESIAN_POINT('Ctrl Pts',(-71.0966021739907,4.96275256726765,12.));
#85010=CARTESIAN_POINT('Ctrl Pts',(-71.1184869853056,4.95715198251684,0.));
#85011=CARTESIAN_POINT('Ctrl Pts',(-71.1184869853056,4.95715198251684,12.));
#85012=CARTESIAN_POINT('Ctrl Pts',(-71.1404104085552,4.95151800085101,0.));
#85013=CARTESIAN_POINT('Ctrl Pts',(-71.1404104085552,4.95151800085101,12.));
#85014=CARTESIAN_POINT('Ctrl Pts',(-71.1623722930001,4.94585058990341,0.));
#85015=CARTESIAN_POINT('Ctrl Pts',(-71.1623722930001,4.94585058990341,12.));
#85016=CARTESIAN_POINT('Ctrl Pts',(-71.1843724885847,4.94014971756114,0.));
#85017=CARTESIAN_POINT('Ctrl Pts',(-71.1843724885847,4.94014971756114,12.));
#85018=CARTESIAN_POINT('Ctrl Pts',(-71.2064108459286,4.93441535196617,0.));
#85019=CARTESIAN_POINT('Ctrl Pts',(-71.2064108459286,4.93441535196617,12.));
#85020=CARTESIAN_POINT('Ctrl Pts',(-71.2284872163273,4.92864746150732,0.));
#85021=CARTESIAN_POINT('Ctrl Pts',(-71.2284872163273,4.92864746150732,12.));
#85022=CARTESIAN_POINT('Ctrl Pts',(-71.250601451747,4.92284601481721,0.));
#85023=CARTESIAN_POINT('Ctrl Pts',(-71.250601451747,4.92284601481721,12.));
#85024=CARTESIAN_POINT('Ctrl Pts',(-71.2727534048192,4.91701098077036,0.));
#85025=CARTESIAN_POINT('Ctrl Pts',(-71.2727534048192,4.91701098077036,12.));
#85026=CARTESIAN_POINT('Ctrl Pts',(-71.294942928829,4.91114232848603,0.));
#85027=CARTESIAN_POINT('Ctrl Pts',(-71.294942928829,4.91114232848603,12.));
#85028=CARTESIAN_POINT('Ctrl Pts',(-71.3171698777084,4.90524002732778,0.));
#85029=CARTESIAN_POINT('Ctrl Pts',(-71.3171698777084,4.90524002732778,12.));
#85030=CARTESIAN_POINT('Ctrl Pts',(-71.3394341060359,4.89930404689574,0.));
#85031=CARTESIAN_POINT('Ctrl Pts',(-71.3394341060359,4.89930404689574,12.));
#85032=CARTESIAN_POINT('Ctrl Pts',(-71.3617354690325,4.89333435702413,0.));
#85033=CARTESIAN_POINT('Ctrl Pts',(-71.3617354690325,4.89333435702413,12.));
#85034=CARTESIAN_POINT('Ctrl Pts',(-71.3840738225562,4.88733092777974,0.));
#85035=CARTESIAN_POINT('Ctrl Pts',(-71.3840738225562,4.88733092777974,12.));
#85036=CARTESIAN_POINT('Ctrl Pts',(-71.4064490230899,4.88129372946551,0.));
#85037=CARTESIAN_POINT('Ctrl Pts',(-71.4064490230899,4.88129372946551,12.));
#85038=CARTESIAN_POINT('Ctrl Pts',(-71.4288609277374,4.87522273261907,0.));
#85039=CARTESIAN_POINT('Ctrl Pts',(-71.4288609277374,4.87522273261907,12.));
#85040=CARTESIAN_POINT('Ctrl Pts',(-71.4513093942255,4.86911790800549,0.));
#85041=CARTESIAN_POINT('Ctrl Pts',(-71.4513093942255,4.86911790800549,12.));
#85042=CARTESIAN_POINT('Ctrl Pts',(-71.4737942808982,4.86297922661502,0.));
#85043=CARTESIAN_POINT('Ctrl Pts',(-71.4737942808982,4.86297922661502,12.));
#85044=CARTESIAN_POINT('Ctrl Pts',(-71.4963154467113,4.8568066596618,0.));
#85045=CARTESIAN_POINT('Ctrl Pts',(-71.4963154467113,4.8568066596618,12.));
#85046=CARTESIAN_POINT('Ctrl Pts',(-71.5188727512197,4.8506001785878,0.));
#85047=CARTESIAN_POINT('Ctrl Pts',(-71.5188727512197,4.8506001785878,12.));
#85048=CARTESIAN_POINT('Ctrl Pts',(-71.5414660545739,4.84435975506048,0.));
#85049=CARTESIAN_POINT('Ctrl Pts',(-71.5414660545739,4.84435975506048,12.));
#85050=CARTESIAN_POINT('Ctrl Pts',(-71.564095217521,4.83808536096583,0.));
#85051=CARTESIAN_POINT('Ctrl Pts',(-71.564095217521,4.83808536096583,12.));
#85052=CARTESIAN_POINT('Ctrl Pts',(-71.5867601014,4.83177696840637,0.));
#85053=CARTESIAN_POINT('Ctrl Pts',(-71.5867601014,4.83177696840637,12.));
#85054=CARTESIAN_POINT('Ctrl Pts',(-71.6094605681366,4.82543454970026,0.));
#85055=CARTESIAN_POINT('Ctrl Pts',(-71.6094605681366,4.82543454970026,12.));
#85056=CARTESIAN_POINT('Ctrl Pts',(-71.6321964802326,4.81905807738557,0.));
#85057=CARTESIAN_POINT('Ctrl Pts',(-71.6321964802326,4.81905807738557,12.));
#85058=CARTESIAN_POINT('Ctrl Pts',(-71.6549677007613,4.81264752421732,0.));
#85059=CARTESIAN_POINT('Ctrl Pts',(-71.6549677007613,4.81264752421732,12.));
#85060=CARTESIAN_POINT('Ctrl Pts',(-71.6777740933705,4.80620286316088,0.));
#85061=CARTESIAN_POINT('Ctrl Pts',(-71.6777740933705,4.80620286316088,12.));
#85062=CARTESIAN_POINT('Ctrl Pts',(-71.7006155222766,4.79972406739013,0.));
#85063=CARTESIAN_POINT('Ctrl Pts',(-71.7006155222766,4.79972406739013,12.));
#85064=CARTESIAN_POINT('Ctrl Pts',(-71.7234918522604,4.79321111028671,0.));
#85065=CARTESIAN_POINT('Ctrl Pts',(-71.7234918522604,4.79321111028671,12.));
#85066=CARTESIAN_POINT('Ctrl Pts',(-71.7464029486552,4.7866639654445,0.));
#85067=CARTESIAN_POINT('Ctrl Pts',(-71.7464029486552,4.7866639654445,12.));
#85068=CARTESIAN_POINT('Ctrl Pts',(-71.7693486773449,4.78008260666642,0.));
#85069=CARTESIAN_POINT('Ctrl Pts',(-71.7693486773449,4.78008260666642,12.));
#85070=CARTESIAN_POINT('Ctrl Pts',(-71.7923289047636,4.77346700795787,0.));
#85071=CARTESIAN_POINT('Ctrl Pts',(-71.7923289047636,4.77346700795787,12.));
#85072=CARTESIAN_POINT('Ctrl Pts',(-71.8153434978924,4.76681714352503,0.));
#85073=CARTESIAN_POINT('Ctrl Pts',(-71.8153434978924,4.76681714352503,12.));
#85074=CARTESIAN_POINT('Ctrl Pts',(-71.8383923242533,4.76013298777422,0.));
#85075=CARTESIAN_POINT('Ctrl Pts',(-71.8383923242533,4.76013298777422,12.));
#85076=CARTESIAN_POINT('Ctrl Pts',(-71.8614752519008,4.7534145153167,0.));
#85077=CARTESIAN_POINT('Ctrl Pts',(-71.8614752519008,4.7534145153167,12.));
#85078=CARTESIAN_POINT('Ctrl Pts',(-71.8845921494186,4.74666170096545,0.));
#85079=CARTESIAN_POINT('Ctrl Pts',(-71.8845921494186,4.74666170096545,12.));
#85080=CARTESIAN_POINT('Ctrl Pts',(-71.9077428859207,4.7398745197286,0.));
#85081=CARTESIAN_POINT('Ctrl Pts',(-71.9077428859207,4.7398745197286,12.));
#85082=CARTESIAN_POINT('Ctrl Pts',(-71.9309273310469,4.73305294680783,0.));
#85083=CARTESIAN_POINT('Ctrl Pts',(-71.9309273310469,4.73305294680783,12.));
#85084=CARTESIAN_POINT('Ctrl Pts',(-71.9541453549582,4.72619695759778,0.));
#85085=CARTESIAN_POINT('Ctrl Pts',(-71.9541453549582,4.72619695759778,12.));
#85086=CARTESIAN_POINT('Ctrl Pts',(-71.9773968283267,4.7193065276908,0.));
#85087=CARTESIAN_POINT('Ctrl Pts',(-71.9773968283267,4.7193065276908,12.));
#85088=CARTESIAN_POINT('Ctrl Pts',(-72.0006816223335,4.7123816328741,0.));
#85089=CARTESIAN_POINT('Ctrl Pts',(-72.0006816223335,4.7123816328741,12.));
#85090=CARTESIAN_POINT('Ctrl Pts',(-72.0239996086694,4.70542224912312,0.));
#85091=CARTESIAN_POINT('Ctrl Pts',(-72.0239996086694,4.70542224912312,12.));
#85092=CARTESIAN_POINT('Ctrl Pts',(-72.047350659532,4.69842835259997,0.));
#85093=CARTESIAN_POINT('Ctrl Pts',(-72.047350659532,4.69842835259997,12.));
#85094=CARTESIAN_POINT('Ctrl Pts',(-72.070734647621,4.69139991965279,0.));
#85095=CARTESIAN_POINT('Ctrl Pts',(-72.070734647621,4.69139991965279,12.));
#85096=CARTESIAN_POINT('Ctrl Pts',(-72.0941514461283,4.6843369268206,0.));
#85097=CARTESIAN_POINT('Ctrl Pts',(-72.0941514461283,4.6843369268206,12.));
#85098=CARTESIAN_POINT('Ctrl Pts',(-72.1176009287349,4.67723935083087,0.));
#85099=CARTESIAN_POINT('Ctrl Pts',(-72.1176009287349,4.67723935083087,12.));
#85100=CARTESIAN_POINT('Ctrl Pts',(-72.1410829696129,4.6701071685928,0.));
#85101=CARTESIAN_POINT('Ctrl Pts',(-72.1410829696129,4.6701071685928,12.));
#85102=CARTESIAN_POINT('Ctrl Pts',(-72.1645974434218,4.6629403571957,0.));
#85103=CARTESIAN_POINT('Ctrl Pts',(-72.1645974434218,4.6629403571957,12.));
#85104=CARTESIAN_POINT('Ctrl Pts',(-72.1881442253052,4.65573889390824,0.));
#85105=CARTESIAN_POINT('Ctrl Pts',(-72.1881442253052,4.65573889390824,12.));
#85106=CARTESIAN_POINT('Ctrl Pts',(-72.2117231908816,4.64850275618324,0.));
#85107=CARTESIAN_POINT('Ctrl Pts',(-72.2117231908816,4.64850275618324,12.));
#85108=CARTESIAN_POINT('Ctrl Pts',(-72.2353342162408,4.64123192165627,0.));
#85109=CARTESIAN_POINT('Ctrl Pts',(-72.2353342162408,4.64123192165627,12.));
#85110=CARTESIAN_POINT('Ctrl Pts',(-72.2589771779447,4.63392636813842,0.));
#85111=CARTESIAN_POINT('Ctrl Pts',(-72.2589771779447,4.63392636813842,12.));
#85112=CARTESIAN_POINT('Ctrl Pts',(-72.2826519530254,4.62658607361465,0.));
#85113=CARTESIAN_POINT('Ctrl Pts',(-72.2826519530254,4.62658607361465,12.));
#85114=CARTESIAN_POINT('Ctrl Pts',(-72.306358418981,4.61921101624294,0.));
#85115=CARTESIAN_POINT('Ctrl Pts',(-72.306358418981,4.61921101624294,12.));
#85116=CARTESIAN_POINT('Ctrl Pts',(-72.330096453767,4.61180117435868,0.));
#85117=CARTESIAN_POINT('Ctrl Pts',(-72.330096453767,4.61180117435868,12.));
#85118=CARTESIAN_POINT('Ctrl Pts',(-72.3538659357932,4.60435652647463,0.));
#85119=CARTESIAN_POINT('Ctrl Pts',(-72.3538659357932,4.60435652647463,12.));
#85120=CARTESIAN_POINT('Ctrl Pts',(-72.3776667439244,4.5968770512734,0.));
#85121=CARTESIAN_POINT('Ctrl Pts',(-72.3776667439244,4.5968770512734,12.));
#85122=CARTESIAN_POINT('Ctrl Pts',(-72.4014987574789,4.5893627276055,0.));
#85123=CARTESIAN_POINT('Ctrl Pts',(-72.4014987574789,4.5893627276055,12.));
#85124=CARTESIAN_POINT('Ctrl Pts',(-72.4253618562249,4.5818135344885,0.));
#85125=CARTESIAN_POINT('Ctrl Pts',(-72.4253618562249,4.5818135344885,12.));
#85126=CARTESIAN_POINT('Ctrl Pts',(-72.449255920373,4.57422945111094,0.));
#85127=CARTESIAN_POINT('Ctrl Pts',(-72.449255920373,4.57422945111094,12.));
#85128=CARTESIAN_POINT('Ctrl Pts',(-72.473180830571,4.56661045683366,0.));
#85129=CARTESIAN_POINT('Ctrl Pts',(-72.473180830571,4.56661045683366,12.));
#85130=CARTESIAN_POINT('Ctrl Pts',(-72.4971364679055,4.55895653118213,0.));
#85131=CARTESIAN_POINT('Ctrl Pts',(-72.4971364679055,4.55895653118213,12.));
#85132=CARTESIAN_POINT('Ctrl Pts',(-72.5211227138997,4.55126765384402,0.));
#85133=CARTESIAN_POINT('Ctrl Pts',(-72.5211227138997,4.55126765384402,12.));
#85134=CARTESIAN_POINT('Ctrl Pts',(-72.5451394505106,4.54354380466824,0.));
#85135=CARTESIAN_POINT('Ctrl Pts',(-72.5451394505106,4.54354380466824,12.));
#85136=CARTESIAN_POINT('Ctrl Pts',(-72.5691865601225,4.53578496366801,0.));
#85137=CARTESIAN_POINT('Ctrl Pts',(-72.5691865601225,4.53578496366801,12.));
#85138=CARTESIAN_POINT('Ctrl Pts',(-72.5932639255406,4.5279911110239,0.));
#85139=CARTESIAN_POINT('Ctrl Pts',(-72.5932639255406,4.5279911110239,12.));
#85140=CARTESIAN_POINT('Ctrl Pts',(-72.6173714299935,4.52016222707632,0.));
#85141=CARTESIAN_POINT('Ctrl Pts',(-72.6173714299935,4.52016222707632,12.));
#85142=CARTESIAN_POINT('Ctrl Pts',(-72.6415089571314,4.51229829232259,0.));
#85143=CARTESIAN_POINT('Ctrl Pts',(-72.6415089571314,4.51229829232259,12.));
#85144=CARTESIAN_POINT('Ctrl Pts',(-72.6656763910241,4.50439928741604,0.));
#85145=CARTESIAN_POINT('Ctrl Pts',(-72.6656763910241,4.50439928741604,12.));
#85146=CARTESIAN_POINT('Ctrl Pts',(-72.689873616155,4.49646519316821,0.));
#85147=CARTESIAN_POINT('Ctrl Pts',(-72.689873616155,4.49646519316821,12.));
#85148=CARTESIAN_POINT('Ctrl Pts',(-72.7141005174153,4.48849599055353,0.));
#85149=CARTESIAN_POINT('Ctrl Pts',(-72.7141005174153,4.48849599055353,12.));
#85150=CARTESIAN_POINT('Ctrl Pts',(-72.7383569801042,4.48049166070223,0.));
#85151=CARTESIAN_POINT('Ctrl Pts',(-72.7383569801042,4.48049166070223,12.));
#85152=CARTESIAN_POINT('Ctrl Pts',(-72.7626428899287,4.47245218489622,0.));
#85153=CARTESIAN_POINT('Ctrl Pts',(-72.7626428899287,4.47245218489622,12.));
#85154=CARTESIAN_POINT('Ctrl Pts',(-72.7869581329994,4.46437754456795,0.));
#85155=CARTESIAN_POINT('Ctrl Pts',(-72.7869581329994,4.46437754456795,12.));
#85156=CARTESIAN_POINT('Ctrl Pts',(-72.8113025958258,4.45626772130138,0.));
#85157=CARTESIAN_POINT('Ctrl Pts',(-72.8113025958258,4.45626772130138,12.));
#85158=CARTESIAN_POINT('Ctrl Pts',(-72.8356761653064,4.44812269683724,0.));
#85159=CARTESIAN_POINT('Ctrl Pts',(-72.8356761653064,4.44812269683724,12.));
#85160=CARTESIAN_POINT('Ctrl Pts',(-72.8600787287316,4.43994245306804,0.));
#85161=CARTESIAN_POINT('Ctrl Pts',(-72.8600787287316,4.43994245306804,12.));
#85162=CARTESIAN_POINT('Ctrl Pts',(-72.8845101737856,4.43172697203341,0.));
#85163=CARTESIAN_POINT('Ctrl Pts',(-72.8845101737856,4.43172697203341,12.));
#85164=CARTESIAN_POINT('Ctrl Pts',(-72.9089703885463,4.42347623591941,0.));
#85165=CARTESIAN_POINT('Ctrl Pts',(-72.9089703885463,4.42347623591941,12.));
#85166=CARTESIAN_POINT('Ctrl Pts',(-72.9334592614828,4.41519022705926,0.));
#85167=CARTESIAN_POINT('Ctrl Pts',(-72.9334592614828,4.41519022705926,12.));
#85168=CARTESIAN_POINT('Ctrl Pts',(-72.9579766814495,4.40686892793964,0.));
#85169=CARTESIAN_POINT('Ctrl Pts',(-72.9579766814495,4.40686892793964,12.));
#85170=CARTESIAN_POINT('Ctrl Pts',(-72.9825225376839,4.3985123211973,0.));
#85171=CARTESIAN_POINT('Ctrl Pts',(-72.9825225376839,4.3985123211973,12.));
#85172=CARTESIAN_POINT('Ctrl Pts',(-73.0070967198033,4.39012038961144,0.));
#85173=CARTESIAN_POINT('Ctrl Pts',(-73.0070967198033,4.39012038961144,12.));
#85174=CARTESIAN_POINT('Ctrl Pts',(-73.031699117799,4.38169311610153,0.));
#85175=CARTESIAN_POINT('Ctrl Pts',(-73.031699117799,4.38169311610153,12.));
#85176=CARTESIAN_POINT('Ctrl Pts',(-73.0563296220301,4.37323048372606,0.));
#85177=CARTESIAN_POINT('Ctrl Pts',(-73.0563296220301,4.37323048372606,12.));
#85178=CARTESIAN_POINT('Ctrl Pts',(-73.0809881232111,4.36473247568638,0.));
#85179=CARTESIAN_POINT('Ctrl Pts',(-73.0809881232111,4.36473247568638,12.));
#85180=CARTESIAN_POINT('Ctrl Pts',(-73.1056745124099,4.35619907532715,0.));
#85181=CARTESIAN_POINT('Ctrl Pts',(-73.1056745124099,4.35619907532715,12.));
#85182=CARTESIAN_POINT('Ctrl Pts',(-73.1303886810602,4.34763026613154,0.));
#85183=CARTESIAN_POINT('Ctrl Pts',(-73.1303886810602,4.34763026613154,12.));
#85184=CARTESIAN_POINT('Ctrl Pts',(-73.1551305209692,4.33902603172139,0.));
#85185=CARTESIAN_POINT('Ctrl Pts',(-73.1551305209692,4.33902603172139,12.));
#85186=CARTESIAN_POINT('Ctrl Pts',(-73.1798999243234,4.33038635585878,0.));
#85187=CARTESIAN_POINT('Ctrl Pts',(-73.1798999243234,4.33038635585878,12.));
#85188=CARTESIAN_POINT('Ctrl Pts',(-73.204696783693,4.32171122245218,0.));
#85189=CARTESIAN_POINT('Ctrl Pts',(-73.204696783693,4.32171122245218,12.));
#85190=CARTESIAN_POINT('Ctrl Pts',(-73.2295209920319,4.31300061556102,0.));
#85191=CARTESIAN_POINT('Ctrl Pts',(-73.2295209920319,4.31300061556102,12.));
#85192=CARTESIAN_POINT('Ctrl Pts',(-73.2543724426562,4.30425451938233,0.));
#85193=CARTESIAN_POINT('Ctrl Pts',(-73.2543724426562,4.30425451938233,12.));
#85194=CARTESIAN_POINT('Ctrl Pts',(-73.2792510292243,4.29547291824288,0.));
#85195=CARTESIAN_POINT('Ctrl Pts',(-73.2792510292243,4.29547291824288,12.));
#85196=CARTESIAN_POINT('Ctrl Pts',(-73.3041566457134,4.28665579659301,0.));
#85197=CARTESIAN_POINT('Ctrl Pts',(-73.3041566457134,4.28665579659301,12.));
#85198=CARTESIAN_POINT('Ctrl Pts',(-73.3290891863959,4.27780313900391,0.));
#85199=CARTESIAN_POINT('Ctrl Pts',(-73.3290891863959,4.27780313900391,12.));
#85200=CARTESIAN_POINT('Ctrl Pts',(-73.354048545808,4.26891493016703,0.));
#85201=CARTESIAN_POINT('Ctrl Pts',(-73.354048545808,4.26891493016703,12.));
#85202=CARTESIAN_POINT('Ctrl Pts',(-73.3790346187953,4.25999115489904,0.));
#85203=CARTESIAN_POINT('Ctrl Pts',(-73.3790346187953,4.25999115489904,12.));
#85204=CARTESIAN_POINT('Ctrl Pts',(-73.4040473005603,4.25103179814891,0.));
#85205=CARTESIAN_POINT('Ctrl Pts',(-73.4040473005603,4.25103179814891,12.));
#85206=CARTESIAN_POINT('Ctrl Pts',(-73.4290864867103,4.24203684500941,0.));
#85207=CARTESIAN_POINT('Ctrl Pts',(-73.4290864867103,4.24203684500941,12.));
#85208=CARTESIAN_POINT('Ctrl Pts',(-73.4541520732943,4.23300628072757,0.));
#85209=CARTESIAN_POINT('Ctrl Pts',(-73.4541520732943,4.23300628072757,12.));
#85210=CARTESIAN_POINT('Ctrl Pts',(-73.4792439568624,4.22394009072752,0.));
#85211=CARTESIAN_POINT('Ctrl Pts',(-73.4792439568624,4.22394009072752,12.));
#85212=CARTESIAN_POINT('Ctrl Pts',(-73.5043620344107,4.21483826059436,0.));
#85213=CARTESIAN_POINT('Ctrl Pts',(-73.5043620344107,4.21483826059436,12.));
#85214=CARTESIAN_POINT('Ctrl Pts',(-73.5295062032621,4.20570077603727,0.));
#85215=CARTESIAN_POINT('Ctrl Pts',(-73.5295062032621,4.20570077603727,12.));
#85216=CARTESIAN_POINT('Ctrl Pts',(-73.554676360957,4.19652762286126,0.));
#85217=CARTESIAN_POINT('Ctrl Pts',(-73.554676360957,4.19652762286126,12.));
#85218=CARTESIAN_POINT('Ctrl Pts',(-73.5798724051519,4.18731878694237,0.));
#85219=CARTESIAN_POINT('Ctrl Pts',(-73.5798724051519,4.18731878694237,12.));
#85220=CARTESIAN_POINT('Ctrl Pts',(-73.6050942334773,4.17807425419816,0.));
#85221=CARTESIAN_POINT('Ctrl Pts',(-73.6050942334773,4.17807425419816,12.));
#85222=CARTESIAN_POINT('Ctrl Pts',(-73.6303417435262,4.16879401058786,0.));
#85223=CARTESIAN_POINT('Ctrl Pts',(-73.6303417435262,4.16879401058786,12.));
#85224=CARTESIAN_POINT('Ctrl Pts',(-73.6556148331504,4.1594780421779,0.));
#85225=CARTESIAN_POINT('Ctrl Pts',(-73.6556148331504,4.1594780421779,12.));
#85226=CARTESIAN_POINT('Ctrl Pts',(-73.6809134006909,4.15012633519727,0.));
#85227=CARTESIAN_POINT('Ctrl Pts',(-73.6809134006909,4.15012633519727,12.));
#85228=CARTESIAN_POINT('Ctrl Pts',(-73.7062373452344,4.14073887610154,0.));
#85229=CARTESIAN_POINT('Ctrl Pts',(-73.7062373452344,4.14073887610154,12.));
#85230=CARTESIAN_POINT('Ctrl Pts',(-73.7315865668508,4.13131565163574,0.));
#85231=CARTESIAN_POINT('Ctrl Pts',(-73.7315865668508,4.13131565163574,12.));
#85232=CARTESIAN_POINT('Ctrl Pts',(-73.7569609668501,4.1218566489055,0.));
#85233=CARTESIAN_POINT('Ctrl Pts',(-73.7569609668501,4.1218566489055,12.));
#85234=CARTESIAN_POINT('Ctrl Pts',(-73.7823604472126,4.1123618552278,0.));
#85235=CARTESIAN_POINT('Ctrl Pts',(-73.7823604472126,4.1123618552278,12.));
#85236=CARTESIAN_POINT('Ctrl Pts',(-73.8077849100314,4.10283125798724,0.));
#85237=CARTESIAN_POINT('Ctrl Pts',(-73.8077849100314,4.10283125798724,12.));
#85238=CARTESIAN_POINT('Ctrl Pts',(-73.8332342568978,4.09326484448231,0.));
#85239=CARTESIAN_POINT('Ctrl Pts',(-73.8332342568978,4.09326484448231,12.));
#85240=CARTESIAN_POINT('Ctrl Pts',(-73.8587083884208,4.08366260180679,0.));
#85241=CARTESIAN_POINT('Ctrl Pts',(-73.8587083884208,4.08366260180679,12.));
#85242=CARTESIAN_POINT('Ctrl Pts',(-73.884207203405,4.07402451665252,0.));
#85243=CARTESIAN_POINT('Ctrl Pts',(-73.884207203405,4.07402451665252,12.));
#85244=CARTESIAN_POINT('Ctrl Pts',(-73.9097305995173,4.06435057547334,0.));
#85245=CARTESIAN_POINT('Ctrl Pts',(-73.9097305995173,4.06435057547334,12.));
#85246=CARTESIAN_POINT('Ctrl Pts',(-73.9352784747665,4.05464076484761,0.));
#85247=CARTESIAN_POINT('Ctrl Pts',(-73.9352784747665,4.05464076484761,12.));
#85248=CARTESIAN_POINT('Ctrl Pts',(-73.9608507287943,4.04489507179963,0.));
#85249=CARTESIAN_POINT('Ctrl Pts',(-73.9608507287943,4.04489507179963,12.));
#85250=CARTESIAN_POINT('Ctrl Pts',(-73.9864472641025,4.03511348410659,0.));
#85251=CARTESIAN_POINT('Ctrl Pts',(-73.9864472641025,4.03511348410659,12.));
#85252=CARTESIAN_POINT('Ctrl Pts',(-74.0120679876396,4.02529599070084,0.));
#85253=CARTESIAN_POINT('Ctrl Pts',(-74.0120679876396,4.02529599070084,12.));
#85254=CARTESIAN_POINT('Ctrl Pts',(-74.0377128111754,4.01544258176692,0.));
#85255=CARTESIAN_POINT('Ctrl Pts',(-74.0377128111754,4.01544258176692,12.));
#85256=CARTESIAN_POINT('Ctrl Pts',(-74.0633816477912,4.00555324785459,0.));
#85257=CARTESIAN_POINT('Ctrl Pts',(-74.0633816477912,4.00555324785459,12.));
#85258=CARTESIAN_POINT('Ctrl Pts',(-74.0890744091088,3.99562797918271,0.));
#85259=CARTESIAN_POINT('Ctrl Pts',(-74.0890744091088,3.99562797918271,12.));
#85260=CARTESIAN_POINT('Ctrl Pts',(-74.1147910020869,3.98566676483638,0.));
#85261=CARTESIAN_POINT('Ctrl Pts',(-74.1147910020869,3.98566676483638,12.));
#85262=CARTESIAN_POINT('Ctrl Pts',(-74.1405313263198,3.97566959209546,0.));
#85263=CARTESIAN_POINT('Ctrl Pts',(-74.1405313263198,3.97566959209546,12.));
#85264=CARTESIAN_POINT('Ctrl Pts',(-74.1662952702689,3.96563644549422,0.));
#85265=CARTESIAN_POINT('Ctrl Pts',(-74.1662952702689,3.96563644549422,12.));
#85266=CARTESIAN_POINT('Ctrl Pts',(-74.1920827166861,3.95556730821159,0.));
#85267=CARTESIAN_POINT('Ctrl Pts',(-74.1920827166861,3.95556730821159,12.));
#85268=CARTESIAN_POINT('Ctrl Pts',(-74.217893549314,3.94546216377498,0.));
#85269=CARTESIAN_POINT('Ctrl Pts',(-74.217893549314,3.94546216377498,12.));
#85270=CARTESIAN_POINT('Ctrl Pts',(-74.2437276593763,3.93532099774229,0.));
#85271=CARTESIAN_POINT('Ctrl Pts',(-74.2437276593763,3.93532099774229,12.));
#85272=CARTESIAN_POINT('Ctrl Pts',(-74.2695849516134,3.92514379920728,0.));
#85273=CARTESIAN_POINT('Ctrl Pts',(-74.2695849516134,3.92514379920728,12.));
#85274=CARTESIAN_POINT('Ctrl Pts',(-74.2954653518345,3.91493056284964,0.));
#85275=CARTESIAN_POINT('Ctrl Pts',(-74.2954653518345,3.91493056284964,12.));
#85276=CARTESIAN_POINT('Ctrl Pts',(-74.3213688089495,3.9046812890452,0.));
#85277=CARTESIAN_POINT('Ctrl Pts',(-74.3213688089495,3.9046812890452,12.));
#85278=CARTESIAN_POINT('Ctrl Pts',(-74.3472952898,3.89439598145193,0.));
#85279=CARTESIAN_POINT('Ctrl Pts',(-74.3472952898,3.89439598145193,12.));
#85280=CARTESIAN_POINT('Ctrl Pts',(-74.3680548786039,3.88613891247869,0.));
#85281=CARTESIAN_POINT('Ctrl Pts',(-74.3680548786039,3.88613891247869,12.));
#85282=CARTESIAN_POINT('Ctrl Pts',(-74.3836349188809,3.87992989995677,0.));
#85283=CARTESIAN_POINT('Ctrl Pts',(-74.3836349188809,3.87992989995677,12.));
#85284=CARTESIAN_POINT('Ctrl Pts',(-74.3940262116251,3.875783353773,0.));
#85285=CARTESIAN_POINT('Ctrl Pts',(-74.3940262116251,3.875783353773,12.));
#85286=CARTESIAN_POINT('Ctrl Pts',(-74.3992230078037,3.87370827955544,0.));
#85287=CARTESIAN_POINT('Ctrl Pts',(-74.3992230078037,3.87370827955544,12.));
#85288=CARTESIAN_POINT('',(-69.8028570375097,5.24987136994592,0.));
#85289=CARTESIAN_POINT('Ctrl Pts',(-69.8028570375097,5.24987136994592,0.));
#85290=CARTESIAN_POINT('Ctrl Pts',(-69.8066748687772,5.24915955997427,0.));
#85291=CARTESIAN_POINT('Ctrl Pts',(-69.8143154684204,5.24773285666376,0.));
#85292=CARTESIAN_POINT('Ctrl Pts',(-69.8257911792159,5.2455835515975,0.));
#85293=CARTESIAN_POINT('Ctrl Pts',(-69.841121750752,5.24269931054569,0.));
#85294=CARTESIAN_POINT('Ctrl Pts',(-69.8603343302743,5.23906316634802,0.));
#85295=CARTESIAN_POINT('Ctrl Pts',(-69.8795962381599,5.2353961627962,0.));
#85296=CARTESIAN_POINT('Ctrl Pts',(-69.8989073936688,5.23169827290555,0.));
#85297=CARTESIAN_POINT('Ctrl Pts',(-69.9182676502048,5.22796945602793,0.));
#85298=CARTESIAN_POINT('Ctrl Pts',(-69.9376767969095,5.22420965879981,0.));
#85299=CARTESIAN_POINT('Ctrl Pts',(-69.9571345870076,5.2204188207572,0.));
#85300=CARTESIAN_POINT('Ctrl Pts',(-69.9766407595385,5.21659687881139,0.));
#85301=CARTESIAN_POINT('Ctrl Pts',(-69.9961950629965,5.21274377203259,0.));
#85302=CARTESIAN_POINT('Ctrl Pts',(-70.0157972802182,5.20885944672836,0.));
#85303=CARTESIAN_POINT('Ctrl Pts',(-70.0354472203546,5.20494385478025,0.));
#85304=CARTESIAN_POINT('Ctrl Pts',(-70.0551447071082,5.20099695122656,0.));
#85305=CARTESIAN_POINT('Ctrl Pts',(-70.0748895689729,5.19701869225528,0.));
#85306=CARTESIAN_POINT('Ctrl Pts',(-70.0946816270997,5.19300903271579,0.));
#85307=CARTESIAN_POINT('Ctrl Pts',(-70.1145206891885,5.18896792486565,0.));
#85308=CARTESIAN_POINT('Ctrl Pts',(-70.1344065558145,5.18489531966264,0.));
#85309=CARTESIAN_POINT('Ctrl Pts',(-70.1543390243892,5.18079116757666,0.));
#85310=CARTESIAN_POINT('Ctrl Pts',(-70.1743178937077,5.17665541952382,0.));
#85311=CARTESIAN_POINT('Ctrl Pts',(-70.1943429691167,5.17248802793389,0.));
#85312=CARTESIAN_POINT('Ctrl Pts',(-70.2144140622953,5.16828894670108,0.));
#85313=CARTESIAN_POINT('Ctrl Pts',(-70.2345309887833,5.16405813066976,0.));
#85314=CARTESIAN_POINT('Ctrl Pts',(-70.2546935662722,5.15979553528203,0.));
#85315=CARTESIAN_POINT('Ctrl Pts',(-70.2749016125105,5.15550111614859,0.));
#85316=CARTESIAN_POINT('Ctrl Pts',(-70.2951549435512,5.15117482869254,0.));
#85317=CARTESIAN_POINT('Ctrl Pts',(-70.3154533746736,5.1468166283308,0.));
#85318=CARTESIAN_POINT('Ctrl Pts',(-70.3357967211796,5.14242647063479,0.));
#85319=CARTESIAN_POINT('Ctrl Pts',(-70.3561847991714,5.13800431148903,0.));
#85320=CARTESIAN_POINT('Ctrl Pts',(-70.3766174264757,5.13355010728567,0.));
#85321=CARTESIAN_POINT('Ctrl Pts',(-70.3970944229851,5.12906381499456,0.));
#85322=CARTESIAN_POINT('Ctrl Pts',(-70.417615610161,5.12454539205328,0.));
#85323=CARTESIAN_POINT('Ctrl Pts',(-70.4381808107245,5.11999479630211,0.));
#85324=CARTESIAN_POINT('Ctrl Pts',(-70.458789848296,5.11541198590932,0.));
#85325=CARTESIAN_POINT('Ctrl Pts',(-70.4794425469825,5.11079691929213,0.));
#85326=CARTESIAN_POINT('Ctrl Pts',(-70.500138731399,5.10614955511663,0.));
#85327=CARTESIAN_POINT('Ctrl Pts',(-70.5208782268497,5.1014698523294,0.));
#85328=CARTESIAN_POINT('Ctrl Pts',(-70.5416608594526,5.09675777018182,0.));
#85329=CARTESIAN_POINT('Ctrl Pts',(-70.5624864562824,5.09201326826134,0.));
#85330=CARTESIAN_POINT('Ctrl Pts',(-70.5833548455014,5.08723630652272,0.));
#85331=CARTESIAN_POINT('Ctrl Pts',(-70.6042658562923,5.08242684526686,0.));
#85332=CARTESIAN_POINT('Ctrl Pts',(-70.6252193187878,5.07758484512302,0.));
#85333=CARTESIAN_POINT('Ctrl Pts',(-70.6462150640015,5.07271026703354,0.));
#85334=CARTESIAN_POINT('Ctrl Pts',(-70.6672529237455,5.06780307224071,0.));
#85335=CARTESIAN_POINT('Ctrl Pts',(-70.6883327305784,5.06286322227819,0.));
#85336=CARTESIAN_POINT('Ctrl Pts',(-70.7094543178438,5.05789067897057,0.));
#85337=CARTESIAN_POINT('Ctrl Pts',(-70.7306175196863,5.05288540443482,0.));
#85338=CARTESIAN_POINT('Ctrl Pts',(-70.7518221710706,5.04784736108346,0.));
#85339=CARTESIAN_POINT('Ctrl Pts',(-70.7730681077983,5.04277651163349,0.));
#85340=CARTESIAN_POINT('Ctrl Pts',(-70.7943551665059,5.03767281910479,0.));
#85341=CARTESIAN_POINT('Ctrl Pts',(-70.8156831846488,5.0325362468094,0.));
#85342=CARTESIAN_POINT('Ctrl Pts',(-70.8370520004843,5.02736675834692,0.));
#85343=CARTESIAN_POINT('Ctrl Pts',(-70.8584614530519,5.0221643176006,0.));
#85344=CARTESIAN_POINT('Ctrl Pts',(-70.8799113821452,5.0169288887379,0.));
#85345=CARTESIAN_POINT('Ctrl Pts',(-70.9014016283124,5.01166043620567,0.));
#85346=CARTESIAN_POINT('Ctrl Pts',(-70.9229320328589,5.00635892472513,0.));
#85347=CARTESIAN_POINT('Ctrl Pts',(-70.9445024378439,5.00102431929039,0.));
#85348=CARTESIAN_POINT('Ctrl Pts',(-70.9661126860773,4.99565658516913,0.));
#85349=CARTESIAN_POINT('Ctrl Pts',(-70.9877626211113,4.99025568790664,0.));
#85350=CARTESIAN_POINT('Ctrl Pts',(-71.0094520872377,4.98482159331863,0.));
#85351=CARTESIAN_POINT('Ctrl Pts',(-71.0311809294821,4.97935426748584,0.));
#85352=CARTESIAN_POINT('Ctrl Pts',(-71.0529489935961,4.97385367675158,0.));
#85353=CARTESIAN_POINT('Ctrl Pts',(-71.0747561260436,4.9683197877219,0.));
#85354=CARTESIAN_POINT('Ctrl Pts',(-71.0966021739907,4.96275256726765,0.));
#85355=CARTESIAN_POINT('Ctrl Pts',(-71.1184869853056,4.95715198251684,0.));
#85356=CARTESIAN_POINT('Ctrl Pts',(-71.1404104085552,4.95151800085101,0.));
#85357=CARTESIAN_POINT('Ctrl Pts',(-71.1623722930001,4.94585058990341,0.));
#85358=CARTESIAN_POINT('Ctrl Pts',(-71.1843724885847,4.94014971756114,0.));
#85359=CARTESIAN_POINT('Ctrl Pts',(-71.2064108459286,4.93441535196617,0.));
#85360=CARTESIAN_POINT('Ctrl Pts',(-71.2284872163273,4.92864746150732,0.));
#85361=CARTESIAN_POINT('Ctrl Pts',(-71.250601451747,4.92284601481721,0.));
#85362=CARTESIAN_POINT('Ctrl Pts',(-71.2727534048192,4.91701098077036,0.));
#85363=CARTESIAN_POINT('Ctrl Pts',(-71.294942928829,4.91114232848603,0.));
#85364=CARTESIAN_POINT('Ctrl Pts',(-71.3171698777084,4.90524002732778,0.));
#85365=CARTESIAN_POINT('Ctrl Pts',(-71.3394341060359,4.89930404689574,0.));
#85366=CARTESIAN_POINT('Ctrl Pts',(-71.3617354690325,4.89333435702413,0.));
#85367=CARTESIAN_POINT('Ctrl Pts',(-71.3840738225562,4.88733092777974,0.));
#85368=CARTESIAN_POINT('Ctrl Pts',(-71.4064490230899,4.88129372946551,0.));
#85369=CARTESIAN_POINT('Ctrl Pts',(-71.4288609277374,4.87522273261907,0.));
#85370=CARTESIAN_POINT('Ctrl Pts',(-71.4513093942255,4.86911790800549,0.));
#85371=CARTESIAN_POINT('Ctrl Pts',(-71.4737942808982,4.86297922661502,0.));
#85372=CARTESIAN_POINT('Ctrl Pts',(-71.4963154467113,4.8568066596618,0.));
#85373=CARTESIAN_POINT('Ctrl Pts',(-71.5188727512197,4.8506001785878,0.));
#85374=CARTESIAN_POINT('Ctrl Pts',(-71.5414660545739,4.84435975506048,0.));
#85375=CARTESIAN_POINT('Ctrl Pts',(-71.564095217521,4.83808536096583,0.));
#85376=CARTESIAN_POINT('Ctrl Pts',(-71.5867601014,4.83177696840637,0.));
#85377=CARTESIAN_POINT('Ctrl Pts',(-71.6094605681366,4.82543454970026,0.));
#85378=CARTESIAN_POINT('Ctrl Pts',(-71.6321964802326,4.81905807738557,0.));
#85379=CARTESIAN_POINT('Ctrl Pts',(-71.6549677007613,4.81264752421732,0.));
#85380=CARTESIAN_POINT('Ctrl Pts',(-71.6777740933705,4.80620286316088,0.));
#85381=CARTESIAN_POINT('Ctrl Pts',(-71.7006155222766,4.79972406739013,0.));
#85382=CARTESIAN_POINT('Ctrl Pts',(-71.7234918522604,4.79321111028671,0.));
#85383=CARTESIAN_POINT('Ctrl Pts',(-71.7464029486552,4.7866639654445,0.));
#85384=CARTESIAN_POINT('Ctrl Pts',(-71.7693486773449,4.78008260666642,0.));
#85385=CARTESIAN_POINT('Ctrl Pts',(-71.7923289047636,4.77346700795787,0.));
#85386=CARTESIAN_POINT('Ctrl Pts',(-71.8153434978924,4.76681714352503,0.));
#85387=CARTESIAN_POINT('Ctrl Pts',(-71.8383923242533,4.76013298777422,0.));
#85388=CARTESIAN_POINT('Ctrl Pts',(-71.8614752519008,4.7534145153167,0.));
#85389=CARTESIAN_POINT('Ctrl Pts',(-71.8845921494186,4.74666170096545,0.));
#85390=CARTESIAN_POINT('Ctrl Pts',(-71.9077428859207,4.7398745197286,0.));
#85391=CARTESIAN_POINT('Ctrl Pts',(-71.9309273310469,4.73305294680783,0.));
#85392=CARTESIAN_POINT('Ctrl Pts',(-71.9541453549582,4.72619695759778,0.));
#85393=CARTESIAN_POINT('Ctrl Pts',(-71.9773968283267,4.7193065276908,0.));
#85394=CARTESIAN_POINT('Ctrl Pts',(-72.0006816223335,4.7123816328741,0.));
#85395=CARTESIAN_POINT('Ctrl Pts',(-72.0239996086694,4.70542224912312,0.));
#85396=CARTESIAN_POINT('Ctrl Pts',(-72.047350659532,4.69842835259997,0.));
#85397=CARTESIAN_POINT('Ctrl Pts',(-72.070734647621,4.69139991965279,0.));
#85398=CARTESIAN_POINT('Ctrl Pts',(-72.0941514461283,4.6843369268206,0.));
#85399=CARTESIAN_POINT('Ctrl Pts',(-72.1176009287349,4.67723935083087,0.));
#85400=CARTESIAN_POINT('Ctrl Pts',(-72.1410829696129,4.6701071685928,0.));
#85401=CARTESIAN_POINT('Ctrl Pts',(-72.1645974434218,4.6629403571957,0.));
#85402=CARTESIAN_POINT('Ctrl Pts',(-72.1881442253052,4.65573889390824,0.));
#85403=CARTESIAN_POINT('Ctrl Pts',(-72.2117231908816,4.64850275618324,0.));
#85404=CARTESIAN_POINT('Ctrl Pts',(-72.2353342162408,4.64123192165627,0.));
#85405=CARTESIAN_POINT('Ctrl Pts',(-72.2589771779447,4.63392636813842,0.));
#85406=CARTESIAN_POINT('Ctrl Pts',(-72.2826519530254,4.62658607361465,0.));
#85407=CARTESIAN_POINT('Ctrl Pts',(-72.306358418981,4.61921101624294,0.));
#85408=CARTESIAN_POINT('Ctrl Pts',(-72.330096453767,4.61180117435868,0.));
#85409=CARTESIAN_POINT('Ctrl Pts',(-72.3538659357932,4.60435652647463,0.));
#85410=CARTESIAN_POINT('Ctrl Pts',(-72.3776667439244,4.5968770512734,0.));
#85411=CARTESIAN_POINT('Ctrl Pts',(-72.4014987574789,4.5893627276055,0.));
#85412=CARTESIAN_POINT('Ctrl Pts',(-72.4253618562249,4.5818135344885,0.));
#85413=CARTESIAN_POINT('Ctrl Pts',(-72.449255920373,4.57422945111094,0.));
#85414=CARTESIAN_POINT('Ctrl Pts',(-72.473180830571,4.56661045683366,0.));
#85415=CARTESIAN_POINT('Ctrl Pts',(-72.4971364679055,4.55895653118213,0.));
#85416=CARTESIAN_POINT('Ctrl Pts',(-72.5211227138997,4.55126765384402,0.));
#85417=CARTESIAN_POINT('Ctrl Pts',(-72.5451394505106,4.54354380466824,0.));
#85418=CARTESIAN_POINT('Ctrl Pts',(-72.5691865601225,4.53578496366801,0.));
#85419=CARTESIAN_POINT('Ctrl Pts',(-72.5932639255406,4.5279911110239,0.));
#85420=CARTESIAN_POINT('Ctrl Pts',(-72.6173714299935,4.52016222707632,0.));
#85421=CARTESIAN_POINT('Ctrl Pts',(-72.6415089571314,4.51229829232259,0.));
#85422=CARTESIAN_POINT('Ctrl Pts',(-72.6656763910241,4.50439928741604,0.));
#85423=CARTESIAN_POINT('Ctrl Pts',(-72.689873616155,4.49646519316821,0.));
#85424=CARTESIAN_POINT('Ctrl Pts',(-72.7141005174153,4.48849599055353,0.));
#85425=CARTESIAN_POINT('Ctrl Pts',(-72.7383569801042,4.48049166070223,0.));
#85426=CARTESIAN_POINT('Ctrl Pts',(-72.7626428899287,4.47245218489622,0.));
#85427=CARTESIAN_POINT('Ctrl Pts',(-72.7869581329994,4.46437754456795,0.));
#85428=CARTESIAN_POINT('Ctrl Pts',(-72.8113025958258,4.45626772130138,0.));
#85429=CARTESIAN_POINT('Ctrl Pts',(-72.8356761653064,4.44812269683724,0.));
#85430=CARTESIAN_POINT('Ctrl Pts',(-72.8600787287316,4.43994245306804,0.));
#85431=CARTESIAN_POINT('Ctrl Pts',(-72.8845101737856,4.43172697203341,0.));
#85432=CARTESIAN_POINT('Ctrl Pts',(-72.9089703885463,4.42347623591941,0.));
#85433=CARTESIAN_POINT('Ctrl Pts',(-72.9334592614828,4.41519022705926,0.));
#85434=CARTESIAN_POINT('Ctrl Pts',(-72.9579766814495,4.40686892793964,0.));
#85435=CARTESIAN_POINT('Ctrl Pts',(-72.9825225376839,4.3985123211973,0.));
#85436=CARTESIAN_POINT('Ctrl Pts',(-73.0070967198033,4.39012038961144,0.));
#85437=CARTESIAN_POINT('Ctrl Pts',(-73.031699117799,4.38169311610153,0.));
#85438=CARTESIAN_POINT('Ctrl Pts',(-73.0563296220301,4.37323048372606,0.));
#85439=CARTESIAN_POINT('Ctrl Pts',(-73.0809881232111,4.36473247568638,0.));
#85440=CARTESIAN_POINT('Ctrl Pts',(-73.1056745124099,4.35619907532715,0.));
#85441=CARTESIAN_POINT('Ctrl Pts',(-73.1303886810602,4.34763026613154,0.));
#85442=CARTESIAN_POINT('Ctrl Pts',(-73.1551305209692,4.33902603172139,0.));
#85443=CARTESIAN_POINT('Ctrl Pts',(-73.1798999243234,4.33038635585878,0.));
#85444=CARTESIAN_POINT('Ctrl Pts',(-73.204696783693,4.32171122245218,0.));
#85445=CARTESIAN_POINT('Ctrl Pts',(-73.2295209920319,4.31300061556102,0.));
#85446=CARTESIAN_POINT('Ctrl Pts',(-73.2543724426562,4.30425451938233,0.));
#85447=CARTESIAN_POINT('Ctrl Pts',(-73.2792510292243,4.29547291824288,0.));
#85448=CARTESIAN_POINT('Ctrl Pts',(-73.3041566457134,4.28665579659301,0.));
#85449=CARTESIAN_POINT('Ctrl Pts',(-73.3290891863959,4.27780313900391,0.));
#85450=CARTESIAN_POINT('Ctrl Pts',(-73.354048545808,4.26891493016703,0.));
#85451=CARTESIAN_POINT('Ctrl Pts',(-73.3790346187953,4.25999115489904,0.));
#85452=CARTESIAN_POINT('Ctrl Pts',(-73.4040473005603,4.25103179814891,0.));
#85453=CARTESIAN_POINT('Ctrl Pts',(-73.4290864867103,4.24203684500941,0.));
#85454=CARTESIAN_POINT('Ctrl Pts',(-73.4541520732943,4.23300628072757,0.));
#85455=CARTESIAN_POINT('Ctrl Pts',(-73.4792439568624,4.22394009072752,0.));
#85456=CARTESIAN_POINT('Ctrl Pts',(-73.5043620344107,4.21483826059436,0.));
#85457=CARTESIAN_POINT('Ctrl Pts',(-73.5295062032621,4.20570077603727,0.));
#85458=CARTESIAN_POINT('Ctrl Pts',(-73.554676360957,4.19652762286126,0.));
#85459=CARTESIAN_POINT('Ctrl Pts',(-73.5798724051519,4.18731878694237,0.));
#85460=CARTESIAN_POINT('Ctrl Pts',(-73.6050942334773,4.17807425419816,0.));
#85461=CARTESIAN_POINT('Ctrl Pts',(-73.6303417435262,4.16879401058786,0.));
#85462=CARTESIAN_POINT('Ctrl Pts',(-73.6556148331504,4.1594780421779,0.));
#85463=CARTESIAN_POINT('Ctrl Pts',(-73.6809134006909,4.15012633519727,0.));
#85464=CARTESIAN_POINT('Ctrl Pts',(-73.7062373452344,4.14073887610154,0.));
#85465=CARTESIAN_POINT('Ctrl Pts',(-73.7315865668508,4.13131565163574,0.));
#85466=CARTESIAN_POINT('Ctrl Pts',(-73.7569609668501,4.1218566489055,0.));
#85467=CARTESIAN_POINT('Ctrl Pts',(-73.7823604472126,4.1123618552278,0.));
#85468=CARTESIAN_POINT('Ctrl Pts',(-73.8077849100314,4.10283125798724,0.));
#85469=CARTESIAN_POINT('Ctrl Pts',(-73.8332342568978,4.09326484448231,0.));
#85470=CARTESIAN_POINT('Ctrl Pts',(-73.8587083884208,4.08366260180679,0.));
#85471=CARTESIAN_POINT('Ctrl Pts',(-73.884207203405,4.07402451665252,0.));
#85472=CARTESIAN_POINT('Ctrl Pts',(-73.9097305995173,4.06435057547334,0.));
#85473=CARTESIAN_POINT('Ctrl Pts',(-73.9352784747665,4.05464076484761,0.));
#85474=CARTESIAN_POINT('Ctrl Pts',(-73.9608507287943,4.04489507179963,0.));
#85475=CARTESIAN_POINT('Ctrl Pts',(-73.9864472641025,4.03511348410659,0.));
#85476=CARTESIAN_POINT('Ctrl Pts',(-74.0120679876396,4.02529599070084,0.));
#85477=CARTESIAN_POINT('Ctrl Pts',(-74.0377128111754,4.01544258176692,0.));
#85478=CARTESIAN_POINT('Ctrl Pts',(-74.0597159781919,4.00696550627606,0.));
#85479=CARTESIAN_POINT('Ctrl Pts',(-74.0765982943431,4.0004468971249,0.));
#85480=CARTESIAN_POINT('Ctrl Pts',(-74.0883491449662,3.99590266747766,0.));
#85481=CARTESIAN_POINT('Ctrl Pts',(-74.0949615399274,3.99334334446571,0.));
#85482=CARTESIAN_POINT('Ctrl Pts',(-74.0964320765797,3.99277406492179,0.));
#85483=CARTESIAN_POINT('',(-69.8028570375097,5.24987136994592,12.));
#85484=CARTESIAN_POINT('',(-69.8028570375097,5.24987136994592,0.));
#85485=CARTESIAN_POINT('Ctrl Pts',(-74.0964320765797,3.99277406492181,12.));
#85486=CARTESIAN_POINT('Ctrl Pts',(-74.0949615399273,3.99334334446573,12.));
#85487=CARTESIAN_POINT('Ctrl Pts',(-74.0883491449662,3.99590266747768,12.));
#85488=CARTESIAN_POINT('Ctrl Pts',(-74.0765982943431,4.00044689712491,12.));
#85489=CARTESIAN_POINT('Ctrl Pts',(-74.0597159781919,4.00696550627606,12.));
#85490=CARTESIAN_POINT('Ctrl Pts',(-74.0377128111754,4.01544258176692,12.));
#85491=CARTESIAN_POINT('Ctrl Pts',(-74.0120679876396,4.02529599070084,12.));
#85492=CARTESIAN_POINT('Ctrl Pts',(-73.9864472641025,4.03511348410659,12.));
#85493=CARTESIAN_POINT('Ctrl Pts',(-73.9608507287943,4.04489507179963,12.));
#85494=CARTESIAN_POINT('Ctrl Pts',(-73.9352784747665,4.05464076484761,12.));
#85495=CARTESIAN_POINT('Ctrl Pts',(-73.9097305995173,4.06435057547334,12.));
#85496=CARTESIAN_POINT('Ctrl Pts',(-73.884207203405,4.07402451665252,12.));
#85497=CARTESIAN_POINT('Ctrl Pts',(-73.8587083884208,4.08366260180679,12.));
#85498=CARTESIAN_POINT('Ctrl Pts',(-73.8332342568978,4.09326484448231,12.));
#85499=CARTESIAN_POINT('Ctrl Pts',(-73.8077849100314,4.10283125798724,12.));
#85500=CARTESIAN_POINT('Ctrl Pts',(-73.7823604472126,4.1123618552278,12.));
#85501=CARTESIAN_POINT('Ctrl Pts',(-73.7569609668501,4.1218566489055,12.));
#85502=CARTESIAN_POINT('Ctrl Pts',(-73.7315865668508,4.13131565163574,12.));
#85503=CARTESIAN_POINT('Ctrl Pts',(-73.7062373452344,4.14073887610154,12.));
#85504=CARTESIAN_POINT('Ctrl Pts',(-73.6809134006909,4.15012633519727,12.));
#85505=CARTESIAN_POINT('Ctrl Pts',(-73.6556148331504,4.1594780421779,12.));
#85506=CARTESIAN_POINT('Ctrl Pts',(-73.6303417435262,4.16879401058786,12.));
#85507=CARTESIAN_POINT('Ctrl Pts',(-73.6050942334773,4.17807425419816,12.));
#85508=CARTESIAN_POINT('Ctrl Pts',(-73.5798724051519,4.18731878694237,12.));
#85509=CARTESIAN_POINT('Ctrl Pts',(-73.554676360957,4.19652762286126,12.));
#85510=CARTESIAN_POINT('Ctrl Pts',(-73.5295062032621,4.20570077603727,12.));
#85511=CARTESIAN_POINT('Ctrl Pts',(-73.5043620344107,4.21483826059436,12.));
#85512=CARTESIAN_POINT('Ctrl Pts',(-73.4792439568624,4.22394009072752,12.));
#85513=CARTESIAN_POINT('Ctrl Pts',(-73.4541520732943,4.23300628072757,12.));
#85514=CARTESIAN_POINT('Ctrl Pts',(-73.4290864867103,4.24203684500941,12.));
#85515=CARTESIAN_POINT('Ctrl Pts',(-73.4040473005603,4.25103179814891,12.));
#85516=CARTESIAN_POINT('Ctrl Pts',(-73.3790346187953,4.25999115489904,12.));
#85517=CARTESIAN_POINT('Ctrl Pts',(-73.354048545808,4.26891493016703,12.));
#85518=CARTESIAN_POINT('Ctrl Pts',(-73.3290891863959,4.27780313900391,12.));
#85519=CARTESIAN_POINT('Ctrl Pts',(-73.3041566457134,4.28665579659301,12.));
#85520=CARTESIAN_POINT('Ctrl Pts',(-73.2792510292243,4.29547291824288,12.));
#85521=CARTESIAN_POINT('Ctrl Pts',(-73.2543724426562,4.30425451938233,12.));
#85522=CARTESIAN_POINT('Ctrl Pts',(-73.2295209920319,4.31300061556102,12.));
#85523=CARTESIAN_POINT('Ctrl Pts',(-73.204696783693,4.32171122245218,12.));
#85524=CARTESIAN_POINT('Ctrl Pts',(-73.1798999243234,4.33038635585878,12.));
#85525=CARTESIAN_POINT('Ctrl Pts',(-73.1551305209692,4.33902603172139,12.));
#85526=CARTESIAN_POINT('Ctrl Pts',(-73.1303886810602,4.34763026613154,12.));
#85527=CARTESIAN_POINT('Ctrl Pts',(-73.1056745124099,4.35619907532715,12.));
#85528=CARTESIAN_POINT('Ctrl Pts',(-73.0809881232111,4.36473247568638,12.));
#85529=CARTESIAN_POINT('Ctrl Pts',(-73.0563296220301,4.37323048372606,12.));
#85530=CARTESIAN_POINT('Ctrl Pts',(-73.031699117799,4.38169311610153,12.));
#85531=CARTESIAN_POINT('Ctrl Pts',(-73.0070967198033,4.39012038961144,12.));
#85532=CARTESIAN_POINT('Ctrl Pts',(-72.9825225376839,4.3985123211973,12.));
#85533=CARTESIAN_POINT('Ctrl Pts',(-72.9579766814495,4.40686892793964,12.));
#85534=CARTESIAN_POINT('Ctrl Pts',(-72.9334592614828,4.41519022705926,12.));
#85535=CARTESIAN_POINT('Ctrl Pts',(-72.9089703885463,4.42347623591941,12.));
#85536=CARTESIAN_POINT('Ctrl Pts',(-72.8845101737856,4.43172697203341,12.));
#85537=CARTESIAN_POINT('Ctrl Pts',(-72.8600787287316,4.43994245306804,12.));
#85538=CARTESIAN_POINT('Ctrl Pts',(-72.8356761653064,4.44812269683724,12.));
#85539=CARTESIAN_POINT('Ctrl Pts',(-72.8113025958258,4.45626772130138,12.));
#85540=CARTESIAN_POINT('Ctrl Pts',(-72.7869581329994,4.46437754456795,12.));
#85541=CARTESIAN_POINT('Ctrl Pts',(-72.7626428899287,4.47245218489622,12.));
#85542=CARTESIAN_POINT('Ctrl Pts',(-72.7383569801042,4.48049166070223,12.));
#85543=CARTESIAN_POINT('Ctrl Pts',(-72.7141005174153,4.48849599055353,12.));
#85544=CARTESIAN_POINT('Ctrl Pts',(-72.689873616155,4.49646519316821,12.));
#85545=CARTESIAN_POINT('Ctrl Pts',(-72.6656763910241,4.50439928741604,12.));
#85546=CARTESIAN_POINT('Ctrl Pts',(-72.6415089571314,4.51229829232259,12.));
#85547=CARTESIAN_POINT('Ctrl Pts',(-72.6173714299935,4.52016222707632,12.));
#85548=CARTESIAN_POINT('Ctrl Pts',(-72.5932639255406,4.5279911110239,12.));
#85549=CARTESIAN_POINT('Ctrl Pts',(-72.5691865601225,4.53578496366801,12.));
#85550=CARTESIAN_POINT('Ctrl Pts',(-72.5451394505106,4.54354380466824,12.));
#85551=CARTESIAN_POINT('Ctrl Pts',(-72.5211227138997,4.55126765384402,12.));
#85552=CARTESIAN_POINT('Ctrl Pts',(-72.4971364679055,4.55895653118213,12.));
#85553=CARTESIAN_POINT('Ctrl Pts',(-72.473180830571,4.56661045683366,12.));
#85554=CARTESIAN_POINT('Ctrl Pts',(-72.449255920373,4.57422945111094,12.));
#85555=CARTESIAN_POINT('Ctrl Pts',(-72.4253618562249,4.5818135344885,12.));
#85556=CARTESIAN_POINT('Ctrl Pts',(-72.4014987574789,4.5893627276055,12.));
#85557=CARTESIAN_POINT('Ctrl Pts',(-72.3776667439244,4.5968770512734,12.));
#85558=CARTESIAN_POINT('Ctrl Pts',(-72.3538659357932,4.60435652647463,12.));
#85559=CARTESIAN_POINT('Ctrl Pts',(-72.330096453767,4.61180117435868,12.));
#85560=CARTESIAN_POINT('Ctrl Pts',(-72.306358418981,4.61921101624294,12.));
#85561=CARTESIAN_POINT('Ctrl Pts',(-72.2826519530254,4.62658607361465,12.));
#85562=CARTESIAN_POINT('Ctrl Pts',(-72.2589771779447,4.63392636813842,12.));
#85563=CARTESIAN_POINT('Ctrl Pts',(-72.2353342162408,4.64123192165627,12.));
#85564=CARTESIAN_POINT('Ctrl Pts',(-72.2117231908816,4.64850275618324,12.));
#85565=CARTESIAN_POINT('Ctrl Pts',(-72.1881442253052,4.65573889390824,12.));
#85566=CARTESIAN_POINT('Ctrl Pts',(-72.1645974434218,4.6629403571957,12.));
#85567=CARTESIAN_POINT('Ctrl Pts',(-72.1410829696129,4.6701071685928,12.));
#85568=CARTESIAN_POINT('Ctrl Pts',(-72.1176009287349,4.67723935083087,12.));
#85569=CARTESIAN_POINT('Ctrl Pts',(-72.0941514461283,4.6843369268206,12.));
#85570=CARTESIAN_POINT('Ctrl Pts',(-72.070734647621,4.69139991965279,12.));
#85571=CARTESIAN_POINT('Ctrl Pts',(-72.047350659532,4.69842835259997,12.));
#85572=CARTESIAN_POINT('Ctrl Pts',(-72.0239996086694,4.70542224912312,12.));
#85573=CARTESIAN_POINT('Ctrl Pts',(-72.0006816223335,4.7123816328741,12.));
#85574=CARTESIAN_POINT('Ctrl Pts',(-71.9773968283267,4.7193065276908,12.));
#85575=CARTESIAN_POINT('Ctrl Pts',(-71.9541453549582,4.72619695759778,12.));
#85576=CARTESIAN_POINT('Ctrl Pts',(-71.9309273310469,4.73305294680783,12.));
#85577=CARTESIAN_POINT('Ctrl Pts',(-71.9077428859207,4.7398745197286,12.));
#85578=CARTESIAN_POINT('Ctrl Pts',(-71.8845921494186,4.74666170096545,12.));
#85579=CARTESIAN_POINT('Ctrl Pts',(-71.8614752519008,4.7534145153167,12.));
#85580=CARTESIAN_POINT('Ctrl Pts',(-71.8383923242533,4.76013298777422,12.));
#85581=CARTESIAN_POINT('Ctrl Pts',(-71.8153434978924,4.76681714352503,12.));
#85582=CARTESIAN_POINT('Ctrl Pts',(-71.7923289047636,4.77346700795787,12.));
#85583=CARTESIAN_POINT('Ctrl Pts',(-71.7693486773449,4.78008260666642,12.));
#85584=CARTESIAN_POINT('Ctrl Pts',(-71.7464029486552,4.7866639654445,12.));
#85585=CARTESIAN_POINT('Ctrl Pts',(-71.7234918522604,4.79321111028671,12.));
#85586=CARTESIAN_POINT('Ctrl Pts',(-71.7006155222766,4.79972406739013,12.));
#85587=CARTESIAN_POINT('Ctrl Pts',(-71.6777740933705,4.80620286316088,12.));
#85588=CARTESIAN_POINT('Ctrl Pts',(-71.6549677007613,4.81264752421732,12.));
#85589=CARTESIAN_POINT('Ctrl Pts',(-71.6321964802326,4.81905807738557,12.));
#85590=CARTESIAN_POINT('Ctrl Pts',(-71.6094605681366,4.82543454970026,12.));
#85591=CARTESIAN_POINT('Ctrl Pts',(-71.5867601014,4.83177696840637,12.));
#85592=CARTESIAN_POINT('Ctrl Pts',(-71.564095217521,4.83808536096583,12.));
#85593=CARTESIAN_POINT('Ctrl Pts',(-71.5414660545739,4.84435975506048,12.));
#85594=CARTESIAN_POINT('Ctrl Pts',(-71.5188727512197,4.8506001785878,12.));
#85595=CARTESIAN_POINT('Ctrl Pts',(-71.4963154467113,4.8568066596618,12.));
#85596=CARTESIAN_POINT('Ctrl Pts',(-71.4737942808982,4.86297922661502,12.));
#85597=CARTESIAN_POINT('Ctrl Pts',(-71.4513093942255,4.86911790800549,12.));
#85598=CARTESIAN_POINT('Ctrl Pts',(-71.4288609277374,4.87522273261907,12.));
#85599=CARTESIAN_POINT('Ctrl Pts',(-71.4064490230899,4.88129372946551,12.));
#85600=CARTESIAN_POINT('Ctrl Pts',(-71.3840738225562,4.88733092777974,12.));
#85601=CARTESIAN_POINT('Ctrl Pts',(-71.3617354690325,4.89333435702413,12.));
#85602=CARTESIAN_POINT('Ctrl Pts',(-71.3394341060359,4.89930404689574,12.));
#85603=CARTESIAN_POINT('Ctrl Pts',(-71.3171698777084,4.90524002732778,12.));
#85604=CARTESIAN_POINT('Ctrl Pts',(-71.294942928829,4.91114232848603,12.));
#85605=CARTESIAN_POINT('Ctrl Pts',(-71.2727534048192,4.91701098077036,12.));
#85606=CARTESIAN_POINT('Ctrl Pts',(-71.250601451747,4.92284601481721,12.));
#85607=CARTESIAN_POINT('Ctrl Pts',(-71.2284872163273,4.92864746150732,12.));
#85608=CARTESIAN_POINT('Ctrl Pts',(-71.2064108459286,4.93441535196617,12.));
#85609=CARTESIAN_POINT('Ctrl Pts',(-71.1843724885847,4.94014971756114,12.));
#85610=CARTESIAN_POINT('Ctrl Pts',(-71.1623722930001,4.94585058990341,12.));
#85611=CARTESIAN_POINT('Ctrl Pts',(-71.1404104085552,4.95151800085101,12.));
#85612=CARTESIAN_POINT('Ctrl Pts',(-71.1184869853056,4.95715198251684,12.));
#85613=CARTESIAN_POINT('Ctrl Pts',(-71.0966021739907,4.96275256726765,12.));
#85614=CARTESIAN_POINT('Ctrl Pts',(-71.0747561260436,4.9683197877219,12.));
#85615=CARTESIAN_POINT('Ctrl Pts',(-71.0529489935961,4.97385367675158,12.));
#85616=CARTESIAN_POINT('Ctrl Pts',(-71.0311809294821,4.97935426748584,12.));
#85617=CARTESIAN_POINT('Ctrl Pts',(-71.0094520872377,4.98482159331863,12.));
#85618=CARTESIAN_POINT('Ctrl Pts',(-70.9877626211113,4.99025568790664,12.));
#85619=CARTESIAN_POINT('Ctrl Pts',(-70.9661126860773,4.99565658516913,12.));
#85620=CARTESIAN_POINT('Ctrl Pts',(-70.9445024378439,5.00102431929039,12.));
#85621=CARTESIAN_POINT('Ctrl Pts',(-70.9229320328589,5.00635892472513,12.));
#85622=CARTESIAN_POINT('Ctrl Pts',(-70.9014016283124,5.01166043620567,12.));
#85623=CARTESIAN_POINT('Ctrl Pts',(-70.8799113821452,5.0169288887379,12.));
#85624=CARTESIAN_POINT('Ctrl Pts',(-70.8584614530519,5.0221643176006,12.));
#85625=CARTESIAN_POINT('Ctrl Pts',(-70.8370520004843,5.02736675834692,12.));
#85626=CARTESIAN_POINT('Ctrl Pts',(-70.8156831846488,5.0325362468094,12.));
#85627=CARTESIAN_POINT('Ctrl Pts',(-70.7943551665059,5.03767281910479,12.));
#85628=CARTESIAN_POINT('Ctrl Pts',(-70.7730681077983,5.04277651163349,12.));
#85629=CARTESIAN_POINT('Ctrl Pts',(-70.7518221710706,5.04784736108346,12.));
#85630=CARTESIAN_POINT('Ctrl Pts',(-70.7306175196863,5.05288540443482,12.));
#85631=CARTESIAN_POINT('Ctrl Pts',(-70.7094543178438,5.05789067897057,12.));
#85632=CARTESIAN_POINT('Ctrl Pts',(-70.6883327305784,5.06286322227819,12.));
#85633=CARTESIAN_POINT('Ctrl Pts',(-70.6672529237455,5.06780307224071,12.));
#85634=CARTESIAN_POINT('Ctrl Pts',(-70.6462150640015,5.07271026703354,12.));
#85635=CARTESIAN_POINT('Ctrl Pts',(-70.6252193187878,5.07758484512302,12.));
#85636=CARTESIAN_POINT('Ctrl Pts',(-70.6042658562923,5.08242684526686,12.));
#85637=CARTESIAN_POINT('Ctrl Pts',(-70.5833548455014,5.08723630652272,12.));
#85638=CARTESIAN_POINT('Ctrl Pts',(-70.5624864562824,5.09201326826134,12.));
#85639=CARTESIAN_POINT('Ctrl Pts',(-70.5416608594526,5.09675777018182,12.));
#85640=CARTESIAN_POINT('Ctrl Pts',(-70.5208782268497,5.1014698523294,12.));
#85641=CARTESIAN_POINT('Ctrl Pts',(-70.500138731399,5.10614955511663,12.));
#85642=CARTESIAN_POINT('Ctrl Pts',(-70.4794425469825,5.11079691929213,12.));
#85643=CARTESIAN_POINT('Ctrl Pts',(-70.458789848296,5.11541198590932,12.));
#85644=CARTESIAN_POINT('Ctrl Pts',(-70.4381808107245,5.11999479630211,12.));
#85645=CARTESIAN_POINT('Ctrl Pts',(-70.417615610161,5.12454539205328,12.));
#85646=CARTESIAN_POINT('Ctrl Pts',(-70.3970944229851,5.12906381499456,12.));
#85647=CARTESIAN_POINT('Ctrl Pts',(-70.3766174264757,5.13355010728567,12.));
#85648=CARTESIAN_POINT('Ctrl Pts',(-70.3561847991714,5.13800431148903,12.));
#85649=CARTESIAN_POINT('Ctrl Pts',(-70.3357967211796,5.14242647063479,12.));
#85650=CARTESIAN_POINT('Ctrl Pts',(-70.3154533746736,5.1468166283308,12.));
#85651=CARTESIAN_POINT('Ctrl Pts',(-70.2951549435512,5.15117482869254,12.));
#85652=CARTESIAN_POINT('Ctrl Pts',(-70.2749016125105,5.15550111614859,12.));
#85653=CARTESIAN_POINT('Ctrl Pts',(-70.2546935662722,5.15979553528203,12.));
#85654=CARTESIAN_POINT('Ctrl Pts',(-70.2345309887833,5.16405813066976,12.));
#85655=CARTESIAN_POINT('Ctrl Pts',(-70.2144140622953,5.16828894670108,12.));
#85656=CARTESIAN_POINT('Ctrl Pts',(-70.1943429691167,5.17248802793389,12.));
#85657=CARTESIAN_POINT('Ctrl Pts',(-70.1743178937077,5.17665541952382,12.));
#85658=CARTESIAN_POINT('Ctrl Pts',(-70.1543390243892,5.18079116757666,12.));
#85659=CARTESIAN_POINT('Ctrl Pts',(-70.1344065558145,5.18489531966264,12.));
#85660=CARTESIAN_POINT('Ctrl Pts',(-70.1145206891885,5.18896792486565,12.));
#85661=CARTESIAN_POINT('Ctrl Pts',(-70.0946816270997,5.19300903271579,12.));
#85662=CARTESIAN_POINT('Ctrl Pts',(-70.0748895689729,5.19701869225528,12.));
#85663=CARTESIAN_POINT('Ctrl Pts',(-70.0551447071082,5.20099695122656,12.));
#85664=CARTESIAN_POINT('Ctrl Pts',(-70.0354472203546,5.20494385478025,12.));
#85665=CARTESIAN_POINT('Ctrl Pts',(-70.0157972802182,5.20885944672836,12.));
#85666=CARTESIAN_POINT('Ctrl Pts',(-69.9961950629965,5.21274377203259,12.));
#85667=CARTESIAN_POINT('Ctrl Pts',(-69.9766407595385,5.21659687881139,12.));
#85668=CARTESIAN_POINT('Ctrl Pts',(-69.9571345870076,5.2204188207572,12.));
#85669=CARTESIAN_POINT('Ctrl Pts',(-69.9376767969095,5.22420965879981,12.));
#85670=CARTESIAN_POINT('Ctrl Pts',(-69.9182676502048,5.22796945602793,12.));
#85671=CARTESIAN_POINT('Ctrl Pts',(-69.8989073936688,5.23169827290555,12.));
#85672=CARTESIAN_POINT('Ctrl Pts',(-69.8795962381599,5.2353961627962,12.));
#85673=CARTESIAN_POINT('Ctrl Pts',(-69.8603343302743,5.23906316634802,12.));
#85674=CARTESIAN_POINT('Ctrl Pts',(-69.841121750752,5.24269931054569,12.));
#85675=CARTESIAN_POINT('Ctrl Pts',(-69.8257911792159,5.2455835515975,12.));
#85676=CARTESIAN_POINT('Ctrl Pts',(-69.8143154684204,5.24773285666376,12.));
#85677=CARTESIAN_POINT('Ctrl Pts',(-69.8066748687772,5.24915955997427,12.));
#85678=CARTESIAN_POINT('Ctrl Pts',(-69.8028570375097,5.24987136994592,12.));
#85679=CARTESIAN_POINT('Ctrl Pts',(-74.1624659714955,2.48034921844904,-2.77555756156289E-15));
#85680=CARTESIAN_POINT('Ctrl Pts',(-74.1624659714955,2.48034921844904,4.));
#85681=CARTESIAN_POINT('Ctrl Pts',(-74.1624659714955,2.48034921844904,8.));
#85682=CARTESIAN_POINT('Ctrl Pts',(-74.1624659714955,2.48034921844904,12.));
#85683=CARTESIAN_POINT('Ctrl Pts',(-74.2610905805698,2.52879860312848,-2.77555756156289E-15));
#85684=CARTESIAN_POINT('Ctrl Pts',(-74.2610905805698,2.52879860312848,4.));
#85685=CARTESIAN_POINT('Ctrl Pts',(-74.2610905805698,2.52879860312849,8.));
#85686=CARTESIAN_POINT('Ctrl Pts',(-74.2610905805698,2.52879860312849,12.));
#85687=CARTESIAN_POINT('Ctrl Pts',(-74.4041075779819,2.67239300265259,-2.55632103913301E-15));
#85688=CARTESIAN_POINT('Ctrl Pts',(-74.4041075779819,2.67239300265259,4.));
#85689=CARTESIAN_POINT('Ctrl Pts',(-74.4041075779819,2.67239300265259,7.99999999999999));
#85690=CARTESIAN_POINT('Ctrl Pts',(-74.4041075779819,2.67239300265259,12.));
#85691=CARTESIAN_POINT('Ctrl Pts',(-74.444876171298,2.86656650944678,-2.03572402097153E-15));
#85692=CARTESIAN_POINT('Ctrl Pts',(-74.444876171298,2.86656650944678,4.));
#85693=CARTESIAN_POINT('Ctrl Pts',(-74.444876171298,2.86656650944676,8.00000000000001));
#85694=CARTESIAN_POINT('Ctrl Pts',(-74.444876171298,2.86656650944676,12.));
#85695=CARTESIAN_POINT('Ctrl Pts',(-74.4416140848739,2.94891377268016,-1.78476208028845E-15));
#85696=CARTESIAN_POINT('Ctrl Pts',(-74.4416140848739,2.94891377268016,4.));
#85697=CARTESIAN_POINT('Ctrl Pts',(-74.4416140848739,2.94891377268014,8.));
#85698=CARTESIAN_POINT('Ctrl Pts',(-74.4416140848739,2.94891377268014,12.));
#85699=CARTESIAN_POINT('',(-74.1624659714955,2.48034921844904,0.));
#85700=CARTESIAN_POINT('',(-74.4416140848739,2.94891377268016,0.));
#85701=CARTESIAN_POINT('Ctrl Pts',(-74.1624659714955,2.48034921844904,-9.71445146547012E-16));
#85702=CARTESIAN_POINT('Ctrl Pts',(-74.2610905805698,2.52879860312848,-9.71445146547012E-16));
#85703=CARTESIAN_POINT('Ctrl Pts',(-74.342814579091,2.61085254571368,-8.46167133729938E-16));
#85704=CARTESIAN_POINT('Ctrl Pts',(-74.3911513436217,2.70942211516259,-6.22485693735197E-16));
#85705=CARTESIAN_POINT('Ctrl Pts',(-74.4274039170197,2.78334929224927,-4.54724613739141E-16));
#85706=CARTESIAN_POINT('Ctrl Pts',(-74.444876171298,2.86656650944678,-2.31611605955647E-16));
#85707=CARTESIAN_POINT('Ctrl Pts',(-74.4416140848739,2.94891377268016,1.93503347274265E-17));
#85708=CARTESIAN_POINT('',(-74.4416140848739,2.94891377268014,12.));
#85709=CARTESIAN_POINT('Ctrl Pts',(-74.4416140848739,2.94891377268016,-1.78476208028845E-15));
#85710=CARTESIAN_POINT('Ctrl Pts',(-74.4416140848739,2.94891377268016,4.));
#85711=CARTESIAN_POINT('Ctrl Pts',(-74.4416140848739,2.94891377268014,8.));
#85712=CARTESIAN_POINT('Ctrl Pts',(-74.4416140848739,2.94891377268014,12.));
#85713=CARTESIAN_POINT('',(-74.1624659714955,2.48034921844905,12.));
#85714=CARTESIAN_POINT('Ctrl Pts',(-74.4416140848739,2.94891377268014,12.));
#85715=CARTESIAN_POINT('Ctrl Pts',(-74.444876171298,2.86656650944676,12.));
#85716=CARTESIAN_POINT('Ctrl Pts',(-74.4274039170196,2.78334929224926,12.));
#85717=CARTESIAN_POINT('Ctrl Pts',(-74.3911513436217,2.70942211516259,12.));
#85718=CARTESIAN_POINT('Ctrl Pts',(-74.342814579091,2.61085254571369,12.));
#85719=CARTESIAN_POINT('Ctrl Pts',(-74.2610905805698,2.52879860312849,12.));
#85720=CARTESIAN_POINT('Ctrl Pts',(-74.1624659714955,2.48034921844904,12.));
#85721=CARTESIAN_POINT('Ctrl Pts',(-74.1624659714955,2.48034921844904,12.));
#85722=CARTESIAN_POINT('Ctrl Pts',(-74.1624659714955,2.48034921844904,8.));
#85723=CARTESIAN_POINT('Ctrl Pts',(-74.1624659714955,2.48034921844904,4.));
#85724=CARTESIAN_POINT('Ctrl Pts',(-74.1624659714955,2.48034921844904,-2.77555756156289E-15));
#85725=CARTESIAN_POINT('Origin',(-3.74491326291036E-10,1.62512913209675E-11,
0.));
#85726=CARTESIAN_POINT('Origin',(-3.74491326291036E-10,1.62512913209675E-11,
12.));
#85727=CARTESIAN_POINT('Origin',(-3.74491326291036E-10,1.62512913209675E-11,
0.));
#85728=CARTESIAN_POINT('Ctrl Pts',(-73.8227522002498,10.0225374821206,0.));
#85729=CARTESIAN_POINT('Ctrl Pts',(-73.8227522002498,10.0225374821206,4.));
#85730=CARTESIAN_POINT('Ctrl Pts',(-73.8227522002498,10.0225374821206,8.));
#85731=CARTESIAN_POINT('Ctrl Pts',(-73.8227522002498,10.0225374821206,12.));
#85732=CARTESIAN_POINT('Ctrl Pts',(-73.8079696346554,10.1314210536418,0.));
#85733=CARTESIAN_POINT('Ctrl Pts',(-73.8079696346554,10.1314210536418,4.));
#85734=CARTESIAN_POINT('Ctrl Pts',(-73.8079696346554,10.1314210536418,8.00000000000001));
#85735=CARTESIAN_POINT('Ctrl Pts',(-73.8079696346554,10.1314210536418,12.));
#85736=CARTESIAN_POINT('Ctrl Pts',(-73.716956764919,10.3125002643521,-7.30802048705264E-17));
#85737=CARTESIAN_POINT('Ctrl Pts',(-73.716956764919,10.3125002643521,4.00000000000001));
#85738=CARTESIAN_POINT('Ctrl Pts',(-73.716956764919,10.3125002643521,7.99999999999999));
#85739=CARTESIAN_POINT('Ctrl Pts',(-73.716956764919,10.3125002643521,12.));
#85740=CARTESIAN_POINT('Ctrl Pts',(-73.5456341632194,10.4125694172281,-2.46611180232542E-16));
#85741=CARTESIAN_POINT('Ctrl Pts',(-73.5456341632194,10.4125694172281,3.99999999999999));
#85742=CARTESIAN_POINT('Ctrl Pts',(-73.5456341632194,10.4125694172281,8.00000000000001));
#85743=CARTESIAN_POINT('Ctrl Pts',(-73.5456341632194,10.4125694172281,12.));
#85744=CARTESIAN_POINT('Ctrl Pts',(-73.4664795929516,10.4355099267394,-3.30265160469984E-16));
#85745=CARTESIAN_POINT('Ctrl Pts',(-73.4664795929516,10.4355099267394,4.));
#85746=CARTESIAN_POINT('Ctrl Pts',(-73.4664795929516,10.4355099267394,8.));
#85747=CARTESIAN_POINT('Ctrl Pts',(-73.4664795929516,10.4355099267394,12.));
#85748=CARTESIAN_POINT('',(-73.8227522002498,10.0225374821206,0.));
#85749=CARTESIAN_POINT('',(-73.4664795929515,10.4355099267392,0.));
#85750=CARTESIAN_POINT('Ctrl Pts',(-73.8227522002498,10.0225374821206,2.7442551750438E-17));
#85751=CARTESIAN_POINT('Ctrl Pts',(-73.8079696346554,10.1314210536418,2.74425517504379E-17));
#85752=CARTESIAN_POINT('Ctrl Pts',(-73.7559622805204,10.2348948883334,-1.43175653184342E-17));
#85753=CARTESIAN_POINT('Ctrl Pts',(-73.6777313404381,10.3119164592424,-8.88779339763642E-17));
#85754=CARTESIAN_POINT('Ctrl Pts',(-73.6190581353764,10.3696826374241,-1.44798210469812E-16));
#85755=CARTESIAN_POINT('Ctrl Pts',(-73.5456341632194,10.4125694172281,-2.19168628482104E-16));
#85756=CARTESIAN_POINT('Ctrl Pts',(-73.4664795929516,10.4355099267394,-3.02822608719546E-16));
#85757=CARTESIAN_POINT('',(-73.4664795929515,10.4355099267392,12.));
#85758=CARTESIAN_POINT('Ctrl Pts',(-73.4664795929516,10.4355099267394,-3.30265160469984E-16));
#85759=CARTESIAN_POINT('Ctrl Pts',(-73.4664795929516,10.4355099267394,4.));
#85760=CARTESIAN_POINT('Ctrl Pts',(-73.4664795929516,10.4355099267394,8.));
#85761=CARTESIAN_POINT('Ctrl Pts',(-73.4664795929516,10.4355099267394,12.));
#85762=CARTESIAN_POINT('',(-73.8227522002498,10.0225374821206,12.));
#85763=CARTESIAN_POINT('Ctrl Pts',(-73.4664795929516,10.4355099267394,12.));
#85764=CARTESIAN_POINT('Ctrl Pts',(-73.5456341632194,10.4125694172281,12.));
#85765=CARTESIAN_POINT('Ctrl Pts',(-73.6190581353764,10.3696826374241,12.));
#85766=CARTESIAN_POINT('Ctrl Pts',(-73.6777313404381,10.3119164592424,12.));
#85767=CARTESIAN_POINT('Ctrl Pts',(-73.7559622805204,10.2348948883334,12.));
#85768=CARTESIAN_POINT('Ctrl Pts',(-73.8079696346554,10.1314210536418,12.));
#85769=CARTESIAN_POINT('Ctrl Pts',(-73.8227522002498,10.0225374821206,12.));
#85770=CARTESIAN_POINT('Ctrl Pts',(-73.8227522002498,10.0225374821206,12.));
#85771=CARTESIAN_POINT('Ctrl Pts',(-73.8227522002498,10.0225374821206,8.));
#85772=CARTESIAN_POINT('Ctrl Pts',(-73.8227522002498,10.0225374821206,4.));
#85773=CARTESIAN_POINT('Ctrl Pts',(-73.8227522002498,10.0225374821206,0.));
#85774=CARTESIAN_POINT('Ctrl Pts',(-69.079679653846,11.3136138754166,0.));
#85775=CARTESIAN_POINT('Ctrl Pts',(-69.079679653846,11.3136138754166,12.));
#85776=CARTESIAN_POINT('Ctrl Pts',(-69.0835449954396,11.3132375200165,0.));
#85777=CARTESIAN_POINT('Ctrl Pts',(-69.0835449954396,11.3132375200165,12.));
#85778=CARTESIAN_POINT('Ctrl Pts',(-69.0912808656811,11.3124821678798,0.));
#85779=CARTESIAN_POINT('Ctrl Pts',(-69.0912808656811,11.3124821678798,12.));
#85780=CARTESIAN_POINT('Ctrl Pts',(-69.1029002322118,11.3113412156662,0.));
#85781=CARTESIAN_POINT('Ctrl Pts',(-69.1029002322118,11.3113412156662,12.));
#85782=CARTESIAN_POINT('Ctrl Pts',(-69.118423844466,11.3098040973713,0.));
#85783=CARTESIAN_POINT('Ctrl Pts',(-69.118423844466,11.3098040973713,12.));
#85784=CARTESIAN_POINT('Ctrl Pts',(-69.1378802251711,11.3078562764385,0.));
#85785=CARTESIAN_POINT('Ctrl Pts',(-69.1378802251711,11.3078562764385,12.));
#85786=CARTESIAN_POINT('Ctrl Pts',(-69.1573884361,11.3058820128308,0.));
#85787=CARTESIAN_POINT('Ctrl Pts',(-69.1573884361,11.3058820128308,12.));
#85788=CARTESIAN_POINT('Ctrl Pts',(-69.1769483991721,11.3038812726293,0.));
#85789=CARTESIAN_POINT('Ctrl Pts',(-69.1769483991721,11.3038812726293,12.));
#85790=CARTESIAN_POINT('Ctrl Pts',(-69.1965599718914,11.3018540025638,0.));
#85791=CARTESIAN_POINT('Ctrl Pts',(-69.1965599718914,11.3018540025638,12.));
#85792=CARTESIAN_POINT('Ctrl Pts',(-69.2162229488531,11.2998001310964,0.));
#85793=CARTESIAN_POINT('Ctrl Pts',(-69.2162229488531,11.2998001310964,12.));
#85794=CARTESIAN_POINT('Ctrl Pts',(-69.2359370894907,11.2977195764853,0.));
#85795=CARTESIAN_POINT('Ctrl Pts',(-69.2359370894907,11.2977195764853,12.));
#85796=CARTESIAN_POINT('Ctrl Pts',(-69.255702139335,11.2956122531375,0.));
#85797=CARTESIAN_POINT('Ctrl Pts',(-69.255702139335,11.2956122531375,12.));
#85798=CARTESIAN_POINT('Ctrl Pts',(-69.2755178531479,11.2934780784351,0.));
#85799=CARTESIAN_POINT('Ctrl Pts',(-69.2755178531479,11.2934780784351,12.));
#85800=CARTESIAN_POINT('Ctrl Pts',(-69.295384019272,11.2913169799628,0.));
#85801=CARTESIAN_POINT('Ctrl Pts',(-69.295384019272,11.2913169799628,12.));
#85802=CARTESIAN_POINT('Ctrl Pts',(-69.3153004517783,11.2891288931517,0.));
#85803=CARTESIAN_POINT('Ctrl Pts',(-69.3153004517783,11.2891288931517,12.));
#85804=CARTESIAN_POINT('Ctrl Pts',(-69.3352669789587,11.2869137578459,0.));
#85805=CARTESIAN_POINT('Ctrl Pts',(-69.3352669789587,11.2869137578459,12.));
#85806=CARTESIAN_POINT('Ctrl Pts',(-69.3552834337784,11.2846715154524,0.));
#85807=CARTESIAN_POINT('Ctrl Pts',(-69.3552834337784,11.2846715154524,12.));
#85808=CARTESIAN_POINT('Ctrl Pts',(-69.3753496420039,11.2824021054045,0.));
#85809=CARTESIAN_POINT('Ctrl Pts',(-69.3753496420039,11.2824021054045,12.));
#85810=CARTESIAN_POINT('Ctrl Pts',(-69.3954654162281,11.2801054633816,0.));
#85811=CARTESIAN_POINT('Ctrl Pts',(-69.3954654162281,11.2801054633816,12.));
#85812=CARTESIAN_POINT('Ctrl Pts',(-69.4156305620593,11.2777815231469,0.));
#85813=CARTESIAN_POINT('Ctrl Pts',(-69.4156305620593,11.2777815231469,12.));
#85814=CARTESIAN_POINT('Ctrl Pts',(-69.4358448819967,11.2754302177021,0.));
#85815=CARTESIAN_POINT('Ctrl Pts',(-69.4358448819967,11.2754302177021,12.));
#85816=CARTESIAN_POINT('Ctrl Pts',(-69.456108179879,11.2730514806139,0.));
#85817=CARTESIAN_POINT('Ctrl Pts',(-69.456108179879,11.2730514806139,12.));
#85818=CARTESIAN_POINT('Ctrl Pts',(-69.4764202659397,11.270645247528,0.));
#85819=CARTESIAN_POINT('Ctrl Pts',(-69.4764202659397,11.270645247528,12.));
#85820=CARTESIAN_POINT('Ctrl Pts',(-69.4967809565929,11.2682114561008,0.));
#85821=CARTESIAN_POINT('Ctrl Pts',(-69.4967809565929,11.2682114561008,12.));
#85822=CARTESIAN_POINT('Ctrl Pts',(-69.5171900720158,11.2657500452716,0.));
#85823=CARTESIAN_POINT('Ctrl Pts',(-69.5171900720158,11.2657500452716,12.));
#85824=CARTESIAN_POINT('Ctrl Pts',(-69.5376474344771,11.263260954763,0.));
#85825=CARTESIAN_POINT('Ctrl Pts',(-69.5376474344771,11.263260954763,12.));
#85826=CARTESIAN_POINT('Ctrl Pts',(-69.5581528662877,11.2607441244703,0.));
#85827=CARTESIAN_POINT('Ctrl Pts',(-69.5581528662877,11.2607441244703,12.));
#85828=CARTESIAN_POINT('Ctrl Pts',(-69.5787061880857,11.2581994939541,0.));
#85829=CARTESIAN_POINT('Ctrl Pts',(-69.5787061880857,11.2581994939541,12.));
#85830=CARTESIAN_POINT('Ctrl Pts',(-69.599307219739,11.2556270027016,0.));
#85831=CARTESIAN_POINT('Ctrl Pts',(-69.599307219739,11.2556270027016,12.));
#85832=CARTESIAN_POINT('Ctrl Pts',(-69.6199557811245,11.2530265903558,0.));
#85833=CARTESIAN_POINT('Ctrl Pts',(-69.6199557811245,11.2530265903558,12.));
#85834=CARTESIAN_POINT('Ctrl Pts',(-69.6406516928891,11.2503981969412,0.));
#85835=CARTESIAN_POINT('Ctrl Pts',(-69.6406516928891,11.2503981969412,12.));
#85836=CARTESIAN_POINT('Ctrl Pts',(-69.6613947773534,11.2477417631386,0.));
#85837=CARTESIAN_POINT('Ctrl Pts',(-69.6613947773534,11.2477417631386,12.));
#85838=CARTESIAN_POINT('Ctrl Pts',(-69.6821848588457,11.2450572303841,0.));
#85839=CARTESIAN_POINT('Ctrl Pts',(-69.6821848588457,11.2450572303841,12.));
#85840=CARTESIAN_POINT('Ctrl Pts',(-69.7030217632164,11.2423445407167,0.));
#85841=CARTESIAN_POINT('Ctrl Pts',(-69.7030217632164,11.2423445407167,12.));
#85842=CARTESIAN_POINT('Ctrl Pts',(-69.7239053175356,11.239603636686,0.));
#85843=CARTESIAN_POINT('Ctrl Pts',(-69.7239053175356,11.239603636686,12.));
#85844=CARTESIAN_POINT('Ctrl Pts',(-69.7448353497408,11.2368344612473,0.));
#85845=CARTESIAN_POINT('Ctrl Pts',(-69.7448353497408,11.2368344612473,12.));
#85846=CARTESIAN_POINT('Ctrl Pts',(-69.7658116882324,11.2340369576456,0.));
#85847=CARTESIAN_POINT('Ctrl Pts',(-69.7658116882324,11.2340369576456,12.));
#85848=CARTESIAN_POINT('Ctrl Pts',(-69.7868341618954,11.2312110694188,0.));
#85849=CARTESIAN_POINT('Ctrl Pts',(-69.7868341618954,11.2312110694188,12.));
#85850=CARTESIAN_POINT('Ctrl Pts',(-69.8079026002768,11.2283567404437,0.));
#85851=CARTESIAN_POINT('Ctrl Pts',(-69.8079026002768,11.2283567404437,12.));
#85852=CARTESIAN_POINT('Ctrl Pts',(-69.8290168337076,11.2254739149721,0.));
#85853=CARTESIAN_POINT('Ctrl Pts',(-69.8290168337076,11.2254739149721,12.));
#85854=CARTESIAN_POINT('Ctrl Pts',(-69.8501766934428,11.2225625376737,0.));
#85855=CARTESIAN_POINT('Ctrl Pts',(-69.8501766934428,11.2225625376737,12.));
#85856=CARTESIAN_POINT('Ctrl Pts',(-69.871382011789,11.219622553679,0.));
#85857=CARTESIAN_POINT('Ctrl Pts',(-69.871382011789,11.219622553679,12.));
#85858=CARTESIAN_POINT('Ctrl Pts',(-69.8926326220385,11.2166539085523,0.));
#85859=CARTESIAN_POINT('Ctrl Pts',(-69.8926326220385,11.2166539085523,12.));
#85860=CARTESIAN_POINT('Ctrl Pts',(-69.9139283584021,11.2136565482678,0.));
#85861=CARTESIAN_POINT('Ctrl Pts',(-69.9139283584021,11.2136565482678,12.));
#85862=CARTESIAN_POINT('Ctrl Pts',(-69.9352690559405,11.2106304191883,0.));
#85863=CARTESIAN_POINT('Ctrl Pts',(-69.9352690559405,11.2106304191883,12.));
#85864=CARTESIAN_POINT('Ctrl Pts',(-69.9566545504837,11.2075754680449,0.));
#85865=CARTESIAN_POINT('Ctrl Pts',(-69.9566545504837,11.2075754680449,12.));
#85866=CARTESIAN_POINT('Ctrl Pts',(-69.97808467858,11.2044916419244,0.));
#85867=CARTESIAN_POINT('Ctrl Pts',(-69.97808467858,11.2044916419244,12.));
#85868=CARTESIAN_POINT('Ctrl Pts',(-69.9995592775343,11.2013788882714,0.));
#85869=CARTESIAN_POINT('Ctrl Pts',(-69.9995592775343,11.2013788882714,12.));
#85870=CARTESIAN_POINT('Ctrl Pts',(-70.0210781854243,11.1982371548919,0.));
#85871=CARTESIAN_POINT('Ctrl Pts',(-70.0210781854243,11.1982371548919,12.));
#85872=CARTESIAN_POINT('Ctrl Pts',(-70.0426412411185,11.1950663899577,0.));
#85873=CARTESIAN_POINT('Ctrl Pts',(-70.0426412411185,11.1950663899577,12.));
#85874=CARTESIAN_POINT('Ctrl Pts',(-70.0642482842928,11.1918665420167,0.));
#85875=CARTESIAN_POINT('Ctrl Pts',(-70.0642482842928,11.1918665420167,12.));
#85876=CARTESIAN_POINT('Ctrl Pts',(-70.0858991554283,11.1886375599914,0.));
#85877=CARTESIAN_POINT('Ctrl Pts',(-70.0858991554283,11.1886375599914,12.));
#85878=CARTESIAN_POINT('Ctrl Pts',(-70.1075936957968,11.185379393167,0.));
#85879=CARTESIAN_POINT('Ctrl Pts',(-70.1075936957968,11.185379393167,12.));
#85880=CARTESIAN_POINT('Ctrl Pts',(-70.1293317474432,11.1820919911846,0.));
#85881=CARTESIAN_POINT('Ctrl Pts',(-70.1293317474432,11.1820919911846,12.));
#85882=CARTESIAN_POINT('Ctrl Pts',(-70.1511131531674,11.1787753040363,0.));
#85883=CARTESIAN_POINT('Ctrl Pts',(-70.1511131531674,11.1787753040363,12.));
#85884=CARTESIAN_POINT('Ctrl Pts',(-70.1729377564956,11.1754292820631,0.));
#85885=CARTESIAN_POINT('Ctrl Pts',(-70.1729377564956,11.1754292820631,12.));
#85886=CARTESIAN_POINT('Ctrl Pts',(-70.1948054016817,11.1720538759499,0.));
#85887=CARTESIAN_POINT('Ctrl Pts',(-70.1948054016817,11.1720538759499,12.));
#85888=CARTESIAN_POINT('Ctrl Pts',(-70.2167159337095,11.168649036721,0.));
#85889=CARTESIAN_POINT('Ctrl Pts',(-70.2167159337095,11.168649036721,12.));
#85890=CARTESIAN_POINT('Ctrl Pts',(-70.2386691982902,11.1652147157383,0.));
#85891=CARTESIAN_POINT('Ctrl Pts',(-70.2386691982902,11.1652147157383,12.));
#85892=CARTESIAN_POINT('Ctrl Pts',(-70.2606650418589,11.1617508647017,0.));
#85893=CARTESIAN_POINT('Ctrl Pts',(-70.2606650418589,11.1617508647017,12.));
#85894=CARTESIAN_POINT('Ctrl Pts',(-70.2827033115662,11.1582574356522,0.));
#85895=CARTESIAN_POINT('Ctrl Pts',(-70.2827033115662,11.1582574356522,12.));
#85896=CARTESIAN_POINT('Ctrl Pts',(-70.3047838552757,11.1547343809647,0.));
#85897=CARTESIAN_POINT('Ctrl Pts',(-70.3047838552757,11.1547343809647,12.));
#85898=CARTESIAN_POINT('Ctrl Pts',(-70.3269065215591,11.1511816533422,0.));
#85899=CARTESIAN_POINT('Ctrl Pts',(-70.3269065215591,11.1511816533422,12.));
#85900=CARTESIAN_POINT('Ctrl Pts',(-70.3490711596882,11.1475992058124,0.));
#85901=CARTESIAN_POINT('Ctrl Pts',(-70.3490711596882,11.1475992058124,12.));
#85902=CARTESIAN_POINT('Ctrl Pts',(-70.3712776196216,11.1439869917269,0.));
#85903=CARTESIAN_POINT('Ctrl Pts',(-70.3712776196216,11.1439869917269,12.));
#85904=CARTESIAN_POINT('Ctrl Pts',(-70.3935257519945,11.1403449647622,0.));
#85905=CARTESIAN_POINT('Ctrl Pts',(-70.3935257519945,11.1403449647622,12.));
#85906=CARTESIAN_POINT('Ctrl Pts',(-70.415815408119,11.1366730789123,0.));
#85907=CARTESIAN_POINT('Ctrl Pts',(-70.415815408119,11.1366730789123,12.));
#85908=CARTESIAN_POINT('Ctrl Pts',(-70.438146439981,11.1329712884845,0.));
#85909=CARTESIAN_POINT('Ctrl Pts',(-70.438146439981,11.1329712884845,12.));
#85910=CARTESIAN_POINT('Ctrl Pts',(-70.4605187002356,11.1292395480975,0.));
#85911=CARTESIAN_POINT('Ctrl Pts',(-70.4605187002356,11.1292395480975,12.));
#85912=CARTESIAN_POINT('Ctrl Pts',(-70.4829320421973,11.1254778126824,0.));
#85913=CARTESIAN_POINT('Ctrl Pts',(-70.4829320421973,11.1254778126824,12.));
#85914=CARTESIAN_POINT('Ctrl Pts',(-70.5053863198306,11.121686037483,0.));
#85915=CARTESIAN_POINT('Ctrl Pts',(-70.5053863198306,11.121686037483,12.));
#85916=CARTESIAN_POINT('Ctrl Pts',(-70.5278813877519,11.117864178048,0.));
#85917=CARTESIAN_POINT('Ctrl Pts',(-70.5278813877519,11.117864178048,12.));
#85918=CARTESIAN_POINT('Ctrl Pts',(-70.5504171012247,11.1140121902274,0.));
#85919=CARTESIAN_POINT('Ctrl Pts',(-70.5504171012247,11.1140121902274,12.));
#85920=CARTESIAN_POINT('Ctrl Pts',(-70.5729933161538,11.1101300301701,0.));
#85921=CARTESIAN_POINT('Ctrl Pts',(-70.5729933161538,11.1101300301701,12.));
#85922=CARTESIAN_POINT('Ctrl Pts',(-70.5956098890744,11.1062176543258,0.));
#85923=CARTESIAN_POINT('Ctrl Pts',(-70.5956098890744,11.1062176543258,12.));
#85924=CARTESIAN_POINT('Ctrl Pts',(-70.6182666771441,11.102275019444,0.));
#85925=CARTESIAN_POINT('Ctrl Pts',(-70.6182666771441,11.102275019444,12.));
#85926=CARTESIAN_POINT('Ctrl Pts',(-70.6409635381446,11.0983020825662,0.));
#85927=CARTESIAN_POINT('Ctrl Pts',(-70.6409635381446,11.0983020825662,12.));
#85928=CARTESIAN_POINT('Ctrl Pts',(-70.6637003304768,11.0942988010231,0.));
#85929=CARTESIAN_POINT('Ctrl Pts',(-70.6637003304768,11.0942988010231,12.));
#85930=CARTESIAN_POINT('Ctrl Pts',(-70.686476913156,11.0902651324326,0.));
#85931=CARTESIAN_POINT('Ctrl Pts',(-70.686476913156,11.0902651324326,12.));
#85932=CARTESIAN_POINT('Ctrl Pts',(-70.7092931457996,11.0862010347022,0.));
#85933=CARTESIAN_POINT('Ctrl Pts',(-70.7092931457996,11.0862010347022,12.));
#85934=CARTESIAN_POINT('Ctrl Pts',(-70.7321488886229,11.0821064660276,0.));
#85935=CARTESIAN_POINT('Ctrl Pts',(-70.7321488886229,11.0821064660276,12.));
#85936=CARTESIAN_POINT('Ctrl Pts',(-70.7550440024422,11.0779813848851,0.));
#85937=CARTESIAN_POINT('Ctrl Pts',(-70.7550440024422,11.0779813848851,12.));
#85938=CARTESIAN_POINT('Ctrl Pts',(-70.7779783486689,11.0738257500292,0.));
#85939=CARTESIAN_POINT('Ctrl Pts',(-70.7779783486689,11.0738257500292,12.));
#85940=CARTESIAN_POINT('Ctrl Pts',(-70.8009517893042,11.0696395204908,0.));
#85941=CARTESIAN_POINT('Ctrl Pts',(-70.8009517893042,11.0696395204908,12.));
#85942=CARTESIAN_POINT('Ctrl Pts',(-70.8239641869266,11.0654226555799,0.));
#85943=CARTESIAN_POINT('Ctrl Pts',(-70.8239641869266,11.0654226555799,12.));
#85944=CARTESIAN_POINT('Ctrl Pts',(-70.847015404688,11.0611751148831,0.));
#85945=CARTESIAN_POINT('Ctrl Pts',(-70.847015404688,11.0611751148831,12.));
#85946=CARTESIAN_POINT('Ctrl Pts',(-70.8701053063158,11.0568968582566,0.));
#85947=CARTESIAN_POINT('Ctrl Pts',(-70.8701053063158,11.0568968582566,12.));
#85948=CARTESIAN_POINT('Ctrl Pts',(-70.8932337561079,11.0525878458242,0.));
#85949=CARTESIAN_POINT('Ctrl Pts',(-70.8932337561079,11.0525878458242,12.));
#85950=CARTESIAN_POINT('Ctrl Pts',(-70.9164006189283,11.0482480379752,0.));
#85951=CARTESIAN_POINT('Ctrl Pts',(-70.9164006189283,11.0482480379752,12.));
#85952=CARTESIAN_POINT('Ctrl Pts',(-70.9396057601953,11.0438773953686,0.));
#85953=CARTESIAN_POINT('Ctrl Pts',(-70.9396057601953,11.0438773953686,12.));
#85954=CARTESIAN_POINT('Ctrl Pts',(-70.9628490458779,11.039475878929,0.));
#85955=CARTESIAN_POINT('Ctrl Pts',(-70.9628490458779,11.039475878929,12.));
#85956=CARTESIAN_POINT('Ctrl Pts',(-70.9861303424989,11.0350434498408,0.));
#85957=CARTESIAN_POINT('Ctrl Pts',(-70.9861303424989,11.0350434498408,12.));
#85958=CARTESIAN_POINT('Ctrl Pts',(-71.0094495171295,11.0305800695457,0.));
#85959=CARTESIAN_POINT('Ctrl Pts',(-71.0094495171295,11.0305800695457,12.));
#85960=CARTESIAN_POINT('Ctrl Pts',(-71.0328064373849,11.0260856997415,0.));
#85961=CARTESIAN_POINT('Ctrl Pts',(-71.0328064373849,11.0260856997415,12.));
#85962=CARTESIAN_POINT('Ctrl Pts',(-71.0562009714125,11.0215603023855,0.));
#85963=CARTESIAN_POINT('Ctrl Pts',(-71.0562009714125,11.0215603023855,12.));
#85964=CARTESIAN_POINT('Ctrl Pts',(-71.0796329878896,11.0170038396913,0.));
#85965=CARTESIAN_POINT('Ctrl Pts',(-71.0796329878896,11.0170038396913,12.));
#85966=CARTESIAN_POINT('Ctrl Pts',(-71.1031023560243,11.0124162741224,0.));
#85967=CARTESIAN_POINT('Ctrl Pts',(-71.1031023560243,11.0124162741224,12.));
#85968=CARTESIAN_POINT('Ctrl Pts',(-71.1266089455517,11.0077975683895,0.));
#85969=CARTESIAN_POINT('Ctrl Pts',(-71.1266089455517,11.0077975683895,12.));
#85970=CARTESIAN_POINT('Ctrl Pts',(-71.1501526267288,11.0031476854503,0.));
#85971=CARTESIAN_POINT('Ctrl Pts',(-71.1501526267288,11.0031476854503,12.));
#85972=CARTESIAN_POINT('Ctrl Pts',(-71.1737332703248,10.9984665885127,0.));
#85973=CARTESIAN_POINT('Ctrl Pts',(-71.1737332703248,10.9984665885127,12.));
#85974=CARTESIAN_POINT('Ctrl Pts',(-71.1973507476188,10.993754241032,0.));
#85975=CARTESIAN_POINT('Ctrl Pts',(-71.1973507476188,10.993754241032,12.));
#85976=CARTESIAN_POINT('Ctrl Pts',(-71.221004930401,10.9890106067039,0.));
#85977=CARTESIAN_POINT('Ctrl Pts',(-71.221004930401,10.9890106067039,12.));
#85978=CARTESIAN_POINT('Ctrl Pts',(-71.2446956909685,10.9842356494627,0.));
#85979=CARTESIAN_POINT('Ctrl Pts',(-71.2446956909685,10.9842356494627,12.));
#85980=CARTESIAN_POINT('Ctrl Pts',(-71.2684229021209,10.9794293334806,0.));
#85981=CARTESIAN_POINT('Ctrl Pts',(-71.2684229021209,10.9794293334806,12.));
#85982=CARTESIAN_POINT('Ctrl Pts',(-71.2921864371499,10.9745916231711,0.));
#85983=CARTESIAN_POINT('Ctrl Pts',(-71.2921864371499,10.9745916231711,12.));
#85984=CARTESIAN_POINT('Ctrl Pts',(-71.3159861698368,10.9697224831863,0.));
#85985=CARTESIAN_POINT('Ctrl Pts',(-71.3159861698368,10.9697224831863,12.));
#85986=CARTESIAN_POINT('Ctrl Pts',(-71.3398219744547,10.96482187841,0.));
#85987=CARTESIAN_POINT('Ctrl Pts',(-71.3398219744547,10.96482187841,12.));
#85988=CARTESIAN_POINT('Ctrl Pts',(-71.3636937257651,10.9598897739565,0.));
#85989=CARTESIAN_POINT('Ctrl Pts',(-71.3636937257651,10.9598897739565,12.));
#85990=CARTESIAN_POINT('Ctrl Pts',(-71.3876012990135,10.954926135169,0.));
#85991=CARTESIAN_POINT('Ctrl Pts',(-71.3876012990135,10.954926135169,12.));
#85992=CARTESIAN_POINT('Ctrl Pts',(-71.411544569919,10.9499309276236,0.));
#85993=CARTESIAN_POINT('Ctrl Pts',(-71.411544569919,10.9499309276236,12.));
#85994=CARTESIAN_POINT('Ctrl Pts',(-71.4355234146718,10.9449041171269,0.));
#85995=CARTESIAN_POINT('Ctrl Pts',(-71.4355234146718,10.9449041171269,12.));
#85996=CARTESIAN_POINT('Ctrl Pts',(-71.4595377099352,10.9398456697095,0.));
#85997=CARTESIAN_POINT('Ctrl Pts',(-71.4595377099352,10.9398456697095,12.));
#85998=CARTESIAN_POINT('Ctrl Pts',(-71.4835873328425,10.9347555516236,0.));
#85999=CARTESIAN_POINT('Ctrl Pts',(-71.4835873328425,10.9347555516236,12.));
#86000=CARTESIAN_POINT('Ctrl Pts',(-71.5076721609936,10.9296337293425,0.));
#86001=CARTESIAN_POINT('Ctrl Pts',(-71.5076721609936,10.9296337293425,12.));
#86002=CARTESIAN_POINT('Ctrl Pts',(-71.5317920724453,10.9244801695642,0.));
#86003=CARTESIAN_POINT('Ctrl Pts',(-71.5317920724453,10.9244801695642,12.));
#86004=CARTESIAN_POINT('Ctrl Pts',(-71.5559469457082,10.91929483921,0.));
#86005=CARTESIAN_POINT('Ctrl Pts',(-71.5559469457082,10.91929483921,12.));
#86006=CARTESIAN_POINT('Ctrl Pts',(-71.5801366597479,10.9140777054169,0.));
#86007=CARTESIAN_POINT('Ctrl Pts',(-71.5801366597479,10.9140777054169,12.));
#86008=CARTESIAN_POINT('Ctrl Pts',(-71.604361093983,10.9088287355364,0.));
#86009=CARTESIAN_POINT('Ctrl Pts',(-71.604361093983,10.9088287355364,12.));
#86010=CARTESIAN_POINT('Ctrl Pts',(-71.6286201282815,10.9035478971329,0.));
#86011=CARTESIAN_POINT('Ctrl Pts',(-71.6286201282815,10.9035478971329,12.));
#86012=CARTESIAN_POINT('Ctrl Pts',(-71.6529136429515,10.8982351579873,0.));
#86013=CARTESIAN_POINT('Ctrl Pts',(-71.6529136429515,10.8982351579873,12.));
#86014=CARTESIAN_POINT('Ctrl Pts',(-71.6772415187382,10.8928904860967,0.));
#86015=CARTESIAN_POINT('Ctrl Pts',(-71.6772415187382,10.8928904860967,12.));
#86016=CARTESIAN_POINT('Ctrl Pts',(-71.7016036368254,10.8875138496674,0.));
#86017=CARTESIAN_POINT('Ctrl Pts',(-71.7016036368254,10.8875138496674,12.));
#86018=CARTESIAN_POINT('Ctrl Pts',(-71.7259998788337,10.8821052171122,0.));
#86019=CARTESIAN_POINT('Ctrl Pts',(-71.7259998788337,10.8821052171122,12.));
#86020=CARTESIAN_POINT('Ctrl Pts',(-71.7504301268177,10.8766645570497,0.));
#86021=CARTESIAN_POINT('Ctrl Pts',(-71.7504301268177,10.8766645570497,12.));
#86022=CARTESIAN_POINT('Ctrl Pts',(-71.7748942632578,10.8711918383071,0.));
#86023=CARTESIAN_POINT('Ctrl Pts',(-71.7748942632578,10.8711918383071,12.));
#86024=CARTESIAN_POINT('Ctrl Pts',(-71.7993921710546,10.8656870299218,0.));
#86025=CARTESIAN_POINT('Ctrl Pts',(-71.7993921710546,10.8656870299218,12.));
#86026=CARTESIAN_POINT('Ctrl Pts',(-71.8239237335317,10.860150101133,0.));
#86027=CARTESIAN_POINT('Ctrl Pts',(-71.8239237335317,10.860150101133,12.));
#86028=CARTESIAN_POINT('Ctrl Pts',(-71.8484888344335,10.8545810213799,0.));
#86029=CARTESIAN_POINT('Ctrl Pts',(-71.8484888344335,10.8545810213799,12.));
#86030=CARTESIAN_POINT('Ctrl Pts',(-71.8730873579226,10.8489797602998,0.));
#86031=CARTESIAN_POINT('Ctrl Pts',(-71.8730873579226,10.8489797602998,12.));
#86032=CARTESIAN_POINT('Ctrl Pts',(-71.8977191885726,10.8433462877312,0.));
#86033=CARTESIAN_POINT('Ctrl Pts',(-71.8977191885726,10.8433462877312,12.));
#86034=CARTESIAN_POINT('Ctrl Pts',(-71.9223842113622,10.8376805737159,0.));
#86035=CARTESIAN_POINT('Ctrl Pts',(-71.9223842113622,10.8376805737159,12.));
#86036=CARTESIAN_POINT('Ctrl Pts',(-71.9470823116777,10.8319825884917,0.));
#86037=CARTESIAN_POINT('Ctrl Pts',(-71.9470823116777,10.8319825884917,12.));
#86038=CARTESIAN_POINT('Ctrl Pts',(-71.971813375312,10.8262523024897,0.));
#86039=CARTESIAN_POINT('Ctrl Pts',(-71.971813375312,10.8262523024897,12.));
#86040=CARTESIAN_POINT('Ctrl Pts',(-71.9965772884619,10.8204896863328,0.));
#86041=CARTESIAN_POINT('Ctrl Pts',(-71.9965772884619,10.8204896863328,12.));
#86042=CARTESIAN_POINT('Ctrl Pts',(-72.0213739377231,10.8146947108377,0.));
#86043=CARTESIAN_POINT('Ctrl Pts',(-72.0213739377231,10.8146947108377,12.));
#86044=CARTESIAN_POINT('Ctrl Pts',(-72.0462032100828,10.8088673470187,0.));
#86045=CARTESIAN_POINT('Ctrl Pts',(-72.0462032100828,10.8088673470187,12.));
#86046=CARTESIAN_POINT('Ctrl Pts',(-72.0710649929214,10.8030075660812,0.));
#86047=CARTESIAN_POINT('Ctrl Pts',(-72.0710649929214,10.8030075660812,12.));
#86048=CARTESIAN_POINT('Ctrl Pts',(-72.095959174012,10.7971153394168,0.));
#86049=CARTESIAN_POINT('Ctrl Pts',(-72.095959174012,10.7971153394168,12.));
#86050=CARTESIAN_POINT('Ctrl Pts',(-72.1208856415171,10.7911906386027,0.));
#86051=CARTESIAN_POINT('Ctrl Pts',(-72.1208856415171,10.7911906386027,12.));
#86052=CARTESIAN_POINT('Ctrl Pts',(-72.145844283983,10.7852334354015,0.));
#86053=CARTESIAN_POINT('Ctrl Pts',(-72.145844283983,10.7852334354015,12.));
#86054=CARTESIAN_POINT('Ctrl Pts',(-72.17083499033,10.779243701766,0.));
#86055=CARTESIAN_POINT('Ctrl Pts',(-72.17083499033,10.779243701766,12.));
#86056=CARTESIAN_POINT('Ctrl Pts',(-72.1958576498556,10.7732214098343,0.));
#86057=CARTESIAN_POINT('Ctrl Pts',(-72.1958576498556,10.7732214098343,12.));
#86058=CARTESIAN_POINT('Ctrl Pts',(-72.2209121522367,10.7671665319254,0.));
#86059=CARTESIAN_POINT('Ctrl Pts',(-72.2209121522367,10.7671665319254,12.));
#86060=CARTESIAN_POINT('Ctrl Pts',(-72.2459983875297,10.7610790405385,0.));
#86061=CARTESIAN_POINT('Ctrl Pts',(-72.2459983875297,10.7610790405385,12.));
#86062=CARTESIAN_POINT('Ctrl Pts',(-72.2711162461679,10.7549589083536,0.));
#86063=CARTESIAN_POINT('Ctrl Pts',(-72.2711162461679,10.7549589083536,12.));
#86064=CARTESIAN_POINT('Ctrl Pts',(-72.296265618955,10.7488061082368,0.));
#86065=CARTESIAN_POINT('Ctrl Pts',(-72.296265618955,10.7488061082368,12.));
#86066=CARTESIAN_POINT('Ctrl Pts',(-72.3214463970634,10.7426206132375,0.));
#86067=CARTESIAN_POINT('Ctrl Pts',(-72.3214463970634,10.7426206132375,12.));
#86068=CARTESIAN_POINT('Ctrl Pts',(-72.3466584720311,10.73640239658,0.));
#86069=CARTESIAN_POINT('Ctrl Pts',(-72.3466584720311,10.73640239658,12.));
#86070=CARTESIAN_POINT('Ctrl Pts',(-72.3719017357568,10.7301514316607,0.));
#86071=CARTESIAN_POINT('Ctrl Pts',(-72.3719017357568,10.7301514316607,12.));
#86072=CARTESIAN_POINT('Ctrl Pts',(-72.3971760804935,10.7238676920469,0.));
#86073=CARTESIAN_POINT('Ctrl Pts',(-72.3971760804935,10.7238676920469,12.));
#86074=CARTESIAN_POINT('Ctrl Pts',(-72.4224813988355,10.7175511514789,0.));
#86075=CARTESIAN_POINT('Ctrl Pts',(-72.4224813988355,10.7175511514789,12.));
#86076=CARTESIAN_POINT('Ctrl Pts',(-72.4478175837168,10.7112017838707,0.));
#86077=CARTESIAN_POINT('Ctrl Pts',(-72.4478175837168,10.7112017838707,12.));
#86078=CARTESIAN_POINT('Ctrl Pts',(-72.4731845284238,10.7048195633062,0.));
#86079=CARTESIAN_POINT('Ctrl Pts',(-72.4731845284238,10.7048195633062,12.));
#86080=CARTESIAN_POINT('Ctrl Pts',(-72.4985821266031,10.6984044640399,0.));
#86081=CARTESIAN_POINT('Ctrl Pts',(-72.4985821266031,10.6984044640399,12.));
#86082=CARTESIAN_POINT('Ctrl Pts',(-72.5240102722662,10.6919564604991,0.));
#86083=CARTESIAN_POINT('Ctrl Pts',(-72.5240102722662,10.6919564604991,12.));
#86084=CARTESIAN_POINT('Ctrl Pts',(-72.5494688597951,10.6854755272904,0.));
#86085=CARTESIAN_POINT('Ctrl Pts',(-72.5494688597951,10.6854755272904,12.));
#86086=CARTESIAN_POINT('Ctrl Pts',(-72.57495778394,10.6789616392041,0.));
#86087=CARTESIAN_POINT('Ctrl Pts',(-72.57495778394,10.6789616392041,12.));
#86088=CARTESIAN_POINT('Ctrl Pts',(-72.6004769398004,10.6724147711994,0.));
#86089=CARTESIAN_POINT('Ctrl Pts',(-72.6004769398004,10.6724147711994,12.));
#86090=CARTESIAN_POINT('Ctrl Pts',(-72.6260262228055,10.6658348983944,0.));
#86091=CARTESIAN_POINT('Ctrl Pts',(-72.6260262228055,10.6658348983944,12.));
#86092=CARTESIAN_POINT('Ctrl Pts',(-72.6516055286908,10.6592219960581,0.));
#86093=CARTESIAN_POINT('Ctrl Pts',(-72.6516055286908,10.6592219960581,12.));
#86094=CARTESIAN_POINT('Ctrl Pts',(-72.6772147534762,10.6525760396056,0.));
#86095=CARTESIAN_POINT('Ctrl Pts',(-72.6772147534762,10.6525760396056,12.));
#86096=CARTESIAN_POINT('Ctrl Pts',(-72.7028537934332,10.6458970045948,0.));
#86097=CARTESIAN_POINT('Ctrl Pts',(-72.7028537934332,10.6458970045948,12.));
#86098=CARTESIAN_POINT('Ctrl Pts',(-72.7285225451309,10.6391848667354,0.));
#86099=CARTESIAN_POINT('Ctrl Pts',(-72.7285225451309,10.6391848667354,12.));
#86100=CARTESIAN_POINT('Ctrl Pts',(-72.7542209054823,10.6324396019,0.));
#86101=CARTESIAN_POINT('Ctrl Pts',(-72.7542209054823,10.6324396019,12.));
#86102=CARTESIAN_POINT('Ctrl Pts',(-72.7799487717914,10.6256611861395,0.));
#86103=CARTESIAN_POINT('Ctrl Pts',(-72.7799487717914,10.6256611861395,12.));
#86104=CARTESIAN_POINT('Ctrl Pts',(-72.8057060417882,10.6188495956973,0.));
#86105=CARTESIAN_POINT('Ctrl Pts',(-72.8057060417882,10.6188495956973,12.));
#86106=CARTESIAN_POINT('Ctrl Pts',(-72.8314926136872,10.6120048070367,0.));
#86107=CARTESIAN_POINT('Ctrl Pts',(-72.8314926136872,10.6120048070367,12.));
#86108=CARTESIAN_POINT('Ctrl Pts',(-72.8573083861328,10.6051267968202,0.));
#86109=CARTESIAN_POINT('Ctrl Pts',(-72.8573083861328,10.6051267968202,12.));
#86110=CARTESIAN_POINT('Ctrl Pts',(-72.8831532580839,10.5982155418625,0.));
#86111=CARTESIAN_POINT('Ctrl Pts',(-72.8831532580839,10.5982155418625,12.));
#86112=CARTESIAN_POINT('Ctrl Pts',(-72.9090271287081,10.5912710190928,0.));
#86113=CARTESIAN_POINT('Ctrl Pts',(-72.9090271287081,10.5912710190928,12.));
#86114=CARTESIAN_POINT('Ctrl Pts',(-72.9349298972823,10.5842932055209,0.));
#86115=CARTESIAN_POINT('Ctrl Pts',(-72.9349298972823,10.5842932055209,12.));
#86116=CARTESIAN_POINT('Ctrl Pts',(-72.9608614630538,10.5772820781959,0.));
#86117=CARTESIAN_POINT('Ctrl Pts',(-72.9608614630538,10.5772820781959,12.));
#86118=CARTESIAN_POINT('Ctrl Pts',(-72.9868217252293,10.5702376142052,0.));
#86119=CARTESIAN_POINT('Ctrl Pts',(-72.9868217252293,10.5702376142052,12.));
#86120=CARTESIAN_POINT('Ctrl Pts',(-73.0128105832635,10.5631597907653,0.));
#86121=CARTESIAN_POINT('Ctrl Pts',(-73.0128105832635,10.5631597907653,12.));
#86122=CARTESIAN_POINT('Ctrl Pts',(-73.0388279370845,10.5560485852976,0.));
#86123=CARTESIAN_POINT('Ctrl Pts',(-73.0388279370845,10.5560485852976,12.));
#86124=CARTESIAN_POINT('Ctrl Pts',(-73.0648736873435,10.5489039755138,0.));
#86125=CARTESIAN_POINT('Ctrl Pts',(-73.0648736873435,10.5489039755138,12.));
#86126=CARTESIAN_POINT('Ctrl Pts',(-73.090947735646,10.5417259395001,0.));
#86127=CARTESIAN_POINT('Ctrl Pts',(-73.090947735646,10.5417259395001,12.));
#86128=CARTESIAN_POINT('Ctrl Pts',(-73.1170499848012,10.5345144558097,0.));
#86129=CARTESIAN_POINT('Ctrl Pts',(-73.1170499848012,10.5345144558097,12.));
#86130=CARTESIAN_POINT('Ctrl Pts',(-73.1431803382677,10.5272695032649,0.));
#86131=CARTESIAN_POINT('Ctrl Pts',(-73.1431803382677,10.5272695032649,12.));
#86132=CARTESIAN_POINT('Ctrl Pts',(-73.169338699611,10.5199910607652,0.));
#86133=CARTESIAN_POINT('Ctrl Pts',(-73.169338699611,10.5199910607652,12.));
#86134=CARTESIAN_POINT('Ctrl Pts',(-73.1955249719037,10.5126791070804,0.));
#86135=CARTESIAN_POINT('Ctrl Pts',(-73.1955249719037,10.5126791070804,12.));
#86136=CARTESIAN_POINT('Ctrl Pts',(-73.2217390572578,10.505333620691,0.));
#86137=CARTESIAN_POINT('Ctrl Pts',(-73.2217390572578,10.505333620691,12.));
#86138=CARTESIAN_POINT('Ctrl Pts',(-73.247980856023,10.4979545795197,0.));
#86139=CARTESIAN_POINT('Ctrl Pts',(-73.247980856023,10.4979545795197,12.));
#86140=CARTESIAN_POINT('Ctrl Pts',(-73.2742502674361,10.4905419611529,0.));
#86141=CARTESIAN_POINT('Ctrl Pts',(-73.2742502674361,10.4905419611529,12.));
#86142=CARTESIAN_POINT('Ctrl Pts',(-73.3005471910639,10.4830957433311,0.));
#86143=CARTESIAN_POINT('Ctrl Pts',(-73.3005471910639,10.4830957433311,12.));
#86144=CARTESIAN_POINT('Ctrl Pts',(-73.3268715280609,10.475615904381,0.));
#86145=CARTESIAN_POINT('Ctrl Pts',(-73.3268715280609,10.475615904381,12.));
#86146=CARTESIAN_POINT('Ctrl Pts',(-73.353223182365,10.4681024236288,0.));
#86147=CARTESIAN_POINT('Ctrl Pts',(-73.353223182365,10.4681024236288,12.));
#86148=CARTESIAN_POINT('Ctrl Pts',(-73.3796020622436,10.4605552819391,0.));
#86149=CARTESIAN_POINT('Ctrl Pts',(-73.3796020622436,10.4605552819391,12.));
#86150=CARTESIAN_POINT('Ctrl Pts',(-73.4060080806577,10.4529744618439,0.));
#86151=CARTESIAN_POINT('Ctrl Pts',(-73.4060080806577,10.4529744618439,12.));
#86152=CARTESIAN_POINT('Ctrl Pts',(-73.432441151843,10.4453599463535,0.));
#86153=CARTESIAN_POINT('Ctrl Pts',(-73.432441151843,10.4453599463535,12.));
#86154=CARTESIAN_POINT('Ctrl Pts',(-73.45890118861,10.4377117180213,0.));
#86155=CARTESIAN_POINT('Ctrl Pts',(-73.45890118861,10.4377117180213,12.));
#86156=CARTESIAN_POINT('Ctrl Pts',(-73.4853880992228,10.4300297578648,0.));
#86157=CARTESIAN_POINT('Ctrl Pts',(-73.4853880992228,10.4300297578648,12.));
#86158=CARTESIAN_POINT('Ctrl Pts',(-73.5119017847664,10.4223140444615,0.));
#86159=CARTESIAN_POINT('Ctrl Pts',(-73.5119017847664,10.4223140444615,12.));
#86160=CARTESIAN_POINT('Ctrl Pts',(-73.5384421354746,10.4145645526832,0.));
#86161=CARTESIAN_POINT('Ctrl Pts',(-73.5384421354746,10.4145645526832,12.));
#86162=CARTESIAN_POINT('Ctrl Pts',(-73.5650090360113,10.4067812555539,0.));
#86163=CARTESIAN_POINT('Ctrl Pts',(-73.5650090360113,10.4067812555539,12.));
#86164=CARTESIAN_POINT('Ctrl Pts',(-73.5916023719976,10.3989641265313,0.));
#86165=CARTESIAN_POINT('Ctrl Pts',(-73.5916023719976,10.3989641265313,12.));
#86166=CARTESIAN_POINT('Ctrl Pts',(-73.6182220363295,10.3911131417478,0.));
#86167=CARTESIAN_POINT('Ctrl Pts',(-73.6182220363295,10.3911131417478,12.));
#86168=CARTESIAN_POINT('Ctrl Pts',(-73.6448679350605,10.3832282820362,0.));
#86169=CARTESIAN_POINT('Ctrl Pts',(-73.6448679350605,10.3832282820362,12.));
#86170=CARTESIAN_POINT('Ctrl Pts',(-73.6715399947459,10.3753095356302,0.));
#86171=CARTESIAN_POINT('Ctrl Pts',(-73.6715399947459,10.3753095356302,12.));
#86172=CARTESIAN_POINT('Ctrl Pts',(-73.6982381644571,10.3673568984515,0.));
#86173=CARTESIAN_POINT('Ctrl Pts',(-73.6982381644571,10.3673568984515,12.));
#86174=CARTESIAN_POINT('Ctrl Pts',(-73.7249624108432,10.3593703712542,0.));
#86175=CARTESIAN_POINT('Ctrl Pts',(-73.7249624108432,10.3593703712542,12.));
#86176=CARTESIAN_POINT('Ctrl Pts',(-73.7463626541235,10.3529540403026,0.));
#86177=CARTESIAN_POINT('Ctrl Pts',(-73.7463626541235,10.3529540403026,12.));
#86178=CARTESIAN_POINT('Ctrl Pts',(-73.7624245587416,10.3481265449303,0.));
#86179=CARTESIAN_POINT('Ctrl Pts',(-73.7624245587416,10.3481265449303,12.));
#86180=CARTESIAN_POINT('Ctrl Pts',(-73.7731377047922,10.3449014384439,0.));
#86181=CARTESIAN_POINT('Ctrl Pts',(-73.7731377047922,10.3449014384439,12.));
#86182=CARTESIAN_POINT('Ctrl Pts',(-73.778495580227,10.343287191141,0.));
#86183=CARTESIAN_POINT('Ctrl Pts',(-73.778495580227,10.343287191141,12.));
#86184=CARTESIAN_POINT('',(-69.079679653846,11.3136138754166,0.));
#86185=CARTESIAN_POINT('Ctrl Pts',(-69.079679653846,11.3136138754166,0.));
#86186=CARTESIAN_POINT('Ctrl Pts',(-69.0835449954396,11.3132375200165,0.));
#86187=CARTESIAN_POINT('Ctrl Pts',(-69.0912808656811,11.3124821678798,0.));
#86188=CARTESIAN_POINT('Ctrl Pts',(-69.1029002322118,11.3113412156662,0.));
#86189=CARTESIAN_POINT('Ctrl Pts',(-69.118423844466,11.3098040973713,0.));
#86190=CARTESIAN_POINT('Ctrl Pts',(-69.1378802251711,11.3078562764385,0.));
#86191=CARTESIAN_POINT('Ctrl Pts',(-69.1573884361,11.3058820128308,0.));
#86192=CARTESIAN_POINT('Ctrl Pts',(-69.1769483991721,11.3038812726293,0.));
#86193=CARTESIAN_POINT('Ctrl Pts',(-69.1965599718914,11.3018540025638,0.));
#86194=CARTESIAN_POINT('Ctrl Pts',(-69.2162229488531,11.2998001310964,0.));
#86195=CARTESIAN_POINT('Ctrl Pts',(-69.2359370894907,11.2977195764853,0.));
#86196=CARTESIAN_POINT('Ctrl Pts',(-69.255702139335,11.2956122531375,0.));
#86197=CARTESIAN_POINT('Ctrl Pts',(-69.2755178531479,11.2934780784351,0.));
#86198=CARTESIAN_POINT('Ctrl Pts',(-69.295384019272,11.2913169799628,0.));
#86199=CARTESIAN_POINT('Ctrl Pts',(-69.3153004517783,11.2891288931517,0.));
#86200=CARTESIAN_POINT('Ctrl Pts',(-69.3352669789587,11.2869137578459,0.));
#86201=CARTESIAN_POINT('Ctrl Pts',(-69.3552834337784,11.2846715154524,0.));
#86202=CARTESIAN_POINT('Ctrl Pts',(-69.3753496420039,11.2824021054045,0.));
#86203=CARTESIAN_POINT('Ctrl Pts',(-69.3954654162281,11.2801054633816,0.));
#86204=CARTESIAN_POINT('Ctrl Pts',(-69.4156305620593,11.2777815231469,0.));
#86205=CARTESIAN_POINT('Ctrl Pts',(-69.4358448819967,11.2754302177021,0.));
#86206=CARTESIAN_POINT('Ctrl Pts',(-69.456108179879,11.2730514806139,0.));
#86207=CARTESIAN_POINT('Ctrl Pts',(-69.4764202659397,11.270645247528,0.));
#86208=CARTESIAN_POINT('Ctrl Pts',(-69.4967809565929,11.2682114561008,0.));
#86209=CARTESIAN_POINT('Ctrl Pts',(-69.5171900720158,11.2657500452716,0.));
#86210=CARTESIAN_POINT('Ctrl Pts',(-69.5376474344771,11.263260954763,0.));
#86211=CARTESIAN_POINT('Ctrl Pts',(-69.5581528662877,11.2607441244703,0.));
#86212=CARTESIAN_POINT('Ctrl Pts',(-69.5787061880857,11.2581994939541,0.));
#86213=CARTESIAN_POINT('Ctrl Pts',(-69.599307219739,11.2556270027016,0.));
#86214=CARTESIAN_POINT('Ctrl Pts',(-69.6199557811245,11.2530265903558,0.));
#86215=CARTESIAN_POINT('Ctrl Pts',(-69.6406516928891,11.2503981969412,0.));
#86216=CARTESIAN_POINT('Ctrl Pts',(-69.6613947773534,11.2477417631386,0.));
#86217=CARTESIAN_POINT('Ctrl Pts',(-69.6821848588457,11.2450572303841,0.));
#86218=CARTESIAN_POINT('Ctrl Pts',(-69.7030217632164,11.2423445407167,0.));
#86219=CARTESIAN_POINT('Ctrl Pts',(-69.7239053175356,11.239603636686,0.));
#86220=CARTESIAN_POINT('Ctrl Pts',(-69.7448353497408,11.2368344612473,0.));
#86221=CARTESIAN_POINT('Ctrl Pts',(-69.7658116882324,11.2340369576456,0.));
#86222=CARTESIAN_POINT('Ctrl Pts',(-69.7868341618954,11.2312110694188,0.));
#86223=CARTESIAN_POINT('Ctrl Pts',(-69.8079026002768,11.2283567404437,0.));
#86224=CARTESIAN_POINT('Ctrl Pts',(-69.8290168337076,11.2254739149721,0.));
#86225=CARTESIAN_POINT('Ctrl Pts',(-69.8501766934428,11.2225625376737,0.));
#86226=CARTESIAN_POINT('Ctrl Pts',(-69.871382011789,11.219622553679,0.));
#86227=CARTESIAN_POINT('Ctrl Pts',(-69.8926326220385,11.2166539085523,0.));
#86228=CARTESIAN_POINT('Ctrl Pts',(-69.9139283584021,11.2136565482678,0.));
#86229=CARTESIAN_POINT('Ctrl Pts',(-69.9352690559405,11.2106304191883,0.));
#86230=CARTESIAN_POINT('Ctrl Pts',(-69.9566545504837,11.2075754680449,0.));
#86231=CARTESIAN_POINT('Ctrl Pts',(-69.97808467858,11.2044916419244,0.));
#86232=CARTESIAN_POINT('Ctrl Pts',(-69.9995592775343,11.2013788882714,0.));
#86233=CARTESIAN_POINT('Ctrl Pts',(-70.0210781854243,11.1982371548919,0.));
#86234=CARTESIAN_POINT('Ctrl Pts',(-70.0426412411185,11.1950663899577,0.));
#86235=CARTESIAN_POINT('Ctrl Pts',(-70.0642482842928,11.1918665420167,0.));
#86236=CARTESIAN_POINT('Ctrl Pts',(-70.0858991554283,11.1886375599914,0.));
#86237=CARTESIAN_POINT('Ctrl Pts',(-70.1075936957968,11.185379393167,0.));
#86238=CARTESIAN_POINT('Ctrl Pts',(-70.1293317474432,11.1820919911846,0.));
#86239=CARTESIAN_POINT('Ctrl Pts',(-70.1511131531674,11.1787753040363,0.));
#86240=CARTESIAN_POINT('Ctrl Pts',(-70.1729377564956,11.1754292820631,0.));
#86241=CARTESIAN_POINT('Ctrl Pts',(-70.1948054016817,11.1720538759499,0.));
#86242=CARTESIAN_POINT('Ctrl Pts',(-70.2167159337095,11.168649036721,0.));
#86243=CARTESIAN_POINT('Ctrl Pts',(-70.2386691982902,11.1652147157383,0.));
#86244=CARTESIAN_POINT('Ctrl Pts',(-70.2606650418589,11.1617508647017,0.));
#86245=CARTESIAN_POINT('Ctrl Pts',(-70.2827033115662,11.1582574356522,0.));
#86246=CARTESIAN_POINT('Ctrl Pts',(-70.3047838552757,11.1547343809647,0.));
#86247=CARTESIAN_POINT('Ctrl Pts',(-70.3269065215591,11.1511816533422,0.));
#86248=CARTESIAN_POINT('Ctrl Pts',(-70.3490711596882,11.1475992058124,0.));
#86249=CARTESIAN_POINT('Ctrl Pts',(-70.3712776196216,11.1439869917269,0.));
#86250=CARTESIAN_POINT('Ctrl Pts',(-70.3935257519945,11.1403449647622,0.));
#86251=CARTESIAN_POINT('Ctrl Pts',(-70.415815408119,11.1366730789123,0.));
#86252=CARTESIAN_POINT('Ctrl Pts',(-70.438146439981,11.1329712884845,0.));
#86253=CARTESIAN_POINT('Ctrl Pts',(-70.4605187002356,11.1292395480975,0.));
#86254=CARTESIAN_POINT('Ctrl Pts',(-70.4829320421973,11.1254778126824,0.));
#86255=CARTESIAN_POINT('Ctrl Pts',(-70.5053863198306,11.121686037483,0.));
#86256=CARTESIAN_POINT('Ctrl Pts',(-70.5278813877519,11.117864178048,0.));
#86257=CARTESIAN_POINT('Ctrl Pts',(-70.5504171012247,11.1140121902274,0.));
#86258=CARTESIAN_POINT('Ctrl Pts',(-70.5729933161538,11.1101300301701,0.));
#86259=CARTESIAN_POINT('Ctrl Pts',(-70.5956098890744,11.1062176543258,0.));
#86260=CARTESIAN_POINT('Ctrl Pts',(-70.6182666771441,11.102275019444,0.));
#86261=CARTESIAN_POINT('Ctrl Pts',(-70.6409635381446,11.0983020825662,0.));
#86262=CARTESIAN_POINT('Ctrl Pts',(-70.6637003304768,11.0942988010231,0.));
#86263=CARTESIAN_POINT('Ctrl Pts',(-70.686476913156,11.0902651324326,0.));
#86264=CARTESIAN_POINT('Ctrl Pts',(-70.7092931457996,11.0862010347022,0.));
#86265=CARTESIAN_POINT('Ctrl Pts',(-70.7321488886229,11.0821064660276,0.));
#86266=CARTESIAN_POINT('Ctrl Pts',(-70.7550440024422,11.0779813848851,0.));
#86267=CARTESIAN_POINT('Ctrl Pts',(-70.7779783486689,11.0738257500292,0.));
#86268=CARTESIAN_POINT('Ctrl Pts',(-70.8009517893042,11.0696395204908,0.));
#86269=CARTESIAN_POINT('Ctrl Pts',(-70.8239641869266,11.0654226555799,0.));
#86270=CARTESIAN_POINT('Ctrl Pts',(-70.847015404688,11.0611751148831,0.));
#86271=CARTESIAN_POINT('Ctrl Pts',(-70.8701053063158,11.0568968582566,0.));
#86272=CARTESIAN_POINT('Ctrl Pts',(-70.8932337561079,11.0525878458242,0.));
#86273=CARTESIAN_POINT('Ctrl Pts',(-70.9164006189283,11.0482480379752,0.));
#86274=CARTESIAN_POINT('Ctrl Pts',(-70.9396057601953,11.0438773953686,0.));
#86275=CARTESIAN_POINT('Ctrl Pts',(-70.9628490458779,11.039475878929,0.));
#86276=CARTESIAN_POINT('Ctrl Pts',(-70.9861303424989,11.0350434498408,0.));
#86277=CARTESIAN_POINT('Ctrl Pts',(-71.0094495171295,11.0305800695457,0.));
#86278=CARTESIAN_POINT('Ctrl Pts',(-71.0328064373849,11.0260856997415,0.));
#86279=CARTESIAN_POINT('Ctrl Pts',(-71.0562009714125,11.0215603023855,0.));
#86280=CARTESIAN_POINT('Ctrl Pts',(-71.0796329878896,11.0170038396913,0.));
#86281=CARTESIAN_POINT('Ctrl Pts',(-71.1031023560243,11.0124162741224,0.));
#86282=CARTESIAN_POINT('Ctrl Pts',(-71.1266089455517,11.0077975683895,0.));
#86283=CARTESIAN_POINT('Ctrl Pts',(-71.1501526267288,11.0031476854503,0.));
#86284=CARTESIAN_POINT('Ctrl Pts',(-71.1737332703248,10.9984665885127,0.));
#86285=CARTESIAN_POINT('Ctrl Pts',(-71.1973507476188,10.993754241032,0.));
#86286=CARTESIAN_POINT('Ctrl Pts',(-71.221004930401,10.9890106067039,0.));
#86287=CARTESIAN_POINT('Ctrl Pts',(-71.2446956909685,10.9842356494627,0.));
#86288=CARTESIAN_POINT('Ctrl Pts',(-71.2684229021209,10.9794293334806,0.));
#86289=CARTESIAN_POINT('Ctrl Pts',(-71.2921864371499,10.9745916231711,0.));
#86290=CARTESIAN_POINT('Ctrl Pts',(-71.3159861698368,10.9697224831863,0.));
#86291=CARTESIAN_POINT('Ctrl Pts',(-71.3398219744547,10.96482187841,0.));
#86292=CARTESIAN_POINT('Ctrl Pts',(-71.3636937257651,10.9598897739565,0.));
#86293=CARTESIAN_POINT('Ctrl Pts',(-71.3876012990135,10.954926135169,0.));
#86294=CARTESIAN_POINT('Ctrl Pts',(-71.411544569919,10.9499309276236,0.));
#86295=CARTESIAN_POINT('Ctrl Pts',(-71.4355234146718,10.9449041171269,0.));
#86296=CARTESIAN_POINT('Ctrl Pts',(-71.4595377099352,10.9398456697095,0.));
#86297=CARTESIAN_POINT('Ctrl Pts',(-71.4835873328425,10.9347555516236,0.));
#86298=CARTESIAN_POINT('Ctrl Pts',(-71.5076721609936,10.9296337293425,0.));
#86299=CARTESIAN_POINT('Ctrl Pts',(-71.5317920724453,10.9244801695642,0.));
#86300=CARTESIAN_POINT('Ctrl Pts',(-71.5559469457082,10.91929483921,0.));
#86301=CARTESIAN_POINT('Ctrl Pts',(-71.5801366597479,10.9140777054169,0.));
#86302=CARTESIAN_POINT('Ctrl Pts',(-71.604361093983,10.9088287355364,0.));
#86303=CARTESIAN_POINT('Ctrl Pts',(-71.6286201282815,10.9035478971329,0.));
#86304=CARTESIAN_POINT('Ctrl Pts',(-71.6529136429515,10.8982351579873,0.));
#86305=CARTESIAN_POINT('Ctrl Pts',(-71.6772415187382,10.8928904860967,0.));
#86306=CARTESIAN_POINT('Ctrl Pts',(-71.7016036368254,10.8875138496674,0.));
#86307=CARTESIAN_POINT('Ctrl Pts',(-71.7259998788337,10.8821052171122,0.));
#86308=CARTESIAN_POINT('Ctrl Pts',(-71.7504301268177,10.8766645570497,0.));
#86309=CARTESIAN_POINT('Ctrl Pts',(-71.7748942632578,10.8711918383071,0.));
#86310=CARTESIAN_POINT('Ctrl Pts',(-71.7993921710546,10.8656870299218,0.));
#86311=CARTESIAN_POINT('Ctrl Pts',(-71.8239237335317,10.860150101133,0.));
#86312=CARTESIAN_POINT('Ctrl Pts',(-71.8484888344335,10.8545810213799,0.));
#86313=CARTESIAN_POINT('Ctrl Pts',(-71.8730873579226,10.8489797602998,0.));
#86314=CARTESIAN_POINT('Ctrl Pts',(-71.8977191885726,10.8433462877312,0.));
#86315=CARTESIAN_POINT('Ctrl Pts',(-71.9223842113622,10.8376805737159,0.));
#86316=CARTESIAN_POINT('Ctrl Pts',(-71.9470823116777,10.8319825884917,0.));
#86317=CARTESIAN_POINT('Ctrl Pts',(-71.971813375312,10.8262523024897,0.));
#86318=CARTESIAN_POINT('Ctrl Pts',(-71.9965772884619,10.8204896863328,0.));
#86319=CARTESIAN_POINT('Ctrl Pts',(-72.0213739377231,10.8146947108377,0.));
#86320=CARTESIAN_POINT('Ctrl Pts',(-72.0462032100828,10.8088673470187,0.));
#86321=CARTESIAN_POINT('Ctrl Pts',(-72.0710649929214,10.8030075660812,0.));
#86322=CARTESIAN_POINT('Ctrl Pts',(-72.095959174012,10.7971153394168,0.));
#86323=CARTESIAN_POINT('Ctrl Pts',(-72.1208856415171,10.7911906386027,0.));
#86324=CARTESIAN_POINT('Ctrl Pts',(-72.145844283983,10.7852334354015,0.));
#86325=CARTESIAN_POINT('Ctrl Pts',(-72.17083499033,10.779243701766,0.));
#86326=CARTESIAN_POINT('Ctrl Pts',(-72.1958576498556,10.7732214098343,0.));
#86327=CARTESIAN_POINT('Ctrl Pts',(-72.2209121522367,10.7671665319254,0.));
#86328=CARTESIAN_POINT('Ctrl Pts',(-72.2459983875297,10.7610790405385,0.));
#86329=CARTESIAN_POINT('Ctrl Pts',(-72.2711162461679,10.7549589083536,0.));
#86330=CARTESIAN_POINT('Ctrl Pts',(-72.296265618955,10.7488061082368,0.));
#86331=CARTESIAN_POINT('Ctrl Pts',(-72.3214463970634,10.7426206132375,0.));
#86332=CARTESIAN_POINT('Ctrl Pts',(-72.3466584720311,10.73640239658,0.));
#86333=CARTESIAN_POINT('Ctrl Pts',(-72.3719017357568,10.7301514316607,0.));
#86334=CARTESIAN_POINT('Ctrl Pts',(-72.3971760804935,10.7238676920469,0.));
#86335=CARTESIAN_POINT('Ctrl Pts',(-72.4224813988355,10.7175511514789,0.));
#86336=CARTESIAN_POINT('Ctrl Pts',(-72.4478175837168,10.7112017838707,0.));
#86337=CARTESIAN_POINT('Ctrl Pts',(-72.4731845284238,10.7048195633062,0.));
#86338=CARTESIAN_POINT('Ctrl Pts',(-72.4985821266031,10.6984044640399,0.));
#86339=CARTESIAN_POINT('Ctrl Pts',(-72.5240102722662,10.6919564604991,0.));
#86340=CARTESIAN_POINT('Ctrl Pts',(-72.5494688597951,10.6854755272904,0.));
#86341=CARTESIAN_POINT('Ctrl Pts',(-72.57495778394,10.6789616392041,0.));
#86342=CARTESIAN_POINT('Ctrl Pts',(-72.6004769398004,10.6724147711994,0.));
#86343=CARTESIAN_POINT('Ctrl Pts',(-72.6260262228055,10.6658348983944,0.));
#86344=CARTESIAN_POINT('Ctrl Pts',(-72.6516055286908,10.6592219960581,0.));
#86345=CARTESIAN_POINT('Ctrl Pts',(-72.6772147534762,10.6525760396056,0.));
#86346=CARTESIAN_POINT('Ctrl Pts',(-72.7028537934332,10.6458970045948,0.));
#86347=CARTESIAN_POINT('Ctrl Pts',(-72.7285225451309,10.6391848667354,0.));
#86348=CARTESIAN_POINT('Ctrl Pts',(-72.7542209054823,10.6324396019,0.));
#86349=CARTESIAN_POINT('Ctrl Pts',(-72.7799487717914,10.6256611861395,0.));
#86350=CARTESIAN_POINT('Ctrl Pts',(-72.8057060417882,10.6188495956973,0.));
#86351=CARTESIAN_POINT('Ctrl Pts',(-72.8314926136872,10.6120048070367,0.));
#86352=CARTESIAN_POINT('Ctrl Pts',(-72.8573083861328,10.6051267968202,0.));
#86353=CARTESIAN_POINT('Ctrl Pts',(-72.8831532580839,10.5982155418625,0.));
#86354=CARTESIAN_POINT('Ctrl Pts',(-72.9090271287081,10.5912710190928,0.));
#86355=CARTESIAN_POINT('Ctrl Pts',(-72.9349298972823,10.5842932055209,0.));
#86356=CARTESIAN_POINT('Ctrl Pts',(-72.9608614630538,10.5772820781959,0.));
#86357=CARTESIAN_POINT('Ctrl Pts',(-72.9868217252293,10.5702376142052,0.));
#86358=CARTESIAN_POINT('Ctrl Pts',(-73.0128105832635,10.5631597907653,0.));
#86359=CARTESIAN_POINT('Ctrl Pts',(-73.0388279370845,10.5560485852976,0.));
#86360=CARTESIAN_POINT('Ctrl Pts',(-73.0648736873435,10.5489039755138,0.));
#86361=CARTESIAN_POINT('Ctrl Pts',(-73.090947735646,10.5417259395001,0.));
#86362=CARTESIAN_POINT('Ctrl Pts',(-73.1170499848012,10.5345144558097,0.));
#86363=CARTESIAN_POINT('Ctrl Pts',(-73.1431803382677,10.5272695032649,0.));
#86364=CARTESIAN_POINT('Ctrl Pts',(-73.169338699611,10.5199910607652,0.));
#86365=CARTESIAN_POINT('Ctrl Pts',(-73.1955249719037,10.5126791070804,0.));
#86366=CARTESIAN_POINT('Ctrl Pts',(-73.2217390572578,10.505333620691,0.));
#86367=CARTESIAN_POINT('Ctrl Pts',(-73.247980856023,10.4979545795197,0.));
#86368=CARTESIAN_POINT('Ctrl Pts',(-73.2742502674361,10.4905419611529,0.));
#86369=CARTESIAN_POINT('Ctrl Pts',(-73.3005471910639,10.4830957433311,0.));
#86370=CARTESIAN_POINT('Ctrl Pts',(-73.3268715280609,10.475615904381,0.));
#86371=CARTESIAN_POINT('Ctrl Pts',(-73.353223182365,10.4681024236288,0.));
#86372=CARTESIAN_POINT('Ctrl Pts',(-73.3796020622436,10.4605552819391,0.));
#86373=CARTESIAN_POINT('Ctrl Pts',(-73.4060080806577,10.4529744618439,0.));
#86374=CARTESIAN_POINT('Ctrl Pts',(-73.4286663447914,10.4464473465487,0.));
#86375=CARTESIAN_POINT('Ctrl Pts',(-73.4460525528549,10.4414249334769,0.));
#86376=CARTESIAN_POINT('Ctrl Pts',(-73.4581547436537,10.4379221501094,0.));
#86377=CARTESIAN_POINT('Ctrl Pts',(-73.4649650361537,10.4359488742884,0.));
#86378=CARTESIAN_POINT('Ctrl Pts',(-73.4664795929515,10.4355099267392,0.));
#86379=CARTESIAN_POINT('',(-69.079679653846,11.3136138754166,12.));
#86380=CARTESIAN_POINT('',(-69.079679653846,11.3136138754166,0.));
#86381=CARTESIAN_POINT('Ctrl Pts',(-73.4664795929515,10.4355099267392,12.));
#86382=CARTESIAN_POINT('Ctrl Pts',(-73.4649650361537,10.4359488742884,12.));
#86383=CARTESIAN_POINT('Ctrl Pts',(-73.4581547436537,10.4379221501094,12.));
#86384=CARTESIAN_POINT('Ctrl Pts',(-73.4460525528549,10.4414249334769,12.));
#86385=CARTESIAN_POINT('Ctrl Pts',(-73.4286663447914,10.4464473465487,12.));
#86386=CARTESIAN_POINT('Ctrl Pts',(-73.4060080806577,10.4529744618439,12.));
#86387=CARTESIAN_POINT('Ctrl Pts',(-73.3796020622436,10.4605552819391,12.));
#86388=CARTESIAN_POINT('Ctrl Pts',(-73.353223182365,10.4681024236288,12.));
#86389=CARTESIAN_POINT('Ctrl Pts',(-73.3268715280609,10.475615904381,12.));
#86390=CARTESIAN_POINT('Ctrl Pts',(-73.3005471910639,10.4830957433311,12.));
#86391=CARTESIAN_POINT('Ctrl Pts',(-73.2742502674361,10.4905419611529,12.));
#86392=CARTESIAN_POINT('Ctrl Pts',(-73.247980856023,10.4979545795197,12.));
#86393=CARTESIAN_POINT('Ctrl Pts',(-73.2217390572578,10.505333620691,12.));
#86394=CARTESIAN_POINT('Ctrl Pts',(-73.1955249719037,10.5126791070804,12.));
#86395=CARTESIAN_POINT('Ctrl Pts',(-73.169338699611,10.5199910607652,12.));
#86396=CARTESIAN_POINT('Ctrl Pts',(-73.1431803382677,10.5272695032649,12.));
#86397=CARTESIAN_POINT('Ctrl Pts',(-73.1170499848012,10.5345144558097,12.));
#86398=CARTESIAN_POINT('Ctrl Pts',(-73.090947735646,10.5417259395001,12.));
#86399=CARTESIAN_POINT('Ctrl Pts',(-73.0648736873435,10.5489039755138,12.));
#86400=CARTESIAN_POINT('Ctrl Pts',(-73.0388279370845,10.5560485852976,12.));
#86401=CARTESIAN_POINT('Ctrl Pts',(-73.0128105832635,10.5631597907653,12.));
#86402=CARTESIAN_POINT('Ctrl Pts',(-72.9868217252293,10.5702376142052,12.));
#86403=CARTESIAN_POINT('Ctrl Pts',(-72.9608614630538,10.5772820781959,12.));
#86404=CARTESIAN_POINT('Ctrl Pts',(-72.9349298972823,10.5842932055209,12.));
#86405=CARTESIAN_POINT('Ctrl Pts',(-72.9090271287081,10.5912710190928,12.));
#86406=CARTESIAN_POINT('Ctrl Pts',(-72.8831532580839,10.5982155418625,12.));
#86407=CARTESIAN_POINT('Ctrl Pts',(-72.8573083861328,10.6051267968202,12.));
#86408=CARTESIAN_POINT('Ctrl Pts',(-72.8314926136872,10.6120048070367,12.));
#86409=CARTESIAN_POINT('Ctrl Pts',(-72.8057060417882,10.6188495956973,12.));
#86410=CARTESIAN_POINT('Ctrl Pts',(-72.7799487717914,10.6256611861395,12.));
#86411=CARTESIAN_POINT('Ctrl Pts',(-72.7542209054823,10.6324396019,12.));
#86412=CARTESIAN_POINT('Ctrl Pts',(-72.7285225451309,10.6391848667354,12.));
#86413=CARTESIAN_POINT('Ctrl Pts',(-72.7028537934332,10.6458970045948,12.));
#86414=CARTESIAN_POINT('Ctrl Pts',(-72.6772147534762,10.6525760396056,12.));
#86415=CARTESIAN_POINT('Ctrl Pts',(-72.6516055286908,10.6592219960581,12.));
#86416=CARTESIAN_POINT('Ctrl Pts',(-72.6260262228055,10.6658348983944,12.));
#86417=CARTESIAN_POINT('Ctrl Pts',(-72.6004769398004,10.6724147711994,12.));
#86418=CARTESIAN_POINT('Ctrl Pts',(-72.57495778394,10.6789616392041,12.));
#86419=CARTESIAN_POINT('Ctrl Pts',(-72.5494688597951,10.6854755272904,12.));
#86420=CARTESIAN_POINT('Ctrl Pts',(-72.5240102722662,10.6919564604991,12.));
#86421=CARTESIAN_POINT('Ctrl Pts',(-72.4985821266031,10.6984044640399,12.));
#86422=CARTESIAN_POINT('Ctrl Pts',(-72.4731845284238,10.7048195633062,12.));
#86423=CARTESIAN_POINT('Ctrl Pts',(-72.4478175837168,10.7112017838707,12.));
#86424=CARTESIAN_POINT('Ctrl Pts',(-72.4224813988355,10.7175511514789,12.));
#86425=CARTESIAN_POINT('Ctrl Pts',(-72.3971760804935,10.7238676920469,12.));
#86426=CARTESIAN_POINT('Ctrl Pts',(-72.3719017357568,10.7301514316607,12.));
#86427=CARTESIAN_POINT('Ctrl Pts',(-72.3466584720311,10.73640239658,12.));
#86428=CARTESIAN_POINT('Ctrl Pts',(-72.3214463970634,10.7426206132375,12.));
#86429=CARTESIAN_POINT('Ctrl Pts',(-72.296265618955,10.7488061082368,12.));
#86430=CARTESIAN_POINT('Ctrl Pts',(-72.2711162461679,10.7549589083536,12.));
#86431=CARTESIAN_POINT('Ctrl Pts',(-72.2459983875297,10.7610790405385,12.));
#86432=CARTESIAN_POINT('Ctrl Pts',(-72.2209121522367,10.7671665319254,12.));
#86433=CARTESIAN_POINT('Ctrl Pts',(-72.1958576498556,10.7732214098343,12.));
#86434=CARTESIAN_POINT('Ctrl Pts',(-72.17083499033,10.779243701766,12.));
#86435=CARTESIAN_POINT('Ctrl Pts',(-72.145844283983,10.7852334354015,12.));
#86436=CARTESIAN_POINT('Ctrl Pts',(-72.1208856415171,10.7911906386027,12.));
#86437=CARTESIAN_POINT('Ctrl Pts',(-72.095959174012,10.7971153394168,12.));
#86438=CARTESIAN_POINT('Ctrl Pts',(-72.0710649929214,10.8030075660812,12.));
#86439=CARTESIAN_POINT('Ctrl Pts',(-72.0462032100828,10.8088673470187,12.));
#86440=CARTESIAN_POINT('Ctrl Pts',(-72.0213739377231,10.8146947108377,12.));
#86441=CARTESIAN_POINT('Ctrl Pts',(-71.9965772884619,10.8204896863328,12.));
#86442=CARTESIAN_POINT('Ctrl Pts',(-71.971813375312,10.8262523024897,12.));
#86443=CARTESIAN_POINT('Ctrl Pts',(-71.9470823116777,10.8319825884917,12.));
#86444=CARTESIAN_POINT('Ctrl Pts',(-71.9223842113622,10.8376805737159,12.));
#86445=CARTESIAN_POINT('Ctrl Pts',(-71.8977191885726,10.8433462877312,12.));
#86446=CARTESIAN_POINT('Ctrl Pts',(-71.8730873579226,10.8489797602998,12.));
#86447=CARTESIAN_POINT('Ctrl Pts',(-71.8484888344335,10.8545810213799,12.));
#86448=CARTESIAN_POINT('Ctrl Pts',(-71.8239237335317,10.860150101133,12.));
#86449=CARTESIAN_POINT('Ctrl Pts',(-71.7993921710546,10.8656870299218,12.));
#86450=CARTESIAN_POINT('Ctrl Pts',(-71.7748942632578,10.8711918383071,12.));
#86451=CARTESIAN_POINT('Ctrl Pts',(-71.7504301268177,10.8766645570497,12.));
#86452=CARTESIAN_POINT('Ctrl Pts',(-71.7259998788337,10.8821052171122,12.));
#86453=CARTESIAN_POINT('Ctrl Pts',(-71.7016036368254,10.8875138496674,12.));
#86454=CARTESIAN_POINT('Ctrl Pts',(-71.6772415187382,10.8928904860967,12.));
#86455=CARTESIAN_POINT('Ctrl Pts',(-71.6529136429515,10.8982351579873,12.));
#86456=CARTESIAN_POINT('Ctrl Pts',(-71.6286201282815,10.9035478971329,12.));
#86457=CARTESIAN_POINT('Ctrl Pts',(-71.604361093983,10.9088287355364,12.));
#86458=CARTESIAN_POINT('Ctrl Pts',(-71.5801366597479,10.9140777054169,12.));
#86459=CARTESIAN_POINT('Ctrl Pts',(-71.5559469457082,10.91929483921,12.));
#86460=CARTESIAN_POINT('Ctrl Pts',(-71.5317920724453,10.9244801695642,12.));
#86461=CARTESIAN_POINT('Ctrl Pts',(-71.5076721609936,10.9296337293425,12.));
#86462=CARTESIAN_POINT('Ctrl Pts',(-71.4835873328425,10.9347555516236,12.));
#86463=CARTESIAN_POINT('Ctrl Pts',(-71.4595377099352,10.9398456697095,12.));
#86464=CARTESIAN_POINT('Ctrl Pts',(-71.4355234146718,10.9449041171269,12.));
#86465=CARTESIAN_POINT('Ctrl Pts',(-71.411544569919,10.9499309276236,12.));
#86466=CARTESIAN_POINT('Ctrl Pts',(-71.3876012990135,10.954926135169,12.));
#86467=CARTESIAN_POINT('Ctrl Pts',(-71.3636937257651,10.9598897739565,12.));
#86468=CARTESIAN_POINT('Ctrl Pts',(-71.3398219744547,10.96482187841,12.));
#86469=CARTESIAN_POINT('Ctrl Pts',(-71.3159861698368,10.9697224831863,12.));
#86470=CARTESIAN_POINT('Ctrl Pts',(-71.2921864371499,10.9745916231711,12.));
#86471=CARTESIAN_POINT('Ctrl Pts',(-71.2684229021209,10.9794293334806,12.));
#86472=CARTESIAN_POINT('Ctrl Pts',(-71.2446956909685,10.9842356494627,12.));
#86473=CARTESIAN_POINT('Ctrl Pts',(-71.221004930401,10.9890106067039,12.));
#86474=CARTESIAN_POINT('Ctrl Pts',(-71.1973507476188,10.993754241032,12.));
#86475=CARTESIAN_POINT('Ctrl Pts',(-71.1737332703248,10.9984665885127,12.));
#86476=CARTESIAN_POINT('Ctrl Pts',(-71.1501526267288,11.0031476854503,12.));
#86477=CARTESIAN_POINT('Ctrl Pts',(-71.1266089455517,11.0077975683895,12.));
#86478=CARTESIAN_POINT('Ctrl Pts',(-71.1031023560243,11.0124162741224,12.));
#86479=CARTESIAN_POINT('Ctrl Pts',(-71.0796329878896,11.0170038396913,12.));
#86480=CARTESIAN_POINT('Ctrl Pts',(-71.0562009714125,11.0215603023855,12.));
#86481=CARTESIAN_POINT('Ctrl Pts',(-71.0328064373849,11.0260856997415,12.));
#86482=CARTESIAN_POINT('Ctrl Pts',(-71.0094495171295,11.0305800695457,12.));
#86483=CARTESIAN_POINT('Ctrl Pts',(-70.9861303424989,11.0350434498408,12.));
#86484=CARTESIAN_POINT('Ctrl Pts',(-70.9628490458779,11.039475878929,12.));
#86485=CARTESIAN_POINT('Ctrl Pts',(-70.9396057601953,11.0438773953686,12.));
#86486=CARTESIAN_POINT('Ctrl Pts',(-70.9164006189283,11.0482480379752,12.));
#86487=CARTESIAN_POINT('Ctrl Pts',(-70.8932337561079,11.0525878458242,12.));
#86488=CARTESIAN_POINT('Ctrl Pts',(-70.8701053063158,11.0568968582566,12.));
#86489=CARTESIAN_POINT('Ctrl Pts',(-70.847015404688,11.0611751148831,12.));
#86490=CARTESIAN_POINT('Ctrl Pts',(-70.8239641869266,11.0654226555799,12.));
#86491=CARTESIAN_POINT('Ctrl Pts',(-70.8009517893042,11.0696395204908,12.));
#86492=CARTESIAN_POINT('Ctrl Pts',(-70.7779783486689,11.0738257500292,12.));
#86493=CARTESIAN_POINT('Ctrl Pts',(-70.7550440024422,11.0779813848851,12.));
#86494=CARTESIAN_POINT('Ctrl Pts',(-70.7321488886229,11.0821064660276,12.));
#86495=CARTESIAN_POINT('Ctrl Pts',(-70.7092931457996,11.0862010347022,12.));
#86496=CARTESIAN_POINT('Ctrl Pts',(-70.686476913156,11.0902651324326,12.));
#86497=CARTESIAN_POINT('Ctrl Pts',(-70.6637003304768,11.0942988010231,12.));
#86498=CARTESIAN_POINT('Ctrl Pts',(-70.6409635381446,11.0983020825662,12.));
#86499=CARTESIAN_POINT('Ctrl Pts',(-70.6182666771441,11.102275019444,12.));
#86500=CARTESIAN_POINT('Ctrl Pts',(-70.5956098890744,11.1062176543258,12.));
#86501=CARTESIAN_POINT('Ctrl Pts',(-70.5729933161538,11.1101300301701,12.));
#86502=CARTESIAN_POINT('Ctrl Pts',(-70.5504171012247,11.1140121902274,12.));
#86503=CARTESIAN_POINT('Ctrl Pts',(-70.5278813877519,11.117864178048,12.));
#86504=CARTESIAN_POINT('Ctrl Pts',(-70.5053863198306,11.121686037483,12.));
#86505=CARTESIAN_POINT('Ctrl Pts',(-70.4829320421973,11.1254778126824,12.));
#86506=CARTESIAN_POINT('Ctrl Pts',(-70.4605187002356,11.1292395480975,12.));
#86507=CARTESIAN_POINT('Ctrl Pts',(-70.438146439981,11.1329712884845,12.));
#86508=CARTESIAN_POINT('Ctrl Pts',(-70.415815408119,11.1366730789123,12.));
#86509=CARTESIAN_POINT('Ctrl Pts',(-70.3935257519945,11.1403449647622,12.));
#86510=CARTESIAN_POINT('Ctrl Pts',(-70.3712776196216,11.1439869917269,12.));
#86511=CARTESIAN_POINT('Ctrl Pts',(-70.3490711596882,11.1475992058124,12.));
#86512=CARTESIAN_POINT('Ctrl Pts',(-70.3269065215591,11.1511816533422,12.));
#86513=CARTESIAN_POINT('Ctrl Pts',(-70.3047838552757,11.1547343809647,12.));
#86514=CARTESIAN_POINT('Ctrl Pts',(-70.2827033115662,11.1582574356522,12.));
#86515=CARTESIAN_POINT('Ctrl Pts',(-70.2606650418589,11.1617508647017,12.));
#86516=CARTESIAN_POINT('Ctrl Pts',(-70.2386691982902,11.1652147157383,12.));
#86517=CARTESIAN_POINT('Ctrl Pts',(-70.2167159337095,11.168649036721,12.));
#86518=CARTESIAN_POINT('Ctrl Pts',(-70.1948054016817,11.1720538759499,12.));
#86519=CARTESIAN_POINT('Ctrl Pts',(-70.1729377564956,11.1754292820631,12.));
#86520=CARTESIAN_POINT('Ctrl Pts',(-70.1511131531674,11.1787753040363,12.));
#86521=CARTESIAN_POINT('Ctrl Pts',(-70.1293317474432,11.1820919911846,12.));
#86522=CARTESIAN_POINT('Ctrl Pts',(-70.1075936957968,11.185379393167,12.));
#86523=CARTESIAN_POINT('Ctrl Pts',(-70.0858991554283,11.1886375599914,12.));
#86524=CARTESIAN_POINT('Ctrl Pts',(-70.0642482842928,11.1918665420167,12.));
#86525=CARTESIAN_POINT('Ctrl Pts',(-70.0426412411185,11.1950663899577,12.));
#86526=CARTESIAN_POINT('Ctrl Pts',(-70.0210781854243,11.1982371548919,12.));
#86527=CARTESIAN_POINT('Ctrl Pts',(-69.9995592775343,11.2013788882714,12.));
#86528=CARTESIAN_POINT('Ctrl Pts',(-69.97808467858,11.2044916419244,12.));
#86529=CARTESIAN_POINT('Ctrl Pts',(-69.9566545504837,11.2075754680449,12.));
#86530=CARTESIAN_POINT('Ctrl Pts',(-69.9352690559405,11.2106304191883,12.));
#86531=CARTESIAN_POINT('Ctrl Pts',(-69.9139283584021,11.2136565482678,12.));
#86532=CARTESIAN_POINT('Ctrl Pts',(-69.8926326220385,11.2166539085523,12.));
#86533=CARTESIAN_POINT('Ctrl Pts',(-69.871382011789,11.219622553679,12.));
#86534=CARTESIAN_POINT('Ctrl Pts',(-69.8501766934428,11.2225625376737,12.));
#86535=CARTESIAN_POINT('Ctrl Pts',(-69.8290168337076,11.2254739149721,12.));
#86536=CARTESIAN_POINT('Ctrl Pts',(-69.8079026002768,11.2283567404437,12.));
#86537=CARTESIAN_POINT('Ctrl Pts',(-69.7868341618954,11.2312110694188,12.));
#86538=CARTESIAN_POINT('Ctrl Pts',(-69.7658116882324,11.2340369576456,12.));
#86539=CARTESIAN_POINT('Ctrl Pts',(-69.7448353497408,11.2368344612473,12.));
#86540=CARTESIAN_POINT('Ctrl Pts',(-69.7239053175356,11.239603636686,12.));
#86541=CARTESIAN_POINT('Ctrl Pts',(-69.7030217632164,11.2423445407167,12.));
#86542=CARTESIAN_POINT('Ctrl Pts',(-69.6821848588457,11.2450572303841,12.));
#86543=CARTESIAN_POINT('Ctrl Pts',(-69.6613947773534,11.2477417631386,12.));
#86544=CARTESIAN_POINT('Ctrl Pts',(-69.6406516928891,11.2503981969412,12.));
#86545=CARTESIAN_POINT('Ctrl Pts',(-69.6199557811245,11.2530265903558,12.));
#86546=CARTESIAN_POINT('Ctrl Pts',(-69.599307219739,11.2556270027016,12.));
#86547=CARTESIAN_POINT('Ctrl Pts',(-69.5787061880857,11.2581994939541,12.));
#86548=CARTESIAN_POINT('Ctrl Pts',(-69.5581528662877,11.2607441244703,12.));
#86549=CARTESIAN_POINT('Ctrl Pts',(-69.5376474344771,11.263260954763,12.));
#86550=CARTESIAN_POINT('Ctrl Pts',(-69.5171900720158,11.2657500452716,12.));
#86551=CARTESIAN_POINT('Ctrl Pts',(-69.4967809565929,11.2682114561008,12.));
#86552=CARTESIAN_POINT('Ctrl Pts',(-69.4764202659397,11.270645247528,12.));
#86553=CARTESIAN_POINT('Ctrl Pts',(-69.456108179879,11.2730514806139,12.));
#86554=CARTESIAN_POINT('Ctrl Pts',(-69.4358448819967,11.2754302177021,12.));
#86555=CARTESIAN_POINT('Ctrl Pts',(-69.4156305620593,11.2777815231469,12.));
#86556=CARTESIAN_POINT('Ctrl Pts',(-69.3954654162281,11.2801054633816,12.));
#86557=CARTESIAN_POINT('Ctrl Pts',(-69.3753496420039,11.2824021054045,12.));
#86558=CARTESIAN_POINT('Ctrl Pts',(-69.3552834337784,11.2846715154524,12.));
#86559=CARTESIAN_POINT('Ctrl Pts',(-69.3352669789587,11.2869137578459,12.));
#86560=CARTESIAN_POINT('Ctrl Pts',(-69.3153004517783,11.2891288931517,12.));
#86561=CARTESIAN_POINT('Ctrl Pts',(-69.295384019272,11.2913169799628,12.));
#86562=CARTESIAN_POINT('Ctrl Pts',(-69.2755178531479,11.2934780784351,12.));
#86563=CARTESIAN_POINT('Ctrl Pts',(-69.255702139335,11.2956122531375,12.));
#86564=CARTESIAN_POINT('Ctrl Pts',(-69.2359370894907,11.2977195764853,12.));
#86565=CARTESIAN_POINT('Ctrl Pts',(-69.2162229488531,11.2998001310964,12.));
#86566=CARTESIAN_POINT('Ctrl Pts',(-69.1965599718914,11.3018540025638,12.));
#86567=CARTESIAN_POINT('Ctrl Pts',(-69.1769483991721,11.3038812726293,12.));
#86568=CARTESIAN_POINT('Ctrl Pts',(-69.1573884361,11.3058820128308,12.));
#86569=CARTESIAN_POINT('Ctrl Pts',(-69.1378802251711,11.3078562764385,12.));
#86570=CARTESIAN_POINT('Ctrl Pts',(-69.118423844466,11.3098040973713,12.));
#86571=CARTESIAN_POINT('Ctrl Pts',(-69.1029002322118,11.3113412156662,12.));
#86572=CARTESIAN_POINT('Ctrl Pts',(-69.0912808656811,11.3124821678798,12.));
#86573=CARTESIAN_POINT('Ctrl Pts',(-69.0835449954396,11.3132375200165,12.));
#86574=CARTESIAN_POINT('Ctrl Pts',(-69.079679653846,11.3136138754166,12.));
#86575=CARTESIAN_POINT('Ctrl Pts',(-73.6640787198055,8.93459554657839,0.));
#86576=CARTESIAN_POINT('Ctrl Pts',(-73.6640787198055,8.93459554657839,4.));
#86577=CARTESIAN_POINT('Ctrl Pts',(-73.6640787198055,8.93459554657838,8.));
#86578=CARTESIAN_POINT('Ctrl Pts',(-73.6640787198055,8.93459554657838,12.));
#86579=CARTESIAN_POINT('Ctrl Pts',(-73.7581053903594,8.99145626777888,0.));
#86580=CARTESIAN_POINT('Ctrl Pts',(-73.7581053903594,8.99145626777888,4.));
#86581=CARTESIAN_POINT('Ctrl Pts',(-73.7581053903594,8.99145626777887,8.));
#86582=CARTESIAN_POINT('Ctrl Pts',(-73.7581053903594,8.99145626777887,12.));
#86583=CARTESIAN_POINT('Ctrl Pts',(-73.8880618019209,9.14696952162286,0.));
#86584=CARTESIAN_POINT('Ctrl Pts',(-73.8880618019209,9.14696952162286,4.));
#86585=CARTESIAN_POINT('Ctrl Pts',(-73.8880618019209,9.14696952162285,8.));
#86586=CARTESIAN_POINT('Ctrl Pts',(-73.8880618019209,9.14696952162285,12.));
#86587=CARTESIAN_POINT('Ctrl Pts',(-73.9117532086773,9.34395683490519,0.));
#86588=CARTESIAN_POINT('Ctrl Pts',(-73.9117532086773,9.34395683490519,4.));
#86589=CARTESIAN_POINT('Ctrl Pts',(-73.9117532086773,9.34395683490518,8.00000000000001));
#86590=CARTESIAN_POINT('Ctrl Pts',(-73.9117532086773,9.34395683490518,12.));
#86591=CARTESIAN_POINT('Ctrl Pts',(-73.9013264985866,9.42570643237552,0.));
#86592=CARTESIAN_POINT('Ctrl Pts',(-73.9013264985866,9.42570643237552,4.));
#86593=CARTESIAN_POINT('Ctrl Pts',(-73.9013264985866,9.42570643237552,8.));
#86594=CARTESIAN_POINT('Ctrl Pts',(-73.9013264985866,9.42570643237552,12.));
#86595=CARTESIAN_POINT('',(-73.6640787198055,8.9345955465784,0.));
#86596=CARTESIAN_POINT('',(-73.9013264985865,9.42570643237551,0.));
#86597=CARTESIAN_POINT('Ctrl Pts',(-73.6640787198055,8.93459554657839,1.8809784878848E-35));
#86598=CARTESIAN_POINT('Ctrl Pts',(-73.7581053903594,8.99145626777888,1.8809784878848E-35));
#86599=CARTESIAN_POINT('Ctrl Pts',(-73.832366196966,9.08032098426116,1.8809784878848E-35));
#86600=CARTESIAN_POINT('Ctrl Pts',(-73.8719282264933,9.18272825076412,1.8809784878848E-35));
#86601=CARTESIAN_POINT('Ctrl Pts',(-73.9015997486389,9.25953370064133,1.8809784878848E-35));
#86602=CARTESIAN_POINT('Ctrl Pts',(-73.9117532086773,9.34395683490519,1.88097848788479E-35));
#86603=CARTESIAN_POINT('Ctrl Pts',(-73.9013264985866,9.42570643237552,1.8809784878848E-35));
#86604=CARTESIAN_POINT('',(-73.9013264985865,9.4257064323755,12.));
#86605=CARTESIAN_POINT('Ctrl Pts',(-73.9013264985866,9.42570643237552,0.));
#86606=CARTESIAN_POINT('Ctrl Pts',(-73.9013264985866,9.42570643237552,4.));
#86607=CARTESIAN_POINT('Ctrl Pts',(-73.9013264985866,9.42570643237552,8.));
#86608=CARTESIAN_POINT('Ctrl Pts',(-73.9013264985866,9.42570643237552,12.));
#86609=CARTESIAN_POINT('',(-73.6640787198055,8.93459554657838,12.));
#86610=CARTESIAN_POINT('Ctrl Pts',(-73.9013264985866,9.42570643237552,12.));
#86611=CARTESIAN_POINT('Ctrl Pts',(-73.9117532086773,9.34395683490518,12.));
#86612=CARTESIAN_POINT('Ctrl Pts',(-73.9015997486388,9.25953370064132,12.));
#86613=CARTESIAN_POINT('Ctrl Pts',(-73.8719282264933,9.1827282507641,12.));
#86614=CARTESIAN_POINT('Ctrl Pts',(-73.832366196966,9.08032098426114,12.));
#86615=CARTESIAN_POINT('Ctrl Pts',(-73.7581053903594,8.99145626777887,12.));
#86616=CARTESIAN_POINT('Ctrl Pts',(-73.6640787198055,8.93459554657838,12.));
#86617=CARTESIAN_POINT('Ctrl Pts',(-73.6640787198055,8.93459554657838,12.));
#86618=CARTESIAN_POINT('Ctrl Pts',(-73.6640787198055,8.93459554657838,8.));
#86619=CARTESIAN_POINT('Ctrl Pts',(-73.6640787198055,8.93459554657839,4.));
#86620=CARTESIAN_POINT('Ctrl Pts',(-73.6640787198055,8.93459554657839,0.));
#86621=CARTESIAN_POINT('Origin',(-3.71649880366789E-10,4.88285199465433E-11,
0.));
#86622=CARTESIAN_POINT('Origin',(-3.71649880366789E-10,4.88285199465433E-11,
12.));
#86623=CARTESIAN_POINT('Origin',(-3.71649880366789E-10,4.88285199465433E-11,
0.));
#86624=CARTESIAN_POINT('Ctrl Pts',(-72.6683126419591,16.4184755008035,0.));
#86625=CARTESIAN_POINT('Ctrl Pts',(-72.6683126419591,16.4184755008035,4.));
#86626=CARTESIAN_POINT('Ctrl Pts',(-72.6683126419591,16.4184755008035,8.));
#86627=CARTESIAN_POINT('Ctrl Pts',(-72.6683126419591,16.4184755008035,12.));
#86628=CARTESIAN_POINT('Ctrl Pts',(-72.6440964999409,16.525656351978,0.));
#86629=CARTESIAN_POINT('Ctrl Pts',(-72.6440964999409,16.525656351978,4.));
#86630=CARTESIAN_POINT('Ctrl Pts',(-72.6440964999409,16.525656351978,8.));
#86631=CARTESIAN_POINT('Ctrl Pts',(-72.6440964999409,16.525656351978,12.));
#86632=CARTESIAN_POINT('Ctrl Pts',(-72.5376471652843,16.698113384133,0.));
#86633=CARTESIAN_POINT('Ctrl Pts',(-72.5376471652843,16.698113384133,4.));
#86634=CARTESIAN_POINT('Ctrl Pts',(-72.5376471652843,16.698113384133,8.));
#86635=CARTESIAN_POINT('Ctrl Pts',(-72.5376471652843,16.698113384133,12.));
#86636=CARTESIAN_POINT('Ctrl Pts',(-72.3582555997242,16.7828708182978,0.));
#86637=CARTESIAN_POINT('Ctrl Pts',(-72.3582555997242,16.7828708182978,4.));
#86638=CARTESIAN_POINT('Ctrl Pts',(-72.3582555997242,16.7828708182978,7.99999999999999));
#86639=CARTESIAN_POINT('Ctrl Pts',(-72.3582555997242,16.7828708182978,12.));
#86640=CARTESIAN_POINT('Ctrl Pts',(-72.2774028393482,16.798825256881,0.));
#86641=CARTESIAN_POINT('Ctrl Pts',(-72.2774028393482,16.798825256881,4.));
#86642=CARTESIAN_POINT('Ctrl Pts',(-72.2774028393482,16.798825256881,8.));
#86643=CARTESIAN_POINT('Ctrl Pts',(-72.2774028393482,16.798825256881,12.));
#86644=CARTESIAN_POINT('',(-72.6683126419591,16.4184755008035,0.));
#86645=CARTESIAN_POINT('',(-72.2774028393482,16.7988252568807,0.));
#86646=CARTESIAN_POINT('Ctrl Pts',(-72.6683126419591,16.4184755008035,2.77555756156289E-16));
#86647=CARTESIAN_POINT('Ctrl Pts',(-72.6440964999409,16.525656351978,2.77555756156289E-16));
#86648=CARTESIAN_POINT('Ctrl Pts',(-72.5832683087086,16.6242032274951,2.77555756156289E-16));
#86649=CARTESIAN_POINT('Ctrl Pts',(-72.4986222461608,16.6941134995869,2.77555756156289E-16));
#86650=CARTESIAN_POINT('Ctrl Pts',(-72.4351376992499,16.7465462036557,2.77555756156289E-16));
#86651=CARTESIAN_POINT('Ctrl Pts',(-72.3582555997242,16.7828708182978,2.77555756156289E-16));
#86652=CARTESIAN_POINT('Ctrl Pts',(-72.2774028393482,16.798825256881,2.77555756156289E-16));
#86653=CARTESIAN_POINT('',(-72.2774028393482,16.7988252568807,12.));
#86654=CARTESIAN_POINT('Ctrl Pts',(-72.2774028393482,16.798825256881,0.));
#86655=CARTESIAN_POINT('Ctrl Pts',(-72.2774028393482,16.798825256881,4.));
#86656=CARTESIAN_POINT('Ctrl Pts',(-72.2774028393482,16.798825256881,8.));
#86657=CARTESIAN_POINT('Ctrl Pts',(-72.2774028393482,16.798825256881,12.));
#86658=CARTESIAN_POINT('',(-72.6683126419591,16.4184755008035,12.));
#86659=CARTESIAN_POINT('Ctrl Pts',(-72.2774028393482,16.798825256881,12.));
#86660=CARTESIAN_POINT('Ctrl Pts',(-72.3582555997242,16.7828708182978,12.));
#86661=CARTESIAN_POINT('Ctrl Pts',(-72.4351376992499,16.7465462036557,12.));
#86662=CARTESIAN_POINT('Ctrl Pts',(-72.4986222461608,16.6941134995869,12.));
#86663=CARTESIAN_POINT('Ctrl Pts',(-72.5832683087086,16.6242032274951,12.));
#86664=CARTESIAN_POINT('Ctrl Pts',(-72.6440964999409,16.525656351978,12.));
#86665=CARTESIAN_POINT('Ctrl Pts',(-72.6683126419591,16.4184755008035,12.));
#86666=CARTESIAN_POINT('Ctrl Pts',(-72.6683126419591,16.4184755008035,12.));
#86667=CARTESIAN_POINT('Ctrl Pts',(-72.6683126419591,16.4184755008035,8.));
#86668=CARTESIAN_POINT('Ctrl Pts',(-72.6683126419591,16.4184755008035,4.));
#86669=CARTESIAN_POINT('Ctrl Pts',(-72.6683126419591,16.4184755008035,0.));
#86670=CARTESIAN_POINT('Ctrl Pts',(-67.8307641965654,17.2912529479484,0.));
#86671=CARTESIAN_POINT('Ctrl Pts',(-67.8307641965654,17.2912529479484,12.));
#86672=CARTESIAN_POINT('Ctrl Pts',(-67.8346476309018,17.2912149114119,0.));
#86673=CARTESIAN_POINT('Ctrl Pts',(-67.8346476309018,17.2912149114119,12.));
#86674=CARTESIAN_POINT('Ctrl Pts',(-67.842419897098,17.2911366591348,0.));
#86675=CARTESIAN_POINT('Ctrl Pts',(-67.842419897098,17.2911366591348,12.));
#86676=CARTESIAN_POINT('Ctrl Pts',(-67.8540944889687,17.291012743109,0.));
#86677=CARTESIAN_POINT('Ctrl Pts',(-67.8540944889687,17.291012743109,12.));
#86678=CARTESIAN_POINT('Ctrl Pts',(-67.8696929978782,17.2908344459695,0.));
#86679=CARTESIAN_POINT('Ctrl Pts',(-67.8696929978782,17.2908344459695,12.));
#86680=CARTESIAN_POINT('Ctrl Pts',(-67.8892451049608,17.2905897723949,0.));
#86681=CARTESIAN_POINT('Ctrl Pts',(-67.8892451049608,17.2905897723949,12.));
#86682=CARTESIAN_POINT('Ctrl Pts',(-67.9088511496685,17.2903232740694,0.));
#86683=CARTESIAN_POINT('Ctrl Pts',(-67.9088511496685,17.2903232740694,12.));
#86684=CARTESIAN_POINT('Ctrl Pts',(-67.9285110571741,17.2900349103981,0.));
#86685=CARTESIAN_POINT('Ctrl Pts',(-67.9285110571741,17.2900349103981,12.));
#86686=CARTESIAN_POINT('Ctrl Pts',(-67.9482246901667,17.2897246158941,0.));
#86687=CARTESIAN_POINT('Ctrl Pts',(-67.9482246901667,17.2897246158941,12.));
#86688=CARTESIAN_POINT('Ctrl Pts',(-67.9679918502579,17.2893923013894,0.));
#86689=CARTESIAN_POINT('Ctrl Pts',(-67.9679918502579,17.2893923013894,12.));
#86690=CARTESIAN_POINT('Ctrl Pts',(-67.987812304921,17.2890378644866,0.));
#86691=CARTESIAN_POINT('Ctrl Pts',(-67.987812304921,17.2890378644866,12.));
#86692=CARTESIAN_POINT('Ctrl Pts',(-68.007685808115,17.2886611977401,0.));
#86693=CARTESIAN_POINT('Ctrl Pts',(-68.007685808115,17.2886611977401,12.));
#86694=CARTESIAN_POINT('Ctrl Pts',(-68.0276121227356,17.2882621974721,0.));
#86695=CARTESIAN_POINT('Ctrl Pts',(-68.0276121227356,17.2882621974721,12.));
#86696=CARTESIAN_POINT('Ctrl Pts',(-68.0475910442424,17.2878407730961,0.));
#86697=CARTESIAN_POINT('Ctrl Pts',(-68.0475910442424,17.2878407730961,12.));
#86698=CARTESIAN_POINT('Ctrl Pts',(-68.0676223930412,17.2873968440839,0.));
#86699=CARTESIAN_POINT('Ctrl Pts',(-68.0676223930412,17.2873968440839,12.));
#86700=CARTESIAN_POINT('Ctrl Pts',(-68.0877060033205,17.2869303355432,0.));
#86701=CARTESIAN_POINT('Ctrl Pts',(-68.0877060033205,17.2869303355432,12.));
#86702=CARTESIAN_POINT('Ctrl Pts',(-68.1078417137877,17.2864411745459,0.));
#86703=CARTESIAN_POINT('Ctrl Pts',(-68.1078417137877,17.2864411745459,12.));
#86704=CARTESIAN_POINT('Ctrl Pts',(-68.1280293561511,17.2859292855705,0.));
#86705=CARTESIAN_POINT('Ctrl Pts',(-68.1280293561511,17.2859292855705,12.));
#86706=CARTESIAN_POINT('Ctrl Pts',(-68.1482687493226,17.2853945882072,0.));
#86707=CARTESIAN_POINT('Ctrl Pts',(-68.1482687493226,17.2853945882072,12.));
#86708=CARTESIAN_POINT('Ctrl Pts',(-68.1685597054231,17.2848369995293,0.));
#86709=CARTESIAN_POINT('Ctrl Pts',(-68.1685597054231,17.2848369995293,12.));
#86710=CARTESIAN_POINT('Ctrl Pts',(-68.1889020335427,17.2842564355799,0.));
#86711=CARTESIAN_POINT('Ctrl Pts',(-68.1889020335427,17.2842564355799,12.));
#86712=CARTESIAN_POINT('Ctrl Pts',(-68.2092955440567,17.2836528130819,0.));
#86713=CARTESIAN_POINT('Ctrl Pts',(-68.2092955440567,17.2836528130819,12.));
#86714=CARTESIAN_POINT('Ctrl Pts',(-68.2297400535294,17.2830260513868,0.));
#86715=CARTESIAN_POINT('Ctrl Pts',(-68.2297400535294,17.2830260513868,12.));
#86716=CARTESIAN_POINT('Ctrl Pts',(-68.2502353845071,17.2823760723874,0.));
#86717=CARTESIAN_POINT('Ctrl Pts',(-68.2502353845071,17.2823760723874,12.));
#86718=CARTESIAN_POINT('Ctrl Pts',(-68.2707813631731,17.2817027995831,0.));
#86719=CARTESIAN_POINT('Ctrl Pts',(-68.2707813631731,17.2817027995831,12.));
#86720=CARTESIAN_POINT('Ctrl Pts',(-68.2913778177261,17.2810061574353,0.));
#86721=CARTESIAN_POINT('Ctrl Pts',(-68.2913778177261,17.2810061574353,12.));
#86722=CARTESIAN_POINT('Ctrl Pts',(-68.3120245763914,17.2802860705815,0.));
#86723=CARTESIAN_POINT('Ctrl Pts',(-68.3120245763914,17.2802860705815,12.));
#86724=CARTESIAN_POINT('Ctrl Pts',(-68.3327214657575,17.2795424631799,0.));
#86725=CARTESIAN_POINT('Ctrl Pts',(-68.3327214657575,17.2795424631799,12.));
#86726=CARTESIAN_POINT('Ctrl Pts',(-68.3534683116514,17.2787752592484,0.));
#86727=CARTESIAN_POINT('Ctrl Pts',(-68.3534683116514,17.2787752592484,12.));
#86728=CARTESIAN_POINT('Ctrl Pts',(-68.3742649398964,17.2779843829608,0.));
#86729=CARTESIAN_POINT('Ctrl Pts',(-68.3742649398964,17.2779843829608,12.));
#86730=CARTESIAN_POINT('Ctrl Pts',(-68.3951111770487,17.2771697589385,0.));
#86731=CARTESIAN_POINT('Ctrl Pts',(-68.3951111770487,17.2771697589385,12.));
#86732=CARTESIAN_POINT('Ctrl Pts',(-68.4160068512753,17.2763313126018,0.));
#86733=CARTESIAN_POINT('Ctrl Pts',(-68.4160068512753,17.2763313126018,12.));
#86734=CARTESIAN_POINT('Ctrl Pts',(-68.436951792677,17.2754689702992,0.));
#86735=CARTESIAN_POINT('Ctrl Pts',(-68.436951792677,17.2754689702992,12.));
#86736=CARTESIAN_POINT('Ctrl Pts',(-68.4579458328185,17.2745826591119,0.));
#86737=CARTESIAN_POINT('Ctrl Pts',(-68.4579458328185,17.2745826591119,12.));
#86738=CARTESIAN_POINT('Ctrl Pts',(-68.4789888044351,17.2736723067365,0.));
#86739=CARTESIAN_POINT('Ctrl Pts',(-68.4789888044351,17.2736723067365,12.));
#86740=CARTESIAN_POINT('Ctrl Pts',(-68.5000805410911,17.2727378413489,0.));
#86741=CARTESIAN_POINT('Ctrl Pts',(-68.5000805410911,17.2727378413489,12.));
#86742=CARTESIAN_POINT('Ctrl Pts',(-68.521220876786,17.2717791914544,0.));
#86743=CARTESIAN_POINT('Ctrl Pts',(-68.521220876786,17.2717791914544,12.));
#86744=CARTESIAN_POINT('Ctrl Pts',(-68.5424096459772,17.2707962858919,0.));
#86745=CARTESIAN_POINT('Ctrl Pts',(-68.5424096459772,17.2707962858919,12.));
#86746=CARTESIAN_POINT('Ctrl Pts',(-68.5636466837517,17.269789053896,0.));
#86747=CARTESIAN_POINT('Ctrl Pts',(-68.5636466837517,17.269789053896,12.));
#86748=CARTESIAN_POINT('Ctrl Pts',(-68.5849318259449,17.2687574251429,0.));
#86749=CARTESIAN_POINT('Ctrl Pts',(-68.5849318259449,17.2687574251429,12.));
#86750=CARTESIAN_POINT('Ctrl Pts',(-68.6062649092764,17.2677013298057,0.));
#86751=CARTESIAN_POINT('Ctrl Pts',(-68.6062649092764,17.2677013298057,12.));
#86752=CARTESIAN_POINT('Ctrl Pts',(-68.6276457714729,17.2666206986084,0.));
#86753=CARTESIAN_POINT('Ctrl Pts',(-68.6276457714729,17.2666206986084,12.));
#86754=CARTESIAN_POINT('Ctrl Pts',(-68.6490742512057,17.2655154627928,0.));
#86755=CARTESIAN_POINT('Ctrl Pts',(-68.6490742512057,17.2655154627928,12.));
#86756=CARTESIAN_POINT('Ctrl Pts',(-68.6705501880249,17.2643855540892,0.));
#86757=CARTESIAN_POINT('Ctrl Pts',(-68.6705501880249,17.2643855540892,12.));
#86758=CARTESIAN_POINT('Ctrl Pts',(-68.6920734222938,17.2632309046892,0.));
#86759=CARTESIAN_POINT('Ctrl Pts',(-68.6920734222938,17.2632309046892,12.));
#86760=CARTESIAN_POINT('Ctrl Pts',(-68.7136437951097,17.2620514472182,0.));
#86761=CARTESIAN_POINT('Ctrl Pts',(-68.7136437951097,17.2620514472182,12.));
#86762=CARTESIAN_POINT('Ctrl Pts',(-68.7352611482547,17.2608471147185,0.));
#86763=CARTESIAN_POINT('Ctrl Pts',(-68.7352611482547,17.2608471147185,12.));
#86764=CARTESIAN_POINT('Ctrl Pts',(-68.7569253242333,17.2596178406551,0.));
#86765=CARTESIAN_POINT('Ctrl Pts',(-68.7569253242333,17.2596178406551,12.));
#86766=CARTESIAN_POINT('Ctrl Pts',(-68.7786361662882,17.2583635589198,0.));
#86767=CARTESIAN_POINT('Ctrl Pts',(-68.7786361662882,17.2583635589198,12.));
#86768=CARTESIAN_POINT('Ctrl Pts',(-68.8003935184184,17.2570842038384,0.));
#86769=CARTESIAN_POINT('Ctrl Pts',(-68.8003935184184,17.2570842038384,12.));
#86770=CARTESIAN_POINT('Ctrl Pts',(-68.8221972253941,17.2557797101813,0.));
#86771=CARTESIAN_POINT('Ctrl Pts',(-68.8221972253941,17.2557797101813,12.));
#86772=CARTESIAN_POINT('Ctrl Pts',(-68.844047132755,17.2544500131625,0.));
#86773=CARTESIAN_POINT('Ctrl Pts',(-68.844047132755,17.2544500131625,12.));
#86774=CARTESIAN_POINT('Ctrl Pts',(-68.8659430867972,17.2530950484258,0.));
#86775=CARTESIAN_POINT('Ctrl Pts',(-68.8659430867972,17.2530950484258,12.));
#86776=CARTESIAN_POINT('Ctrl Pts',(-68.8878849345557,17.2517147520376,0.));
#86777=CARTESIAN_POINT('Ctrl Pts',(-68.8878849345557,17.2517147520376,12.));
#86778=CARTESIAN_POINT('Ctrl Pts',(-68.909872523787,17.2503090604792,0.));
#86779=CARTESIAN_POINT('Ctrl Pts',(-68.909872523787,17.2503090604792,12.));
#86780=CARTESIAN_POINT('Ctrl Pts',(-68.9319057029409,17.248877910643,0.));
#86781=CARTESIAN_POINT('Ctrl Pts',(-68.9319057029409,17.248877910643,12.));
#86782=CARTESIAN_POINT('Ctrl Pts',(-68.9539843211619,17.2474212398275,0.));
#86783=CARTESIAN_POINT('Ctrl Pts',(-68.9539843211619,17.2474212398275,12.));
#86784=CARTESIAN_POINT('Ctrl Pts',(-68.9761082282922,17.2459389857327,0.));
#86785=CARTESIAN_POINT('Ctrl Pts',(-68.9761082282922,17.2459389857327,12.));
#86786=CARTESIAN_POINT('Ctrl Pts',(-68.9982772748694,17.2444310864585,0.));
#86787=CARTESIAN_POINT('Ctrl Pts',(-68.9982772748694,17.2444310864585,12.));
#86788=CARTESIAN_POINT('Ctrl Pts',(-69.0204913121225,17.2428974805044,0.));
#86789=CARTESIAN_POINT('Ctrl Pts',(-69.0204913121225,17.2428974805044,12.));
#86790=CARTESIAN_POINT('Ctrl Pts',(-69.0427501919636,17.2413381067724,0.));
#86791=CARTESIAN_POINT('Ctrl Pts',(-69.0427501919636,17.2413381067724,12.));
#86792=CARTESIAN_POINT('Ctrl Pts',(-69.065053766986,17.2397529045589,0.));
#86793=CARTESIAN_POINT('Ctrl Pts',(-69.065053766986,17.2397529045589,12.));
#86794=CARTESIAN_POINT('Ctrl Pts',(-69.0874018904598,17.2381418135491,0.));
#86795=CARTESIAN_POINT('Ctrl Pts',(-69.0874018904598,17.2381418135491,12.));
#86796=CARTESIAN_POINT('Ctrl Pts',(-69.1097944163245,17.2365047738126,0.));
#86797=CARTESIAN_POINT('Ctrl Pts',(-69.1097944163245,17.2365047738126,12.));
#86798=CARTESIAN_POINT('Ctrl Pts',(-69.1322311991752,17.2348417258015,0.));
#86799=CARTESIAN_POINT('Ctrl Pts',(-69.1322311991752,17.2348417258015,12.));
#86800=CARTESIAN_POINT('Ctrl Pts',(-69.1547120942527,17.2331526103506,0.));
#86801=CARTESIAN_POINT('Ctrl Pts',(-69.1547120942527,17.2331526103506,12.));
#86802=CARTESIAN_POINT('Ctrl Pts',(-69.1772369574447,17.2314373686701,0.));
#86803=CARTESIAN_POINT('Ctrl Pts',(-69.1772369574447,17.2314373686701,12.));
#86804=CARTESIAN_POINT('Ctrl Pts',(-69.1998056452828,17.2296959423407,0.));
#86805=CARTESIAN_POINT('Ctrl Pts',(-69.1998056452828,17.2296959423407,12.));
#86806=CARTESIAN_POINT('Ctrl Pts',(-69.222418014938,17.227928273312,0.));
#86807=CARTESIAN_POINT('Ctrl Pts',(-69.222418014938,17.227928273312,12.));
#86808=CARTESIAN_POINT('Ctrl Pts',(-69.2450739242109,17.226134303902,0.));
#86809=CARTESIAN_POINT('Ctrl Pts',(-69.2450739242109,17.226134303902,12.));
#86810=CARTESIAN_POINT('Ctrl Pts',(-69.2677732315224,17.224313976797,0.));
#86811=CARTESIAN_POINT('Ctrl Pts',(-69.2677732315224,17.224313976797,12.));
#86812=CARTESIAN_POINT('Ctrl Pts',(-69.2905157959166,17.2224672350439,0.));
#86813=CARTESIAN_POINT('Ctrl Pts',(-69.2905157959166,17.2224672350439,12.));
#86814=CARTESIAN_POINT('Ctrl Pts',(-69.3133014770554,17.2205940220459,0.));
#86815=CARTESIAN_POINT('Ctrl Pts',(-69.3133014770554,17.2205940220459,12.));
#86816=CARTESIAN_POINT('Ctrl Pts',(-69.3361301352141,17.2186942815602,0.));
#86817=CARTESIAN_POINT('Ctrl Pts',(-69.3361301352141,17.2186942815602,12.));
#86818=CARTESIAN_POINT('Ctrl Pts',(-69.3590016312692,17.2167679576984,0.));
#86819=CARTESIAN_POINT('Ctrl Pts',(-69.3590016312692,17.2167679576984,12.));
#86820=CARTESIAN_POINT('Ctrl Pts',(-69.3819158266915,17.2148149949252,0.));
#86821=CARTESIAN_POINT('Ctrl Pts',(-69.3819158266915,17.2148149949252,12.));
#86822=CARTESIAN_POINT('Ctrl Pts',(-69.404872583548,17.2128353380502,0.));
#86823=CARTESIAN_POINT('Ctrl Pts',(-69.404872583548,17.2128353380502,12.));
#86824=CARTESIAN_POINT('Ctrl Pts',(-69.4278717644973,17.2108289322254,0.));
#86825=CARTESIAN_POINT('Ctrl Pts',(-69.4278717644973,17.2108289322254,12.));
#86826=CARTESIAN_POINT('Ctrl Pts',(-69.4509132327849,17.2087957229424,0.));
#86827=CARTESIAN_POINT('Ctrl Pts',(-69.4509132327849,17.2087957229424,12.));
#86828=CARTESIAN_POINT('Ctrl Pts',(-69.4739968522313,17.2067356560337,0.));
#86829=CARTESIAN_POINT('Ctrl Pts',(-69.4739968522313,17.2067356560337,12.));
#86830=CARTESIAN_POINT('Ctrl Pts',(-69.4971224872269,17.2046486776708,0.));
#86831=CARTESIAN_POINT('Ctrl Pts',(-69.4971224872269,17.2046486776708,12.));
#86832=CARTESIAN_POINT('Ctrl Pts',(-69.5202900027367,17.2025347343577,0.));
#86833=CARTESIAN_POINT('Ctrl Pts',(-69.5202900027367,17.2025347343577,12.));
#86834=CARTESIAN_POINT('Ctrl Pts',(-69.5434992642944,17.2003937729268,0.));
#86835=CARTESIAN_POINT('Ctrl Pts',(-69.5434992642944,17.2003937729268,12.));
#86836=CARTESIAN_POINT('Ctrl Pts',(-69.5667501379969,17.1982257405377,0.));
#86837=CARTESIAN_POINT('Ctrl Pts',(-69.5667501379969,17.1982257405377,12.));
#86838=CARTESIAN_POINT('Ctrl Pts',(-69.5900424904921,17.1960305846781,0.));
#86839=CARTESIAN_POINT('Ctrl Pts',(-69.5900424904921,17.1960305846781,12.));
#86840=CARTESIAN_POINT('Ctrl Pts',(-69.6133761889749,17.1938082531612,0.));
#86841=CARTESIAN_POINT('Ctrl Pts',(-69.6133761889749,17.1938082531612,12.));
#86842=CARTESIAN_POINT('Ctrl Pts',(-69.6367511011898,17.1915586941192,0.));
#86843=CARTESIAN_POINT('Ctrl Pts',(-69.6367511011898,17.1915586941192,12.));
#86844=CARTESIAN_POINT('Ctrl Pts',(-69.6601670954269,17.1892818560003,0.));
#86845=CARTESIAN_POINT('Ctrl Pts',(-69.6601670954269,17.1892818560003,12.));
#86846=CARTESIAN_POINT('Ctrl Pts',(-69.6836240405164,17.1869776875666,0.));
#86847=CARTESIAN_POINT('Ctrl Pts',(-69.6836240405164,17.1869776875666,12.));
#86848=CARTESIAN_POINT('Ctrl Pts',(-69.7071218058178,17.1846461378973,0.));
#86849=CARTESIAN_POINT('Ctrl Pts',(-69.7071218058178,17.1846461378973,12.));
#86850=CARTESIAN_POINT('Ctrl Pts',(-69.7306602612155,17.1822871563842,0.));
#86851=CARTESIAN_POINT('Ctrl Pts',(-69.7306602612155,17.1822871563842,12.));
#86852=CARTESIAN_POINT('Ctrl Pts',(-69.7542392771234,17.179900692726,0.));
#86853=CARTESIAN_POINT('Ctrl Pts',(-69.7542392771234,17.179900692726,12.));
#86854=CARTESIAN_POINT('Ctrl Pts',(-69.777858724479,17.1774866969257,0.));
#86855=CARTESIAN_POINT('Ctrl Pts',(-69.777858724479,17.1774866969257,12.));
#86856=CARTESIAN_POINT('Ctrl Pts',(-69.8015184747398,17.1750451192886,0.));
#86857=CARTESIAN_POINT('Ctrl Pts',(-69.8015184747398,17.1750451192886,12.));
#86858=CARTESIAN_POINT('Ctrl Pts',(-69.8252183998702,17.1725759104252,0.));
#86859=CARTESIAN_POINT('Ctrl Pts',(-69.8252183998702,17.1725759104252,12.));
#86860=CARTESIAN_POINT('Ctrl Pts',(-69.8489583723407,17.1700790212474,0.));
#86861=CARTESIAN_POINT('Ctrl Pts',(-69.8489583723407,17.1700790212474,12.));
#86862=CARTESIAN_POINT('Ctrl Pts',(-69.8727382651285,17.167554402962,0.));
#86863=CARTESIAN_POINT('Ctrl Pts',(-69.8727382651285,17.167554402962,12.));
#86864=CARTESIAN_POINT('Ctrl Pts',(-69.8965579517147,17.1650020070686,0.));
#86865=CARTESIAN_POINT('Ctrl Pts',(-69.8965579517147,17.1650020070686,12.));
#86866=CARTESIAN_POINT('Ctrl Pts',(-69.9204173060781,17.1624217853578,0.));
#86867=CARTESIAN_POINT('Ctrl Pts',(-69.9204173060781,17.1624217853578,12.));
#86868=CARTESIAN_POINT('Ctrl Pts',(-69.9443162026865,17.1598136899145,0.));
#86869=CARTESIAN_POINT('Ctrl Pts',(-69.9443162026865,17.1598136899145,12.));
#86870=CARTESIAN_POINT('Ctrl Pts',(-69.9682545164939,17.157177673114,0.));
#86871=CARTESIAN_POINT('Ctrl Pts',(-69.9682545164939,17.157177673114,12.));
#86872=CARTESIAN_POINT('Ctrl Pts',(-69.9922321229424,17.1545136876161,0.));
#86873=CARTESIAN_POINT('Ctrl Pts',(-69.9922321229424,17.1545136876161,12.));
#86874=CARTESIAN_POINT('Ctrl Pts',(-70.0162488979584,17.1518216863623,0.));
#86875=CARTESIAN_POINT('Ctrl Pts',(-70.0162488979584,17.1518216863623,12.));
#86876=CARTESIAN_POINT('Ctrl Pts',(-70.0403047179483,17.1491016225749,0.));
#86877=CARTESIAN_POINT('Ctrl Pts',(-70.0403047179483,17.1491016225749,12.));
#86878=CARTESIAN_POINT('Ctrl Pts',(-70.0643994597873,17.1463534497595,0.));
#86879=CARTESIAN_POINT('Ctrl Pts',(-70.0643994597873,17.1463534497595,12.));
#86880=CARTESIAN_POINT('Ctrl Pts',(-70.0885330008179,17.1435771217018,0.));
#86881=CARTESIAN_POINT('Ctrl Pts',(-70.0885330008179,17.1435771217018,12.));
#86882=CARTESIAN_POINT('Ctrl Pts',(-70.1127052188522,17.1407725924617,0.));
#86883=CARTESIAN_POINT('Ctrl Pts',(-70.1127052188522,17.1407725924617,12.));
#86884=CARTESIAN_POINT('Ctrl Pts',(-70.1369159921687,17.1379398163709,0.));
#86885=CARTESIAN_POINT('Ctrl Pts',(-70.1369159921687,17.1379398163709,12.));
#86886=CARTESIAN_POINT('Ctrl Pts',(-70.1611651995082,17.1350787480312,0.));
#86887=CARTESIAN_POINT('Ctrl Pts',(-70.1611651995082,17.1350787480312,12.));
#86888=CARTESIAN_POINT('Ctrl Pts',(-70.1854527200631,17.1321893423182,0.));
#86889=CARTESIAN_POINT('Ctrl Pts',(-70.1854527200631,17.1321893423182,12.));
#86890=CARTESIAN_POINT('Ctrl Pts',(-70.2097784334747,17.1292715543778,0.));
#86891=CARTESIAN_POINT('Ctrl Pts',(-70.2097784334747,17.1292715543778,12.));
#86892=CARTESIAN_POINT('Ctrl Pts',(-70.2341422198363,17.1263253396202,0.));
#86893=CARTESIAN_POINT('Ctrl Pts',(-70.2341422198363,17.1263253396202,12.));
#86894=CARTESIAN_POINT('Ctrl Pts',(-70.2585439596901,17.1233506537177,0.));
#86895=CARTESIAN_POINT('Ctrl Pts',(-70.2585439596901,17.1233506537177,12.));
#86896=CARTESIAN_POINT('Ctrl Pts',(-70.2829835340238,17.1203474526031,0.));
#86897=CARTESIAN_POINT('Ctrl Pts',(-70.2829835340238,17.1203474526031,12.));
#86898=CARTESIAN_POINT('Ctrl Pts',(-70.3074608242608,17.1173156924733,0.));
#86899=CARTESIAN_POINT('Ctrl Pts',(-70.3074608242608,17.1173156924733,12.));
#86900=CARTESIAN_POINT('Ctrl Pts',(-70.3319757122568,17.1142553297867,0.));
#86901=CARTESIAN_POINT('Ctrl Pts',(-70.3319757122568,17.1142553297867,12.));
#86902=CARTESIAN_POINT('Ctrl Pts',(-70.3565280803022,17.1111663212568,0.));
#86903=CARTESIAN_POINT('Ctrl Pts',(-70.3565280803022,17.1111663212568,12.));
#86904=CARTESIAN_POINT('Ctrl Pts',(-70.3811178111201,17.1080486238499,0.));
#86905=CARTESIAN_POINT('Ctrl Pts',(-70.3811178111201,17.1080486238499,12.));
#86906=CARTESIAN_POINT('Ctrl Pts',(-70.4057447878624,17.1049021947834,0.));
#86907=CARTESIAN_POINT('Ctrl Pts',(-70.4057447878624,17.1049021947834,12.));
#86908=CARTESIAN_POINT('Ctrl Pts',(-70.430408894101,17.1017269915292,0.));
#86909=CARTESIAN_POINT('Ctrl Pts',(-70.430408894101,17.1017269915292,12.));
#86910=CARTESIAN_POINT('Ctrl Pts',(-70.4551100138238,17.0985229718125,0.));
#86911=CARTESIAN_POINT('Ctrl Pts',(-70.4551100138238,17.0985229718125,12.));
#86912=CARTESIAN_POINT('Ctrl Pts',(-70.4798480314381,17.0952900936048,0.));
#86913=CARTESIAN_POINT('Ctrl Pts',(-70.4798480314381,17.0952900936048,12.));
#86914=CARTESIAN_POINT('Ctrl Pts',(-70.5046228317677,17.0920283151219,0.));
#86915=CARTESIAN_POINT('Ctrl Pts',(-70.5046228317677,17.0920283151219,12.));
#86916=CARTESIAN_POINT('Ctrl Pts',(-70.5294343000513,17.088737594822,0.));
#86917=CARTESIAN_POINT('Ctrl Pts',(-70.5294343000513,17.088737594822,12.));
#86918=CARTESIAN_POINT('Ctrl Pts',(-70.5542823219331,17.0854178914087,0.));
#86919=CARTESIAN_POINT('Ctrl Pts',(-70.5542823219331,17.0854178914087,12.));
#86920=CARTESIAN_POINT('Ctrl Pts',(-70.5791667834582,17.082069163831,0.));
#86921=CARTESIAN_POINT('Ctrl Pts',(-70.5791667834582,17.082069163831,12.));
#86922=CARTESIAN_POINT('Ctrl Pts',(-70.6040875710749,17.0786913712764,0.));
#86923=CARTESIAN_POINT('Ctrl Pts',(-70.6040875710749,17.0786913712764,12.));
#86924=CARTESIAN_POINT('Ctrl Pts',(-70.6290445716337,17.0752844731678,0.));
#86925=CARTESIAN_POINT('Ctrl Pts',(-70.6290445716337,17.0752844731678,12.));
#86926=CARTESIAN_POINT('Ctrl Pts',(-70.6540376723841,17.0718484291624,0.));
#86927=CARTESIAN_POINT('Ctrl Pts',(-70.6540376723841,17.0718484291624,12.));
#86928=CARTESIAN_POINT('Ctrl Pts',(-70.6790667609679,17.0683831991532,0.));
#86929=CARTESIAN_POINT('Ctrl Pts',(-70.6790667609679,17.0683831991532,12.));
#86930=CARTESIAN_POINT('Ctrl Pts',(-70.7041317254125,17.0648887432714,0.));
#86931=CARTESIAN_POINT('Ctrl Pts',(-70.7041317254125,17.0648887432714,12.));
#86932=CARTESIAN_POINT('Ctrl Pts',(-70.7292324541341,17.0613650218787,0.));
#86933=CARTESIAN_POINT('Ctrl Pts',(-70.7292324541341,17.0613650218787,12.));
#86934=CARTESIAN_POINT('Ctrl Pts',(-70.7543688359374,17.0578119955649,0.));
#86935=CARTESIAN_POINT('Ctrl Pts',(-70.7543688359374,17.0578119955649,12.));
#86936=CARTESIAN_POINT('Ctrl Pts',(-70.7795407600127,17.0542296251462,0.));
#86937=CARTESIAN_POINT('Ctrl Pts',(-70.7795407600127,17.0542296251462,12.));
#86938=CARTESIAN_POINT('Ctrl Pts',(-70.8047481159306,17.0506178716664,0.));
#86939=CARTESIAN_POINT('Ctrl Pts',(-70.8047481159306,17.0506178716664,12.));
#86940=CARTESIAN_POINT('Ctrl Pts',(-70.8299907936346,17.0469766964005,0.));
#86941=CARTESIAN_POINT('Ctrl Pts',(-70.8299907936346,17.0469766964005,12.));
#86942=CARTESIAN_POINT('Ctrl Pts',(-70.8552686834435,17.0433060608479,0.));
#86943=CARTESIAN_POINT('Ctrl Pts',(-70.8552686834435,17.0433060608479,12.));
#86944=CARTESIAN_POINT('Ctrl Pts',(-70.8805816760507,17.039605926728,0.));
#86945=CARTESIAN_POINT('Ctrl Pts',(-70.8805816760507,17.039605926728,12.));
#86946=CARTESIAN_POINT('Ctrl Pts',(-70.9059296625214,17.0358762559786,0.));
#86947=CARTESIAN_POINT('Ctrl Pts',(-70.9059296625214,17.0358762559786,12.));
#86948=CARTESIAN_POINT('Ctrl Pts',(-70.9313125342872,17.0321170107562,0.));
#86949=CARTESIAN_POINT('Ctrl Pts',(-70.9313125342872,17.0321170107562,12.));
#86950=CARTESIAN_POINT('Ctrl Pts',(-70.9567301831355,17.028328153439,0.));
#86951=CARTESIAN_POINT('Ctrl Pts',(-70.9567301831355,17.028328153439,12.));
#86952=CARTESIAN_POINT('Ctrl Pts',(-70.9821825012134,17.0245096466228,0.));
#86953=CARTESIAN_POINT('Ctrl Pts',(-70.9821825012134,17.0245096466228,12.));
#86954=CARTESIAN_POINT('Ctrl Pts',(-71.0076693810302,17.0206614531166,0.));
#86955=CARTESIAN_POINT('Ctrl Pts',(-71.0076693810302,17.0206614531166,12.));
#86956=CARTESIAN_POINT('Ctrl Pts',(-71.0331907154575,17.016783535942,0.));
#86957=CARTESIAN_POINT('Ctrl Pts',(-71.0331907154575,17.016783535942,12.));
#86958=CARTESIAN_POINT('Ctrl Pts',(-71.0587463977266,17.0128758583335,0.));
#86959=CARTESIAN_POINT('Ctrl Pts',(-71.0587463977266,17.0128758583335,12.));
#86960=CARTESIAN_POINT('Ctrl Pts',(-71.0843363214216,17.0089383837437,0.));
#86961=CARTESIAN_POINT('Ctrl Pts',(-71.0843363214216,17.0089383837437,12.));
#86962=CARTESIAN_POINT('Ctrl Pts',(-71.1099603804779,17.0049710758393,0.));
#86963=CARTESIAN_POINT('Ctrl Pts',(-71.1099603804779,17.0049710758393,12.));
#86964=CARTESIAN_POINT('Ctrl Pts',(-71.1356184691799,17.0009738984935,0.));
#86965=CARTESIAN_POINT('Ctrl Pts',(-71.1356184691799,17.0009738984935,12.));
#86966=CARTESIAN_POINT('Ctrl Pts',(-71.1613104821565,16.9969468157824,0.));
#86967=CARTESIAN_POINT('Ctrl Pts',(-71.1613104821565,16.9969468157824,12.));
#86968=CARTESIAN_POINT('Ctrl Pts',(-71.1870363143742,16.9928897919829,0.));
#86969=CARTESIAN_POINT('Ctrl Pts',(-71.1870363143742,16.9928897919829,12.));
#86970=CARTESIAN_POINT('Ctrl Pts',(-71.2127958611248,16.9888027915743,0.));
#86971=CARTESIAN_POINT('Ctrl Pts',(-71.2127958611248,16.9888027915743,12.));
#86972=CARTESIAN_POINT('Ctrl Pts',(-71.2385890180233,16.9846857792385,0.));
#86973=CARTESIAN_POINT('Ctrl Pts',(-71.2385890180233,16.9846857792385,12.));
#86974=CARTESIAN_POINT('Ctrl Pts',(-71.2644156810209,16.9805387198573,0.));
#86975=CARTESIAN_POINT('Ctrl Pts',(-71.2644156810209,16.9805387198573,12.));
#86976=CARTESIAN_POINT('Ctrl Pts',(-71.2902757464127,16.9763615785138,0.));
#86977=CARTESIAN_POINT('Ctrl Pts',(-71.2902757464127,16.9763615785138,12.));
#86978=CARTESIAN_POINT('Ctrl Pts',(-71.3161691108425,16.9721543204951,0.));
#86979=CARTESIAN_POINT('Ctrl Pts',(-71.3161691108425,16.9721543204951,12.));
#86980=CARTESIAN_POINT('Ctrl Pts',(-71.3420956713072,16.9679169112993,0.));
#86981=CARTESIAN_POINT('Ctrl Pts',(-71.3420956713072,16.9679169112993,12.));
#86982=CARTESIAN_POINT('Ctrl Pts',(-71.3680553251547,16.9636493166395,0.));
#86983=CARTESIAN_POINT('Ctrl Pts',(-71.3680553251547,16.9636493166395,12.));
#86984=CARTESIAN_POINT('Ctrl Pts',(-71.3940479700662,16.9593515024274,0.));
#86985=CARTESIAN_POINT('Ctrl Pts',(-71.3940479700662,16.9593515024274,12.));
#86986=CARTESIAN_POINT('Ctrl Pts',(-71.4200735040374,16.9550234347619,0.));
#86987=CARTESIAN_POINT('Ctrl Pts',(-71.4200735040374,16.9550234347619,12.));
#86988=CARTESIAN_POINT('Ctrl Pts',(-71.4461318253561,16.9506650799189,0.));
#86989=CARTESIAN_POINT('Ctrl Pts',(-71.4461318253561,16.9506650799189,12.));
#86990=CARTESIAN_POINT('Ctrl Pts',(-71.4722228325805,16.9462764043445,0.));
#86991=CARTESIAN_POINT('Ctrl Pts',(-71.4722228325805,16.9462764043445,12.));
#86992=CARTESIAN_POINT('Ctrl Pts',(-71.4983464245069,16.9418573746492,0.));
#86993=CARTESIAN_POINT('Ctrl Pts',(-71.4983464245069,16.9418573746492,12.));
#86994=CARTESIAN_POINT('Ctrl Pts',(-71.5245025002154,16.9374079576204,0.));
#86995=CARTESIAN_POINT('Ctrl Pts',(-71.5245025002154,16.9374079576204,12.));
#86996=CARTESIAN_POINT('Ctrl Pts',(-71.5506909591139,16.9329281202379,0.));
#86997=CARTESIAN_POINT('Ctrl Pts',(-71.5506909591139,16.9329281202379,12.));
#86998=CARTESIAN_POINT('Ctrl Pts',(-71.5769117009845,16.9284178296934,0.));
#86999=CARTESIAN_POINT('Ctrl Pts',(-71.5769117009845,16.9284178296934,12.));
#87000=CARTESIAN_POINT('Ctrl Pts',(-71.6031646260169,16.923877053407,0.));
#87001=CARTESIAN_POINT('Ctrl Pts',(-71.6031646260169,16.923877053407,12.));
#87002=CARTESIAN_POINT('Ctrl Pts',(-71.6294496348644,16.9193057590605,0.));
#87003=CARTESIAN_POINT('Ctrl Pts',(-71.6294496348644,16.9193057590605,12.));
#87004=CARTESIAN_POINT('Ctrl Pts',(-71.6557666285908,16.9147039145716,0.));
#87005=CARTESIAN_POINT('Ctrl Pts',(-71.6557666285908,16.9147039145716,12.));
#87006=CARTESIAN_POINT('Ctrl Pts',(-71.6821155085605,16.9100714880367,0.));
#87007=CARTESIAN_POINT('Ctrl Pts',(-71.6821155085605,16.9100714880367,12.));
#87008=CARTESIAN_POINT('Ctrl Pts',(-71.7084961763355,16.9054084476847,0.));
#87009=CARTESIAN_POINT('Ctrl Pts',(-71.7084961763355,16.9054084476847,12.));
#87010=CARTESIAN_POINT('Ctrl Pts',(-71.7349085335796,16.9007147618344,0.));
#87011=CARTESIAN_POINT('Ctrl Pts',(-71.7349085335796,16.9007147618344,12.));
#87012=CARTESIAN_POINT('Ctrl Pts',(-71.7613524819239,16.8959903988411,0.));
#87013=CARTESIAN_POINT('Ctrl Pts',(-71.7613524819239,16.8959903988411,12.));
#87014=CARTESIAN_POINT('Ctrl Pts',(-71.7878279229556,16.8912353270944,0.));
#87015=CARTESIAN_POINT('Ctrl Pts',(-71.7878279229556,16.8912353270944,12.));
#87016=CARTESIAN_POINT('Ctrl Pts',(-71.8143347584977,16.8864495151347,0.));
#87017=CARTESIAN_POINT('Ctrl Pts',(-71.8143347584977,16.8864495151347,12.));
#87018=CARTESIAN_POINT('Ctrl Pts',(-71.8408728908269,16.8816329317473,0.));
#87019=CARTESIAN_POINT('Ctrl Pts',(-71.8408728908269,16.8816329317473,12.));
#87020=CARTESIAN_POINT('Ctrl Pts',(-71.8674422229151,16.8767855460701,0.));
#87021=CARTESIAN_POINT('Ctrl Pts',(-71.8674422229151,16.8767855460701,12.));
#87022=CARTESIAN_POINT('Ctrl Pts',(-71.8940426586521,16.8719073276967,0.));
#87023=CARTESIAN_POINT('Ctrl Pts',(-71.8940426586521,16.8719073276967,12.));
#87024=CARTESIAN_POINT('Ctrl Pts',(-71.920674103086,16.8669982467915,0.));
#87025=CARTESIAN_POINT('Ctrl Pts',(-71.920674103086,16.8669982467915,12.));
#87026=CARTESIAN_POINT('Ctrl Pts',(-71.9473364618889,16.8620582738431,0.));
#87027=CARTESIAN_POINT('Ctrl Pts',(-71.9473364618889,16.8620582738431,12.));
#87028=CARTESIAN_POINT('Ctrl Pts',(-71.9740296408319,16.8570873794264,0.));
#87029=CARTESIAN_POINT('Ctrl Pts',(-71.9740296408319,16.8570873794264,12.));
#87030=CARTESIAN_POINT('Ctrl Pts',(-72.0007535452071,16.8520855339444,0.));
#87031=CARTESIAN_POINT('Ctrl Pts',(-72.0007535452071,16.8520855339444,12.));
#87032=CARTESIAN_POINT('Ctrl Pts',(-72.0275080793742,16.8470527074278,0.));
#87033=CARTESIAN_POINT('Ctrl Pts',(-72.0275080793742,16.8470527074278,12.));
#87034=CARTESIAN_POINT('Ctrl Pts',(-72.0542931459865,16.8419888691984,0.));
#87035=CARTESIAN_POINT('Ctrl Pts',(-72.0542931459865,16.8419888691984,12.));
#87036=CARTESIAN_POINT('Ctrl Pts',(-72.0811086466178,16.8368939881457,0.));
#87037=CARTESIAN_POINT('Ctrl Pts',(-72.0811086466178,16.8368939881457,12.));
#87038=CARTESIAN_POINT('Ctrl Pts',(-72.1079544831568,16.8317680333415,0.));
#87039=CARTESIAN_POINT('Ctrl Pts',(-72.1079544831568,16.8317680333415,12.));
#87040=CARTESIAN_POINT('Ctrl Pts',(-72.1348305590233,16.8266109745802,0.));
#87041=CARTESIAN_POINT('Ctrl Pts',(-72.1348305590233,16.8266109745802,12.));
#87042=CARTESIAN_POINT('Ctrl Pts',(-72.1617367803226,16.8214227828941,0.));
#87043=CARTESIAN_POINT('Ctrl Pts',(-72.1617367803226,16.8214227828941,12.));
#87044=CARTESIAN_POINT('Ctrl Pts',(-72.1886730573389,16.8162034312257,0.));
#87045=CARTESIAN_POINT('Ctrl Pts',(-72.1886730573389,16.8162034312257,12.));
#87046=CARTESIAN_POINT('Ctrl Pts',(-72.2156393048868,16.8109528945876,0.));
#87047=CARTESIAN_POINT('Ctrl Pts',(-72.2156393048868,16.8109528945876,12.));
#87048=CARTESIAN_POINT('Ctrl Pts',(-72.242635439009,16.8056711485798,0.));
#87049=CARTESIAN_POINT('Ctrl Pts',(-72.242635439009,16.8056711485798,12.));
#87050=CARTESIAN_POINT('Ctrl Pts',(-72.2696613743687,16.800358168223,0.));
#87051=CARTESIAN_POINT('Ctrl Pts',(-72.2696613743687,16.800358168223,12.));
#87052=CARTESIAN_POINT('Ctrl Pts',(-72.2967170212331,16.7950139266118,0.));
#87053=CARTESIAN_POINT('Ctrl Pts',(-72.2967170212331,16.7950139266118,12.));
#87054=CARTESIAN_POINT('Ctrl Pts',(-72.323802282931,16.7896383937839,0.));
#87055=CARTESIAN_POINT('Ctrl Pts',(-72.323802282931,16.7896383937839,12.));
#87056=CARTESIAN_POINT('Ctrl Pts',(-72.3509170523038,16.7842315351402,0.));
#87057=CARTESIAN_POINT('Ctrl Pts',(-72.3509170523038,16.7842315351402,12.));
#87058=CARTESIAN_POINT('Ctrl Pts',(-72.3780612168056,16.7787933137551,0.));
#87059=CARTESIAN_POINT('Ctrl Pts',(-72.3780612168056,16.7787933137551,12.));
#87060=CARTESIAN_POINT('Ctrl Pts',(-72.4052346648058,16.7733236932185,0.));
#87061=CARTESIAN_POINT('Ctrl Pts',(-72.4052346648058,16.7733236932185,12.));
#87062=CARTESIAN_POINT('Ctrl Pts',(-72.4324372916884,16.7678226404189,0.));
#87063=CARTESIAN_POINT('Ctrl Pts',(-72.4324372916884,16.7678226404189,12.));
#87064=CARTESIAN_POINT('Ctrl Pts',(-72.4596690055347,16.7622901280741,0.));
#87065=CARTESIAN_POINT('Ctrl Pts',(-72.4596690055347,16.7622901280741,12.));
#87066=CARTESIAN_POINT('Ctrl Pts',(-72.4869297342051,16.7567261380614,0.));
#87067=CARTESIAN_POINT('Ctrl Pts',(-72.4869297342051,16.7567261380614,12.));
#87068=CARTESIAN_POINT('Ctrl Pts',(-72.5142194273203,16.7511306618794,0.));
#87069=CARTESIAN_POINT('Ctrl Pts',(-72.5142194273203,16.7511306618794,12.));
#87070=CARTESIAN_POINT('Ctrl Pts',(-72.5415380515905,16.7455036973724,0.));
#87071=CARTESIAN_POINT('Ctrl Pts',(-72.5415380515905,16.7455036973724,12.));
#87072=CARTESIAN_POINT('Ctrl Pts',(-72.563416080574,16.7409769365953,0.));
#87073=CARTESIAN_POINT('Ctrl Pts',(-72.563416080574,16.7409769365953,12.));
#87074=CARTESIAN_POINT('Ctrl Pts',(-72.5798376087405,16.7375676985272,0.));
#87075=CARTESIAN_POINT('Ctrl Pts',(-72.5798376087405,16.7375676985272,12.));
#87076=CARTESIAN_POINT('Ctrl Pts',(-72.5907910745874,16.7352885767459,0.));
#87077=CARTESIAN_POINT('Ctrl Pts',(-72.5907910745874,16.7352885767459,12.));
#87078=CARTESIAN_POINT('Ctrl Pts',(-72.5962692526112,16.7341474417545,0.));
#87079=CARTESIAN_POINT('Ctrl Pts',(-72.5962692526112,16.7341474417545,12.));
#87080=CARTESIAN_POINT('',(-67.8307641965654,17.2912529479484,0.));
#87081=CARTESIAN_POINT('Ctrl Pts',(-67.8307641965654,17.2912529479484,0.));
#87082=CARTESIAN_POINT('Ctrl Pts',(-67.8346476309018,17.2912149114119,0.));
#87083=CARTESIAN_POINT('Ctrl Pts',(-67.842419897098,17.2911366591348,0.));
#87084=CARTESIAN_POINT('Ctrl Pts',(-67.8540944889687,17.291012743109,0.));
#87085=CARTESIAN_POINT('Ctrl Pts',(-67.8696929978782,17.2908344459695,0.));
#87086=CARTESIAN_POINT('Ctrl Pts',(-67.8892451049608,17.2905897723949,0.));
#87087=CARTESIAN_POINT('Ctrl Pts',(-67.9088511496685,17.2903232740694,0.));
#87088=CARTESIAN_POINT('Ctrl Pts',(-67.9285110571741,17.2900349103981,0.));
#87089=CARTESIAN_POINT('Ctrl Pts',(-67.9482246901667,17.2897246158941,0.));
#87090=CARTESIAN_POINT('Ctrl Pts',(-67.9679918502579,17.2893923013894,0.));
#87091=CARTESIAN_POINT('Ctrl Pts',(-67.987812304921,17.2890378644866,0.));
#87092=CARTESIAN_POINT('Ctrl Pts',(-68.007685808115,17.2886611977401,0.));
#87093=CARTESIAN_POINT('Ctrl Pts',(-68.0276121227356,17.2882621974721,0.));
#87094=CARTESIAN_POINT('Ctrl Pts',(-68.0475910442424,17.2878407730961,0.));
#87095=CARTESIAN_POINT('Ctrl Pts',(-68.0676223930412,17.2873968440839,0.));
#87096=CARTESIAN_POINT('Ctrl Pts',(-68.0877060033205,17.2869303355432,0.));
#87097=CARTESIAN_POINT('Ctrl Pts',(-68.1078417137877,17.2864411745459,0.));
#87098=CARTESIAN_POINT('Ctrl Pts',(-68.1280293561511,17.2859292855705,0.));
#87099=CARTESIAN_POINT('Ctrl Pts',(-68.1482687493226,17.2853945882072,0.));
#87100=CARTESIAN_POINT('Ctrl Pts',(-68.1685597054231,17.2848369995293,0.));
#87101=CARTESIAN_POINT('Ctrl Pts',(-68.1889020335427,17.2842564355799,0.));
#87102=CARTESIAN_POINT('Ctrl Pts',(-68.2092955440567,17.2836528130819,0.));
#87103=CARTESIAN_POINT('Ctrl Pts',(-68.2297400535294,17.2830260513868,0.));
#87104=CARTESIAN_POINT('Ctrl Pts',(-68.2502353845071,17.2823760723874,0.));
#87105=CARTESIAN_POINT('Ctrl Pts',(-68.2707813631731,17.2817027995831,0.));
#87106=CARTESIAN_POINT('Ctrl Pts',(-68.2913778177261,17.2810061574353,0.));
#87107=CARTESIAN_POINT('Ctrl Pts',(-68.3120245763914,17.2802860705815,0.));
#87108=CARTESIAN_POINT('Ctrl Pts',(-68.3327214657575,17.2795424631799,0.));
#87109=CARTESIAN_POINT('Ctrl Pts',(-68.3534683116514,17.2787752592484,0.));
#87110=CARTESIAN_POINT('Ctrl Pts',(-68.3742649398964,17.2779843829608,0.));
#87111=CARTESIAN_POINT('Ctrl Pts',(-68.3951111770487,17.2771697589385,0.));
#87112=CARTESIAN_POINT('Ctrl Pts',(-68.4160068512753,17.2763313126018,0.));
#87113=CARTESIAN_POINT('Ctrl Pts',(-68.436951792677,17.2754689702992,0.));
#87114=CARTESIAN_POINT('Ctrl Pts',(-68.4579458328185,17.2745826591119,0.));
#87115=CARTESIAN_POINT('Ctrl Pts',(-68.4789888044351,17.2736723067365,0.));
#87116=CARTESIAN_POINT('Ctrl Pts',(-68.5000805410911,17.2727378413489,0.));
#87117=CARTESIAN_POINT('Ctrl Pts',(-68.521220876786,17.2717791914544,0.));
#87118=CARTESIAN_POINT('Ctrl Pts',(-68.5424096459772,17.2707962858919,0.));
#87119=CARTESIAN_POINT('Ctrl Pts',(-68.5636466837517,17.269789053896,0.));
#87120=CARTESIAN_POINT('Ctrl Pts',(-68.5849318259449,17.2687574251429,0.));
#87121=CARTESIAN_POINT('Ctrl Pts',(-68.6062649092764,17.2677013298057,0.));
#87122=CARTESIAN_POINT('Ctrl Pts',(-68.6276457714729,17.2666206986084,0.));
#87123=CARTESIAN_POINT('Ctrl Pts',(-68.6490742512057,17.2655154627928,0.));
#87124=CARTESIAN_POINT('Ctrl Pts',(-68.6705501880249,17.2643855540892,0.));
#87125=CARTESIAN_POINT('Ctrl Pts',(-68.6920734222938,17.2632309046892,0.));
#87126=CARTESIAN_POINT('Ctrl Pts',(-68.7136437951097,17.2620514472182,0.));
#87127=CARTESIAN_POINT('Ctrl Pts',(-68.7352611482547,17.2608471147185,0.));
#87128=CARTESIAN_POINT('Ctrl Pts',(-68.7569253242333,17.2596178406551,0.));
#87129=CARTESIAN_POINT('Ctrl Pts',(-68.7786361662882,17.2583635589198,0.));
#87130=CARTESIAN_POINT('Ctrl Pts',(-68.8003935184184,17.2570842038384,0.));
#87131=CARTESIAN_POINT('Ctrl Pts',(-68.8221972253941,17.2557797101813,0.));
#87132=CARTESIAN_POINT('Ctrl Pts',(-68.844047132755,17.2544500131625,0.));
#87133=CARTESIAN_POINT('Ctrl Pts',(-68.8659430867972,17.2530950484258,0.));
#87134=CARTESIAN_POINT('Ctrl Pts',(-68.8878849345557,17.2517147520376,0.));
#87135=CARTESIAN_POINT('Ctrl Pts',(-68.909872523787,17.2503090604792,0.));
#87136=CARTESIAN_POINT('Ctrl Pts',(-68.9319057029409,17.248877910643,0.));
#87137=CARTESIAN_POINT('Ctrl Pts',(-68.9539843211619,17.2474212398275,0.));
#87138=CARTESIAN_POINT('Ctrl Pts',(-68.9761082282922,17.2459389857327,0.));
#87139=CARTESIAN_POINT('Ctrl Pts',(-68.9982772748694,17.2444310864585,0.));
#87140=CARTESIAN_POINT('Ctrl Pts',(-69.0204913121225,17.2428974805044,0.));
#87141=CARTESIAN_POINT('Ctrl Pts',(-69.0427501919636,17.2413381067724,0.));
#87142=CARTESIAN_POINT('Ctrl Pts',(-69.065053766986,17.2397529045589,0.));
#87143=CARTESIAN_POINT('Ctrl Pts',(-69.0874018904598,17.2381418135491,0.));
#87144=CARTESIAN_POINT('Ctrl Pts',(-69.1097944163245,17.2365047738126,0.));
#87145=CARTESIAN_POINT('Ctrl Pts',(-69.1322311991752,17.2348417258015,0.));
#87146=CARTESIAN_POINT('Ctrl Pts',(-69.1547120942527,17.2331526103506,0.));
#87147=CARTESIAN_POINT('Ctrl Pts',(-69.1772369574447,17.2314373686701,0.));
#87148=CARTESIAN_POINT('Ctrl Pts',(-69.1998056452828,17.2296959423407,0.));
#87149=CARTESIAN_POINT('Ctrl Pts',(-69.222418014938,17.227928273312,0.));
#87150=CARTESIAN_POINT('Ctrl Pts',(-69.2450739242109,17.226134303902,0.));
#87151=CARTESIAN_POINT('Ctrl Pts',(-69.2677732315224,17.224313976797,0.));
#87152=CARTESIAN_POINT('Ctrl Pts',(-69.2905157959166,17.2224672350439,0.));
#87153=CARTESIAN_POINT('Ctrl Pts',(-69.3133014770554,17.2205940220459,0.));
#87154=CARTESIAN_POINT('Ctrl Pts',(-69.3361301352141,17.2186942815602,0.));
#87155=CARTESIAN_POINT('Ctrl Pts',(-69.3590016312692,17.2167679576984,0.));
#87156=CARTESIAN_POINT('Ctrl Pts',(-69.3819158266915,17.2148149949252,0.));
#87157=CARTESIAN_POINT('Ctrl Pts',(-69.404872583548,17.2128353380502,0.));
#87158=CARTESIAN_POINT('Ctrl Pts',(-69.4278717644973,17.2108289322254,0.));
#87159=CARTESIAN_POINT('Ctrl Pts',(-69.4509132327849,17.2087957229424,0.));
#87160=CARTESIAN_POINT('Ctrl Pts',(-69.4739968522313,17.2067356560337,0.));
#87161=CARTESIAN_POINT('Ctrl Pts',(-69.4971224872269,17.2046486776708,0.));
#87162=CARTESIAN_POINT('Ctrl Pts',(-69.5202900027367,17.2025347343577,0.));
#87163=CARTESIAN_POINT('Ctrl Pts',(-69.5434992642944,17.2003937729268,0.));
#87164=CARTESIAN_POINT('Ctrl Pts',(-69.5667501379969,17.1982257405377,0.));
#87165=CARTESIAN_POINT('Ctrl Pts',(-69.5900424904921,17.1960305846781,0.));
#87166=CARTESIAN_POINT('Ctrl Pts',(-69.6133761889749,17.1938082531612,0.));
#87167=CARTESIAN_POINT('Ctrl Pts',(-69.6367511011898,17.1915586941192,0.));
#87168=CARTESIAN_POINT('Ctrl Pts',(-69.6601670954269,17.1892818560003,0.));
#87169=CARTESIAN_POINT('Ctrl Pts',(-69.6836240405164,17.1869776875666,0.));
#87170=CARTESIAN_POINT('Ctrl Pts',(-69.7071218058178,17.1846461378973,0.));
#87171=CARTESIAN_POINT('Ctrl Pts',(-69.7306602612155,17.1822871563842,0.));
#87172=CARTESIAN_POINT('Ctrl Pts',(-69.7542392771234,17.179900692726,0.));
#87173=CARTESIAN_POINT('Ctrl Pts',(-69.777858724479,17.1774866969257,0.));
#87174=CARTESIAN_POINT('Ctrl Pts',(-69.8015184747398,17.1750451192886,0.));
#87175=CARTESIAN_POINT('Ctrl Pts',(-69.8252183998702,17.1725759104252,0.));
#87176=CARTESIAN_POINT('Ctrl Pts',(-69.8489583723407,17.1700790212474,0.));
#87177=CARTESIAN_POINT('Ctrl Pts',(-69.8727382651285,17.167554402962,0.));
#87178=CARTESIAN_POINT('Ctrl Pts',(-69.8965579517147,17.1650020070686,0.));
#87179=CARTESIAN_POINT('Ctrl Pts',(-69.9204173060781,17.1624217853578,0.));
#87180=CARTESIAN_POINT('Ctrl Pts',(-69.9443162026865,17.1598136899145,0.));
#87181=CARTESIAN_POINT('Ctrl Pts',(-69.9682545164939,17.157177673114,0.));
#87182=CARTESIAN_POINT('Ctrl Pts',(-69.9922321229424,17.1545136876161,0.));
#87183=CARTESIAN_POINT('Ctrl Pts',(-70.0162488979584,17.1518216863623,0.));
#87184=CARTESIAN_POINT('Ctrl Pts',(-70.0403047179483,17.1491016225749,0.));
#87185=CARTESIAN_POINT('Ctrl Pts',(-70.0643994597873,17.1463534497595,0.));
#87186=CARTESIAN_POINT('Ctrl Pts',(-70.0885330008179,17.1435771217018,0.));
#87187=CARTESIAN_POINT('Ctrl Pts',(-70.1127052188522,17.1407725924617,0.));
#87188=CARTESIAN_POINT('Ctrl Pts',(-70.1369159921687,17.1379398163709,0.));
#87189=CARTESIAN_POINT('Ctrl Pts',(-70.1611651995082,17.1350787480312,0.));
#87190=CARTESIAN_POINT('Ctrl Pts',(-70.1854527200631,17.1321893423182,0.));
#87191=CARTESIAN_POINT('Ctrl Pts',(-70.2097784334747,17.1292715543778,0.));
#87192=CARTESIAN_POINT('Ctrl Pts',(-70.2341422198363,17.1263253396202,0.));
#87193=CARTESIAN_POINT('Ctrl Pts',(-70.2585439596901,17.1233506537177,0.));
#87194=CARTESIAN_POINT('Ctrl Pts',(-70.2829835340238,17.1203474526031,0.));
#87195=CARTESIAN_POINT('Ctrl Pts',(-70.3074608242608,17.1173156924733,0.));
#87196=CARTESIAN_POINT('Ctrl Pts',(-70.3319757122568,17.1142553297867,0.));
#87197=CARTESIAN_POINT('Ctrl Pts',(-70.3565280803022,17.1111663212568,0.));
#87198=CARTESIAN_POINT('Ctrl Pts',(-70.3811178111201,17.1080486238499,0.));
#87199=CARTESIAN_POINT('Ctrl Pts',(-70.4057447878624,17.1049021947834,0.));
#87200=CARTESIAN_POINT('Ctrl Pts',(-70.430408894101,17.1017269915292,0.));
#87201=CARTESIAN_POINT('Ctrl Pts',(-70.4551100138238,17.0985229718125,0.));
#87202=CARTESIAN_POINT('Ctrl Pts',(-70.4798480314381,17.0952900936048,0.));
#87203=CARTESIAN_POINT('Ctrl Pts',(-70.5046228317677,17.0920283151219,0.));
#87204=CARTESIAN_POINT('Ctrl Pts',(-70.5294343000513,17.088737594822,0.));
#87205=CARTESIAN_POINT('Ctrl Pts',(-70.5542823219331,17.0854178914087,0.));
#87206=CARTESIAN_POINT('Ctrl Pts',(-70.5791667834582,17.082069163831,0.));
#87207=CARTESIAN_POINT('Ctrl Pts',(-70.6040875710749,17.0786913712764,0.));
#87208=CARTESIAN_POINT('Ctrl Pts',(-70.6290445716337,17.0752844731678,0.));
#87209=CARTESIAN_POINT('Ctrl Pts',(-70.6540376723841,17.0718484291624,0.));
#87210=CARTESIAN_POINT('Ctrl Pts',(-70.6790667609679,17.0683831991532,0.));
#87211=CARTESIAN_POINT('Ctrl Pts',(-70.7041317254125,17.0648887432714,0.));
#87212=CARTESIAN_POINT('Ctrl Pts',(-70.7292324541341,17.0613650218787,0.));
#87213=CARTESIAN_POINT('Ctrl Pts',(-70.7543688359374,17.0578119955649,0.));
#87214=CARTESIAN_POINT('Ctrl Pts',(-70.7795407600127,17.0542296251462,0.));
#87215=CARTESIAN_POINT('Ctrl Pts',(-70.8047481159306,17.0506178716664,0.));
#87216=CARTESIAN_POINT('Ctrl Pts',(-70.8299907936346,17.0469766964005,0.));
#87217=CARTESIAN_POINT('Ctrl Pts',(-70.8552686834435,17.0433060608479,0.));
#87218=CARTESIAN_POINT('Ctrl Pts',(-70.8805816760507,17.039605926728,0.));
#87219=CARTESIAN_POINT('Ctrl Pts',(-70.9059296625214,17.0358762559786,0.));
#87220=CARTESIAN_POINT('Ctrl Pts',(-70.9313125342872,17.0321170107562,0.));
#87221=CARTESIAN_POINT('Ctrl Pts',(-70.9567301831355,17.028328153439,0.));
#87222=CARTESIAN_POINT('Ctrl Pts',(-70.9821825012134,17.0245096466228,0.));
#87223=CARTESIAN_POINT('Ctrl Pts',(-71.0076693810302,17.0206614531166,0.));
#87224=CARTESIAN_POINT('Ctrl Pts',(-71.0331907154575,17.016783535942,0.));
#87225=CARTESIAN_POINT('Ctrl Pts',(-71.0587463977266,17.0128758583335,0.));
#87226=CARTESIAN_POINT('Ctrl Pts',(-71.0843363214216,17.0089383837437,0.));
#87227=CARTESIAN_POINT('Ctrl Pts',(-71.1099603804779,17.0049710758393,0.));
#87228=CARTESIAN_POINT('Ctrl Pts',(-71.1356184691799,17.0009738984935,0.));
#87229=CARTESIAN_POINT('Ctrl Pts',(-71.1613104821565,16.9969468157824,0.));
#87230=CARTESIAN_POINT('Ctrl Pts',(-71.1870363143742,16.9928897919829,0.));
#87231=CARTESIAN_POINT('Ctrl Pts',(-71.2127958611248,16.9888027915743,0.));
#87232=CARTESIAN_POINT('Ctrl Pts',(-71.2385890180233,16.9846857792385,0.));
#87233=CARTESIAN_POINT('Ctrl Pts',(-71.2644156810209,16.9805387198573,0.));
#87234=CARTESIAN_POINT('Ctrl Pts',(-71.2902757464127,16.9763615785138,0.));
#87235=CARTESIAN_POINT('Ctrl Pts',(-71.3161691108425,16.9721543204951,0.));
#87236=CARTESIAN_POINT('Ctrl Pts',(-71.3420956713072,16.9679169112993,0.));
#87237=CARTESIAN_POINT('Ctrl Pts',(-71.3680553251547,16.9636493166395,0.));
#87238=CARTESIAN_POINT('Ctrl Pts',(-71.3940479700662,16.9593515024274,0.));
#87239=CARTESIAN_POINT('Ctrl Pts',(-71.4200735040374,16.9550234347619,0.));
#87240=CARTESIAN_POINT('Ctrl Pts',(-71.4461318253561,16.9506650799189,0.));
#87241=CARTESIAN_POINT('Ctrl Pts',(-71.4722228325805,16.9462764043445,0.));
#87242=CARTESIAN_POINT('Ctrl Pts',(-71.4983464245069,16.9418573746492,0.));
#87243=CARTESIAN_POINT('Ctrl Pts',(-71.5245025002154,16.9374079576204,0.));
#87244=CARTESIAN_POINT('Ctrl Pts',(-71.5506909591139,16.9329281202379,0.));
#87245=CARTESIAN_POINT('Ctrl Pts',(-71.5769117009845,16.9284178296934,0.));
#87246=CARTESIAN_POINT('Ctrl Pts',(-71.6031646260169,16.923877053407,0.));
#87247=CARTESIAN_POINT('Ctrl Pts',(-71.6294496348644,16.9193057590605,0.));
#87248=CARTESIAN_POINT('Ctrl Pts',(-71.6557666285908,16.9147039145716,0.));
#87249=CARTESIAN_POINT('Ctrl Pts',(-71.6821155085605,16.9100714880367,0.));
#87250=CARTESIAN_POINT('Ctrl Pts',(-71.7084961763355,16.9054084476847,0.));
#87251=CARTESIAN_POINT('Ctrl Pts',(-71.7349085335796,16.9007147618344,0.));
#87252=CARTESIAN_POINT('Ctrl Pts',(-71.7613524819239,16.8959903988411,0.));
#87253=CARTESIAN_POINT('Ctrl Pts',(-71.7878279229556,16.8912353270944,0.));
#87254=CARTESIAN_POINT('Ctrl Pts',(-71.8143347584977,16.8864495151347,0.));
#87255=CARTESIAN_POINT('Ctrl Pts',(-71.8408728908269,16.8816329317473,0.));
#87256=CARTESIAN_POINT('Ctrl Pts',(-71.8674422229151,16.8767855460701,0.));
#87257=CARTESIAN_POINT('Ctrl Pts',(-71.8940426586521,16.8719073276967,0.));
#87258=CARTESIAN_POINT('Ctrl Pts',(-71.920674103086,16.8669982467915,0.));
#87259=CARTESIAN_POINT('Ctrl Pts',(-71.9473364618889,16.8620582738431,0.));
#87260=CARTESIAN_POINT('Ctrl Pts',(-71.9740296408319,16.8570873794264,0.));
#87261=CARTESIAN_POINT('Ctrl Pts',(-72.0007535452071,16.8520855339444,0.));
#87262=CARTESIAN_POINT('Ctrl Pts',(-72.0275080793742,16.8470527074278,0.));
#87263=CARTESIAN_POINT('Ctrl Pts',(-72.0542931459865,16.8419888691984,0.));
#87264=CARTESIAN_POINT('Ctrl Pts',(-72.0811086466178,16.8368939881457,0.));
#87265=CARTESIAN_POINT('Ctrl Pts',(-72.1079544831568,16.8317680333415,0.));
#87266=CARTESIAN_POINT('Ctrl Pts',(-72.1348305590233,16.8266109745802,0.));
#87267=CARTESIAN_POINT('Ctrl Pts',(-72.1617367803226,16.8214227828941,0.));
#87268=CARTESIAN_POINT('Ctrl Pts',(-72.1886730573389,16.8162034312257,0.));
#87269=CARTESIAN_POINT('Ctrl Pts',(-72.2156393048868,16.8109528945876,0.));
#87270=CARTESIAN_POINT('Ctrl Pts',(-72.2387802230662,16.8064254147767,0.));
#87271=CARTESIAN_POINT('Ctrl Pts',(-72.2565380035007,16.8029374213802,0.));
#87272=CARTESIAN_POINT('Ctrl Pts',(-72.2688994294958,16.8005027425889,0.));
#87273=CARTESIAN_POINT('Ctrl Pts',(-72.2758557890966,16.7991305317793,0.));
#87274=CARTESIAN_POINT('Ctrl Pts',(-72.2774028393482,16.7988252568807,0.));
#87275=CARTESIAN_POINT('',(-67.8307641965654,17.2912529479484,12.));
#87276=CARTESIAN_POINT('',(-67.8307641965654,17.2912529479484,0.));
#87277=CARTESIAN_POINT('Ctrl Pts',(-72.2774028393482,16.7988252568807,12.));
#87278=CARTESIAN_POINT('Ctrl Pts',(-72.2758557890966,16.7991305317793,12.));
#87279=CARTESIAN_POINT('Ctrl Pts',(-72.2688994294958,16.8005027425889,12.));
#87280=CARTESIAN_POINT('Ctrl Pts',(-72.2565380035007,16.8029374213802,12.));
#87281=CARTESIAN_POINT('Ctrl Pts',(-72.2387802230662,16.8064254147767,12.));
#87282=CARTESIAN_POINT('Ctrl Pts',(-72.2156393048868,16.8109528945876,12.));
#87283=CARTESIAN_POINT('Ctrl Pts',(-72.1886730573389,16.8162034312257,12.));
#87284=CARTESIAN_POINT('Ctrl Pts',(-72.1617367803226,16.8214227828941,12.));
#87285=CARTESIAN_POINT('Ctrl Pts',(-72.1348305590233,16.8266109745802,12.));
#87286=CARTESIAN_POINT('Ctrl Pts',(-72.1079544831568,16.8317680333415,12.));
#87287=CARTESIAN_POINT('Ctrl Pts',(-72.0811086466178,16.8368939881457,12.));
#87288=CARTESIAN_POINT('Ctrl Pts',(-72.0542931459865,16.8419888691984,12.));
#87289=CARTESIAN_POINT('Ctrl Pts',(-72.0275080793742,16.8470527074278,12.));
#87290=CARTESIAN_POINT('Ctrl Pts',(-72.0007535452071,16.8520855339444,12.));
#87291=CARTESIAN_POINT('Ctrl Pts',(-71.9740296408319,16.8570873794264,12.));
#87292=CARTESIAN_POINT('Ctrl Pts',(-71.9473364618889,16.8620582738431,12.));
#87293=CARTESIAN_POINT('Ctrl Pts',(-71.920674103086,16.8669982467915,12.));
#87294=CARTESIAN_POINT('Ctrl Pts',(-71.8940426586521,16.8719073276967,12.));
#87295=CARTESIAN_POINT('Ctrl Pts',(-71.8674422229151,16.8767855460701,12.));
#87296=CARTESIAN_POINT('Ctrl Pts',(-71.8408728908269,16.8816329317473,12.));
#87297=CARTESIAN_POINT('Ctrl Pts',(-71.8143347584977,16.8864495151347,12.));
#87298=CARTESIAN_POINT('Ctrl Pts',(-71.7878279229556,16.8912353270944,12.));
#87299=CARTESIAN_POINT('Ctrl Pts',(-71.7613524819239,16.8959903988411,12.));
#87300=CARTESIAN_POINT('Ctrl Pts',(-71.7349085335796,16.9007147618344,12.));
#87301=CARTESIAN_POINT('Ctrl Pts',(-71.7084961763355,16.9054084476847,12.));
#87302=CARTESIAN_POINT('Ctrl Pts',(-71.6821155085605,16.9100714880367,12.));
#87303=CARTESIAN_POINT('Ctrl Pts',(-71.6557666285908,16.9147039145716,12.));
#87304=CARTESIAN_POINT('Ctrl Pts',(-71.6294496348644,16.9193057590605,12.));
#87305=CARTESIAN_POINT('Ctrl Pts',(-71.6031646260169,16.923877053407,12.));
#87306=CARTESIAN_POINT('Ctrl Pts',(-71.5769117009845,16.9284178296934,12.));
#87307=CARTESIAN_POINT('Ctrl Pts',(-71.5506909591139,16.9329281202379,12.));
#87308=CARTESIAN_POINT('Ctrl Pts',(-71.5245025002154,16.9374079576204,12.));
#87309=CARTESIAN_POINT('Ctrl Pts',(-71.4983464245069,16.9418573746492,12.));
#87310=CARTESIAN_POINT('Ctrl Pts',(-71.4722228325805,16.9462764043445,12.));
#87311=CARTESIAN_POINT('Ctrl Pts',(-71.4461318253561,16.9506650799189,12.));
#87312=CARTESIAN_POINT('Ctrl Pts',(-71.4200735040374,16.9550234347619,12.));
#87313=CARTESIAN_POINT('Ctrl Pts',(-71.3940479700662,16.9593515024274,12.));
#87314=CARTESIAN_POINT('Ctrl Pts',(-71.3680553251547,16.9636493166395,12.));
#87315=CARTESIAN_POINT('Ctrl Pts',(-71.3420956713072,16.9679169112993,12.));
#87316=CARTESIAN_POINT('Ctrl Pts',(-71.3161691108425,16.9721543204951,12.));
#87317=CARTESIAN_POINT('Ctrl Pts',(-71.2902757464127,16.9763615785138,12.));
#87318=CARTESIAN_POINT('Ctrl Pts',(-71.2644156810209,16.9805387198573,12.));
#87319=CARTESIAN_POINT('Ctrl Pts',(-71.2385890180233,16.9846857792385,12.));
#87320=CARTESIAN_POINT('Ctrl Pts',(-71.2127958611248,16.9888027915743,12.));
#87321=CARTESIAN_POINT('Ctrl Pts',(-71.1870363143742,16.9928897919829,12.));
#87322=CARTESIAN_POINT('Ctrl Pts',(-71.1613104821565,16.9969468157824,12.));
#87323=CARTESIAN_POINT('Ctrl Pts',(-71.1356184691799,17.0009738984935,12.));
#87324=CARTESIAN_POINT('Ctrl Pts',(-71.1099603804779,17.0049710758393,12.));
#87325=CARTESIAN_POINT('Ctrl Pts',(-71.0843363214216,17.0089383837437,12.));
#87326=CARTESIAN_POINT('Ctrl Pts',(-71.0587463977266,17.0128758583335,12.));
#87327=CARTESIAN_POINT('Ctrl Pts',(-71.0331907154575,17.016783535942,12.));
#87328=CARTESIAN_POINT('Ctrl Pts',(-71.0076693810302,17.0206614531166,12.));
#87329=CARTESIAN_POINT('Ctrl Pts',(-70.9821825012134,17.0245096466228,12.));
#87330=CARTESIAN_POINT('Ctrl Pts',(-70.9567301831355,17.028328153439,12.));
#87331=CARTESIAN_POINT('Ctrl Pts',(-70.9313125342872,17.0321170107562,12.));
#87332=CARTESIAN_POINT('Ctrl Pts',(-70.9059296625214,17.0358762559786,12.));
#87333=CARTESIAN_POINT('Ctrl Pts',(-70.8805816760507,17.039605926728,12.));
#87334=CARTESIAN_POINT('Ctrl Pts',(-70.8552686834435,17.0433060608479,12.));
#87335=CARTESIAN_POINT('Ctrl Pts',(-70.8299907936346,17.0469766964005,12.));
#87336=CARTESIAN_POINT('Ctrl Pts',(-70.8047481159306,17.0506178716664,12.));
#87337=CARTESIAN_POINT('Ctrl Pts',(-70.7795407600127,17.0542296251462,12.));
#87338=CARTESIAN_POINT('Ctrl Pts',(-70.7543688359374,17.0578119955649,12.));
#87339=CARTESIAN_POINT('Ctrl Pts',(-70.7292324541341,17.0613650218787,12.));
#87340=CARTESIAN_POINT('Ctrl Pts',(-70.7041317254125,17.0648887432714,12.));
#87341=CARTESIAN_POINT('Ctrl Pts',(-70.6790667609679,17.0683831991532,12.));
#87342=CARTESIAN_POINT('Ctrl Pts',(-70.6540376723841,17.0718484291624,12.));
#87343=CARTESIAN_POINT('Ctrl Pts',(-70.6290445716337,17.0752844731678,12.));
#87344=CARTESIAN_POINT('Ctrl Pts',(-70.6040875710749,17.0786913712764,12.));
#87345=CARTESIAN_POINT('Ctrl Pts',(-70.5791667834582,17.082069163831,12.));
#87346=CARTESIAN_POINT('Ctrl Pts',(-70.5542823219331,17.0854178914087,12.));
#87347=CARTESIAN_POINT('Ctrl Pts',(-70.5294343000513,17.088737594822,12.));
#87348=CARTESIAN_POINT('Ctrl Pts',(-70.5046228317677,17.0920283151219,12.));
#87349=CARTESIAN_POINT('Ctrl Pts',(-70.4798480314381,17.0952900936048,12.));
#87350=CARTESIAN_POINT('Ctrl Pts',(-70.4551100138238,17.0985229718125,12.));
#87351=CARTESIAN_POINT('Ctrl Pts',(-70.430408894101,17.1017269915292,12.));
#87352=CARTESIAN_POINT('Ctrl Pts',(-70.4057447878624,17.1049021947834,12.));
#87353=CARTESIAN_POINT('Ctrl Pts',(-70.3811178111201,17.1080486238499,12.));
#87354=CARTESIAN_POINT('Ctrl Pts',(-70.3565280803022,17.1111663212568,12.));
#87355=CARTESIAN_POINT('Ctrl Pts',(-70.3319757122568,17.1142553297867,12.));
#87356=CARTESIAN_POINT('Ctrl Pts',(-70.3074608242608,17.1173156924733,12.));
#87357=CARTESIAN_POINT('Ctrl Pts',(-70.2829835340238,17.1203474526031,12.));
#87358=CARTESIAN_POINT('Ctrl Pts',(-70.2585439596901,17.1233506537177,12.));
#87359=CARTESIAN_POINT('Ctrl Pts',(-70.2341422198363,17.1263253396202,12.));
#87360=CARTESIAN_POINT('Ctrl Pts',(-70.2097784334747,17.1292715543778,12.));
#87361=CARTESIAN_POINT('Ctrl Pts',(-70.1854527200631,17.1321893423182,12.));
#87362=CARTESIAN_POINT('Ctrl Pts',(-70.1611651995082,17.1350787480312,12.));
#87363=CARTESIAN_POINT('Ctrl Pts',(-70.1369159921687,17.1379398163709,12.));
#87364=CARTESIAN_POINT('Ctrl Pts',(-70.1127052188522,17.1407725924617,12.));
#87365=CARTESIAN_POINT('Ctrl Pts',(-70.0885330008179,17.1435771217018,12.));
#87366=CARTESIAN_POINT('Ctrl Pts',(-70.0643994597873,17.1463534497595,12.));
#87367=CARTESIAN_POINT('Ctrl Pts',(-70.0403047179483,17.1491016225749,12.));
#87368=CARTESIAN_POINT('Ctrl Pts',(-70.0162488979584,17.1518216863623,12.));
#87369=CARTESIAN_POINT('Ctrl Pts',(-69.9922321229424,17.1545136876161,12.));
#87370=CARTESIAN_POINT('Ctrl Pts',(-69.9682545164939,17.157177673114,12.));
#87371=CARTESIAN_POINT('Ctrl Pts',(-69.9443162026865,17.1598136899145,12.));
#87372=CARTESIAN_POINT('Ctrl Pts',(-69.9204173060781,17.1624217853578,12.));
#87373=CARTESIAN_POINT('Ctrl Pts',(-69.8965579517147,17.1650020070686,12.));
#87374=CARTESIAN_POINT('Ctrl Pts',(-69.8727382651285,17.167554402962,12.));
#87375=CARTESIAN_POINT('Ctrl Pts',(-69.8489583723407,17.1700790212474,12.));
#87376=CARTESIAN_POINT('Ctrl Pts',(-69.8252183998702,17.1725759104252,12.));
#87377=CARTESIAN_POINT('Ctrl Pts',(-69.8015184747398,17.1750451192886,12.));
#87378=CARTESIAN_POINT('Ctrl Pts',(-69.777858724479,17.1774866969257,12.));
#87379=CARTESIAN_POINT('Ctrl Pts',(-69.7542392771234,17.179900692726,12.));
#87380=CARTESIAN_POINT('Ctrl Pts',(-69.7306602612155,17.1822871563842,12.));
#87381=CARTESIAN_POINT('Ctrl Pts',(-69.7071218058178,17.1846461378973,12.));
#87382=CARTESIAN_POINT('Ctrl Pts',(-69.6836240405164,17.1869776875666,12.));
#87383=CARTESIAN_POINT('Ctrl Pts',(-69.6601670954269,17.1892818560003,12.));
#87384=CARTESIAN_POINT('Ctrl Pts',(-69.6367511011898,17.1915586941192,12.));
#87385=CARTESIAN_POINT('Ctrl Pts',(-69.6133761889749,17.1938082531612,12.));
#87386=CARTESIAN_POINT('Ctrl Pts',(-69.5900424904921,17.1960305846781,12.));
#87387=CARTESIAN_POINT('Ctrl Pts',(-69.5667501379969,17.1982257405377,12.));
#87388=CARTESIAN_POINT('Ctrl Pts',(-69.5434992642944,17.2003937729268,12.));
#87389=CARTESIAN_POINT('Ctrl Pts',(-69.5202900027367,17.2025347343577,12.));
#87390=CARTESIAN_POINT('Ctrl Pts',(-69.4971224872269,17.2046486776708,12.));
#87391=CARTESIAN_POINT('Ctrl Pts',(-69.4739968522313,17.2067356560337,12.));
#87392=CARTESIAN_POINT('Ctrl Pts',(-69.4509132327849,17.2087957229424,12.));
#87393=CARTESIAN_POINT('Ctrl Pts',(-69.4278717644973,17.2108289322254,12.));
#87394=CARTESIAN_POINT('Ctrl Pts',(-69.404872583548,17.2128353380502,12.));
#87395=CARTESIAN_POINT('Ctrl Pts',(-69.3819158266915,17.2148149949252,12.));
#87396=CARTESIAN_POINT('Ctrl Pts',(-69.3590016312692,17.2167679576984,12.));
#87397=CARTESIAN_POINT('Ctrl Pts',(-69.3361301352141,17.2186942815602,12.));
#87398=CARTESIAN_POINT('Ctrl Pts',(-69.3133014770554,17.2205940220459,12.));
#87399=CARTESIAN_POINT('Ctrl Pts',(-69.2905157959166,17.2224672350439,12.));
#87400=CARTESIAN_POINT('Ctrl Pts',(-69.2677732315224,17.224313976797,12.));
#87401=CARTESIAN_POINT('Ctrl Pts',(-69.2450739242109,17.226134303902,12.));
#87402=CARTESIAN_POINT('Ctrl Pts',(-69.222418014938,17.227928273312,12.));
#87403=CARTESIAN_POINT('Ctrl Pts',(-69.1998056452828,17.2296959423407,12.));
#87404=CARTESIAN_POINT('Ctrl Pts',(-69.1772369574447,17.2314373686701,12.));
#87405=CARTESIAN_POINT('Ctrl Pts',(-69.1547120942527,17.2331526103506,12.));
#87406=CARTESIAN_POINT('Ctrl Pts',(-69.1322311991752,17.2348417258015,12.));
#87407=CARTESIAN_POINT('Ctrl Pts',(-69.1097944163245,17.2365047738126,12.));
#87408=CARTESIAN_POINT('Ctrl Pts',(-69.0874018904598,17.2381418135491,12.));
#87409=CARTESIAN_POINT('Ctrl Pts',(-69.065053766986,17.2397529045589,12.));
#87410=CARTESIAN_POINT('Ctrl Pts',(-69.0427501919636,17.2413381067724,12.));
#87411=CARTESIAN_POINT('Ctrl Pts',(-69.0204913121225,17.2428974805044,12.));
#87412=CARTESIAN_POINT('Ctrl Pts',(-68.9982772748694,17.2444310864585,12.));
#87413=CARTESIAN_POINT('Ctrl Pts',(-68.9761082282922,17.2459389857327,12.));
#87414=CARTESIAN_POINT('Ctrl Pts',(-68.9539843211619,17.2474212398275,12.));
#87415=CARTESIAN_POINT('Ctrl Pts',(-68.9319057029409,17.248877910643,12.));
#87416=CARTESIAN_POINT('Ctrl Pts',(-68.909872523787,17.2503090604792,12.));
#87417=CARTESIAN_POINT('Ctrl Pts',(-68.8878849345557,17.2517147520376,12.));
#87418=CARTESIAN_POINT('Ctrl Pts',(-68.8659430867972,17.2530950484258,12.));
#87419=CARTESIAN_POINT('Ctrl Pts',(-68.844047132755,17.2544500131625,12.));
#87420=CARTESIAN_POINT('Ctrl Pts',(-68.8221972253941,17.2557797101813,12.));
#87421=CARTESIAN_POINT('Ctrl Pts',(-68.8003935184184,17.2570842038384,12.));
#87422=CARTESIAN_POINT('Ctrl Pts',(-68.7786361662882,17.2583635589198,12.));
#87423=CARTESIAN_POINT('Ctrl Pts',(-68.7569253242333,17.2596178406551,12.));
#87424=CARTESIAN_POINT('Ctrl Pts',(-68.7352611482547,17.2608471147185,12.));
#87425=CARTESIAN_POINT('Ctrl Pts',(-68.7136437951097,17.2620514472182,12.));
#87426=CARTESIAN_POINT('Ctrl Pts',(-68.6920734222938,17.2632309046892,12.));
#87427=CARTESIAN_POINT('Ctrl Pts',(-68.6705501880249,17.2643855540892,12.));
#87428=CARTESIAN_POINT('Ctrl Pts',(-68.6490742512057,17.2655154627928,12.));
#87429=CARTESIAN_POINT('Ctrl Pts',(-68.6276457714729,17.2666206986084,12.));
#87430=CARTESIAN_POINT('Ctrl Pts',(-68.6062649092764,17.2677013298057,12.));
#87431=CARTESIAN_POINT('Ctrl Pts',(-68.5849318259449,17.2687574251429,12.));
#87432=CARTESIAN_POINT('Ctrl Pts',(-68.5636466837517,17.269789053896,12.));
#87433=CARTESIAN_POINT('Ctrl Pts',(-68.5424096459772,17.2707962858919,12.));
#87434=CARTESIAN_POINT('Ctrl Pts',(-68.521220876786,17.2717791914544,12.));
#87435=CARTESIAN_POINT('Ctrl Pts',(-68.5000805410911,17.2727378413489,12.));
#87436=CARTESIAN_POINT('Ctrl Pts',(-68.4789888044351,17.2736723067365,12.));
#87437=CARTESIAN_POINT('Ctrl Pts',(-68.4579458328185,17.2745826591119,12.));
#87438=CARTESIAN_POINT('Ctrl Pts',(-68.436951792677,17.2754689702992,12.));
#87439=CARTESIAN_POINT('Ctrl Pts',(-68.4160068512753,17.2763313126018,12.));
#87440=CARTESIAN_POINT('Ctrl Pts',(-68.3951111770487,17.2771697589385,12.));
#87441=CARTESIAN_POINT('Ctrl Pts',(-68.3742649398964,17.2779843829608,12.));
#87442=CARTESIAN_POINT('Ctrl Pts',(-68.3534683116514,17.2787752592484,12.));
#87443=CARTESIAN_POINT('Ctrl Pts',(-68.3327214657575,17.2795424631799,12.));
#87444=CARTESIAN_POINT('Ctrl Pts',(-68.3120245763914,17.2802860705815,12.));
#87445=CARTESIAN_POINT('Ctrl Pts',(-68.2913778177261,17.2810061574353,12.));
#87446=CARTESIAN_POINT('Ctrl Pts',(-68.2707813631731,17.2817027995831,12.));
#87447=CARTESIAN_POINT('Ctrl Pts',(-68.2502353845071,17.2823760723874,12.));
#87448=CARTESIAN_POINT('Ctrl Pts',(-68.2297400535294,17.2830260513868,12.));
#87449=CARTESIAN_POINT('Ctrl Pts',(-68.2092955440567,17.2836528130819,12.));
#87450=CARTESIAN_POINT('Ctrl Pts',(-68.1889020335427,17.2842564355799,12.));
#87451=CARTESIAN_POINT('Ctrl Pts',(-68.1685597054231,17.2848369995293,12.));
#87452=CARTESIAN_POINT('Ctrl Pts',(-68.1482687493226,17.2853945882072,12.));
#87453=CARTESIAN_POINT('Ctrl Pts',(-68.1280293561511,17.2859292855705,12.));
#87454=CARTESIAN_POINT('Ctrl Pts',(-68.1078417137877,17.2864411745459,12.));
#87455=CARTESIAN_POINT('Ctrl Pts',(-68.0877060033205,17.2869303355432,12.));
#87456=CARTESIAN_POINT('Ctrl Pts',(-68.0676223930412,17.2873968440839,12.));
#87457=CARTESIAN_POINT('Ctrl Pts',(-68.0475910442424,17.2878407730961,12.));
#87458=CARTESIAN_POINT('Ctrl Pts',(-68.0276121227356,17.2882621974721,12.));
#87459=CARTESIAN_POINT('Ctrl Pts',(-68.007685808115,17.2886611977401,12.));
#87460=CARTESIAN_POINT('Ctrl Pts',(-67.987812304921,17.2890378644866,12.));
#87461=CARTESIAN_POINT('Ctrl Pts',(-67.9679918502579,17.2893923013894,12.));
#87462=CARTESIAN_POINT('Ctrl Pts',(-67.9482246901667,17.2897246158941,12.));
#87463=CARTESIAN_POINT('Ctrl Pts',(-67.9285110571741,17.2900349103981,12.));
#87464=CARTESIAN_POINT('Ctrl Pts',(-67.9088511496685,17.2903232740694,12.));
#87465=CARTESIAN_POINT('Ctrl Pts',(-67.8892451049608,17.2905897723949,12.));
#87466=CARTESIAN_POINT('Ctrl Pts',(-67.8696929978782,17.2908344459695,12.));
#87467=CARTESIAN_POINT('Ctrl Pts',(-67.8540944889687,17.291012743109,12.));
#87468=CARTESIAN_POINT('Ctrl Pts',(-67.842419897098,17.2911366591348,12.));
#87469=CARTESIAN_POINT('Ctrl Pts',(-67.8346476309018,17.2912149114119,12.));
#87470=CARTESIAN_POINT('Ctrl Pts',(-67.8307641965654,17.2912529479484,12.));
#87471=CARTESIAN_POINT('Ctrl Pts',(-72.6050633494711,15.320844207742,-1.11022302462516E-15));
#87472=CARTESIAN_POINT('Ctrl Pts',(-72.6050633494711,15.320844207742,4.));
#87473=CARTESIAN_POINT('Ctrl Pts',(-72.6050633494711,15.320844207742,8.));
#87474=CARTESIAN_POINT('Ctrl Pts',(-72.6050633494711,15.320844207742,12.));
#87475=CARTESIAN_POINT('Ctrl Pts',(-72.6937764817667,15.3856835210418,-1.11022302462516E-15));
#87476=CARTESIAN_POINT('Ctrl Pts',(-72.6937764817667,15.3856835210418,4.));
#87477=CARTESIAN_POINT('Ctrl Pts',(-72.6937764817667,15.3856835210418,8.00000000000001));
#87478=CARTESIAN_POINT('Ctrl Pts',(-72.6937764817667,15.3856835210418,12.));
#87479=CARTESIAN_POINT('Ctrl Pts',(-72.8096834307708,15.5519317750286,-1.11022302462516E-15));
#87480=CARTESIAN_POINT('Ctrl Pts',(-72.8096834307708,15.5519317750286,4.));
#87481=CARTESIAN_POINT('Ctrl Pts',(-72.8096834307708,15.5519317750286,7.99999999999999));
#87482=CARTESIAN_POINT('Ctrl Pts',(-72.8096834307708,15.5519317750286,12.));
#87483=CARTESIAN_POINT('Ctrl Pts',(-72.8161171750014,15.7502340068143,-1.11022302462516E-15));
#87484=CARTESIAN_POINT('Ctrl Pts',(-72.8161171750014,15.7502340068143,4.));
#87485=CARTESIAN_POINT('Ctrl Pts',(-72.8161171750014,15.7502340068143,8.00000000000001));
#87486=CARTESIAN_POINT('Ctrl Pts',(-72.8161171750014,15.7502340068143,12.));
#87487=CARTESIAN_POINT('Ctrl Pts',(-72.7986051948036,15.830763774723,-1.11022302462516E-15));
#87488=CARTESIAN_POINT('Ctrl Pts',(-72.7986051948036,15.830763774723,4.));
#87489=CARTESIAN_POINT('Ctrl Pts',(-72.7986051948036,15.830763774723,8.));
#87490=CARTESIAN_POINT('Ctrl Pts',(-72.7986051948036,15.830763774723,12.));
#87491=CARTESIAN_POINT('',(-72.6050633494711,15.320844207742,0.));
#87492=CARTESIAN_POINT('',(-72.7986051948038,15.8307637747231,-2.77555756156289E-16));
#87493=CARTESIAN_POINT('Ctrl Pts',(-72.6050633494711,15.320844207742,0.));
#87494=CARTESIAN_POINT('Ctrl Pts',(-72.6937764817667,15.3856835210418,-3.08148791101957E-31));
#87495=CARTESIAN_POINT('Ctrl Pts',(-72.7600090240548,15.48068252332,3.08148791101958E-31));
#87496=CARTESIAN_POINT('Ctrl Pts',(-72.7904952137637,15.5861481305937,2.18952885050753E-46));
#87497=CARTESIAN_POINT('Ctrl Pts',(-72.8133598560454,15.665247336049,-1.54074395550979E-31));
#87498=CARTESIAN_POINT('Ctrl Pts',(-72.8161171750014,15.7502340068143,-9.24446373305873E-31));
#87499=CARTESIAN_POINT('Ctrl Pts',(-72.7986051948036,15.830763774723,-1.09476442525376E-46));
#87500=CARTESIAN_POINT('',(-72.7986051948038,15.8307637747231,12.));
#87501=CARTESIAN_POINT('Ctrl Pts',(-72.7986051948036,15.830763774723,-1.11022302462516E-15));
#87502=CARTESIAN_POINT('Ctrl Pts',(-72.7986051948036,15.830763774723,4.));
#87503=CARTESIAN_POINT('Ctrl Pts',(-72.7986051948036,15.830763774723,8.));
#87504=CARTESIAN_POINT('Ctrl Pts',(-72.7986051948036,15.830763774723,12.));
#87505=CARTESIAN_POINT('',(-72.6050633494711,15.320844207742,12.));
#87506=CARTESIAN_POINT('Ctrl Pts',(-72.7986051948036,15.830763774723,12.));
#87507=CARTESIAN_POINT('Ctrl Pts',(-72.8161171750014,15.7502340068143,12.));
#87508=CARTESIAN_POINT('Ctrl Pts',(-72.8133598560454,15.665247336049,12.));
#87509=CARTESIAN_POINT('Ctrl Pts',(-72.7904952137637,15.5861481305937,12.));
#87510=CARTESIAN_POINT('Ctrl Pts',(-72.7600090240548,15.48068252332,12.));
#87511=CARTESIAN_POINT('Ctrl Pts',(-72.6937764817667,15.3856835210418,12.));
#87512=CARTESIAN_POINT('Ctrl Pts',(-72.6050633494711,15.320844207742,12.));
#87513=CARTESIAN_POINT('Ctrl Pts',(-72.6050633494711,15.320844207742,12.));
#87514=CARTESIAN_POINT('Ctrl Pts',(-72.6050633494711,15.320844207742,8.));
#87515=CARTESIAN_POINT('Ctrl Pts',(-72.6050633494711,15.320844207742,4.));
#87516=CARTESIAN_POINT('Ctrl Pts',(-72.6050633494711,15.320844207742,-1.11022302462516E-15));
#87517=CARTESIAN_POINT('Origin',(-3.65979954444617E-10,8.10341340518592E-11,
0.));
#87518=CARTESIAN_POINT('Origin',(-3.65979954444617E-10,8.10341340518592E-11,
12.));
#87519=CARTESIAN_POINT('Origin',(-3.65979954444617E-10,8.10341340518592E-11,
0.));
#87520=CARTESIAN_POINT('Ctrl Pts',(-70.9608233461363,22.6894590071785,0.));
#87521=CARTESIAN_POINT('Ctrl Pts',(-70.9608233461363,22.6894590071785,4.));
#87522=CARTESIAN_POINT('Ctrl Pts',(-70.9608233461364,22.6894590071785,8.));
#87523=CARTESIAN_POINT('Ctrl Pts',(-70.9608233461364,22.6894590071785,12.));
#87524=CARTESIAN_POINT('Ctrl Pts',(-70.9273579271571,22.7941214270114,0.));
#87525=CARTESIAN_POINT('Ctrl Pts',(-70.9273579271571,22.7941214270114,4.));
#87526=CARTESIAN_POINT('Ctrl Pts',(-70.9273579271571,22.7941214270114,8.00000000000001));
#87527=CARTESIAN_POINT('Ctrl Pts',(-70.9273579271571,22.7941214270114,12.));
#87528=CARTESIAN_POINT('Ctrl Pts',(-70.8062825417802,22.9566438338675,0.));
#87529=CARTESIAN_POINT('Ctrl Pts',(-70.8062825417802,22.9566438338675,4.));
#87530=CARTESIAN_POINT('Ctrl Pts',(-70.8062825417802,22.9566438338675,7.99999999999999));
#87531=CARTESIAN_POINT('Ctrl Pts',(-70.8062825417802,22.9566438338675,12.));
#87532=CARTESIAN_POINT('Ctrl Pts',(-70.6201870200062,23.0254444386656,0.));
#87533=CARTESIAN_POINT('Ctrl Pts',(-70.6201870200062,23.0254444386656,4.));
#87534=CARTESIAN_POINT('Ctrl Pts',(-70.6201870200063,23.0254444386655,8.00000000000001));
#87535=CARTESIAN_POINT('Ctrl Pts',(-70.6201870200063,23.0254444386655,12.));
#87536=CARTESIAN_POINT('Ctrl Pts',(-70.5382514078488,23.0342913834094,0.));
#87537=CARTESIAN_POINT('Ctrl Pts',(-70.5382514078488,23.0342913834094,4.));
#87538=CARTESIAN_POINT('Ctrl Pts',(-70.5382514078489,23.0342913834093,8.));
#87539=CARTESIAN_POINT('Ctrl Pts',(-70.5382514078489,23.0342913834093,12.));
#87540=CARTESIAN_POINT('',(-70.9608233461363,22.6894590071785,0.));
#87541=CARTESIAN_POINT('',(-70.5382514078488,23.0342913834093,0.));
#87542=CARTESIAN_POINT('Ctrl Pts',(-70.9608233461363,22.6894590071785,0.));
#87543=CARTESIAN_POINT('Ctrl Pts',(-70.9273579271571,22.7941214270114,0.));
#87544=CARTESIAN_POINT('Ctrl Pts',(-70.858171992656,22.8869913737863,0.));
#87545=CARTESIAN_POINT('Ctrl Pts',(-70.767754993209,22.9492582831545,0.));
#87546=CARTESIAN_POINT('Ctrl Pts',(-70.6999422436237,22.9959584651807,0.));
#87547=CARTESIAN_POINT('Ctrl Pts',(-70.6201870200062,23.0254444386656,0.));
#87548=CARTESIAN_POINT('Ctrl Pts',(-70.5382514078488,23.0342913834094,0.));
#87549=CARTESIAN_POINT('',(-70.5382514078489,23.0342913834093,12.));
#87550=CARTESIAN_POINT('Ctrl Pts',(-70.5382514078488,23.0342913834094,0.));
#87551=CARTESIAN_POINT('Ctrl Pts',(-70.5382514078488,23.0342913834094,4.));
#87552=CARTESIAN_POINT('Ctrl Pts',(-70.5382514078489,23.0342913834093,8.));
#87553=CARTESIAN_POINT('Ctrl Pts',(-70.5382514078489,23.0342913834093,12.));
#87554=CARTESIAN_POINT('',(-70.9608233461364,22.6894590071785,12.));
#87555=CARTESIAN_POINT('Ctrl Pts',(-70.5382514078489,23.0342913834093,12.));
#87556=CARTESIAN_POINT('Ctrl Pts',(-70.6201870200063,23.0254444386655,12.));
#87557=CARTESIAN_POINT('Ctrl Pts',(-70.6999422436237,22.9959584651806,12.));
#87558=CARTESIAN_POINT('Ctrl Pts',(-70.767754993209,22.9492582831545,12.));
#87559=CARTESIAN_POINT('Ctrl Pts',(-70.858171992656,22.8869913737863,12.));
#87560=CARTESIAN_POINT('Ctrl Pts',(-70.9273579271571,22.7941214270114,12.));
#87561=CARTESIAN_POINT('Ctrl Pts',(-70.9608233461364,22.6894590071785,12.));
#87562=CARTESIAN_POINT('Ctrl Pts',(-70.9608233461364,22.6894590071785,12.));
#87563=CARTESIAN_POINT('Ctrl Pts',(-70.9608233461364,22.6894590071785,8.));
#87564=CARTESIAN_POINT('Ctrl Pts',(-70.9608233461363,22.6894590071785,4.));
#87565=CARTESIAN_POINT('Ctrl Pts',(-70.9608233461363,22.6894590071785,0.));
#87566=CARTESIAN_POINT('Ctrl Pts',(-66.0656156664138,23.1372951448024,0.));
#87567=CARTESIAN_POINT('Ctrl Pts',(-66.0656156664138,23.1372951448024,12.));
#87568=CARTESIAN_POINT('Ctrl Pts',(-66.0694876382127,23.1375957166104,0.));
#87569=CARTESIAN_POINT('Ctrl Pts',(-66.0694876382127,23.1375957166104,12.));
#87570=CARTESIAN_POINT('Ctrl Pts',(-66.0772371487248,23.13819515974,0.));
#87571=CARTESIAN_POINT('Ctrl Pts',(-66.0772371487248,23.13819515974,12.));
#87572=CARTESIAN_POINT('Ctrl Pts',(-66.0888781152421,23.1390892229778,0.));
#87573=CARTESIAN_POINT('Ctrl Pts',(-66.0888781152421,23.1390892229778,12.));
#87574=CARTESIAN_POINT('Ctrl Pts',(-66.1044328067355,23.1402711039425,0.));
#87575=CARTESIAN_POINT('Ctrl Pts',(-66.1044328067355,23.1402711039425,12.));
#87576=CARTESIAN_POINT('Ctrl Pts',(-66.1239318368548,23.1417314398398,0.));
#87577=CARTESIAN_POINT('Ctrl Pts',(-66.1239318368548,23.1417314398398,12.));
#87578=CARTESIAN_POINT('Ctrl Pts',(-66.1434865015027,23.1431747350098,0.));
#87579=CARTESIAN_POINT('Ctrl Pts',(-66.1434865015027,23.1431747350098,12.));
#87580=CARTESIAN_POINT('Ctrl Pts',(-66.1630967296747,23.1446009424903,0.));
#87581=CARTESIAN_POINT('Ctrl Pts',(-66.1630967296747,23.1446009424903,12.));
#87582=CARTESIAN_POINT('Ctrl Pts',(-66.18276239029,23.1460099850763,0.));
#87583=CARTESIAN_POINT('Ctrl Pts',(-66.18276239029,23.1460099850763,12.));
#87584=CARTESIAN_POINT('Ctrl Pts',(-66.2024832934866,23.1474017566484,0.));
#87585=CARTESIAN_POINT('Ctrl Pts',(-66.2024832934866,23.1474017566484,12.));
#87586=CARTESIAN_POINT('Ctrl Pts',(-66.2222592165473,23.1487761349328,0.));
#87587=CARTESIAN_POINT('Ctrl Pts',(-66.2222592165473,23.1487761349328,12.));
#87588=CARTESIAN_POINT('Ctrl Pts',(-66.2420899237317,23.1501329914488,0.));
#87589=CARTESIAN_POINT('Ctrl Pts',(-66.2420899237317,23.1501329914488,12.));
#87590=CARTESIAN_POINT('Ctrl Pts',(-66.2619751878741,23.1514722022483,0.));
#87591=CARTESIAN_POINT('Ctrl Pts',(-66.2619751878741,23.1514722022483,12.));
#87592=CARTESIAN_POINT('Ctrl Pts',(-66.2819148131072,23.1527936592625,0.));
#87593=CARTESIAN_POINT('Ctrl Pts',(-66.2819148131072,23.1527936592625,12.));
#87594=CARTESIAN_POINT('Ctrl Pts',(-66.301908627539,23.154097266617,0.));
#87595=CARTESIAN_POINT('Ctrl Pts',(-66.301908627539,23.154097266617,12.));
#87596=CARTESIAN_POINT('Ctrl Pts',(-66.3219564725161,23.1553829352531,0.));
#87597=CARTESIAN_POINT('Ctrl Pts',(-66.3219564725161,23.1553829352531,12.));
#87598=CARTESIAN_POINT('Ctrl Pts',(-66.3420581937159,23.1566505784626,0.));
#87599=CARTESIAN_POINT('Ctrl Pts',(-66.3420581937159,23.1566505784626,12.));
#87600=CARTESIAN_POINT('Ctrl Pts',(-66.3622136300692,23.1579001063438,0.));
#87601=CARTESIAN_POINT('Ctrl Pts',(-66.3622136300692,23.1579001063438,12.));
#87602=CARTESIAN_POINT('Ctrl Pts',(-66.382422608185,23.15913142301,0.));
#87603=CARTESIAN_POINT('Ctrl Pts',(-66.382422608185,23.15913142301,12.));
#87604=CARTESIAN_POINT('Ctrl Pts',(-66.402684948127,23.1603444294754,0.));
#87605=CARTESIAN_POINT('Ctrl Pts',(-66.402684948127,23.1603444294754,12.));
#87606=CARTESIAN_POINT('Ctrl Pts',(-66.4230004670288,23.1615390254635,0.));
#87607=CARTESIAN_POINT('Ctrl Pts',(-66.4230004670288,23.1615390254635,12.));
#87608=CARTESIAN_POINT('Ctrl Pts',(-66.4433689832454,23.1627151114875,0.));
#87609=CARTESIAN_POINT('Ctrl Pts',(-66.4433689832454,23.1627151114875,12.));
#87610=CARTESIAN_POINT('Ctrl Pts',(-66.4637903210682,23.163872591218,0.));
#87611=CARTESIAN_POINT('Ctrl Pts',(-66.4637903210682,23.163872591218,12.));
#87612=CARTESIAN_POINT('Ctrl Pts',(-66.4842643105263,23.1650113713792,0.));
#87613=CARTESIAN_POINT('Ctrl Pts',(-66.4842643105263,23.1650113713792,12.));
#87614=CARTESIAN_POINT('Ctrl Pts',(-66.5047907851319,23.1661313606123,0.));
#87615=CARTESIAN_POINT('Ctrl Pts',(-66.5047907851319,23.1661313606123,12.));
#87616=CARTESIAN_POINT('Ctrl Pts',(-66.5253695803209,23.1672324686927,0.));
#87617=CARTESIAN_POINT('Ctrl Pts',(-66.5253695803209,23.1672324686927,12.));
#87618=CARTESIAN_POINT('Ctrl Pts',(-66.5460005315406,23.1683146055736,0.));
#87619=CARTESIAN_POINT('Ctrl Pts',(-66.5460005315406,23.1683146055736,12.));
#87620=CARTESIAN_POINT('Ctrl Pts',(-66.5666834726495,23.169377680588,0.));
#87621=CARTESIAN_POINT('Ctrl Pts',(-66.5666834726495,23.169377680588,12.));
#87622=CARTESIAN_POINT('Ctrl Pts',(-66.5874182367597,23.1704216028626,0.));
#87623=CARTESIAN_POINT('Ctrl Pts',(-66.5874182367597,23.1704216028626,12.));
#87624=CARTESIAN_POINT('Ctrl Pts',(-66.6082046569657,23.1714462816794,0.));
#87625=CARTESIAN_POINT('Ctrl Pts',(-66.6082046569657,23.1714462816794,12.));
#87626=CARTESIAN_POINT('Ctrl Pts',(-66.6290425670538,23.1724516268299,0.));
#87627=CARTESIAN_POINT('Ctrl Pts',(-66.6290425670538,23.1724516268299,12.));
#87628=CARTESIAN_POINT('Ctrl Pts',(-66.6499318023445,23.1734375490421,0.));
#87629=CARTESIAN_POINT('Ctrl Pts',(-66.6499318023445,23.1734375490421,12.));
#87630=CARTESIAN_POINT('Ctrl Pts',(-66.6708722000047,23.174403960137,0.));
#87631=CARTESIAN_POINT('Ctrl Pts',(-66.6708722000047,23.174403960137,12.));
#87632=CARTESIAN_POINT('Ctrl Pts',(-66.691863598595,23.1753507727931,0.));
#87633=CARTESIAN_POINT('Ctrl Pts',(-66.691863598595,23.1753507727931,12.));
#87634=CARTESIAN_POINT('Ctrl Pts',(-66.712905837789,23.1762779004043,0.));
#87635=CARTESIAN_POINT('Ctrl Pts',(-66.712905837789,23.1762779004043,12.));
#87636=CARTESIAN_POINT('Ctrl Pts',(-66.7339987580441,23.1771852569136,0.));
#87637=CARTESIAN_POINT('Ctrl Pts',(-66.7339987580441,23.1771852569136,12.));
#87638=CARTESIAN_POINT('Ctrl Pts',(-66.7551422002229,23.1780727566309,0.));
#87639=CARTESIAN_POINT('Ctrl Pts',(-66.7551422002229,23.1780727566309,12.));
#87640=CARTESIAN_POINT('Ctrl Pts',(-66.7763360056146,23.1789403142375,0.));
#87641=CARTESIAN_POINT('Ctrl Pts',(-66.7763360056146,23.1789403142375,12.));
#87642=CARTESIAN_POINT('Ctrl Pts',(-66.7975800161014,23.1797878448645,0.));
#87643=CARTESIAN_POINT('Ctrl Pts',(-66.7975800161014,23.1797878448645,12.));
#87644=CARTESIAN_POINT('Ctrl Pts',(-66.8188740742727,23.1806152641475,0.));
#87645=CARTESIAN_POINT('Ctrl Pts',(-66.8188740742727,23.1806152641475,12.));
#87646=CARTESIAN_POINT('Ctrl Pts',(-66.840218023555,23.1814224882948,0.));
#87647=CARTESIAN_POINT('Ctrl Pts',(-66.840218023555,23.1814224882948,12.));
#87648=CARTESIAN_POINT('Ctrl Pts',(-66.8616117083304,23.1822094341508,0.));
#87649=CARTESIAN_POINT('Ctrl Pts',(-66.8616117083304,23.1822094341508,12.));
#87650=CARTESIAN_POINT('Ctrl Pts',(-66.8830549738768,23.1829760191582,0.));
#87651=CARTESIAN_POINT('Ctrl Pts',(-66.8830549738768,23.1829760191582,12.));
#87652=CARTESIAN_POINT('Ctrl Pts',(-66.904547666305,23.1837221613231,0.));
#87653=CARTESIAN_POINT('Ctrl Pts',(-66.904547666305,23.1837221613231,12.));
#87654=CARTESIAN_POINT('Ctrl Pts',(-66.9260896324955,23.1844477791816,0.));
#87655=CARTESIAN_POINT('Ctrl Pts',(-66.9260896324955,23.1844477791816,12.));
#87656=CARTESIAN_POINT('Ctrl Pts',(-66.9476807200225,23.1851527917665,0.));
#87657=CARTESIAN_POINT('Ctrl Pts',(-66.9476807200225,23.1851527917665,12.));
#87658=CARTESIAN_POINT('Ctrl Pts',(-66.9693207771059,23.1858371185852,0.));
#87659=CARTESIAN_POINT('Ctrl Pts',(-66.9693207771059,23.1858371185852,12.));
#87660=CARTESIAN_POINT('Ctrl Pts',(-66.9910096526483,23.1865006796291,0.));
#87661=CARTESIAN_POINT('Ctrl Pts',(-66.9910096526483,23.1865006796291,12.));
#87662=CARTESIAN_POINT('Ctrl Pts',(-67.0127471962507,23.1871433953795,0.));
#87663=CARTESIAN_POINT('Ctrl Pts',(-67.0127471962507,23.1871433953795,12.));
#87664=CARTESIAN_POINT('Ctrl Pts',(-67.0345332582297,23.1877651868155,0.));
#87665=CARTESIAN_POINT('Ctrl Pts',(-67.0345332582297,23.1877651868155,12.));
#87666=CARTESIAN_POINT('Ctrl Pts',(-67.0563676896312,23.1883659754267,0.));
#87667=CARTESIAN_POINT('Ctrl Pts',(-67.0563676896312,23.1883659754267,12.));
#87668=CARTESIAN_POINT('Ctrl Pts',(-67.0782503422293,23.1889456832115,0.));
#87669=CARTESIAN_POINT('Ctrl Pts',(-67.0782503422293,23.1889456832115,12.));
#87670=CARTESIAN_POINT('Ctrl Pts',(-67.1001810685138,23.1895042326625,0.));
#87671=CARTESIAN_POINT('Ctrl Pts',(-67.1001810685138,23.1895042326625,12.));
#87672=CARTESIAN_POINT('Ctrl Pts',(-67.122159721674,23.1900415467574,0.));
#87673=CARTESIAN_POINT('Ctrl Pts',(-67.122159721674,23.1900415467574,12.));
#87674=CARTESIAN_POINT('Ctrl Pts',(-67.1441861555819,23.1905575489505,0.));
#87675=CARTESIAN_POINT('Ctrl Pts',(-67.1441861555819,23.1905575489505,12.));
#87676=CARTESIAN_POINT('Ctrl Pts',(-67.1662602247641,23.1910521631658,0.));
#87677=CARTESIAN_POINT('Ctrl Pts',(-67.1662602247641,23.1910521631658,12.));
#87678=CARTESIAN_POINT('Ctrl Pts',(-67.1883817844039,23.1915253137923,0.));
#87679=CARTESIAN_POINT('Ctrl Pts',(-67.1883817844039,23.1915253137923,12.));
#87680=CARTESIAN_POINT('Ctrl Pts',(-67.2105506903448,23.1919769256803,0.));
#87681=CARTESIAN_POINT('Ctrl Pts',(-67.2105506903448,23.1919769256803,12.));
#87682=CARTESIAN_POINT('Ctrl Pts',(-67.232766799088,23.1924069241385,0.));
#87683=CARTESIAN_POINT('Ctrl Pts',(-67.232766799088,23.1924069241385,12.));
#87684=CARTESIAN_POINT('Ctrl Pts',(-67.2550299677888,23.1928152349343,0.));
#87685=CARTESIAN_POINT('Ctrl Pts',(-67.2550299677888,23.1928152349343,12.));
#87686=CARTESIAN_POINT('Ctrl Pts',(-67.2773400542477,23.1932017842954,0.));
#87687=CARTESIAN_POINT('Ctrl Pts',(-67.2773400542477,23.1932017842954,12.));
#87688=CARTESIAN_POINT('Ctrl Pts',(-67.2996969169099,23.193566498902,0.));
#87689=CARTESIAN_POINT('Ctrl Pts',(-67.2996969169099,23.193566498902,12.));
#87690=CARTESIAN_POINT('Ctrl Pts',(-67.3221004148604,23.1939093058802,0.));
#87691=CARTESIAN_POINT('Ctrl Pts',(-67.3221004148604,23.1939093058802,12.));
#87692=CARTESIAN_POINT('Ctrl Pts',(-67.3445504078178,23.1942301327979,0.));
#87693=CARTESIAN_POINT('Ctrl Pts',(-67.3445504078178,23.1942301327979,12.));
#87694=CARTESIAN_POINT('Ctrl Pts',(-67.3670467561205,23.1945289076608,0.));
#87695=CARTESIAN_POINT('Ctrl Pts',(-67.3670467561205,23.1945289076608,12.));
#87696=CARTESIAN_POINT('Ctrl Pts',(-67.3895893207168,23.1948055589123,0.));
#87697=CARTESIAN_POINT('Ctrl Pts',(-67.3895893207168,23.1948055589123,12.));
#87698=CARTESIAN_POINT('Ctrl Pts',(-67.4121779631666,23.1950600154259,0.));
#87699=CARTESIAN_POINT('Ctrl Pts',(-67.4121779631666,23.1950600154259,12.));
#87700=CARTESIAN_POINT('Ctrl Pts',(-67.4348125456389,23.1952922065009,0.));
#87701=CARTESIAN_POINT('Ctrl Pts',(-67.4348125456389,23.1952922065009,12.));
#87702=CARTESIAN_POINT('Ctrl Pts',(-67.4574929309079,23.1955020618591,0.));
#87703=CARTESIAN_POINT('Ctrl Pts',(-67.4574929309079,23.1955020618591,12.));
#87704=CARTESIAN_POINT('Ctrl Pts',(-67.4802189823424,23.1956895116446,0.));
#87705=CARTESIAN_POINT('Ctrl Pts',(-67.4802189823424,23.1956895116446,12.));
#87706=CARTESIAN_POINT('Ctrl Pts',(-67.5029905638974,23.1958544864224,0.));
#87707=CARTESIAN_POINT('Ctrl Pts',(-67.5029905638974,23.1958544864224,12.));
#87708=CARTESIAN_POINT('Ctrl Pts',(-67.525807540117,23.1959969171709,0.));
#87709=CARTESIAN_POINT('Ctrl Pts',(-67.525807540117,23.1959969171709,12.));
#87710=CARTESIAN_POINT('Ctrl Pts',(-67.5486697761301,23.1961167352776,0.));
#87711=CARTESIAN_POINT('Ctrl Pts',(-67.5486697761301,23.1961167352776,12.));
#87712=CARTESIAN_POINT('Ctrl Pts',(-67.5715771376454,23.1962138725358,0.));
#87713=CARTESIAN_POINT('Ctrl Pts',(-67.5715771376454,23.1962138725358,12.));
#87714=CARTESIAN_POINT('Ctrl Pts',(-67.5945294909398,23.1962882611443,0.));
#87715=CARTESIAN_POINT('Ctrl Pts',(-67.5945294909398,23.1962882611443,12.));
#87716=CARTESIAN_POINT('Ctrl Pts',(-67.6175267028517,23.1963398337056,0.));
#87717=CARTESIAN_POINT('Ctrl Pts',(-67.6175267028517,23.1963398337056,12.));
#87718=CARTESIAN_POINT('Ctrl Pts',(-67.6405686407828,23.1963685232176,0.));
#87719=CARTESIAN_POINT('Ctrl Pts',(-67.6405686407828,23.1963685232176,12.));
#87720=CARTESIAN_POINT('Ctrl Pts',(-67.6636551726948,23.1963742630709,0.));
#87721=CARTESIAN_POINT('Ctrl Pts',(-67.6636551726948,23.1963742630709,12.));
#87722=CARTESIAN_POINT('Ctrl Pts',(-67.6867861671045,23.1963569870456,0.));
#87723=CARTESIAN_POINT('Ctrl Pts',(-67.6867861671045,23.1963569870456,12.));
#87724=CARTESIAN_POINT('Ctrl Pts',(-67.7099614930712,23.1963166293116,0.));
#87725=CARTESIAN_POINT('Ctrl Pts',(-67.7099614930712,23.1963166293116,12.));
#87726=CARTESIAN_POINT('Ctrl Pts',(-67.7331810201931,23.1962531244261,0.));
#87727=CARTESIAN_POINT('Ctrl Pts',(-67.7331810201931,23.1962531244261,12.));
#87728=CARTESIAN_POINT('Ctrl Pts',(-67.7564446186115,23.1961664073273,0.));
#87729=CARTESIAN_POINT('Ctrl Pts',(-67.7564446186115,23.1961664073273,12.));
#87730=CARTESIAN_POINT('Ctrl Pts',(-67.7797521590056,23.1960564133308,0.));
#87731=CARTESIAN_POINT('Ctrl Pts',(-67.7797521590056,23.1960564133308,12.));
#87732=CARTESIAN_POINT('Ctrl Pts',(-67.8031035125873,23.1959230781265,0.));
#87733=CARTESIAN_POINT('Ctrl Pts',(-67.8031035125873,23.1959230781265,12.));
#87734=CARTESIAN_POINT('Ctrl Pts',(-67.8264985510885,23.1957663377797,0.));
#87735=CARTESIAN_POINT('Ctrl Pts',(-67.8264985510885,23.1957663377797,12.));
#87736=CARTESIAN_POINT('Ctrl Pts',(-67.8499371467578,23.1955861287275,0.));
#87737=CARTESIAN_POINT('Ctrl Pts',(-67.8499371467578,23.1955861287275,12.));
#87738=CARTESIAN_POINT('Ctrl Pts',(-67.8734191723639,23.1953823877726,0.));
#87739=CARTESIAN_POINT('Ctrl Pts',(-67.8734191723639,23.1953823877726,12.));
#87740=CARTESIAN_POINT('Ctrl Pts',(-67.8969445011908,23.19515505208,0.));
#87741=CARTESIAN_POINT('Ctrl Pts',(-67.8969445011908,23.19515505208,12.));
#87742=CARTESIAN_POINT('Ctrl Pts',(-67.9205130070337,23.1949040591748,0.));
#87743=CARTESIAN_POINT('Ctrl Pts',(-67.9205130070337,23.1949040591748,12.));
#87744=CARTESIAN_POINT('Ctrl Pts',(-67.9441245641871,23.1946293469436,0.));
#87745=CARTESIAN_POINT('Ctrl Pts',(-67.9441245641871,23.1946293469436,12.));
#87746=CARTESIAN_POINT('Ctrl Pts',(-67.9677790474414,23.1943308536307,0.));
#87747=CARTESIAN_POINT('Ctrl Pts',(-67.9677790474414,23.1943308536307,12.));
#87748=CARTESIAN_POINT('Ctrl Pts',(-67.9914763320878,23.1940085178319,0.));
#87749=CARTESIAN_POINT('Ctrl Pts',(-67.9914763320878,23.1940085178319,12.));
#87750=CARTESIAN_POINT('Ctrl Pts',(-68.0152162939123,23.193662278492,0.));
#87751=CARTESIAN_POINT('Ctrl Pts',(-68.0152162939123,23.193662278492,12.));
#87752=CARTESIAN_POINT('Ctrl Pts',(-68.0389988091926,23.1932920749021,0.));
#87753=CARTESIAN_POINT('Ctrl Pts',(-68.0389988091926,23.1932920749021,12.));
#87754=CARTESIAN_POINT('Ctrl Pts',(-68.0628237546853,23.1928978467017,0.));
#87755=CARTESIAN_POINT('Ctrl Pts',(-68.0628237546853,23.1928978467017,12.));
#87756=CARTESIAN_POINT('Ctrl Pts',(-68.0866910076241,23.1924795338745,0.));
#87757=CARTESIAN_POINT('Ctrl Pts',(-68.0866910076241,23.1924795338745,12.));
#87758=CARTESIAN_POINT('Ctrl Pts',(-68.1106004457223,23.1920370767423,0.));
#87759=CARTESIAN_POINT('Ctrl Pts',(-68.1106004457223,23.1920370767423,12.));
#87760=CARTESIAN_POINT('Ctrl Pts',(-68.1345519471695,23.1915704159623,0.));
#87761=CARTESIAN_POINT('Ctrl Pts',(-68.1345519471695,23.1915704159623,12.));
#87762=CARTESIAN_POINT('Ctrl Pts',(-68.1585453906259,23.1910794925252,0.));
#87763=CARTESIAN_POINT('Ctrl Pts',(-68.1585453906259,23.1910794925252,12.));
#87764=CARTESIAN_POINT('Ctrl Pts',(-68.182580655213,23.1905642477571,0.));
#87765=CARTESIAN_POINT('Ctrl Pts',(-68.182580655213,23.1905642477571,12.));
#87766=CARTESIAN_POINT('Ctrl Pts',(-68.2066576205113,23.1900246233164,0.));
#87767=CARTESIAN_POINT('Ctrl Pts',(-68.2066576205113,23.1900246233164,12.));
#87768=CARTESIAN_POINT('Ctrl Pts',(-68.2307761665629,23.1894605611869,0.));
#87769=CARTESIAN_POINT('Ctrl Pts',(-68.2307761665629,23.1894605611869,12.));
#87770=CARTESIAN_POINT('Ctrl Pts',(-68.2549361738679,23.1888720036756,0.));
#87771=CARTESIAN_POINT('Ctrl Pts',(-68.2549361738679,23.1888720036756,12.));
#87772=CARTESIAN_POINT('Ctrl Pts',(-68.2791375233798,23.1882588934108,0.));
#87773=CARTESIAN_POINT('Ctrl Pts',(-68.2791375233798,23.1882588934108,12.));
#87774=CARTESIAN_POINT('Ctrl Pts',(-68.3033800964946,23.1876211733439,0.));
#87775=CARTESIAN_POINT('Ctrl Pts',(-68.3033800964946,23.1876211733439,12.));
#87776=CARTESIAN_POINT('Ctrl Pts',(-68.3276637750494,23.1869587867463,0.));
#87777=CARTESIAN_POINT('Ctrl Pts',(-68.3276637750494,23.1869587867463,12.));
#87778=CARTESIAN_POINT('Ctrl Pts',(-68.3519884413253,23.1862716772034,0.));
#87779=CARTESIAN_POINT('Ctrl Pts',(-68.3519884413253,23.1862716772034,12.));
#87780=CARTESIAN_POINT('Ctrl Pts',(-68.3763539780442,23.1855597886117,0.));
#87781=CARTESIAN_POINT('Ctrl Pts',(-68.3763539780442,23.1855597886117,12.));
#87782=CARTESIAN_POINT('Ctrl Pts',(-68.4007602683649,23.1848230651775,0.));
#87783=CARTESIAN_POINT('Ctrl Pts',(-68.4007602683649,23.1848230651775,12.));
#87784=CARTESIAN_POINT('Ctrl Pts',(-68.4252071958725,23.184061451419,0.));
#87785=CARTESIAN_POINT('Ctrl Pts',(-68.4252071958725,23.184061451419,12.));
#87786=CARTESIAN_POINT('Ctrl Pts',(-68.4496946445756,23.1832748921629,0.));
#87787=CARTESIAN_POINT('Ctrl Pts',(-68.4496946445756,23.1832748921629,12.));
#87788=CARTESIAN_POINT('Ctrl Pts',(-68.4742224989099,23.1824633325384,0.));
#87789=CARTESIAN_POINT('Ctrl Pts',(-68.4742224989099,23.1824633325384,12.));
#87790=CARTESIAN_POINT('Ctrl Pts',(-68.4987906437357,23.1816267179751,0.));
#87791=CARTESIAN_POINT('Ctrl Pts',(-68.4987906437357,23.1816267179751,12.));
#87792=CARTESIAN_POINT('Ctrl Pts',(-68.5233989643344,23.180764994201,0.));
#87793=CARTESIAN_POINT('Ctrl Pts',(-68.5233989643344,23.180764994201,12.));
#87794=CARTESIAN_POINT('Ctrl Pts',(-68.548047346398,23.1798781072449,0.));
#87795=CARTESIAN_POINT('Ctrl Pts',(-68.548047346398,23.1798781072449,12.));
#87796=CARTESIAN_POINT('Ctrl Pts',(-68.572735676027,23.1789660034339,0.));
#87797=CARTESIAN_POINT('Ctrl Pts',(-68.572735676027,23.1789660034339,12.));
#87798=CARTESIAN_POINT('Ctrl Pts',(-68.5974638397322,23.1780286293873,0.));
#87799=CARTESIAN_POINT('Ctrl Pts',(-68.5974638397322,23.1780286293873,12.));
#87800=CARTESIAN_POINT('Ctrl Pts',(-68.6222317244337,23.1770659320136,0.));
#87801=CARTESIAN_POINT('Ctrl Pts',(-68.6222317244337,23.1770659320136,12.));
#87802=CARTESIAN_POINT('Ctrl Pts',(-68.6470392174567,23.1760778585093,0.));
#87803=CARTESIAN_POINT('Ctrl Pts',(-68.6470392174567,23.1760778585093,12.));
#87804=CARTESIAN_POINT('Ctrl Pts',(-68.6718862065227,23.1750643563605,0.));
#87805=CARTESIAN_POINT('Ctrl Pts',(-68.6718862065227,23.1750643563605,12.));
#87806=CARTESIAN_POINT('Ctrl Pts',(-68.6967725797458,23.1740253733423,0.));
#87807=CARTESIAN_POINT('Ctrl Pts',(-68.6967725797458,23.1740253733423,12.));
#87808=CARTESIAN_POINT('Ctrl Pts',(-68.7216982256357,23.1729608575115,0.));
#87809=CARTESIAN_POINT('Ctrl Pts',(-68.7216982256357,23.1729608575115,12.));
#87810=CARTESIAN_POINT('Ctrl Pts',(-68.7466630330968,23.1718707572046,0.));
#87811=CARTESIAN_POINT('Ctrl Pts',(-68.7466630330968,23.1718707572046,12.));
#87812=CARTESIAN_POINT('Ctrl Pts',(-68.7716668914246,23.1707550210359,0.));
#87813=CARTESIAN_POINT('Ctrl Pts',(-68.7716668914246,23.1707550210359,12.));
#87814=CARTESIAN_POINT('Ctrl Pts',(-68.7967096902981,23.1696135978992,0.));
#87815=CARTESIAN_POINT('Ctrl Pts',(-68.7967096902981,23.1696135978992,12.));
#87816=CARTESIAN_POINT('Ctrl Pts',(-68.8217913197735,23.1684464369681,0.));
#87817=CARTESIAN_POINT('Ctrl Pts',(-68.8217913197735,23.1684464369681,12.));
#87818=CARTESIAN_POINT('Ctrl Pts',(-68.8469116702885,23.1672534876885,0.));
#87819=CARTESIAN_POINT('Ctrl Pts',(-68.8469116702885,23.1672534876885,12.));
#87820=CARTESIAN_POINT('Ctrl Pts',(-68.8720706326606,23.1660346997762,0.));
#87821=CARTESIAN_POINT('Ctrl Pts',(-68.8720706326606,23.1660346997762,12.));
#87822=CARTESIAN_POINT('Ctrl Pts',(-68.8972680980844,23.1647900232151,0.));
#87823=CARTESIAN_POINT('Ctrl Pts',(-68.8972680980844,23.1647900232151,12.));
#87824=CARTESIAN_POINT('Ctrl Pts',(-68.9225039581249,23.1635194082581,0.));
#87825=CARTESIAN_POINT('Ctrl Pts',(-68.9225039581249,23.1635194082581,12.));
#87826=CARTESIAN_POINT('Ctrl Pts',(-68.9477781047103,23.162222805429,0.));
#87827=CARTESIAN_POINT('Ctrl Pts',(-68.9477781047103,23.162222805429,12.));
#87828=CARTESIAN_POINT('Ctrl Pts',(-68.9730904301363,23.1609001655153,0.));
#87829=CARTESIAN_POINT('Ctrl Pts',(-68.9730904301363,23.1609001655153,12.));
#87830=CARTESIAN_POINT('Ctrl Pts',(-68.9984408270653,23.1595514395654,0.));
#87831=CARTESIAN_POINT('Ctrl Pts',(-68.9984408270653,23.1595514395654,12.));
#87832=CARTESIAN_POINT('Ctrl Pts',(-69.0238291885245,23.1581765788869,0.));
#87833=CARTESIAN_POINT('Ctrl Pts',(-69.0238291885245,23.1581765788869,12.));
#87834=CARTESIAN_POINT('Ctrl Pts',(-69.0492554078999,23.1567755350472,0.));
#87835=CARTESIAN_POINT('Ctrl Pts',(-69.0492554078999,23.1567755350472,12.));
#87836=CARTESIAN_POINT('Ctrl Pts',(-69.0747193789292,23.1553482598767,0.));
#87837=CARTESIAN_POINT('Ctrl Pts',(-69.0747193789292,23.1553482598767,12.));
#87838=CARTESIAN_POINT('Ctrl Pts',(-69.1002209957037,23.1538947054619,0.));
#87839=CARTESIAN_POINT('Ctrl Pts',(-69.1002209957037,23.1538947054619,12.));
#87840=CARTESIAN_POINT('Ctrl Pts',(-69.1257601526693,23.1524148241413,0.));
#87841=CARTESIAN_POINT('Ctrl Pts',(-69.1257601526693,23.1524148241413,12.));
#87842=CARTESIAN_POINT('Ctrl Pts',(-69.1513367446231,23.1509085685032,0.));
#87843=CARTESIAN_POINT('Ctrl Pts',(-69.1513367446231,23.1509085685032,12.));
#87844=CARTESIAN_POINT('Ctrl Pts',(-69.176950666708,23.1493758913857,0.));
#87845=CARTESIAN_POINT('Ctrl Pts',(-69.176950666708,23.1493758913857,12.));
#87846=CARTESIAN_POINT('Ctrl Pts',(-69.2026018144023,23.1478167458787,0.));
#87847=CARTESIAN_POINT('Ctrl Pts',(-69.2026018144023,23.1478167458787,12.));
#87848=CARTESIAN_POINT('Ctrl Pts',(-69.2282900835234,23.1462310853205,0.));
#87849=CARTESIAN_POINT('Ctrl Pts',(-69.2282900835234,23.1462310853205,12.));
#87850=CARTESIAN_POINT('Ctrl Pts',(-69.2540153702311,23.1446188632931,0.));
#87851=CARTESIAN_POINT('Ctrl Pts',(-69.2540153702311,23.1446188632931,12.));
#87852=CARTESIAN_POINT('Ctrl Pts',(-69.2797775710275,23.142980033622,0.));
#87853=CARTESIAN_POINT('Ctrl Pts',(-69.2797775710275,23.142980033622,12.));
#87854=CARTESIAN_POINT('Ctrl Pts',(-69.3055765827544,23.1413145503762,0.));
#87855=CARTESIAN_POINT('Ctrl Pts',(-69.3055765827544,23.1413145503762,12.));
#87856=CARTESIAN_POINT('Ctrl Pts',(-69.3314123025863,23.1396223678725,0.));
#87857=CARTESIAN_POINT('Ctrl Pts',(-69.3314123025863,23.1396223678725,12.));
#87858=CARTESIAN_POINT('Ctrl Pts',(-69.3572846280289,23.1379034406717,0.));
#87859=CARTESIAN_POINT('Ctrl Pts',(-69.3572846280289,23.1379034406717,12.));
#87860=CARTESIAN_POINT('Ctrl Pts',(-69.3831934569176,23.1361577235708,0.));
#87861=CARTESIAN_POINT('Ctrl Pts',(-69.3831934569176,23.1361577235708,12.));
#87862=CARTESIAN_POINT('Ctrl Pts',(-69.4091386874129,23.1343851715988,0.));
#87863=CARTESIAN_POINT('Ctrl Pts',(-69.4091386874129,23.1343851715988,12.));
#87864=CARTESIAN_POINT('Ctrl Pts',(-69.4351202179948,23.1325857400145,0.));
#87865=CARTESIAN_POINT('Ctrl Pts',(-69.4351202179948,23.1325857400145,12.));
#87866=CARTESIAN_POINT('Ctrl Pts',(-69.4611379474492,23.1307593843063,0.));
#87867=CARTESIAN_POINT('Ctrl Pts',(-69.4611379474492,23.1307593843063,12.));
#87868=CARTESIAN_POINT('Ctrl Pts',(-69.4871917748665,23.1289060601927,0.));
#87869=CARTESIAN_POINT('Ctrl Pts',(-69.4871917748665,23.1289060601927,12.));
#87870=CARTESIAN_POINT('Ctrl Pts',(-69.5132815996548,23.1270257236207,0.));
#87871=CARTESIAN_POINT('Ctrl Pts',(-69.5132815996548,23.1270257236207,12.));
#87872=CARTESIAN_POINT('Ctrl Pts',(-69.5394073215467,23.1251183307678,0.));
#87873=CARTESIAN_POINT('Ctrl Pts',(-69.5394073215467,23.1251183307678,12.));
#87874=CARTESIAN_POINT('Ctrl Pts',(-69.565568840605,23.1231838380452,0.));
#87875=CARTESIAN_POINT('Ctrl Pts',(-69.565568840605,23.1231838380452,12.));
#87876=CARTESIAN_POINT('Ctrl Pts',(-69.5917660572255,23.1212222021049,0.));
#87877=CARTESIAN_POINT('Ctrl Pts',(-69.5917660572255,23.1212222021049,12.));
#87878=CARTESIAN_POINT('Ctrl Pts',(-69.617998872135,23.1192333798437,0.));
#87879=CARTESIAN_POINT('Ctrl Pts',(-69.617998872135,23.1192333798437,12.));
#87880=CARTESIAN_POINT('Ctrl Pts',(-69.6442671863751,23.1172173283855,0.));
#87881=CARTESIAN_POINT('Ctrl Pts',(-69.6442671863751,23.1172173283855,12.));
#87882=CARTESIAN_POINT('Ctrl Pts',(-69.6705709012842,23.1151740050678,0.));
#87883=CARTESIAN_POINT('Ctrl Pts',(-69.6705709012842,23.1151740050678,12.));
#87884=CARTESIAN_POINT('Ctrl Pts',(-69.6969099184766,23.1131033674301,0.));
#87885=CARTESIAN_POINT('Ctrl Pts',(-69.6969099184766,23.1131033674301,12.));
#87886=CARTESIAN_POINT('Ctrl Pts',(-69.7232841398207,23.1110053732049,0.));
#87887=CARTESIAN_POINT('Ctrl Pts',(-69.7232841398207,23.1110053732049,12.));
#87888=CARTESIAN_POINT('Ctrl Pts',(-69.7496934674083,23.1088799803093,0.));
#87889=CARTESIAN_POINT('Ctrl Pts',(-69.7496934674083,23.1088799803093,12.));
#87890=CARTESIAN_POINT('Ctrl Pts',(-69.7761378035979,23.1067271468614,0.));
#87891=CARTESIAN_POINT('Ctrl Pts',(-69.7761378035979,23.1067271468614,12.));
#87892=CARTESIAN_POINT('Ctrl Pts',(-69.8026170510582,23.1045468311994,0.));
#87893=CARTESIAN_POINT('Ctrl Pts',(-69.8026170510582,23.1045468311994,12.));
#87894=CARTESIAN_POINT('Ctrl Pts',(-69.8291311128121,23.1023389919052,0.));
#87895=CARTESIAN_POINT('Ctrl Pts',(-69.8291311128121,23.1023389919052,12.));
#87896=CARTESIAN_POINT('Ctrl Pts',(-69.8556798922688,23.100103587824,0.));
#87897=CARTESIAN_POINT('Ctrl Pts',(-69.8556798922688,23.100103587824,12.));
#87898=CARTESIAN_POINT('Ctrl Pts',(-69.882263293276,23.0978405781018,0.));
#87899=CARTESIAN_POINT('Ctrl Pts',(-69.882263293276,23.0978405781018,12.));
#87900=CARTESIAN_POINT('Ctrl Pts',(-69.9088812200704,23.0955499221556,0.));
#87901=CARTESIAN_POINT('Ctrl Pts',(-69.9088812200704,23.0955499221556,12.));
#87902=CARTESIAN_POINT('Ctrl Pts',(-69.9355335771722,23.0932315796066,0.));
#87903=CARTESIAN_POINT('Ctrl Pts',(-69.9355335771722,23.0932315796066,12.));
#87904=CARTESIAN_POINT('Ctrl Pts',(-69.9622202692871,23.090885510225,0.));
#87905=CARTESIAN_POINT('Ctrl Pts',(-69.9622202692871,23.090885510225,12.));
#87906=CARTESIAN_POINT('Ctrl Pts',(-69.9889412012143,23.0885116738798,0.));
#87907=CARTESIAN_POINT('Ctrl Pts',(-69.9889412012143,23.0885116738798,12.));
#87908=CARTESIAN_POINT('Ctrl Pts',(-70.0156962777173,23.0861100304731,0.));
#87909=CARTESIAN_POINT('Ctrl Pts',(-70.0156962777173,23.0861100304731,12.));
#87910=CARTESIAN_POINT('Ctrl Pts',(-70.0424854035125,23.0836805399377,0.));
#87911=CARTESIAN_POINT('Ctrl Pts',(-70.0424854035125,23.0836805399377,12.));
#87912=CARTESIAN_POINT('Ctrl Pts',(-70.0693084835388,23.081223162377,0.));
#87913=CARTESIAN_POINT('Ctrl Pts',(-70.0693084835388,23.081223162377,12.));
#87914=CARTESIAN_POINT('Ctrl Pts',(-70.096165423165,23.0787378581778,0.));
#87915=CARTESIAN_POINT('Ctrl Pts',(-70.096165423165,23.0787378581778,12.));
#87916=CARTESIAN_POINT('Ctrl Pts',(-70.1230561284222,23.076224588139,0.));
#87917=CARTESIAN_POINT('Ctrl Pts',(-70.1230561284222,23.076224588139,12.));
#87918=CARTESIAN_POINT('Ctrl Pts',(-70.1499805062159,23.0736833135934,0.));
#87919=CARTESIAN_POINT('Ctrl Pts',(-70.1499805062159,23.0736833135934,12.));
#87920=CARTESIAN_POINT('Ctrl Pts',(-70.176938464556,23.0711139965432,0.));
#87921=CARTESIAN_POINT('Ctrl Pts',(-70.176938464556,23.0711139965432,12.));
#87922=CARTESIAN_POINT('Ctrl Pts',(-70.2039299120456,23.0685165993681,0.));
#87923=CARTESIAN_POINT('Ctrl Pts',(-70.2039299120456,23.0685165993681,12.));
#87924=CARTESIAN_POINT('Ctrl Pts',(-70.2309547573789,23.0658910845425,0.));
#87925=CARTESIAN_POINT('Ctrl Pts',(-70.2309547573789,23.0658910845425,12.));
#87926=CARTESIAN_POINT('Ctrl Pts',(-70.2580129087878,23.0632374143276,0.));
#87927=CARTESIAN_POINT('Ctrl Pts',(-70.2580129087878,23.0632374143276,12.));
#87928=CARTESIAN_POINT('Ctrl Pts',(-70.2851042736081,23.0605555505326,0.));
#87929=CARTESIAN_POINT('Ctrl Pts',(-70.2851042736081,23.0605555505326,12.));
#87930=CARTESIAN_POINT('Ctrl Pts',(-70.3122287575374,23.0578454541116,0.));
#87931=CARTESIAN_POINT('Ctrl Pts',(-70.3122287575374,23.0578454541116,12.));
#87932=CARTESIAN_POINT('Ctrl Pts',(-70.3393862652353,23.0551070854942,0.));
#87933=CARTESIAN_POINT('Ctrl Pts',(-70.3393862652353,23.0551070854942,12.));
#87934=CARTESIAN_POINT('Ctrl Pts',(-70.3665767016596,23.0523404053188,0.));
#87935=CARTESIAN_POINT('Ctrl Pts',(-70.3665767016596,23.0523404053188,12.));
#87936=CARTESIAN_POINT('Ctrl Pts',(-70.39379997323,23.0495453750773,0.));
#87937=CARTESIAN_POINT('Ctrl Pts',(-70.39379997323,23.0495453750773,12.));
#87938=CARTESIAN_POINT('Ctrl Pts',(-70.421055988934,23.0467219577288,0.));
#87939=CARTESIAN_POINT('Ctrl Pts',(-70.421055988934,23.0467219577288,12.));
#87940=CARTESIAN_POINT('Ctrl Pts',(-70.4483446617553,23.0438701184995,0.));
#87941=CARTESIAN_POINT('Ctrl Pts',(-70.4483446617553,23.0438701184995,12.));
#87942=CARTESIAN_POINT('Ctrl Pts',(-70.4756659090104,23.0409898250726,0.));
#87943=CARTESIAN_POINT('Ctrl Pts',(-70.4756659090104,23.0409898250726,12.));
#87944=CARTESIAN_POINT('Ctrl Pts',(-70.5030196491883,23.0380810458237,0.));
#87945=CARTESIAN_POINT('Ctrl Pts',(-70.5030196491883,23.0380810458237,12.));
#87946=CARTESIAN_POINT('Ctrl Pts',(-70.5304057994537,23.0351437484309,0.));
#87947=CARTESIAN_POINT('Ctrl Pts',(-70.5304057994537,23.0351437484309,12.));
#87948=CARTESIAN_POINT('Ctrl Pts',(-70.5578242727606,23.0321778982705,0.));
#87949=CARTESIAN_POINT('Ctrl Pts',(-70.5578242727606,23.0321778982705,12.));
#87950=CARTESIAN_POINT('Ctrl Pts',(-70.5852749754168,23.0291834570688,0.));
#87951=CARTESIAN_POINT('Ctrl Pts',(-70.5852749754168,23.0291834570688,12.));
#87952=CARTESIAN_POINT('Ctrl Pts',(-70.6127578036869,23.0261603810187,0.));
#87953=CARTESIAN_POINT('Ctrl Pts',(-70.6127578036869,23.0261603810187,12.));
#87954=CARTESIAN_POINT('Ctrl Pts',(-70.6402726486718,23.0231086235262,0.));
#87955=CARTESIAN_POINT('Ctrl Pts',(-70.6402726486718,23.0231086235262,12.));
#87956=CARTESIAN_POINT('Ctrl Pts',(-70.6678194023389,23.0200281385906,0.));
#87957=CARTESIAN_POINT('Ctrl Pts',(-70.6678194023389,23.0200281385906,12.));
#87958=CARTESIAN_POINT('Ctrl Pts',(-70.6953979633561,23.0169188841083,0.));
#87959=CARTESIAN_POINT('Ctrl Pts',(-70.6953979633561,23.0169188841083,12.));
#87960=CARTESIAN_POINT('Ctrl Pts',(-70.7230082425324,23.0137808248898,0.));
#87961=CARTESIAN_POINT('Ctrl Pts',(-70.7230082425324,23.0137808248898,12.));
#87962=CARTESIAN_POINT('Ctrl Pts',(-70.7506501695822,23.0106139365941,0.));
#87963=CARTESIAN_POINT('Ctrl Pts',(-70.7506501695822,23.0106139365941,12.));
#87964=CARTESIAN_POINT('Ctrl Pts',(-70.7783236950588,23.007418206361,0.));
#87965=CARTESIAN_POINT('Ctrl Pts',(-70.7783236950588,23.007418206361,12.));
#87966=CARTESIAN_POINT('Ctrl Pts',(-70.806028785987,23.004193629142,0.));
#87967=CARTESIAN_POINT('Ctrl Pts',(-70.806028785987,23.004193629142,12.));
#87968=CARTESIAN_POINT('Ctrl Pts',(-70.8282180956627,23.0015908899222,0.));
#87969=CARTESIAN_POINT('Ctrl Pts',(-70.8282180956627,23.0015908899222,12.));
#87970=CARTESIAN_POINT('Ctrl Pts',(-70.8448742696329,22.9996258555187,0.));
#87971=CARTESIAN_POINT('Ctrl Pts',(-70.8448742696329,22.9996258555187,12.));
#87972=CARTESIAN_POINT('Ctrl Pts',(-70.8559846927868,22.9983100639353,0.));
#87973=CARTESIAN_POINT('Ctrl Pts',(-70.8559846927868,22.9983100639353,12.));
#87974=CARTESIAN_POINT('Ctrl Pts',(-70.8615414811572,22.9976507259816,0.));
#87975=CARTESIAN_POINT('Ctrl Pts',(-70.8615414811572,22.9976507259816,12.));
#87976=CARTESIAN_POINT('',(-66.0656156664138,23.1372951448024,0.));
#87977=CARTESIAN_POINT('Ctrl Pts',(-66.0656156664138,23.1372951448024,0.));
#87978=CARTESIAN_POINT('Ctrl Pts',(-66.0694876382127,23.1375957166104,0.));
#87979=CARTESIAN_POINT('Ctrl Pts',(-66.0772371487248,23.13819515974,0.));
#87980=CARTESIAN_POINT('Ctrl Pts',(-66.0888781152421,23.1390892229778,0.));
#87981=CARTESIAN_POINT('Ctrl Pts',(-66.1044328067355,23.1402711039425,0.));
#87982=CARTESIAN_POINT('Ctrl Pts',(-66.1239318368548,23.1417314398398,0.));
#87983=CARTESIAN_POINT('Ctrl Pts',(-66.1434865015027,23.1431747350098,0.));
#87984=CARTESIAN_POINT('Ctrl Pts',(-66.1630967296747,23.1446009424903,0.));
#87985=CARTESIAN_POINT('Ctrl Pts',(-66.18276239029,23.1460099850763,0.));
#87986=CARTESIAN_POINT('Ctrl Pts',(-66.2024832934866,23.1474017566484,0.));
#87987=CARTESIAN_POINT('Ctrl Pts',(-66.2222592165473,23.1487761349328,0.));
#87988=CARTESIAN_POINT('Ctrl Pts',(-66.2420899237317,23.1501329914488,0.));
#87989=CARTESIAN_POINT('Ctrl Pts',(-66.2619751878741,23.1514722022483,0.));
#87990=CARTESIAN_POINT('Ctrl Pts',(-66.2819148131072,23.1527936592625,0.));
#87991=CARTESIAN_POINT('Ctrl Pts',(-66.301908627539,23.154097266617,0.));
#87992=CARTESIAN_POINT('Ctrl Pts',(-66.3219564725161,23.1553829352531,0.));
#87993=CARTESIAN_POINT('Ctrl Pts',(-66.3420581937159,23.1566505784626,0.));
#87994=CARTESIAN_POINT('Ctrl Pts',(-66.3622136300692,23.1579001063438,0.));
#87995=CARTESIAN_POINT('Ctrl Pts',(-66.382422608185,23.15913142301,0.));
#87996=CARTESIAN_POINT('Ctrl Pts',(-66.402684948127,23.1603444294754,0.));
#87997=CARTESIAN_POINT('Ctrl Pts',(-66.4230004670288,23.1615390254635,0.));
#87998=CARTESIAN_POINT('Ctrl Pts',(-66.4433689832454,23.1627151114875,0.));
#87999=CARTESIAN_POINT('Ctrl Pts',(-66.4637903210682,23.163872591218,0.));
#88000=CARTESIAN_POINT('Ctrl Pts',(-66.4842643105263,23.1650113713792,0.));
#88001=CARTESIAN_POINT('Ctrl Pts',(-66.5047907851319,23.1661313606123,0.));
#88002=CARTESIAN_POINT('Ctrl Pts',(-66.5253695803209,23.1672324686927,0.));
#88003=CARTESIAN_POINT('Ctrl Pts',(-66.5460005315406,23.1683146055736,0.));
#88004=CARTESIAN_POINT('Ctrl Pts',(-66.5666834726495,23.169377680588,0.));
#88005=CARTESIAN_POINT('Ctrl Pts',(-66.5874182367597,23.1704216028626,0.));
#88006=CARTESIAN_POINT('Ctrl Pts',(-66.6082046569657,23.1714462816794,0.));
#88007=CARTESIAN_POINT('Ctrl Pts',(-66.6290425670538,23.1724516268299,0.));
#88008=CARTESIAN_POINT('Ctrl Pts',(-66.6499318023445,23.1734375490421,0.));
#88009=CARTESIAN_POINT('Ctrl Pts',(-66.6708722000047,23.174403960137,0.));
#88010=CARTESIAN_POINT('Ctrl Pts',(-66.691863598595,23.1753507727931,0.));
#88011=CARTESIAN_POINT('Ctrl Pts',(-66.712905837789,23.1762779004043,0.));
#88012=CARTESIAN_POINT('Ctrl Pts',(-66.7339987580441,23.1771852569136,0.));
#88013=CARTESIAN_POINT('Ctrl Pts',(-66.7551422002229,23.1780727566309,0.));
#88014=CARTESIAN_POINT('Ctrl Pts',(-66.7763360056146,23.1789403142375,0.));
#88015=CARTESIAN_POINT('Ctrl Pts',(-66.7975800161014,23.1797878448645,0.));
#88016=CARTESIAN_POINT('Ctrl Pts',(-66.8188740742727,23.1806152641475,0.));
#88017=CARTESIAN_POINT('Ctrl Pts',(-66.840218023555,23.1814224882948,0.));
#88018=CARTESIAN_POINT('Ctrl Pts',(-66.8616117083304,23.1822094341508,0.));
#88019=CARTESIAN_POINT('Ctrl Pts',(-66.8830549738768,23.1829760191582,0.));
#88020=CARTESIAN_POINT('Ctrl Pts',(-66.904547666305,23.1837221613231,0.));
#88021=CARTESIAN_POINT('Ctrl Pts',(-66.9260896324955,23.1844477791816,0.));
#88022=CARTESIAN_POINT('Ctrl Pts',(-66.9476807200225,23.1851527917665,0.));
#88023=CARTESIAN_POINT('Ctrl Pts',(-66.9693207771059,23.1858371185852,0.));
#88024=CARTESIAN_POINT('Ctrl Pts',(-66.9910096526483,23.1865006796291,0.));
#88025=CARTESIAN_POINT('Ctrl Pts',(-67.0127471962507,23.1871433953795,0.));
#88026=CARTESIAN_POINT('Ctrl Pts',(-67.0345332582297,23.1877651868155,0.));
#88027=CARTESIAN_POINT('Ctrl Pts',(-67.0563676896312,23.1883659754267,0.));
#88028=CARTESIAN_POINT('Ctrl Pts',(-67.0782503422293,23.1889456832115,0.));
#88029=CARTESIAN_POINT('Ctrl Pts',(-67.1001810685138,23.1895042326625,0.));
#88030=CARTESIAN_POINT('Ctrl Pts',(-67.122159721674,23.1900415467574,0.));
#88031=CARTESIAN_POINT('Ctrl Pts',(-67.1441861555819,23.1905575489505,0.));
#88032=CARTESIAN_POINT('Ctrl Pts',(-67.1662602247641,23.1910521631658,0.));
#88033=CARTESIAN_POINT('Ctrl Pts',(-67.1883817844039,23.1915253137923,0.));
#88034=CARTESIAN_POINT('Ctrl Pts',(-67.2105506903448,23.1919769256803,0.));
#88035=CARTESIAN_POINT('Ctrl Pts',(-67.232766799088,23.1924069241385,0.));
#88036=CARTESIAN_POINT('Ctrl Pts',(-67.2550299677888,23.1928152349343,0.));
#88037=CARTESIAN_POINT('Ctrl Pts',(-67.2773400542477,23.1932017842954,0.));
#88038=CARTESIAN_POINT('Ctrl Pts',(-67.2996969169099,23.193566498902,0.));
#88039=CARTESIAN_POINT('Ctrl Pts',(-67.3221004148604,23.1939093058802,0.));
#88040=CARTESIAN_POINT('Ctrl Pts',(-67.3445504078178,23.1942301327979,0.));
#88041=CARTESIAN_POINT('Ctrl Pts',(-67.3670467561205,23.1945289076608,0.));
#88042=CARTESIAN_POINT('Ctrl Pts',(-67.3895893207168,23.1948055589123,0.));
#88043=CARTESIAN_POINT('Ctrl Pts',(-67.4121779631666,23.1950600154259,0.));
#88044=CARTESIAN_POINT('Ctrl Pts',(-67.4348125456389,23.1952922065009,0.));
#88045=CARTESIAN_POINT('Ctrl Pts',(-67.4574929309079,23.1955020618591,0.));
#88046=CARTESIAN_POINT('Ctrl Pts',(-67.4802189823424,23.1956895116446,0.));
#88047=CARTESIAN_POINT('Ctrl Pts',(-67.5029905638974,23.1958544864224,0.));
#88048=CARTESIAN_POINT('Ctrl Pts',(-67.525807540117,23.1959969171709,0.));
#88049=CARTESIAN_POINT('Ctrl Pts',(-67.5486697761301,23.1961167352776,0.));
#88050=CARTESIAN_POINT('Ctrl Pts',(-67.5715771376454,23.1962138725358,0.));
#88051=CARTESIAN_POINT('Ctrl Pts',(-67.5945294909398,23.1962882611443,0.));
#88052=CARTESIAN_POINT('Ctrl Pts',(-67.6175267028517,23.1963398337056,0.));
#88053=CARTESIAN_POINT('Ctrl Pts',(-67.6405686407828,23.1963685232176,0.));
#88054=CARTESIAN_POINT('Ctrl Pts',(-67.6636551726948,23.1963742630709,0.));
#88055=CARTESIAN_POINT('Ctrl Pts',(-67.6867861671045,23.1963569870456,0.));
#88056=CARTESIAN_POINT('Ctrl Pts',(-67.7099614930712,23.1963166293116,0.));
#88057=CARTESIAN_POINT('Ctrl Pts',(-67.7331810201931,23.1962531244261,0.));
#88058=CARTESIAN_POINT('Ctrl Pts',(-67.7564446186115,23.1961664073273,0.));
#88059=CARTESIAN_POINT('Ctrl Pts',(-67.7797521590056,23.1960564133308,0.));
#88060=CARTESIAN_POINT('Ctrl Pts',(-67.8031035125873,23.1959230781265,0.));
#88061=CARTESIAN_POINT('Ctrl Pts',(-67.8264985510885,23.1957663377797,0.));
#88062=CARTESIAN_POINT('Ctrl Pts',(-67.8499371467578,23.1955861287275,0.));
#88063=CARTESIAN_POINT('Ctrl Pts',(-67.8734191723639,23.1953823877726,0.));
#88064=CARTESIAN_POINT('Ctrl Pts',(-67.8969445011908,23.19515505208,0.));
#88065=CARTESIAN_POINT('Ctrl Pts',(-67.9205130070337,23.1949040591748,0.));
#88066=CARTESIAN_POINT('Ctrl Pts',(-67.9441245641871,23.1946293469436,0.));
#88067=CARTESIAN_POINT('Ctrl Pts',(-67.9677790474414,23.1943308536307,0.));
#88068=CARTESIAN_POINT('Ctrl Pts',(-67.9914763320878,23.1940085178319,0.));
#88069=CARTESIAN_POINT('Ctrl Pts',(-68.0152162939123,23.193662278492,0.));
#88070=CARTESIAN_POINT('Ctrl Pts',(-68.0389988091926,23.1932920749021,0.));
#88071=CARTESIAN_POINT('Ctrl Pts',(-68.0628237546853,23.1928978467017,0.));
#88072=CARTESIAN_POINT('Ctrl Pts',(-68.0866910076241,23.1924795338745,0.));
#88073=CARTESIAN_POINT('Ctrl Pts',(-68.1106004457223,23.1920370767423,0.));
#88074=CARTESIAN_POINT('Ctrl Pts',(-68.1345519471695,23.1915704159623,0.));
#88075=CARTESIAN_POINT('Ctrl Pts',(-68.1585453906259,23.1910794925252,0.));
#88076=CARTESIAN_POINT('Ctrl Pts',(-68.182580655213,23.1905642477571,0.));
#88077=CARTESIAN_POINT('Ctrl Pts',(-68.2066576205113,23.1900246233164,0.));
#88078=CARTESIAN_POINT('Ctrl Pts',(-68.2307761665629,23.1894605611869,0.));
#88079=CARTESIAN_POINT('Ctrl Pts',(-68.2549361738679,23.1888720036756,0.));
#88080=CARTESIAN_POINT('Ctrl Pts',(-68.2791375233798,23.1882588934108,0.));
#88081=CARTESIAN_POINT('Ctrl Pts',(-68.3033800964946,23.1876211733439,0.));
#88082=CARTESIAN_POINT('Ctrl Pts',(-68.3276637750494,23.1869587867463,0.));
#88083=CARTESIAN_POINT('Ctrl Pts',(-68.3519884413253,23.1862716772034,0.));
#88084=CARTESIAN_POINT('Ctrl Pts',(-68.3763539780442,23.1855597886117,0.));
#88085=CARTESIAN_POINT('Ctrl Pts',(-68.4007602683649,23.1848230651775,0.));
#88086=CARTESIAN_POINT('Ctrl Pts',(-68.4252071958725,23.184061451419,0.));
#88087=CARTESIAN_POINT('Ctrl Pts',(-68.4496946445756,23.1832748921629,0.));
#88088=CARTESIAN_POINT('Ctrl Pts',(-68.4742224989099,23.1824633325384,0.));
#88089=CARTESIAN_POINT('Ctrl Pts',(-68.4987906437357,23.1816267179751,0.));
#88090=CARTESIAN_POINT('Ctrl Pts',(-68.5233989643344,23.180764994201,0.));
#88091=CARTESIAN_POINT('Ctrl Pts',(-68.548047346398,23.1798781072449,0.));
#88092=CARTESIAN_POINT('Ctrl Pts',(-68.572735676027,23.1789660034339,0.));
#88093=CARTESIAN_POINT('Ctrl Pts',(-68.5974638397322,23.1780286293873,0.));
#88094=CARTESIAN_POINT('Ctrl Pts',(-68.6222317244337,23.1770659320136,0.));
#88095=CARTESIAN_POINT('Ctrl Pts',(-68.6470392174567,23.1760778585093,0.));
#88096=CARTESIAN_POINT('Ctrl Pts',(-68.6718862065227,23.1750643563605,0.));
#88097=CARTESIAN_POINT('Ctrl Pts',(-68.6967725797458,23.1740253733423,0.));
#88098=CARTESIAN_POINT('Ctrl Pts',(-68.7216982256357,23.1729608575115,0.));
#88099=CARTESIAN_POINT('Ctrl Pts',(-68.7466630330968,23.1718707572046,0.));
#88100=CARTESIAN_POINT('Ctrl Pts',(-68.7716668914246,23.1707550210359,0.));
#88101=CARTESIAN_POINT('Ctrl Pts',(-68.7967096902981,23.1696135978992,0.));
#88102=CARTESIAN_POINT('Ctrl Pts',(-68.8217913197735,23.1684464369681,0.));
#88103=CARTESIAN_POINT('Ctrl Pts',(-68.8469116702885,23.1672534876885,0.));
#88104=CARTESIAN_POINT('Ctrl Pts',(-68.8720706326606,23.1660346997762,0.));
#88105=CARTESIAN_POINT('Ctrl Pts',(-68.8972680980844,23.1647900232151,0.));
#88106=CARTESIAN_POINT('Ctrl Pts',(-68.9225039581249,23.1635194082581,0.));
#88107=CARTESIAN_POINT('Ctrl Pts',(-68.9477781047103,23.162222805429,0.));
#88108=CARTESIAN_POINT('Ctrl Pts',(-68.9730904301363,23.1609001655153,0.));
#88109=CARTESIAN_POINT('Ctrl Pts',(-68.9984408270653,23.1595514395654,0.));
#88110=CARTESIAN_POINT('Ctrl Pts',(-69.0238291885245,23.1581765788869,0.));
#88111=CARTESIAN_POINT('Ctrl Pts',(-69.0492554078999,23.1567755350472,0.));
#88112=CARTESIAN_POINT('Ctrl Pts',(-69.0747193789292,23.1553482598767,0.));
#88113=CARTESIAN_POINT('Ctrl Pts',(-69.1002209957037,23.1538947054619,0.));
#88114=CARTESIAN_POINT('Ctrl Pts',(-69.1257601526693,23.1524148241413,0.));
#88115=CARTESIAN_POINT('Ctrl Pts',(-69.1513367446231,23.1509085685032,0.));
#88116=CARTESIAN_POINT('Ctrl Pts',(-69.176950666708,23.1493758913857,0.));
#88117=CARTESIAN_POINT('Ctrl Pts',(-69.2026018144023,23.1478167458787,0.));
#88118=CARTESIAN_POINT('Ctrl Pts',(-69.2282900835234,23.1462310853205,0.));
#88119=CARTESIAN_POINT('Ctrl Pts',(-69.2540153702311,23.1446188632931,0.));
#88120=CARTESIAN_POINT('Ctrl Pts',(-69.2797775710275,23.142980033622,0.));
#88121=CARTESIAN_POINT('Ctrl Pts',(-69.3055765827544,23.1413145503762,0.));
#88122=CARTESIAN_POINT('Ctrl Pts',(-69.3314123025863,23.1396223678725,0.));
#88123=CARTESIAN_POINT('Ctrl Pts',(-69.3572846280289,23.1379034406717,0.));
#88124=CARTESIAN_POINT('Ctrl Pts',(-69.3831934569176,23.1361577235708,0.));
#88125=CARTESIAN_POINT('Ctrl Pts',(-69.4091386874129,23.1343851715988,0.));
#88126=CARTESIAN_POINT('Ctrl Pts',(-69.4351202179948,23.1325857400145,0.));
#88127=CARTESIAN_POINT('Ctrl Pts',(-69.4611379474492,23.1307593843063,0.));
#88128=CARTESIAN_POINT('Ctrl Pts',(-69.4871917748665,23.1289060601927,0.));
#88129=CARTESIAN_POINT('Ctrl Pts',(-69.5132815996548,23.1270257236207,0.));
#88130=CARTESIAN_POINT('Ctrl Pts',(-69.5394073215467,23.1251183307678,0.));
#88131=CARTESIAN_POINT('Ctrl Pts',(-69.565568840605,23.1231838380452,0.));
#88132=CARTESIAN_POINT('Ctrl Pts',(-69.5917660572255,23.1212222021049,0.));
#88133=CARTESIAN_POINT('Ctrl Pts',(-69.617998872135,23.1192333798437,0.));
#88134=CARTESIAN_POINT('Ctrl Pts',(-69.6442671863751,23.1172173283855,0.));
#88135=CARTESIAN_POINT('Ctrl Pts',(-69.6705709012842,23.1151740050678,0.));
#88136=CARTESIAN_POINT('Ctrl Pts',(-69.6969099184766,23.1131033674301,0.));
#88137=CARTESIAN_POINT('Ctrl Pts',(-69.7232841398207,23.1110053732049,0.));
#88138=CARTESIAN_POINT('Ctrl Pts',(-69.7496934674083,23.1088799803093,0.));
#88139=CARTESIAN_POINT('Ctrl Pts',(-69.7761378035979,23.1067271468614,0.));
#88140=CARTESIAN_POINT('Ctrl Pts',(-69.8026170510582,23.1045468311994,0.));
#88141=CARTESIAN_POINT('Ctrl Pts',(-69.8291311128121,23.1023389919052,0.));
#88142=CARTESIAN_POINT('Ctrl Pts',(-69.8556798922688,23.100103587824,0.));
#88143=CARTESIAN_POINT('Ctrl Pts',(-69.882263293276,23.0978405781018,0.));
#88144=CARTESIAN_POINT('Ctrl Pts',(-69.9088812200704,23.0955499221556,0.));
#88145=CARTESIAN_POINT('Ctrl Pts',(-69.9355335771722,23.0932315796066,0.));
#88146=CARTESIAN_POINT('Ctrl Pts',(-69.9622202692871,23.090885510225,0.));
#88147=CARTESIAN_POINT('Ctrl Pts',(-69.9889412012143,23.0885116738798,0.));
#88148=CARTESIAN_POINT('Ctrl Pts',(-70.0156962777173,23.0861100304731,0.));
#88149=CARTESIAN_POINT('Ctrl Pts',(-70.0424854035125,23.0836805399377,0.));
#88150=CARTESIAN_POINT('Ctrl Pts',(-70.0693084835388,23.081223162377,0.));
#88151=CARTESIAN_POINT('Ctrl Pts',(-70.096165423165,23.0787378581778,0.));
#88152=CARTESIAN_POINT('Ctrl Pts',(-70.1230561284222,23.076224588139,0.));
#88153=CARTESIAN_POINT('Ctrl Pts',(-70.1499805062159,23.0736833135934,0.));
#88154=CARTESIAN_POINT('Ctrl Pts',(-70.176938464556,23.0711139965432,0.));
#88155=CARTESIAN_POINT('Ctrl Pts',(-70.2039299120456,23.0685165993681,0.));
#88156=CARTESIAN_POINT('Ctrl Pts',(-70.2309547573789,23.0658910845425,0.));
#88157=CARTESIAN_POINT('Ctrl Pts',(-70.2580129087878,23.0632374143276,0.));
#88158=CARTESIAN_POINT('Ctrl Pts',(-70.2851042736081,23.0605555505326,0.));
#88159=CARTESIAN_POINT('Ctrl Pts',(-70.3122287575374,23.0578454541116,0.));
#88160=CARTESIAN_POINT('Ctrl Pts',(-70.3393862652353,23.0551070854942,0.));
#88161=CARTESIAN_POINT('Ctrl Pts',(-70.3665767016596,23.0523404053188,0.));
#88162=CARTESIAN_POINT('Ctrl Pts',(-70.39379997323,23.0495453750773,0.));
#88163=CARTESIAN_POINT('Ctrl Pts',(-70.421055988934,23.0467219577288,0.));
#88164=CARTESIAN_POINT('Ctrl Pts',(-70.4483446617553,23.0438701184995,0.));
#88165=CARTESIAN_POINT('Ctrl Pts',(-70.4756659090104,23.0409898250726,0.));
#88166=CARTESIAN_POINT('Ctrl Pts',(-70.4991133648756,23.038496437601,0.));
#88167=CARTESIAN_POINT('Ctrl Pts',(-70.5171075702495,23.0365694096158,0.));
#88168=CARTESIAN_POINT('Ctrl Pts',(-70.5296341535252,23.0352213647764,0.));
#88169=CARTESIAN_POINT('Ctrl Pts',(-70.5366836381299,23.034460662331,0.));
#88170=CARTESIAN_POINT('Ctrl Pts',(-70.5382514078488,23.0342913834093,0.));
#88171=CARTESIAN_POINT('',(-66.0656156664138,23.1372951448024,12.));
#88172=CARTESIAN_POINT('',(-66.0656156664138,23.1372951448024,0.));
#88173=CARTESIAN_POINT('Ctrl Pts',(-70.5382514078489,23.0342913834093,12.));
#88174=CARTESIAN_POINT('Ctrl Pts',(-70.5366836381299,23.034460662331,12.));
#88175=CARTESIAN_POINT('Ctrl Pts',(-70.5296341535252,23.0352213647764,12.));
#88176=CARTESIAN_POINT('Ctrl Pts',(-70.5171075702495,23.0365694096158,12.));
#88177=CARTESIAN_POINT('Ctrl Pts',(-70.4991133648756,23.038496437601,12.));
#88178=CARTESIAN_POINT('Ctrl Pts',(-70.4756659090104,23.0409898250726,12.));
#88179=CARTESIAN_POINT('Ctrl Pts',(-70.4483446617553,23.0438701184995,12.));
#88180=CARTESIAN_POINT('Ctrl Pts',(-70.421055988934,23.0467219577288,12.));
#88181=CARTESIAN_POINT('Ctrl Pts',(-70.39379997323,23.0495453750773,12.));
#88182=CARTESIAN_POINT('Ctrl Pts',(-70.3665767016596,23.0523404053188,12.));
#88183=CARTESIAN_POINT('Ctrl Pts',(-70.3393862652353,23.0551070854942,12.));
#88184=CARTESIAN_POINT('Ctrl Pts',(-70.3122287575374,23.0578454541116,12.));
#88185=CARTESIAN_POINT('Ctrl Pts',(-70.2851042736081,23.0605555505326,12.));
#88186=CARTESIAN_POINT('Ctrl Pts',(-70.2580129087878,23.0632374143276,12.));
#88187=CARTESIAN_POINT('Ctrl Pts',(-70.2309547573789,23.0658910845425,12.));
#88188=CARTESIAN_POINT('Ctrl Pts',(-70.2039299120456,23.0685165993681,12.));
#88189=CARTESIAN_POINT('Ctrl Pts',(-70.176938464556,23.0711139965432,12.));
#88190=CARTESIAN_POINT('Ctrl Pts',(-70.1499805062159,23.0736833135934,12.));
#88191=CARTESIAN_POINT('Ctrl Pts',(-70.1230561284222,23.076224588139,12.));
#88192=CARTESIAN_POINT('Ctrl Pts',(-70.096165423165,23.0787378581778,12.));
#88193=CARTESIAN_POINT('Ctrl Pts',(-70.0693084835388,23.081223162377,12.));
#88194=CARTESIAN_POINT('Ctrl Pts',(-70.0424854035125,23.0836805399377,12.));
#88195=CARTESIAN_POINT('Ctrl Pts',(-70.0156962777173,23.0861100304731,12.));
#88196=CARTESIAN_POINT('Ctrl Pts',(-69.9889412012143,23.0885116738798,12.));
#88197=CARTESIAN_POINT('Ctrl Pts',(-69.9622202692871,23.090885510225,12.));
#88198=CARTESIAN_POINT('Ctrl Pts',(-69.9355335771722,23.0932315796066,12.));
#88199=CARTESIAN_POINT('Ctrl Pts',(-69.9088812200704,23.0955499221556,12.));
#88200=CARTESIAN_POINT('Ctrl Pts',(-69.882263293276,23.0978405781018,12.));
#88201=CARTESIAN_POINT('Ctrl Pts',(-69.8556798922688,23.100103587824,12.));
#88202=CARTESIAN_POINT('Ctrl Pts',(-69.8291311128121,23.1023389919052,12.));
#88203=CARTESIAN_POINT('Ctrl Pts',(-69.8026170510582,23.1045468311994,12.));
#88204=CARTESIAN_POINT('Ctrl Pts',(-69.7761378035979,23.1067271468614,12.));
#88205=CARTESIAN_POINT('Ctrl Pts',(-69.7496934674083,23.1088799803093,12.));
#88206=CARTESIAN_POINT('Ctrl Pts',(-69.7232841398207,23.1110053732049,12.));
#88207=CARTESIAN_POINT('Ctrl Pts',(-69.6969099184766,23.1131033674301,12.));
#88208=CARTESIAN_POINT('Ctrl Pts',(-69.6705709012842,23.1151740050678,12.));
#88209=CARTESIAN_POINT('Ctrl Pts',(-69.6442671863751,23.1172173283855,12.));
#88210=CARTESIAN_POINT('Ctrl Pts',(-69.617998872135,23.1192333798437,12.));
#88211=CARTESIAN_POINT('Ctrl Pts',(-69.5917660572255,23.1212222021049,12.));
#88212=CARTESIAN_POINT('Ctrl Pts',(-69.565568840605,23.1231838380452,12.));
#88213=CARTESIAN_POINT('Ctrl Pts',(-69.5394073215467,23.1251183307678,12.));
#88214=CARTESIAN_POINT('Ctrl Pts',(-69.5132815996548,23.1270257236207,12.));
#88215=CARTESIAN_POINT('Ctrl Pts',(-69.4871917748665,23.1289060601927,12.));
#88216=CARTESIAN_POINT('Ctrl Pts',(-69.4611379474492,23.1307593843063,12.));
#88217=CARTESIAN_POINT('Ctrl Pts',(-69.4351202179948,23.1325857400145,12.));
#88218=CARTESIAN_POINT('Ctrl Pts',(-69.4091386874129,23.1343851715988,12.));
#88219=CARTESIAN_POINT('Ctrl Pts',(-69.3831934569176,23.1361577235708,12.));
#88220=CARTESIAN_POINT('Ctrl Pts',(-69.3572846280289,23.1379034406717,12.));
#88221=CARTESIAN_POINT('Ctrl Pts',(-69.3314123025863,23.1396223678725,12.));
#88222=CARTESIAN_POINT('Ctrl Pts',(-69.3055765827544,23.1413145503762,12.));
#88223=CARTESIAN_POINT('Ctrl Pts',(-69.2797775710275,23.142980033622,12.));
#88224=CARTESIAN_POINT('Ctrl Pts',(-69.2540153702311,23.1446188632931,12.));
#88225=CARTESIAN_POINT('Ctrl Pts',(-69.2282900835234,23.1462310853205,12.));
#88226=CARTESIAN_POINT('Ctrl Pts',(-69.2026018144023,23.1478167458787,12.));
#88227=CARTESIAN_POINT('Ctrl Pts',(-69.176950666708,23.1493758913857,12.));
#88228=CARTESIAN_POINT('Ctrl Pts',(-69.1513367446231,23.1509085685032,12.));
#88229=CARTESIAN_POINT('Ctrl Pts',(-69.1257601526693,23.1524148241413,12.));
#88230=CARTESIAN_POINT('Ctrl Pts',(-69.1002209957037,23.1538947054619,12.));
#88231=CARTESIAN_POINT('Ctrl Pts',(-69.0747193789292,23.1553482598767,12.));
#88232=CARTESIAN_POINT('Ctrl Pts',(-69.0492554078999,23.1567755350472,12.));
#88233=CARTESIAN_POINT('Ctrl Pts',(-69.0238291885245,23.1581765788869,12.));
#88234=CARTESIAN_POINT('Ctrl Pts',(-68.9984408270653,23.1595514395654,12.));
#88235=CARTESIAN_POINT('Ctrl Pts',(-68.9730904301363,23.1609001655153,12.));
#88236=CARTESIAN_POINT('Ctrl Pts',(-68.9477781047103,23.162222805429,12.));
#88237=CARTESIAN_POINT('Ctrl Pts',(-68.9225039581249,23.1635194082581,12.));
#88238=CARTESIAN_POINT('Ctrl Pts',(-68.8972680980844,23.1647900232151,12.));
#88239=CARTESIAN_POINT('Ctrl Pts',(-68.8720706326606,23.1660346997762,12.));
#88240=CARTESIAN_POINT('Ctrl Pts',(-68.8469116702885,23.1672534876885,12.));
#88241=CARTESIAN_POINT('Ctrl Pts',(-68.8217913197735,23.1684464369681,12.));
#88242=CARTESIAN_POINT('Ctrl Pts',(-68.7967096902981,23.1696135978992,12.));
#88243=CARTESIAN_POINT('Ctrl Pts',(-68.7716668914246,23.1707550210359,12.));
#88244=CARTESIAN_POINT('Ctrl Pts',(-68.7466630330968,23.1718707572046,12.));
#88245=CARTESIAN_POINT('Ctrl Pts',(-68.7216982256357,23.1729608575115,12.));
#88246=CARTESIAN_POINT('Ctrl Pts',(-68.6967725797458,23.1740253733423,12.));
#88247=CARTESIAN_POINT('Ctrl Pts',(-68.6718862065227,23.1750643563605,12.));
#88248=CARTESIAN_POINT('Ctrl Pts',(-68.6470392174567,23.1760778585093,12.));
#88249=CARTESIAN_POINT('Ctrl Pts',(-68.6222317244337,23.1770659320136,12.));
#88250=CARTESIAN_POINT('Ctrl Pts',(-68.5974638397322,23.1780286293873,12.));
#88251=CARTESIAN_POINT('Ctrl Pts',(-68.572735676027,23.1789660034339,12.));
#88252=CARTESIAN_POINT('Ctrl Pts',(-68.548047346398,23.1798781072449,12.));
#88253=CARTESIAN_POINT('Ctrl Pts',(-68.5233989643344,23.180764994201,12.));
#88254=CARTESIAN_POINT('Ctrl Pts',(-68.4987906437357,23.1816267179751,12.));
#88255=CARTESIAN_POINT('Ctrl Pts',(-68.4742224989099,23.1824633325384,12.));
#88256=CARTESIAN_POINT('Ctrl Pts',(-68.4496946445756,23.1832748921629,12.));
#88257=CARTESIAN_POINT('Ctrl Pts',(-68.4252071958725,23.184061451419,12.));
#88258=CARTESIAN_POINT('Ctrl Pts',(-68.4007602683649,23.1848230651775,12.));
#88259=CARTESIAN_POINT('Ctrl Pts',(-68.3763539780442,23.1855597886117,12.));
#88260=CARTESIAN_POINT('Ctrl Pts',(-68.3519884413253,23.1862716772034,12.));
#88261=CARTESIAN_POINT('Ctrl Pts',(-68.3276637750494,23.1869587867463,12.));
#88262=CARTESIAN_POINT('Ctrl Pts',(-68.3033800964946,23.1876211733439,12.));
#88263=CARTESIAN_POINT('Ctrl Pts',(-68.2791375233798,23.1882588934108,12.));
#88264=CARTESIAN_POINT('Ctrl Pts',(-68.2549361738679,23.1888720036756,12.));
#88265=CARTESIAN_POINT('Ctrl Pts',(-68.2307761665629,23.1894605611869,12.));
#88266=CARTESIAN_POINT('Ctrl Pts',(-68.2066576205113,23.1900246233164,12.));
#88267=CARTESIAN_POINT('Ctrl Pts',(-68.182580655213,23.1905642477571,12.));
#88268=CARTESIAN_POINT('Ctrl Pts',(-68.1585453906259,23.1910794925252,12.));
#88269=CARTESIAN_POINT('Ctrl Pts',(-68.1345519471695,23.1915704159623,12.));
#88270=CARTESIAN_POINT('Ctrl Pts',(-68.1106004457223,23.1920370767423,12.));
#88271=CARTESIAN_POINT('Ctrl Pts',(-68.0866910076241,23.1924795338745,12.));
#88272=CARTESIAN_POINT('Ctrl Pts',(-68.0628237546853,23.1928978467017,12.));
#88273=CARTESIAN_POINT('Ctrl Pts',(-68.0389988091926,23.1932920749021,12.));
#88274=CARTESIAN_POINT('Ctrl Pts',(-68.0152162939123,23.193662278492,12.));
#88275=CARTESIAN_POINT('Ctrl Pts',(-67.9914763320878,23.1940085178319,12.));
#88276=CARTESIAN_POINT('Ctrl Pts',(-67.9677790474414,23.1943308536307,12.));
#88277=CARTESIAN_POINT('Ctrl Pts',(-67.9441245641871,23.1946293469436,12.));
#88278=CARTESIAN_POINT('Ctrl Pts',(-67.9205130070337,23.1949040591748,12.));
#88279=CARTESIAN_POINT('Ctrl Pts',(-67.8969445011908,23.19515505208,12.));
#88280=CARTESIAN_POINT('Ctrl Pts',(-67.8734191723639,23.1953823877726,12.));
#88281=CARTESIAN_POINT('Ctrl Pts',(-67.8499371467578,23.1955861287275,12.));
#88282=CARTESIAN_POINT('Ctrl Pts',(-67.8264985510885,23.1957663377797,12.));
#88283=CARTESIAN_POINT('Ctrl Pts',(-67.8031035125873,23.1959230781265,12.));
#88284=CARTESIAN_POINT('Ctrl Pts',(-67.7797521590056,23.1960564133308,12.));
#88285=CARTESIAN_POINT('Ctrl Pts',(-67.7564446186115,23.1961664073273,12.));
#88286=CARTESIAN_POINT('Ctrl Pts',(-67.7331810201931,23.1962531244261,12.));
#88287=CARTESIAN_POINT('Ctrl Pts',(-67.7099614930712,23.1963166293116,12.));
#88288=CARTESIAN_POINT('Ctrl Pts',(-67.6867861671045,23.1963569870456,12.));
#88289=CARTESIAN_POINT('Ctrl Pts',(-67.6636551726948,23.1963742630709,12.));
#88290=CARTESIAN_POINT('Ctrl Pts',(-67.6405686407828,23.1963685232176,12.));
#88291=CARTESIAN_POINT('Ctrl Pts',(-67.6175267028517,23.1963398337056,12.));
#88292=CARTESIAN_POINT('Ctrl Pts',(-67.5945294909398,23.1962882611443,12.));
#88293=CARTESIAN_POINT('Ctrl Pts',(-67.5715771376454,23.1962138725358,12.));
#88294=CARTESIAN_POINT('Ctrl Pts',(-67.5486697761301,23.1961167352776,12.));
#88295=CARTESIAN_POINT('Ctrl Pts',(-67.525807540117,23.1959969171709,12.));
#88296=CARTESIAN_POINT('Ctrl Pts',(-67.5029905638974,23.1958544864224,12.));
#88297=CARTESIAN_POINT('Ctrl Pts',(-67.4802189823424,23.1956895116446,12.));
#88298=CARTESIAN_POINT('Ctrl Pts',(-67.4574929309079,23.1955020618591,12.));
#88299=CARTESIAN_POINT('Ctrl Pts',(-67.4348125456389,23.1952922065009,12.));
#88300=CARTESIAN_POINT('Ctrl Pts',(-67.4121779631666,23.1950600154259,12.));
#88301=CARTESIAN_POINT('Ctrl Pts',(-67.3895893207168,23.1948055589123,12.));
#88302=CARTESIAN_POINT('Ctrl Pts',(-67.3670467561205,23.1945289076608,12.));
#88303=CARTESIAN_POINT('Ctrl Pts',(-67.3445504078178,23.1942301327979,12.));
#88304=CARTESIAN_POINT('Ctrl Pts',(-67.3221004148604,23.1939093058802,12.));
#88305=CARTESIAN_POINT('Ctrl Pts',(-67.2996969169099,23.193566498902,12.));
#88306=CARTESIAN_POINT('Ctrl Pts',(-67.2773400542477,23.1932017842954,12.));
#88307=CARTESIAN_POINT('Ctrl Pts',(-67.2550299677888,23.1928152349343,12.));
#88308=CARTESIAN_POINT('Ctrl Pts',(-67.232766799088,23.1924069241385,12.));
#88309=CARTESIAN_POINT('Ctrl Pts',(-67.2105506903448,23.1919769256803,12.));
#88310=CARTESIAN_POINT('Ctrl Pts',(-67.1883817844039,23.1915253137923,12.));
#88311=CARTESIAN_POINT('Ctrl Pts',(-67.1662602247641,23.1910521631658,12.));
#88312=CARTESIAN_POINT('Ctrl Pts',(-67.1441861555819,23.1905575489505,12.));
#88313=CARTESIAN_POINT('Ctrl Pts',(-67.122159721674,23.1900415467574,12.));
#88314=CARTESIAN_POINT('Ctrl Pts',(-67.1001810685138,23.1895042326625,12.));
#88315=CARTESIAN_POINT('Ctrl Pts',(-67.0782503422293,23.1889456832115,12.));
#88316=CARTESIAN_POINT('Ctrl Pts',(-67.0563676896312,23.1883659754267,12.));
#88317=CARTESIAN_POINT('Ctrl Pts',(-67.0345332582297,23.1877651868155,12.));
#88318=CARTESIAN_POINT('Ctrl Pts',(-67.0127471962507,23.1871433953795,12.));
#88319=CARTESIAN_POINT('Ctrl Pts',(-66.9910096526483,23.1865006796291,12.));
#88320=CARTESIAN_POINT('Ctrl Pts',(-66.9693207771059,23.1858371185852,12.));
#88321=CARTESIAN_POINT('Ctrl Pts',(-66.9476807200225,23.1851527917665,12.));
#88322=CARTESIAN_POINT('Ctrl Pts',(-66.9260896324955,23.1844477791816,12.));
#88323=CARTESIAN_POINT('Ctrl Pts',(-66.904547666305,23.1837221613231,12.));
#88324=CARTESIAN_POINT('Ctrl Pts',(-66.8830549738768,23.1829760191582,12.));
#88325=CARTESIAN_POINT('Ctrl Pts',(-66.8616117083304,23.1822094341508,12.));
#88326=CARTESIAN_POINT('Ctrl Pts',(-66.840218023555,23.1814224882948,12.));
#88327=CARTESIAN_POINT('Ctrl Pts',(-66.8188740742727,23.1806152641475,12.));
#88328=CARTESIAN_POINT('Ctrl Pts',(-66.7975800161014,23.1797878448645,12.));
#88329=CARTESIAN_POINT('Ctrl Pts',(-66.7763360056146,23.1789403142375,12.));
#88330=CARTESIAN_POINT('Ctrl Pts',(-66.7551422002229,23.1780727566309,12.));
#88331=CARTESIAN_POINT('Ctrl Pts',(-66.7339987580441,23.1771852569136,12.));
#88332=CARTESIAN_POINT('Ctrl Pts',(-66.712905837789,23.1762779004043,12.));
#88333=CARTESIAN_POINT('Ctrl Pts',(-66.691863598595,23.1753507727931,12.));
#88334=CARTESIAN_POINT('Ctrl Pts',(-66.6708722000047,23.174403960137,12.));
#88335=CARTESIAN_POINT('Ctrl Pts',(-66.6499318023445,23.1734375490421,12.));
#88336=CARTESIAN_POINT('Ctrl Pts',(-66.6290425670538,23.1724516268299,12.));
#88337=CARTESIAN_POINT('Ctrl Pts',(-66.6082046569657,23.1714462816794,12.));
#88338=CARTESIAN_POINT('Ctrl Pts',(-66.5874182367597,23.1704216028626,12.));
#88339=CARTESIAN_POINT('Ctrl Pts',(-66.5666834726495,23.169377680588,12.));
#88340=CARTESIAN_POINT('Ctrl Pts',(-66.5460005315406,23.1683146055736,12.));
#88341=CARTESIAN_POINT('Ctrl Pts',(-66.5253695803209,23.1672324686927,12.));
#88342=CARTESIAN_POINT('Ctrl Pts',(-66.5047907851319,23.1661313606123,12.));
#88343=CARTESIAN_POINT('Ctrl Pts',(-66.4842643105263,23.1650113713792,12.));
#88344=CARTESIAN_POINT('Ctrl Pts',(-66.4637903210682,23.163872591218,12.));
#88345=CARTESIAN_POINT('Ctrl Pts',(-66.4433689832454,23.1627151114875,12.));
#88346=CARTESIAN_POINT('Ctrl Pts',(-66.4230004670288,23.1615390254635,12.));
#88347=CARTESIAN_POINT('Ctrl Pts',(-66.402684948127,23.1603444294754,12.));
#88348=CARTESIAN_POINT('Ctrl Pts',(-66.382422608185,23.15913142301,12.));
#88349=CARTESIAN_POINT('Ctrl Pts',(-66.3622136300692,23.1579001063438,12.));
#88350=CARTESIAN_POINT('Ctrl Pts',(-66.3420581937159,23.1566505784626,12.));
#88351=CARTESIAN_POINT('Ctrl Pts',(-66.3219564725161,23.1553829352531,12.));
#88352=CARTESIAN_POINT('Ctrl Pts',(-66.301908627539,23.154097266617,12.));
#88353=CARTESIAN_POINT('Ctrl Pts',(-66.2819148131072,23.1527936592625,12.));
#88354=CARTESIAN_POINT('Ctrl Pts',(-66.2619751878741,23.1514722022483,12.));
#88355=CARTESIAN_POINT('Ctrl Pts',(-66.2420899237317,23.1501329914488,12.));
#88356=CARTESIAN_POINT('Ctrl Pts',(-66.2222592165473,23.1487761349328,12.));
#88357=CARTESIAN_POINT('Ctrl Pts',(-66.2024832934866,23.1474017566484,12.));
#88358=CARTESIAN_POINT('Ctrl Pts',(-66.18276239029,23.1460099850763,12.));
#88359=CARTESIAN_POINT('Ctrl Pts',(-66.1630967296747,23.1446009424903,12.));
#88360=CARTESIAN_POINT('Ctrl Pts',(-66.1434865015027,23.1431747350098,12.));
#88361=CARTESIAN_POINT('Ctrl Pts',(-66.1239318368548,23.1417314398398,12.));
#88362=CARTESIAN_POINT('Ctrl Pts',(-66.1044328067355,23.1402711039425,12.));
#88363=CARTESIAN_POINT('Ctrl Pts',(-66.0888781152421,23.1390892229778,12.));
#88364=CARTESIAN_POINT('Ctrl Pts',(-66.0772371487248,23.13819515974,12.));
#88365=CARTESIAN_POINT('Ctrl Pts',(-66.0694876382127,23.1375957166104,12.));
#88366=CARTESIAN_POINT('Ctrl Pts',(-66.0656156664138,23.1372951448024,12.));
#88367=CARTESIAN_POINT('Ctrl Pts',(-70.9934796069113,21.5904919935059,-5.55111512312578E-16));
#88368=CARTESIAN_POINT('Ctrl Pts',(-70.9934796069113,21.5904919935059,4.));
#88369=CARTESIAN_POINT('Ctrl Pts',(-70.9934796069113,21.5904919935059,8.));
#88370=CARTESIAN_POINT('Ctrl Pts',(-70.9934796069113,21.5904919935059,12.));
#88371=CARTESIAN_POINT('Ctrl Pts',(-71.0762040404458,21.6628164325797,-5.55111512312578E-16));
#88372=CARTESIAN_POINT('Ctrl Pts',(-71.0762040404458,21.6628164325797,4.));
#88373=CARTESIAN_POINT('Ctrl Pts',(-71.0762040404458,21.6628164325797,8.00000000000001));
#88374=CARTESIAN_POINT('Ctrl Pts',(-71.0762040404458,21.6628164325797,12.));
#88375=CARTESIAN_POINT('Ctrl Pts',(-71.1771795679088,21.8385342042356,-5.55111512312578E-16));
#88376=CARTESIAN_POINT('Ctrl Pts',(-71.1771795679088,21.8385342042356,4.));
#88377=CARTESIAN_POINT('Ctrl Pts',(-71.1771795679088,21.8385342042356,7.99999999999999));
#88378=CARTESIAN_POINT('Ctrl Pts',(-71.1771795679088,21.8385342042356,12.));
#88379=CARTESIAN_POINT('Ctrl Pts',(-71.1663065220513,22.0366423876811,-5.55111512312578E-16));
#88380=CARTESIAN_POINT('Ctrl Pts',(-71.1663065220513,22.0366423876811,4.));
#88381=CARTESIAN_POINT('Ctrl Pts',(-71.1663065220513,22.0366423876811,8.00000000000001));
#88382=CARTESIAN_POINT('Ctrl Pts',(-71.1663065220513,22.0366423876811,12.));
#88383=CARTESIAN_POINT('Ctrl Pts',(-71.1418425484898,22.1153394458694,-5.55111512312578E-16));
#88384=CARTESIAN_POINT('Ctrl Pts',(-71.1418425484898,22.1153394458694,4.));
#88385=CARTESIAN_POINT('Ctrl Pts',(-71.1418425484898,22.1153394458694,8.));
#88386=CARTESIAN_POINT('Ctrl Pts',(-71.1418425484898,22.1153394458694,12.));
#88387=CARTESIAN_POINT('',(-70.9934796069113,21.5904919935059,2.77555756156289E-16));
#88388=CARTESIAN_POINT('',(-71.1418425484889,22.1153394458691,0.));
#88389=CARTESIAN_POINT('Ctrl Pts',(-70.9934796069113,21.5904919935059,-1.38777878078145E-16));
#88390=CARTESIAN_POINT('Ctrl Pts',(-71.0762040404458,21.6628164325797,-1.38777878078145E-16));
#88391=CARTESIAN_POINT('Ctrl Pts',(-71.1339043418532,21.7632265878116,-1.38777878078144E-16));
#88392=CARTESIAN_POINT('Ctrl Pts',(-71.1550826601356,21.8709478979137,-1.38777878078145E-16));
#88393=CARTESIAN_POINT('Ctrl Pts',(-71.1709663988474,21.9517388804902,-1.38777878078145E-16));
#88394=CARTESIAN_POINT('Ctrl Pts',(-71.1663065220513,22.0366423876811,-1.38777878078145E-16));
#88395=CARTESIAN_POINT('Ctrl Pts',(-71.1418425484898,22.1153394458694,-1.38777878078145E-16));
#88396=CARTESIAN_POINT('',(-71.1418425484889,22.1153394458691,12.));
#88397=CARTESIAN_POINT('Ctrl Pts',(-71.1418425484898,22.1153394458694,-5.55111512312578E-16));
#88398=CARTESIAN_POINT('Ctrl Pts',(-71.1418425484898,22.1153394458694,4.));
#88399=CARTESIAN_POINT('Ctrl Pts',(-71.1418425484898,22.1153394458694,8.));
#88400=CARTESIAN_POINT('Ctrl Pts',(-71.1418425484898,22.1153394458694,12.));
#88401=CARTESIAN_POINT('',(-70.9934796069113,21.5904919935059,12.));
#88402=CARTESIAN_POINT('Ctrl Pts',(-71.1418425484898,22.1153394458694,12.));
#88403=CARTESIAN_POINT('Ctrl Pts',(-71.1663065220513,22.0366423876811,12.));
#88404=CARTESIAN_POINT('Ctrl Pts',(-71.1709663988474,21.9517388804902,12.));
#88405=CARTESIAN_POINT('Ctrl Pts',(-71.1550826601356,21.8709478979137,12.));
#88406=CARTESIAN_POINT('Ctrl Pts',(-71.1339043418532,21.7632265878116,12.));
#88407=CARTESIAN_POINT('Ctrl Pts',(-71.0762040404458,21.6628164325797,12.));
#88408=CARTESIAN_POINT('Ctrl Pts',(-70.9934796069113,21.5904919935059,12.));
#88409=CARTESIAN_POINT('Ctrl Pts',(-70.9934796069113,21.5904919935059,12.));
#88410=CARTESIAN_POINT('Ctrl Pts',(-70.9934796069113,21.5904919935059,8.));
#88411=CARTESIAN_POINT('Ctrl Pts',(-70.9934796069113,21.5904919935059,4.));
#88412=CARTESIAN_POINT('Ctrl Pts',(-70.9934796069113,21.5904919935059,-5.55111512312578E-16));
#88413=CARTESIAN_POINT('Origin',(-3.57524700084383E-10,1.12623029467293E-10,
0.));
#88414=CARTESIAN_POINT('Origin',(-3.57524700084383E-10,1.12623029467293E-10,
12.));
#88415=CARTESIAN_POINT('Origin',(-3.57524700084383E-10,1.12623029467293E-10,
0.));
#88416=CARTESIAN_POINT('Ctrl Pts',(-68.7132793373328,28.7877620302391,-5.55111512312578E-16));
#88417=CARTESIAN_POINT('Ctrl Pts',(-68.7132793373328,28.7877620302391,4.));
#88418=CARTESIAN_POINT('Ctrl Pts',(-68.7132793373328,28.7877620302391,8.));
#88419=CARTESIAN_POINT('Ctrl Pts',(-68.7132793373328,28.7877620302391,12.));
#88420=CARTESIAN_POINT('Ctrl Pts',(-68.6708193334379,28.8891094745186,-5.55111512312578E-16));
#88421=CARTESIAN_POINT('Ctrl Pts',(-68.6708193334379,28.8891094745186,4.));
#88422=CARTESIAN_POINT('Ctrl Pts',(-68.6708193334379,28.8891094745186,8.));
#88423=CARTESIAN_POINT('Ctrl Pts',(-68.6708193334379,28.8891094745186,12.));
#88424=CARTESIAN_POINT('Ctrl Pts',(-68.5360395709812,29.0404604348957,-5.55111512312578E-16));
#88425=CARTESIAN_POINT('Ctrl Pts',(-68.5360395709812,29.0404604348957,4.));
#88426=CARTESIAN_POINT('Ctrl Pts',(-68.5360395709812,29.0404604348957,7.99999999999999));
#88427=CARTESIAN_POINT('Ctrl Pts',(-68.5360395709812,29.0404604348957,12.));
#88428=CARTESIAN_POINT('Ctrl Pts',(-68.3446561754307,29.0927805237118,-5.55111512312578E-16));
#88429=CARTESIAN_POINT('Ctrl Pts',(-68.3446561754307,29.0927805237118,4.));
#88430=CARTESIAN_POINT('Ctrl Pts',(-68.3446561754307,29.0927805237118,8.00000000000001));
#88431=CARTESIAN_POINT('Ctrl Pts',(-68.3446561754307,29.0927805237118,12.));
#88432=CARTESIAN_POINT('Ctrl Pts',(-68.2622612909744,29.0944526440248,-5.55111512312578E-16));
#88433=CARTESIAN_POINT('Ctrl Pts',(-68.2622612909744,29.0944526440248,4.));
#88434=CARTESIAN_POINT('Ctrl Pts',(-68.2622612909744,29.0944526440248,8.));
#88435=CARTESIAN_POINT('Ctrl Pts',(-68.2622612909744,29.0944526440248,12.));
#88436=CARTESIAN_POINT('',(-68.7132793373328,28.7877620302391,0.));
#88437=CARTESIAN_POINT('',(-68.2622612909744,29.0944526440249,0.));
#88438=CARTESIAN_POINT('Ctrl Pts',(-68.7132793373328,28.7877620302391,0.));
#88439=CARTESIAN_POINT('Ctrl Pts',(-68.6708193334379,28.8891094745186,-1.54074395550979E-31));
#88440=CARTESIAN_POINT('Ctrl Pts',(-68.5938023263198,28.9755957375912,1.54074395550979E-31));
#88441=CARTESIAN_POINT('Ctrl Pts',(-68.4983025002323,29.0297453895419,7.70371977754892E-32));
#88442=CARTESIAN_POINT('Ctrl Pts',(-68.4266776306666,29.0703576285049,-7.70371977754894E-32));
#88443=CARTESIAN_POINT('Ctrl Pts',(-68.3446561754307,29.0927805237118,-5.39260384428426E-31));
#88444=CARTESIAN_POINT('Ctrl Pts',(-68.2622612909744,29.0944526440248,-7.70371977754895E-32));
#88445=CARTESIAN_POINT('',(-68.2622612909744,29.0944526440249,12.));
#88446=CARTESIAN_POINT('Ctrl Pts',(-68.2622612909744,29.0944526440248,-5.55111512312578E-16));
#88447=CARTESIAN_POINT('Ctrl Pts',(-68.2622612909744,29.0944526440248,4.));
#88448=CARTESIAN_POINT('Ctrl Pts',(-68.2622612909744,29.0944526440248,8.));
#88449=CARTESIAN_POINT('Ctrl Pts',(-68.2622612909744,29.0944526440248,12.));
#88450=CARTESIAN_POINT('',(-68.7132793373328,28.7877620302391,12.));
#88451=CARTESIAN_POINT('Ctrl Pts',(-68.2622612909744,29.0944526440248,12.));
#88452=CARTESIAN_POINT('Ctrl Pts',(-68.3446561754307,29.0927805237118,12.));
#88453=CARTESIAN_POINT('Ctrl Pts',(-68.4266776306666,29.0703576285049,12.));
#88454=CARTESIAN_POINT('Ctrl Pts',(-68.4983025002323,29.0297453895419,12.));
#88455=CARTESIAN_POINT('Ctrl Pts',(-68.5938023263198,28.9755957375912,12.));
#88456=CARTESIAN_POINT('Ctrl Pts',(-68.6708193334379,28.8891094745186,12.));
#88457=CARTESIAN_POINT('Ctrl Pts',(-68.7132793373328,28.7877620302391,12.));
#88458=CARTESIAN_POINT('Ctrl Pts',(-68.7132793373328,28.7877620302391,12.));
#88459=CARTESIAN_POINT('Ctrl Pts',(-68.7132793373328,28.7877620302391,8.));
#88460=CARTESIAN_POINT('Ctrl Pts',(-68.7132793373328,28.7877620302391,4.));
#88461=CARTESIAN_POINT('Ctrl Pts',(-68.7132793373328,28.7877620302391,-5.55111512312578E-16));
#88462=CARTESIAN_POINT('Ctrl Pts',(-63.7976679095314,28.8072485549236,0.));
#88463=CARTESIAN_POINT('Ctrl Pts',(-63.7976679095314,28.8072485549236,12.));
#88464=CARTESIAN_POINT('Ctrl Pts',(-63.8014989507494,28.8078854475432,0.));
#88465=CARTESIAN_POINT('Ctrl Pts',(-63.8014989507494,28.8078854475432,12.));
#88466=CARTESIAN_POINT('Ctrl Pts',(-63.8091667271232,28.8091580239553,0.));
#88467=CARTESIAN_POINT('Ctrl Pts',(-63.8091667271232,28.8091580239553,12.));
#88468=CARTESIAN_POINT('Ctrl Pts',(-63.8206854735028,28.8110632620957,0.));
#88469=CARTESIAN_POINT('Ctrl Pts',(-63.8206854735028,28.8110632620957,12.));
#88470=CARTESIAN_POINT('Ctrl Pts',(-63.8360779669856,28.8135963263368,0.));
#88471=CARTESIAN_POINT('Ctrl Pts',(-63.8360779669856,28.8135963263368,12.));
#88472=CARTESIAN_POINT('Ctrl Pts',(-63.8553755207487,28.8167505576681,0.));
#88473=CARTESIAN_POINT('Ctrl Pts',(-63.8553755207487,28.8167505576681,12.));
#88474=CARTESIAN_POINT('Ctrl Pts',(-63.8747299825313,28.8198926619858,0.));
#88475=CARTESIAN_POINT('Ctrl Pts',(-63.8747299825313,28.8198926619858,12.));
#88476=CARTESIAN_POINT('Ctrl Pts',(-63.8941412856924,28.823022586318,0.));
#88477=CARTESIAN_POINT('Ctrl Pts',(-63.8941412856924,28.823022586318,12.));
#88478=CARTESIAN_POINT('Ctrl Pts',(-63.9136093063786,28.8261402423291,0.));
#88479=CARTESIAN_POINT('Ctrl Pts',(-63.9136093063786,28.8261402423291,12.));
#88480=CARTESIAN_POINT('Ctrl Pts',(-63.9331338646996,28.8292455077559,0.));
#88481=CARTESIAN_POINT('Ctrl Pts',(-63.9331338646996,28.8292455077559,12.));
#88482=CARTESIAN_POINT('Ctrl Pts',(-63.9527147494423,28.8323382413789,0.));
#88483=CARTESIAN_POINT('Ctrl Pts',(-63.9527147494423,28.8323382413789,12.));
#88484=CARTESIAN_POINT('Ctrl Pts',(-63.9723517369614,28.8354182946601,0.));
#88485=CARTESIAN_POINT('Ctrl Pts',(-63.9723517369614,28.8354182946601,12.));
#88486=CARTESIAN_POINT('Ctrl Pts',(-63.9920446117582,28.8384855243243,0.));
#88487=CARTESIAN_POINT('Ctrl Pts',(-63.9920446117582,28.8384855243243,12.));
#88488=CARTESIAN_POINT('Ctrl Pts',(-64.0117931881298,28.8415398056428,0.));
#88489=CARTESIAN_POINT('Ctrl Pts',(-64.0117931881298,28.8415398056428,12.));
#88490=CARTESIAN_POINT('Ctrl Pts',(-64.0315973031942,28.844581028125,0.));
#88491=CARTESIAN_POINT('Ctrl Pts',(-64.0315973031942,28.844581028125,12.));
#88492=CARTESIAN_POINT('Ctrl Pts',(-64.0514568066637,28.8476090892232,0.));
#88493=CARTESIAN_POINT('Ctrl Pts',(-64.0514568066637,28.8476090892232,12.));
#88494=CARTESIAN_POINT('Ctrl Pts',(-64.0713715523599,28.8506238891093,0.));
#88495=CARTESIAN_POINT('Ctrl Pts',(-64.0713715523599,28.8506238891093,12.));
#88496=CARTESIAN_POINT('Ctrl Pts',(-64.0913413876622,28.8536253241854,0.));
#88497=CARTESIAN_POINT('Ctrl Pts',(-64.0913413876622,28.8536253241854,12.));
#88498=CARTESIAN_POINT('Ctrl Pts',(-64.1113661481965,28.8566132838178,0.));
#88499=CARTESIAN_POINT('Ctrl Pts',(-64.1113661481965,28.8566132838178,12.));
#88500=CARTESIAN_POINT('Ctrl Pts',(-64.1314456633381,28.8595876537148,0.));
#88501=CARTESIAN_POINT('Ctrl Pts',(-64.1314456633381,28.8595876537148,12.));
#88502=CARTESIAN_POINT('Ctrl Pts',(-64.1515797596564,28.8625483180437,0.));
#88503=CARTESIAN_POINT('Ctrl Pts',(-64.1515797596564,28.8625483180437,12.));
#88504=CARTESIAN_POINT('Ctrl Pts',(-64.1717682648685,28.8654951618649,0.));
#88505=CARTESIAN_POINT('Ctrl Pts',(-64.1717682648685,28.8654951618649,12.));
#88506=CARTESIAN_POINT('Ctrl Pts',(-64.1920110123299,28.8684280739014,0.));
#88507=CARTESIAN_POINT('Ctrl Pts',(-64.1920110123299,28.8684280739014,12.));
#88508=CARTESIAN_POINT('Ctrl Pts',(-64.2123078408461,28.8713469464185,0.));
#88509=CARTESIAN_POINT('Ctrl Pts',(-64.2123078408461,28.8713469464185,12.));
#88510=CARTESIAN_POINT('Ctrl Pts',(-64.2326585925252,28.8742516738947,0.));
#88511=CARTESIAN_POINT('Ctrl Pts',(-64.2326585925252,28.8742516738947,12.));
#88512=CARTESIAN_POINT('Ctrl Pts',(-64.2530631112929,28.877142152106,0.));
#88513=CARTESIAN_POINT('Ctrl Pts',(-64.2530631112929,28.877142152106,12.));
#88514=CARTESIAN_POINT('Ctrl Pts',(-64.2735212410711,28.8800182770065,0.));
#88515=CARTESIAN_POINT('Ctrl Pts',(-64.2735212410711,28.8800182770065,12.));
#88516=CARTESIAN_POINT('Ctrl Pts',(-64.2940328242521,28.882879943794,0.));
#88517=CARTESIAN_POINT('Ctrl Pts',(-64.2940328242521,28.882879943794,12.));
#88518=CARTESIAN_POINT('Ctrl Pts',(-64.3145977025037,28.8857270473959,0.));
#88519=CARTESIAN_POINT('Ctrl Pts',(-64.3145977025037,28.8857270473959,12.));
#88520=CARTESIAN_POINT('Ctrl Pts',(-64.3352157174619,28.8885594828926,0.));
#88521=CARTESIAN_POINT('Ctrl Pts',(-64.3352157174619,28.8885594828926,12.));
#88522=CARTESIAN_POINT('Ctrl Pts',(-64.3558867114076,28.8913771459323,0.));
#88523=CARTESIAN_POINT('Ctrl Pts',(-64.3558867114076,28.8913771459323,12.));
#88524=CARTESIAN_POINT('Ctrl Pts',(-64.3766105280688,28.89417993323,0.));
#88525=CARTESIAN_POINT('Ctrl Pts',(-64.3766105280688,28.89417993323,12.));
#88526=CARTESIAN_POINT('Ctrl Pts',(-64.397387012917,28.8969677427504,0.));
#88527=CARTESIAN_POINT('Ctrl Pts',(-64.397387012917,28.8969677427504,12.));
#88528=CARTESIAN_POINT('Ctrl Pts',(-64.4182160127379,28.899740473434,0.));
#88529=CARTESIAN_POINT('Ctrl Pts',(-64.4182160127379,28.899740473434,12.));
#88530=CARTESIAN_POINT('Ctrl Pts',(-64.4390973753634,28.9024980250307,0.));
#88531=CARTESIAN_POINT('Ctrl Pts',(-64.4390973753634,28.9024980250307,12.));
#88532=CARTESIAN_POINT('Ctrl Pts',(-64.4600309493583,28.9052402979062,0.));
#88533=CARTESIAN_POINT('Ctrl Pts',(-64.4600309493583,28.9052402979062,12.));
#88534=CARTESIAN_POINT('Ctrl Pts',(-64.4810165836592,28.9079671928264,0.));
#88535=CARTESIAN_POINT('Ctrl Pts',(-64.4810165836592,28.9079671928264,12.));
#88536=CARTESIAN_POINT('Ctrl Pts',(-64.5020541275951,28.910678610965,0.));
#88537=CARTESIAN_POINT('Ctrl Pts',(-64.5020541275951,28.910678610965,12.));
#88538=CARTESIAN_POINT('Ctrl Pts',(-64.523143431047,28.9133744539949,0.));
#88539=CARTESIAN_POINT('Ctrl Pts',(-64.523143431047,28.9133744539949,12.));
#88540=CARTESIAN_POINT('Ctrl Pts',(-64.5442843445559,28.9160546241538,0.));
#88541=CARTESIAN_POINT('Ctrl Pts',(-64.5442843445559,28.9160546241538,12.));
#88542=CARTESIAN_POINT('Ctrl Pts',(-64.5654767194472,28.9187190243224,0.));
#88543=CARTESIAN_POINT('Ctrl Pts',(-64.5654767194472,28.9187190243224,12.));
#88544=CARTESIAN_POINT('Ctrl Pts',(-64.5867204079426,28.9213675580985,0.));
#88545=CARTESIAN_POINT('Ctrl Pts',(-64.5867204079426,28.9213675580985,12.));
#88546=CARTESIAN_POINT('Ctrl Pts',(-64.6080152631039,28.9240001297542,0.));
#88547=CARTESIAN_POINT('Ctrl Pts',(-64.6080152631039,28.9240001297542,12.));
#88548=CARTESIAN_POINT('Ctrl Pts',(-64.629361138774,28.926616644195,0.));
#88549=CARTESIAN_POINT('Ctrl Pts',(-64.629361138774,28.926616644195,12.));
#88550=CARTESIAN_POINT('Ctrl Pts',(-64.6507578895161,28.9292170069221,0.));
#88551=CARTESIAN_POINT('Ctrl Pts',(-64.6507578895161,28.9292170069221,12.));
#88552=CARTESIAN_POINT('Ctrl Pts',(-64.672205370541,28.9318011239915,0.));
#88553=CARTESIAN_POINT('Ctrl Pts',(-64.672205370541,28.9318011239915,12.));
#88554=CARTESIAN_POINT('Ctrl Pts',(-64.6937034376617,28.9343689019882,0.));
#88555=CARTESIAN_POINT('Ctrl Pts',(-64.6937034376617,28.9343689019882,12.));
#88556=CARTESIAN_POINT('Ctrl Pts',(-64.715251947329,28.9369202480393,0.));
#88557=CARTESIAN_POINT('Ctrl Pts',(-64.715251947329,28.9369202480393,12.));
#88558=CARTESIAN_POINT('Ctrl Pts',(-64.7368507566467,28.9394550698204,0.));
#88559=CARTESIAN_POINT('Ctrl Pts',(-64.7368507566467,28.9394550698204,12.));
#88560=CARTESIAN_POINT('Ctrl Pts',(-64.758499723388,28.9419732755656,0.));
#88561=CARTESIAN_POINT('Ctrl Pts',(-64.758499723388,28.9419732755656,12.));
#88562=CARTESIAN_POINT('Ctrl Pts',(-64.7801987060084,28.944474774081,0.));
#88563=CARTESIAN_POINT('Ctrl Pts',(-64.7801987060084,28.944474774081,12.));
#88564=CARTESIAN_POINT('Ctrl Pts',(-64.8019475636442,28.9469594747431,0.));
#88565=CARTESIAN_POINT('Ctrl Pts',(-64.8019475636442,28.9469594747431,12.));
#88566=CARTESIAN_POINT('Ctrl Pts',(-64.8237461561019,28.9494272874832,0.));
#88567=CARTESIAN_POINT('Ctrl Pts',(-64.8237461561019,28.9494272874832,12.));
#88568=CARTESIAN_POINT('Ctrl Pts',(-64.8455943438423,28.9518781227765,0.));
#88569=CARTESIAN_POINT('Ctrl Pts',(-64.8455943438423,28.9518781227765,12.));
#88570=CARTESIAN_POINT('Ctrl Pts',(-64.8674919879648,28.9543118916328,0.));
#88571=CARTESIAN_POINT('Ctrl Pts',(-64.8674919879648,28.9543118916328,12.));
#88572=CARTESIAN_POINT('Ctrl Pts',(-64.8894389501801,28.9567285055866,0.));
#88573=CARTESIAN_POINT('Ctrl Pts',(-64.8894389501801,28.9567285055866,12.));
#88574=CARTESIAN_POINT('Ctrl Pts',(-64.9114350928125,28.9591278766934,0.));
#88575=CARTESIAN_POINT('Ctrl Pts',(-64.9114350928125,28.9591278766934,12.));
#88576=CARTESIAN_POINT('Ctrl Pts',(-64.9334802788038,28.9615099175249,0.));
#88577=CARTESIAN_POINT('Ctrl Pts',(-64.9334802788038,28.9615099175249,12.));
#88578=CARTESIAN_POINT('Ctrl Pts',(-64.955574371711,28.9638745411677,0.));
#88579=CARTESIAN_POINT('Ctrl Pts',(-64.955574371711,28.9638745411677,12.));
#88580=CARTESIAN_POINT('Ctrl Pts',(-64.9777172357027,28.9662216612217,0.));
#88581=CARTESIAN_POINT('Ctrl Pts',(-64.9777172357027,28.9662216612217,12.));
#88582=CARTESIAN_POINT('Ctrl Pts',(-64.9999087355504,28.9685511918018,0.));
#88583=CARTESIAN_POINT('Ctrl Pts',(-64.9999087355504,28.9685511918018,12.));
#88584=CARTESIAN_POINT('Ctrl Pts',(-65.022148736628,28.97086304753,0.));
#88585=CARTESIAN_POINT('Ctrl Pts',(-65.022148736628,28.97086304753,12.));
#88586=CARTESIAN_POINT('Ctrl Pts',(-65.0444371049082,28.9731571435282,0.));
#88587=CARTESIAN_POINT('Ctrl Pts',(-65.0444371049082,28.9731571435282,12.));
#88588=CARTESIAN_POINT('Ctrl Pts',(-65.0667737069563,28.9754333954135,0.));
#88589=CARTESIAN_POINT('Ctrl Pts',(-65.0667737069563,28.9754333954135,12.));
#88590=CARTESIAN_POINT('Ctrl Pts',(-65.0891584099168,28.9776917192933,0.));
#88591=CARTESIAN_POINT('Ctrl Pts',(-65.0891584099168,28.9776917192933,12.));
#88592=CARTESIAN_POINT('Ctrl Pts',(-65.1115910815037,28.9799320317641,0.));
#88593=CARTESIAN_POINT('Ctrl Pts',(-65.1115910815037,28.9799320317641,12.));
#88594=CARTESIAN_POINT('Ctrl Pts',(-65.1340715900028,28.9821542499042,0.));
#88595=CARTESIAN_POINT('Ctrl Pts',(-65.1340715900028,28.9821542499042,12.));
#88596=CARTESIAN_POINT('Ctrl Pts',(-65.1565998042697,28.9843582912692,0.));
#88597=CARTESIAN_POINT('Ctrl Pts',(-65.1565998042697,28.9843582912692,12.));
#88598=CARTESIAN_POINT('Ctrl Pts',(-65.1791755937256,28.9865440738884,0.));
#88599=CARTESIAN_POINT('Ctrl Pts',(-65.1791755937256,28.9865440738884,12.));
#88600=CARTESIAN_POINT('Ctrl Pts',(-65.2017988283479,28.9887115162633,0.));
#88601=CARTESIAN_POINT('Ctrl Pts',(-65.2017988283479,28.9887115162633,12.));
#88602=CARTESIAN_POINT('Ctrl Pts',(-65.2244693786609,28.9908605373663,0.));
#88603=CARTESIAN_POINT('Ctrl Pts',(-65.2244693786609,28.9908605373663,12.));
#88604=CARTESIAN_POINT('Ctrl Pts',(-65.2471871157397,28.9929910566325,0.));
#88605=CARTESIAN_POINT('Ctrl Pts',(-65.2471871157397,28.9929910566325,12.));
#88606=CARTESIAN_POINT('Ctrl Pts',(-65.2699519112064,28.9951029939557,0.));
#88607=CARTESIAN_POINT('Ctrl Pts',(-65.2699519112064,28.9951029939557,12.));
#88608=CARTESIAN_POINT('Ctrl Pts',(-65.2927636372254,28.9971962696845,0.));
#88609=CARTESIAN_POINT('Ctrl Pts',(-65.2927636372254,28.9971962696845,12.));
#88610=CARTESIAN_POINT('Ctrl Pts',(-65.3156221664916,28.9992708046211,0.));
#88611=CARTESIAN_POINT('Ctrl Pts',(-65.3156221664916,28.9992708046211,12.));
#88612=CARTESIAN_POINT('Ctrl Pts',(-65.3385273722242,29.0013265200185,0.));
#88613=CARTESIAN_POINT('Ctrl Pts',(-65.3385273722242,29.0013265200185,12.));
#88614=CARTESIAN_POINT('Ctrl Pts',(-65.3614791281692,29.003363337573,0.));
#88615=CARTESIAN_POINT('Ctrl Pts',(-65.3614791281692,29.003363337573,12.));
#88616=CARTESIAN_POINT('Ctrl Pts',(-65.3844773085961,29.0053811794207,0.));
#88617=CARTESIAN_POINT('Ctrl Pts',(-65.3844773085961,29.0053811794207,12.));
#88618=CARTESIAN_POINT('Ctrl Pts',(-65.4075217882934,29.0073799681342,0.));
#88619=CARTESIAN_POINT('Ctrl Pts',(-65.4075217882934,29.0073799681342,12.));
#88620=CARTESIAN_POINT('Ctrl Pts',(-65.4306124425562,29.0093596267215,0.));
#88621=CARTESIAN_POINT('Ctrl Pts',(-65.4306124425562,29.0093596267215,12.));
#88622=CARTESIAN_POINT('Ctrl Pts',(-65.4537491471828,29.0113200786239,0.));
#88623=CARTESIAN_POINT('Ctrl Pts',(-65.4537491471828,29.0113200786239,12.));
#88624=CARTESIAN_POINT('Ctrl Pts',(-65.4769317784789,29.013261247709,0.));
#88625=CARTESIAN_POINT('Ctrl Pts',(-65.4769317784789,29.013261247709,12.));
#88626=CARTESIAN_POINT('Ctrl Pts',(-65.5001602132535,29.0151830582675,0.));
#88627=CARTESIAN_POINT('Ctrl Pts',(-65.5001602132535,29.0151830582675,12.));
#88628=CARTESIAN_POINT('Ctrl Pts',(-65.5234343288136,29.0170854350095,0.));
#88629=CARTESIAN_POINT('Ctrl Pts',(-65.5234343288136,29.0170854350095,12.));
#88630=CARTESIAN_POINT('Ctrl Pts',(-65.5467540029514,29.0189683030642,0.));
#88631=CARTESIAN_POINT('Ctrl Pts',(-65.5467540029514,29.0189683030642,12.));
#88632=CARTESIAN_POINT('Ctrl Pts',(-65.5701191139418,29.0208315879764,0.));
#88633=CARTESIAN_POINT('Ctrl Pts',(-65.5701191139418,29.0208315879764,12.));
#88634=CARTESIAN_POINT('Ctrl Pts',(-65.5935295405453,29.0226752157003,0.));
#88635=CARTESIAN_POINT('Ctrl Pts',(-65.5935295405453,29.0226752157003,12.));
#88636=CARTESIAN_POINT('Ctrl Pts',(-65.6169851620046,29.0244991125959,0.));
#88637=CARTESIAN_POINT('Ctrl Pts',(-65.6169851620046,29.0244991125959,12.));
#88638=CARTESIAN_POINT('Ctrl Pts',(-65.6404858580403,29.0263032054266,0.));
#88639=CARTESIAN_POINT('Ctrl Pts',(-65.6404858580403,29.0263032054266,12.));
#88640=CARTESIAN_POINT('Ctrl Pts',(-65.6640315088388,29.0280874213596,0.));
#88641=CARTESIAN_POINT('Ctrl Pts',(-65.6640315088388,29.0280874213596,12.));
#88642=CARTESIAN_POINT('Ctrl Pts',(-65.6876219950493,29.0298516879611,0.));
#88643=CARTESIAN_POINT('Ctrl Pts',(-65.6876219950493,29.0298516879611,12.));
#88644=CARTESIAN_POINT('Ctrl Pts',(-65.7112571977891,29.0315959331919,0.));
#88645=CARTESIAN_POINT('Ctrl Pts',(-65.7112571977891,29.0315959331919,12.));
#88646=CARTESIAN_POINT('Ctrl Pts',(-65.7349369986384,29.0333200854027,0.));
#88647=CARTESIAN_POINT('Ctrl Pts',(-65.7349369986384,29.0333200854027,12.));
#88648=CARTESIAN_POINT('Ctrl Pts',(-65.7586612796368,29.035024073333,0.));
#88649=CARTESIAN_POINT('Ctrl Pts',(-65.7586612796368,29.035024073333,12.));
#88650=CARTESIAN_POINT('Ctrl Pts',(-65.7824299232705,29.0367078261103,0.));
#88651=CARTESIAN_POINT('Ctrl Pts',(-65.7824299232705,29.0367078261103,12.));
#88652=CARTESIAN_POINT('Ctrl Pts',(-65.8062428124713,29.0383712732469,0.));
#88653=CARTESIAN_POINT('Ctrl Pts',(-65.8062428124713,29.0383712732469,12.));
#88654=CARTESIAN_POINT('Ctrl Pts',(-65.8300998306191,29.0400143446338,0.));
#88655=CARTESIAN_POINT('Ctrl Pts',(-65.8300998306191,29.0400143446338,12.));
#88656=CARTESIAN_POINT('Ctrl Pts',(-65.854000861539,29.0416369705375,0.));
#88657=CARTESIAN_POINT('Ctrl Pts',(-65.854000861539,29.0416369705375,12.));
#88658=CARTESIAN_POINT('Ctrl Pts',(-65.8779457894961,29.0432390815978,0.));
#88659=CARTESIAN_POINT('Ctrl Pts',(-65.8779457894961,29.0432390815978,12.));
#88660=CARTESIAN_POINT('Ctrl Pts',(-65.9019344991854,29.0448206088288,0.));
#88661=CARTESIAN_POINT('Ctrl Pts',(-65.9019344991854,29.0448206088288,12.));
#88662=CARTESIAN_POINT('Ctrl Pts',(-65.9259668757307,29.0463814836157,0.));
#88663=CARTESIAN_POINT('Ctrl Pts',(-65.9259668757307,29.0463814836157,12.));
#88664=CARTESIAN_POINT('Ctrl Pts',(-65.9500428046868,29.0479216377081,0.));
#88665=CARTESIAN_POINT('Ctrl Pts',(-65.9500428046868,29.0479216377081,12.));
#88666=CARTESIAN_POINT('Ctrl Pts',(-65.974162172037,29.0494410032172,0.));
#88667=CARTESIAN_POINT('Ctrl Pts',(-65.974162172037,29.0494410032172,12.));
#88668=CARTESIAN_POINT('Ctrl Pts',(-65.9983248641879,29.0509395126142,0.));
#88669=CARTESIAN_POINT('Ctrl Pts',(-65.9983248641879,29.0509395126142,12.));
#88670=CARTESIAN_POINT('Ctrl Pts',(-66.0225307679591,29.0524170987307,0.));
#88671=CARTESIAN_POINT('Ctrl Pts',(-66.0225307679591,29.0524170987307,12.));
#88672=CARTESIAN_POINT('Ctrl Pts',(-66.0467797705815,29.0538736947552,0.));
#88673=CARTESIAN_POINT('Ctrl Pts',(-66.0467797705815,29.0538736947552,12.));
#88674=CARTESIAN_POINT('Ctrl Pts',(-66.0710717597009,29.0553092342278,0.));
#88675=CARTESIAN_POINT('Ctrl Pts',(-66.0710717597009,29.0553092342278,12.));
#88676=CARTESIAN_POINT('Ctrl Pts',(-66.0954066233754,29.0567236510373,0.));
#88677=CARTESIAN_POINT('Ctrl Pts',(-66.0954066233754,29.0567236510373,12.));
#88678=CARTESIAN_POINT('Ctrl Pts',(-66.1197842500711,29.0581168794189,0.));
#88679=CARTESIAN_POINT('Ctrl Pts',(-66.1197842500711,29.0581168794189,12.));
#88680=CARTESIAN_POINT('Ctrl Pts',(-66.1442045286516,29.0594888539555,0.));
#88681=CARTESIAN_POINT('Ctrl Pts',(-66.1442045286516,29.0594888539555,12.));
#88682=CARTESIAN_POINT('Ctrl Pts',(-66.1686673483755,29.0608395095745,0.));
#88683=CARTESIAN_POINT('Ctrl Pts',(-66.1686673483755,29.0608395095745,12.));
#88684=CARTESIAN_POINT('Ctrl Pts',(-66.1931725989008,29.062168781542,0.));
#88685=CARTESIAN_POINT('Ctrl Pts',(-66.1931725989008,29.062168781542,12.));
#88686=CARTESIAN_POINT('Ctrl Pts',(-66.2177201702819,29.0634766054599,0.));
#88687=CARTESIAN_POINT('Ctrl Pts',(-66.2177201702819,29.0634766054599,12.));
#88688=CARTESIAN_POINT('Ctrl Pts',(-66.2423099529668,29.0647629172645,0.));
#88689=CARTESIAN_POINT('Ctrl Pts',(-66.2423099529668,29.0647629172645,12.));
#88690=CARTESIAN_POINT('Ctrl Pts',(-66.2669418377866,29.0660276532272,0.));
#88691=CARTESIAN_POINT('Ctrl Pts',(-66.2669418377866,29.0660276532272,12.));
#88692=CARTESIAN_POINT('Ctrl Pts',(-66.2916157159528,29.0672707499527,0.));
#88693=CARTESIAN_POINT('Ctrl Pts',(-66.2916157159528,29.0672707499527,12.));
#88694=CARTESIAN_POINT('Ctrl Pts',(-66.3163314790607,29.0684921443718,0.));
#88695=CARTESIAN_POINT('Ctrl Pts',(-66.3163314790607,29.0684921443718,12.));
#88696=CARTESIAN_POINT('Ctrl Pts',(-66.3410890190879,29.0696917737397,0.));
#88697=CARTESIAN_POINT('Ctrl Pts',(-66.3410890190879,29.0696917737397,12.));
#88698=CARTESIAN_POINT('Ctrl Pts',(-66.3658882283906,29.0708695756335,0.));
#88699=CARTESIAN_POINT('Ctrl Pts',(-66.3658882283906,29.0708695756335,12.));
#88700=CARTESIAN_POINT('Ctrl Pts',(-66.3907289996942,29.0720254879535,0.));
#88701=CARTESIAN_POINT('Ctrl Pts',(-66.3907289996942,29.0720254879535,12.));
#88702=CARTESIAN_POINT('Ctrl Pts',(-66.4156112260904,29.0731594489218,0.));
#88703=CARTESIAN_POINT('Ctrl Pts',(-66.4156112260904,29.0731594489218,12.));
#88704=CARTESIAN_POINT('Ctrl Pts',(-66.4405348010404,29.0742713970762,0.));
#88705=CARTESIAN_POINT('Ctrl Pts',(-66.4405348010404,29.0742713970762,12.));
#88706=CARTESIAN_POINT('Ctrl Pts',(-66.4654996183739,29.0753612712669,0.));
#88707=CARTESIAN_POINT('Ctrl Pts',(-66.4654996183739,29.0753612712669,12.));
#88708=CARTESIAN_POINT('Ctrl Pts',(-66.4905055722864,29.0764290106553,0.));
#88709=CARTESIAN_POINT('Ctrl Pts',(-66.4905055722864,29.0764290106553,12.));
#88710=CARTESIAN_POINT('Ctrl Pts',(-66.5155525573308,29.0774745547146,0.));
#88711=CARTESIAN_POINT('Ctrl Pts',(-66.5155525573308,29.0774745547146,12.));
#88712=CARTESIAN_POINT('Ctrl Pts',(-66.5406404684116,29.0784978432294,0.));
#88713=CARTESIAN_POINT('Ctrl Pts',(-66.5406404684116,29.0784978432294,12.));
#88714=CARTESIAN_POINT('Ctrl Pts',(-66.5657692007894,29.0794988162892,0.));
#88715=CARTESIAN_POINT('Ctrl Pts',(-66.5657692007894,29.0794988162892,12.));
#88716=CARTESIAN_POINT('Ctrl Pts',(-66.5909386500796,29.0804774142852,0.));
#88717=CARTESIAN_POINT('Ctrl Pts',(-66.5909386500796,29.0804774142852,12.));
#88718=CARTESIAN_POINT('Ctrl Pts',(-66.6161487122504,29.0814335779085,0.));
#88719=CARTESIAN_POINT('Ctrl Pts',(-66.6161487122504,29.0814335779085,12.));
#88720=CARTESIAN_POINT('Ctrl Pts',(-66.6413992836148,29.0823672481508,0.));
#88721=CARTESIAN_POINT('Ctrl Pts',(-66.6413992836148,29.0823672481508,12.));
#88722=CARTESIAN_POINT('Ctrl Pts',(-66.6666902608246,29.0832783663048,0.));
#88723=CARTESIAN_POINT('Ctrl Pts',(-66.6666902608246,29.0832783663048,12.));
#88724=CARTESIAN_POINT('Ctrl Pts',(-66.6920215408744,29.0841668739585,0.));
#88725=CARTESIAN_POINT('Ctrl Pts',(-66.6920215408744,29.0841668739585,12.));
#88726=CARTESIAN_POINT('Ctrl Pts',(-66.7173930211015,29.0850327129913,0.));
#88727=CARTESIAN_POINT('Ctrl Pts',(-66.7173930211015,29.0850327129913,12.));
#88728=CARTESIAN_POINT('Ctrl Pts',(-66.7428045991841,29.0858758255729,0.));
#88729=CARTESIAN_POINT('Ctrl Pts',(-66.7428045991841,29.0858758255729,12.));
#88730=CARTESIAN_POINT('Ctrl Pts',(-66.7682561731349,29.0866961541629,0.));
#88731=CARTESIAN_POINT('Ctrl Pts',(-66.7682561731349,29.0866961541629,12.));
#88732=CARTESIAN_POINT('Ctrl Pts',(-66.7937476412941,29.0874936415138,0.));
#88733=CARTESIAN_POINT('Ctrl Pts',(-66.7937476412941,29.0874936415138,12.));
#88734=CARTESIAN_POINT('Ctrl Pts',(-66.8192789023323,29.0882682306636,0.));
#88735=CARTESIAN_POINT('Ctrl Pts',(-66.8192789023323,29.0882682306636,12.));
#88736=CARTESIAN_POINT('Ctrl Pts',(-66.8448498552508,29.0890198649327,0.));
#88737=CARTESIAN_POINT('Ctrl Pts',(-66.8448498552508,29.0890198649327,12.));
#88738=CARTESIAN_POINT('Ctrl Pts',(-66.8704603993794,29.0897484879207,0.));
#88739=CARTESIAN_POINT('Ctrl Pts',(-66.8704603993794,29.0897484879207,12.));
#88740=CARTESIAN_POINT('Ctrl Pts',(-66.8961104343703,29.0904540435063,0.));
#88741=CARTESIAN_POINT('Ctrl Pts',(-66.8961104343703,29.0904540435063,12.));
#88742=CARTESIAN_POINT('Ctrl Pts',(-66.9217998601881,29.0911364758484,0.));
#88743=CARTESIAN_POINT('Ctrl Pts',(-66.9217998601881,29.0911364758484,12.));
#88744=CARTESIAN_POINT('Ctrl Pts',(-66.9475285771133,29.0917957293824,0.));
#88745=CARTESIAN_POINT('Ctrl Pts',(-66.9475285771133,29.0917957293824,12.));
#88746=CARTESIAN_POINT('Ctrl Pts',(-66.9732964857467,29.092431748817,0.));
#88747=CARTESIAN_POINT('Ctrl Pts',(-66.9732964857467,29.092431748817,12.));
#88748=CARTESIAN_POINT('Ctrl Pts',(-66.9991034870084,29.0930444791329,0.));
#88749=CARTESIAN_POINT('Ctrl Pts',(-66.9991034870084,29.0930444791329,12.));
#88750=CARTESIAN_POINT('Ctrl Pts',(-67.0249494821361,29.0936338655828,0.));
#88751=CARTESIAN_POINT('Ctrl Pts',(-67.0249494821361,29.0936338655828,12.));
#88752=CARTESIAN_POINT('Ctrl Pts',(-67.0508343726771,29.0941998536957,0.));
#88753=CARTESIAN_POINT('Ctrl Pts',(-67.0508343726771,29.0941998536957,12.));
#88754=CARTESIAN_POINT('Ctrl Pts',(-67.0767580604872,29.0947423892725,0.));
#88755=CARTESIAN_POINT('Ctrl Pts',(-67.0767580604872,29.0947423892725,12.));
#88756=CARTESIAN_POINT('Ctrl Pts',(-67.1027204477304,29.0952614183777,0.));
#88757=CARTESIAN_POINT('Ctrl Pts',(-67.1027204477304,29.0952614183777,12.));
#88758=CARTESIAN_POINT('Ctrl Pts',(-67.1287214368743,29.0957568873357,0.));
#88759=CARTESIAN_POINT('Ctrl Pts',(-67.1287214368743,29.0957568873357,12.));
#88760=CARTESIAN_POINT('Ctrl Pts',(-67.1547609306845,29.0962287427274,0.));
#88761=CARTESIAN_POINT('Ctrl Pts',(-67.1547609306845,29.0962287427274,12.));
#88762=CARTESIAN_POINT('Ctrl Pts',(-67.1808388322116,29.0966769313893,0.));
#88763=CARTESIAN_POINT('Ctrl Pts',(-67.1808388322116,29.0966769313893,12.));
#88764=CARTESIAN_POINT('Ctrl Pts',(-67.2069550447895,29.0971014004134,0.));
#88765=CARTESIAN_POINT('Ctrl Pts',(-67.2069550447895,29.0971014004134,12.));
#88766=CARTESIAN_POINT('Ctrl Pts',(-67.2331094720482,29.0975020971473,0.));
#88767=CARTESIAN_POINT('Ctrl Pts',(-67.2331094720482,29.0975020971473,12.));
#88768=CARTESIAN_POINT('Ctrl Pts',(-67.2593020179216,29.0978789691965,0.));
#88769=CARTESIAN_POINT('Ctrl Pts',(-67.2593020179216,29.0978789691965,12.));
#88770=CARTESIAN_POINT('Ctrl Pts',(-67.2855325866516,29.0982319644276,0.));
#88771=CARTESIAN_POINT('Ctrl Pts',(-67.2855325866516,29.0982319644276,12.));
#88772=CARTESIAN_POINT('Ctrl Pts',(-67.311801082791,29.0985610309768,0.));
#88773=CARTESIAN_POINT('Ctrl Pts',(-67.311801082791,29.0985610309768,12.));
#88774=CARTESIAN_POINT('Ctrl Pts',(-67.3381074112013,29.0988661172526,0.));
#88775=CARTESIAN_POINT('Ctrl Pts',(-67.3381074112013,29.0988661172526,12.));
#88776=CARTESIAN_POINT('Ctrl Pts',(-67.3644514770373,29.0991471719172,0.));
#88777=CARTESIAN_POINT('Ctrl Pts',(-67.3644514770373,29.0991471719172,12.));
#88778=CARTESIAN_POINT('Ctrl Pts',(-67.3908331857313,29.0994041438715,0.));
#88779=CARTESIAN_POINT('Ctrl Pts',(-67.3908331857313,29.0994041438715,12.));
#88780=CARTESIAN_POINT('Ctrl Pts',(-67.4172524429726,29.0996369822418,0.));
#88781=CARTESIAN_POINT('Ctrl Pts',(-67.4172524429726,29.0996369822418,12.));
#88782=CARTESIAN_POINT('Ctrl Pts',(-67.4437091546869,29.0998456363687,0.));
#88783=CARTESIAN_POINT('Ctrl Pts',(-67.4437091546869,29.0998456363687,12.));
#88784=CARTESIAN_POINT('Ctrl Pts',(-67.4702032270063,29.1000300557961,0.));
#88785=CARTESIAN_POINT('Ctrl Pts',(-67.4702032270063,29.1000300557961,12.));
#88786=CARTESIAN_POINT('Ctrl Pts',(-67.496734566311,29.1001901902915,0.));
#88787=CARTESIAN_POINT('Ctrl Pts',(-67.496734566311,29.1001901902915,12.));
#88788=CARTESIAN_POINT('Ctrl Pts',(-67.5233030792714,29.1003259898686,0.));
#88789=CARTESIAN_POINT('Ctrl Pts',(-67.5233030792714,29.1003259898686,12.));
#88790=CARTESIAN_POINT('Ctrl Pts',(-67.5499086728891,29.1004374048149,0.));
#88791=CARTESIAN_POINT('Ctrl Pts',(-67.5499086728891,29.1004374048149,12.));
#88792=CARTESIAN_POINT('Ctrl Pts',(-67.5765512545277,29.1005243857137,0.));
#88793=CARTESIAN_POINT('Ctrl Pts',(-67.5765512545277,29.1005243857137,12.));
#88794=CARTESIAN_POINT('Ctrl Pts',(-67.6032307319614,29.1005868834863,0.));
#88795=CARTESIAN_POINT('Ctrl Pts',(-67.6032307319614,29.1005868834863,12.));
#88796=CARTESIAN_POINT('Ctrl Pts',(-67.6299470133286,29.1006248493576,0.));
#88797=CARTESIAN_POINT('Ctrl Pts',(-67.6299470133286,29.1006248493576,12.));
#88798=CARTESIAN_POINT('Ctrl Pts',(-67.6567000070319,29.1006382347812,0.));
#88799=CARTESIAN_POINT('Ctrl Pts',(-67.6567000070319,29.1006382347812,12.));
#88800=CARTESIAN_POINT('Ctrl Pts',(-67.6834896216458,29.1006269913747,0.));
#88801=CARTESIAN_POINT('Ctrl Pts',(-67.6834896216458,29.1006269913747,12.));
#88802=CARTESIAN_POINT('Ctrl Pts',(-67.7103157658297,29.1005910708624,0.));
#88803=CARTESIAN_POINT('Ctrl Pts',(-67.7103157658297,29.1005910708624,12.));
#88804=CARTESIAN_POINT('Ctrl Pts',(-67.7371783482039,29.1005304249989,0.));
#88805=CARTESIAN_POINT('Ctrl Pts',(-67.7371783482039,29.1005304249989,12.));
#88806=CARTESIAN_POINT('Ctrl Pts',(-67.7640772773397,29.1004450055647,0.));
#88807=CARTESIAN_POINT('Ctrl Pts',(-67.7640772773397,29.1004450055647,12.));
#88808=CARTESIAN_POINT('Ctrl Pts',(-67.7910124620149,29.1003347645299,0.));
#88809=CARTESIAN_POINT('Ctrl Pts',(-67.7910124620149,29.1003347645299,12.));
#88810=CARTESIAN_POINT('Ctrl Pts',(-67.8179838114109,29.1001996541846,0.));
#88811=CARTESIAN_POINT('Ctrl Pts',(-67.8179838114109,29.1001996541846,12.));
#88812=CARTESIAN_POINT('Ctrl Pts',(-67.844991235333,29.1000396272868,0.));
#88813=CARTESIAN_POINT('Ctrl Pts',(-67.844991235333,29.1000396272868,12.));
#88814=CARTESIAN_POINT('Ctrl Pts',(-67.8720346444111,29.0998546372027,0.));
#88815=CARTESIAN_POINT('Ctrl Pts',(-67.8720346444111,29.0998546372027,12.));
#88816=CARTESIAN_POINT('Ctrl Pts',(-67.8991139503168,29.0996446380617,0.));
#88817=CARTESIAN_POINT('Ctrl Pts',(-67.8991139503168,29.0996446380617,12.));
#88818=CARTESIAN_POINT('Ctrl Pts',(-67.9262290652797,29.0994095844208,0.));
#88819=CARTESIAN_POINT('Ctrl Pts',(-67.9262290652797,29.0994095844208,12.));
#88820=CARTESIAN_POINT('Ctrl Pts',(-67.9533799016122,29.0991494309394,0.));
#88821=CARTESIAN_POINT('Ctrl Pts',(-67.9533799016122,29.0991494309394,12.));
#88822=CARTESIAN_POINT('Ctrl Pts',(-67.9805663711845,29.0988641320243,0.));
#88823=CARTESIAN_POINT('Ctrl Pts',(-67.9805663711845,29.0988641320243,12.));
#88824=CARTESIAN_POINT('Ctrl Pts',(-68.0077883850136,29.0985536415537,0.));
#88825=CARTESIAN_POINT('Ctrl Pts',(-68.0077883850136,29.0985536415537,12.));
#88826=CARTESIAN_POINT('Ctrl Pts',(-68.0350458525589,29.0982179124112,0.));
#88827=CARTESIAN_POINT('Ctrl Pts',(-68.0350458525589,29.0982179124112,12.));
#88828=CARTESIAN_POINT('Ctrl Pts',(-68.0623386822917,29.0978568968677,0.));
#88829=CARTESIAN_POINT('Ctrl Pts',(-68.0623386822917,29.0978568968677,12.));
#88830=CARTESIAN_POINT('Ctrl Pts',(-68.089666782962,29.0974705474279,0.));
#88831=CARTESIAN_POINT('Ctrl Pts',(-68.089666782962,29.0974705474279,12.));
#88832=CARTESIAN_POINT('Ctrl Pts',(-68.1170300647019,29.097058817574,0.));
#88833=CARTESIAN_POINT('Ctrl Pts',(-68.1170300647019,29.097058817574,12.));
#88834=CARTESIAN_POINT('Ctrl Pts',(-68.1444284400734,29.096621662474,0.));
#88835=CARTESIAN_POINT('Ctrl Pts',(-68.1444284400734,29.096621662474,12.));
#88836=CARTESIAN_POINT('Ctrl Pts',(-68.1718618254221,29.0961590399023,0.));
#88837=CARTESIAN_POINT('Ctrl Pts',(-68.1718618254221,29.0961590399023,12.));
#88838=CARTESIAN_POINT('Ctrl Pts',(-68.1993301411959,29.0956709104588,0.));
#88839=CARTESIAN_POINT('Ctrl Pts',(-68.1993301411959,29.0956709104588,12.));
#88840=CARTESIAN_POINT('Ctrl Pts',(-68.22683330895,29.0951572355352,0.));
#88841=CARTESIAN_POINT('Ctrl Pts',(-68.22683330895,29.0951572355352,12.));
#88842=CARTESIAN_POINT('Ctrl Pts',(-68.2543712489815,29.0946179757132,0.));
#88843=CARTESIAN_POINT('Ctrl Pts',(-68.2543712489815,29.0946179757132,12.));
#88844=CARTESIAN_POINT('Ctrl Pts',(-68.2819438775932,29.0940530889141,0.));
#88845=CARTESIAN_POINT('Ctrl Pts',(-68.2819438775932,29.0940530889141,12.));
#88846=CARTESIAN_POINT('Ctrl Pts',(-68.3095511047852,29.0934625288442,0.));
#88847=CARTESIAN_POINT('Ctrl Pts',(-68.3095511047852,29.0934625288442,12.));
#88848=CARTESIAN_POINT('Ctrl Pts',(-68.3371928310351,29.0928462428218,0.));
#88849=CARTESIAN_POINT('Ctrl Pts',(-68.3371928310351,29.0928462428218,12.));
#88850=CARTESIAN_POINT('Ctrl Pts',(-68.3648689519188,29.0922041749393,0.));
#88851=CARTESIAN_POINT('Ctrl Pts',(-68.3648689519188,29.0922041749393,12.));
#88852=CARTESIAN_POINT('Ctrl Pts',(-68.3925793638241,29.091536269955,0.));
#88853=CARTESIAN_POINT('Ctrl Pts',(-68.3925793638241,29.091536269955,12.));
#88854=CARTESIAN_POINT('Ctrl Pts',(-68.4203239694742,29.0908424770941,0.));
#88855=CARTESIAN_POINT('Ctrl Pts',(-68.4203239694742,29.0908424770941,12.));
#88856=CARTESIAN_POINT('Ctrl Pts',(-68.4481026830845,29.0901227535274,0.));
#88857=CARTESIAN_POINT('Ctrl Pts',(-68.4481026830845,29.0901227535274,12.));
#88858=CARTESIAN_POINT('Ctrl Pts',(-68.4759154367582,29.0893770688807,0.));
#88859=CARTESIAN_POINT('Ctrl Pts',(-68.4759154367582,29.0893770688807,12.));
#88860=CARTESIAN_POINT('Ctrl Pts',(-68.5037621823575,29.0886054060334,0.));
#88861=CARTESIAN_POINT('Ctrl Pts',(-68.5037621823575,29.0886054060334,12.));
#88862=CARTESIAN_POINT('Ctrl Pts',(-68.5316428874729,29.0878077570819,0.));
#88863=CARTESIAN_POINT('Ctrl Pts',(-68.5316428874729,29.0878077570819,12.));
#88864=CARTESIAN_POINT('Ctrl Pts',(-68.5539746037961,29.0871488478365,0.));
#88865=CARTESIAN_POINT('Ctrl Pts',(-68.5539746037961,29.0871488478365,12.));
#88866=CARTESIAN_POINT('Ctrl Pts',(-68.5707386600286,29.0866429721959,0.));
#88867=CARTESIAN_POINT('Ctrl Pts',(-68.5707386600286,29.0866429721959,12.));
#88868=CARTESIAN_POINT('Ctrl Pts',(-68.5819214834609,29.0863005247789,0.));
#88869=CARTESIAN_POINT('Ctrl Pts',(-68.5819214834609,29.0863005247789,12.));
#88870=CARTESIAN_POINT('Ctrl Pts',(-68.5875145916629,29.0861280018229,0.));
#88871=CARTESIAN_POINT('Ctrl Pts',(-68.5875145916629,29.0861280018229,12.));
#88872=CARTESIAN_POINT('',(-63.7976679095314,28.8072485549236,0.));
#88873=CARTESIAN_POINT('Ctrl Pts',(-63.7976679095314,28.8072485549236,0.));
#88874=CARTESIAN_POINT('Ctrl Pts',(-63.8014989507494,28.8078854475432,0.));
#88875=CARTESIAN_POINT('Ctrl Pts',(-63.8091667271232,28.8091580239553,0.));
#88876=CARTESIAN_POINT('Ctrl Pts',(-63.8206854735028,28.8110632620957,0.));
#88877=CARTESIAN_POINT('Ctrl Pts',(-63.8360779669856,28.8135963263368,0.));
#88878=CARTESIAN_POINT('Ctrl Pts',(-63.8553755207487,28.8167505576681,0.));
#88879=CARTESIAN_POINT('Ctrl Pts',(-63.8747299825313,28.8198926619858,0.));
#88880=CARTESIAN_POINT('Ctrl Pts',(-63.8941412856924,28.823022586318,0.));
#88881=CARTESIAN_POINT('Ctrl Pts',(-63.9136093063786,28.8261402423291,0.));
#88882=CARTESIAN_POINT('Ctrl Pts',(-63.9331338646996,28.8292455077559,0.));
#88883=CARTESIAN_POINT('Ctrl Pts',(-63.9527147494423,28.8323382413789,0.));
#88884=CARTESIAN_POINT('Ctrl Pts',(-63.9723517369614,28.8354182946601,0.));
#88885=CARTESIAN_POINT('Ctrl Pts',(-63.9920446117582,28.8384855243243,0.));
#88886=CARTESIAN_POINT('Ctrl Pts',(-64.0117931881298,28.8415398056428,0.));
#88887=CARTESIAN_POINT('Ctrl Pts',(-64.0315973031942,28.844581028125,0.));
#88888=CARTESIAN_POINT('Ctrl Pts',(-64.0514568066637,28.8476090892232,0.));
#88889=CARTESIAN_POINT('Ctrl Pts',(-64.0713715523599,28.8506238891093,0.));
#88890=CARTESIAN_POINT('Ctrl Pts',(-64.0913413876622,28.8536253241854,0.));
#88891=CARTESIAN_POINT('Ctrl Pts',(-64.1113661481965,28.8566132838178,0.));
#88892=CARTESIAN_POINT('Ctrl Pts',(-64.1314456633381,28.8595876537148,0.));
#88893=CARTESIAN_POINT('Ctrl Pts',(-64.1515797596564,28.8625483180437,0.));
#88894=CARTESIAN_POINT('Ctrl Pts',(-64.1717682648685,28.8654951618649,0.));
#88895=CARTESIAN_POINT('Ctrl Pts',(-64.1920110123299,28.8684280739014,0.));
#88896=CARTESIAN_POINT('Ctrl Pts',(-64.2123078408461,28.8713469464185,0.));
#88897=CARTESIAN_POINT('Ctrl Pts',(-64.2326585925252,28.8742516738947,0.));
#88898=CARTESIAN_POINT('Ctrl Pts',(-64.2530631112929,28.877142152106,0.));
#88899=CARTESIAN_POINT('Ctrl Pts',(-64.2735212410711,28.8800182770065,0.));
#88900=CARTESIAN_POINT('Ctrl Pts',(-64.2940328242521,28.882879943794,0.));
#88901=CARTESIAN_POINT('Ctrl Pts',(-64.3145977025037,28.8857270473959,0.));
#88902=CARTESIAN_POINT('Ctrl Pts',(-64.3352157174619,28.8885594828926,0.));
#88903=CARTESIAN_POINT('Ctrl Pts',(-64.3558867114076,28.8913771459323,0.));
#88904=CARTESIAN_POINT('Ctrl Pts',(-64.3766105280688,28.89417993323,0.));
#88905=CARTESIAN_POINT('Ctrl Pts',(-64.397387012917,28.8969677427504,0.));
#88906=CARTESIAN_POINT('Ctrl Pts',(-64.4182160127379,28.899740473434,0.));
#88907=CARTESIAN_POINT('Ctrl Pts',(-64.4390973753634,28.9024980250307,0.));
#88908=CARTESIAN_POINT('Ctrl Pts',(-64.4600309493583,28.9052402979062,0.));
#88909=CARTESIAN_POINT('Ctrl Pts',(-64.4810165836592,28.9079671928264,0.));
#88910=CARTESIAN_POINT('Ctrl Pts',(-64.5020541275951,28.910678610965,0.));
#88911=CARTESIAN_POINT('Ctrl Pts',(-64.523143431047,28.9133744539949,0.));
#88912=CARTESIAN_POINT('Ctrl Pts',(-64.5442843445559,28.9160546241538,0.));
#88913=CARTESIAN_POINT('Ctrl Pts',(-64.5654767194472,28.9187190243224,0.));
#88914=CARTESIAN_POINT('Ctrl Pts',(-64.5867204079426,28.9213675580985,0.));
#88915=CARTESIAN_POINT('Ctrl Pts',(-64.6080152631039,28.9240001297542,0.));
#88916=CARTESIAN_POINT('Ctrl Pts',(-64.629361138774,28.926616644195,0.));
#88917=CARTESIAN_POINT('Ctrl Pts',(-64.6507578895161,28.9292170069221,0.));
#88918=CARTESIAN_POINT('Ctrl Pts',(-64.672205370541,28.9318011239915,0.));
#88919=CARTESIAN_POINT('Ctrl Pts',(-64.6937034376617,28.9343689019882,0.));
#88920=CARTESIAN_POINT('Ctrl Pts',(-64.715251947329,28.9369202480393,0.));
#88921=CARTESIAN_POINT('Ctrl Pts',(-64.7368507566467,28.9394550698204,0.));
#88922=CARTESIAN_POINT('Ctrl Pts',(-64.758499723388,28.9419732755656,0.));
#88923=CARTESIAN_POINT('Ctrl Pts',(-64.7801987060084,28.944474774081,0.));
#88924=CARTESIAN_POINT('Ctrl Pts',(-64.8019475636442,28.9469594747431,0.));
#88925=CARTESIAN_POINT('Ctrl Pts',(-64.8237461561019,28.9494272874832,0.));
#88926=CARTESIAN_POINT('Ctrl Pts',(-64.8455943438423,28.9518781227765,0.));
#88927=CARTESIAN_POINT('Ctrl Pts',(-64.8674919879648,28.9543118916328,0.));
#88928=CARTESIAN_POINT('Ctrl Pts',(-64.8894389501801,28.9567285055866,0.));
#88929=CARTESIAN_POINT('Ctrl Pts',(-64.9114350928125,28.9591278766934,0.));
#88930=CARTESIAN_POINT('Ctrl Pts',(-64.9334802788038,28.9615099175249,0.));
#88931=CARTESIAN_POINT('Ctrl Pts',(-64.955574371711,28.9638745411677,0.));
#88932=CARTESIAN_POINT('Ctrl Pts',(-64.9777172357027,28.9662216612217,0.));
#88933=CARTESIAN_POINT('Ctrl Pts',(-64.9999087355504,28.9685511918018,0.));
#88934=CARTESIAN_POINT('Ctrl Pts',(-65.022148736628,28.97086304753,0.));
#88935=CARTESIAN_POINT('Ctrl Pts',(-65.0444371049082,28.9731571435282,0.));
#88936=CARTESIAN_POINT('Ctrl Pts',(-65.0667737069563,28.9754333954135,0.));
#88937=CARTESIAN_POINT('Ctrl Pts',(-65.0891584099168,28.9776917192933,0.));
#88938=CARTESIAN_POINT('Ctrl Pts',(-65.1115910815037,28.9799320317641,0.));
#88939=CARTESIAN_POINT('Ctrl Pts',(-65.1340715900028,28.9821542499042,0.));
#88940=CARTESIAN_POINT('Ctrl Pts',(-65.1565998042697,28.9843582912692,0.));
#88941=CARTESIAN_POINT('Ctrl Pts',(-65.1791755937256,28.9865440738884,0.));
#88942=CARTESIAN_POINT('Ctrl Pts',(-65.2017988283479,28.9887115162633,0.));
#88943=CARTESIAN_POINT('Ctrl Pts',(-65.2244693786609,28.9908605373663,0.));
#88944=CARTESIAN_POINT('Ctrl Pts',(-65.2471871157397,28.9929910566325,0.));
#88945=CARTESIAN_POINT('Ctrl Pts',(-65.2699519112064,28.9951029939557,0.));
#88946=CARTESIAN_POINT('Ctrl Pts',(-65.2927636372254,28.9971962696845,0.));
#88947=CARTESIAN_POINT('Ctrl Pts',(-65.3156221664916,28.9992708046211,0.));
#88948=CARTESIAN_POINT('Ctrl Pts',(-65.3385273722242,29.0013265200185,0.));
#88949=CARTESIAN_POINT('Ctrl Pts',(-65.3614791281692,29.003363337573,0.));
#88950=CARTESIAN_POINT('Ctrl Pts',(-65.3844773085961,29.0053811794207,0.));
#88951=CARTESIAN_POINT('Ctrl Pts',(-65.4075217882934,29.0073799681342,0.));
#88952=CARTESIAN_POINT('Ctrl Pts',(-65.4306124425562,29.0093596267215,0.));
#88953=CARTESIAN_POINT('Ctrl Pts',(-65.4537491471828,29.0113200786239,0.));
#88954=CARTESIAN_POINT('Ctrl Pts',(-65.4769317784789,29.013261247709,0.));
#88955=CARTESIAN_POINT('Ctrl Pts',(-65.5001602132535,29.0151830582675,0.));
#88956=CARTESIAN_POINT('Ctrl Pts',(-65.5234343288136,29.0170854350095,0.));
#88957=CARTESIAN_POINT('Ctrl Pts',(-65.5467540029514,29.0189683030642,0.));
#88958=CARTESIAN_POINT('Ctrl Pts',(-65.5701191139418,29.0208315879764,0.));
#88959=CARTESIAN_POINT('Ctrl Pts',(-65.5935295405453,29.0226752157003,0.));
#88960=CARTESIAN_POINT('Ctrl Pts',(-65.6169851620046,29.0244991125959,0.));
#88961=CARTESIAN_POINT('Ctrl Pts',(-65.6404858580403,29.0263032054266,0.));
#88962=CARTESIAN_POINT('Ctrl Pts',(-65.6640315088388,29.0280874213596,0.));
#88963=CARTESIAN_POINT('Ctrl Pts',(-65.6876219950493,29.0298516879611,0.));
#88964=CARTESIAN_POINT('Ctrl Pts',(-65.7112571977891,29.0315959331919,0.));
#88965=CARTESIAN_POINT('Ctrl Pts',(-65.7349369986384,29.0333200854027,0.));
#88966=CARTESIAN_POINT('Ctrl Pts',(-65.7586612796368,29.035024073333,0.));
#88967=CARTESIAN_POINT('Ctrl Pts',(-65.7824299232705,29.0367078261103,0.));
#88968=CARTESIAN_POINT('Ctrl Pts',(-65.8062428124713,29.0383712732469,0.));
#88969=CARTESIAN_POINT('Ctrl Pts',(-65.8300998306191,29.0400143446338,0.));
#88970=CARTESIAN_POINT('Ctrl Pts',(-65.854000861539,29.0416369705375,0.));
#88971=CARTESIAN_POINT('Ctrl Pts',(-65.8779457894961,29.0432390815978,0.));
#88972=CARTESIAN_POINT('Ctrl Pts',(-65.9019344991854,29.0448206088288,0.));
#88973=CARTESIAN_POINT('Ctrl Pts',(-65.9259668757307,29.0463814836157,0.));
#88974=CARTESIAN_POINT('Ctrl Pts',(-65.9500428046868,29.0479216377081,0.));
#88975=CARTESIAN_POINT('Ctrl Pts',(-65.974162172037,29.0494410032172,0.));
#88976=CARTESIAN_POINT('Ctrl Pts',(-65.9983248641879,29.0509395126142,0.));
#88977=CARTESIAN_POINT('Ctrl Pts',(-66.0225307679591,29.0524170987307,0.));
#88978=CARTESIAN_POINT('Ctrl Pts',(-66.0467797705815,29.0538736947552,0.));
#88979=CARTESIAN_POINT('Ctrl Pts',(-66.0710717597009,29.0553092342278,0.));
#88980=CARTESIAN_POINT('Ctrl Pts',(-66.0954066233754,29.0567236510373,0.));
#88981=CARTESIAN_POINT('Ctrl Pts',(-66.1197842500711,29.0581168794189,0.));
#88982=CARTESIAN_POINT('Ctrl Pts',(-66.1442045286516,29.0594888539555,0.));
#88983=CARTESIAN_POINT('Ctrl Pts',(-66.1686673483755,29.0608395095745,0.));
#88984=CARTESIAN_POINT('Ctrl Pts',(-66.1931725989008,29.062168781542,0.));
#88985=CARTESIAN_POINT('Ctrl Pts',(-66.2177201702819,29.0634766054599,0.));
#88986=CARTESIAN_POINT('Ctrl Pts',(-66.2423099529668,29.0647629172645,0.));
#88987=CARTESIAN_POINT('Ctrl Pts',(-66.2669418377866,29.0660276532272,0.));
#88988=CARTESIAN_POINT('Ctrl Pts',(-66.2916157159528,29.0672707499527,0.));
#88989=CARTESIAN_POINT('Ctrl Pts',(-66.3163314790607,29.0684921443718,0.));
#88990=CARTESIAN_POINT('Ctrl Pts',(-66.3410890190879,29.0696917737397,0.));
#88991=CARTESIAN_POINT('Ctrl Pts',(-66.3658882283906,29.0708695756335,0.));
#88992=CARTESIAN_POINT('Ctrl Pts',(-66.3907289996942,29.0720254879535,0.));
#88993=CARTESIAN_POINT('Ctrl Pts',(-66.4156112260904,29.0731594489218,0.));
#88994=CARTESIAN_POINT('Ctrl Pts',(-66.4405348010404,29.0742713970762,0.));
#88995=CARTESIAN_POINT('Ctrl Pts',(-66.4654996183739,29.0753612712669,0.));
#88996=CARTESIAN_POINT('Ctrl Pts',(-66.4905055722864,29.0764290106553,0.));
#88997=CARTESIAN_POINT('Ctrl Pts',(-66.5155525573308,29.0774745547146,0.));
#88998=CARTESIAN_POINT('Ctrl Pts',(-66.5406404684116,29.0784978432294,0.));
#88999=CARTESIAN_POINT('Ctrl Pts',(-66.5657692007894,29.0794988162892,0.));
#89000=CARTESIAN_POINT('Ctrl Pts',(-66.5909386500796,29.0804774142852,0.));
#89001=CARTESIAN_POINT('Ctrl Pts',(-66.6161487122504,29.0814335779085,0.));
#89002=CARTESIAN_POINT('Ctrl Pts',(-66.6413992836148,29.0823672481508,0.));
#89003=CARTESIAN_POINT('Ctrl Pts',(-66.6666902608246,29.0832783663048,0.));
#89004=CARTESIAN_POINT('Ctrl Pts',(-66.6920215408744,29.0841668739585,0.));
#89005=CARTESIAN_POINT('Ctrl Pts',(-66.7173930211015,29.0850327129913,0.));
#89006=CARTESIAN_POINT('Ctrl Pts',(-66.7428045991841,29.0858758255729,0.));
#89007=CARTESIAN_POINT('Ctrl Pts',(-66.7682561731349,29.0866961541629,0.));
#89008=CARTESIAN_POINT('Ctrl Pts',(-66.7937476412941,29.0874936415138,0.));
#89009=CARTESIAN_POINT('Ctrl Pts',(-66.8192789023323,29.0882682306636,0.));
#89010=CARTESIAN_POINT('Ctrl Pts',(-66.8448498552508,29.0890198649327,0.));
#89011=CARTESIAN_POINT('Ctrl Pts',(-66.8704603993794,29.0897484879207,0.));
#89012=CARTESIAN_POINT('Ctrl Pts',(-66.8961104343703,29.0904540435063,0.));
#89013=CARTESIAN_POINT('Ctrl Pts',(-66.9217998601881,29.0911364758484,0.));
#89014=CARTESIAN_POINT('Ctrl Pts',(-66.9475285771133,29.0917957293824,0.));
#89015=CARTESIAN_POINT('Ctrl Pts',(-66.9732964857467,29.092431748817,0.));
#89016=CARTESIAN_POINT('Ctrl Pts',(-66.9991034870084,29.0930444791329,0.));
#89017=CARTESIAN_POINT('Ctrl Pts',(-67.0249494821361,29.0936338655828,0.));
#89018=CARTESIAN_POINT('Ctrl Pts',(-67.0508343726771,29.0941998536957,0.));
#89019=CARTESIAN_POINT('Ctrl Pts',(-67.0767580604872,29.0947423892725,0.));
#89020=CARTESIAN_POINT('Ctrl Pts',(-67.1027204477304,29.0952614183777,0.));
#89021=CARTESIAN_POINT('Ctrl Pts',(-67.1287214368743,29.0957568873357,0.));
#89022=CARTESIAN_POINT('Ctrl Pts',(-67.1547609306845,29.0962287427274,0.));
#89023=CARTESIAN_POINT('Ctrl Pts',(-67.1808388322116,29.0966769313893,0.));
#89024=CARTESIAN_POINT('Ctrl Pts',(-67.2069550447895,29.0971014004134,0.));
#89025=CARTESIAN_POINT('Ctrl Pts',(-67.2331094720482,29.0975020971473,0.));
#89026=CARTESIAN_POINT('Ctrl Pts',(-67.2593020179216,29.0978789691965,0.));
#89027=CARTESIAN_POINT('Ctrl Pts',(-67.2855325866516,29.0982319644276,0.));
#89028=CARTESIAN_POINT('Ctrl Pts',(-67.311801082791,29.0985610309768,0.));
#89029=CARTESIAN_POINT('Ctrl Pts',(-67.3381074112013,29.0988661172526,0.));
#89030=CARTESIAN_POINT('Ctrl Pts',(-67.3644514770373,29.0991471719172,0.));
#89031=CARTESIAN_POINT('Ctrl Pts',(-67.3908331857313,29.0994041438715,0.));
#89032=CARTESIAN_POINT('Ctrl Pts',(-67.4172524429726,29.0996369822418,0.));
#89033=CARTESIAN_POINT('Ctrl Pts',(-67.4437091546869,29.0998456363687,0.));
#89034=CARTESIAN_POINT('Ctrl Pts',(-67.4702032270063,29.1000300557961,0.));
#89035=CARTESIAN_POINT('Ctrl Pts',(-67.496734566311,29.1001901902915,0.));
#89036=CARTESIAN_POINT('Ctrl Pts',(-67.5233030792714,29.1003259898686,0.));
#89037=CARTESIAN_POINT('Ctrl Pts',(-67.5499086728891,29.1004374048149,0.));
#89038=CARTESIAN_POINT('Ctrl Pts',(-67.5765512545277,29.1005243857137,0.));
#89039=CARTESIAN_POINT('Ctrl Pts',(-67.6032307319614,29.1005868834863,0.));
#89040=CARTESIAN_POINT('Ctrl Pts',(-67.6299470133286,29.1006248493576,0.));
#89041=CARTESIAN_POINT('Ctrl Pts',(-67.6567000070319,29.1006382347812,0.));
#89042=CARTESIAN_POINT('Ctrl Pts',(-67.6834896216458,29.1006269913747,0.));
#89043=CARTESIAN_POINT('Ctrl Pts',(-67.7103157658297,29.1005910708624,0.));
#89044=CARTESIAN_POINT('Ctrl Pts',(-67.7371783482039,29.1005304249989,0.));
#89045=CARTESIAN_POINT('Ctrl Pts',(-67.7640772773397,29.1004450055647,0.));
#89046=CARTESIAN_POINT('Ctrl Pts',(-67.7910124620149,29.1003347645299,0.));
#89047=CARTESIAN_POINT('Ctrl Pts',(-67.8179838114109,29.1001996541846,0.));
#89048=CARTESIAN_POINT('Ctrl Pts',(-67.844991235333,29.1000396272868,0.));
#89049=CARTESIAN_POINT('Ctrl Pts',(-67.8720346444111,29.0998546372027,0.));
#89050=CARTESIAN_POINT('Ctrl Pts',(-67.8991139503168,29.0996446380617,0.));
#89051=CARTESIAN_POINT('Ctrl Pts',(-67.9262290652797,29.0994095844208,0.));
#89052=CARTESIAN_POINT('Ctrl Pts',(-67.9533799016122,29.0991494309394,0.));
#89053=CARTESIAN_POINT('Ctrl Pts',(-67.9805663711845,29.0988641320243,0.));
#89054=CARTESIAN_POINT('Ctrl Pts',(-68.0077883850136,29.0985536415537,0.));
#89055=CARTESIAN_POINT('Ctrl Pts',(-68.0350458525589,29.0982179124112,0.));
#89056=CARTESIAN_POINT('Ctrl Pts',(-68.0623386822917,29.0978568968677,0.));
#89057=CARTESIAN_POINT('Ctrl Pts',(-68.089666782962,29.0974705474279,0.));
#89058=CARTESIAN_POINT('Ctrl Pts',(-68.1170300647019,29.097058817574,0.));
#89059=CARTESIAN_POINT('Ctrl Pts',(-68.1444284400734,29.096621662474,0.));
#89060=CARTESIAN_POINT('Ctrl Pts',(-68.1718618254221,29.0961590399023,0.));
#89061=CARTESIAN_POINT('Ctrl Pts',(-68.1993301411959,29.0956709104588,0.));
#89062=CARTESIAN_POINT('Ctrl Pts',(-68.2229056854495,29.0952305915108,0.));
#89063=CARTESIAN_POINT('Ctrl Pts',(-68.2409993689947,29.0948791947834,0.));
#89064=CARTESIAN_POINT('Ctrl Pts',(-68.2535957746884,29.094628043331,0.));
#89065=CARTESIAN_POINT('Ctrl Pts',(-68.2606847334624,29.0944846386548,0.));
#89066=CARTESIAN_POINT('Ctrl Pts',(-68.2622612909744,29.0944526440249,0.));
#89067=CARTESIAN_POINT('',(-63.7976679095314,28.8072485549236,12.));
#89068=CARTESIAN_POINT('',(-63.7976679095314,28.8072485549236,0.));
#89069=CARTESIAN_POINT('Ctrl Pts',(-68.2622612909744,29.0944526440249,12.));
#89070=CARTESIAN_POINT('Ctrl Pts',(-68.2606847334624,29.0944846386548,12.));
#89071=CARTESIAN_POINT('Ctrl Pts',(-68.2535957746883,29.094628043331,12.));
#89072=CARTESIAN_POINT('Ctrl Pts',(-68.2409993689947,29.0948791947834,12.));
#89073=CARTESIAN_POINT('Ctrl Pts',(-68.2229056854495,29.0952305915108,12.));
#89074=CARTESIAN_POINT('Ctrl Pts',(-68.1993301411959,29.0956709104588,12.));
#89075=CARTESIAN_POINT('Ctrl Pts',(-68.1718618254221,29.0961590399023,12.));
#89076=CARTESIAN_POINT('Ctrl Pts',(-68.1444284400734,29.096621662474,12.));
#89077=CARTESIAN_POINT('Ctrl Pts',(-68.1170300647019,29.097058817574,12.));
#89078=CARTESIAN_POINT('Ctrl Pts',(-68.089666782962,29.0974705474279,12.));
#89079=CARTESIAN_POINT('Ctrl Pts',(-68.0623386822917,29.0978568968677,12.));
#89080=CARTESIAN_POINT('Ctrl Pts',(-68.0350458525589,29.0982179124112,12.));
#89081=CARTESIAN_POINT('Ctrl Pts',(-68.0077883850136,29.0985536415537,12.));
#89082=CARTESIAN_POINT('Ctrl Pts',(-67.9805663711845,29.0988641320243,12.));
#89083=CARTESIAN_POINT('Ctrl Pts',(-67.9533799016122,29.0991494309394,12.));
#89084=CARTESIAN_POINT('Ctrl Pts',(-67.9262290652797,29.0994095844208,12.));
#89085=CARTESIAN_POINT('Ctrl Pts',(-67.8991139503168,29.0996446380617,12.));
#89086=CARTESIAN_POINT('Ctrl Pts',(-67.8720346444111,29.0998546372027,12.));
#89087=CARTESIAN_POINT('Ctrl Pts',(-67.844991235333,29.1000396272868,12.));
#89088=CARTESIAN_POINT('Ctrl Pts',(-67.8179838114109,29.1001996541846,12.));
#89089=CARTESIAN_POINT('Ctrl Pts',(-67.7910124620149,29.1003347645299,12.));
#89090=CARTESIAN_POINT('Ctrl Pts',(-67.7640772773397,29.1004450055647,12.));
#89091=CARTESIAN_POINT('Ctrl Pts',(-67.7371783482039,29.1005304249989,12.));
#89092=CARTESIAN_POINT('Ctrl Pts',(-67.7103157658297,29.1005910708624,12.));
#89093=CARTESIAN_POINT('Ctrl Pts',(-67.6834896216458,29.1006269913747,12.));
#89094=CARTESIAN_POINT('Ctrl Pts',(-67.6567000070319,29.1006382347812,12.));
#89095=CARTESIAN_POINT('Ctrl Pts',(-67.6299470133286,29.1006248493576,12.));
#89096=CARTESIAN_POINT('Ctrl Pts',(-67.6032307319614,29.1005868834863,12.));
#89097=CARTESIAN_POINT('Ctrl Pts',(-67.5765512545277,29.1005243857137,12.));
#89098=CARTESIAN_POINT('Ctrl Pts',(-67.5499086728891,29.1004374048149,12.));
#89099=CARTESIAN_POINT('Ctrl Pts',(-67.5233030792714,29.1003259898686,12.));
#89100=CARTESIAN_POINT('Ctrl Pts',(-67.496734566311,29.1001901902915,12.));
#89101=CARTESIAN_POINT('Ctrl Pts',(-67.4702032270063,29.1000300557961,12.));
#89102=CARTESIAN_POINT('Ctrl Pts',(-67.4437091546869,29.0998456363687,12.));
#89103=CARTESIAN_POINT('Ctrl Pts',(-67.4172524429726,29.0996369822418,12.));
#89104=CARTESIAN_POINT('Ctrl Pts',(-67.3908331857313,29.0994041438715,12.));
#89105=CARTESIAN_POINT('Ctrl Pts',(-67.3644514770373,29.0991471719172,12.));
#89106=CARTESIAN_POINT('Ctrl Pts',(-67.3381074112013,29.0988661172526,12.));
#89107=CARTESIAN_POINT('Ctrl Pts',(-67.311801082791,29.0985610309768,12.));
#89108=CARTESIAN_POINT('Ctrl Pts',(-67.2855325866516,29.0982319644276,12.));
#89109=CARTESIAN_POINT('Ctrl Pts',(-67.2593020179216,29.0978789691965,12.));
#89110=CARTESIAN_POINT('Ctrl Pts',(-67.2331094720482,29.0975020971473,12.));
#89111=CARTESIAN_POINT('Ctrl Pts',(-67.2069550447895,29.0971014004134,12.));
#89112=CARTESIAN_POINT('Ctrl Pts',(-67.1808388322116,29.0966769313893,12.));
#89113=CARTESIAN_POINT('Ctrl Pts',(-67.1547609306845,29.0962287427274,12.));
#89114=CARTESIAN_POINT('Ctrl Pts',(-67.1287214368743,29.0957568873357,12.));
#89115=CARTESIAN_POINT('Ctrl Pts',(-67.1027204477304,29.0952614183777,12.));
#89116=CARTESIAN_POINT('Ctrl Pts',(-67.0767580604872,29.0947423892725,12.));
#89117=CARTESIAN_POINT('Ctrl Pts',(-67.0508343726771,29.0941998536957,12.));
#89118=CARTESIAN_POINT('Ctrl Pts',(-67.0249494821361,29.0936338655828,12.));
#89119=CARTESIAN_POINT('Ctrl Pts',(-66.9991034870084,29.0930444791329,12.));
#89120=CARTESIAN_POINT('Ctrl Pts',(-66.9732964857467,29.092431748817,12.));
#89121=CARTESIAN_POINT('Ctrl Pts',(-66.9475285771133,29.0917957293824,12.));
#89122=CARTESIAN_POINT('Ctrl Pts',(-66.9217998601881,29.0911364758484,12.));
#89123=CARTESIAN_POINT('Ctrl Pts',(-66.8961104343703,29.0904540435063,12.));
#89124=CARTESIAN_POINT('Ctrl Pts',(-66.8704603993794,29.0897484879207,12.));
#89125=CARTESIAN_POINT('Ctrl Pts',(-66.8448498552508,29.0890198649327,12.));
#89126=CARTESIAN_POINT('Ctrl Pts',(-66.8192789023323,29.0882682306636,12.));
#89127=CARTESIAN_POINT('Ctrl Pts',(-66.7937476412941,29.0874936415138,12.));
#89128=CARTESIAN_POINT('Ctrl Pts',(-66.7682561731349,29.0866961541629,12.));
#89129=CARTESIAN_POINT('Ctrl Pts',(-66.7428045991841,29.0858758255729,12.));
#89130=CARTESIAN_POINT('Ctrl Pts',(-66.7173930211015,29.0850327129913,12.));
#89131=CARTESIAN_POINT('Ctrl Pts',(-66.6920215408744,29.0841668739585,12.));
#89132=CARTESIAN_POINT('Ctrl Pts',(-66.6666902608246,29.0832783663048,12.));
#89133=CARTESIAN_POINT('Ctrl Pts',(-66.6413992836148,29.0823672481508,12.));
#89134=CARTESIAN_POINT('Ctrl Pts',(-66.6161487122504,29.0814335779085,12.));
#89135=CARTESIAN_POINT('Ctrl Pts',(-66.5909386500796,29.0804774142852,12.));
#89136=CARTESIAN_POINT('Ctrl Pts',(-66.5657692007894,29.0794988162892,12.));
#89137=CARTESIAN_POINT('Ctrl Pts',(-66.5406404684116,29.0784978432294,12.));
#89138=CARTESIAN_POINT('Ctrl Pts',(-66.5155525573308,29.0774745547146,12.));
#89139=CARTESIAN_POINT('Ctrl Pts',(-66.4905055722864,29.0764290106553,12.));
#89140=CARTESIAN_POINT('Ctrl Pts',(-66.4654996183739,29.0753612712669,12.));
#89141=CARTESIAN_POINT('Ctrl Pts',(-66.4405348010404,29.0742713970762,12.));
#89142=CARTESIAN_POINT('Ctrl Pts',(-66.4156112260904,29.0731594489218,12.));
#89143=CARTESIAN_POINT('Ctrl Pts',(-66.3907289996942,29.0720254879535,12.));
#89144=CARTESIAN_POINT('Ctrl Pts',(-66.3658882283906,29.0708695756335,12.));
#89145=CARTESIAN_POINT('Ctrl Pts',(-66.3410890190879,29.0696917737397,12.));
#89146=CARTESIAN_POINT('Ctrl Pts',(-66.3163314790607,29.0684921443718,12.));
#89147=CARTESIAN_POINT('Ctrl Pts',(-66.2916157159528,29.0672707499527,12.));
#89148=CARTESIAN_POINT('Ctrl Pts',(-66.2669418377866,29.0660276532272,12.));
#89149=CARTESIAN_POINT('Ctrl Pts',(-66.2423099529668,29.0647629172645,12.));
#89150=CARTESIAN_POINT('Ctrl Pts',(-66.2177201702819,29.0634766054599,12.));
#89151=CARTESIAN_POINT('Ctrl Pts',(-66.1931725989008,29.062168781542,12.));
#89152=CARTESIAN_POINT('Ctrl Pts',(-66.1686673483755,29.0608395095745,12.));
#89153=CARTESIAN_POINT('Ctrl Pts',(-66.1442045286516,29.0594888539555,12.));
#89154=CARTESIAN_POINT('Ctrl Pts',(-66.1197842500711,29.0581168794189,12.));
#89155=CARTESIAN_POINT('Ctrl Pts',(-66.0954066233754,29.0567236510373,12.));
#89156=CARTESIAN_POINT('Ctrl Pts',(-66.0710717597009,29.0553092342278,12.));
#89157=CARTESIAN_POINT('Ctrl Pts',(-66.0467797705815,29.0538736947552,12.));
#89158=CARTESIAN_POINT('Ctrl Pts',(-66.0225307679591,29.0524170987307,12.));
#89159=CARTESIAN_POINT('Ctrl Pts',(-65.9983248641879,29.0509395126142,12.));
#89160=CARTESIAN_POINT('Ctrl Pts',(-65.974162172037,29.0494410032172,12.));
#89161=CARTESIAN_POINT('Ctrl Pts',(-65.9500428046868,29.0479216377081,12.));
#89162=CARTESIAN_POINT('Ctrl Pts',(-65.9259668757307,29.0463814836157,12.));
#89163=CARTESIAN_POINT('Ctrl Pts',(-65.9019344991854,29.0448206088288,12.));
#89164=CARTESIAN_POINT('Ctrl Pts',(-65.8779457894961,29.0432390815978,12.));
#89165=CARTESIAN_POINT('Ctrl Pts',(-65.854000861539,29.0416369705375,12.));
#89166=CARTESIAN_POINT('Ctrl Pts',(-65.8300998306191,29.0400143446338,12.));
#89167=CARTESIAN_POINT('Ctrl Pts',(-65.8062428124713,29.0383712732469,12.));
#89168=CARTESIAN_POINT('Ctrl Pts',(-65.7824299232705,29.0367078261103,12.));
#89169=CARTESIAN_POINT('Ctrl Pts',(-65.7586612796368,29.035024073333,12.));
#89170=CARTESIAN_POINT('Ctrl Pts',(-65.7349369986384,29.0333200854027,12.));
#89171=CARTESIAN_POINT('Ctrl Pts',(-65.7112571977891,29.0315959331919,12.));
#89172=CARTESIAN_POINT('Ctrl Pts',(-65.6876219950493,29.0298516879611,12.));
#89173=CARTESIAN_POINT('Ctrl Pts',(-65.6640315088388,29.0280874213596,12.));
#89174=CARTESIAN_POINT('Ctrl Pts',(-65.6404858580403,29.0263032054266,12.));
#89175=CARTESIAN_POINT('Ctrl Pts',(-65.6169851620046,29.0244991125959,12.));
#89176=CARTESIAN_POINT('Ctrl Pts',(-65.5935295405453,29.0226752157003,12.));
#89177=CARTESIAN_POINT('Ctrl Pts',(-65.5701191139418,29.0208315879764,12.));
#89178=CARTESIAN_POINT('Ctrl Pts',(-65.5467540029514,29.0189683030642,12.));
#89179=CARTESIAN_POINT('Ctrl Pts',(-65.5234343288136,29.0170854350095,12.));
#89180=CARTESIAN_POINT('Ctrl Pts',(-65.5001602132535,29.0151830582675,12.));
#89181=CARTESIAN_POINT('Ctrl Pts',(-65.4769317784789,29.013261247709,12.));
#89182=CARTESIAN_POINT('Ctrl Pts',(-65.4537491471828,29.0113200786239,12.));
#89183=CARTESIAN_POINT('Ctrl Pts',(-65.4306124425562,29.0093596267215,12.));
#89184=CARTESIAN_POINT('Ctrl Pts',(-65.4075217882934,29.0073799681342,12.));
#89185=CARTESIAN_POINT('Ctrl Pts',(-65.3844773085961,29.0053811794207,12.));
#89186=CARTESIAN_POINT('Ctrl Pts',(-65.3614791281692,29.003363337573,12.));
#89187=CARTESIAN_POINT('Ctrl Pts',(-65.3385273722242,29.0013265200185,12.));
#89188=CARTESIAN_POINT('Ctrl Pts',(-65.3156221664916,28.9992708046211,12.));
#89189=CARTESIAN_POINT('Ctrl Pts',(-65.2927636372254,28.9971962696845,12.));
#89190=CARTESIAN_POINT('Ctrl Pts',(-65.2699519112064,28.9951029939557,12.));
#89191=CARTESIAN_POINT('Ctrl Pts',(-65.2471871157397,28.9929910566325,12.));
#89192=CARTESIAN_POINT('Ctrl Pts',(-65.2244693786609,28.9908605373663,12.));
#89193=CARTESIAN_POINT('Ctrl Pts',(-65.2017988283479,28.9887115162633,12.));
#89194=CARTESIAN_POINT('Ctrl Pts',(-65.1791755937256,28.9865440738884,12.));
#89195=CARTESIAN_POINT('Ctrl Pts',(-65.1565998042697,28.9843582912692,12.));
#89196=CARTESIAN_POINT('Ctrl Pts',(-65.1340715900028,28.9821542499042,12.));
#89197=CARTESIAN_POINT('Ctrl Pts',(-65.1115910815037,28.9799320317641,12.));
#89198=CARTESIAN_POINT('Ctrl Pts',(-65.0891584099168,28.9776917192933,12.));
#89199=CARTESIAN_POINT('Ctrl Pts',(-65.0667737069563,28.9754333954135,12.));
#89200=CARTESIAN_POINT('Ctrl Pts',(-65.0444371049082,28.9731571435282,12.));
#89201=CARTESIAN_POINT('Ctrl Pts',(-65.022148736628,28.97086304753,12.));
#89202=CARTESIAN_POINT('Ctrl Pts',(-64.9999087355504,28.9685511918018,12.));
#89203=CARTESIAN_POINT('Ctrl Pts',(-64.9777172357027,28.9662216612217,12.));
#89204=CARTESIAN_POINT('Ctrl Pts',(-64.955574371711,28.9638745411677,12.));
#89205=CARTESIAN_POINT('Ctrl Pts',(-64.9334802788038,28.9615099175249,12.));
#89206=CARTESIAN_POINT('Ctrl Pts',(-64.9114350928125,28.9591278766934,12.));
#89207=CARTESIAN_POINT('Ctrl Pts',(-64.8894389501801,28.9567285055866,12.));
#89208=CARTESIAN_POINT('Ctrl Pts',(-64.8674919879648,28.9543118916328,12.));
#89209=CARTESIAN_POINT('Ctrl Pts',(-64.8455943438423,28.9518781227765,12.));
#89210=CARTESIAN_POINT('Ctrl Pts',(-64.8237461561019,28.9494272874832,12.));
#89211=CARTESIAN_POINT('Ctrl Pts',(-64.8019475636442,28.9469594747431,12.));
#89212=CARTESIAN_POINT('Ctrl Pts',(-64.7801987060084,28.944474774081,12.));
#89213=CARTESIAN_POINT('Ctrl Pts',(-64.758499723388,28.9419732755656,12.));
#89214=CARTESIAN_POINT('Ctrl Pts',(-64.7368507566467,28.9394550698204,12.));
#89215=CARTESIAN_POINT('Ctrl Pts',(-64.715251947329,28.9369202480393,12.));
#89216=CARTESIAN_POINT('Ctrl Pts',(-64.6937034376617,28.9343689019882,12.));
#89217=CARTESIAN_POINT('Ctrl Pts',(-64.672205370541,28.9318011239915,12.));
#89218=CARTESIAN_POINT('Ctrl Pts',(-64.6507578895161,28.9292170069221,12.));
#89219=CARTESIAN_POINT('Ctrl Pts',(-64.629361138774,28.926616644195,12.));
#89220=CARTESIAN_POINT('Ctrl Pts',(-64.6080152631039,28.9240001297542,12.));
#89221=CARTESIAN_POINT('Ctrl Pts',(-64.5867204079426,28.9213675580985,12.));
#89222=CARTESIAN_POINT('Ctrl Pts',(-64.5654767194472,28.9187190243224,12.));
#89223=CARTESIAN_POINT('Ctrl Pts',(-64.5442843445559,28.9160546241538,12.));
#89224=CARTESIAN_POINT('Ctrl Pts',(-64.523143431047,28.9133744539949,12.));
#89225=CARTESIAN_POINT('Ctrl Pts',(-64.5020541275951,28.910678610965,12.));
#89226=CARTESIAN_POINT('Ctrl Pts',(-64.4810165836592,28.9079671928264,12.));
#89227=CARTESIAN_POINT('Ctrl Pts',(-64.4600309493583,28.9052402979062,12.));
#89228=CARTESIAN_POINT('Ctrl Pts',(-64.4390973753634,28.9024980250307,12.));
#89229=CARTESIAN_POINT('Ctrl Pts',(-64.4182160127379,28.899740473434,12.));
#89230=CARTESIAN_POINT('Ctrl Pts',(-64.397387012917,28.8969677427504,12.));
#89231=CARTESIAN_POINT('Ctrl Pts',(-64.3766105280688,28.89417993323,12.));
#89232=CARTESIAN_POINT('Ctrl Pts',(-64.3558867114076,28.8913771459323,12.));
#89233=CARTESIAN_POINT('Ctrl Pts',(-64.3352157174619,28.8885594828926,12.));
#89234=CARTESIAN_POINT('Ctrl Pts',(-64.3145977025037,28.8857270473959,12.));
#89235=CARTESIAN_POINT('Ctrl Pts',(-64.2940328242521,28.882879943794,12.));
#89236=CARTESIAN_POINT('Ctrl Pts',(-64.2735212410711,28.8800182770065,12.));
#89237=CARTESIAN_POINT('Ctrl Pts',(-64.2530631112929,28.877142152106,12.));
#89238=CARTESIAN_POINT('Ctrl Pts',(-64.2326585925252,28.8742516738947,12.));
#89239=CARTESIAN_POINT('Ctrl Pts',(-64.2123078408461,28.8713469464185,12.));
#89240=CARTESIAN_POINT('Ctrl Pts',(-64.1920110123299,28.8684280739014,12.));
#89241=CARTESIAN_POINT('Ctrl Pts',(-64.1717682648685,28.8654951618649,12.));
#89242=CARTESIAN_POINT('Ctrl Pts',(-64.1515797596564,28.8625483180437,12.));
#89243=CARTESIAN_POINT('Ctrl Pts',(-64.1314456633381,28.8595876537148,12.));
#89244=CARTESIAN_POINT('Ctrl Pts',(-64.1113661481965,28.8566132838178,12.));
#89245=CARTESIAN_POINT('Ctrl Pts',(-64.0913413876622,28.8536253241854,12.));
#89246=CARTESIAN_POINT('Ctrl Pts',(-64.0713715523599,28.8506238891093,12.));
#89247=CARTESIAN_POINT('Ctrl Pts',(-64.0514568066637,28.8476090892232,12.));
#89248=CARTESIAN_POINT('Ctrl Pts',(-64.0315973031942,28.844581028125,12.));
#89249=CARTESIAN_POINT('Ctrl Pts',(-64.0117931881298,28.8415398056428,12.));
#89250=CARTESIAN_POINT('Ctrl Pts',(-63.9920446117582,28.8384855243243,12.));
#89251=CARTESIAN_POINT('Ctrl Pts',(-63.9723517369614,28.8354182946601,12.));
#89252=CARTESIAN_POINT('Ctrl Pts',(-63.9527147494423,28.8323382413789,12.));
#89253=CARTESIAN_POINT('Ctrl Pts',(-63.9331338646996,28.8292455077559,12.));
#89254=CARTESIAN_POINT('Ctrl Pts',(-63.9136093063786,28.8261402423291,12.));
#89255=CARTESIAN_POINT('Ctrl Pts',(-63.8941412856924,28.823022586318,12.));
#89256=CARTESIAN_POINT('Ctrl Pts',(-63.8747299825313,28.8198926619858,12.));
#89257=CARTESIAN_POINT('Ctrl Pts',(-63.8553755207487,28.8167505576681,12.));
#89258=CARTESIAN_POINT('Ctrl Pts',(-63.8360779669856,28.8135963263368,12.));
#89259=CARTESIAN_POINT('Ctrl Pts',(-63.8206854735028,28.8110632620957,12.));
#89260=CARTESIAN_POINT('Ctrl Pts',(-63.8091667271232,28.8091580239553,12.));
#89261=CARTESIAN_POINT('Ctrl Pts',(-63.8014989507494,28.8078854475432,12.));
#89262=CARTESIAN_POINT('Ctrl Pts',(-63.7976679095314,28.8072485549236,12.));
#89263=CARTESIAN_POINT('Ctrl Pts',(-68.8415926175085,27.6958230985044,-5.55111512312578E-16));
#89264=CARTESIAN_POINT('Ctrl Pts',(-68.8415926175085,27.6958230985044,4.));
#89265=CARTESIAN_POINT('Ctrl Pts',(-68.8415926175085,27.6958230985044,8.));
#89266=CARTESIAN_POINT('Ctrl Pts',(-68.8415926175085,27.6958230985044,12.));
#89267=CARTESIAN_POINT('Ctrl Pts',(-68.9176987693914,27.7750822307003,-5.55111512312578E-16));
#89268=CARTESIAN_POINT('Ctrl Pts',(-68.9176987693914,27.7750822307003,4.));
#89269=CARTESIAN_POINT('Ctrl Pts',(-68.9176987693914,27.7750822307003,8.00000000000001));
#89270=CARTESIAN_POINT('Ctrl Pts',(-68.9176987693914,27.7750822307003,12.));
#89271=CARTESIAN_POINT('Ctrl Pts',(-69.0029745467578,27.9589320265197,-5.55111512312578E-16));
#89272=CARTESIAN_POINT('Ctrl Pts',(-69.0029745467578,27.9589320265197,4.));
#89273=CARTESIAN_POINT('Ctrl Pts',(-69.0029745467578,27.9589320265197,8.));
#89274=CARTESIAN_POINT('Ctrl Pts',(-69.0029745467578,27.9589320265197,12.));
#89275=CARTESIAN_POINT('Ctrl Pts',(-68.9748773050757,28.1553386138879,-5.55111512312578E-16));
#89276=CARTESIAN_POINT('Ctrl Pts',(-68.9748773050757,28.1553386138879,4.));
#89277=CARTESIAN_POINT('Ctrl Pts',(-68.9748773050757,28.1553386138879,8.00000000000001));
#89278=CARTESIAN_POINT('Ctrl Pts',(-68.9748773050757,28.1553386138879,12.));
#89279=CARTESIAN_POINT('Ctrl Pts',(-68.943647523761,28.231604030224,-5.55111512312578E-16));
#89280=CARTESIAN_POINT('Ctrl Pts',(-68.943647523761,28.231604030224,4.));
#89281=CARTESIAN_POINT('Ctrl Pts',(-68.943647523761,28.231604030224,8.));
#89282=CARTESIAN_POINT('Ctrl Pts',(-68.943647523761,28.231604030224,12.));
#89283=CARTESIAN_POINT('',(-68.8415926175085,27.6958230985044,2.77555756156289E-16));
#89284=CARTESIAN_POINT('',(-68.9436475237613,28.2316040302241,0.));
#89285=CARTESIAN_POINT('Ctrl Pts',(-68.8415926175085,27.6958230985044,-1.38777878078145E-16));
#89286=CARTESIAN_POINT('Ctrl Pts',(-68.9176987693914,27.7750822307003,-1.38777878078145E-16));
#89287=CARTESIAN_POINT('Ctrl Pts',(-68.9664277850293,27.8801392568828,-1.38777878078145E-16));
#89288=CARTESIAN_POINT('Ctrl Pts',(-68.9781370393453,27.9892964598976,-1.38777878078145E-16));
#89289=CARTESIAN_POINT('Ctrl Pts',(-68.9869189800823,28.0711643621587,-1.38777878078145E-16));
#89290=CARTESIAN_POINT('Ctrl Pts',(-68.9748773050757,28.1553386138879,-1.38777878078145E-16));
#89291=CARTESIAN_POINT('Ctrl Pts',(-68.943647523761,28.231604030224,-1.38777878078145E-16));
#89292=CARTESIAN_POINT('',(-68.9436475237613,28.2316040302241,12.));
#89293=CARTESIAN_POINT('Ctrl Pts',(-68.943647523761,28.231604030224,-5.55111512312578E-16));
#89294=CARTESIAN_POINT('Ctrl Pts',(-68.943647523761,28.231604030224,4.));
#89295=CARTESIAN_POINT('Ctrl Pts',(-68.943647523761,28.231604030224,8.));
#89296=CARTESIAN_POINT('Ctrl Pts',(-68.943647523761,28.231604030224,12.));
#89297=CARTESIAN_POINT('',(-68.8415926175085,27.6958230985044,12.));
#89298=CARTESIAN_POINT('Ctrl Pts',(-68.943647523761,28.231604030224,12.));
#89299=CARTESIAN_POINT('Ctrl Pts',(-68.9748773050757,28.1553386138879,12.));
#89300=CARTESIAN_POINT('Ctrl Pts',(-68.9869189800823,28.0711643621587,12.));
#89301=CARTESIAN_POINT('Ctrl Pts',(-68.9781370393453,27.9892964598976,12.));
#89302=CARTESIAN_POINT('Ctrl Pts',(-68.9664277850293,27.8801392568828,12.));
#89303=CARTESIAN_POINT('Ctrl Pts',(-68.9176987693914,27.7750822307003,12.));
#89304=CARTESIAN_POINT('Ctrl Pts',(-68.8415926175085,27.6958230985044,12.));
#89305=CARTESIAN_POINT('Ctrl Pts',(-68.8415926175085,27.6958230985044,12.));
#89306=CARTESIAN_POINT('Ctrl Pts',(-68.8415926175085,27.6958230985044,8.));
#89307=CARTESIAN_POINT('Ctrl Pts',(-68.8415926175085,27.6958230985044,4.));
#89308=CARTESIAN_POINT('Ctrl Pts',(-68.8415926175085,27.6958230985044,-5.55111512312578E-16));
#89309=CARTESIAN_POINT('Origin',(-3.4634846687719E-10,1.43354795624835E-10,
0.));
#89310=CARTESIAN_POINT('Origin',(-3.4634846687719E-10,1.43354795624835E-10,
12.));
#89311=CARTESIAN_POINT('Origin',(-3.4634846687719E-10,1.43354795624835E-10,
0.));
#89312=CARTESIAN_POINT('Ctrl Pts',(-65.9427857825598,34.6669728017235,0.));
#89313=CARTESIAN_POINT('Ctrl Pts',(-65.9427857825598,34.6669728017235,4.));
#89314=CARTESIAN_POINT('Ctrl Pts',(-65.9427857825598,34.6669728017235,8.));
#89315=CARTESIAN_POINT('Ctrl Pts',(-65.9427857825598,34.6669728017235,12.));
#89316=CARTESIAN_POINT('Ctrl Pts',(-65.891654340017,34.7642339552033,0.));
#89317=CARTESIAN_POINT('Ctrl Pts',(-65.891654340017,34.7642339552033,4.));
#89318=CARTESIAN_POINT('Ctrl Pts',(-65.891654340017,34.7642339552033,8.00000000000001));
#89319=CARTESIAN_POINT('Ctrl Pts',(-65.891654340017,34.7642339552033,12.));
#89320=CARTESIAN_POINT('Ctrl Pts',(-65.7441961270806,34.9032616822021,0.));
#89321=CARTESIAN_POINT('Ctrl Pts',(-65.7441961270806,34.9032616822021,4.));
#89322=CARTESIAN_POINT('Ctrl Pts',(-65.7441961270806,34.9032616822021,7.99999999999999));
#89323=CARTESIAN_POINT('Ctrl Pts',(-65.7441961270806,34.9032616822021,12.));
#89324=CARTESIAN_POINT('Ctrl Pts',(-65.5489812297289,34.9387029822713,0.));
#89325=CARTESIAN_POINT('Ctrl Pts',(-65.5489812297289,34.9387029822713,4.));
#89326=CARTESIAN_POINT('Ctrl Pts',(-65.5489812297289,34.9387029822712,8.00000000000001));
#89327=CARTESIAN_POINT('Ctrl Pts',(-65.5489812297289,34.9387029822712,12.));
#89328=CARTESIAN_POINT('Ctrl Pts',(-65.4667541477958,34.9331875523083,0.));
#89329=CARTESIAN_POINT('Ctrl Pts',(-65.4667541477958,34.9331875523083,4.));
#89330=CARTESIAN_POINT('Ctrl Pts',(-65.4667541477958,34.9331875523082,8.));
#89331=CARTESIAN_POINT('Ctrl Pts',(-65.4667541477958,34.9331875523082,12.));
#89332=CARTESIAN_POINT('',(-65.9427857825598,34.6669728017235,0.));
#89333=CARTESIAN_POINT('',(-65.4667541477958,34.9331875523085,0.));
#89334=CARTESIAN_POINT('Ctrl Pts',(-65.9427857825598,34.6669728017235,0.));
#89335=CARTESIAN_POINT('Ctrl Pts',(-65.891654340017,34.7642339552033,0.));
#89336=CARTESIAN_POINT('Ctrl Pts',(-65.8073925040534,34.8436783706312,0.));
#89337=CARTESIAN_POINT('Ctrl Pts',(-65.7075366486888,34.8892986466535,0.));
#89338=CARTESIAN_POINT('Ctrl Pts',(-65.6326447571654,34.9235138536702,0.));
#89339=CARTESIAN_POINT('Ctrl Pts',(-65.5489812297289,34.9387029822713,0.));
#89340=CARTESIAN_POINT('Ctrl Pts',(-65.4667541477958,34.9331875523083,0.));
#89341=CARTESIAN_POINT('',(-65.4667541477958,34.9331875523085,12.));
#89342=CARTESIAN_POINT('Ctrl Pts',(-65.4667541477958,34.9331875523083,0.));
#89343=CARTESIAN_POINT('Ctrl Pts',(-65.4667541477958,34.9331875523083,4.));
#89344=CARTESIAN_POINT('Ctrl Pts',(-65.4667541477958,34.9331875523082,8.));
#89345=CARTESIAN_POINT('Ctrl Pts',(-65.4667541477958,34.9331875523082,12.));
#89346=CARTESIAN_POINT('',(-65.9427857825598,34.6669728017235,12.));
#89347=CARTESIAN_POINT('Ctrl Pts',(-65.4667541477958,34.9331875523082,12.));
#89348=CARTESIAN_POINT('Ctrl Pts',(-65.5489812297289,34.9387029822712,12.));
#89349=CARTESIAN_POINT('Ctrl Pts',(-65.6326447571654,34.9235138536702,12.));
#89350=CARTESIAN_POINT('Ctrl Pts',(-65.7075366486888,34.8892986466535,12.));
#89351=CARTESIAN_POINT('Ctrl Pts',(-65.8073925040534,34.8436783706312,12.));
#89352=CARTESIAN_POINT('Ctrl Pts',(-65.891654340017,34.7642339552033,12.));
#89353=CARTESIAN_POINT('Ctrl Pts',(-65.9427857825598,34.6669728017235,12.));
#89354=CARTESIAN_POINT('Ctrl Pts',(-65.9427857825598,34.6669728017235,12.));
#89355=CARTESIAN_POINT('Ctrl Pts',(-65.9427857825598,34.6669728017235,8.));
#89356=CARTESIAN_POINT('Ctrl Pts',(-65.9427857825598,34.6669728017235,4.));
#89357=CARTESIAN_POINT('Ctrl Pts',(-65.9427857825598,34.6669728017235,0.));
#89358=CARTESIAN_POINT('Ctrl Pts',(-61.0441813777723,34.2579614092497,0.));
#89359=CARTESIAN_POINT('Ctrl Pts',(-61.0441813777723,34.2579614092497,12.));
#89360=CARTESIAN_POINT('Ctrl Pts',(-61.0479423318725,34.2589297755433,0.));
#89361=CARTESIAN_POINT('Ctrl Pts',(-61.0479423318725,34.2589297755433,12.));
#89362=CARTESIAN_POINT('Ctrl Pts',(-61.0554700176998,34.2608658001631,0.));
#89363=CARTESIAN_POINT('Ctrl Pts',(-61.0554700176998,34.2608658001631,12.));
#89364=CARTESIAN_POINT('Ctrl Pts',(-61.0667788793266,34.2637677131934,0.));
#89365=CARTESIAN_POINT('Ctrl Pts',(-61.0667788793266,34.2637677131934,12.));
#89366=CARTESIAN_POINT('Ctrl Pts',(-61.0818920286293,34.2676326825626,0.));
#89367=CARTESIAN_POINT('Ctrl Pts',(-61.0818920286293,34.2676326825626,12.));
#89368=CARTESIAN_POINT('Ctrl Pts',(-61.1008412399997,34.2724568037227,0.));
#89369=CARTESIAN_POINT('Ctrl Pts',(-61.1008412399997,34.2724568037227,12.));
#89370=CARTESIAN_POINT('Ctrl Pts',(-61.1198481997764,34.277273803877,0.));
#89371=CARTESIAN_POINT('Ctrl Pts',(-61.1198481997764,34.277273803877,12.));
#89372=CARTESIAN_POINT('Ctrl Pts',(-61.1389128461886,34.2820836244469,0.));
#89373=CARTESIAN_POINT('Ctrl Pts',(-61.1389128461886,34.2820836244469,12.));
#89374=CARTESIAN_POINT('Ctrl Pts',(-61.1580350635533,34.2868861666384,0.));
#89375=CARTESIAN_POINT('Ctrl Pts',(-61.1580350635533,34.2868861666384,12.));
#89376=CARTESIAN_POINT('Ctrl Pts',(-61.1772146833205,34.2916812929751,0.));
#89377=CARTESIAN_POINT('Ctrl Pts',(-61.1772146833205,34.2916812929751,12.));
#89378=CARTESIAN_POINT('Ctrl Pts',(-61.1964515073891,34.2964688443663,0.));
#89379=CARTESIAN_POINT('Ctrl Pts',(-61.1964515073891,34.2964688443663,12.));
#89380=CARTESIAN_POINT('Ctrl Pts',(-61.2157453259107,34.3012486533474,0.));
#89381=CARTESIAN_POINT('Ctrl Pts',(-61.2157453259107,34.3012486533474,12.));
#89382=CARTESIAN_POINT('Ctrl Pts',(-61.235095936694,34.3060205584064,0.));
#89383=CARTESIAN_POINT('Ctrl Pts',(-61.235095936694,34.3060205584064,12.));
#89384=CARTESIAN_POINT('Ctrl Pts',(-61.2545031656133,34.3107844191043,0.));
#89385=CARTESIAN_POINT('Ctrl Pts',(-61.2545031656133,34.3107844191043,12.));
#89386=CARTESIAN_POINT('Ctrl Pts',(-61.2739668600365,34.3155401111747,0.));
#89387=CARTESIAN_POINT('Ctrl Pts',(-61.2739668600365,34.3155401111747,12.));
#89388=CARTESIAN_POINT('Ctrl Pts',(-61.2934868791855,34.3202875193617,0.));
#89389=CARTESIAN_POINT('Ctrl Pts',(-61.2934868791855,34.3202875193617,12.));
#89390=CARTESIAN_POINT('Ctrl Pts',(-61.3130630861386,34.3250265314768,0.));
#89391=CARTESIAN_POINT('Ctrl Pts',(-61.3130630861386,34.3250265314768,12.));
#89392=CARTESIAN_POINT('Ctrl Pts',(-61.3326953378851,34.3297570310146,0.));
#89393=CARTESIAN_POINT('Ctrl Pts',(-61.3326953378851,34.3297570310146,12.));
#89394=CARTESIAN_POINT('Ctrl Pts',(-61.3523834803188,34.3344788934363,0.));
#89395=CARTESIAN_POINT('Ctrl Pts',(-61.3523834803188,34.3344788934363,12.));
#89396=CARTESIAN_POINT('Ctrl Pts',(-61.3721273534257,34.339191990014,0.));
#89397=CARTESIAN_POINT('Ctrl Pts',(-61.3721273534257,34.339191990014,12.));
#89398=CARTESIAN_POINT('Ctrl Pts',(-61.3919267945302,34.3438961902405,0.));
#89399=CARTESIAN_POINT('Ctrl Pts',(-61.3919267945302,34.3438961902405,12.));
#89400=CARTESIAN_POINT('Ctrl Pts',(-61.4117816420229,34.3485913645979,0.));
#89401=CARTESIAN_POINT('Ctrl Pts',(-61.4117816420229,34.3485913645979,12.));
#89402=CARTESIAN_POINT('Ctrl Pts',(-61.4316917395918,34.3532773877089,0.));
#89403=CARTESIAN_POINT('Ctrl Pts',(-61.4316917395918,34.3532773877089,12.));
#89404=CARTESIAN_POINT('Ctrl Pts',(-61.4516569360454,34.3579541381996,0.));
#89405=CARTESIAN_POINT('Ctrl Pts',(-61.4516569360454,34.3579541381996,12.));
#89406=CARTESIAN_POINT('Ctrl Pts',(-61.4716770832897,34.3626214971888,0.));
#89407=CARTESIAN_POINT('Ctrl Pts',(-61.4716770832897,34.3626214971888,12.));
#89408=CARTESIAN_POINT('Ctrl Pts',(-61.4917520349279,34.3672793472465,0.));
#89409=CARTESIAN_POINT('Ctrl Pts',(-61.4917520349279,34.3672793472465,12.));
#89410=CARTESIAN_POINT('Ctrl Pts',(-61.5118816445437,34.3719275711195,0.));
#89411=CARTESIAN_POINT('Ctrl Pts',(-61.5118816445437,34.3719275711195,12.));
#89412=CARTESIAN_POINT('Ctrl Pts',(-61.5320657642639,34.376566050668,0.));
#89413=CARTESIAN_POINT('Ctrl Pts',(-61.5320657642639,34.376566050668,12.));
#89414=CARTESIAN_POINT('Ctrl Pts',(-61.5523042455158,34.3811946674196,0.));
#89415=CARTESIAN_POINT('Ctrl Pts',(-61.5523042455158,34.3811946674196,12.));
#89416=CARTESIAN_POINT('Ctrl Pts',(-61.5725969396829,34.3858133030518,0.));
#89417=CARTESIAN_POINT('Ctrl Pts',(-61.5725969396829,34.3858133030518,12.));
#89418=CARTESIAN_POINT('Ctrl Pts',(-61.5929436987409,34.3904218398636,0.));
#89419=CARTESIAN_POINT('Ctrl Pts',(-61.5929436987409,34.3904218398636,12.));
#89420=CARTESIAN_POINT('Ctrl Pts',(-61.6133443760142,34.3950201613432,0.));
#89421=CARTESIAN_POINT('Ctrl Pts',(-61.6133443760142,34.3950201613432,12.));
#89422=CARTESIAN_POINT('Ctrl Pts',(-61.6337988264556,34.3996081523753,0.));
#89423=CARTESIAN_POINT('Ctrl Pts',(-61.6337988264556,34.3996081523753,12.));
#89424=CARTESIAN_POINT('Ctrl Pts',(-61.6543069062416,34.4041856989316,0.));
#89425=CARTESIAN_POINT('Ctrl Pts',(-61.6543069062416,34.4041856989316,12.));
#89426=CARTESIAN_POINT('Ctrl Pts',(-61.6748684725205,34.4087526878812,0.));
#89427=CARTESIAN_POINT('Ctrl Pts',(-61.6748684725205,34.4087526878812,12.));
#89428=CARTESIAN_POINT('Ctrl Pts',(-61.695483383117,34.4133090067703,0.));
#89429=CARTESIAN_POINT('Ctrl Pts',(-61.695483383117,34.4133090067703,12.));
#89430=CARTESIAN_POINT('Ctrl Pts',(-61.7161514961915,34.4178545435766,0.));
#89431=CARTESIAN_POINT('Ctrl Pts',(-61.7161514961915,34.4178545435766,12.));
#89432=CARTESIAN_POINT('Ctrl Pts',(-61.7368726702596,34.4223891867179,0.));
#89433=CARTESIAN_POINT('Ctrl Pts',(-61.7368726702596,34.4223891867179,12.));
#89434=CARTESIAN_POINT('Ctrl Pts',(-61.7576467643432,34.4269128251576,0.));
#89435=CARTESIAN_POINT('Ctrl Pts',(-61.7576467643432,34.4269128251576,12.));
#89436=CARTESIAN_POINT('Ctrl Pts',(-61.7784736380727,34.4314253484791,0.));
#89437=CARTESIAN_POINT('Ctrl Pts',(-61.7784736380727,34.4314253484791,12.));
#89438=CARTESIAN_POINT('Ctrl Pts',(-61.7993531518037,34.4359266469749,0.));
#89439=CARTESIAN_POINT('Ctrl Pts',(-61.7993531518037,34.4359266469749,12.));
#89440=CARTESIAN_POINT('Ctrl Pts',(-61.8202851667222,34.4404166117299,0.));
#89441=CARTESIAN_POINT('Ctrl Pts',(-61.8202851667222,34.4404166117299,12.));
#89442=CARTESIAN_POINT('Ctrl Pts',(-61.8412695447926,34.4448951345739,0.));
#89443=CARTESIAN_POINT('Ctrl Pts',(-61.8412695447926,34.4448951345739,12.));
#89444=CARTESIAN_POINT('Ctrl Pts',(-61.8623061487018,34.449362108036,0.));
#89445=CARTESIAN_POINT('Ctrl Pts',(-61.8623061487018,34.449362108036,12.));
#89446=CARTESIAN_POINT('Ctrl Pts',(-61.8833948418025,34.4538174253012,0.));
#89447=CARTESIAN_POINT('Ctrl Pts',(-61.8833948418025,34.4538174253012,12.));
#89448=CARTESIAN_POINT('Ctrl Pts',(-61.9045354880445,34.4582609801637,0.));
#89449=CARTESIAN_POINT('Ctrl Pts',(-61.9045354880445,34.4582609801637,12.));
#89450=CARTESIAN_POINT('Ctrl Pts',(-61.9257279519308,34.4626926669974,0.));
#89451=CARTESIAN_POINT('Ctrl Pts',(-61.9257279519308,34.4626926669974,12.));
#89452=CARTESIAN_POINT('Ctrl Pts',(-61.9469720985531,34.4671123807717,0.));
#89453=CARTESIAN_POINT('Ctrl Pts',(-61.9469720985531,34.4671123807717,12.));
#89454=CARTESIAN_POINT('Ctrl Pts',(-61.9682677936054,34.4715200170592,0.));
#89455=CARTESIAN_POINT('Ctrl Pts',(-61.9682677936054,34.4715200170592,12.));
#89456=CARTESIAN_POINT('Ctrl Pts',(-61.9896149034001,34.4759154720473,0.));
#89457=CARTESIAN_POINT('Ctrl Pts',(-61.9896149034001,34.4759154720473,12.));
#89458=CARTESIAN_POINT('Ctrl Pts',(-62.0110132948794,34.4802986425528,0.));
#89459=CARTESIAN_POINT('Ctrl Pts',(-62.0110132948794,34.4802986425528,12.));
#89460=CARTESIAN_POINT('Ctrl Pts',(-62.0324628356141,34.4846694260199,0.));
#89461=CARTESIAN_POINT('Ctrl Pts',(-62.0324628356141,34.4846694260199,12.));
#89462=CARTESIAN_POINT('Ctrl Pts',(-62.0539633937939,34.4890277205039,0.));
#89463=CARTESIAN_POINT('Ctrl Pts',(-62.0539633937939,34.4890277205039,12.));
#89464=CARTESIAN_POINT('Ctrl Pts',(-62.0755148382135,34.4933734246592,0.));
#89465=CARTESIAN_POINT('Ctrl Pts',(-62.0755148382135,34.4933734246592,12.));
#89466=CARTESIAN_POINT('Ctrl Pts',(-62.0971170382567,34.4977064377282,0.));
#89467=CARTESIAN_POINT('Ctrl Pts',(-62.0971170382567,34.4977064377282,12.));
#89468=CARTESIAN_POINT('Ctrl Pts',(-62.1187698638707,34.5020266595293,0.));
#89469=CARTESIAN_POINT('Ctrl Pts',(-62.1187698638707,34.5020266595293,12.));
#89470=CARTESIAN_POINT('Ctrl Pts',(-62.1404731855687,34.5063339904533,0.));
#89471=CARTESIAN_POINT('Ctrl Pts',(-62.1404731855687,34.5063339904533,12.));
#89472=CARTESIAN_POINT('Ctrl Pts',(-62.1622268744337,34.5106283314594,0.));
#89473=CARTESIAN_POINT('Ctrl Pts',(-62.1622268744337,34.5106283314594,12.));
#89474=CARTESIAN_POINT('Ctrl Pts',(-62.1840308021171,34.5149095840729,0.));
#89475=CARTESIAN_POINT('Ctrl Pts',(-62.1840308021171,34.5149095840729,12.));
#89476=CARTESIAN_POINT('Ctrl Pts',(-62.2058848408346,34.5191776503843,0.));
#89477=CARTESIAN_POINT('Ctrl Pts',(-62.2058848408346,34.5191776503843,12.));
#89478=CARTESIAN_POINT('Ctrl Pts',(-62.2277888633577,34.5234324330492,0.));
#89479=CARTESIAN_POINT('Ctrl Pts',(-62.2277888633577,34.5234324330492,12.));
#89480=CARTESIAN_POINT('Ctrl Pts',(-62.2497427430136,34.527673835281,0.));
#89481=CARTESIAN_POINT('Ctrl Pts',(-62.2497427430136,34.527673835281,12.));
#89482=CARTESIAN_POINT('Ctrl Pts',(-62.2717463536828,34.5319017608434,0.));
#89483=CARTESIAN_POINT('Ctrl Pts',(-62.2717463536828,34.5319017608434,12.));
#89484=CARTESIAN_POINT('Ctrl Pts',(-62.2937995697927,34.536116114045,0.));
#89485=CARTESIAN_POINT('Ctrl Pts',(-62.2937995697927,34.536116114045,12.));
#89486=CARTESIAN_POINT('Ctrl Pts',(-62.3159022663052,34.5403167997333,0.));
#89487=CARTESIAN_POINT('Ctrl Pts',(-62.3159022663052,34.5403167997333,12.));
#89488=CARTESIAN_POINT('Ctrl Pts',(-62.3380543187067,34.5445037232928,0.));
#89489=CARTESIAN_POINT('Ctrl Pts',(-62.3380543187067,34.5445037232928,12.));
#89490=CARTESIAN_POINT('Ctrl Pts',(-62.3602556030114,34.5486767906376,0.));
#89491=CARTESIAN_POINT('Ctrl Pts',(-62.3602556030114,34.5486767906376,12.));
#89492=CARTESIAN_POINT('Ctrl Pts',(-62.3825059957593,34.552835908207,0.));
#89493=CARTESIAN_POINT('Ctrl Pts',(-62.3825059957593,34.552835908207,12.));
#89494=CARTESIAN_POINT('Ctrl Pts',(-62.4048053740129,34.5569809829615,0.));
#89495=CARTESIAN_POINT('Ctrl Pts',(-62.4048053740129,34.5569809829615,12.));
#89496=CARTESIAN_POINT('Ctrl Pts',(-62.4271536153473,34.5611119223807,0.));
#89497=CARTESIAN_POINT('Ctrl Pts',(-62.4271536153473,34.5611119223807,12.));
#89498=CARTESIAN_POINT('Ctrl Pts',(-62.4495505978415,34.5652286344606,0.));
#89499=CARTESIAN_POINT('Ctrl Pts',(-62.4495505978415,34.5652286344606,12.));
#89500=CARTESIAN_POINT('Ctrl Pts',(-62.471996200083,34.5693310277064,0.));
#89501=CARTESIAN_POINT('Ctrl Pts',(-62.471996200083,34.5693310277064,12.));
#89502=CARTESIAN_POINT('Ctrl Pts',(-62.494490301164,34.5734190111279,0.));
#89503=CARTESIAN_POINT('Ctrl Pts',(-62.494490301164,34.5734190111279,12.));
#89504=CARTESIAN_POINT('Ctrl Pts',(-62.5170327806774,34.5774924942351,0.));
#89505=CARTESIAN_POINT('Ctrl Pts',(-62.5170327806774,34.5774924942351,12.));
#89506=CARTESIAN_POINT('Ctrl Pts',(-62.5396235187053,34.5815513870363,0.));
#89507=CARTESIAN_POINT('Ctrl Pts',(-62.5396235187053,34.5815513870363,12.));
#89508=CARTESIAN_POINT('Ctrl Pts',(-62.5622623958125,34.5855956000343,0.));
#89509=CARTESIAN_POINT('Ctrl Pts',(-62.5622623958125,34.5855956000343,12.));
#89510=CARTESIAN_POINT('Ctrl Pts',(-62.5849492930501,34.5896250442199,0.));
#89511=CARTESIAN_POINT('Ctrl Pts',(-62.5849492930501,34.5896250442199,12.));
#89512=CARTESIAN_POINT('Ctrl Pts',(-62.6076840919521,34.5936396310671,0.));
#89513=CARTESIAN_POINT('Ctrl Pts',(-62.6076840919521,34.5936396310671,12.));
#89514=CARTESIAN_POINT('Ctrl Pts',(-62.6304666745319,34.5976392725303,0.));
#89515=CARTESIAN_POINT('Ctrl Pts',(-62.6304666745319,34.5976392725303,12.));
#89516=CARTESIAN_POINT('Ctrl Pts',(-62.6532969232695,34.6016238810419,0.));
#89517=CARTESIAN_POINT('Ctrl Pts',(-62.6532969232695,34.6016238810419,12.));
#89518=CARTESIAN_POINT('Ctrl Pts',(-62.6761747211081,34.6055933695093,0.));
#89519=CARTESIAN_POINT('Ctrl Pts',(-62.6761747211081,34.6055933695093,12.));
#89520=CARTESIAN_POINT('Ctrl Pts',(-62.6990999514597,34.6095476513094,0.));
#89521=CARTESIAN_POINT('Ctrl Pts',(-62.6990999514597,34.6095476513094,12.));
#89522=CARTESIAN_POINT('Ctrl Pts',(-62.7220724982005,34.6134866402842,0.));
#89523=CARTESIAN_POINT('Ctrl Pts',(-62.7220724982005,34.6134866402842,12.));
#89524=CARTESIAN_POINT('Ctrl Pts',(-62.7450922456663,34.6174102507368,0.));
#89525=CARTESIAN_POINT('Ctrl Pts',(-62.7450922456663,34.6174102507368,12.));
#89526=CARTESIAN_POINT('Ctrl Pts',(-62.7681590786398,34.6213183974302,0.));
#89527=CARTESIAN_POINT('Ctrl Pts',(-62.7681590786398,34.6213183974302,12.));
#89528=CARTESIAN_POINT('Ctrl Pts',(-62.7912728823483,34.6252109955836,0.));
#89529=CARTESIAN_POINT('Ctrl Pts',(-62.7912728823483,34.6252109955836,12.));
#89530=CARTESIAN_POINT('Ctrl Pts',(-62.8144335424671,34.629087960866,0.));
#89531=CARTESIAN_POINT('Ctrl Pts',(-62.8144335424671,34.629087960866,12.));
#89532=CARTESIAN_POINT('Ctrl Pts',(-62.8376409451167,34.6329492093931,0.));
#89533=CARTESIAN_POINT('Ctrl Pts',(-62.8376409451167,34.6329492093931,12.));
#89534=CARTESIAN_POINT('Ctrl Pts',(-62.8608949768583,34.6367946577241,0.));
#89535=CARTESIAN_POINT('Ctrl Pts',(-62.8608949768583,34.6367946577241,12.));
#89536=CARTESIAN_POINT('Ctrl Pts',(-62.884195524682,34.6406242228606,0.));
#89537=CARTESIAN_POINT('Ctrl Pts',(-62.884195524682,34.6406242228606,12.));
#89538=CARTESIAN_POINT('Ctrl Pts',(-62.9075424760042,34.6444378222425,0.));
#89539=CARTESIAN_POINT('Ctrl Pts',(-62.9075424760042,34.6444378222425,12.));
#89540=CARTESIAN_POINT('Ctrl Pts',(-62.9309357186733,34.6482353737433,0.));
#89541=CARTESIAN_POINT('Ctrl Pts',(-62.9309357186733,34.6482353737433,12.));
#89542=CARTESIAN_POINT('Ctrl Pts',(-62.9543751409648,34.6520167956656,0.));
#89543=CARTESIAN_POINT('Ctrl Pts',(-62.9543751409648,34.6520167956656,12.));
#89544=CARTESIAN_POINT('Ctrl Pts',(-62.9778606315777,34.6557820067389,0.));
#89545=CARTESIAN_POINT('Ctrl Pts',(-62.9778606315777,34.6557820067389,12.));
#89546=CARTESIAN_POINT('Ctrl Pts',(-63.0013920796225,34.6595309261185,0.));
#89547=CARTESIAN_POINT('Ctrl Pts',(-63.0013920796225,34.6595309261185,12.));
#89548=CARTESIAN_POINT('Ctrl Pts',(-63.0249693746199,34.6632634733819,0.));
#89549=CARTESIAN_POINT('Ctrl Pts',(-63.0249693746199,34.6632634733819,12.));
#89550=CARTESIAN_POINT('Ctrl Pts',(-63.0485924065039,34.6669795685225,0.));
#89551=CARTESIAN_POINT('Ctrl Pts',(-63.0485924065039,34.6669795685225,12.));
#89552=CARTESIAN_POINT('Ctrl Pts',(-63.0722610656194,34.670679131947,0.));
#89553=CARTESIAN_POINT('Ctrl Pts',(-63.0722610656194,34.670679131947,12.));
#89554=CARTESIAN_POINT('Ctrl Pts',(-63.095975242717,34.6743620844721,0.));
#89555=CARTESIAN_POINT('Ctrl Pts',(-63.095975242717,34.6743620844721,12.));
#89556=CARTESIAN_POINT('Ctrl Pts',(-63.1197348289431,34.6780283473252,0.));
#89557=CARTESIAN_POINT('Ctrl Pts',(-63.1197348289431,34.6780283473252,12.));
#89558=CARTESIAN_POINT('Ctrl Pts',(-63.1435397158386,34.68167784214,0.));
#89559=CARTESIAN_POINT('Ctrl Pts',(-63.1435397158386,34.68167784214,12.));
#89560=CARTESIAN_POINT('Ctrl Pts',(-63.1673897953425,34.6853104909516,0.));
#89561=CARTESIAN_POINT('Ctrl Pts',(-63.1673897953425,34.6853104909516,12.));
#89562=CARTESIAN_POINT('Ctrl Pts',(-63.1912849597885,34.6889262161923,0.));
#89563=CARTESIAN_POINT('Ctrl Pts',(-63.1912849597885,34.6889262161923,12.));
#89564=CARTESIAN_POINT('Ctrl Pts',(-63.2152251019014,34.6925249406898,0.));
#89565=CARTESIAN_POINT('Ctrl Pts',(-63.2152251019014,34.6925249406898,12.));
#89566=CARTESIAN_POINT('Ctrl Pts',(-63.2392101147854,34.696106587667,0.));
#89567=CARTESIAN_POINT('Ctrl Pts',(-63.2392101147854,34.696106587667,12.));
#89568=CARTESIAN_POINT('Ctrl Pts',(-63.2632398919234,34.6996710807384,0.));
#89569=CARTESIAN_POINT('Ctrl Pts',(-63.2632398919234,34.6996710807384,12.));
#89570=CARTESIAN_POINT('Ctrl Pts',(-63.2873143271813,34.7032183439045,0.));
#89571=CARTESIAN_POINT('Ctrl Pts',(-63.2873143271813,34.7032183439045,12.));
#89572=CARTESIAN_POINT('Ctrl Pts',(-63.311433314805,34.7067483015492,0.));
#89573=CARTESIAN_POINT('Ctrl Pts',(-63.311433314805,34.7067483015492,12.));
#89574=CARTESIAN_POINT('Ctrl Pts',(-63.3355967494169,34.7102608784372,0.));
#89575=CARTESIAN_POINT('Ctrl Pts',(-63.3355967494169,34.7102608784372,12.));
#89576=CARTESIAN_POINT('Ctrl Pts',(-63.359804526005,34.7137559997143,0.));
#89577=CARTESIAN_POINT('Ctrl Pts',(-63.359804526005,34.7137559997143,12.));
#89578=CARTESIAN_POINT('Ctrl Pts',(-63.3840565399207,34.7172335909037,0.));
#89579=CARTESIAN_POINT('Ctrl Pts',(-63.3840565399207,34.7172335909037,12.));
#89580=CARTESIAN_POINT('Ctrl Pts',(-63.4083526868837,34.7206935779007,0.));
#89581=CARTESIAN_POINT('Ctrl Pts',(-63.4083526868837,34.7206935779007,12.));
#89582=CARTESIAN_POINT('Ctrl Pts',(-63.4326928629797,34.7241358869701,0.));
#89583=CARTESIAN_POINT('Ctrl Pts',(-63.4326928629797,34.7241358869701,12.));
#89584=CARTESIAN_POINT('Ctrl Pts',(-63.4570769646568,34.7275604447438,0.));
#89585=CARTESIAN_POINT('Ctrl Pts',(-63.4570769646568,34.7275604447438,12.));
#89586=CARTESIAN_POINT('Ctrl Pts',(-63.4815048887161,34.7309671782211,0.));
#89587=CARTESIAN_POINT('Ctrl Pts',(-63.4815048887161,34.7309671782211,12.));
#89588=CARTESIAN_POINT('Ctrl Pts',(-63.5059765323082,34.7343560147663,0.));
#89589=CARTESIAN_POINT('Ctrl Pts',(-63.5059765323082,34.7343560147663,12.));
#89590=CARTESIAN_POINT('Ctrl Pts',(-63.5304917929378,34.7377268821022,0.));
#89591=CARTESIAN_POINT('Ctrl Pts',(-63.5304917929378,34.7377268821022,12.));
#89592=CARTESIAN_POINT('Ctrl Pts',(-63.5550505684621,34.7410797083079,0.));
#89593=CARTESIAN_POINT('Ctrl Pts',(-63.5550505684621,34.7410797083079,12.));
#89594=CARTESIAN_POINT('Ctrl Pts',(-63.5796527570874,34.7444144218162,0.));
#89595=CARTESIAN_POINT('Ctrl Pts',(-63.5796527570874,34.7444144218162,12.));
#89596=CARTESIAN_POINT('Ctrl Pts',(-63.6042982573599,34.7477309514142,0.));
#89597=CARTESIAN_POINT('Ctrl Pts',(-63.6042982573599,34.7477309514142,12.));
#89598=CARTESIAN_POINT('Ctrl Pts',(-63.628986968162,34.7510292262415,0.));
#89599=CARTESIAN_POINT('Ctrl Pts',(-63.628986968162,34.7510292262415,12.));
#89600=CARTESIAN_POINT('Ctrl Pts',(-63.6537187887174,34.7543091757841,0.));
#89601=CARTESIAN_POINT('Ctrl Pts',(-63.6537187887174,34.7543091757841,12.));
#89602=CARTESIAN_POINT('Ctrl Pts',(-63.6784936185893,34.7575707298718,0.));
#89603=CARTESIAN_POINT('Ctrl Pts',(-63.6784936185893,34.7575707298718,12.));
#89604=CARTESIAN_POINT('Ctrl Pts',(-63.7033113576782,34.7608138186757,0.));
#89605=CARTESIAN_POINT('Ctrl Pts',(-63.7033113576782,34.7608138186757,12.));
#89606=CARTESIAN_POINT('Ctrl Pts',(-63.7281719062136,34.7640383727093,0.));
#89607=CARTESIAN_POINT('Ctrl Pts',(-63.7281719062136,34.7640383727093,12.));
#89608=CARTESIAN_POINT('Ctrl Pts',(-63.7530751647479,34.7672443228266,0.));
#89609=CARTESIAN_POINT('Ctrl Pts',(-63.7530751647479,34.7672443228266,12.));
#89610=CARTESIAN_POINT('Ctrl Pts',(-63.7780210341619,34.7704316002165,0.));
#89611=CARTESIAN_POINT('Ctrl Pts',(-63.7780210341619,34.7704316002165,12.));
#89612=CARTESIAN_POINT('Ctrl Pts',(-63.8030094156635,34.7736001363991,0.));
#89613=CARTESIAN_POINT('Ctrl Pts',(-63.8030094156635,34.7736001363991,12.));
#89614=CARTESIAN_POINT('Ctrl Pts',(-63.8280402107858,34.7767498632244,0.));
#89615=CARTESIAN_POINT('Ctrl Pts',(-63.8280402107858,34.7767498632244,12.));
#89616=CARTESIAN_POINT('Ctrl Pts',(-63.8531133213794,34.7798807128715,0.));
#89617=CARTESIAN_POINT('Ctrl Pts',(-63.8531133213794,34.7798807128715,12.));
#89618=CARTESIAN_POINT('Ctrl Pts',(-63.8782286496059,34.7829926178495,0.));
#89619=CARTESIAN_POINT('Ctrl Pts',(-63.8782286496059,34.7829926178495,12.));
#89620=CARTESIAN_POINT('Ctrl Pts',(-63.9033860979429,34.7860855109907,0.));
#89621=CARTESIAN_POINT('Ctrl Pts',(-63.9033860979429,34.7860855109907,12.));
#89622=CARTESIAN_POINT('Ctrl Pts',(-63.9285855691839,34.7891593254485,0.));
#89623=CARTESIAN_POINT('Ctrl Pts',(-63.9285855691839,34.7891593254485,12.));
#89624=CARTESIAN_POINT('Ctrl Pts',(-63.9538269664366,34.7922139946943,0.));
#89625=CARTESIAN_POINT('Ctrl Pts',(-63.9538269664366,34.7922139946943,12.));
#89626=CARTESIAN_POINT('Ctrl Pts',(-63.9791101931169,34.7952494525182,0.));
#89627=CARTESIAN_POINT('Ctrl Pts',(-63.9791101931169,34.7952494525182,12.));
#89628=CARTESIAN_POINT('Ctrl Pts',(-64.0044351529413,34.79826563303,0.));
#89629=CARTESIAN_POINT('Ctrl Pts',(-64.0044351529413,34.79826563303,12.));
#89630=CARTESIAN_POINT('Ctrl Pts',(-64.0298017499305,34.8012624706533,0.));
#89631=CARTESIAN_POINT('Ctrl Pts',(-64.0298017499305,34.8012624706533,12.));
#89632=CARTESIAN_POINT('Ctrl Pts',(-64.0552098884101,34.8042399001214,0.));
#89633=CARTESIAN_POINT('Ctrl Pts',(-64.0552098884101,34.8042399001214,12.));
#89634=CARTESIAN_POINT('Ctrl Pts',(-64.0806594730085,34.8071978564748,0.));
#89635=CARTESIAN_POINT('Ctrl Pts',(-64.0806594730085,34.8071978564748,12.));
#89636=CARTESIAN_POINT('Ctrl Pts',(-64.1061504086512,34.8101362750595,0.));
#89637=CARTESIAN_POINT('Ctrl Pts',(-64.1061504086512,34.8101362750595,12.));
#89638=CARTESIAN_POINT('Ctrl Pts',(-64.1316826005502,34.8130550915283,0.));
#89639=CARTESIAN_POINT('Ctrl Pts',(-64.1316826005502,34.8130550915283,12.));
#89640=CARTESIAN_POINT('Ctrl Pts',(-64.1572559542085,34.8159542418372,0.));
#89641=CARTESIAN_POINT('Ctrl Pts',(-64.1572559542085,34.8159542418372,12.));
#89642=CARTESIAN_POINT('Ctrl Pts',(-64.1828703754237,34.8188336622418,0.));
#89643=CARTESIAN_POINT('Ctrl Pts',(-64.1828703754237,34.8188336622418,12.));
#89644=CARTESIAN_POINT('Ctrl Pts',(-64.2085257702885,34.8216932892969,0.));
#89645=CARTESIAN_POINT('Ctrl Pts',(-64.2085257702885,34.8216932892969,12.));
#89646=CARTESIAN_POINT('Ctrl Pts',(-64.2342220451878,34.8245330598559,0.));
#89647=CARTESIAN_POINT('Ctrl Pts',(-64.2342220451878,34.8245330598559,12.));
#89648=CARTESIAN_POINT('Ctrl Pts',(-64.259959106791,34.8273529110742,0.));
#89649=CARTESIAN_POINT('Ctrl Pts',(-64.259959106791,34.8273529110742,12.));
#89650=CARTESIAN_POINT('Ctrl Pts',(-64.2857368620513,34.8301527804052,0.));
#89651=CARTESIAN_POINT('Ctrl Pts',(-64.2857368620513,34.8301527804052,12.));
#89652=CARTESIAN_POINT('Ctrl Pts',(-64.3115552182056,34.8329326055916,0.));
#89653=CARTESIAN_POINT('Ctrl Pts',(-64.3115552182056,34.8329326055916,12.));
#89654=CARTESIAN_POINT('Ctrl Pts',(-64.3374140827708,34.8356923246617,0.));
#89655=CARTESIAN_POINT('Ctrl Pts',(-64.3374140827708,34.8356923246617,12.));
#89656=CARTESIAN_POINT('Ctrl Pts',(-64.3633133635385,34.8384318759249,0.));
#89657=CARTESIAN_POINT('Ctrl Pts',(-64.3633133635385,34.8384318759249,12.));
#89658=CARTESIAN_POINT('Ctrl Pts',(-64.3892529685614,34.8411511979705,0.));
#89659=CARTESIAN_POINT('Ctrl Pts',(-64.3892529685614,34.8411511979705,12.));
#89660=CARTESIAN_POINT('Ctrl Pts',(-64.4152328061526,34.8438502296669,0.));
#89661=CARTESIAN_POINT('Ctrl Pts',(-64.4152328061526,34.8438502296669,12.));
#89662=CARTESIAN_POINT('Ctrl Pts',(-64.441252784898,34.8465289101626,0.));
#89663=CARTESIAN_POINT('Ctrl Pts',(-64.441252784898,34.8465289101626,12.));
#89664=CARTESIAN_POINT('Ctrl Pts',(-64.4673128136631,34.8491871788898,0.));
#89665=CARTESIAN_POINT('Ctrl Pts',(-64.4673128136631,34.8491871788898,12.));
#89666=CARTESIAN_POINT('Ctrl Pts',(-64.4934128015983,34.8518249755679,0.));
#89667=CARTESIAN_POINT('Ctrl Pts',(-64.4934128015983,34.8518249755679,12.));
#89668=CARTESIAN_POINT('Ctrl Pts',(-64.5195526581398,34.8544422402114,0.));
#89669=CARTESIAN_POINT('Ctrl Pts',(-64.5195526581398,34.8544422402114,12.));
#89670=CARTESIAN_POINT('Ctrl Pts',(-64.5457322930074,34.8570389131334,0.));
#89671=CARTESIAN_POINT('Ctrl Pts',(-64.5457322930074,34.8570389131334,12.));
#89672=CARTESIAN_POINT('Ctrl Pts',(-64.5719516161914,34.859614934925,0.));
#89673=CARTESIAN_POINT('Ctrl Pts',(-64.5719516161914,34.859614934925,12.));
#89674=CARTESIAN_POINT('Ctrl Pts',(-64.5982105379374,34.8621702464397,0.));
#89675=CARTESIAN_POINT('Ctrl Pts',(-64.5982105379374,34.8621702464397,12.));
#89676=CARTESIAN_POINT('Ctrl Pts',(-64.6245089687276,34.8647047887774,0.));
#89677=CARTESIAN_POINT('Ctrl Pts',(-64.6245089687276,34.8647047887774,12.));
#89678=CARTESIAN_POINT('Ctrl Pts',(-64.6508468192609,34.8672185032724,0.));
#89679=CARTESIAN_POINT('Ctrl Pts',(-64.6508468192609,34.8672185032724,12.));
#89680=CARTESIAN_POINT('Ctrl Pts',(-64.6772240004241,34.8697113314797,0.));
#89681=CARTESIAN_POINT('Ctrl Pts',(-64.6772240004241,34.8697113314797,12.));
#89682=CARTESIAN_POINT('Ctrl Pts',(-64.7036404233319,34.8721832151981,0.));
#89683=CARTESIAN_POINT('Ctrl Pts',(-64.7036404233319,34.8721832151981,12.));
#89684=CARTESIAN_POINT('Ctrl Pts',(-64.7300959993662,34.8746340964976,0.));
#89685=CARTESIAN_POINT('Ctrl Pts',(-64.7300959993662,34.8746340964976,12.));
#89686=CARTESIAN_POINT('Ctrl Pts',(-64.7565906402154,34.8770639177494,0.));
#89687=CARTESIAN_POINT('Ctrl Pts',(-64.7565906402154,34.8770639177494,12.));
#89688=CARTESIAN_POINT('Ctrl Pts',(-64.7831242579023,34.8794726216511,0.));
#89689=CARTESIAN_POINT('Ctrl Pts',(-64.7831242579023,34.8794726216511,12.));
#89690=CARTESIAN_POINT('Ctrl Pts',(-64.80969676483,34.8818601512726,0.));
#89691=CARTESIAN_POINT('Ctrl Pts',(-64.80969676483,34.8818601512726,12.));
#89692=CARTESIAN_POINT('Ctrl Pts',(-64.8363080737369,34.8842264500184,0.));
#89693=CARTESIAN_POINT('Ctrl Pts',(-64.8363080737369,34.8842264500184,12.));
#89694=CARTESIAN_POINT('Ctrl Pts',(-64.8629580976057,34.8865714615433,0.));
#89695=CARTESIAN_POINT('Ctrl Pts',(-64.8629580976057,34.8865714615433,12.));
#89696=CARTESIAN_POINT('Ctrl Pts',(-64.8896467495755,34.8888951296809,0.));
#89697=CARTESIAN_POINT('Ctrl Pts',(-64.8896467495755,34.8888951296809,12.));
#89698=CARTESIAN_POINT('Ctrl Pts',(-64.9163739428606,34.8911973983785,0.));
#89699=CARTESIAN_POINT('Ctrl Pts',(-64.9163739428606,34.8911973983785,12.));
#89700=CARTESIAN_POINT('Ctrl Pts',(-64.9431395906341,34.8934782116097,0.));
#89701=CARTESIAN_POINT('Ctrl Pts',(-64.9431395906341,34.8934782116097,12.));
#89702=CARTESIAN_POINT('Ctrl Pts',(-64.9699436060178,34.8957375133702,0.));
#89703=CARTESIAN_POINT('Ctrl Pts',(-64.9699436060178,34.8957375133702,12.));
#89704=CARTESIAN_POINT('Ctrl Pts',(-64.9967859023225,34.8979752478623,0.));
#89705=CARTESIAN_POINT('Ctrl Pts',(-64.9967859023225,34.8979752478623,12.));
#89706=CARTESIAN_POINT('Ctrl Pts',(-65.0236663932338,34.9001913596421,0.));
#89707=CARTESIAN_POINT('Ctrl Pts',(-65.0236663932338,34.9001913596421,12.));
#89708=CARTESIAN_POINT('Ctrl Pts',(-65.0505849930173,34.9023857937866,0.));
#89709=CARTESIAN_POINT('Ctrl Pts',(-65.0505849930173,34.9023857937866,12.));
#89710=CARTESIAN_POINT('Ctrl Pts',(-65.0775416167073,34.9045584960503,0.));
#89711=CARTESIAN_POINT('Ctrl Pts',(-65.0775416167073,34.9045584960503,12.));
#89712=CARTESIAN_POINT('Ctrl Pts',(-65.1045361803097,34.9067094130386,0.));
#89713=CARTESIAN_POINT('Ctrl Pts',(-65.1045361803097,34.9067094130386,12.));
#89714=CARTESIAN_POINT('Ctrl Pts',(-65.1315686003485,34.9088384918321,0.));
#89715=CARTESIAN_POINT('Ctrl Pts',(-65.1315686003485,34.9088384918321,12.));
#89716=CARTESIAN_POINT('Ctrl Pts',(-65.1586387934216,34.9109456796201,0.));
#89717=CARTESIAN_POINT('Ctrl Pts',(-65.1586387934216,34.9109456796201,12.));
#89718=CARTESIAN_POINT('Ctrl Pts',(-65.1857466757082,34.9130309233017,0.));
#89719=CARTESIAN_POINT('Ctrl Pts',(-65.1857466757082,34.9130309233017,12.));
#89720=CARTESIAN_POINT('Ctrl Pts',(-65.2128921625838,34.9150941691754,0.));
#89721=CARTESIAN_POINT('Ctrl Pts',(-65.2128921625838,34.9150941691754,12.));
#89722=CARTESIAN_POINT('Ctrl Pts',(-65.2400751679586,34.9171353624131,0.));
#89723=CARTESIAN_POINT('Ctrl Pts',(-65.2400751679586,34.9171353624131,12.));
#89724=CARTESIAN_POINT('Ctrl Pts',(-65.2672956048121,34.9191544474898,0.));
#89725=CARTESIAN_POINT('Ctrl Pts',(-65.2672956048121,34.9191544474898,12.));
#89726=CARTESIAN_POINT('Ctrl Pts',(-65.2945533863812,34.921151369138,0.));
#89727=CARTESIAN_POINT('Ctrl Pts',(-65.2945533863812,34.921151369138,12.));
#89728=CARTESIAN_POINT('Ctrl Pts',(-65.3218484271941,34.9231260731846,0.));
#89729=CARTESIAN_POINT('Ctrl Pts',(-65.3218484271941,34.9231260731846,12.));
#89730=CARTESIAN_POINT('Ctrl Pts',(-65.3491806440529,34.9250785073473,0.));
#89731=CARTESIAN_POINT('Ctrl Pts',(-65.3491806440529,34.9250785073473,12.));
#89732=CARTESIAN_POINT('Ctrl Pts',(-65.3765499573019,34.9270086222703,0.));
#89733=CARTESIAN_POINT('Ctrl Pts',(-65.3765499573019,34.9270086222703,12.));
#89734=CARTESIAN_POINT('Ctrl Pts',(-65.4039562911255,34.92891637177,0.));
#89735=CARTESIAN_POINT('Ctrl Pts',(-65.4039562911255,34.92891637177,12.));
#89736=CARTESIAN_POINT('Ctrl Pts',(-65.4313995707423,34.9308017105481,0.));
#89737=CARTESIAN_POINT('Ctrl Pts',(-65.4313995707423,34.9308017105481,12.));
#89738=CARTESIAN_POINT('Ctrl Pts',(-65.4588797201884,34.9326645923897,0.));
#89739=CARTESIAN_POINT('Ctrl Pts',(-65.4588797201884,34.9326645923897,12.));
#89740=CARTESIAN_POINT('Ctrl Pts',(-65.4863966597524,34.9345049680816,0.));
#89741=CARTESIAN_POINT('Ctrl Pts',(-65.4863966597524,34.9345049680816,12.));
#89742=CARTESIAN_POINT('Ctrl Pts',(-65.5139503038116,34.9363227836621,0.));
#89743=CARTESIAN_POINT('Ctrl Pts',(-65.5139503038116,34.9363227836621,12.));
#89744=CARTESIAN_POINT('Ctrl Pts',(-65.5415405578138,34.9381179779762,0.));
#89745=CARTESIAN_POINT('Ctrl Pts',(-65.5415405578138,34.9381179779762,12.));
#89746=CARTESIAN_POINT('Ctrl Pts',(-65.5691673226051,34.9398904862278,0.));
#89747=CARTESIAN_POINT('Ctrl Pts',(-65.5691673226051,34.9398904862278,12.));
#89748=CARTESIAN_POINT('Ctrl Pts',(-65.5968304997822,34.9416402443551,0.));
#89749=CARTESIAN_POINT('Ctrl Pts',(-65.5968304997822,34.9416402443551,12.));
#89750=CARTESIAN_POINT('Ctrl Pts',(-65.6245299968636,34.9433671932982,0.));
#89751=CARTESIAN_POINT('Ctrl Pts',(-65.6245299968636,34.9433671932982,12.));
#89752=CARTESIAN_POINT('Ctrl Pts',(-65.652265732124,34.9450712829142,0.));
#89753=CARTESIAN_POINT('Ctrl Pts',(-65.652265732124,34.9450712829142,12.));
#89754=CARTESIAN_POINT('Ctrl Pts',(-65.6800376405722,34.9467524770271,0.));
#89755=CARTESIAN_POINT('Ctrl Pts',(-65.6800376405722,34.9467524770271,12.));
#89756=CARTESIAN_POINT('Ctrl Pts',(-65.707845675746,34.9484107543856,0.));
#89757=CARTESIAN_POINT('Ctrl Pts',(-65.707845675746,34.9484107543856,12.));
#89758=CARTESIAN_POINT('Ctrl Pts',(-65.7356898060478,34.9500461042919,0.));
#89759=CARTESIAN_POINT('Ctrl Pts',(-65.7356898060478,34.9500461042919,12.));
#89760=CARTESIAN_POINT('Ctrl Pts',(-65.757993971173,34.9513360397181,0.));
#89761=CARTESIAN_POINT('Ctrl Pts',(-65.757993971173,34.9513360397181,12.));
#89762=CARTESIAN_POINT('Ctrl Pts',(-65.7747383250775,34.9522931728594,0.));
#89763=CARTESIAN_POINT('Ctrl Pts',(-65.7747383250775,34.9522931728594,12.));
#89764=CARTESIAN_POINT('Ctrl Pts',(-65.7859084407494,34.9529266758405,0.));
#89765=CARTESIAN_POINT('Ctrl Pts',(-65.7859084407494,34.9529266758405,12.));
#89766=CARTESIAN_POINT('Ctrl Pts',(-65.7914953018525,34.9532422808861,0.));
#89767=CARTESIAN_POINT('Ctrl Pts',(-65.7914953018525,34.9532422808861,12.));
#89768=CARTESIAN_POINT('',(-61.0441813777723,34.2579614092497,0.));
#89769=CARTESIAN_POINT('Ctrl Pts',(-61.0441813777723,34.2579614092497,0.));
#89770=CARTESIAN_POINT('Ctrl Pts',(-61.0479423318725,34.2589297755433,0.));
#89771=CARTESIAN_POINT('Ctrl Pts',(-61.0554700176998,34.2608658001631,0.));
#89772=CARTESIAN_POINT('Ctrl Pts',(-61.0667788793266,34.2637677131934,0.));
#89773=CARTESIAN_POINT('Ctrl Pts',(-61.0818920286293,34.2676326825626,0.));
#89774=CARTESIAN_POINT('Ctrl Pts',(-61.1008412399997,34.2724568037227,0.));
#89775=CARTESIAN_POINT('Ctrl Pts',(-61.1198481997764,34.277273803877,0.));
#89776=CARTESIAN_POINT('Ctrl Pts',(-61.1389128461886,34.2820836244469,0.));
#89777=CARTESIAN_POINT('Ctrl Pts',(-61.1580350635533,34.2868861666384,0.));
#89778=CARTESIAN_POINT('Ctrl Pts',(-61.1772146833205,34.2916812929751,0.));
#89779=CARTESIAN_POINT('Ctrl Pts',(-61.1964515073891,34.2964688443663,0.));
#89780=CARTESIAN_POINT('Ctrl Pts',(-61.2157453259107,34.3012486533474,0.));
#89781=CARTESIAN_POINT('Ctrl Pts',(-61.235095936694,34.3060205584064,0.));
#89782=CARTESIAN_POINT('Ctrl Pts',(-61.2545031656133,34.3107844191043,0.));
#89783=CARTESIAN_POINT('Ctrl Pts',(-61.2739668600365,34.3155401111747,0.));
#89784=CARTESIAN_POINT('Ctrl Pts',(-61.2934868791855,34.3202875193617,0.));
#89785=CARTESIAN_POINT('Ctrl Pts',(-61.3130630861386,34.3250265314768,0.));
#89786=CARTESIAN_POINT('Ctrl Pts',(-61.3326953378851,34.3297570310146,0.));
#89787=CARTESIAN_POINT('Ctrl Pts',(-61.3523834803188,34.3344788934363,0.));
#89788=CARTESIAN_POINT('Ctrl Pts',(-61.3721273534257,34.339191990014,0.));
#89789=CARTESIAN_POINT('Ctrl Pts',(-61.3919267945302,34.3438961902405,0.));
#89790=CARTESIAN_POINT('Ctrl Pts',(-61.4117816420229,34.3485913645979,0.));
#89791=CARTESIAN_POINT('Ctrl Pts',(-61.4316917395918,34.3532773877089,0.));
#89792=CARTESIAN_POINT('Ctrl Pts',(-61.4516569360454,34.3579541381996,0.));
#89793=CARTESIAN_POINT('Ctrl Pts',(-61.4716770832897,34.3626214971888,0.));
#89794=CARTESIAN_POINT('Ctrl Pts',(-61.4917520349279,34.3672793472465,0.));
#89795=CARTESIAN_POINT('Ctrl Pts',(-61.5118816445437,34.3719275711195,0.));
#89796=CARTESIAN_POINT('Ctrl Pts',(-61.5320657642639,34.376566050668,0.));
#89797=CARTESIAN_POINT('Ctrl Pts',(-61.5523042455158,34.3811946674196,0.));
#89798=CARTESIAN_POINT('Ctrl Pts',(-61.5725969396829,34.3858133030518,0.));
#89799=CARTESIAN_POINT('Ctrl Pts',(-61.5929436987409,34.3904218398636,0.));
#89800=CARTESIAN_POINT('Ctrl Pts',(-61.6133443760142,34.3950201613432,0.));
#89801=CARTESIAN_POINT('Ctrl Pts',(-61.6337988264556,34.3996081523753,0.));
#89802=CARTESIAN_POINT('Ctrl Pts',(-61.6543069062416,34.4041856989316,0.));
#89803=CARTESIAN_POINT('Ctrl Pts',(-61.6748684725205,34.4087526878812,0.));
#89804=CARTESIAN_POINT('Ctrl Pts',(-61.695483383117,34.4133090067703,0.));
#89805=CARTESIAN_POINT('Ctrl Pts',(-61.7161514961915,34.4178545435766,0.));
#89806=CARTESIAN_POINT('Ctrl Pts',(-61.7368726702596,34.4223891867179,0.));
#89807=CARTESIAN_POINT('Ctrl Pts',(-61.7576467643432,34.4269128251576,0.));
#89808=CARTESIAN_POINT('Ctrl Pts',(-61.7784736380727,34.4314253484791,0.));
#89809=CARTESIAN_POINT('Ctrl Pts',(-61.7993531518037,34.4359266469749,0.));
#89810=CARTESIAN_POINT('Ctrl Pts',(-61.8202851667222,34.4404166117299,0.));
#89811=CARTESIAN_POINT('Ctrl Pts',(-61.8412695447926,34.4448951345739,0.));
#89812=CARTESIAN_POINT('Ctrl Pts',(-61.8623061487018,34.449362108036,0.));
#89813=CARTESIAN_POINT('Ctrl Pts',(-61.8833948418025,34.4538174253012,0.));
#89814=CARTESIAN_POINT('Ctrl Pts',(-61.9045354880445,34.4582609801637,0.));
#89815=CARTESIAN_POINT('Ctrl Pts',(-61.9257279519308,34.4626926669974,0.));
#89816=CARTESIAN_POINT('Ctrl Pts',(-61.9469720985531,34.4671123807717,0.));
#89817=CARTESIAN_POINT('Ctrl Pts',(-61.9682677936054,34.4715200170592,0.));
#89818=CARTESIAN_POINT('Ctrl Pts',(-61.9896149034001,34.4759154720473,0.));
#89819=CARTESIAN_POINT('Ctrl Pts',(-62.0110132948794,34.4802986425528,0.));
#89820=CARTESIAN_POINT('Ctrl Pts',(-62.0324628356141,34.4846694260199,0.));
#89821=CARTESIAN_POINT('Ctrl Pts',(-62.0539633937939,34.4890277205039,0.));
#89822=CARTESIAN_POINT('Ctrl Pts',(-62.0755148382135,34.4933734246592,0.));
#89823=CARTESIAN_POINT('Ctrl Pts',(-62.0971170382567,34.4977064377282,0.));
#89824=CARTESIAN_POINT('Ctrl Pts',(-62.1187698638707,34.5020266595293,0.));
#89825=CARTESIAN_POINT('Ctrl Pts',(-62.1404731855687,34.5063339904533,0.));
#89826=CARTESIAN_POINT('Ctrl Pts',(-62.1622268744337,34.5106283314594,0.));
#89827=CARTESIAN_POINT('Ctrl Pts',(-62.1840308021171,34.5149095840729,0.));
#89828=CARTESIAN_POINT('Ctrl Pts',(-62.2058848408346,34.5191776503843,0.));
#89829=CARTESIAN_POINT('Ctrl Pts',(-62.2277888633577,34.5234324330492,0.));
#89830=CARTESIAN_POINT('Ctrl Pts',(-62.2497427430136,34.527673835281,0.));
#89831=CARTESIAN_POINT('Ctrl Pts',(-62.2717463536828,34.5319017608434,0.));
#89832=CARTESIAN_POINT('Ctrl Pts',(-62.2937995697927,34.536116114045,0.));
#89833=CARTESIAN_POINT('Ctrl Pts',(-62.3159022663052,34.5403167997333,0.));
#89834=CARTESIAN_POINT('Ctrl Pts',(-62.3380543187067,34.5445037232928,0.));
#89835=CARTESIAN_POINT('Ctrl Pts',(-62.3602556030114,34.5486767906376,0.));
#89836=CARTESIAN_POINT('Ctrl Pts',(-62.3825059957593,34.552835908207,0.));
#89837=CARTESIAN_POINT('Ctrl Pts',(-62.4048053740129,34.5569809829615,0.));
#89838=CARTESIAN_POINT('Ctrl Pts',(-62.4271536153473,34.5611119223807,0.));
#89839=CARTESIAN_POINT('Ctrl Pts',(-62.4495505978415,34.5652286344606,0.));
#89840=CARTESIAN_POINT('Ctrl Pts',(-62.471996200083,34.5693310277064,0.));
#89841=CARTESIAN_POINT('Ctrl Pts',(-62.494490301164,34.5734190111279,0.));
#89842=CARTESIAN_POINT('Ctrl Pts',(-62.5170327806774,34.5774924942351,0.));
#89843=CARTESIAN_POINT('Ctrl Pts',(-62.5396235187053,34.5815513870363,0.));
#89844=CARTESIAN_POINT('Ctrl Pts',(-62.5622623958125,34.5855956000343,0.));
#89845=CARTESIAN_POINT('Ctrl Pts',(-62.5849492930501,34.5896250442199,0.));
#89846=CARTESIAN_POINT('Ctrl Pts',(-62.6076840919521,34.5936396310671,0.));
#89847=CARTESIAN_POINT('Ctrl Pts',(-62.6304666745319,34.5976392725303,0.));
#89848=CARTESIAN_POINT('Ctrl Pts',(-62.6532969232695,34.6016238810419,0.));
#89849=CARTESIAN_POINT('Ctrl Pts',(-62.6761747211081,34.6055933695093,0.));
#89850=CARTESIAN_POINT('Ctrl Pts',(-62.6990999514597,34.6095476513094,0.));
#89851=CARTESIAN_POINT('Ctrl Pts',(-62.7220724982005,34.6134866402842,0.));
#89852=CARTESIAN_POINT('Ctrl Pts',(-62.7450922456663,34.6174102507368,0.));
#89853=CARTESIAN_POINT('Ctrl Pts',(-62.7681590786398,34.6213183974302,0.));
#89854=CARTESIAN_POINT('Ctrl Pts',(-62.7912728823483,34.6252109955836,0.));
#89855=CARTESIAN_POINT('Ctrl Pts',(-62.8144335424671,34.629087960866,0.));
#89856=CARTESIAN_POINT('Ctrl Pts',(-62.8376409451167,34.6329492093931,0.));
#89857=CARTESIAN_POINT('Ctrl Pts',(-62.8608949768583,34.6367946577241,0.));
#89858=CARTESIAN_POINT('Ctrl Pts',(-62.884195524682,34.6406242228606,0.));
#89859=CARTESIAN_POINT('Ctrl Pts',(-62.9075424760042,34.6444378222425,0.));
#89860=CARTESIAN_POINT('Ctrl Pts',(-62.9309357186733,34.6482353737433,0.));
#89861=CARTESIAN_POINT('Ctrl Pts',(-62.9543751409648,34.6520167956656,0.));
#89862=CARTESIAN_POINT('Ctrl Pts',(-62.9778606315777,34.6557820067389,0.));
#89863=CARTESIAN_POINT('Ctrl Pts',(-63.0013920796225,34.6595309261185,0.));
#89864=CARTESIAN_POINT('Ctrl Pts',(-63.0249693746199,34.6632634733819,0.));
#89865=CARTESIAN_POINT('Ctrl Pts',(-63.0485924065039,34.6669795685225,0.));
#89866=CARTESIAN_POINT('Ctrl Pts',(-63.0722610656194,34.670679131947,0.));
#89867=CARTESIAN_POINT('Ctrl Pts',(-63.095975242717,34.6743620844721,0.));
#89868=CARTESIAN_POINT('Ctrl Pts',(-63.1197348289431,34.6780283473252,0.));
#89869=CARTESIAN_POINT('Ctrl Pts',(-63.1435397158386,34.68167784214,0.));
#89870=CARTESIAN_POINT('Ctrl Pts',(-63.1673897953425,34.6853104909516,0.));
#89871=CARTESIAN_POINT('Ctrl Pts',(-63.1912849597885,34.6889262161923,0.));
#89872=CARTESIAN_POINT('Ctrl Pts',(-63.2152251019014,34.6925249406898,0.));
#89873=CARTESIAN_POINT('Ctrl Pts',(-63.2392101147854,34.696106587667,0.));
#89874=CARTESIAN_POINT('Ctrl Pts',(-63.2632398919234,34.6996710807384,0.));
#89875=CARTESIAN_POINT('Ctrl Pts',(-63.2873143271813,34.7032183439045,0.));
#89876=CARTESIAN_POINT('Ctrl Pts',(-63.311433314805,34.7067483015492,0.));
#89877=CARTESIAN_POINT('Ctrl Pts',(-63.3355967494169,34.7102608784372,0.));
#89878=CARTESIAN_POINT('Ctrl Pts',(-63.359804526005,34.7137559997143,0.));
#89879=CARTESIAN_POINT('Ctrl Pts',(-63.3840565399207,34.7172335909037,0.));
#89880=CARTESIAN_POINT('Ctrl Pts',(-63.4083526868837,34.7206935779007,0.));
#89881=CARTESIAN_POINT('Ctrl Pts',(-63.4326928629797,34.7241358869701,0.));
#89882=CARTESIAN_POINT('Ctrl Pts',(-63.4570769646568,34.7275604447438,0.));
#89883=CARTESIAN_POINT('Ctrl Pts',(-63.4815048887161,34.7309671782211,0.));
#89884=CARTESIAN_POINT('Ctrl Pts',(-63.5059765323082,34.7343560147663,0.));
#89885=CARTESIAN_POINT('Ctrl Pts',(-63.5304917929378,34.7377268821022,0.));
#89886=CARTESIAN_POINT('Ctrl Pts',(-63.5550505684621,34.7410797083079,0.));
#89887=CARTESIAN_POINT('Ctrl Pts',(-63.5796527570874,34.7444144218162,0.));
#89888=CARTESIAN_POINT('Ctrl Pts',(-63.6042982573599,34.7477309514142,0.));
#89889=CARTESIAN_POINT('Ctrl Pts',(-63.628986968162,34.7510292262415,0.));
#89890=CARTESIAN_POINT('Ctrl Pts',(-63.6537187887174,34.7543091757841,0.));
#89891=CARTESIAN_POINT('Ctrl Pts',(-63.6784936185893,34.7575707298718,0.));
#89892=CARTESIAN_POINT('Ctrl Pts',(-63.7033113576782,34.7608138186757,0.));
#89893=CARTESIAN_POINT('Ctrl Pts',(-63.7281719062136,34.7640383727093,0.));
#89894=CARTESIAN_POINT('Ctrl Pts',(-63.7530751647479,34.7672443228266,0.));
#89895=CARTESIAN_POINT('Ctrl Pts',(-63.7780210341619,34.7704316002165,0.));
#89896=CARTESIAN_POINT('Ctrl Pts',(-63.8030094156635,34.7736001363991,0.));
#89897=CARTESIAN_POINT('Ctrl Pts',(-63.8280402107858,34.7767498632244,0.));
#89898=CARTESIAN_POINT('Ctrl Pts',(-63.8531133213794,34.7798807128715,0.));
#89899=CARTESIAN_POINT('Ctrl Pts',(-63.8782286496059,34.7829926178495,0.));
#89900=CARTESIAN_POINT('Ctrl Pts',(-63.9033860979429,34.7860855109907,0.));
#89901=CARTESIAN_POINT('Ctrl Pts',(-63.9285855691839,34.7891593254485,0.));
#89902=CARTESIAN_POINT('Ctrl Pts',(-63.9538269664366,34.7922139946943,0.));
#89903=CARTESIAN_POINT('Ctrl Pts',(-63.9791101931169,34.7952494525182,0.));
#89904=CARTESIAN_POINT('Ctrl Pts',(-64.0044351529413,34.79826563303,0.));
#89905=CARTESIAN_POINT('Ctrl Pts',(-64.0298017499305,34.8012624706533,0.));
#89906=CARTESIAN_POINT('Ctrl Pts',(-64.0552098884101,34.8042399001214,0.));
#89907=CARTESIAN_POINT('Ctrl Pts',(-64.0806594730085,34.8071978564748,0.));
#89908=CARTESIAN_POINT('Ctrl Pts',(-64.1061504086512,34.8101362750595,0.));
#89909=CARTESIAN_POINT('Ctrl Pts',(-64.1316826005502,34.8130550915283,0.));
#89910=CARTESIAN_POINT('Ctrl Pts',(-64.1572559542085,34.8159542418372,0.));
#89911=CARTESIAN_POINT('Ctrl Pts',(-64.1828703754237,34.8188336622418,0.));
#89912=CARTESIAN_POINT('Ctrl Pts',(-64.2085257702885,34.8216932892969,0.));
#89913=CARTESIAN_POINT('Ctrl Pts',(-64.2342220451878,34.8245330598559,0.));
#89914=CARTESIAN_POINT('Ctrl Pts',(-64.259959106791,34.8273529110742,0.));
#89915=CARTESIAN_POINT('Ctrl Pts',(-64.2857368620513,34.8301527804052,0.));
#89916=CARTESIAN_POINT('Ctrl Pts',(-64.3115552182056,34.8329326055916,0.));
#89917=CARTESIAN_POINT('Ctrl Pts',(-64.3374140827708,34.8356923246617,0.));
#89918=CARTESIAN_POINT('Ctrl Pts',(-64.3633133635385,34.8384318759249,0.));
#89919=CARTESIAN_POINT('Ctrl Pts',(-64.3892529685614,34.8411511979705,0.));
#89920=CARTESIAN_POINT('Ctrl Pts',(-64.4152328061526,34.8438502296669,0.));
#89921=CARTESIAN_POINT('Ctrl Pts',(-64.441252784898,34.8465289101626,0.));
#89922=CARTESIAN_POINT('Ctrl Pts',(-64.4673128136631,34.8491871788898,0.));
#89923=CARTESIAN_POINT('Ctrl Pts',(-64.4934128015983,34.8518249755679,0.));
#89924=CARTESIAN_POINT('Ctrl Pts',(-64.5195526581398,34.8544422402114,0.));
#89925=CARTESIAN_POINT('Ctrl Pts',(-64.5457322930074,34.8570389131334,0.));
#89926=CARTESIAN_POINT('Ctrl Pts',(-64.5719516161914,34.859614934925,0.));
#89927=CARTESIAN_POINT('Ctrl Pts',(-64.5982105379374,34.8621702464397,0.));
#89928=CARTESIAN_POINT('Ctrl Pts',(-64.6245089687276,34.8647047887774,0.));
#89929=CARTESIAN_POINT('Ctrl Pts',(-64.6508468192609,34.8672185032724,0.));
#89930=CARTESIAN_POINT('Ctrl Pts',(-64.6772240004241,34.8697113314797,0.));
#89931=CARTESIAN_POINT('Ctrl Pts',(-64.7036404233319,34.8721832151981,0.));
#89932=CARTESIAN_POINT('Ctrl Pts',(-64.7300959993662,34.8746340964976,0.));
#89933=CARTESIAN_POINT('Ctrl Pts',(-64.7565906402154,34.8770639177494,0.));
#89934=CARTESIAN_POINT('Ctrl Pts',(-64.7831242579023,34.8794726216511,0.));
#89935=CARTESIAN_POINT('Ctrl Pts',(-64.80969676483,34.8818601512726,0.));
#89936=CARTESIAN_POINT('Ctrl Pts',(-64.8363080737369,34.8842264500184,0.));
#89937=CARTESIAN_POINT('Ctrl Pts',(-64.8629580976057,34.8865714615433,0.));
#89938=CARTESIAN_POINT('Ctrl Pts',(-64.8896467495755,34.8888951296809,0.));
#89939=CARTESIAN_POINT('Ctrl Pts',(-64.9163739428606,34.8911973983785,0.));
#89940=CARTESIAN_POINT('Ctrl Pts',(-64.9431395906341,34.8934782116097,0.));
#89941=CARTESIAN_POINT('Ctrl Pts',(-64.9699436060178,34.8957375133702,0.));
#89942=CARTESIAN_POINT('Ctrl Pts',(-64.9967859023225,34.8979752478623,0.));
#89943=CARTESIAN_POINT('Ctrl Pts',(-65.0236663932338,34.9001913596421,0.));
#89944=CARTESIAN_POINT('Ctrl Pts',(-65.0505849930173,34.9023857937866,0.));
#89945=CARTESIAN_POINT('Ctrl Pts',(-65.0775416167073,34.9045584960503,0.));
#89946=CARTESIAN_POINT('Ctrl Pts',(-65.1045361803097,34.9067094130386,0.));
#89947=CARTESIAN_POINT('Ctrl Pts',(-65.1315686003485,34.9088384918321,0.));
#89948=CARTESIAN_POINT('Ctrl Pts',(-65.1586387934216,34.9109456796201,0.));
#89949=CARTESIAN_POINT('Ctrl Pts',(-65.1857466757082,34.9130309233017,0.));
#89950=CARTESIAN_POINT('Ctrl Pts',(-65.2128921625838,34.9150941691754,0.));
#89951=CARTESIAN_POINT('Ctrl Pts',(-65.2400751679586,34.9171353624131,0.));
#89952=CARTESIAN_POINT('Ctrl Pts',(-65.2672956048121,34.9191544474898,0.));
#89953=CARTESIAN_POINT('Ctrl Pts',(-65.2945533863812,34.921151369138,0.));
#89954=CARTESIAN_POINT('Ctrl Pts',(-65.3218484271941,34.9231260731846,0.));
#89955=CARTESIAN_POINT('Ctrl Pts',(-65.3491806440529,34.9250785073473,0.));
#89956=CARTESIAN_POINT('Ctrl Pts',(-65.3765499573019,34.9270086222703,0.));
#89957=CARTESIAN_POINT('Ctrl Pts',(-65.4039562911255,34.92891637177,0.));
#89958=CARTESIAN_POINT('Ctrl Pts',(-65.4274804996406,34.9305324724386,0.));
#89959=CARTESIAN_POINT('Ctrl Pts',(-65.4455359575001,34.9317593813102,0.));
#89960=CARTESIAN_POINT('Ctrl Pts',(-65.4581063193586,34.9326070346592,0.));
#89961=CARTESIAN_POINT('Ctrl Pts',(-65.4651808010454,34.9330820191483,0.));
#89962=CARTESIAN_POINT('Ctrl Pts',(-65.4667541477958,34.9331875523085,0.));
#89963=CARTESIAN_POINT('',(-61.0441813777723,34.2579614092497,12.));
#89964=CARTESIAN_POINT('',(-61.0441813777723,34.2579614092497,0.));
#89965=CARTESIAN_POINT('Ctrl Pts',(-65.4667541477958,34.9331875523085,12.));
#89966=CARTESIAN_POINT('Ctrl Pts',(-65.4651808010454,34.9330820191483,12.));
#89967=CARTESIAN_POINT('Ctrl Pts',(-65.4581063193585,34.9326070346592,12.));
#89968=CARTESIAN_POINT('Ctrl Pts',(-65.4455359575001,34.9317593813102,12.));
#89969=CARTESIAN_POINT('Ctrl Pts',(-65.4274804996406,34.9305324724386,12.));
#89970=CARTESIAN_POINT('Ctrl Pts',(-65.4039562911255,34.92891637177,12.));
#89971=CARTESIAN_POINT('Ctrl Pts',(-65.3765499573019,34.9270086222703,12.));
#89972=CARTESIAN_POINT('Ctrl Pts',(-65.3491806440529,34.9250785073473,12.));
#89973=CARTESIAN_POINT('Ctrl Pts',(-65.3218484271941,34.9231260731846,12.));
#89974=CARTESIAN_POINT('Ctrl Pts',(-65.2945533863812,34.921151369138,12.));
#89975=CARTESIAN_POINT('Ctrl Pts',(-65.2672956048121,34.9191544474898,12.));
#89976=CARTESIAN_POINT('Ctrl Pts',(-65.2400751679586,34.9171353624131,12.));
#89977=CARTESIAN_POINT('Ctrl Pts',(-65.2128921625838,34.9150941691754,12.));
#89978=CARTESIAN_POINT('Ctrl Pts',(-65.1857466757082,34.9130309233017,12.));
#89979=CARTESIAN_POINT('Ctrl Pts',(-65.1586387934216,34.9109456796201,12.));
#89980=CARTESIAN_POINT('Ctrl Pts',(-65.1315686003485,34.9088384918321,12.));
#89981=CARTESIAN_POINT('Ctrl Pts',(-65.1045361803097,34.9067094130386,12.));
#89982=CARTESIAN_POINT('Ctrl Pts',(-65.0775416167073,34.9045584960503,12.));
#89983=CARTESIAN_POINT('Ctrl Pts',(-65.0505849930173,34.9023857937866,12.));
#89984=CARTESIAN_POINT('Ctrl Pts',(-65.0236663932338,34.9001913596421,12.));
#89985=CARTESIAN_POINT('Ctrl Pts',(-64.9967859023225,34.8979752478623,12.));
#89986=CARTESIAN_POINT('Ctrl Pts',(-64.9699436060178,34.8957375133702,12.));
#89987=CARTESIAN_POINT('Ctrl Pts',(-64.9431395906341,34.8934782116097,12.));
#89988=CARTESIAN_POINT('Ctrl Pts',(-64.9163739428606,34.8911973983785,12.));
#89989=CARTESIAN_POINT('Ctrl Pts',(-64.8896467495755,34.8888951296809,12.));
#89990=CARTESIAN_POINT('Ctrl Pts',(-64.8629580976057,34.8865714615433,12.));
#89991=CARTESIAN_POINT('Ctrl Pts',(-64.8363080737369,34.8842264500184,12.));
#89992=CARTESIAN_POINT('Ctrl Pts',(-64.80969676483,34.8818601512726,12.));
#89993=CARTESIAN_POINT('Ctrl Pts',(-64.7831242579023,34.8794726216511,12.));
#89994=CARTESIAN_POINT('Ctrl Pts',(-64.7565906402154,34.8770639177494,12.));
#89995=CARTESIAN_POINT('Ctrl Pts',(-64.7300959993662,34.8746340964976,12.));
#89996=CARTESIAN_POINT('Ctrl Pts',(-64.7036404233319,34.8721832151981,12.));
#89997=CARTESIAN_POINT('Ctrl Pts',(-64.6772240004241,34.8697113314797,12.));
#89998=CARTESIAN_POINT('Ctrl Pts',(-64.6508468192609,34.8672185032724,12.));
#89999=CARTESIAN_POINT('Ctrl Pts',(-64.6245089687276,34.8647047887774,12.));
#90000=CARTESIAN_POINT('Ctrl Pts',(-64.5982105379374,34.8621702464397,12.));
#90001=CARTESIAN_POINT('Ctrl Pts',(-64.5719516161914,34.859614934925,12.));
#90002=CARTESIAN_POINT('Ctrl Pts',(-64.5457322930074,34.8570389131334,12.));
#90003=CARTESIAN_POINT('Ctrl Pts',(-64.5195526581398,34.8544422402114,12.));
#90004=CARTESIAN_POINT('Ctrl Pts',(-64.4934128015983,34.8518249755679,12.));
#90005=CARTESIAN_POINT('Ctrl Pts',(-64.4673128136631,34.8491871788898,12.));
#90006=CARTESIAN_POINT('Ctrl Pts',(-64.441252784898,34.8465289101626,12.));
#90007=CARTESIAN_POINT('Ctrl Pts',(-64.4152328061526,34.8438502296669,12.));
#90008=CARTESIAN_POINT('Ctrl Pts',(-64.3892529685614,34.8411511979705,12.));
#90009=CARTESIAN_POINT('Ctrl Pts',(-64.3633133635385,34.8384318759249,12.));
#90010=CARTESIAN_POINT('Ctrl Pts',(-64.3374140827708,34.8356923246617,12.));
#90011=CARTESIAN_POINT('Ctrl Pts',(-64.3115552182056,34.8329326055916,12.));
#90012=CARTESIAN_POINT('Ctrl Pts',(-64.2857368620513,34.8301527804052,12.));
#90013=CARTESIAN_POINT('Ctrl Pts',(-64.259959106791,34.8273529110742,12.));
#90014=CARTESIAN_POINT('Ctrl Pts',(-64.2342220451878,34.8245330598559,12.));
#90015=CARTESIAN_POINT('Ctrl Pts',(-64.2085257702885,34.8216932892969,12.));
#90016=CARTESIAN_POINT('Ctrl Pts',(-64.1828703754237,34.8188336622418,12.));
#90017=CARTESIAN_POINT('Ctrl Pts',(-64.1572559542085,34.8159542418372,12.));
#90018=CARTESIAN_POINT('Ctrl Pts',(-64.1316826005502,34.8130550915283,12.));
#90019=CARTESIAN_POINT('Ctrl Pts',(-64.1061504086512,34.8101362750595,12.));
#90020=CARTESIAN_POINT('Ctrl Pts',(-64.0806594730085,34.8071978564748,12.));
#90021=CARTESIAN_POINT('Ctrl Pts',(-64.0552098884101,34.8042399001214,12.));
#90022=CARTESIAN_POINT('Ctrl Pts',(-64.0298017499305,34.8012624706533,12.));
#90023=CARTESIAN_POINT('Ctrl Pts',(-64.0044351529413,34.79826563303,12.));
#90024=CARTESIAN_POINT('Ctrl Pts',(-63.9791101931169,34.7952494525182,12.));
#90025=CARTESIAN_POINT('Ctrl Pts',(-63.9538269664366,34.7922139946943,12.));
#90026=CARTESIAN_POINT('Ctrl Pts',(-63.9285855691839,34.7891593254485,12.));
#90027=CARTESIAN_POINT('Ctrl Pts',(-63.9033860979429,34.7860855109907,12.));
#90028=CARTESIAN_POINT('Ctrl Pts',(-63.8782286496059,34.7829926178495,12.));
#90029=CARTESIAN_POINT('Ctrl Pts',(-63.8531133213794,34.7798807128715,12.));
#90030=CARTESIAN_POINT('Ctrl Pts',(-63.8280402107858,34.7767498632244,12.));
#90031=CARTESIAN_POINT('Ctrl Pts',(-63.8030094156635,34.7736001363991,12.));
#90032=CARTESIAN_POINT('Ctrl Pts',(-63.7780210341619,34.7704316002165,12.));
#90033=CARTESIAN_POINT('Ctrl Pts',(-63.7530751647479,34.7672443228266,12.));
#90034=CARTESIAN_POINT('Ctrl Pts',(-63.7281719062136,34.7640383727093,12.));
#90035=CARTESIAN_POINT('Ctrl Pts',(-63.7033113576782,34.7608138186757,12.));
#90036=CARTESIAN_POINT('Ctrl Pts',(-63.6784936185893,34.7575707298718,12.));
#90037=CARTESIAN_POINT('Ctrl Pts',(-63.6537187887174,34.7543091757841,12.));
#90038=CARTESIAN_POINT('Ctrl Pts',(-63.628986968162,34.7510292262415,12.));
#90039=CARTESIAN_POINT('Ctrl Pts',(-63.6042982573599,34.7477309514142,12.));
#90040=CARTESIAN_POINT('Ctrl Pts',(-63.5796527570874,34.7444144218162,12.));
#90041=CARTESIAN_POINT('Ctrl Pts',(-63.5550505684621,34.7410797083079,12.));
#90042=CARTESIAN_POINT('Ctrl Pts',(-63.5304917929378,34.7377268821022,12.));
#90043=CARTESIAN_POINT('Ctrl Pts',(-63.5059765323082,34.7343560147663,12.));
#90044=CARTESIAN_POINT('Ctrl Pts',(-63.4815048887161,34.7309671782211,12.));
#90045=CARTESIAN_POINT('Ctrl Pts',(-63.4570769646568,34.7275604447438,12.));
#90046=CARTESIAN_POINT('Ctrl Pts',(-63.4326928629797,34.7241358869701,12.));
#90047=CARTESIAN_POINT('Ctrl Pts',(-63.4083526868837,34.7206935779007,12.));
#90048=CARTESIAN_POINT('Ctrl Pts',(-63.3840565399207,34.7172335909037,12.));
#90049=CARTESIAN_POINT('Ctrl Pts',(-63.359804526005,34.7137559997143,12.));
#90050=CARTESIAN_POINT('Ctrl Pts',(-63.3355967494169,34.7102608784372,12.));
#90051=CARTESIAN_POINT('Ctrl Pts',(-63.311433314805,34.7067483015492,12.));
#90052=CARTESIAN_POINT('Ctrl Pts',(-63.2873143271813,34.7032183439045,12.));
#90053=CARTESIAN_POINT('Ctrl Pts',(-63.2632398919234,34.6996710807384,12.));
#90054=CARTESIAN_POINT('Ctrl Pts',(-63.2392101147854,34.696106587667,12.));
#90055=CARTESIAN_POINT('Ctrl Pts',(-63.2152251019014,34.6925249406898,12.));
#90056=CARTESIAN_POINT('Ctrl Pts',(-63.1912849597885,34.6889262161923,12.));
#90057=CARTESIAN_POINT('Ctrl Pts',(-63.1673897953425,34.6853104909516,12.));
#90058=CARTESIAN_POINT('Ctrl Pts',(-63.1435397158386,34.68167784214,12.));
#90059=CARTESIAN_POINT('Ctrl Pts',(-63.1197348289431,34.6780283473252,12.));
#90060=CARTESIAN_POINT('Ctrl Pts',(-63.095975242717,34.6743620844721,12.));
#90061=CARTESIAN_POINT('Ctrl Pts',(-63.0722610656194,34.670679131947,12.));
#90062=CARTESIAN_POINT('Ctrl Pts',(-63.0485924065039,34.6669795685225,12.));
#90063=CARTESIAN_POINT('Ctrl Pts',(-63.0249693746199,34.6632634733819,12.));
#90064=CARTESIAN_POINT('Ctrl Pts',(-63.0013920796225,34.6595309261185,12.));
#90065=CARTESIAN_POINT('Ctrl Pts',(-62.9778606315777,34.6557820067389,12.));
#90066=CARTESIAN_POINT('Ctrl Pts',(-62.9543751409648,34.6520167956656,12.));
#90067=CARTESIAN_POINT('Ctrl Pts',(-62.9309357186733,34.6482353737433,12.));
#90068=CARTESIAN_POINT('Ctrl Pts',(-62.9075424760042,34.6444378222425,12.));
#90069=CARTESIAN_POINT('Ctrl Pts',(-62.884195524682,34.6406242228606,12.));
#90070=CARTESIAN_POINT('Ctrl Pts',(-62.8608949768583,34.6367946577241,12.));
#90071=CARTESIAN_POINT('Ctrl Pts',(-62.8376409451167,34.6329492093931,12.));
#90072=CARTESIAN_POINT('Ctrl Pts',(-62.8144335424671,34.629087960866,12.));
#90073=CARTESIAN_POINT('Ctrl Pts',(-62.7912728823483,34.6252109955836,12.));
#90074=CARTESIAN_POINT('Ctrl Pts',(-62.7681590786398,34.6213183974302,12.));
#90075=CARTESIAN_POINT('Ctrl Pts',(-62.7450922456663,34.6174102507368,12.));
#90076=CARTESIAN_POINT('Ctrl Pts',(-62.7220724982005,34.6134866402842,12.));
#90077=CARTESIAN_POINT('Ctrl Pts',(-62.6990999514597,34.6095476513094,12.));
#90078=CARTESIAN_POINT('Ctrl Pts',(-62.6761747211081,34.6055933695093,12.));
#90079=CARTESIAN_POINT('Ctrl Pts',(-62.6532969232695,34.6016238810419,12.));
#90080=CARTESIAN_POINT('Ctrl Pts',(-62.6304666745319,34.5976392725303,12.));
#90081=CARTESIAN_POINT('Ctrl Pts',(-62.6076840919521,34.5936396310671,12.));
#90082=CARTESIAN_POINT('Ctrl Pts',(-62.5849492930501,34.5896250442199,12.));
#90083=CARTESIAN_POINT('Ctrl Pts',(-62.5622623958125,34.5855956000343,12.));
#90084=CARTESIAN_POINT('Ctrl Pts',(-62.5396235187053,34.5815513870363,12.));
#90085=CARTESIAN_POINT('Ctrl Pts',(-62.5170327806774,34.5774924942351,12.));
#90086=CARTESIAN_POINT('Ctrl Pts',(-62.494490301164,34.5734190111279,12.));
#90087=CARTESIAN_POINT('Ctrl Pts',(-62.471996200083,34.5693310277064,12.));
#90088=CARTESIAN_POINT('Ctrl Pts',(-62.4495505978415,34.5652286344606,12.));
#90089=CARTESIAN_POINT('Ctrl Pts',(-62.4271536153473,34.5611119223807,12.));
#90090=CARTESIAN_POINT('Ctrl Pts',(-62.4048053740129,34.5569809829615,12.));
#90091=CARTESIAN_POINT('Ctrl Pts',(-62.3825059957593,34.552835908207,12.));
#90092=CARTESIAN_POINT('Ctrl Pts',(-62.3602556030114,34.5486767906376,12.));
#90093=CARTESIAN_POINT('Ctrl Pts',(-62.3380543187067,34.5445037232928,12.));
#90094=CARTESIAN_POINT('Ctrl Pts',(-62.3159022663052,34.5403167997333,12.));
#90095=CARTESIAN_POINT('Ctrl Pts',(-62.2937995697927,34.536116114045,12.));
#90096=CARTESIAN_POINT('Ctrl Pts',(-62.2717463536828,34.5319017608434,12.));
#90097=CARTESIAN_POINT('Ctrl Pts',(-62.2497427430136,34.527673835281,12.));
#90098=CARTESIAN_POINT('Ctrl Pts',(-62.2277888633577,34.5234324330492,12.));
#90099=CARTESIAN_POINT('Ctrl Pts',(-62.2058848408346,34.5191776503843,12.));
#90100=CARTESIAN_POINT('Ctrl Pts',(-62.1840308021171,34.5149095840729,12.));
#90101=CARTESIAN_POINT('Ctrl Pts',(-62.1622268744337,34.5106283314594,12.));
#90102=CARTESIAN_POINT('Ctrl Pts',(-62.1404731855687,34.5063339904533,12.));
#90103=CARTESIAN_POINT('Ctrl Pts',(-62.1187698638707,34.5020266595293,12.));
#90104=CARTESIAN_POINT('Ctrl Pts',(-62.0971170382567,34.4977064377282,12.));
#90105=CARTESIAN_POINT('Ctrl Pts',(-62.0755148382135,34.4933734246592,12.));
#90106=CARTESIAN_POINT('Ctrl Pts',(-62.0539633937939,34.4890277205039,12.));
#90107=CARTESIAN_POINT('Ctrl Pts',(-62.0324628356141,34.4846694260199,12.));
#90108=CARTESIAN_POINT('Ctrl Pts',(-62.0110132948794,34.4802986425528,12.));
#90109=CARTESIAN_POINT('Ctrl Pts',(-61.9896149034001,34.4759154720473,12.));
#90110=CARTESIAN_POINT('Ctrl Pts',(-61.9682677936054,34.4715200170592,12.));
#90111=CARTESIAN_POINT('Ctrl Pts',(-61.9469720985531,34.4671123807717,12.));
#90112=CARTESIAN_POINT('Ctrl Pts',(-61.9257279519308,34.4626926669974,12.));
#90113=CARTESIAN_POINT('Ctrl Pts',(-61.9045354880445,34.4582609801637,12.));
#90114=CARTESIAN_POINT('Ctrl Pts',(-61.8833948418025,34.4538174253012,12.));
#90115=CARTESIAN_POINT('Ctrl Pts',(-61.8623061487018,34.449362108036,12.));
#90116=CARTESIAN_POINT('Ctrl Pts',(-61.8412695447926,34.4448951345739,12.));
#90117=CARTESIAN_POINT('Ctrl Pts',(-61.8202851667222,34.4404166117299,12.));
#90118=CARTESIAN_POINT('Ctrl Pts',(-61.7993531518037,34.4359266469749,12.));
#90119=CARTESIAN_POINT('Ctrl Pts',(-61.7784736380727,34.4314253484791,12.));
#90120=CARTESIAN_POINT('Ctrl Pts',(-61.7576467643432,34.4269128251576,12.));
#90121=CARTESIAN_POINT('Ctrl Pts',(-61.7368726702596,34.4223891867179,12.));
#90122=CARTESIAN_POINT('Ctrl Pts',(-61.7161514961915,34.4178545435766,12.));
#90123=CARTESIAN_POINT('Ctrl Pts',(-61.695483383117,34.4133090067703,12.));
#90124=CARTESIAN_POINT('Ctrl Pts',(-61.6748684725205,34.4087526878812,12.));
#90125=CARTESIAN_POINT('Ctrl Pts',(-61.6543069062416,34.4041856989316,12.));
#90126=CARTESIAN_POINT('Ctrl Pts',(-61.6337988264556,34.3996081523753,12.));
#90127=CARTESIAN_POINT('Ctrl Pts',(-61.6133443760142,34.3950201613432,12.));
#90128=CARTESIAN_POINT('Ctrl Pts',(-61.5929436987409,34.3904218398636,12.));
#90129=CARTESIAN_POINT('Ctrl Pts',(-61.5725969396829,34.3858133030518,12.));
#90130=CARTESIAN_POINT('Ctrl Pts',(-61.5523042455158,34.3811946674196,12.));
#90131=CARTESIAN_POINT('Ctrl Pts',(-61.5320657642639,34.376566050668,12.));
#90132=CARTESIAN_POINT('Ctrl Pts',(-61.5118816445437,34.3719275711195,12.));
#90133=CARTESIAN_POINT('Ctrl Pts',(-61.4917520349279,34.3672793472465,12.));
#90134=CARTESIAN_POINT('Ctrl Pts',(-61.4716770832897,34.3626214971888,12.));
#90135=CARTESIAN_POINT('Ctrl Pts',(-61.4516569360454,34.3579541381996,12.));
#90136=CARTESIAN_POINT('Ctrl Pts',(-61.4316917395918,34.3532773877089,12.));
#90137=CARTESIAN_POINT('Ctrl Pts',(-61.4117816420229,34.3485913645979,12.));
#90138=CARTESIAN_POINT('Ctrl Pts',(-61.3919267945302,34.3438961902405,12.));
#90139=CARTESIAN_POINT('Ctrl Pts',(-61.3721273534257,34.339191990014,12.));
#90140=CARTESIAN_POINT('Ctrl Pts',(-61.3523834803188,34.3344788934363,12.));
#90141=CARTESIAN_POINT('Ctrl Pts',(-61.3326953378851,34.3297570310146,12.));
#90142=CARTESIAN_POINT('Ctrl Pts',(-61.3130630861386,34.3250265314768,12.));
#90143=CARTESIAN_POINT('Ctrl Pts',(-61.2934868791855,34.3202875193617,12.));
#90144=CARTESIAN_POINT('Ctrl Pts',(-61.2739668600365,34.3155401111747,12.));
#90145=CARTESIAN_POINT('Ctrl Pts',(-61.2545031656133,34.3107844191043,12.));
#90146=CARTESIAN_POINT('Ctrl Pts',(-61.235095936694,34.3060205584064,12.));
#90147=CARTESIAN_POINT('Ctrl Pts',(-61.2157453259107,34.3012486533474,12.));
#90148=CARTESIAN_POINT('Ctrl Pts',(-61.1964515073891,34.2964688443663,12.));
#90149=CARTESIAN_POINT('Ctrl Pts',(-61.1772146833205,34.2916812929751,12.));
#90150=CARTESIAN_POINT('Ctrl Pts',(-61.1580350635533,34.2868861666384,12.));
#90151=CARTESIAN_POINT('Ctrl Pts',(-61.1389128461886,34.2820836244469,12.));
#90152=CARTESIAN_POINT('Ctrl Pts',(-61.1198481997764,34.277273803877,12.));
#90153=CARTESIAN_POINT('Ctrl Pts',(-61.1008412399997,34.2724568037227,12.));
#90154=CARTESIAN_POINT('Ctrl Pts',(-61.0818920286293,34.2676326825626,12.));
#90155=CARTESIAN_POINT('Ctrl Pts',(-61.0667788793266,34.2637677131934,12.));
#90156=CARTESIAN_POINT('Ctrl Pts',(-61.0554700176998,34.2608658001631,12.));
#90157=CARTESIAN_POINT('Ctrl Pts',(-61.0479423318725,34.2589297755433,12.));
#90158=CARTESIAN_POINT('Ctrl Pts',(-61.0441813777723,34.2579614092497,12.));
#90159=CARTESIAN_POINT('Ctrl Pts',(-66.1657795405966,33.5903722665284,0.));
#90160=CARTESIAN_POINT('Ctrl Pts',(-66.1657795405966,33.5903722665284,4.));
#90161=CARTESIAN_POINT('Ctrl Pts',(-66.1657795405966,33.5903722665284,8.));
#90162=CARTESIAN_POINT('Ctrl Pts',(-66.1657795405966,33.5903722665284,12.));
#90163=CARTESIAN_POINT('Ctrl Pts',(-66.2346881970584,33.6759628819924,0.));
#90164=CARTESIAN_POINT('Ctrl Pts',(-66.2346881970584,33.6759628819924,4.));
#90165=CARTESIAN_POINT('Ctrl Pts',(-66.2346881970584,33.6759628819924,8.00000000000001));
#90166=CARTESIAN_POINT('Ctrl Pts',(-66.2346881970584,33.6759628819924,12.));
#90167=CARTESIAN_POINT('Ctrl Pts',(-66.3036153738446,33.8665453669337,0.));
#90168=CARTESIAN_POINT('Ctrl Pts',(-66.3036153738446,33.8665453669337,4.));
#90169=CARTESIAN_POINT('Ctrl Pts',(-66.3036153738446,33.8665453669337,7.99999999999999));
#90170=CARTESIAN_POINT('Ctrl Pts',(-66.3036153738446,33.8665453669337,12.));
#90171=CARTESIAN_POINT('Ctrl Pts',(-66.2585076236404,34.0597557125862,0.));
#90172=CARTESIAN_POINT('Ctrl Pts',(-66.2585076236404,34.0597557125862,4.));
#90173=CARTESIAN_POINT('Ctrl Pts',(-66.2585076236404,34.0597557125862,8.00000000000001));
#90174=CARTESIAN_POINT('Ctrl Pts',(-66.2585076236404,34.0597557125862,12.));
#90175=CARTESIAN_POINT('Ctrl Pts',(-66.2207497120656,34.1330090612016,0.));
#90176=CARTESIAN_POINT('Ctrl Pts',(-66.2207497120656,34.1330090612016,4.));
#90177=CARTESIAN_POINT('Ctrl Pts',(-66.2207497120656,34.1330090612016,8.));
#90178=CARTESIAN_POINT('Ctrl Pts',(-66.2207497120656,34.1330090612016,12.));
#90179=CARTESIAN_POINT('',(-66.1657795405966,33.5903722665284,0.));
#90180=CARTESIAN_POINT('',(-66.220749712065,34.1330090612013,0.));
#90181=CARTESIAN_POINT('Ctrl Pts',(-66.1657795405966,33.5903722665284,7.5239139515392E-35));
#90182=CARTESIAN_POINT('Ctrl Pts',(-66.2346881970584,33.6759628819924,7.52391395153919E-35));
#90183=CARTESIAN_POINT('Ctrl Pts',(-66.274075155222,33.7848671591017,7.5239139515392E-35));
#90184=CARTESIAN_POINT('Ctrl Pts',(-66.276226218858,33.8946295131779,7.5239139515392E-35));
#90185=CARTESIAN_POINT('Ctrl Pts',(-66.2778395165851,33.9769512787351,7.5239139515392E-35));
#90186=CARTESIAN_POINT('Ctrl Pts',(-66.2585076236404,34.0597557125862,7.52391395153919E-35));
#90187=CARTESIAN_POINT('Ctrl Pts',(-66.2207497120656,34.1330090612016,7.52391395153919E-35));
#90188=CARTESIAN_POINT('',(-66.220749712065,34.1330090612013,12.));
#90189=CARTESIAN_POINT('Ctrl Pts',(-66.2207497120656,34.1330090612016,0.));
#90190=CARTESIAN_POINT('Ctrl Pts',(-66.2207497120656,34.1330090612016,4.));
#90191=CARTESIAN_POINT('Ctrl Pts',(-66.2207497120656,34.1330090612016,8.));
#90192=CARTESIAN_POINT('Ctrl Pts',(-66.2207497120656,34.1330090612016,12.));
#90193=CARTESIAN_POINT('',(-66.1657795405966,33.5903722665284,12.));
#90194=CARTESIAN_POINT('Ctrl Pts',(-66.2207497120656,34.1330090612016,12.));
#90195=CARTESIAN_POINT('Ctrl Pts',(-66.2585076236404,34.0597557125862,12.));
#90196=CARTESIAN_POINT('Ctrl Pts',(-66.2778395165851,33.9769512787351,12.));
#90197=CARTESIAN_POINT('Ctrl Pts',(-66.276226218858,33.8946295131779,12.));
#90198=CARTESIAN_POINT('Ctrl Pts',(-66.274075155222,33.7848671591017,12.));
#90199=CARTESIAN_POINT('Ctrl Pts',(-66.2346881970584,33.6759628819924,12.));
#90200=CARTESIAN_POINT('Ctrl Pts',(-66.1657795405966,33.5903722665284,12.));
#90201=CARTESIAN_POINT('Ctrl Pts',(-66.1657795405966,33.5903722665284,12.));
#90202=CARTESIAN_POINT('Ctrl Pts',(-66.1657795405966,33.5903722665284,8.));
#90203=CARTESIAN_POINT('Ctrl Pts',(-66.1657795405966,33.5903722665284,4.));
#90204=CARTESIAN_POINT('Ctrl Pts',(-66.1657795405966,33.5903722665284,0.));
#90205=CARTESIAN_POINT('Origin',(-3.3253631270614E-10,1.72995545227681E-10,
0.));
#90206=CARTESIAN_POINT('Origin',(-3.3253631270614E-10,1.72995545227681E-10,
12.));
#90207=CARTESIAN_POINT('Origin',(-3.3253631270614E-10,1.72995545227681E-10,
0.));
#90208=CARTESIAN_POINT('Ctrl Pts',(-62.6704278106387,40.2823469776964,-5.55111512312578E-16));
#90209=CARTESIAN_POINT('Ctrl Pts',(-62.6704278106387,40.2823469776964,4.));
#90210=CARTESIAN_POINT('Ctrl Pts',(-62.6704278106387,40.2823469776964,8.));
#90211=CARTESIAN_POINT('Ctrl Pts',(-62.6704278106387,40.2823469776964,12.));
#90212=CARTESIAN_POINT('Ctrl Pts',(-62.6110140705998,40.3747816242707,-5.55111512312578E-16));
#90213=CARTESIAN_POINT('Ctrl Pts',(-62.6110140705998,40.3747816242707,3.99999999999999));
#90214=CARTESIAN_POINT('Ctrl Pts',(-62.6110140705998,40.3747816242707,8.00000000000001));
#90215=CARTESIAN_POINT('Ctrl Pts',(-62.6110140705998,40.3747816242707,12.));
#90216=CARTESIAN_POINT('Ctrl Pts',(-62.4519997852064,40.5004281293554,-6.28194844081531E-16));
#90217=CARTESIAN_POINT('Ctrl Pts',(-62.4519997852064,40.5004281293554,4.00000000000001));
#90218=CARTESIAN_POINT('Ctrl Pts',(-62.4519997852064,40.5004281293554,7.99999999999999));
#90219=CARTESIAN_POINT('Ctrl Pts',(-62.4519997852064,40.5004281293554,12.));
#90220=CARTESIAN_POINT('Ctrl Pts',(-62.2544389573118,40.5187208145703,-8.01722692544941E-16));
#90221=CARTESIAN_POINT('Ctrl Pts',(-62.2544389573118,40.5187208145703,3.99999999999999));
#90222=CARTESIAN_POINT('Ctrl Pts',(-62.2544389573118,40.5187208145703,8.00000000000001));
#90223=CARTESIAN_POINT('Ctrl Pts',(-62.2544389573118,40.5187208145703,12.));
#90224=CARTESIAN_POINT('Ctrl Pts',(-62.1730054756455,40.5060598100836,-8.85376672782334E-16));
#90225=CARTESIAN_POINT('Ctrl Pts',(-62.1730054756455,40.5060598100836,4.));
#90226=CARTESIAN_POINT('Ctrl Pts',(-62.1730054756455,40.5060598100836,8.));
#90227=CARTESIAN_POINT('Ctrl Pts',(-62.1730054756455,40.5060598100836,12.));
#90228=CARTESIAN_POINT('',(-62.6704278106387,40.2823469776964,0.));
#90229=CARTESIAN_POINT('',(-62.1730054756455,40.5060598100838,0.));
#90230=CARTESIAN_POINT('Ctrl Pts',(-62.6704278106387,40.2823469776964,-5.2766896056214E-16));
#90231=CARTESIAN_POINT('Ctrl Pts',(-62.6110140705998,40.3747816242707,-5.2766896056214E-16));
#90232=CARTESIAN_POINT('Ctrl Pts',(-62.5201487646607,40.4465796271763,-5.69430864430113E-16));
#90233=CARTESIAN_POINT('Ctrl Pts',(-62.4166968325988,40.4833233215529,-6.4399097783097E-16));
#90234=CARTESIAN_POINT('Ctrl Pts',(-62.3391078835523,40.5108810923353,-6.99911062881613E-16));
#90235=CARTESIAN_POINT('Ctrl Pts',(-62.2544389573118,40.5187208145703,-7.74280140794503E-16));
#90236=CARTESIAN_POINT('Ctrl Pts',(-62.1730054756455,40.5060598100836,-8.57934121031896E-16));
#90237=CARTESIAN_POINT('',(-62.1730054756454,40.5060598100838,12.));
#90238=CARTESIAN_POINT('Ctrl Pts',(-62.1730054756455,40.5060598100836,-8.85376672782334E-16));
#90239=CARTESIAN_POINT('Ctrl Pts',(-62.1730054756455,40.5060598100836,4.));
#90240=CARTESIAN_POINT('Ctrl Pts',(-62.1730054756455,40.5060598100836,8.));
#90241=CARTESIAN_POINT('Ctrl Pts',(-62.1730054756455,40.5060598100836,12.));
#90242=CARTESIAN_POINT('',(-62.6704278106387,40.2823469776964,12.));
#90243=CARTESIAN_POINT('Ctrl Pts',(-62.1730054756455,40.5060598100836,12.));
#90244=CARTESIAN_POINT('Ctrl Pts',(-62.2544389573118,40.5187208145703,12.));
#90245=CARTESIAN_POINT('Ctrl Pts',(-62.3391078835523,40.5108810923354,12.));
#90246=CARTESIAN_POINT('Ctrl Pts',(-62.4166968325988,40.4833233215529,12.));
#90247=CARTESIAN_POINT('Ctrl Pts',(-62.5201487646607,40.4465796271763,12.));
#90248=CARTESIAN_POINT('Ctrl Pts',(-62.6110140705998,40.3747816242707,12.));
#90249=CARTESIAN_POINT('Ctrl Pts',(-62.6704278106387,40.2823469776964,12.));
#90250=CARTESIAN_POINT('Ctrl Pts',(-62.6704278106387,40.2823469776964,12.));
#90251=CARTESIAN_POINT('Ctrl Pts',(-62.6704278106387,40.2823469776964,8.));
#90252=CARTESIAN_POINT('Ctrl Pts',(-62.6704278106387,40.2823469776964,4.));
#90253=CARTESIAN_POINT('Ctrl Pts',(-62.6704278106387,40.2823469776964,-5.55111512312578E-16));
#90254=CARTESIAN_POINT('Ctrl Pts',(-57.8261117662438,39.4479504917287,0.));
#90255=CARTESIAN_POINT('Ctrl Pts',(-57.8261117662438,39.4479504917287,12.));
#90256=CARTESIAN_POINT('Ctrl Pts',(-57.8297740100947,39.4492429618443,0.));
#90257=CARTESIAN_POINT('Ctrl Pts',(-57.8297740100947,39.4492429618443,12.));
#90258=CARTESIAN_POINT('Ctrl Pts',(-57.837104315141,39.4518277003553,0.));
#90259=CARTESIAN_POINT('Ctrl Pts',(-57.837104315141,39.4518277003553,12.));
#90260=CARTESIAN_POINT('Ctrl Pts',(-57.8481172247496,39.4557042029652,0.));
#90261=CARTESIAN_POINT('Ctrl Pts',(-57.8481172247496,39.4557042029652,12.));
#90262=CARTESIAN_POINT('Ctrl Pts',(-57.8628360096803,39.4608716627117,0.));
#90263=CARTESIAN_POINT('Ctrl Pts',(-57.8628360096803,39.4608716627117,12.));
#90264=CARTESIAN_POINT('Ctrl Pts',(-57.8812926637177,39.4673289592259,0.));
#90265=CARTESIAN_POINT('Ctrl Pts',(-57.8812926637177,39.4673289592259,12.));
#90266=CARTESIAN_POINT('Ctrl Pts',(-57.8998074670478,39.473784194937,0.));
#90267=CARTESIAN_POINT('Ctrl Pts',(-57.8998074670478,39.473784194937,12.));
#90268=CARTESIAN_POINT('Ctrl Pts',(-57.9183803632403,39.4802373061058,0.));
#90269=CARTESIAN_POINT('Ctrl Pts',(-57.9183803632403,39.4802373061058,12.));
#90270=CARTESIAN_POINT('Ctrl Pts',(-57.937011245663,39.4866881842317,0.));
#90271=CARTESIAN_POINT('Ctrl Pts',(-57.937011245663,39.4866881842317,12.));
#90272=CARTESIAN_POINT('Ctrl Pts',(-57.9556999583892,39.4931366776714,0.));
#90273=CARTESIAN_POINT('Ctrl Pts',(-57.9556999583892,39.4931366776714,12.));
#90274=CARTESIAN_POINT('Ctrl Pts',(-57.974446317937,39.499582610674,0.));
#90275=CARTESIAN_POINT('Ctrl Pts',(-57.974446317937,39.499582610674,12.));
#90276=CARTESIAN_POINT('Ctrl Pts',(-57.9932501298522,39.5060257981225,0.));
#90277=CARTESIAN_POINT('Ctrl Pts',(-57.9932501298522,39.5060257981225,12.));
#90278=CARTESIAN_POINT('Ctrl Pts',(-58.0121112067895,39.5124660614976,0.));
#90279=CARTESIAN_POINT('Ctrl Pts',(-58.0121112067895,39.5124660614976,12.));
#90280=CARTESIAN_POINT('Ctrl Pts',(-58.0310293875262,39.5189032457184,0.));
#90281=CARTESIAN_POINT('Ctrl Pts',(-58.0310293875262,39.5189032457184,12.));
#90282=CARTESIAN_POINT('Ctrl Pts',(-58.0500045308412,39.5253372136887,0.));
#90283=CARTESIAN_POINT('Ctrl Pts',(-58.0500045308412,39.5253372136887,12.));
#90284=CARTESIAN_POINT('Ctrl Pts',(-58.0690365065374,39.5317678383217,0.));
#90285=CARTESIAN_POINT('Ctrl Pts',(-58.0690365065374,39.5317678383217,12.));
#90286=CARTESIAN_POINT('Ctrl Pts',(-58.0881251879921,39.5381949959221,0.));
#90287=CARTESIAN_POINT('Ctrl Pts',(-58.0881251879921,39.5381949959221,12.));
#90288=CARTESIAN_POINT('Ctrl Pts',(-58.1072704428928,39.5446185579638,0.));
#90289=CARTESIAN_POINT('Ctrl Pts',(-58.1072704428928,39.5446185579638,12.));
#90290=CARTESIAN_POINT('Ctrl Pts',(-58.126472128574,39.5510383869505,0.));
#90291=CARTESIAN_POINT('Ctrl Pts',(-58.126472128574,39.5510383869505,12.));
#90292=CARTESIAN_POINT('Ctrl Pts',(-58.1457300968499,39.5574543406982,0.));
#90293=CARTESIAN_POINT('Ctrl Pts',(-58.1457300968499,39.5574543406982,12.));
#90294=CARTESIAN_POINT('Ctrl Pts',(-58.1650441970387,39.563866275018,0.));
#90295=CARTESIAN_POINT('Ctrl Pts',(-58.1650441970387,39.563866275018,12.));
#90296=CARTESIAN_POINT('Ctrl Pts',(-58.1844142794338,39.5702740467999,0.));
#90297=CARTESIAN_POINT('Ctrl Pts',(-58.1844142794338,39.5702740467999,12.));
#90298=CARTESIAN_POINT('Ctrl Pts',(-58.2038401992457,39.57667751752,0.));
#90299=CARTESIAN_POINT('Ctrl Pts',(-58.2038401992457,39.57667751752,12.));
#90300=CARTESIAN_POINT('Ctrl Pts',(-58.2233218164365,39.5830765530891,0.));
#90301=CARTESIAN_POINT('Ctrl Pts',(-58.2233218164365,39.5830765530891,12.));
#90302=CARTESIAN_POINT('Ctrl Pts',(-58.2428589938369,39.5894710221713,0.));
#90303=CARTESIAN_POINT('Ctrl Pts',(-58.2428589938369,39.5894710221713,12.));
#90304=CARTESIAN_POINT('Ctrl Pts',(-58.2624515958419,39.5958607950239,0.));
#90305=CARTESIAN_POINT('Ctrl Pts',(-58.2624515958419,39.5958607950239,12.));
#90306=CARTESIAN_POINT('Ctrl Pts',(-58.2820994868118,39.602245742079,0.));
#90307=CARTESIAN_POINT('Ctrl Pts',(-58.2820994868118,39.602245742079,12.));
#90308=CARTESIAN_POINT('Ctrl Pts',(-58.3018025297323,39.6086257327583,0.));
#90309=CARTESIAN_POINT('Ctrl Pts',(-58.3018025297323,39.6086257327583,12.));
#90310=CARTESIAN_POINT('Ctrl Pts',(-58.3215605869221,39.6150006360914,0.));
#90311=CARTESIAN_POINT('Ctrl Pts',(-58.3215605869221,39.6150006360914,12.));
#90312=CARTESIAN_POINT('Ctrl Pts',(-58.3413735206423,39.6213703212531,0.));
#90313=CARTESIAN_POINT('Ctrl Pts',(-58.3413735206423,39.6213703212531,12.));
#90314=CARTESIAN_POINT('Ctrl Pts',(-58.3612411936905,39.6277346580892,0.));
#90315=CARTESIAN_POINT('Ctrl Pts',(-58.3612411936905,39.6277346580892,12.));
#90316=CARTESIAN_POINT('Ctrl Pts',(-58.3811634701037,39.6340935177476,0.));
#90317=CARTESIAN_POINT('Ctrl Pts',(-58.3811634701037,39.6340935177476,12.));
#90318=CARTESIAN_POINT('Ctrl Pts',(-58.4011402154196,39.6404467729094,0.));
#90319=CARTESIAN_POINT('Ctrl Pts',(-58.4011402154196,39.6404467729094,12.));
#90320=CARTESIAN_POINT('Ctrl Pts',(-58.4211712963004,39.6467942974451,0.));
#90321=CARTESIAN_POINT('Ctrl Pts',(-58.4211712963004,39.6467942974451,12.));
#90322=CARTESIAN_POINT('Ctrl Pts',(-58.4412565802979,39.653135966204,0.));
#90323=CARTESIAN_POINT('Ctrl Pts',(-58.4412565802979,39.653135966204,12.));
#90324=CARTESIAN_POINT('Ctrl Pts',(-58.4613959355788,39.6594716547689,0.));
#90325=CARTESIAN_POINT('Ctrl Pts',(-58.4613959355788,39.6594716547689,12.));
#90326=CARTESIAN_POINT('Ctrl Pts',(-58.4815892306066,39.6658012391815,0.));
#90327=CARTESIAN_POINT('Ctrl Pts',(-58.4815892306066,39.6658012391815,12.));
#90328=CARTESIAN_POINT('Ctrl Pts',(-58.5018363341604,39.6721245959531,0.));
#90329=CARTESIAN_POINT('Ctrl Pts',(-58.5018363341604,39.6721245959531,12.));
#90330=CARTESIAN_POINT('Ctrl Pts',(-58.5221371154761,39.6784416021826,0.));
#90331=CARTESIAN_POINT('Ctrl Pts',(-58.5221371154761,39.6784416021826,12.));
#90332=CARTESIAN_POINT('Ctrl Pts',(-58.5424914443415,39.6847521356395,0.));
#90333=CARTESIAN_POINT('Ctrl Pts',(-58.5424914443415,39.6847521356395,12.));
#90334=CARTESIAN_POINT('Ctrl Pts',(-58.5628991912052,39.6910560748629,0.));
#90335=CARTESIAN_POINT('Ctrl Pts',(-58.5628991912052,39.6910560748629,12.));
#90336=CARTESIAN_POINT('Ctrl Pts',(-58.5833602272744,39.6973532992539,0.));
#90337=CARTESIAN_POINT('Ctrl Pts',(-58.5833602272744,39.6973532992539,12.));
#90338=CARTESIAN_POINT('Ctrl Pts',(-58.6038744244659,39.7036436890233,0.));
#90339=CARTESIAN_POINT('Ctrl Pts',(-58.6038744244659,39.7036436890233,12.));
#90340=CARTESIAN_POINT('Ctrl Pts',(-58.6244416553562,39.7099271251413,0.));
#90341=CARTESIAN_POINT('Ctrl Pts',(-58.6244416553562,39.7099271251413,12.));
#90342=CARTESIAN_POINT('Ctrl Pts',(-58.6450617931274,39.7162034892899,0.));
#90343=CARTESIAN_POINT('Ctrl Pts',(-58.6450617931274,39.7162034892899,12.));
#90344=CARTESIAN_POINT('Ctrl Pts',(-58.6657347115034,39.72247266381,0.));
#90345=CARTESIAN_POINT('Ctrl Pts',(-58.6657347115034,39.72247266381,12.));
#90346=CARTESIAN_POINT('Ctrl Pts',(-58.6864602847088,39.7287345316681,0.));
#90347=CARTESIAN_POINT('Ctrl Pts',(-58.6864602847088,39.7287345316681,12.));
#90348=CARTESIAN_POINT('Ctrl Pts',(-58.7072383875027,39.734988976475,0.));
#90349=CARTESIAN_POINT('Ctrl Pts',(-58.7072383875027,39.734988976475,12.));
#90350=CARTESIAN_POINT('Ctrl Pts',(-58.7280688951916,39.7412358824953,0.));
#90351=CARTESIAN_POINT('Ctrl Pts',(-58.7280688951916,39.7412358824953,12.));
#90352=CARTESIAN_POINT('Ctrl Pts',(-58.7489516836445,39.7474751346598,0.));
#90353=CARTESIAN_POINT('Ctrl Pts',(-58.7489516836445,39.7474751346598,12.));
#90354=CARTESIAN_POINT('Ctrl Pts',(-58.7698866293029,39.7537066185813,0.));
#90355=CARTESIAN_POINT('Ctrl Pts',(-58.7698866293029,39.7537066185813,12.));
#90356=CARTESIAN_POINT('Ctrl Pts',(-58.7908736091798,39.7599302205521,0.));
#90357=CARTESIAN_POINT('Ctrl Pts',(-58.7908736091798,39.7599302205521,12.));
#90358=CARTESIAN_POINT('Ctrl Pts',(-58.8119125008517,39.7661458275274,0.));
#90359=CARTESIAN_POINT('Ctrl Pts',(-58.8119125008517,39.7661458275274,12.));
#90360=CARTESIAN_POINT('Ctrl Pts',(-58.8330031824453,39.772353327112,0.));
#90361=CARTESIAN_POINT('Ctrl Pts',(-58.8330031824453,39.772353327112,12.));
#90362=CARTESIAN_POINT('Ctrl Pts',(-58.8541455326231,39.7785526075478,0.));
#90363=CARTESIAN_POINT('Ctrl Pts',(-58.8541455326231,39.7785526075478,12.));
#90364=CARTESIAN_POINT('Ctrl Pts',(-58.8753394305585,39.7847435576996,0.));
#90365=CARTESIAN_POINT('Ctrl Pts',(-58.8753394305585,39.7847435576996,12.));
#90366=CARTESIAN_POINT('Ctrl Pts',(-58.8965847559391,39.7909260670517,0.));
#90367=CARTESIAN_POINT('Ctrl Pts',(-58.8965847559391,39.7909260670517,12.));
#90368=CARTESIAN_POINT('Ctrl Pts',(-58.9178813889704,39.7971000257044,0.));
#90369=CARTESIAN_POINT('Ctrl Pts',(-58.9178813889704,39.7971000257044,12.));
#90370=CARTESIAN_POINT('Ctrl Pts',(-58.9392292103747,39.8032653243712,0.));
#90371=CARTESIAN_POINT('Ctrl Pts',(-58.9392292103747,39.8032653243712,12.));
#90372=CARTESIAN_POINT('Ctrl Pts',(-58.9606281013875,39.8094218543782,0.));
#90373=CARTESIAN_POINT('Ctrl Pts',(-58.9606281013875,39.8094218543782,12.));
#90374=CARTESIAN_POINT('Ctrl Pts',(-58.9820779437484,39.8155695076626,0.));
#90375=CARTESIAN_POINT('Ctrl Pts',(-58.9820779437484,39.8155695076626,12.));
#90376=CARTESIAN_POINT('Ctrl Pts',(-59.0035786197024,39.821708176766,0.));
#90377=CARTESIAN_POINT('Ctrl Pts',(-59.0035786197024,39.821708176766,12.));
#90378=CARTESIAN_POINT('Ctrl Pts',(-59.0251300119973,39.8278377548262,0.));
#90379=CARTESIAN_POINT('Ctrl Pts',(-59.0251300119973,39.8278377548262,12.));
#90380=CARTESIAN_POINT('Ctrl Pts',(-59.0467320038784,39.8339581355716,0.));
#90381=CARTESIAN_POINT('Ctrl Pts',(-59.0467320038784,39.8339581355716,12.));
#90382=CARTESIAN_POINT('Ctrl Pts',(-59.0683844790764,39.8400692133139,0.));
#90383=CARTESIAN_POINT('Ctrl Pts',(-59.0683844790764,39.8400692133139,12.));
#90384=CARTESIAN_POINT('Ctrl Pts',(-59.090087321798,39.8461708829456,0.));
#90385=CARTESIAN_POINT('Ctrl Pts',(-59.090087321798,39.8461708829456,12.));
#90386=CARTESIAN_POINT('Ctrl Pts',(-59.1118404167292,39.8522630399328,0.));
#90387=CARTESIAN_POINT('Ctrl Pts',(-59.1118404167292,39.8522630399328,12.));
#90388=CARTESIAN_POINT('Ctrl Pts',(-59.1336436490342,39.8583455803105,0.));
#90389=CARTESIAN_POINT('Ctrl Pts',(-59.1336436490342,39.8583455803105,12.));
#90390=CARTESIAN_POINT('Ctrl Pts',(-59.1554969043522,39.8644184006787,0.));
#90391=CARTESIAN_POINT('Ctrl Pts',(-59.1554969043522,39.8644184006787,12.));
#90392=CARTESIAN_POINT('Ctrl Pts',(-59.1774000687879,39.8704813981988,0.));
#90393=CARTESIAN_POINT('Ctrl Pts',(-59.1774000687879,39.8704813981988,12.));
#90394=CARTESIAN_POINT('Ctrl Pts',(-59.1993530289028,39.876534470591,0.));
#90395=CARTESIAN_POINT('Ctrl Pts',(-59.1993530289028,39.876534470591,12.));
#90396=CARTESIAN_POINT('Ctrl Pts',(-59.2213556717209,39.8825775161267,0.));
#90397=CARTESIAN_POINT('Ctrl Pts',(-59.2213556717209,39.8825775161267,12.));
#90398=CARTESIAN_POINT('Ctrl Pts',(-59.2434078847247,39.8886104336242,0.));
#90399=CARTESIAN_POINT('Ctrl Pts',(-59.2434078847247,39.8886104336242,12.));
#90400=CARTESIAN_POINT('Ctrl Pts',(-59.2655095558521,39.8946331224438,0.));
#90401=CARTESIAN_POINT('Ctrl Pts',(-59.2655095558521,39.8946331224438,12.));
#90402=CARTESIAN_POINT('Ctrl Pts',(-59.2876605734846,39.9006454824845,0.));
#90403=CARTESIAN_POINT('Ctrl Pts',(-59.2876605734846,39.9006454824845,12.));
#90404=CARTESIAN_POINT('Ctrl Pts',(-59.3098608264419,39.9066474141803,0.));
#90405=CARTESIAN_POINT('Ctrl Pts',(-59.3098608264419,39.9066474141803,12.));
#90406=CARTESIAN_POINT('Ctrl Pts',(-59.3321102039852,39.9126388184936,0.));
#90407=CARTESIAN_POINT('Ctrl Pts',(-59.3321102039852,39.9126388184936,12.));
#90408=CARTESIAN_POINT('Ctrl Pts',(-59.3544085958151,39.9186195969104,0.));
#90409=CARTESIAN_POINT('Ctrl Pts',(-59.3544085958151,39.9186195969104,12.));
#90410=CARTESIAN_POINT('Ctrl Pts',(-59.3767558920675,39.9245896514367,0.));
#90411=CARTESIAN_POINT('Ctrl Pts',(-59.3767558920675,39.9245896514367,12.));
#90412=CARTESIAN_POINT('Ctrl Pts',(-59.3991519833016,39.9305488845958,0.));
#90413=CARTESIAN_POINT('Ctrl Pts',(-59.3991519833016,39.9305488845958,12.));
#90414=CARTESIAN_POINT('Ctrl Pts',(-59.4215967604967,39.9364971994242,0.));
#90415=CARTESIAN_POINT('Ctrl Pts',(-59.4215967604967,39.9364971994242,12.));
#90416=CARTESIAN_POINT('Ctrl Pts',(-59.4440901150582,39.9424344994672,0.));
#90417=CARTESIAN_POINT('Ctrl Pts',(-59.4440901150582,39.9424344994672,12.));
#90418=CARTESIAN_POINT('Ctrl Pts',(-59.4666319388133,39.9483606887737,0.));
#90419=CARTESIAN_POINT('Ctrl Pts',(-59.4666319388133,39.9483606887737,12.));
#90420=CARTESIAN_POINT('Ctrl Pts',(-59.4892221240068,39.9542756718922,0.));
#90421=CARTESIAN_POINT('Ctrl Pts',(-59.4892221240068,39.9542756718922,12.));
#90422=CARTESIAN_POINT('Ctrl Pts',(-59.5118605632891,39.9601793538682,0.));
#90423=CARTESIAN_POINT('Ctrl Pts',(-59.5118605632891,39.9601793538682,12.));
#90424=CARTESIAN_POINT('Ctrl Pts',(-59.5345471497129,39.9660716402403,0.));
#90425=CARTESIAN_POINT('Ctrl Pts',(-59.5345471497129,39.9660716402403,12.));
#90426=CARTESIAN_POINT('Ctrl Pts',(-59.5572817767388,39.9719524370345,0.));
#90427=CARTESIAN_POINT('Ctrl Pts',(-59.5572817767388,39.9719524370345,12.));
#90428=CARTESIAN_POINT('Ctrl Pts',(-59.5800643382314,39.9778216507605,0.));
#90429=CARTESIAN_POINT('Ctrl Pts',(-59.5800643382314,39.9778216507605,12.));
#90430=CARTESIAN_POINT('Ctrl Pts',(-59.6028947284562,39.9836791884079,0.));
#90431=CARTESIAN_POINT('Ctrl Pts',(-59.6028947284562,39.9836791884079,12.));
#90432=CARTESIAN_POINT('Ctrl Pts',(-59.6257728420669,39.9895249574448,0.));
#90433=CARTESIAN_POINT('Ctrl Pts',(-59.6257728420669,39.9895249574448,12.));
#90434=CARTESIAN_POINT('Ctrl Pts',(-59.6486985741041,39.9953588658132,0.));
#90435=CARTESIAN_POINT('Ctrl Pts',(-59.6486985741041,39.9953588658132,12.));
#90436=CARTESIAN_POINT('Ctrl Pts',(-59.6716718200005,40.0011808219241,0.));
#90437=CARTESIAN_POINT('Ctrl Pts',(-59.6716718200005,40.0011808219241,12.));
#90438=CARTESIAN_POINT('Ctrl Pts',(-59.6946924755773,40.0069907346537,0.));
#90439=CARTESIAN_POINT('Ctrl Pts',(-59.6946924755773,40.0069907346537,12.));
#90440=CARTESIAN_POINT('Ctrl Pts',(-59.7177604370403,40.0127885133403,0.));
#90441=CARTESIAN_POINT('Ctrl Pts',(-59.7177604370403,40.0127885133403,12.));
#90442=CARTESIAN_POINT('Ctrl Pts',(-59.7408756009679,40.0185740677821,0.));
#90443=CARTESIAN_POINT('Ctrl Pts',(-59.7408756009679,40.0185740677821,12.));
#90444=CARTESIAN_POINT('Ctrl Pts',(-59.7640378643106,40.0243473082337,0.));
#90445=CARTESIAN_POINT('Ctrl Pts',(-59.7640378643106,40.0243473082337,12.));
#90446=CARTESIAN_POINT('Ctrl Pts',(-59.7872471243942,40.0301081454002,0.));
#90447=CARTESIAN_POINT('Ctrl Pts',(-59.7872471243942,40.0301081454002,12.));
#90448=CARTESIAN_POINT('Ctrl Pts',(-59.8105032789179,40.035856490434,0.));
#90449=CARTESIAN_POINT('Ctrl Pts',(-59.8105032789179,40.035856490434,12.));
#90450=CARTESIAN_POINT('Ctrl Pts',(-59.8338062259492,40.0415922549315,0.));
#90451=CARTESIAN_POINT('Ctrl Pts',(-59.8338062259492,40.0415922549315,12.));
#90452=CARTESIAN_POINT('Ctrl Pts',(-59.8571558639145,40.0473153509324,0.));
#90453=CARTESIAN_POINT('Ctrl Pts',(-59.8571558639145,40.0473153509324,12.));
#90454=CARTESIAN_POINT('Ctrl Pts',(-59.8805520915972,40.0530256909161,0.));
#90455=CARTESIAN_POINT('Ctrl Pts',(-59.8805520915972,40.0530256909161,12.));
#90456=CARTESIAN_POINT('Ctrl Pts',(-59.9039948081428,40.0587231877959,0.));
#90457=CARTESIAN_POINT('Ctrl Pts',(-59.9039948081428,40.0587231877959,12.));
#90458=CARTESIAN_POINT('Ctrl Pts',(-59.927483913055,40.0644077549158,0.));
#90459=CARTESIAN_POINT('Ctrl Pts',(-59.927483913055,40.0644077549158,12.));
#90460=CARTESIAN_POINT('Ctrl Pts',(-59.9510193061929,40.0700793060475,0.));
#90461=CARTESIAN_POINT('Ctrl Pts',(-59.9510193061929,40.0700793060475,12.));
#90462=CARTESIAN_POINT('Ctrl Pts',(-59.974600887759,40.0757377553893,0.));
#90463=CARTESIAN_POINT('Ctrl Pts',(-59.974600887759,40.0757377553893,12.));
#90464=CARTESIAN_POINT('Ctrl Pts',(-59.9982285582991,40.0813830175629,0.));
#90465=CARTESIAN_POINT('Ctrl Pts',(-59.9982285582991,40.0813830175629,12.));
#90466=CARTESIAN_POINT('Ctrl Pts',(-60.0219022187066,40.0870150076078,0.));
#90467=CARTESIAN_POINT('Ctrl Pts',(-60.0219022187066,40.0870150076078,12.));
#90468=CARTESIAN_POINT('Ctrl Pts',(-60.0456217702203,40.0926336409787,0.));
#90469=CARTESIAN_POINT('Ctrl Pts',(-60.0456217702203,40.0926336409787,12.));
#90470=CARTESIAN_POINT('Ctrl Pts',(-60.0693871144207,40.0982388335421,0.));
#90471=CARTESIAN_POINT('Ctrl Pts',(-60.0693871144207,40.0982388335421,12.));
#90472=CARTESIAN_POINT('Ctrl Pts',(-60.0931981532194,40.1038305015763,0.));
#90473=CARTESIAN_POINT('Ctrl Pts',(-60.0931981532194,40.1038305015763,12.));
#90474=CARTESIAN_POINT('Ctrl Pts',(-60.1170547888572,40.1094085617672,0.));
#90475=CARTESIAN_POINT('Ctrl Pts',(-60.1170547888572,40.1094085617672,12.));
#90476=CARTESIAN_POINT('Ctrl Pts',(-60.1409569239093,40.1149729312036,0.));
#90477=CARTESIAN_POINT('Ctrl Pts',(-60.1409569239093,40.1149729312036,12.));
#90478=CARTESIAN_POINT('Ctrl Pts',(-60.1649044612829,40.120523527374,0.));
#90479=CARTESIAN_POINT('Ctrl Pts',(-60.1649044612829,40.120523527374,12.));
#90480=CARTESIAN_POINT('Ctrl Pts',(-60.1888973042151,40.1260602681644,0.));
#90481=CARTESIAN_POINT('Ctrl Pts',(-60.1888973042151,40.1260602681644,12.));
#90482=CARTESIAN_POINT('Ctrl Pts',(-60.2129353562617,40.1315830718575,0.));
#90483=CARTESIAN_POINT('Ctrl Pts',(-60.2129353562617,40.1315830718575,12.));
#90484=CARTESIAN_POINT('Ctrl Pts',(-60.2370185212957,40.13709185713,0.));
#90485=CARTESIAN_POINT('Ctrl Pts',(-60.2370185212957,40.13709185713,12.));
#90486=CARTESIAN_POINT('Ctrl Pts',(-60.2611467035109,40.1425865430468,0.));
#90487=CARTESIAN_POINT('Ctrl Pts',(-60.2611467035109,40.1425865430468,12.));
#90488=CARTESIAN_POINT('Ctrl Pts',(-60.2853198074215,40.1480670490583,0.));
#90489=CARTESIAN_POINT('Ctrl Pts',(-60.2853198074215,40.1480670490583,12.));
#90490=CARTESIAN_POINT('Ctrl Pts',(-60.3095377378589,40.1535332949978,0.));
#90491=CARTESIAN_POINT('Ctrl Pts',(-60.3095377378589,40.1535332949978,12.));
#90492=CARTESIAN_POINT('Ctrl Pts',(-60.3338003999616,40.1589852010811,0.));
#90493=CARTESIAN_POINT('Ctrl Pts',(-60.3338003999616,40.1589852010811,12.));
#90494=CARTESIAN_POINT('Ctrl Pts',(-60.3581076991731,40.1644226879043,0.));
#90495=CARTESIAN_POINT('Ctrl Pts',(-60.3581076991731,40.1644226879043,12.));
#90496=CARTESIAN_POINT('Ctrl Pts',(-60.382459541246,40.1698456764387,0.));
#90497=CARTESIAN_POINT('Ctrl Pts',(-60.382459541246,40.1698456764387,12.));
#90498=CARTESIAN_POINT('Ctrl Pts',(-60.4068558322415,40.1752540880273,0.));
#90499=CARTESIAN_POINT('Ctrl Pts',(-60.4068558322415,40.1752540880273,12.));
#90500=CARTESIAN_POINT('Ctrl Pts',(-60.4312964785269,40.1806478443828,0.));
#90501=CARTESIAN_POINT('Ctrl Pts',(-60.4312964785269,40.1806478443828,12.));
#90502=CARTESIAN_POINT('Ctrl Pts',(-60.4557813867677,40.1860268675875,0.));
#90503=CARTESIAN_POINT('Ctrl Pts',(-60.4557813867677,40.1860268675875,12.));
#90504=CARTESIAN_POINT('Ctrl Pts',(-60.4803104639211,40.1913910800911,0.));
#90505=CARTESIAN_POINT('Ctrl Pts',(-60.4803104639211,40.1913910800911,12.));
#90506=CARTESIAN_POINT('Ctrl Pts',(-60.5048836172424,40.1967404047055,0.));
#90507=CARTESIAN_POINT('Ctrl Pts',(-60.5048836172424,40.1967404047055,12.));
#90508=CARTESIAN_POINT('Ctrl Pts',(-60.5295007542838,40.2020747646012,0.));
#90509=CARTESIAN_POINT('Ctrl Pts',(-60.5295007542838,40.2020747646012,12.));
#90510=CARTESIAN_POINT('Ctrl Pts',(-60.5541617828927,40.2073940833054,0.));
#90511=CARTESIAN_POINT('Ctrl Pts',(-60.5541617828927,40.2073940833054,12.));
#90512=CARTESIAN_POINT('Ctrl Pts',(-60.5788666112043,40.2126982847012,0.));
#90513=CARTESIAN_POINT('Ctrl Pts',(-60.5788666112043,40.2126982847012,12.));
#90514=CARTESIAN_POINT('Ctrl Pts',(-60.6036151476347,40.2179872930272,0.));
#90515=CARTESIAN_POINT('Ctrl Pts',(-60.6036151476347,40.2179872930272,12.));
#90516=CARTESIAN_POINT('Ctrl Pts',(-60.6284073008865,40.2232610328717,0.));
#90517=CARTESIAN_POINT('Ctrl Pts',(-60.6284073008865,40.2232610328717,12.));
#90518=CARTESIAN_POINT('Ctrl Pts',(-60.6532429799493,40.2285194291702,0.));
#90519=CARTESIAN_POINT('Ctrl Pts',(-60.6532429799493,40.2285194291702,12.));
#90520=CARTESIAN_POINT('Ctrl Pts',(-60.678122094098,40.2337624072029,0.));
#90521=CARTESIAN_POINT('Ctrl Pts',(-60.678122094098,40.2337624072029,12.));
#90522=CARTESIAN_POINT('Ctrl Pts',(-60.7030445528863,40.2389898925937,0.));
#90523=CARTESIAN_POINT('Ctrl Pts',(-60.7030445528863,40.2389898925937,12.));
#90524=CARTESIAN_POINT('Ctrl Pts',(-60.72801026614,40.2442018113116,0.));
#90525=CARTESIAN_POINT('Ctrl Pts',(-60.72801026614,40.2442018113116,12.));
#90526=CARTESIAN_POINT('Ctrl Pts',(-60.7530191439603,40.2493980896646,0.));
#90527=CARTESIAN_POINT('Ctrl Pts',(-60.7530191439603,40.2493980896646,12.));
#90528=CARTESIAN_POINT('Ctrl Pts',(-60.7780710967253,40.2545786542957,0.));
#90529=CARTESIAN_POINT('Ctrl Pts',(-60.7780710967253,40.2545786542957,12.));
#90530=CARTESIAN_POINT('Ctrl Pts',(-60.8031660350879,40.2597434321804,0.));
#90531=CARTESIAN_POINT('Ctrl Pts',(-60.8031660350879,40.2597434321804,12.));
#90532=CARTESIAN_POINT('Ctrl Pts',(-60.8283038699703,40.2648923506245,0.));
#90533=CARTESIAN_POINT('Ctrl Pts',(-60.8283038699703,40.2648923506245,12.));
#90534=CARTESIAN_POINT('Ctrl Pts',(-60.8534845125535,40.2700253372644,0.));
#90535=CARTESIAN_POINT('Ctrl Pts',(-60.8534845125535,40.2700253372644,12.));
#90536=CARTESIAN_POINT('Ctrl Pts',(-60.8787078742817,40.2751423200637,0.));
#90537=CARTESIAN_POINT('Ctrl Pts',(-60.8787078742817,40.2751423200637,12.));
#90538=CARTESIAN_POINT('Ctrl Pts',(-60.903973866867,40.2802432273105,0.));
#90539=CARTESIAN_POINT('Ctrl Pts',(-60.903973866867,40.2802432273105,12.));
#90540=CARTESIAN_POINT('Ctrl Pts',(-60.9292824022888,40.2853279876162,0.));
#90541=CARTESIAN_POINT('Ctrl Pts',(-60.9292824022888,40.2853279876162,12.));
#90542=CARTESIAN_POINT('Ctrl Pts',(-60.9546333927919,40.2903965299155,0.));
#90543=CARTESIAN_POINT('Ctrl Pts',(-60.9546333927919,40.2903965299155,12.));
#90544=CARTESIAN_POINT('Ctrl Pts',(-60.9800267508781,40.2954487834688,0.));
#90545=CARTESIAN_POINT('Ctrl Pts',(-60.9800267508781,40.2954487834688,12.));
#90546=CARTESIAN_POINT('Ctrl Pts',(-61.005462389306,40.3004846778577,0.));
#90547=CARTESIAN_POINT('Ctrl Pts',(-61.005462389306,40.3004846778577,12.));
#90548=CARTESIAN_POINT('Ctrl Pts',(-61.0309402210915,40.3055041429772,0.));
#90549=CARTESIAN_POINT('Ctrl Pts',(-61.0309402210915,40.3055041429772,12.));
#90550=CARTESIAN_POINT('Ctrl Pts',(-61.0564601595047,40.3105071090308,0.));
#90551=CARTESIAN_POINT('Ctrl Pts',(-61.0564601595047,40.3105071090308,12.));
#90552=CARTESIAN_POINT('Ctrl Pts',(-61.0820221180646,40.3154935065264,0.));
#90553=CARTESIAN_POINT('Ctrl Pts',(-61.0820221180646,40.3154935065264,12.));
#90554=CARTESIAN_POINT('Ctrl Pts',(-61.1076260105265,40.3204632662729,0.));
#90555=CARTESIAN_POINT('Ctrl Pts',(-61.1076260105265,40.3204632662729,12.));
#90556=CARTESIAN_POINT('Ctrl Pts',(-61.1332717508799,40.3254163193806,0.));
#90557=CARTESIAN_POINT('Ctrl Pts',(-61.1332717508799,40.3254163193806,12.));
#90558=CARTESIAN_POINT('Ctrl Pts',(-61.1589592533623,40.3303525972621,0.));
#90559=CARTESIAN_POINT('Ctrl Pts',(-61.1589592533623,40.3303525972621,12.));
#90560=CARTESIAN_POINT('Ctrl Pts',(-61.184688432465,40.3352720316373,0.));
#90561=CARTESIAN_POINT('Ctrl Pts',(-61.184688432465,40.3352720316373,12.));
#90562=CARTESIAN_POINT('Ctrl Pts',(-61.2104592029375,40.3401745545369,0.));
#90563=CARTESIAN_POINT('Ctrl Pts',(-61.2104592029375,40.3401745545369,12.));
#90564=CARTESIAN_POINT('Ctrl Pts',(-61.236271479789,40.3450600983104,0.));
#90565=CARTESIAN_POINT('Ctrl Pts',(-61.236271479789,40.3450600983104,12.));
#90566=CARTESIAN_POINT('Ctrl Pts',(-61.2621251782849,40.3499285956297,0.));
#90567=CARTESIAN_POINT('Ctrl Pts',(-61.2621251782849,40.3499285956297,12.));
#90568=CARTESIAN_POINT('Ctrl Pts',(-61.2880202139358,40.3547799794672,0.));
#90569=CARTESIAN_POINT('Ctrl Pts',(-61.2880202139358,40.3547799794672,12.));
#90570=CARTESIAN_POINT('Ctrl Pts',(-61.3139565024838,40.3596141830786,0.));
#90571=CARTESIAN_POINT('Ctrl Pts',(-61.3139565024838,40.3596141830786,12.));
#90572=CARTESIAN_POINT('Ctrl Pts',(-61.3399339598851,40.3644311399861,0.));
#90573=CARTESIAN_POINT('Ctrl Pts',(-61.3399339598851,40.3644311399861,12.));
#90574=CARTESIAN_POINT('Ctrl Pts',(-61.3659525022917,40.3692307839642,0.));
#90575=CARTESIAN_POINT('Ctrl Pts',(-61.3659525022917,40.3692307839642,12.));
#90576=CARTESIAN_POINT('Ctrl Pts',(-61.3920120460232,40.3740130490233,0.));
#90577=CARTESIAN_POINT('Ctrl Pts',(-61.3920120460232,40.3740130490233,12.));
#90578=CARTESIAN_POINT('Ctrl Pts',(-61.418112507605,40.3787778694373,0.));
#90579=CARTESIAN_POINT('Ctrl Pts',(-61.418112507605,40.3787778694373,12.));
#90580=CARTESIAN_POINT('Ctrl Pts',(-61.4442538038053,40.3835251797725,0.));
#90581=CARTESIAN_POINT('Ctrl Pts',(-61.4442538038053,40.3835251797725,12.));
#90582=CARTESIAN_POINT('Ctrl Pts',(-61.4704358516711,40.3882549149229,0.));
#90583=CARTESIAN_POINT('Ctrl Pts',(-61.4704358516711,40.3882549149229,12.));
#90584=CARTESIAN_POINT('Ctrl Pts',(-61.4966585685544,40.3929670101363,0.));
#90585=CARTESIAN_POINT('Ctrl Pts',(-61.4966585685544,40.3929670101363,12.));
#90586=CARTESIAN_POINT('Ctrl Pts',(-61.5229218721532,40.3976614010648,0.));
#90587=CARTESIAN_POINT('Ctrl Pts',(-61.5229218721532,40.3976614010648,12.));
#90588=CARTESIAN_POINT('Ctrl Pts',(-61.5492256804709,40.4023380237227,0.));
#90589=CARTESIAN_POINT('Ctrl Pts',(-61.5492256804709,40.4023380237227,12.));
#90590=CARTESIAN_POINT('Ctrl Pts',(-61.5755699117318,40.4069968143953,0.));
#90591=CARTESIAN_POINT('Ctrl Pts',(-61.5755699117318,40.4069968143953,12.));
#90592=CARTESIAN_POINT('Ctrl Pts',(-61.6019544843009,40.4116377095595,0.));
#90593=CARTESIAN_POINT('Ctrl Pts',(-61.6019544843009,40.4116377095595,12.));
#90594=CARTESIAN_POINT('Ctrl Pts',(-61.628379316608,40.4162606458119,0.));
#90595=CARTESIAN_POINT('Ctrl Pts',(-61.628379316608,40.4162606458119,12.));
#90596=CARTESIAN_POINT('Ctrl Pts',(-61.6548443270397,40.420865559772,0.));
#90597=CARTESIAN_POINT('Ctrl Pts',(-61.6548443270397,40.420865559772,12.));
#90598=CARTESIAN_POINT('Ctrl Pts',(-61.6813494339295,40.4254523880766,0.));
#90599=CARTESIAN_POINT('Ctrl Pts',(-61.6813494339295,40.4254523880766,12.));
#90600=CARTESIAN_POINT('Ctrl Pts',(-61.7078945557812,40.4300210675848,0.));
#90601=CARTESIAN_POINT('Ctrl Pts',(-61.7078945557812,40.4300210675848,12.));
#90602=CARTESIAN_POINT('Ctrl Pts',(-61.7344796114409,40.4345715355411,0.));
#90603=CARTESIAN_POINT('Ctrl Pts',(-61.7344796114409,40.4345715355411,12.));
#90604=CARTESIAN_POINT('Ctrl Pts',(-61.7611045202875,40.439103729759,0.));
#90605=CARTESIAN_POINT('Ctrl Pts',(-61.7611045202875,40.439103729759,12.));
#90606=CARTESIAN_POINT('Ctrl Pts',(-61.7877692024064,40.4436175887942,0.));
#90607=CARTESIAN_POINT('Ctrl Pts',(-61.7877692024064,40.4436175887942,12.));
#90608=CARTESIAN_POINT('Ctrl Pts',(-61.8144735787767,40.448113052135,0.));
#90609=CARTESIAN_POINT('Ctrl Pts',(-61.8144735787767,40.448113052135,12.));
#90610=CARTESIAN_POINT('Ctrl Pts',(-61.8412175708524,40.4525900597877,0.));
#90611=CARTESIAN_POINT('Ctrl Pts',(-61.8412175708524,40.4525900597877,12.));
#90612=CARTESIAN_POINT('Ctrl Pts',(-61.8680011001513,40.4570485518735,0.));
#90613=CARTESIAN_POINT('Ctrl Pts',(-61.8680011001513,40.4570485518735,12.));
#90614=CARTESIAN_POINT('Ctrl Pts',(-61.8948240877998,40.4614884681884,0.));
#90615=CARTESIAN_POINT('Ctrl Pts',(-61.8948240877998,40.4614884681884,12.));
#90616=CARTESIAN_POINT('Ctrl Pts',(-61.9216864541758,40.4659097478595,0.));
#90617=CARTESIAN_POINT('Ctrl Pts',(-61.9216864541758,40.4659097478595,12.));
#90618=CARTESIAN_POINT('Ctrl Pts',(-61.9485881182957,40.4703123287642,0.));
#90619=CARTESIAN_POINT('Ctrl Pts',(-61.9485881182957,40.4703123287642,12.));
#90620=CARTESIAN_POINT('Ctrl Pts',(-61.9755289983094,40.4746961480045,0.));
#90621=CARTESIAN_POINT('Ctrl Pts',(-61.9755289983094,40.4746961480045,12.));
#90622=CARTESIAN_POINT('Ctrl Pts',(-62.0025090126008,40.4790611429613,0.));
#90623=CARTESIAN_POINT('Ctrl Pts',(-62.0025090126008,40.4790611429613,12.));
#90624=CARTESIAN_POINT('Ctrl Pts',(-62.0295280807449,40.4834072522181,0.));
#90625=CARTESIAN_POINT('Ctrl Pts',(-62.0295280807449,40.4834072522181,12.));
#90626=CARTESIAN_POINT('Ctrl Pts',(-62.0565861244171,40.4877344164407,0.));
#90627=CARTESIAN_POINT('Ctrl Pts',(-62.0565861244171,40.4877344164407,12.));
#90628=CARTESIAN_POINT('Ctrl Pts',(-62.0836830685665,40.4920425795184,0.));
#90629=CARTESIAN_POINT('Ctrl Pts',(-62.0836830685665,40.4920425795184,12.));
#90630=CARTESIAN_POINT('Ctrl Pts',(-62.110818841691,40.4963316888357,0.));
#90631=CARTESIAN_POINT('Ctrl Pts',(-62.110818841691,40.4963316888357,12.));
#90632=CARTESIAN_POINT('Ctrl Pts',(-62.137993373242,40.5006016927489,0.));
#90633=CARTESIAN_POINT('Ctrl Pts',(-62.137993373242,40.5006016927489,12.));
#90634=CARTESIAN_POINT('Ctrl Pts',(-62.1652065915724,40.5048525385985,0.));
#90635=CARTESIAN_POINT('Ctrl Pts',(-62.1652065915724,40.5048525385985,12.));
#90636=CARTESIAN_POINT('Ctrl Pts',(-62.1924584215634,40.5090841704111,0.));
#90637=CARTESIAN_POINT('Ctrl Pts',(-62.1924584215634,40.5090841704111,12.));
#90638=CARTESIAN_POINT('Ctrl Pts',(-62.2197487826212,40.5132965269679,0.));
#90639=CARTESIAN_POINT('Ctrl Pts',(-62.2197487826212,40.5132965269679,12.));
#90640=CARTESIAN_POINT('Ctrl Pts',(-62.2470775858834,40.5174895391059,0.));
#90641=CARTESIAN_POINT('Ctrl Pts',(-62.2470775858834,40.5174895391059,12.));
#90642=CARTESIAN_POINT('Ctrl Pts',(-62.2744447382207,40.5216631336335,0.));
#90643=CARTESIAN_POINT('Ctrl Pts',(-62.2744447382207,40.5216631336335,12.));
#90644=CARTESIAN_POINT('Ctrl Pts',(-62.3018501471876,40.5258172381565,0.));
#90645=CARTESIAN_POINT('Ctrl Pts',(-62.3018501471876,40.5258172381565,12.));
#90646=CARTESIAN_POINT('Ctrl Pts',(-62.3292937258021,40.5299517857793,0.));
#90647=CARTESIAN_POINT('Ctrl Pts',(-62.3292937258021,40.5299517857793,12.));
#90648=CARTESIAN_POINT('Ctrl Pts',(-62.35677539702,40.5340667194272,0.));
#90649=CARTESIAN_POINT('Ctrl Pts',(-62.35677539702,40.5340667194272,12.));
#90650=CARTESIAN_POINT('Ctrl Pts',(-62.3842950992504,40.5381619973972,0.));
#90651=CARTESIAN_POINT('Ctrl Pts',(-62.3842950992504,40.5381619973972,12.));
#90652=CARTESIAN_POINT('Ctrl Pts',(-62.4118527880601,40.5422375944697,0.));
#90653=CARTESIAN_POINT('Ctrl Pts',(-62.4118527880601,40.5422375944697,12.));
#90654=CARTESIAN_POINT('Ctrl Pts',(-62.439448432904,40.5462934972334,0.));
#90655=CARTESIAN_POINT('Ctrl Pts',(-62.439448432904,40.5462934972334,12.));
#90656=CARTESIAN_POINT('Ctrl Pts',(-62.4615552986669,40.5495224601437,0.));
#90657=CARTESIAN_POINT('Ctrl Pts',(-62.4615552986669,40.5495224601437,12.));
#90658=CARTESIAN_POINT('Ctrl Pts',(-62.4781525155997,40.5519353177058,0.));
#90659=CARTESIAN_POINT('Ctrl Pts',(-62.4781525155997,40.5519353177058,12.));
#90660=CARTESIAN_POINT('Ctrl Pts',(-62.4892249121863,40.5535399497449,0.));
#90661=CARTESIAN_POINT('Ctrl Pts',(-62.4892249121863,40.5535399497449,12.));
#90662=CARTESIAN_POINT('Ctrl Pts',(-62.4947630068039,40.554341280847,0.));
#90663=CARTESIAN_POINT('Ctrl Pts',(-62.4947630068039,40.554341280847,12.));
#90664=CARTESIAN_POINT('',(-57.8261117662438,39.4479504917287,0.));
#90665=CARTESIAN_POINT('Ctrl Pts',(-57.8261117662438,39.4479504917287,0.));
#90666=CARTESIAN_POINT('Ctrl Pts',(-57.8297740100947,39.4492429618443,0.));
#90667=CARTESIAN_POINT('Ctrl Pts',(-57.837104315141,39.4518277003553,0.));
#90668=CARTESIAN_POINT('Ctrl Pts',(-57.8481172247496,39.4557042029652,0.));
#90669=CARTESIAN_POINT('Ctrl Pts',(-57.8628360096803,39.4608716627117,0.));
#90670=CARTESIAN_POINT('Ctrl Pts',(-57.8812926637177,39.4673289592259,0.));
#90671=CARTESIAN_POINT('Ctrl Pts',(-57.8998074670478,39.473784194937,0.));
#90672=CARTESIAN_POINT('Ctrl Pts',(-57.9183803632403,39.4802373061058,0.));
#90673=CARTESIAN_POINT('Ctrl Pts',(-57.937011245663,39.4866881842317,0.));
#90674=CARTESIAN_POINT('Ctrl Pts',(-57.9556999583892,39.4931366776714,0.));
#90675=CARTESIAN_POINT('Ctrl Pts',(-57.974446317937,39.499582610674,0.));
#90676=CARTESIAN_POINT('Ctrl Pts',(-57.9932501298522,39.5060257981225,0.));
#90677=CARTESIAN_POINT('Ctrl Pts',(-58.0121112067895,39.5124660614976,0.));
#90678=CARTESIAN_POINT('Ctrl Pts',(-58.0310293875262,39.5189032457184,0.));
#90679=CARTESIAN_POINT('Ctrl Pts',(-58.0500045308412,39.5253372136887,0.));
#90680=CARTESIAN_POINT('Ctrl Pts',(-58.0690365065374,39.5317678383217,0.));
#90681=CARTESIAN_POINT('Ctrl Pts',(-58.0881251879921,39.5381949959221,0.));
#90682=CARTESIAN_POINT('Ctrl Pts',(-58.1072704428928,39.5446185579638,0.));
#90683=CARTESIAN_POINT('Ctrl Pts',(-58.126472128574,39.5510383869505,0.));
#90684=CARTESIAN_POINT('Ctrl Pts',(-58.1457300968499,39.5574543406982,0.));
#90685=CARTESIAN_POINT('Ctrl Pts',(-58.1650441970387,39.563866275018,0.));
#90686=CARTESIAN_POINT('Ctrl Pts',(-58.1844142794338,39.5702740467999,0.));
#90687=CARTESIAN_POINT('Ctrl Pts',(-58.2038401992457,39.57667751752,0.));
#90688=CARTESIAN_POINT('Ctrl Pts',(-58.2233218164365,39.5830765530891,0.));
#90689=CARTESIAN_POINT('Ctrl Pts',(-58.2428589938369,39.5894710221713,0.));
#90690=CARTESIAN_POINT('Ctrl Pts',(-58.2624515958419,39.5958607950239,0.));
#90691=CARTESIAN_POINT('Ctrl Pts',(-58.2820994868118,39.602245742079,0.));
#90692=CARTESIAN_POINT('Ctrl Pts',(-58.3018025297323,39.6086257327583,0.));
#90693=CARTESIAN_POINT('Ctrl Pts',(-58.3215605869221,39.6150006360914,0.));
#90694=CARTESIAN_POINT('Ctrl Pts',(-58.3413735206423,39.6213703212531,0.));
#90695=CARTESIAN_POINT('Ctrl Pts',(-58.3612411936905,39.6277346580892,0.));
#90696=CARTESIAN_POINT('Ctrl Pts',(-58.3811634701037,39.6340935177476,0.));
#90697=CARTESIAN_POINT('Ctrl Pts',(-58.4011402154196,39.6404467729094,0.));
#90698=CARTESIAN_POINT('Ctrl Pts',(-58.4211712963004,39.6467942974451,0.));
#90699=CARTESIAN_POINT('Ctrl Pts',(-58.4412565802979,39.653135966204,0.));
#90700=CARTESIAN_POINT('Ctrl Pts',(-58.4613959355788,39.6594716547689,0.));
#90701=CARTESIAN_POINT('Ctrl Pts',(-58.4815892306066,39.6658012391815,0.));
#90702=CARTESIAN_POINT('Ctrl Pts',(-58.5018363341604,39.6721245959531,0.));
#90703=CARTESIAN_POINT('Ctrl Pts',(-58.5221371154761,39.6784416021826,0.));
#90704=CARTESIAN_POINT('Ctrl Pts',(-58.5424914443415,39.6847521356395,0.));
#90705=CARTESIAN_POINT('Ctrl Pts',(-58.5628991912052,39.6910560748629,0.));
#90706=CARTESIAN_POINT('Ctrl Pts',(-58.5833602272744,39.6973532992539,0.));
#90707=CARTESIAN_POINT('Ctrl Pts',(-58.6038744244659,39.7036436890233,0.));
#90708=CARTESIAN_POINT('Ctrl Pts',(-58.6244416553562,39.7099271251413,0.));
#90709=CARTESIAN_POINT('Ctrl Pts',(-58.6450617931274,39.7162034892899,0.));
#90710=CARTESIAN_POINT('Ctrl Pts',(-58.6657347115034,39.72247266381,0.));
#90711=CARTESIAN_POINT('Ctrl Pts',(-58.6864602847088,39.7287345316681,0.));
#90712=CARTESIAN_POINT('Ctrl Pts',(-58.7072383875027,39.734988976475,0.));
#90713=CARTESIAN_POINT('Ctrl Pts',(-58.7280688951916,39.7412358824953,0.));
#90714=CARTESIAN_POINT('Ctrl Pts',(-58.7489516836445,39.7474751346598,0.));
#90715=CARTESIAN_POINT('Ctrl Pts',(-58.7698866293029,39.7537066185813,0.));
#90716=CARTESIAN_POINT('Ctrl Pts',(-58.7908736091798,39.7599302205521,0.));
#90717=CARTESIAN_POINT('Ctrl Pts',(-58.8119125008517,39.7661458275274,0.));
#90718=CARTESIAN_POINT('Ctrl Pts',(-58.8330031824453,39.772353327112,0.));
#90719=CARTESIAN_POINT('Ctrl Pts',(-58.8541455326231,39.7785526075478,0.));
#90720=CARTESIAN_POINT('Ctrl Pts',(-58.8753394305585,39.7847435576996,0.));
#90721=CARTESIAN_POINT('Ctrl Pts',(-58.8965847559391,39.7909260670517,0.));
#90722=CARTESIAN_POINT('Ctrl Pts',(-58.9178813889704,39.7971000257044,0.));
#90723=CARTESIAN_POINT('Ctrl Pts',(-58.9392292103747,39.8032653243712,0.));
#90724=CARTESIAN_POINT('Ctrl Pts',(-58.9606281013875,39.8094218543782,0.));
#90725=CARTESIAN_POINT('Ctrl Pts',(-58.9820779437484,39.8155695076626,0.));
#90726=CARTESIAN_POINT('Ctrl Pts',(-59.0035786197024,39.821708176766,0.));
#90727=CARTESIAN_POINT('Ctrl Pts',(-59.0251300119973,39.8278377548262,0.));
#90728=CARTESIAN_POINT('Ctrl Pts',(-59.0467320038784,39.8339581355716,0.));
#90729=CARTESIAN_POINT('Ctrl Pts',(-59.0683844790764,39.8400692133139,0.));
#90730=CARTESIAN_POINT('Ctrl Pts',(-59.090087321798,39.8461708829456,0.));
#90731=CARTESIAN_POINT('Ctrl Pts',(-59.1118404167292,39.8522630399328,0.));
#90732=CARTESIAN_POINT('Ctrl Pts',(-59.1336436490342,39.8583455803105,0.));
#90733=CARTESIAN_POINT('Ctrl Pts',(-59.1554969043522,39.8644184006787,0.));
#90734=CARTESIAN_POINT('Ctrl Pts',(-59.1774000687879,39.8704813981988,0.));
#90735=CARTESIAN_POINT('Ctrl Pts',(-59.1993530289028,39.876534470591,0.));
#90736=CARTESIAN_POINT('Ctrl Pts',(-59.2213556717209,39.8825775161267,0.));
#90737=CARTESIAN_POINT('Ctrl Pts',(-59.2434078847247,39.8886104336242,0.));
#90738=CARTESIAN_POINT('Ctrl Pts',(-59.2655095558521,39.8946331224438,0.));
#90739=CARTESIAN_POINT('Ctrl Pts',(-59.2876605734846,39.9006454824845,0.));
#90740=CARTESIAN_POINT('Ctrl Pts',(-59.3098608264419,39.9066474141803,0.));
#90741=CARTESIAN_POINT('Ctrl Pts',(-59.3321102039852,39.9126388184936,0.));
#90742=CARTESIAN_POINT('Ctrl Pts',(-59.3544085958151,39.9186195969104,0.));
#90743=CARTESIAN_POINT('Ctrl Pts',(-59.3767558920675,39.9245896514367,0.));
#90744=CARTESIAN_POINT('Ctrl Pts',(-59.3991519833016,39.9305488845958,0.));
#90745=CARTESIAN_POINT('Ctrl Pts',(-59.4215967604967,39.9364971994242,0.));
#90746=CARTESIAN_POINT('Ctrl Pts',(-59.4440901150582,39.9424344994672,0.));
#90747=CARTESIAN_POINT('Ctrl Pts',(-59.4666319388133,39.9483606887737,0.));
#90748=CARTESIAN_POINT('Ctrl Pts',(-59.4892221240068,39.9542756718922,0.));
#90749=CARTESIAN_POINT('Ctrl Pts',(-59.5118605632891,39.9601793538682,0.));
#90750=CARTESIAN_POINT('Ctrl Pts',(-59.5345471497129,39.9660716402403,0.));
#90751=CARTESIAN_POINT('Ctrl Pts',(-59.5572817767388,39.9719524370345,0.));
#90752=CARTESIAN_POINT('Ctrl Pts',(-59.5800643382314,39.9778216507605,0.));
#90753=CARTESIAN_POINT('Ctrl Pts',(-59.6028947284562,39.9836791884079,0.));
#90754=CARTESIAN_POINT('Ctrl Pts',(-59.6257728420669,39.9895249574448,0.));
#90755=CARTESIAN_POINT('Ctrl Pts',(-59.6486985741041,39.9953588658132,0.));
#90756=CARTESIAN_POINT('Ctrl Pts',(-59.6716718200005,40.0011808219241,0.));
#90757=CARTESIAN_POINT('Ctrl Pts',(-59.6946924755773,40.0069907346537,0.));
#90758=CARTESIAN_POINT('Ctrl Pts',(-59.7177604370403,40.0127885133403,0.));
#90759=CARTESIAN_POINT('Ctrl Pts',(-59.7408756009679,40.0185740677821,0.));
#90760=CARTESIAN_POINT('Ctrl Pts',(-59.7640378643106,40.0243473082337,0.));
#90761=CARTESIAN_POINT('Ctrl Pts',(-59.7872471243942,40.0301081454002,0.));
#90762=CARTESIAN_POINT('Ctrl Pts',(-59.8105032789179,40.035856490434,0.));
#90763=CARTESIAN_POINT('Ctrl Pts',(-59.8338062259492,40.0415922549315,0.));
#90764=CARTESIAN_POINT('Ctrl Pts',(-59.8571558639145,40.0473153509324,0.));
#90765=CARTESIAN_POINT('Ctrl Pts',(-59.8805520915972,40.0530256909161,0.));
#90766=CARTESIAN_POINT('Ctrl Pts',(-59.9039948081428,40.0587231877959,0.));
#90767=CARTESIAN_POINT('Ctrl Pts',(-59.927483913055,40.0644077549158,0.));
#90768=CARTESIAN_POINT('Ctrl Pts',(-59.9510193061929,40.0700793060475,0.));
#90769=CARTESIAN_POINT('Ctrl Pts',(-59.974600887759,40.0757377553893,0.));
#90770=CARTESIAN_POINT('Ctrl Pts',(-59.9982285582991,40.0813830175629,0.));
#90771=CARTESIAN_POINT('Ctrl Pts',(-60.0219022187066,40.0870150076078,0.));
#90772=CARTESIAN_POINT('Ctrl Pts',(-60.0456217702203,40.0926336409787,0.));
#90773=CARTESIAN_POINT('Ctrl Pts',(-60.0693871144207,40.0982388335421,0.));
#90774=CARTESIAN_POINT('Ctrl Pts',(-60.0931981532194,40.1038305015763,0.));
#90775=CARTESIAN_POINT('Ctrl Pts',(-60.1170547888572,40.1094085617672,0.));
#90776=CARTESIAN_POINT('Ctrl Pts',(-60.1409569239093,40.1149729312036,0.));
#90777=CARTESIAN_POINT('Ctrl Pts',(-60.1649044612829,40.120523527374,0.));
#90778=CARTESIAN_POINT('Ctrl Pts',(-60.1888973042151,40.1260602681644,0.));
#90779=CARTESIAN_POINT('Ctrl Pts',(-60.2129353562617,40.1315830718575,0.));
#90780=CARTESIAN_POINT('Ctrl Pts',(-60.2370185212957,40.13709185713,0.));
#90781=CARTESIAN_POINT('Ctrl Pts',(-60.2611467035109,40.1425865430468,0.));
#90782=CARTESIAN_POINT('Ctrl Pts',(-60.2853198074215,40.1480670490583,0.));
#90783=CARTESIAN_POINT('Ctrl Pts',(-60.3095377378589,40.1535332949978,0.));
#90784=CARTESIAN_POINT('Ctrl Pts',(-60.3338003999616,40.1589852010811,0.));
#90785=CARTESIAN_POINT('Ctrl Pts',(-60.3581076991731,40.1644226879043,0.));
#90786=CARTESIAN_POINT('Ctrl Pts',(-60.382459541246,40.1698456764387,0.));
#90787=CARTESIAN_POINT('Ctrl Pts',(-60.4068558322415,40.1752540880273,0.));
#90788=CARTESIAN_POINT('Ctrl Pts',(-60.4312964785269,40.1806478443828,0.));
#90789=CARTESIAN_POINT('Ctrl Pts',(-60.4557813867677,40.1860268675875,0.));
#90790=CARTESIAN_POINT('Ctrl Pts',(-60.4803104639211,40.1913910800911,0.));
#90791=CARTESIAN_POINT('Ctrl Pts',(-60.5048836172424,40.1967404047055,0.));
#90792=CARTESIAN_POINT('Ctrl Pts',(-60.5295007542838,40.2020747646012,0.));
#90793=CARTESIAN_POINT('Ctrl Pts',(-60.5541617828927,40.2073940833054,0.));
#90794=CARTESIAN_POINT('Ctrl Pts',(-60.5788666112043,40.2126982847012,0.));
#90795=CARTESIAN_POINT('Ctrl Pts',(-60.6036151476347,40.2179872930272,0.));
#90796=CARTESIAN_POINT('Ctrl Pts',(-60.6284073008865,40.2232610328717,0.));
#90797=CARTESIAN_POINT('Ctrl Pts',(-60.6532429799493,40.2285194291702,0.));
#90798=CARTESIAN_POINT('Ctrl Pts',(-60.678122094098,40.2337624072029,0.));
#90799=CARTESIAN_POINT('Ctrl Pts',(-60.7030445528863,40.2389898925937,0.));
#90800=CARTESIAN_POINT('Ctrl Pts',(-60.72801026614,40.2442018113116,0.));
#90801=CARTESIAN_POINT('Ctrl Pts',(-60.7530191439603,40.2493980896646,0.));
#90802=CARTESIAN_POINT('Ctrl Pts',(-60.7780710967253,40.2545786542957,0.));
#90803=CARTESIAN_POINT('Ctrl Pts',(-60.8031660350879,40.2597434321804,0.));
#90804=CARTESIAN_POINT('Ctrl Pts',(-60.8283038699703,40.2648923506245,0.));
#90805=CARTESIAN_POINT('Ctrl Pts',(-60.8534845125535,40.2700253372644,0.));
#90806=CARTESIAN_POINT('Ctrl Pts',(-60.8787078742817,40.2751423200637,0.));
#90807=CARTESIAN_POINT('Ctrl Pts',(-60.903973866867,40.2802432273105,0.));
#90808=CARTESIAN_POINT('Ctrl Pts',(-60.9292824022888,40.2853279876162,0.));
#90809=CARTESIAN_POINT('Ctrl Pts',(-60.9546333927919,40.2903965299155,0.));
#90810=CARTESIAN_POINT('Ctrl Pts',(-60.9800267508781,40.2954487834688,0.));
#90811=CARTESIAN_POINT('Ctrl Pts',(-61.005462389306,40.3004846778577,0.));
#90812=CARTESIAN_POINT('Ctrl Pts',(-61.0309402210915,40.3055041429772,0.));
#90813=CARTESIAN_POINT('Ctrl Pts',(-61.0564601595047,40.3105071090308,0.));
#90814=CARTESIAN_POINT('Ctrl Pts',(-61.0820221180646,40.3154935065264,0.));
#90815=CARTESIAN_POINT('Ctrl Pts',(-61.1076260105265,40.3204632662729,0.));
#90816=CARTESIAN_POINT('Ctrl Pts',(-61.1332717508799,40.3254163193806,0.));
#90817=CARTESIAN_POINT('Ctrl Pts',(-61.1589592533623,40.3303525972621,0.));
#90818=CARTESIAN_POINT('Ctrl Pts',(-61.184688432465,40.3352720316373,0.));
#90819=CARTESIAN_POINT('Ctrl Pts',(-61.2104592029375,40.3401745545369,0.));
#90820=CARTESIAN_POINT('Ctrl Pts',(-61.236271479789,40.3450600983104,0.));
#90821=CARTESIAN_POINT('Ctrl Pts',(-61.2621251782849,40.3499285956297,0.));
#90822=CARTESIAN_POINT('Ctrl Pts',(-61.2880202139358,40.3547799794672,0.));
#90823=CARTESIAN_POINT('Ctrl Pts',(-61.3139565024838,40.3596141830786,0.));
#90824=CARTESIAN_POINT('Ctrl Pts',(-61.3399339598851,40.3644311399861,0.));
#90825=CARTESIAN_POINT('Ctrl Pts',(-61.3659525022917,40.3692307839642,0.));
#90826=CARTESIAN_POINT('Ctrl Pts',(-61.3920120460232,40.3740130490233,0.));
#90827=CARTESIAN_POINT('Ctrl Pts',(-61.418112507605,40.3787778694373,0.));
#90828=CARTESIAN_POINT('Ctrl Pts',(-61.4442538038053,40.3835251797725,0.));
#90829=CARTESIAN_POINT('Ctrl Pts',(-61.4704358516711,40.3882549149229,0.));
#90830=CARTESIAN_POINT('Ctrl Pts',(-61.4966585685544,40.3929670101363,0.));
#90831=CARTESIAN_POINT('Ctrl Pts',(-61.5229218721532,40.3976614010648,0.));
#90832=CARTESIAN_POINT('Ctrl Pts',(-61.5492256804709,40.4023380237227,0.));
#90833=CARTESIAN_POINT('Ctrl Pts',(-61.5755699117318,40.4069968143953,0.));
#90834=CARTESIAN_POINT('Ctrl Pts',(-61.6019544843009,40.4116377095595,0.));
#90835=CARTESIAN_POINT('Ctrl Pts',(-61.628379316608,40.4162606458119,0.));
#90836=CARTESIAN_POINT('Ctrl Pts',(-61.6548443270397,40.420865559772,0.));
#90837=CARTESIAN_POINT('Ctrl Pts',(-61.6813494339295,40.4254523880766,0.));
#90838=CARTESIAN_POINT('Ctrl Pts',(-61.7078945557812,40.4300210675848,0.));
#90839=CARTESIAN_POINT('Ctrl Pts',(-61.7344796114409,40.4345715355411,0.));
#90840=CARTESIAN_POINT('Ctrl Pts',(-61.7611045202875,40.439103729759,0.));
#90841=CARTESIAN_POINT('Ctrl Pts',(-61.7877692024064,40.4436175887942,0.));
#90842=CARTESIAN_POINT('Ctrl Pts',(-61.8144735787767,40.448113052135,0.));
#90843=CARTESIAN_POINT('Ctrl Pts',(-61.8412175708524,40.4525900597877,0.));
#90844=CARTESIAN_POINT('Ctrl Pts',(-61.8680011001513,40.4570485518735,0.));
#90845=CARTESIAN_POINT('Ctrl Pts',(-61.8948240877998,40.4614884681884,0.));
#90846=CARTESIAN_POINT('Ctrl Pts',(-61.9216864541758,40.4659097478595,0.));
#90847=CARTESIAN_POINT('Ctrl Pts',(-61.9485881182957,40.4703123287642,0.));
#90848=CARTESIAN_POINT('Ctrl Pts',(-61.9755289983094,40.4746961480045,0.));
#90849=CARTESIAN_POINT('Ctrl Pts',(-62.0025090126008,40.4790611429613,0.));
#90850=CARTESIAN_POINT('Ctrl Pts',(-62.0295280807449,40.4834072522181,0.));
#90851=CARTESIAN_POINT('Ctrl Pts',(-62.0565861244171,40.4877344164407,0.));
#90852=CARTESIAN_POINT('Ctrl Pts',(-62.0836830685665,40.4920425795184,0.));
#90853=CARTESIAN_POINT('Ctrl Pts',(-62.110818841691,40.4963316888357,0.));
#90854=CARTESIAN_POINT('Ctrl Pts',(-62.1341126810364,40.499991909619,0.));
#90855=CARTESIAN_POINT('Ctrl Pts',(-62.1519925002737,40.5027877865724,0.));
#90856=CARTESIAN_POINT('Ctrl Pts',(-62.1644411502531,40.5047277935688,0.));
#90857=CARTESIAN_POINT('Ctrl Pts',(-62.1714473137753,40.5058175523045,0.));
#90858=CARTESIAN_POINT('Ctrl Pts',(-62.1730054756455,40.5060598100838,0.));
#90859=CARTESIAN_POINT('',(-57.8261117662438,39.4479504917287,12.));
#90860=CARTESIAN_POINT('',(-57.8261117662438,39.4479504917287,0.));
#90861=CARTESIAN_POINT('Ctrl Pts',(-62.1730054756454,40.5060598100838,12.));
#90862=CARTESIAN_POINT('Ctrl Pts',(-62.1714473137753,40.5058175523045,12.));
#90863=CARTESIAN_POINT('Ctrl Pts',(-62.1644411502531,40.5047277935688,12.));
#90864=CARTESIAN_POINT('Ctrl Pts',(-62.1519925002737,40.5027877865724,12.));
#90865=CARTESIAN_POINT('Ctrl Pts',(-62.1341126810364,40.499991909619,12.));
#90866=CARTESIAN_POINT('Ctrl Pts',(-62.110818841691,40.4963316888357,12.));
#90867=CARTESIAN_POINT('Ctrl Pts',(-62.0836830685665,40.4920425795184,12.));
#90868=CARTESIAN_POINT('Ctrl Pts',(-62.0565861244171,40.4877344164407,12.));
#90869=CARTESIAN_POINT('Ctrl Pts',(-62.0295280807449,40.4834072522181,12.));
#90870=CARTESIAN_POINT('Ctrl Pts',(-62.0025090126008,40.4790611429613,12.));
#90871=CARTESIAN_POINT('Ctrl Pts',(-61.9755289983094,40.4746961480045,12.));
#90872=CARTESIAN_POINT('Ctrl Pts',(-61.9485881182957,40.4703123287642,12.));
#90873=CARTESIAN_POINT('Ctrl Pts',(-61.9216864541758,40.4659097478595,12.));
#90874=CARTESIAN_POINT('Ctrl Pts',(-61.8948240877998,40.4614884681884,12.));
#90875=CARTESIAN_POINT('Ctrl Pts',(-61.8680011001513,40.4570485518735,12.));
#90876=CARTESIAN_POINT('Ctrl Pts',(-61.8412175708524,40.4525900597877,12.));
#90877=CARTESIAN_POINT('Ctrl Pts',(-61.8144735787767,40.448113052135,12.));
#90878=CARTESIAN_POINT('Ctrl Pts',(-61.7877692024064,40.4436175887942,12.));
#90879=CARTESIAN_POINT('Ctrl Pts',(-61.7611045202875,40.439103729759,12.));
#90880=CARTESIAN_POINT('Ctrl Pts',(-61.7344796114409,40.4345715355411,12.));
#90881=CARTESIAN_POINT('Ctrl Pts',(-61.7078945557812,40.4300210675848,12.));
#90882=CARTESIAN_POINT('Ctrl Pts',(-61.6813494339295,40.4254523880766,12.));
#90883=CARTESIAN_POINT('Ctrl Pts',(-61.6548443270397,40.420865559772,12.));
#90884=CARTESIAN_POINT('Ctrl Pts',(-61.628379316608,40.4162606458119,12.));
#90885=CARTESIAN_POINT('Ctrl Pts',(-61.6019544843009,40.4116377095595,12.));
#90886=CARTESIAN_POINT('Ctrl Pts',(-61.5755699117318,40.4069968143953,12.));
#90887=CARTESIAN_POINT('Ctrl Pts',(-61.5492256804709,40.4023380237227,12.));
#90888=CARTESIAN_POINT('Ctrl Pts',(-61.5229218721532,40.3976614010648,12.));
#90889=CARTESIAN_POINT('Ctrl Pts',(-61.4966585685544,40.3929670101363,12.));
#90890=CARTESIAN_POINT('Ctrl Pts',(-61.4704358516711,40.3882549149229,12.));
#90891=CARTESIAN_POINT('Ctrl Pts',(-61.4442538038053,40.3835251797725,12.));
#90892=CARTESIAN_POINT('Ctrl Pts',(-61.418112507605,40.3787778694373,12.));
#90893=CARTESIAN_POINT('Ctrl Pts',(-61.3920120460232,40.3740130490233,12.));
#90894=CARTESIAN_POINT('Ctrl Pts',(-61.3659525022917,40.3692307839642,12.));
#90895=CARTESIAN_POINT('Ctrl Pts',(-61.3399339598851,40.3644311399861,12.));
#90896=CARTESIAN_POINT('Ctrl Pts',(-61.3139565024838,40.3596141830786,12.));
#90897=CARTESIAN_POINT('Ctrl Pts',(-61.2880202139358,40.3547799794672,12.));
#90898=CARTESIAN_POINT('Ctrl Pts',(-61.2621251782849,40.3499285956297,12.));
#90899=CARTESIAN_POINT('Ctrl Pts',(-61.236271479789,40.3450600983104,12.));
#90900=CARTESIAN_POINT('Ctrl Pts',(-61.2104592029375,40.3401745545369,12.));
#90901=CARTESIAN_POINT('Ctrl Pts',(-61.184688432465,40.3352720316373,12.));
#90902=CARTESIAN_POINT('Ctrl Pts',(-61.1589592533623,40.3303525972621,12.));
#90903=CARTESIAN_POINT('Ctrl Pts',(-61.1332717508799,40.3254163193806,12.));
#90904=CARTESIAN_POINT('Ctrl Pts',(-61.1076260105265,40.3204632662729,12.));
#90905=CARTESIAN_POINT('Ctrl Pts',(-61.0820221180646,40.3154935065264,12.));
#90906=CARTESIAN_POINT('Ctrl Pts',(-61.0564601595047,40.3105071090308,12.));
#90907=CARTESIAN_POINT('Ctrl Pts',(-61.0309402210915,40.3055041429772,12.));
#90908=CARTESIAN_POINT('Ctrl Pts',(-61.005462389306,40.3004846778577,12.));
#90909=CARTESIAN_POINT('Ctrl Pts',(-60.9800267508781,40.2954487834688,12.));
#90910=CARTESIAN_POINT('Ctrl Pts',(-60.9546333927919,40.2903965299155,12.));
#90911=CARTESIAN_POINT('Ctrl Pts',(-60.9292824022888,40.2853279876162,12.));
#90912=CARTESIAN_POINT('Ctrl Pts',(-60.903973866867,40.2802432273105,12.));
#90913=CARTESIAN_POINT('Ctrl Pts',(-60.8787078742817,40.2751423200637,12.));
#90914=CARTESIAN_POINT('Ctrl Pts',(-60.8534845125535,40.2700253372644,12.));
#90915=CARTESIAN_POINT('Ctrl Pts',(-60.8283038699703,40.2648923506245,12.));
#90916=CARTESIAN_POINT('Ctrl Pts',(-60.8031660350879,40.2597434321804,12.));
#90917=CARTESIAN_POINT('Ctrl Pts',(-60.7780710967253,40.2545786542957,12.));
#90918=CARTESIAN_POINT('Ctrl Pts',(-60.7530191439603,40.2493980896646,12.));
#90919=CARTESIAN_POINT('Ctrl Pts',(-60.72801026614,40.2442018113116,12.));
#90920=CARTESIAN_POINT('Ctrl Pts',(-60.7030445528863,40.2389898925937,12.));
#90921=CARTESIAN_POINT('Ctrl Pts',(-60.678122094098,40.2337624072029,12.));
#90922=CARTESIAN_POINT('Ctrl Pts',(-60.6532429799493,40.2285194291702,12.));
#90923=CARTESIAN_POINT('Ctrl Pts',(-60.6284073008865,40.2232610328717,12.));
#90924=CARTESIAN_POINT('Ctrl Pts',(-60.6036151476347,40.2179872930272,12.));
#90925=CARTESIAN_POINT('Ctrl Pts',(-60.5788666112043,40.2126982847012,12.));
#90926=CARTESIAN_POINT('Ctrl Pts',(-60.5541617828927,40.2073940833054,12.));
#90927=CARTESIAN_POINT('Ctrl Pts',(-60.5295007542838,40.2020747646012,12.));
#90928=CARTESIAN_POINT('Ctrl Pts',(-60.5048836172424,40.1967404047055,12.));
#90929=CARTESIAN_POINT('Ctrl Pts',(-60.4803104639211,40.1913910800911,12.));
#90930=CARTESIAN_POINT('Ctrl Pts',(-60.4557813867677,40.1860268675875,12.));
#90931=CARTESIAN_POINT('Ctrl Pts',(-60.4312964785269,40.1806478443828,12.));
#90932=CARTESIAN_POINT('Ctrl Pts',(-60.4068558322415,40.1752540880273,12.));
#90933=CARTESIAN_POINT('Ctrl Pts',(-60.382459541246,40.1698456764387,12.));
#90934=CARTESIAN_POINT('Ctrl Pts',(-60.3581076991731,40.1644226879043,12.));
#90935=CARTESIAN_POINT('Ctrl Pts',(-60.3338003999616,40.1589852010811,12.));
#90936=CARTESIAN_POINT('Ctrl Pts',(-60.3095377378589,40.1535332949978,12.));
#90937=CARTESIAN_POINT('Ctrl Pts',(-60.2853198074215,40.1480670490583,12.));
#90938=CARTESIAN_POINT('Ctrl Pts',(-60.2611467035109,40.1425865430468,12.));
#90939=CARTESIAN_POINT('Ctrl Pts',(-60.2370185212957,40.13709185713,12.));
#90940=CARTESIAN_POINT('Ctrl Pts',(-60.2129353562617,40.1315830718575,12.));
#90941=CARTESIAN_POINT('Ctrl Pts',(-60.1888973042151,40.1260602681644,12.));
#90942=CARTESIAN_POINT('Ctrl Pts',(-60.1649044612829,40.120523527374,12.));
#90943=CARTESIAN_POINT('Ctrl Pts',(-60.1409569239093,40.1149729312036,12.));
#90944=CARTESIAN_POINT('Ctrl Pts',(-60.1170547888572,40.1094085617672,12.));
#90945=CARTESIAN_POINT('Ctrl Pts',(-60.0931981532194,40.1038305015763,12.));
#90946=CARTESIAN_POINT('Ctrl Pts',(-60.0693871144207,40.0982388335421,12.));
#90947=CARTESIAN_POINT('Ctrl Pts',(-60.0456217702203,40.0926336409787,12.));
#90948=CARTESIAN_POINT('Ctrl Pts',(-60.0219022187066,40.0870150076078,12.));
#90949=CARTESIAN_POINT('Ctrl Pts',(-59.9982285582991,40.0813830175629,12.));
#90950=CARTESIAN_POINT('Ctrl Pts',(-59.974600887759,40.0757377553893,12.));
#90951=CARTESIAN_POINT('Ctrl Pts',(-59.9510193061929,40.0700793060475,12.));
#90952=CARTESIAN_POINT('Ctrl Pts',(-59.927483913055,40.0644077549158,12.));
#90953=CARTESIAN_POINT('Ctrl Pts',(-59.9039948081428,40.0587231877959,12.));
#90954=CARTESIAN_POINT('Ctrl Pts',(-59.8805520915972,40.0530256909161,12.));
#90955=CARTESIAN_POINT('Ctrl Pts',(-59.8571558639145,40.0473153509324,12.));
#90956=CARTESIAN_POINT('Ctrl Pts',(-59.8338062259492,40.0415922549315,12.));
#90957=CARTESIAN_POINT('Ctrl Pts',(-59.8105032789179,40.035856490434,12.));
#90958=CARTESIAN_POINT('Ctrl Pts',(-59.7872471243942,40.0301081454002,12.));
#90959=CARTESIAN_POINT('Ctrl Pts',(-59.7640378643106,40.0243473082337,12.));
#90960=CARTESIAN_POINT('Ctrl Pts',(-59.7408756009679,40.0185740677821,12.));
#90961=CARTESIAN_POINT('Ctrl Pts',(-59.7177604370403,40.0127885133403,12.));
#90962=CARTESIAN_POINT('Ctrl Pts',(-59.6946924755773,40.0069907346537,12.));
#90963=CARTESIAN_POINT('Ctrl Pts',(-59.6716718200005,40.0011808219241,12.));
#90964=CARTESIAN_POINT('Ctrl Pts',(-59.6486985741041,39.9953588658132,12.));
#90965=CARTESIAN_POINT('Ctrl Pts',(-59.6257728420669,39.9895249574448,12.));
#90966=CARTESIAN_POINT('Ctrl Pts',(-59.6028947284562,39.9836791884079,12.));
#90967=CARTESIAN_POINT('Ctrl Pts',(-59.5800643382314,39.9778216507605,12.));
#90968=CARTESIAN_POINT('Ctrl Pts',(-59.5572817767388,39.9719524370345,12.));
#90969=CARTESIAN_POINT('Ctrl Pts',(-59.5345471497129,39.9660716402403,12.));
#90970=CARTESIAN_POINT('Ctrl Pts',(-59.5118605632891,39.9601793538682,12.));
#90971=CARTESIAN_POINT('Ctrl Pts',(-59.4892221240068,39.9542756718922,12.));
#90972=CARTESIAN_POINT('Ctrl Pts',(-59.4666319388133,39.9483606887737,12.));
#90973=CARTESIAN_POINT('Ctrl Pts',(-59.4440901150582,39.9424344994672,12.));
#90974=CARTESIAN_POINT('Ctrl Pts',(-59.4215967604967,39.9364971994242,12.));
#90975=CARTESIAN_POINT('Ctrl Pts',(-59.3991519833016,39.9305488845958,12.));
#90976=CARTESIAN_POINT('Ctrl Pts',(-59.3767558920675,39.9245896514367,12.));
#90977=CARTESIAN_POINT('Ctrl Pts',(-59.3544085958151,39.9186195969104,12.));
#90978=CARTESIAN_POINT('Ctrl Pts',(-59.3321102039852,39.9126388184936,12.));
#90979=CARTESIAN_POINT('Ctrl Pts',(-59.3098608264419,39.9066474141803,12.));
#90980=CARTESIAN_POINT('Ctrl Pts',(-59.2876605734846,39.9006454824845,12.));
#90981=CARTESIAN_POINT('Ctrl Pts',(-59.2655095558521,39.8946331224438,12.));
#90982=CARTESIAN_POINT('Ctrl Pts',(-59.2434078847247,39.8886104336242,12.));
#90983=CARTESIAN_POINT('Ctrl Pts',(-59.2213556717209,39.8825775161267,12.));
#90984=CARTESIAN_POINT('Ctrl Pts',(-59.1993530289028,39.876534470591,12.));
#90985=CARTESIAN_POINT('Ctrl Pts',(-59.1774000687879,39.8704813981988,12.));
#90986=CARTESIAN_POINT('Ctrl Pts',(-59.1554969043522,39.8644184006787,12.));
#90987=CARTESIAN_POINT('Ctrl Pts',(-59.1336436490342,39.8583455803105,12.));
#90988=CARTESIAN_POINT('Ctrl Pts',(-59.1118404167292,39.8522630399328,12.));
#90989=CARTESIAN_POINT('Ctrl Pts',(-59.090087321798,39.8461708829456,12.));
#90990=CARTESIAN_POINT('Ctrl Pts',(-59.0683844790764,39.8400692133139,12.));
#90991=CARTESIAN_POINT('Ctrl Pts',(-59.0467320038784,39.8339581355716,12.));
#90992=CARTESIAN_POINT('Ctrl Pts',(-59.0251300119973,39.8278377548262,12.));
#90993=CARTESIAN_POINT('Ctrl Pts',(-59.0035786197024,39.821708176766,12.));
#90994=CARTESIAN_POINT('Ctrl Pts',(-58.9820779437484,39.8155695076626,12.));
#90995=CARTESIAN_POINT('Ctrl Pts',(-58.9606281013875,39.8094218543782,12.));
#90996=CARTESIAN_POINT('Ctrl Pts',(-58.9392292103747,39.8032653243712,12.));
#90997=CARTESIAN_POINT('Ctrl Pts',(-58.9178813889704,39.7971000257044,12.));
#90998=CARTESIAN_POINT('Ctrl Pts',(-58.8965847559391,39.7909260670517,12.));
#90999=CARTESIAN_POINT('Ctrl Pts',(-58.8753394305585,39.7847435576996,12.));
#91000=CARTESIAN_POINT('Ctrl Pts',(-58.8541455326231,39.7785526075478,12.));
#91001=CARTESIAN_POINT('Ctrl Pts',(-58.8330031824453,39.772353327112,12.));
#91002=CARTESIAN_POINT('Ctrl Pts',(-58.8119125008517,39.7661458275274,12.));
#91003=CARTESIAN_POINT('Ctrl Pts',(-58.7908736091798,39.7599302205521,12.));
#91004=CARTESIAN_POINT('Ctrl Pts',(-58.7698866293029,39.7537066185813,12.));
#91005=CARTESIAN_POINT('Ctrl Pts',(-58.7489516836445,39.7474751346598,12.));
#91006=CARTESIAN_POINT('Ctrl Pts',(-58.7280688951916,39.7412358824953,12.));
#91007=CARTESIAN_POINT('Ctrl Pts',(-58.7072383875027,39.734988976475,12.));
#91008=CARTESIAN_POINT('Ctrl Pts',(-58.6864602847088,39.7287345316681,12.));
#91009=CARTESIAN_POINT('Ctrl Pts',(-58.6657347115034,39.72247266381,12.));
#91010=CARTESIAN_POINT('Ctrl Pts',(-58.6450617931274,39.7162034892899,12.));
#91011=CARTESIAN_POINT('Ctrl Pts',(-58.6244416553562,39.7099271251413,12.));
#91012=CARTESIAN_POINT('Ctrl Pts',(-58.6038744244659,39.7036436890233,12.));
#91013=CARTESIAN_POINT('Ctrl Pts',(-58.5833602272744,39.6973532992539,12.));
#91014=CARTESIAN_POINT('Ctrl Pts',(-58.5628991912052,39.6910560748629,12.));
#91015=CARTESIAN_POINT('Ctrl Pts',(-58.5424914443415,39.6847521356395,12.));
#91016=CARTESIAN_POINT('Ctrl Pts',(-58.5221371154761,39.6784416021826,12.));
#91017=CARTESIAN_POINT('Ctrl Pts',(-58.5018363341604,39.6721245959531,12.));
#91018=CARTESIAN_POINT('Ctrl Pts',(-58.4815892306066,39.6658012391815,12.));
#91019=CARTESIAN_POINT('Ctrl Pts',(-58.4613959355788,39.6594716547689,12.));
#91020=CARTESIAN_POINT('Ctrl Pts',(-58.4412565802979,39.653135966204,12.));
#91021=CARTESIAN_POINT('Ctrl Pts',(-58.4211712963004,39.6467942974451,12.));
#91022=CARTESIAN_POINT('Ctrl Pts',(-58.4011402154196,39.6404467729094,12.));
#91023=CARTESIAN_POINT('Ctrl Pts',(-58.3811634701037,39.6340935177476,12.));
#91024=CARTESIAN_POINT('Ctrl Pts',(-58.3612411936905,39.6277346580892,12.));
#91025=CARTESIAN_POINT('Ctrl Pts',(-58.3413735206423,39.6213703212531,12.));
#91026=CARTESIAN_POINT('Ctrl Pts',(-58.3215605869221,39.6150006360914,12.));
#91027=CARTESIAN_POINT('Ctrl Pts',(-58.3018025297323,39.6086257327583,12.));
#91028=CARTESIAN_POINT('Ctrl Pts',(-58.2820994868118,39.602245742079,12.));
#91029=CARTESIAN_POINT('Ctrl Pts',(-58.2624515958419,39.5958607950239,12.));
#91030=CARTESIAN_POINT('Ctrl Pts',(-58.2428589938369,39.5894710221713,12.));
#91031=CARTESIAN_POINT('Ctrl Pts',(-58.2233218164365,39.5830765530891,12.));
#91032=CARTESIAN_POINT('Ctrl Pts',(-58.2038401992457,39.57667751752,12.));
#91033=CARTESIAN_POINT('Ctrl Pts',(-58.1844142794338,39.5702740467999,12.));
#91034=CARTESIAN_POINT('Ctrl Pts',(-58.1650441970387,39.563866275018,12.));
#91035=CARTESIAN_POINT('Ctrl Pts',(-58.1457300968499,39.5574543406982,12.));
#91036=CARTESIAN_POINT('Ctrl Pts',(-58.126472128574,39.5510383869505,12.));
#91037=CARTESIAN_POINT('Ctrl Pts',(-58.1072704428928,39.5446185579638,12.));
#91038=CARTESIAN_POINT('Ctrl Pts',(-58.0881251879921,39.5381949959221,12.));
#91039=CARTESIAN_POINT('Ctrl Pts',(-58.0690365065374,39.5317678383217,12.));
#91040=CARTESIAN_POINT('Ctrl Pts',(-58.0500045308412,39.5253372136887,12.));
#91041=CARTESIAN_POINT('Ctrl Pts',(-58.0310293875262,39.5189032457184,12.));
#91042=CARTESIAN_POINT('Ctrl Pts',(-58.0121112067895,39.5124660614976,12.));
#91043=CARTESIAN_POINT('Ctrl Pts',(-57.9932501298522,39.5060257981225,12.));
#91044=CARTESIAN_POINT('Ctrl Pts',(-57.974446317937,39.499582610674,12.));
#91045=CARTESIAN_POINT('Ctrl Pts',(-57.9556999583892,39.4931366776714,12.));
#91046=CARTESIAN_POINT('Ctrl Pts',(-57.937011245663,39.4866881842317,12.));
#91047=CARTESIAN_POINT('Ctrl Pts',(-57.9183803632403,39.4802373061058,12.));
#91048=CARTESIAN_POINT('Ctrl Pts',(-57.8998074670478,39.473784194937,12.));
#91049=CARTESIAN_POINT('Ctrl Pts',(-57.8812926637177,39.4673289592259,12.));
#91050=CARTESIAN_POINT('Ctrl Pts',(-57.8628360096803,39.4608716627117,12.));
#91051=CARTESIAN_POINT('Ctrl Pts',(-57.8481172247496,39.4557042029652,12.));
#91052=CARTESIAN_POINT('Ctrl Pts',(-57.837104315141,39.4518277003553,12.));
#91053=CARTESIAN_POINT('Ctrl Pts',(-57.8297740100947,39.4492429618443,12.));
#91054=CARTESIAN_POINT('Ctrl Pts',(-57.8261117662438,39.4479504917287,12.));
#91055=CARTESIAN_POINT('Ctrl Pts',(-62.9864049293893,39.2292784191812,0.));
#91056=CARTESIAN_POINT('Ctrl Pts',(-62.9864049293893,39.2292784191812,4.));
#91057=CARTESIAN_POINT('Ctrl Pts',(-62.9864049293894,39.2292784191812,8.));
#91058=CARTESIAN_POINT('Ctrl Pts',(-62.9864049293894,39.2292784191812,12.));
#91059=CARTESIAN_POINT('Ctrl Pts',(-63.0475916539464,39.3205491216485,0.));
#91060=CARTESIAN_POINT('Ctrl Pts',(-63.0475916539464,39.3205491216485,4.));
#91061=CARTESIAN_POINT('Ctrl Pts',(-63.0475916539464,39.3205491216485,8.));
#91062=CARTESIAN_POINT('Ctrl Pts',(-63.0475916539464,39.3205491216485,12.));
#91063=CARTESIAN_POINT('Ctrl Pts',(-63.0996457958585,39.5164137621549,0.));
#91064=CARTESIAN_POINT('Ctrl Pts',(-63.0996457958585,39.5164137621549,4.00000000000001));
#91065=CARTESIAN_POINT('Ctrl Pts',(-63.0996457958585,39.516413762155,7.99999999999999));
#91066=CARTESIAN_POINT('Ctrl Pts',(-63.0996457958585,39.516413762155,12.));
#91067=CARTESIAN_POINT('Ctrl Pts',(-63.0378706912077,39.7049575044677,0.));
#91068=CARTESIAN_POINT('Ctrl Pts',(-63.0378706912077,39.7049575044677,4.));
#91069=CARTESIAN_POINT('Ctrl Pts',(-63.0378706912076,39.7049575044677,8.00000000000001));
#91070=CARTESIAN_POINT('Ctrl Pts',(-63.0378706912076,39.7049575044677,12.));
#91071=CARTESIAN_POINT('Ctrl Pts',(-62.9938720098783,39.774641283148,0.));
#91072=CARTESIAN_POINT('Ctrl Pts',(-62.9938720098783,39.774641283148,4.));
#91073=CARTESIAN_POINT('Ctrl Pts',(-62.9938720098783,39.774641283148,8.));
#91074=CARTESIAN_POINT('Ctrl Pts',(-62.9938720098783,39.774641283148,12.));
#91075=CARTESIAN_POINT('',(-62.9864049293893,39.2292784191812,0.));
#91076=CARTESIAN_POINT('',(-62.9938720098781,39.7746412831479,0.));
#91077=CARTESIAN_POINT('Ctrl Pts',(-62.9864049293893,39.2292784191812,2.77555756156289E-16));
#91078=CARTESIAN_POINT('Ctrl Pts',(-63.0475916539464,39.3205491216485,2.77555756156289E-16));
#91079=CARTESIAN_POINT('Ctrl Pts',(-63.0773368778962,39.4324717733665,2.77555756156289E-16));
#91080=CARTESIAN_POINT('Ctrl Pts',(-63.0699133682744,39.5420039277151,2.77555756156289E-16));
#91081=CARTESIAN_POINT('Ctrl Pts',(-63.064345736058,39.6241530434765,2.77555756156289E-16));
#91082=CARTESIAN_POINT('Ctrl Pts',(-63.0378706912077,39.7049575044677,2.77555756156289E-16));
#91083=CARTESIAN_POINT('Ctrl Pts',(-62.9938720098783,39.774641283148,2.77555756156289E-16));
#91084=CARTESIAN_POINT('',(-62.9938720098782,39.7746412831479,12.));
#91085=CARTESIAN_POINT('Ctrl Pts',(-62.9938720098783,39.774641283148,0.));
#91086=CARTESIAN_POINT('Ctrl Pts',(-62.9938720098783,39.774641283148,4.));
#91087=CARTESIAN_POINT('Ctrl Pts',(-62.9938720098783,39.774641283148,8.));
#91088=CARTESIAN_POINT('Ctrl Pts',(-62.9938720098783,39.774641283148,12.));
#91089=CARTESIAN_POINT('',(-62.9864049293894,39.2292784191812,12.));
#91090=CARTESIAN_POINT('Ctrl Pts',(-62.9938720098783,39.774641283148,12.));
#91091=CARTESIAN_POINT('Ctrl Pts',(-63.0378706912076,39.7049575044677,12.));
#91092=CARTESIAN_POINT('Ctrl Pts',(-63.064345736058,39.6241530434765,12.));
#91093=CARTESIAN_POINT('Ctrl Pts',(-63.0699133682744,39.5420039277151,12.));
#91094=CARTESIAN_POINT('Ctrl Pts',(-63.0773368778962,39.4324717733665,12.));
#91095=CARTESIAN_POINT('Ctrl Pts',(-63.0475916539464,39.3205491216485,12.));
#91096=CARTESIAN_POINT('Ctrl Pts',(-62.9864049293894,39.2292784191812,12.));
#91097=CARTESIAN_POINT('Ctrl Pts',(-62.9864049293894,39.2292784191812,12.));
#91098=CARTESIAN_POINT('Ctrl Pts',(-62.9864049293894,39.2292784191812,8.));
#91099=CARTESIAN_POINT('Ctrl Pts',(-62.9864049293893,39.2292784191812,4.));
#91100=CARTESIAN_POINT('Ctrl Pts',(-62.9864049293893,39.2292784191812,0.));
#91101=CARTESIAN_POINT('Origin',(-3.16193356404481E-10,2.01319694273778E-10,
0.));
#91102=CARTESIAN_POINT('Origin',(-3.16193356404481E-10,2.01319694273778E-10,
12.));
#91103=CARTESIAN_POINT('Origin',(-3.16193356404481E-10,2.01319694273778E-10,
0.));
#91104=CARTESIAN_POINT('Ctrl Pts',(-58.9211100416396,45.591148170023,0.));
#91105=CARTESIAN_POINT('Ctrl Pts',(-58.9211100416396,45.591148170023,4.));
#91106=CARTESIAN_POINT('Ctrl Pts',(-58.9211100416396,45.5911481700231,8.));
#91107=CARTESIAN_POINT('Ctrl Pts',(-58.9211100416396,45.5911481700231,12.));
#91108=CARTESIAN_POINT('Ctrl Pts',(-58.8538661785413,45.6780528262179,0.));
#91109=CARTESIAN_POINT('Ctrl Pts',(-58.8538661785413,45.6780528262179,4.));
#91110=CARTESIAN_POINT('Ctrl Pts',(-58.8538661785413,45.6780528262179,8.));
#91111=CARTESIAN_POINT('Ctrl Pts',(-58.8538661785413,45.6780528262179,12.));
#91112=CARTESIAN_POINT('Ctrl Pts',(-58.6845061116499,45.7893619681937,0.));
#91113=CARTESIAN_POINT('Ctrl Pts',(-58.6845061116499,45.7893619681937,4.00000000000001));
#91114=CARTESIAN_POINT('Ctrl Pts',(-58.6845061116498,45.7893619681937,7.99999999999999));
#91115=CARTESIAN_POINT('Ctrl Pts',(-58.6845061116498,45.7893619681937,12.));
#91116=CARTESIAN_POINT('Ctrl Pts',(-58.486102814171,45.790366715598,0.));
#91117=CARTESIAN_POINT('Ctrl Pts',(-58.486102814171,45.790366715598,4.));
#91118=CARTESIAN_POINT('Ctrl Pts',(-58.486102814171,45.7903667155981,8.00000000000001));
#91119=CARTESIAN_POINT('Ctrl Pts',(-58.486102814171,45.7903667155981,12.));
#91120=CARTESIAN_POINT('Ctrl Pts',(-58.4060826907379,45.7706564944768,0.));
#91121=CARTESIAN_POINT('Ctrl Pts',(-58.4060826907379,45.7706564944768,4.));
#91122=CARTESIAN_POINT('Ctrl Pts',(-58.4060826907378,45.7706564944768,8.));
#91123=CARTESIAN_POINT('Ctrl Pts',(-58.4060826907378,45.7706564944768,12.));
#91124=CARTESIAN_POINT('',(-58.9211100416396,45.591148170023,0.));
#91125=CARTESIAN_POINT('',(-58.4060826907379,45.7706564944767,0.));
#91126=CARTESIAN_POINT('Ctrl Pts',(-58.9211100416396,45.591148170023,0.));
#91127=CARTESIAN_POINT('Ctrl Pts',(-58.8538661785413,45.6780528262179,0.));
#91128=CARTESIAN_POINT('Ctrl Pts',(-58.7570889974605,45.741658050204,0.));
#91129=CARTESIAN_POINT('Ctrl Pts',(-58.6508283125144,45.7692455126975,0.));
#91130=CARTESIAN_POINT('Ctrl Pts',(-58.5711327988048,45.7899361095676,0.));
#91131=CARTESIAN_POINT('Ctrl Pts',(-58.486102814171,45.790366715598,0.));
#91132=CARTESIAN_POINT('Ctrl Pts',(-58.4060826907379,45.7706564944768,0.));
#91133=CARTESIAN_POINT('',(-58.4060826907378,45.7706564944767,12.));
#91134=CARTESIAN_POINT('Ctrl Pts',(-58.4060826907379,45.7706564944768,0.));
#91135=CARTESIAN_POINT('Ctrl Pts',(-58.4060826907379,45.7706564944768,4.));
#91136=CARTESIAN_POINT('Ctrl Pts',(-58.4060826907378,45.7706564944768,8.));
#91137=CARTESIAN_POINT('Ctrl Pts',(-58.4060826907378,45.7706564944768,12.));
#91138=CARTESIAN_POINT('',(-58.9211100416396,45.5911481700231,12.));
#91139=CARTESIAN_POINT('Ctrl Pts',(-58.4060826907378,45.7706564944768,12.));
#91140=CARTESIAN_POINT('Ctrl Pts',(-58.486102814171,45.7903667155981,12.));
#91141=CARTESIAN_POINT('Ctrl Pts',(-58.5711327988048,45.7899361095676,12.));
#91142=CARTESIAN_POINT('Ctrl Pts',(-58.6508283125143,45.7692455126975,12.));
#91143=CARTESIAN_POINT('Ctrl Pts',(-58.7570889974604,45.7416580502041,12.));
#91144=CARTESIAN_POINT('Ctrl Pts',(-58.8538661785413,45.6780528262179,12.));
#91145=CARTESIAN_POINT('Ctrl Pts',(-58.9211100416396,45.5911481700231,12.));
#91146=CARTESIAN_POINT('Ctrl Pts',(-58.9211100416396,45.5911481700231,12.));
#91147=CARTESIAN_POINT('Ctrl Pts',(-58.9211100416396,45.5911481700231,8.));
#91148=CARTESIAN_POINT('Ctrl Pts',(-58.9211100416396,45.591148170023,4.));
#91149=CARTESIAN_POINT('Ctrl Pts',(-58.9211100416396,45.591148170023,0.));
#91150=CARTESIAN_POINT('Ctrl Pts',(-54.1679505278134,44.3377168516418,0.));
#91151=CARTESIAN_POINT('Ctrl Pts',(-54.1679505278134,44.3377168516418,12.));
#91152=CARTESIAN_POINT('Ctrl Pts',(-54.1714861895278,44.3393235891014,0.));
#91153=CARTESIAN_POINT('Ctrl Pts',(-54.1714861895278,44.3393235891014,12.));
#91154=CARTESIAN_POINT('Ctrl Pts',(-54.1785633257456,44.3425373700829,0.));
#91155=CARTESIAN_POINT('Ctrl Pts',(-54.1785633257456,44.3425373700829,12.));
#91156=CARTESIAN_POINT('Ctrl Pts',(-54.1891964684439,44.3473589597468,0.));
#91157=CARTESIAN_POINT('Ctrl Pts',(-54.1891964684439,44.3473589597468,12.));
#91158=CARTESIAN_POINT('Ctrl Pts',(-54.203408870162,44.3537895823819,0.));
#91159=CARTESIAN_POINT('Ctrl Pts',(-54.203408870162,44.3537895823819,12.));
#91160=CARTESIAN_POINT('Ctrl Pts',(-54.2212325005847,44.3618309103245,0.));
#91161=CARTESIAN_POINT('Ctrl Pts',(-54.2212325005847,44.3618309103245,12.));
#91162=CARTESIAN_POINT('Ctrl Pts',(-54.2391142386354,44.369875253351,0.));
#91163=CARTESIAN_POINT('Ctrl Pts',(-54.2391142386354,44.369875253351,12.));
#91164=CARTESIAN_POINT('Ctrl Pts',(-54.2570540336536,44.3779225430461,0.));
#91165=CARTESIAN_POINT('Ctrl Pts',(-54.2570540336536,44.3779225430461,12.));
#91166=CARTESIAN_POINT('Ctrl Pts',(-54.2750517888695,44.3859726620288,0.));
#91167=CARTESIAN_POINT('Ctrl Pts',(-54.2750517888695,44.3859726620288,12.));
#91168=CARTESIAN_POINT('Ctrl Pts',(-54.2931073621661,44.3940254456427,0.));
#91169=CARTESIAN_POINT('Ctrl Pts',(-54.2931073621661,44.3940254456427,12.));
#91170=CARTESIAN_POINT('Ctrl Pts',(-54.3112205860776,44.4020807028144,0.));
#91171=CARTESIAN_POINT('Ctrl Pts',(-54.3112205860776,44.4020807028144,12.));
#91172=CARTESIAN_POINT('Ctrl Pts',(-54.3293912830237,44.4101382321834,0.));
#91173=CARTESIAN_POINT('Ctrl Pts',(-54.3293912830237,44.4101382321834,12.));
#91174=CARTESIAN_POINT('Ctrl Pts',(-54.347619281931,44.4181978395814,0.));
#91175=CARTESIAN_POINT('Ctrl Pts',(-54.347619281931,44.4181978395814,12.));
#91176=CARTESIAN_POINT('Ctrl Pts',(-54.3659044357064,44.4262593564664,0.));
#91177=CARTESIAN_POINT('Ctrl Pts',(-54.3659044357064,44.4262593564664,12.));
#91178=CARTESIAN_POINT('Ctrl Pts',(-54.3842466156151,44.4343226339555,0.));
#91179=CARTESIAN_POINT('Ctrl Pts',(-54.3842466156151,44.4343226339555,12.));
#91180=CARTESIAN_POINT('Ctrl Pts',(-54.4026457030316,44.442387534098,0.));
#91181=CARTESIAN_POINT('Ctrl Pts',(-54.4026457030316,44.442387534098,12.));
#91182=CARTESIAN_POINT('Ctrl Pts',(-54.4211015825959,44.4504539226336,0.));
#91183=CARTESIAN_POINT('Ctrl Pts',(-54.4211015825959,44.4504539226336,12.));
#91184=CARTESIAN_POINT('Ctrl Pts',(-54.4396141337008,44.4585216599933,0.));
#91185=CARTESIAN_POINT('Ctrl Pts',(-54.4396141337008,44.4585216599933,12.));
#91186=CARTESIAN_POINT('Ctrl Pts',(-54.4581832262072,44.4665905967701,0.));
#91187=CARTESIAN_POINT('Ctrl Pts',(-54.4581832262072,44.4665905967701,12.));
#91188=CARTESIAN_POINT('Ctrl Pts',(-54.4768087248854,44.4746605784056,0.));
#91189=CARTESIAN_POINT('Ctrl Pts',(-54.4768087248854,44.4746605784056,12.));
#91190=CARTESIAN_POINT('Ctrl Pts',(-54.4954904921938,44.482731448127,0.));
#91191=CARTESIAN_POINT('Ctrl Pts',(-54.4954904921938,44.482731448127,12.));
#91192=CARTESIAN_POINT('Ctrl Pts',(-54.5142283914684,44.4908030503209,0.));
#91193=CARTESIAN_POINT('Ctrl Pts',(-54.5142283914684,44.4908030503209,12.));
#91194=CARTESIAN_POINT('Ctrl Pts',(-54.5330222905438,44.4988752343715,0.));
#91195=CARTESIAN_POINT('Ctrl Pts',(-54.5330222905438,44.4988752343715,12.));
#91196=CARTESIAN_POINT('Ctrl Pts',(-54.5518720616016,44.5069478544945,0.));
#91197=CARTESIAN_POINT('Ctrl Pts',(-54.5518720616016,44.5069478544945,12.));
#91198=CARTESIAN_POINT('Ctrl Pts',(-54.5707775794412,44.5150207678988,0.));
#91199=CARTESIAN_POINT('Ctrl Pts',(-54.5707775794412,44.5150207678988,12.));
#91200=CARTESIAN_POINT('Ctrl Pts',(-54.5897387202815,44.5230938335167,0.));
#91201=CARTESIAN_POINT('Ctrl Pts',(-54.5897387202815,44.5230938335167,12.));
#91202=CARTESIAN_POINT('Ctrl Pts',(-54.6087553602914,44.5311669104515,0.));
#91203=CARTESIAN_POINT('Ctrl Pts',(-54.6087553602914,44.5311669104515,12.));
#91204=CARTESIAN_POINT('Ctrl Pts',(-54.6278273743587,44.5392398566802,0.));
#91205=CARTESIAN_POINT('Ctrl Pts',(-54.6278273743587,44.5392398566802,12.));
#91206=CARTESIAN_POINT('Ctrl Pts',(-54.6469546367408,44.5473125297311,0.));
#91207=CARTESIAN_POINT('Ctrl Pts',(-54.6469546367408,44.5473125297311,12.));
#91208=CARTESIAN_POINT('Ctrl Pts',(-54.6661370216252,44.5553847872721,0.));
#91209=CARTESIAN_POINT('Ctrl Pts',(-54.6661370216252,44.5553847872721,12.));
#91210=CARTESIAN_POINT('Ctrl Pts',(-54.6853744036751,44.5634564876863,0.));
#91211=CARTESIAN_POINT('Ctrl Pts',(-54.6853744036751,44.5634564876863,12.));
#91212=CARTESIAN_POINT('Ctrl Pts',(-54.7046666586754,44.5715274907619,0.));
#91213=CARTESIAN_POINT('Ctrl Pts',(-54.7046666586754,44.5715274907619,12.));
#91214=CARTESIAN_POINT('Ctrl Pts',(-54.7240136637717,44.5795976579454,0.));
#91215=CARTESIAN_POINT('Ctrl Pts',(-54.7240136637717,44.5795976579454,12.));
#91216=CARTESIAN_POINT('Ctrl Pts',(-54.7434152971267,44.5876668519661,0.));
#91217=CARTESIAN_POINT('Ctrl Pts',(-54.7434152971267,44.5876668519661,12.));
#91218=CARTESIAN_POINT('Ctrl Pts',(-54.7628714377037,44.5957349366059,0.));
#91219=CARTESIAN_POINT('Ctrl Pts',(-54.7628714377037,44.5957349366059,12.));
#91220=CARTESIAN_POINT('Ctrl Pts',(-54.7823819650149,44.6038017764309,0.));
#91221=CARTESIAN_POINT('Ctrl Pts',(-54.7823819650149,44.6038017764309,12.));
#91222=CARTESIAN_POINT('Ctrl Pts',(-54.8019467588278,44.6118672364906,0.));
#91223=CARTESIAN_POINT('Ctrl Pts',(-54.8019467588278,44.6118672364906,12.));
#91224=CARTESIAN_POINT('Ctrl Pts',(-54.8215656991837,44.6199311823293,0.));
#91225=CARTESIAN_POINT('Ctrl Pts',(-54.8215656991837,44.6199311823293,12.));
#91226=CARTESIAN_POINT('Ctrl Pts',(-54.8412386665276,44.6279934801169,0.));
#91227=CARTESIAN_POINT('Ctrl Pts',(-54.8412386665276,44.6279934801169,12.));
#91228=CARTESIAN_POINT('Ctrl Pts',(-54.860965541796,44.6360539967392,0.));
#91229=CARTESIAN_POINT('Ctrl Pts',(-54.860965541796,44.6360539967392,12.));
#91230=CARTESIAN_POINT('Ctrl Pts',(-54.8807462065164,44.6441125999063,0.));
#91231=CARTESIAN_POINT('Ctrl Pts',(-54.8807462065164,44.6441125999063,12.));
#91232=CARTESIAN_POINT('Ctrl Pts',(-54.9005805428969,44.6521691582533,0.));
#91233=CARTESIAN_POINT('Ctrl Pts',(-54.9005805428969,44.6521691582533,12.));
#91234=CARTESIAN_POINT('Ctrl Pts',(-54.9204684337822,44.6602235412836,0.));
#91235=CARTESIAN_POINT('Ctrl Pts',(-54.9204684337822,44.6602235412836,12.));
#91236=CARTESIAN_POINT('Ctrl Pts',(-54.9404097626077,44.6682756193147,0.));
#91237=CARTESIAN_POINT('Ctrl Pts',(-54.9404097626077,44.6682756193147,12.));
#91238=CARTESIAN_POINT('Ctrl Pts',(-54.9604044133501,44.6763252634258,0.));
#91239=CARTESIAN_POINT('Ctrl Pts',(-54.9604044133501,44.6763252634258,12.));
#91240=CARTESIAN_POINT('Ctrl Pts',(-54.9804522704686,44.6843723454,0.));
#91241=CARTESIAN_POINT('Ctrl Pts',(-54.9804522704686,44.6843723454,12.));
#91242=CARTESIAN_POINT('Ctrl Pts',(-55.0005532188667,44.6924167376869,0.));
#91243=CARTESIAN_POINT('Ctrl Pts',(-55.0005532188667,44.6924167376869,12.));
#91244=CARTESIAN_POINT('Ctrl Pts',(-55.0207071439237,44.7004583134249,0.));
#91245=CARTESIAN_POINT('Ctrl Pts',(-55.0207071439237,44.7004583134249,12.));
#91246=CARTESIAN_POINT('Ctrl Pts',(-55.0409139315078,44.7084969464513,0.));
#91247=CARTESIAN_POINT('Ctrl Pts',(-55.0409139315078,44.7084969464513,12.));
#91248=CARTESIAN_POINT('Ctrl Pts',(-55.0611734679894,44.7165325113159,0.));
#91249=CARTESIAN_POINT('Ctrl Pts',(-55.0611734679894,44.7165325113159,12.));
#91250=CARTESIAN_POINT('Ctrl Pts',(-55.0814856402496,44.7245648832979,0.));
#91251=CARTESIAN_POINT('Ctrl Pts',(-55.0814856402496,44.7245648832979,12.));
#91252=CARTESIAN_POINT('Ctrl Pts',(-55.1018503356796,44.7325939384035,0.));
#91253=CARTESIAN_POINT('Ctrl Pts',(-55.1018503356796,44.7325939384035,12.));
#91254=CARTESIAN_POINT('Ctrl Pts',(-55.1222674421743,44.740619553348,0.));
#91255=CARTESIAN_POINT('Ctrl Pts',(-55.1222674421743,44.740619553348,12.));
#91256=CARTESIAN_POINT('Ctrl Pts',(-55.14273684812,44.748641605542,0.));
#91257=CARTESIAN_POINT('Ctrl Pts',(-55.14273684812,44.748641605542,12.));
#91258=CARTESIAN_POINT('Ctrl Pts',(-55.1632584423815,44.7566599730773,0.));
#91259=CARTESIAN_POINT('Ctrl Pts',(-55.1632584423815,44.7566599730773,12.));
#91260=CARTESIAN_POINT('Ctrl Pts',(-55.1838321142779,44.7646745347109,0.));
#91261=CARTESIAN_POINT('Ctrl Pts',(-55.1838321142779,44.7646745347109,12.));
#91262=CARTESIAN_POINT('Ctrl Pts',(-55.2044577535866,44.7726851698619,0.));
#91263=CARTESIAN_POINT('Ctrl Pts',(-55.2044577535866,44.7726851698619,12.));
#91264=CARTESIAN_POINT('Ctrl Pts',(-55.2251352505475,44.7806917586077,0.));
#91265=CARTESIAN_POINT('Ctrl Pts',(-55.2251352505475,44.7806917586077,12.));
#91266=CARTESIAN_POINT('Ctrl Pts',(-55.2458644958617,44.7886941816823,0.));
#91267=CARTESIAN_POINT('Ctrl Pts',(-55.2458644958617,44.7886941816823,12.));
#91268=CARTESIAN_POINT('Ctrl Pts',(-55.2666453806883,44.7966923204741,0.));
#91269=CARTESIAN_POINT('Ctrl Pts',(-55.2666453806883,44.7966923204741,12.));
#91270=CARTESIAN_POINT('Ctrl Pts',(-55.287477796635,44.8046860570245,0.));
#91271=CARTESIAN_POINT('Ctrl Pts',(-55.287477796635,44.8046860570245,12.));
#91272=CARTESIAN_POINT('Ctrl Pts',(-55.3083616357605,44.812675274021,0.));
#91273=CARTESIAN_POINT('Ctrl Pts',(-55.3083616357605,44.812675274021,12.));
#91274=CARTESIAN_POINT('Ctrl Pts',(-55.3292967905726,44.8206598547889,0.));
#91275=CARTESIAN_POINT('Ctrl Pts',(-55.3292967905726,44.8206598547889,12.));
#91276=CARTESIAN_POINT('Ctrl Pts',(-55.350283154023,44.8286396832849,0.));
#91277=CARTESIAN_POINT('Ctrl Pts',(-55.350283154023,44.8286396832849,12.));
#91278=CARTESIAN_POINT('Ctrl Pts',(-55.3713206194962,44.8366146440896,0.));
#91279=CARTESIAN_POINT('Ctrl Pts',(-55.3713206194962,44.8366146440896,12.));
#91280=CARTESIAN_POINT('Ctrl Pts',(-55.3924090808002,44.8445846224034,0.));
#91281=CARTESIAN_POINT('Ctrl Pts',(-55.3924090808002,44.8445846224034,12.));
#91282=CARTESIAN_POINT('Ctrl Pts',(-55.4135484321706,44.8525495040397,0.));
#91283=CARTESIAN_POINT('Ctrl Pts',(-55.4135484321706,44.8525495040397,12.));
#91284=CARTESIAN_POINT('Ctrl Pts',(-55.4347385682697,44.8605091754208,0.));
#91285=CARTESIAN_POINT('Ctrl Pts',(-55.4347385682697,44.8605091754208,12.));
#91286=CARTESIAN_POINT('Ctrl Pts',(-55.4559793841838,44.8684635235727,0.));
#91287=CARTESIAN_POINT('Ctrl Pts',(-55.4559793841838,44.8684635235727,12.));
#91288=CARTESIAN_POINT('Ctrl Pts',(-55.4772707754139,44.8764124361218,0.));
#91289=CARTESIAN_POINT('Ctrl Pts',(-55.4772707754139,44.8764124361218,12.));
#91290=CARTESIAN_POINT('Ctrl Pts',(-55.4986126378676,44.8843558012903,0.));
#91291=CARTESIAN_POINT('Ctrl Pts',(-55.4986126378676,44.8843558012903,12.));
#91292=CARTESIAN_POINT('Ctrl Pts',(-55.5200048678648,44.8922935078905,0.));
#91293=CARTESIAN_POINT('Ctrl Pts',(-55.5200048678648,44.8922935078905,12.));
#91294=CARTESIAN_POINT('Ctrl Pts',(-55.541447362135,44.9002254453192,0.));
#91295=CARTESIAN_POINT('Ctrl Pts',(-55.541447362135,44.9002254453192,12.));
#91296=CARTESIAN_POINT('Ctrl Pts',(-55.5629400178136,44.9081515035525,0.));
#91297=CARTESIAN_POINT('Ctrl Pts',(-55.5629400178136,44.9081515035525,12.));
#91298=CARTESIAN_POINT('Ctrl Pts',(-55.5844827324315,44.9160715731425,0.));
#91299=CARTESIAN_POINT('Ctrl Pts',(-55.5844827324315,44.9160715731425,12.));
#91300=CARTESIAN_POINT('Ctrl Pts',(-55.6060754039089,44.9239855452119,0.));
#91301=CARTESIAN_POINT('Ctrl Pts',(-55.6060754039089,44.9239855452119,12.));
#91302=CARTESIAN_POINT('Ctrl Pts',(-55.6277179305604,44.9318933114483,0.));
#91303=CARTESIAN_POINT('Ctrl Pts',(-55.6277179305604,44.9318933114483,12.));
#91304=CARTESIAN_POINT('Ctrl Pts',(-55.6494102110922,44.9397947640996,0.));
#91305=CARTESIAN_POINT('Ctrl Pts',(-55.6494102110922,44.9397947640996,12.));
#91306=CARTESIAN_POINT('Ctrl Pts',(-55.671152144599,44.9476897959694,0.));
#91307=CARTESIAN_POINT('Ctrl Pts',(-55.671152144599,44.9476897959694,12.));
#91308=CARTESIAN_POINT('Ctrl Pts',(-55.6929436305522,44.9555783004133,0.));
#91309=CARTESIAN_POINT('Ctrl Pts',(-55.6929436305522,44.9555783004133,12.));
#91310=CARTESIAN_POINT('Ctrl Pts',(-55.7147845687969,44.9634601713352,0.));
#91311=CARTESIAN_POINT('Ctrl Pts',(-55.7147845687969,44.9634601713352,12.));
#91312=CARTESIAN_POINT('Ctrl Pts',(-55.7366748595582,44.9713353031827,0.));
#91313=CARTESIAN_POINT('Ctrl Pts',(-55.7366748595582,44.9713353031827,12.));
#91314=CARTESIAN_POINT('Ctrl Pts',(-55.7586144034376,44.979203590942,0.));
#91315=CARTESIAN_POINT('Ctrl Pts',(-55.7586144034376,44.979203590942,12.));
#91316=CARTESIAN_POINT('Ctrl Pts',(-55.7806031014093,44.9870649301333,0.));
#91317=CARTESIAN_POINT('Ctrl Pts',(-55.7806031014093,44.9870649301333,12.));
#91318=CARTESIAN_POINT('Ctrl Pts',(-55.8026408548078,44.9949192168073,0.));
#91319=CARTESIAN_POINT('Ctrl Pts',(-55.8026408548078,44.9949192168073,12.));
#91320=CARTESIAN_POINT('Ctrl Pts',(-55.8247275653257,45.002766347541,0.));
#91321=CARTESIAN_POINT('Ctrl Pts',(-55.8247275653257,45.002766347541,12.));
#91322=CARTESIAN_POINT('Ctrl Pts',(-55.8468631350195,45.0106062194325,0.));
#91323=CARTESIAN_POINT('Ctrl Pts',(-55.8468631350195,45.0106062194325,12.));
#91324=CARTESIAN_POINT('Ctrl Pts',(-55.8690474663058,45.0184387300968,0.));
#91325=CARTESIAN_POINT('Ctrl Pts',(-55.8690474663058,45.0184387300968,12.));
#91326=CARTESIAN_POINT('Ctrl Pts',(-55.8912804619588,45.0262637776623,0.));
#91327=CARTESIAN_POINT('Ctrl Pts',(-55.8912804619588,45.0262637776623,12.));
#91328=CARTESIAN_POINT('Ctrl Pts',(-55.9135620250977,45.0340812607676,0.));
#91329=CARTESIAN_POINT('Ctrl Pts',(-55.9135620250977,45.0340812607676,12.));
#91330=CARTESIAN_POINT('Ctrl Pts',(-55.9358920591861,45.041891078557,0.));
#91331=CARTESIAN_POINT('Ctrl Pts',(-55.9358920591861,45.041891078557,12.));
#91332=CARTESIAN_POINT('Ctrl Pts',(-55.958270468037,45.0496931306766,0.));
#91333=CARTESIAN_POINT('Ctrl Pts',(-55.958270468037,45.0496931306766,12.));
#91334=CARTESIAN_POINT('Ctrl Pts',(-55.9806971558099,45.0574873172696,0.));
#91335=CARTESIAN_POINT('Ctrl Pts',(-55.9806971558099,45.0574873172696,12.));
#91336=CARTESIAN_POINT('Ctrl Pts',(-56.0031720270074,45.0652735389729,0.));
#91337=CARTESIAN_POINT('Ctrl Pts',(-56.0031720270074,45.0652735389729,12.));
#91338=CARTESIAN_POINT('Ctrl Pts',(-56.025694986463,45.0730516969142,0.));
#91339=CARTESIAN_POINT('Ctrl Pts',(-56.025694986463,45.0730516969142,12.));
#91340=CARTESIAN_POINT('Ctrl Pts',(-56.0482659393412,45.0808216927082,0.));
#91341=CARTESIAN_POINT('Ctrl Pts',(-56.0482659393412,45.0808216927082,12.));
#91342=CARTESIAN_POINT('Ctrl Pts',(-56.070884791141,45.0885834284513,0.));
#91343=CARTESIAN_POINT('Ctrl Pts',(-56.070884791141,45.0885834284513,12.));
#91344=CARTESIAN_POINT('Ctrl Pts',(-56.0935514476945,45.0963368067177,0.));
#91345=CARTESIAN_POINT('Ctrl Pts',(-56.0935514476945,45.0963368067177,12.));
#91346=CARTESIAN_POINT('Ctrl Pts',(-56.1162658151621,45.1040817305563,0.));
#91347=CARTESIAN_POINT('Ctrl Pts',(-56.1162658151621,45.1040817305563,12.));
#91348=CARTESIAN_POINT('Ctrl Pts',(-56.1390278000226,45.1118181034888,0.));
#91349=CARTESIAN_POINT('Ctrl Pts',(-56.1390278000226,45.1118181034888,12.));
#91350=CARTESIAN_POINT('Ctrl Pts',(-56.1618373090729,45.119545829506,0.));
#91351=CARTESIAN_POINT('Ctrl Pts',(-56.1618373090729,45.119545829506,12.));
#91352=CARTESIAN_POINT('Ctrl Pts',(-56.1846942494321,45.1272648130627,0.));
#91353=CARTESIAN_POINT('Ctrl Pts',(-56.1846942494321,45.1272648130627,12.));
#91354=CARTESIAN_POINT('Ctrl Pts',(-56.2075985285391,45.1349749590736,0.));
#91355=CARTESIAN_POINT('Ctrl Pts',(-56.2075985285391,45.1349749590736,12.));
#91356=CARTESIAN_POINT('Ctrl Pts',(-56.2305500541491,45.1426761729107,0.));
#91357=CARTESIAN_POINT('Ctrl Pts',(-56.2305500541491,45.1426761729107,12.));
#91358=CARTESIAN_POINT('Ctrl Pts',(-56.2535487343227,45.150368360401,0.));
#91359=CARTESIAN_POINT('Ctrl Pts',(-56.2535487343227,45.150368360401,12.));
#91360=CARTESIAN_POINT('Ctrl Pts',(-56.2765944774252,45.158051427823,0.));
#91361=CARTESIAN_POINT('Ctrl Pts',(-56.2765944774252,45.158051427823,12.));
#91362=CARTESIAN_POINT('Ctrl Pts',(-56.2996871921321,45.1657252819018,0.));
#91363=CARTESIAN_POINT('Ctrl Pts',(-56.2996871921321,45.1657252819018,12.));
#91364=CARTESIAN_POINT('Ctrl Pts',(-56.3228267874265,45.1733898298062,0.));
#91365=CARTESIAN_POINT('Ctrl Pts',(-56.3228267874265,45.1733898298062,12.));
#91366=CARTESIAN_POINT('Ctrl Pts',(-56.3460131725962,45.1810449791451,0.));
#91367=CARTESIAN_POINT('Ctrl Pts',(-56.3460131725962,45.1810449791451,12.));
#91368=CARTESIAN_POINT('Ctrl Pts',(-56.3692462572228,45.1886906379664,0.));
#91369=CARTESIAN_POINT('Ctrl Pts',(-56.3692462572228,45.1886906379664,12.));
#91370=CARTESIAN_POINT('Ctrl Pts',(-56.3925259511804,45.1963267147527,0.));
#91371=CARTESIAN_POINT('Ctrl Pts',(-56.3925259511804,45.1963267147527,12.));
#91372=CARTESIAN_POINT('Ctrl Pts',(-56.4158521646412,45.2039531184172,0.));
#91373=CARTESIAN_POINT('Ctrl Pts',(-56.4158521646412,45.2039531184172,12.));
#91374=CARTESIAN_POINT('Ctrl Pts',(-56.4392248080733,45.2115697583002,0.));
#91375=CARTESIAN_POINT('Ctrl Pts',(-56.4392248080733,45.2115697583002,12.));
#91376=CARTESIAN_POINT('Ctrl Pts',(-56.4626437922385,45.2191765441666,0.));
#91377=CARTESIAN_POINT('Ctrl Pts',(-56.4626437922385,45.2191765441666,12.));
#91378=CARTESIAN_POINT('Ctrl Pts',(-56.4861090281819,45.2267733862046,0.));
#91379=CARTESIAN_POINT('Ctrl Pts',(-56.4861090281819,45.2267733862046,12.));
#91380=CARTESIAN_POINT('Ctrl Pts',(-56.5096204272299,45.2343601950222,0.));
#91381=CARTESIAN_POINT('Ctrl Pts',(-56.5096204272299,45.2343601950222,12.));
#91382=CARTESIAN_POINT('Ctrl Pts',(-56.533177900995,45.2419368816423,0.));
#91383=CARTESIAN_POINT('Ctrl Pts',(-56.533177900995,45.2419368816423,12.));
#91384=CARTESIAN_POINT('Ctrl Pts',(-56.5567813613752,45.2495033574997,0.));
#91385=CARTESIAN_POINT('Ctrl Pts',(-56.5567813613752,45.2495033574997,12.));
#91386=CARTESIAN_POINT('Ctrl Pts',(-56.5804307205507,45.2570595344382,0.));
#91387=CARTESIAN_POINT('Ctrl Pts',(-56.5804307205507,45.2570595344382,12.));
#91388=CARTESIAN_POINT('Ctrl Pts',(-56.604125890975,45.2646053247094,0.));
#91389=CARTESIAN_POINT('Ctrl Pts',(-56.604125890975,45.2646053247094,12.));
#91390=CARTESIAN_POINT('Ctrl Pts',(-56.6278667853716,45.2721406409706,0.));
#91391=CARTESIAN_POINT('Ctrl Pts',(-56.6278667853716,45.2721406409706,12.));
#91392=CARTESIAN_POINT('Ctrl Pts',(-56.6516533167398,45.2796653962796,0.));
#91393=CARTESIAN_POINT('Ctrl Pts',(-56.6516533167398,45.2796653962796,12.));
#91394=CARTESIAN_POINT('Ctrl Pts',(-56.6754853983535,45.2871795040912,0.));
#91395=CARTESIAN_POINT('Ctrl Pts',(-56.6754853983535,45.2871795040912,12.));
#91396=CARTESIAN_POINT('Ctrl Pts',(-56.6993629437596,45.2946828782557,0.));
#91397=CARTESIAN_POINT('Ctrl Pts',(-56.6993629437596,45.2946828782557,12.));
#91398=CARTESIAN_POINT('Ctrl Pts',(-56.7232858667697,45.3021754330169,0.));
#91399=CARTESIAN_POINT('Ctrl Pts',(-56.7232858667697,45.3021754330169,12.));
#91400=CARTESIAN_POINT('Ctrl Pts',(-56.747254081454,45.3096570830107,0.));
#91401=CARTESIAN_POINT('Ctrl Pts',(-56.747254081454,45.3096570830107,12.));
#91402=CARTESIAN_POINT('Ctrl Pts',(-56.771267502148,45.3171277432592,0.));
#91403=CARTESIAN_POINT('Ctrl Pts',(-56.771267502148,45.3171277432592,12.));
#91404=CARTESIAN_POINT('Ctrl Pts',(-56.7953260434521,45.3245873291682,0.));
#91405=CARTESIAN_POINT('Ctrl Pts',(-56.7953260434521,45.3245873291682,12.));
#91406=CARTESIAN_POINT('Ctrl Pts',(-56.8194296202293,45.3320357565241,0.));
#91407=CARTESIAN_POINT('Ctrl Pts',(-56.8194296202293,45.3320357565241,12.));
#91408=CARTESIAN_POINT('Ctrl Pts',(-56.8435781475982,45.3394729414932,0.));
#91409=CARTESIAN_POINT('Ctrl Pts',(-56.8435781475982,45.3394729414932,12.));
#91410=CARTESIAN_POINT('Ctrl Pts',(-56.8677715409266,45.3468988006202,0.));
#91411=CARTESIAN_POINT('Ctrl Pts',(-56.8677715409266,45.3468988006202,12.));
#91412=CARTESIAN_POINT('Ctrl Pts',(-56.8920097158371,45.3543132508234,0.));
#91413=CARTESIAN_POINT('Ctrl Pts',(-56.8920097158371,45.3543132508234,12.));
#91414=CARTESIAN_POINT('Ctrl Pts',(-56.916292588208,45.3617162093918,0.));
#91415=CARTESIAN_POINT('Ctrl Pts',(-56.916292588208,45.3617162093918,12.));
#91416=CARTESIAN_POINT('Ctrl Pts',(-56.9406200741714,45.3691075939827,0.));
#91417=CARTESIAN_POINT('Ctrl Pts',(-56.9406200741714,45.3691075939827,12.));
#91418=CARTESIAN_POINT('Ctrl Pts',(-56.9649920901079,45.3764873226202,0.));
#91419=CARTESIAN_POINT('Ctrl Pts',(-56.9649920901079,45.3764873226202,12.));
#91420=CARTESIAN_POINT('Ctrl Pts',(-56.9894085526383,45.3838553136957,0.));
#91421=CARTESIAN_POINT('Ctrl Pts',(-56.9894085526383,45.3838553136957,12.));
#91422=CARTESIAN_POINT('Ctrl Pts',(-57.0138693786287,45.3912114859625,0.));
#91423=CARTESIAN_POINT('Ctrl Pts',(-57.0138693786287,45.3912114859625,12.));
#91424=CARTESIAN_POINT('Ctrl Pts',(-57.0383744851917,45.3985557585316,0.));
#91425=CARTESIAN_POINT('Ctrl Pts',(-57.0383744851917,45.3985557585316,12.));
#91426=CARTESIAN_POINT('Ctrl Pts',(-57.0629237896848,45.4058880508693,0.));
#91427=CARTESIAN_POINT('Ctrl Pts',(-57.0629237896848,45.4058880508693,12.));
#91428=CARTESIAN_POINT('Ctrl Pts',(-57.0875172097048,45.4132082827945,0.));
#91429=CARTESIAN_POINT('Ctrl Pts',(-57.0875172097048,45.4132082827945,12.));
#91430=CARTESIAN_POINT('Ctrl Pts',(-57.1121546630776,45.4205163744778,0.));
#91431=CARTESIAN_POINT('Ctrl Pts',(-57.1121546630776,45.4205163744778,12.));
#91432=CARTESIAN_POINT('Ctrl Pts',(-57.1368360678629,45.4278122464387,0.));
#91433=CARTESIAN_POINT('Ctrl Pts',(-57.1368360678629,45.4278122464387,12.));
#91434=CARTESIAN_POINT('Ctrl Pts',(-57.1615613423586,45.4350958195434,0.));
#91435=CARTESIAN_POINT('Ctrl Pts',(-57.1615613423586,45.4350958195434,12.));
#91436=CARTESIAN_POINT('Ctrl Pts',(-57.1863304051011,45.4423670150035,0.));
#91437=CARTESIAN_POINT('Ctrl Pts',(-57.1863304051011,45.4423670150035,12.));
#91438=CARTESIAN_POINT('Ctrl Pts',(-57.2111431748629,45.4496257543759,0.));
#91439=CARTESIAN_POINT('Ctrl Pts',(-57.2111431748629,45.4496257543759,12.));
#91440=CARTESIAN_POINT('Ctrl Pts',(-57.2359995706441,45.4568719595639,0.));
#91441=CARTESIAN_POINT('Ctrl Pts',(-57.2359995706441,45.4568719595639,12.));
#91442=CARTESIAN_POINT('Ctrl Pts',(-57.2608995116727,45.4641055528138,0.));
#91443=CARTESIAN_POINT('Ctrl Pts',(-57.2608995116727,45.4641055528138,12.));
#91444=CARTESIAN_POINT('Ctrl Pts',(-57.2858429174056,45.4713264567059,0.));
#91445=CARTESIAN_POINT('Ctrl Pts',(-57.2858429174056,45.4713264567059,12.));
#91446=CARTESIAN_POINT('Ctrl Pts',(-57.3108297075262,45.4785345941505,0.));
#91447=CARTESIAN_POINT('Ctrl Pts',(-57.3108297075262,45.4785345941505,12.));
#91448=CARTESIAN_POINT('Ctrl Pts',(-57.3358598019391,45.4857298883826,0.));
#91449=CARTESIAN_POINT('Ctrl Pts',(-57.3358598019391,45.4857298883826,12.));
#91450=CARTESIAN_POINT('Ctrl Pts',(-57.360933120758,45.4929122629576,0.));
#91451=CARTESIAN_POINT('Ctrl Pts',(-57.360933120758,45.4929122629576,12.));
#91452=CARTESIAN_POINT('Ctrl Pts',(-57.3860495843043,45.5000816417516,0.));
#91453=CARTESIAN_POINT('Ctrl Pts',(-57.3860495843043,45.5000816417516,12.));
#91454=CARTESIAN_POINT('Ctrl Pts',(-57.4112091131193,45.5072379489637,0.));
#91455=CARTESIAN_POINT('Ctrl Pts',(-57.4112091131193,45.5072379489637,12.));
#91456=CARTESIAN_POINT('Ctrl Pts',(-57.4364116279708,45.5143811091209,0.));
#91457=CARTESIAN_POINT('Ctrl Pts',(-57.4364116279708,45.5143811091209,12.));
#91458=CARTESIAN_POINT('Ctrl Pts',(-57.4616570498566,45.5215110470825,0.));
#91459=CARTESIAN_POINT('Ctrl Pts',(-57.4616570498566,45.5215110470825,12.));
#91460=CARTESIAN_POINT('Ctrl Pts',(-57.4869453000055,45.5286276880479,0.));
#91461=CARTESIAN_POINT('Ctrl Pts',(-57.4869453000055,45.5286276880479,12.));
#91462=CARTESIAN_POINT('Ctrl Pts',(-57.5122762998732,45.5357309575603,0.));
#91463=CARTESIAN_POINT('Ctrl Pts',(-57.5122762998732,45.5357309575603,12.));
#91464=CARTESIAN_POINT('Ctrl Pts',(-57.5376499711338,45.5428207814832,0.));
#91465=CARTESIAN_POINT('Ctrl Pts',(-57.5376499711338,45.5428207814832,12.));
#91466=CARTESIAN_POINT('Ctrl Pts',(-57.5630662356671,45.5498970859829,0.));
#91467=CARTESIAN_POINT('Ctrl Pts',(-57.5630662356671,45.5498970859829,12.));
#91468=CARTESIAN_POINT('Ctrl Pts',(-57.5885250155432,45.5569597975096,0.));
#91469=CARTESIAN_POINT('Ctrl Pts',(-57.5885250155432,45.5569597975096,12.));
#91470=CARTESIAN_POINT('Ctrl Pts',(-57.6140262330048,45.5640088427819,0.));
#91471=CARTESIAN_POINT('Ctrl Pts',(-57.6140262330048,45.5640088427819,12.));
#91472=CARTESIAN_POINT('Ctrl Pts',(-57.6395698104416,45.5710441487683,0.));
#91473=CARTESIAN_POINT('Ctrl Pts',(-57.6395698104416,45.5710441487683,12.));
#91474=CARTESIAN_POINT('Ctrl Pts',(-57.6651556704249,45.5780656427172,0.));
#91475=CARTESIAN_POINT('Ctrl Pts',(-57.6651556704249,45.5780656427172,12.));
#91476=CARTESIAN_POINT('Ctrl Pts',(-57.6907837357425,45.5850732521902,0.));
#91477=CARTESIAN_POINT('Ctrl Pts',(-57.6907837357425,45.5850732521902,12.));
#91478=CARTESIAN_POINT('Ctrl Pts',(-57.7164539294316,45.5920669050988,0.));
#91479=CARTESIAN_POINT('Ctrl Pts',(-57.7164539294316,45.5920669050988,12.));
#91480=CARTESIAN_POINT('Ctrl Pts',(-57.7421661748022,45.5990465297341,0.));
#91481=CARTESIAN_POINT('Ctrl Pts',(-57.7421661748022,45.5990465297341,12.));
#91482=CARTESIAN_POINT('Ctrl Pts',(-57.7679203954735,45.6060120548199,0.));
#91483=CARTESIAN_POINT('Ctrl Pts',(-57.7679203954735,45.6060120548199,12.));
#91484=CARTESIAN_POINT('Ctrl Pts',(-57.7937165153379,45.6129634094677,0.));
#91485=CARTESIAN_POINT('Ctrl Pts',(-57.7937165153379,45.6129634094677,12.));
#91486=CARTESIAN_POINT('Ctrl Pts',(-57.819554458484,45.619900523078,0.));
#91487=CARTESIAN_POINT('Ctrl Pts',(-57.819554458484,45.619900523078,12.));
#91488=CARTESIAN_POINT('Ctrl Pts',(-57.8454341491236,45.6268233252543,0.));
#91489=CARTESIAN_POINT('Ctrl Pts',(-57.8454341491236,45.6268233252543,12.));
#91490=CARTESIAN_POINT('Ctrl Pts',(-57.8713555115232,45.6337317457253,0.));
#91491=CARTESIAN_POINT('Ctrl Pts',(-57.8713555115232,45.6337317457253,12.));
#91492=CARTESIAN_POINT('Ctrl Pts',(-57.8973184699037,45.6406257142385,0.));
#91493=CARTESIAN_POINT('Ctrl Pts',(-57.8973184699037,45.6406257142385,12.));
#91494=CARTESIAN_POINT('Ctrl Pts',(-57.923322948432,45.6475051605542,0.));
#91495=CARTESIAN_POINT('Ctrl Pts',(-57.923322948432,45.6475051605542,12.));
#91496=CARTESIAN_POINT('Ctrl Pts',(-57.9493688714249,45.6543700146689,0.));
#91497=CARTESIAN_POINT('Ctrl Pts',(-57.9493688714249,45.6543700146689,12.));
#91498=CARTESIAN_POINT('Ctrl Pts',(-57.975456163507,45.6612202069927,0.));
#91499=CARTESIAN_POINT('Ctrl Pts',(-57.975456163507,45.6612202069927,12.));
#91500=CARTESIAN_POINT('Ctrl Pts',(-58.0015847497838,45.6680556685494,0.));
#91501=CARTESIAN_POINT('Ctrl Pts',(-58.0015847497838,45.6680556685494,12.));
#91502=CARTESIAN_POINT('Ctrl Pts',(-58.0277545560001,45.6748763311635,0.));
#91503=CARTESIAN_POINT('Ctrl Pts',(-58.0277545560001,45.6748763311635,12.));
#91504=CARTESIAN_POINT('Ctrl Pts',(-58.0539655087095,45.6816821276662,0.));
#91505=CARTESIAN_POINT('Ctrl Pts',(-58.0539655087095,45.6816821276662,12.));
#91506=CARTESIAN_POINT('Ctrl Pts',(-58.0802175348939,45.6884729914465,0.));
#91507=CARTESIAN_POINT('Ctrl Pts',(-58.0802175348939,45.6884729914465,12.));
#91508=CARTESIAN_POINT('Ctrl Pts',(-58.1065105615884,45.6952488560133,0.));
#91509=CARTESIAN_POINT('Ctrl Pts',(-58.1065105615884,45.6952488560133,12.));
#91510=CARTESIAN_POINT('Ctrl Pts',(-58.1328445154667,45.7020096545174,0.));
#91511=CARTESIAN_POINT('Ctrl Pts',(-58.1328445154667,45.7020096545174,12.));
#91512=CARTESIAN_POINT('Ctrl Pts',(-58.159219322515,45.708755319378,0.));
#91513=CARTESIAN_POINT('Ctrl Pts',(-58.159219322515,45.708755319378,12.));
#91514=CARTESIAN_POINT('Ctrl Pts',(-58.1856349074723,45.7154857816507,0.));
#91515=CARTESIAN_POINT('Ctrl Pts',(-58.1856349074723,45.7154857816507,12.));
#91516=CARTESIAN_POINT('Ctrl Pts',(-58.2120911942819,45.7222009715431,0.));
#91517=CARTESIAN_POINT('Ctrl Pts',(-58.2120911942819,45.7222009715431,12.));
#91518=CARTESIAN_POINT('Ctrl Pts',(-58.2385881070959,45.7289008195612,0.));
#91519=CARTESIAN_POINT('Ctrl Pts',(-58.2385881070959,45.7289008195612,12.));
#91520=CARTESIAN_POINT('Ctrl Pts',(-58.2651255711481,45.7355852575127,0.));
#91521=CARTESIAN_POINT('Ctrl Pts',(-58.2651255711481,45.7355852575127,12.));
#91522=CARTESIAN_POINT('Ctrl Pts',(-58.2917035135833,45.7422542194625,0.));
#91523=CARTESIAN_POINT('Ctrl Pts',(-58.2917035135833,45.7422542194625,12.));
#91524=CARTESIAN_POINT('Ctrl Pts',(-58.3183218645265,45.7489076429725,0.));
#91525=CARTESIAN_POINT('Ctrl Pts',(-58.3183218645265,45.7489076429725,12.));
#91526=CARTESIAN_POINT('Ctrl Pts',(-58.3449805573335,45.7555454693956,0.));
#91527=CARTESIAN_POINT('Ctrl Pts',(-58.3449805573335,45.7555454693956,12.));
#91528=CARTESIAN_POINT('Ctrl Pts',(-58.3716795262251,45.762167641136,0.));
#91529=CARTESIAN_POINT('Ctrl Pts',(-58.3716795262251,45.762167641136,12.));
#91530=CARTESIAN_POINT('Ctrl Pts',(-58.3984187044166,45.7687740994899,0.));
#91531=CARTESIAN_POINT('Ctrl Pts',(-58.3984187044166,45.7687740994899,12.));
#91532=CARTESIAN_POINT('Ctrl Pts',(-58.4251980219532,45.77536478215,0.));
#91533=CARTESIAN_POINT('Ctrl Pts',(-58.4251980219532,45.77536478215,12.));
#91534=CARTESIAN_POINT('Ctrl Pts',(-58.4520174038836,45.7819396211062,0.));
#91535=CARTESIAN_POINT('Ctrl Pts',(-58.4520174038836,45.7819396211062,12.));
#91536=CARTESIAN_POINT('Ctrl Pts',(-58.4788767677114,45.7884985397138,0.));
#91537=CARTESIAN_POINT('Ctrl Pts',(-58.4788767677114,45.7884985397138,12.));
#91538=CARTESIAN_POINT('Ctrl Pts',(-58.5057760270407,45.7950414569431,0.));
#91539=CARTESIAN_POINT('Ctrl Pts',(-58.5057760270407,45.7950414569431,12.));
#91540=CARTESIAN_POINT('Ctrl Pts',(-58.5327150960874,45.801568292618,0.));
#91541=CARTESIAN_POINT('Ctrl Pts',(-58.5327150960874,45.801568292618,12.));
#91542=CARTESIAN_POINT('Ctrl Pts',(-58.5596938940308,45.8080789725167,0.));
#91543=CARTESIAN_POINT('Ctrl Pts',(-58.5596938940308,45.8080789725167,12.));
#91544=CARTESIAN_POINT('Ctrl Pts',(-58.5867123490943,45.8145734330666,0.));
#91545=CARTESIAN_POINT('Ctrl Pts',(-58.5867123490943,45.8145734330666,12.));
#91546=CARTESIAN_POINT('Ctrl Pts',(-58.6137704035561,45.8210516273556,0.));
#91547=CARTESIAN_POINT('Ctrl Pts',(-58.6137704035561,45.8210516273556,12.));
#91548=CARTESIAN_POINT('Ctrl Pts',(-58.64086801535,45.8275135263874,0.));
#91549=CARTESIAN_POINT('Ctrl Pts',(-58.64086801535,45.8275135263874,12.));
#91550=CARTESIAN_POINT('Ctrl Pts',(-58.668005155216,45.8339591141396,0.));
#91551=CARTESIAN_POINT('Ctrl Pts',(-58.668005155216,45.8339591141396,12.));
#91552=CARTESIAN_POINT('Ctrl Pts',(-58.6897464750196,45.8391025301766,0.));
#91553=CARTESIAN_POINT('Ctrl Pts',(-58.6897464750196,45.8391025301766,12.));
#91554=CARTESIAN_POINT('Ctrl Pts',(-58.7060702401382,45.8429527488565,0.));
#91555=CARTESIAN_POINT('Ctrl Pts',(-58.7060702401382,45.8429527488565,12.));
#91556=CARTESIAN_POINT('Ctrl Pts',(-58.7169606500157,45.8455162977347,0.));
#91557=CARTESIAN_POINT('Ctrl Pts',(-58.7169606500157,45.8455162977347,12.));
#91558=CARTESIAN_POINT('Ctrl Pts',(-58.722407829904,45.8467972562798,0.));
#91559=CARTESIAN_POINT('Ctrl Pts',(-58.722407829904,45.8467972562798,12.));
#91560=CARTESIAN_POINT('',(-54.1679505278134,44.3377168516418,0.));
#91561=CARTESIAN_POINT('Ctrl Pts',(-54.1679505278134,44.3377168516418,0.));
#91562=CARTESIAN_POINT('Ctrl Pts',(-54.1714861895278,44.3393235891014,0.));
#91563=CARTESIAN_POINT('Ctrl Pts',(-54.1785633257456,44.3425373700829,0.));
#91564=CARTESIAN_POINT('Ctrl Pts',(-54.1891964684439,44.3473589597468,0.));
#91565=CARTESIAN_POINT('Ctrl Pts',(-54.203408870162,44.3537895823819,0.));
#91566=CARTESIAN_POINT('Ctrl Pts',(-54.2212325005847,44.3618309103245,0.));
#91567=CARTESIAN_POINT('Ctrl Pts',(-54.2391142386354,44.369875253351,0.));
#91568=CARTESIAN_POINT('Ctrl Pts',(-54.2570540336536,44.3779225430461,0.));
#91569=CARTESIAN_POINT('Ctrl Pts',(-54.2750517888695,44.3859726620288,0.));
#91570=CARTESIAN_POINT('Ctrl Pts',(-54.2931073621661,44.3940254456427,0.));
#91571=CARTESIAN_POINT('Ctrl Pts',(-54.3112205860776,44.4020807028144,0.));
#91572=CARTESIAN_POINT('Ctrl Pts',(-54.3293912830237,44.4101382321834,0.));
#91573=CARTESIAN_POINT('Ctrl Pts',(-54.347619281931,44.4181978395814,0.));
#91574=CARTESIAN_POINT('Ctrl Pts',(-54.3659044357064,44.4262593564664,0.));
#91575=CARTESIAN_POINT('Ctrl Pts',(-54.3842466156151,44.4343226339555,0.));
#91576=CARTESIAN_POINT('Ctrl Pts',(-54.4026457030316,44.442387534098,0.));
#91577=CARTESIAN_POINT('Ctrl Pts',(-54.4211015825959,44.4504539226336,0.));
#91578=CARTESIAN_POINT('Ctrl Pts',(-54.4396141337008,44.4585216599933,0.));
#91579=CARTESIAN_POINT('Ctrl Pts',(-54.4581832262072,44.4665905967701,0.));
#91580=CARTESIAN_POINT('Ctrl Pts',(-54.4768087248854,44.4746605784056,0.));
#91581=CARTESIAN_POINT('Ctrl Pts',(-54.4954904921938,44.482731448127,0.));
#91582=CARTESIAN_POINT('Ctrl Pts',(-54.5142283914684,44.4908030503209,0.));
#91583=CARTESIAN_POINT('Ctrl Pts',(-54.5330222905438,44.4988752343715,0.));
#91584=CARTESIAN_POINT('Ctrl Pts',(-54.5518720616016,44.5069478544945,0.));
#91585=CARTESIAN_POINT('Ctrl Pts',(-54.5707775794412,44.5150207678988,0.));
#91586=CARTESIAN_POINT('Ctrl Pts',(-54.5897387202815,44.5230938335167,0.));
#91587=CARTESIAN_POINT('Ctrl Pts',(-54.6087553602914,44.5311669104515,0.));
#91588=CARTESIAN_POINT('Ctrl Pts',(-54.6278273743587,44.5392398566802,0.));
#91589=CARTESIAN_POINT('Ctrl Pts',(-54.6469546367408,44.5473125297311,0.));
#91590=CARTESIAN_POINT('Ctrl Pts',(-54.6661370216252,44.5553847872721,0.));
#91591=CARTESIAN_POINT('Ctrl Pts',(-54.6853744036751,44.5634564876863,0.));
#91592=CARTESIAN_POINT('Ctrl Pts',(-54.7046666586754,44.5715274907619,0.));
#91593=CARTESIAN_POINT('Ctrl Pts',(-54.7240136637717,44.5795976579454,0.));
#91594=CARTESIAN_POINT('Ctrl Pts',(-54.7434152971267,44.5876668519661,0.));
#91595=CARTESIAN_POINT('Ctrl Pts',(-54.7628714377037,44.5957349366059,0.));
#91596=CARTESIAN_POINT('Ctrl Pts',(-54.7823819650149,44.6038017764309,0.));
#91597=CARTESIAN_POINT('Ctrl Pts',(-54.8019467588278,44.6118672364906,0.));
#91598=CARTESIAN_POINT('Ctrl Pts',(-54.8215656991837,44.6199311823293,0.));
#91599=CARTESIAN_POINT('Ctrl Pts',(-54.8412386665276,44.6279934801169,0.));
#91600=CARTESIAN_POINT('Ctrl Pts',(-54.860965541796,44.6360539967392,0.));
#91601=CARTESIAN_POINT('Ctrl Pts',(-54.8807462065164,44.6441125999063,0.));
#91602=CARTESIAN_POINT('Ctrl Pts',(-54.9005805428969,44.6521691582533,0.));
#91603=CARTESIAN_POINT('Ctrl Pts',(-54.9204684337822,44.6602235412836,0.));
#91604=CARTESIAN_POINT('Ctrl Pts',(-54.9404097626077,44.6682756193147,0.));
#91605=CARTESIAN_POINT('Ctrl Pts',(-54.9604044133501,44.6763252634258,0.));
#91606=CARTESIAN_POINT('Ctrl Pts',(-54.9804522704686,44.6843723454,0.));
#91607=CARTESIAN_POINT('Ctrl Pts',(-55.0005532188667,44.6924167376869,0.));
#91608=CARTESIAN_POINT('Ctrl Pts',(-55.0207071439237,44.7004583134249,0.));
#91609=CARTESIAN_POINT('Ctrl Pts',(-55.0409139315078,44.7084969464513,0.));
#91610=CARTESIAN_POINT('Ctrl Pts',(-55.0611734679894,44.7165325113159,0.));
#91611=CARTESIAN_POINT('Ctrl Pts',(-55.0814856402496,44.7245648832979,0.));
#91612=CARTESIAN_POINT('Ctrl Pts',(-55.1018503356796,44.7325939384035,0.));
#91613=CARTESIAN_POINT('Ctrl Pts',(-55.1222674421743,44.740619553348,0.));
#91614=CARTESIAN_POINT('Ctrl Pts',(-55.14273684812,44.748641605542,0.));
#91615=CARTESIAN_POINT('Ctrl Pts',(-55.1632584423815,44.7566599730773,0.));
#91616=CARTESIAN_POINT('Ctrl Pts',(-55.1838321142779,44.7646745347109,0.));
#91617=CARTESIAN_POINT('Ctrl Pts',(-55.2044577535866,44.7726851698619,0.));
#91618=CARTESIAN_POINT('Ctrl Pts',(-55.2251352505475,44.7806917586077,0.));
#91619=CARTESIAN_POINT('Ctrl Pts',(-55.2458644958617,44.7886941816823,0.));
#91620=CARTESIAN_POINT('Ctrl Pts',(-55.2666453806883,44.7966923204741,0.));
#91621=CARTESIAN_POINT('Ctrl Pts',(-55.287477796635,44.8046860570245,0.));
#91622=CARTESIAN_POINT('Ctrl Pts',(-55.3083616357605,44.812675274021,0.));
#91623=CARTESIAN_POINT('Ctrl Pts',(-55.3292967905726,44.8206598547889,0.));
#91624=CARTESIAN_POINT('Ctrl Pts',(-55.350283154023,44.8286396832849,0.));
#91625=CARTESIAN_POINT('Ctrl Pts',(-55.3713206194962,44.8366146440896,0.));
#91626=CARTESIAN_POINT('Ctrl Pts',(-55.3924090808002,44.8445846224034,0.));
#91627=CARTESIAN_POINT('Ctrl Pts',(-55.4135484321706,44.8525495040397,0.));
#91628=CARTESIAN_POINT('Ctrl Pts',(-55.4347385682697,44.8605091754208,0.));
#91629=CARTESIAN_POINT('Ctrl Pts',(-55.4559793841838,44.8684635235727,0.));
#91630=CARTESIAN_POINT('Ctrl Pts',(-55.4772707754139,44.8764124361218,0.));
#91631=CARTESIAN_POINT('Ctrl Pts',(-55.4986126378676,44.8843558012903,0.));
#91632=CARTESIAN_POINT('Ctrl Pts',(-55.5200048678648,44.8922935078905,0.));
#91633=CARTESIAN_POINT('Ctrl Pts',(-55.541447362135,44.9002254453192,0.));
#91634=CARTESIAN_POINT('Ctrl Pts',(-55.5629400178136,44.9081515035525,0.));
#91635=CARTESIAN_POINT('Ctrl Pts',(-55.5844827324315,44.9160715731425,0.));
#91636=CARTESIAN_POINT('Ctrl Pts',(-55.6060754039089,44.9239855452119,0.));
#91637=CARTESIAN_POINT('Ctrl Pts',(-55.6277179305604,44.9318933114483,0.));
#91638=CARTESIAN_POINT('Ctrl Pts',(-55.6494102110922,44.9397947640996,0.));
#91639=CARTESIAN_POINT('Ctrl Pts',(-55.671152144599,44.9476897959694,0.));
#91640=CARTESIAN_POINT('Ctrl Pts',(-55.6929436305522,44.9555783004133,0.));
#91641=CARTESIAN_POINT('Ctrl Pts',(-55.7147845687969,44.9634601713352,0.));
#91642=CARTESIAN_POINT('Ctrl Pts',(-55.7366748595582,44.9713353031827,0.));
#91643=CARTESIAN_POINT('Ctrl Pts',(-55.7586144034376,44.979203590942,0.));
#91644=CARTESIAN_POINT('Ctrl Pts',(-55.7806031014093,44.9870649301333,0.));
#91645=CARTESIAN_POINT('Ctrl Pts',(-55.8026408548078,44.9949192168073,0.));
#91646=CARTESIAN_POINT('Ctrl Pts',(-55.8247275653257,45.002766347541,0.));
#91647=CARTESIAN_POINT('Ctrl Pts',(-55.8468631350195,45.0106062194325,0.));
#91648=CARTESIAN_POINT('Ctrl Pts',(-55.8690474663058,45.0184387300968,0.));
#91649=CARTESIAN_POINT('Ctrl Pts',(-55.8912804619588,45.0262637776623,0.));
#91650=CARTESIAN_POINT('Ctrl Pts',(-55.9135620250977,45.0340812607676,0.));
#91651=CARTESIAN_POINT('Ctrl Pts',(-55.9358920591861,45.041891078557,0.));
#91652=CARTESIAN_POINT('Ctrl Pts',(-55.958270468037,45.0496931306766,0.));
#91653=CARTESIAN_POINT('Ctrl Pts',(-55.9806971558099,45.0574873172696,0.));
#91654=CARTESIAN_POINT('Ctrl Pts',(-56.0031720270074,45.0652735389729,0.));
#91655=CARTESIAN_POINT('Ctrl Pts',(-56.025694986463,45.0730516969142,0.));
#91656=CARTESIAN_POINT('Ctrl Pts',(-56.0482659393412,45.0808216927082,0.));
#91657=CARTESIAN_POINT('Ctrl Pts',(-56.070884791141,45.0885834284513,0.));
#91658=CARTESIAN_POINT('Ctrl Pts',(-56.0935514476945,45.0963368067177,0.));
#91659=CARTESIAN_POINT('Ctrl Pts',(-56.1162658151621,45.1040817305563,0.));
#91660=CARTESIAN_POINT('Ctrl Pts',(-56.1390278000226,45.1118181034888,0.));
#91661=CARTESIAN_POINT('Ctrl Pts',(-56.1618373090729,45.119545829506,0.));
#91662=CARTESIAN_POINT('Ctrl Pts',(-56.1846942494321,45.1272648130627,0.));
#91663=CARTESIAN_POINT('Ctrl Pts',(-56.2075985285391,45.1349749590736,0.));
#91664=CARTESIAN_POINT('Ctrl Pts',(-56.2305500541491,45.1426761729107,0.));
#91665=CARTESIAN_POINT('Ctrl Pts',(-56.2535487343227,45.150368360401,0.));
#91666=CARTESIAN_POINT('Ctrl Pts',(-56.2765944774252,45.158051427823,0.));
#91667=CARTESIAN_POINT('Ctrl Pts',(-56.2996871921321,45.1657252819018,0.));
#91668=CARTESIAN_POINT('Ctrl Pts',(-56.3228267874265,45.1733898298062,0.));
#91669=CARTESIAN_POINT('Ctrl Pts',(-56.3460131725962,45.1810449791451,0.));
#91670=CARTESIAN_POINT('Ctrl Pts',(-56.3692462572228,45.1886906379664,0.));
#91671=CARTESIAN_POINT('Ctrl Pts',(-56.3925259511804,45.1963267147527,0.));
#91672=CARTESIAN_POINT('Ctrl Pts',(-56.4158521646412,45.2039531184172,0.));
#91673=CARTESIAN_POINT('Ctrl Pts',(-56.4392248080733,45.2115697583002,0.));
#91674=CARTESIAN_POINT('Ctrl Pts',(-56.4626437922385,45.2191765441666,0.));
#91675=CARTESIAN_POINT('Ctrl Pts',(-56.4861090281819,45.2267733862046,0.));
#91676=CARTESIAN_POINT('Ctrl Pts',(-56.5096204272299,45.2343601950222,0.));
#91677=CARTESIAN_POINT('Ctrl Pts',(-56.533177900995,45.2419368816423,0.));
#91678=CARTESIAN_POINT('Ctrl Pts',(-56.5567813613752,45.2495033574997,0.));
#91679=CARTESIAN_POINT('Ctrl Pts',(-56.5804307205507,45.2570595344382,0.));
#91680=CARTESIAN_POINT('Ctrl Pts',(-56.604125890975,45.2646053247094,0.));
#91681=CARTESIAN_POINT('Ctrl Pts',(-56.6278667853716,45.2721406409706,0.));
#91682=CARTESIAN_POINT('Ctrl Pts',(-56.6516533167398,45.2796653962796,0.));
#91683=CARTESIAN_POINT('Ctrl Pts',(-56.6754853983535,45.2871795040912,0.));
#91684=CARTESIAN_POINT('Ctrl Pts',(-56.6993629437596,45.2946828782557,0.));
#91685=CARTESIAN_POINT('Ctrl Pts',(-56.7232858667697,45.3021754330169,0.));
#91686=CARTESIAN_POINT('Ctrl Pts',(-56.747254081454,45.3096570830107,0.));
#91687=CARTESIAN_POINT('Ctrl Pts',(-56.771267502148,45.3171277432592,0.));
#91688=CARTESIAN_POINT('Ctrl Pts',(-56.7953260434521,45.3245873291682,0.));
#91689=CARTESIAN_POINT('Ctrl Pts',(-56.8194296202293,45.3320357565241,0.));
#91690=CARTESIAN_POINT('Ctrl Pts',(-56.8435781475982,45.3394729414932,0.));
#91691=CARTESIAN_POINT('Ctrl Pts',(-56.8677715409266,45.3468988006202,0.));
#91692=CARTESIAN_POINT('Ctrl Pts',(-56.8920097158371,45.3543132508234,0.));
#91693=CARTESIAN_POINT('Ctrl Pts',(-56.916292588208,45.3617162093918,0.));
#91694=CARTESIAN_POINT('Ctrl Pts',(-56.9406200741714,45.3691075939827,0.));
#91695=CARTESIAN_POINT('Ctrl Pts',(-56.9649920901079,45.3764873226202,0.));
#91696=CARTESIAN_POINT('Ctrl Pts',(-56.9894085526383,45.3838553136957,0.));
#91697=CARTESIAN_POINT('Ctrl Pts',(-57.0138693786287,45.3912114859625,0.));
#91698=CARTESIAN_POINT('Ctrl Pts',(-57.0383744851917,45.3985557585316,0.));
#91699=CARTESIAN_POINT('Ctrl Pts',(-57.0629237896848,45.4058880508693,0.));
#91700=CARTESIAN_POINT('Ctrl Pts',(-57.0875172097048,45.4132082827945,0.));
#91701=CARTESIAN_POINT('Ctrl Pts',(-57.1121546630776,45.4205163744778,0.));
#91702=CARTESIAN_POINT('Ctrl Pts',(-57.1368360678629,45.4278122464387,0.));
#91703=CARTESIAN_POINT('Ctrl Pts',(-57.1615613423586,45.4350958195434,0.));
#91704=CARTESIAN_POINT('Ctrl Pts',(-57.1863304051011,45.4423670150035,0.));
#91705=CARTESIAN_POINT('Ctrl Pts',(-57.2111431748629,45.4496257543759,0.));
#91706=CARTESIAN_POINT('Ctrl Pts',(-57.2359995706441,45.4568719595639,0.));
#91707=CARTESIAN_POINT('Ctrl Pts',(-57.2608995116727,45.4641055528138,0.));
#91708=CARTESIAN_POINT('Ctrl Pts',(-57.2858429174056,45.4713264567059,0.));
#91709=CARTESIAN_POINT('Ctrl Pts',(-57.3108297075262,45.4785345941505,0.));
#91710=CARTESIAN_POINT('Ctrl Pts',(-57.3358598019391,45.4857298883826,0.));
#91711=CARTESIAN_POINT('Ctrl Pts',(-57.360933120758,45.4929122629576,0.));
#91712=CARTESIAN_POINT('Ctrl Pts',(-57.3860495843043,45.5000816417516,0.));
#91713=CARTESIAN_POINT('Ctrl Pts',(-57.4112091131193,45.5072379489637,0.));
#91714=CARTESIAN_POINT('Ctrl Pts',(-57.4364116279708,45.5143811091209,0.));
#91715=CARTESIAN_POINT('Ctrl Pts',(-57.4616570498566,45.5215110470825,0.));
#91716=CARTESIAN_POINT('Ctrl Pts',(-57.4869453000055,45.5286276880479,0.));
#91717=CARTESIAN_POINT('Ctrl Pts',(-57.5122762998732,45.5357309575603,0.));
#91718=CARTESIAN_POINT('Ctrl Pts',(-57.5376499711338,45.5428207814832,0.));
#91719=CARTESIAN_POINT('Ctrl Pts',(-57.5630662356671,45.5498970859829,0.));
#91720=CARTESIAN_POINT('Ctrl Pts',(-57.5885250155432,45.5569597975096,0.));
#91721=CARTESIAN_POINT('Ctrl Pts',(-57.6140262330048,45.5640088427819,0.));
#91722=CARTESIAN_POINT('Ctrl Pts',(-57.6395698104416,45.5710441487683,0.));
#91723=CARTESIAN_POINT('Ctrl Pts',(-57.6651556704249,45.5780656427172,0.));
#91724=CARTESIAN_POINT('Ctrl Pts',(-57.6907837357425,45.5850732521902,0.));
#91725=CARTESIAN_POINT('Ctrl Pts',(-57.7164539294316,45.5920669050988,0.));
#91726=CARTESIAN_POINT('Ctrl Pts',(-57.7421661748022,45.5990465297341,0.));
#91727=CARTESIAN_POINT('Ctrl Pts',(-57.7679203954735,45.6060120548199,0.));
#91728=CARTESIAN_POINT('Ctrl Pts',(-57.7937165153379,45.6129634094677,0.));
#91729=CARTESIAN_POINT('Ctrl Pts',(-57.819554458484,45.619900523078,0.));
#91730=CARTESIAN_POINT('Ctrl Pts',(-57.8454341491236,45.6268233252543,0.));
#91731=CARTESIAN_POINT('Ctrl Pts',(-57.8713555115232,45.6337317457253,0.));
#91732=CARTESIAN_POINT('Ctrl Pts',(-57.8973184699037,45.6406257142385,0.));
#91733=CARTESIAN_POINT('Ctrl Pts',(-57.923322948432,45.6475051605542,0.));
#91734=CARTESIAN_POINT('Ctrl Pts',(-57.9493688714249,45.6543700146689,0.));
#91735=CARTESIAN_POINT('Ctrl Pts',(-57.975456163507,45.6612202069927,0.));
#91736=CARTESIAN_POINT('Ctrl Pts',(-58.0015847497838,45.6680556685494,0.));
#91737=CARTESIAN_POINT('Ctrl Pts',(-58.0277545560001,45.6748763311635,0.));
#91738=CARTESIAN_POINT('Ctrl Pts',(-58.0539655087095,45.6816821276662,0.));
#91739=CARTESIAN_POINT('Ctrl Pts',(-58.0802175348939,45.6884729914465,0.));
#91740=CARTESIAN_POINT('Ctrl Pts',(-58.1065105615884,45.6952488560133,0.));
#91741=CARTESIAN_POINT('Ctrl Pts',(-58.1328445154667,45.7020096545174,0.));
#91742=CARTESIAN_POINT('Ctrl Pts',(-58.159219322515,45.708755319378,0.));
#91743=CARTESIAN_POINT('Ctrl Pts',(-58.1856349074723,45.7154857816507,0.));
#91744=CARTESIAN_POINT('Ctrl Pts',(-58.2120911942819,45.7222009715431,0.));
#91745=CARTESIAN_POINT('Ctrl Pts',(-58.2385881070959,45.7289008195612,0.));
#91746=CARTESIAN_POINT('Ctrl Pts',(-58.2651255711481,45.7355852575127,0.));
#91747=CARTESIAN_POINT('Ctrl Pts',(-58.2917035135833,45.7422542194625,0.));
#91748=CARTESIAN_POINT('Ctrl Pts',(-58.3183218645265,45.7489076429725,0.));
#91749=CARTESIAN_POINT('Ctrl Pts',(-58.3449805573335,45.7555454693956,0.));
#91750=CARTESIAN_POINT('Ctrl Pts',(-58.3678667473266,45.7612219538034,0.));
#91751=CARTESIAN_POINT('Ctrl Pts',(-58.385434851721,45.7655655205267,0.));
#91752=CARTESIAN_POINT('Ctrl Pts',(-58.3976670480781,45.7685831165459,0.));
#91753=CARTESIAN_POINT('Ctrl Pts',(-58.4045515723008,45.7702793558063,0.));
#91754=CARTESIAN_POINT('Ctrl Pts',(-58.4060826907379,45.7706564944767,0.));
#91755=CARTESIAN_POINT('',(-54.1679505278134,44.3377168516418,12.));
#91756=CARTESIAN_POINT('',(-54.1679505278134,44.3377168516418,0.));
#91757=CARTESIAN_POINT('Ctrl Pts',(-58.4060826907378,45.7706564944767,12.));
#91758=CARTESIAN_POINT('Ctrl Pts',(-58.4045515723008,45.7702793558063,12.));
#91759=CARTESIAN_POINT('Ctrl Pts',(-58.397667048078,45.7685831165459,12.));
#91760=CARTESIAN_POINT('Ctrl Pts',(-58.385434851721,45.7655655205267,12.));
#91761=CARTESIAN_POINT('Ctrl Pts',(-58.3678667473265,45.7612219538034,12.));
#91762=CARTESIAN_POINT('Ctrl Pts',(-58.3449805573335,45.7555454693956,12.));
#91763=CARTESIAN_POINT('Ctrl Pts',(-58.3183218645265,45.7489076429725,12.));
#91764=CARTESIAN_POINT('Ctrl Pts',(-58.2917035135833,45.7422542194625,12.));
#91765=CARTESIAN_POINT('Ctrl Pts',(-58.2651255711481,45.7355852575127,12.));
#91766=CARTESIAN_POINT('Ctrl Pts',(-58.2385881070959,45.7289008195612,12.));
#91767=CARTESIAN_POINT('Ctrl Pts',(-58.2120911942819,45.7222009715431,12.));
#91768=CARTESIAN_POINT('Ctrl Pts',(-58.1856349074723,45.7154857816507,12.));
#91769=CARTESIAN_POINT('Ctrl Pts',(-58.159219322515,45.708755319378,12.));
#91770=CARTESIAN_POINT('Ctrl Pts',(-58.1328445154667,45.7020096545174,12.));
#91771=CARTESIAN_POINT('Ctrl Pts',(-58.1065105615884,45.6952488560133,12.));
#91772=CARTESIAN_POINT('Ctrl Pts',(-58.0802175348939,45.6884729914465,12.));
#91773=CARTESIAN_POINT('Ctrl Pts',(-58.0539655087095,45.6816821276662,12.));
#91774=CARTESIAN_POINT('Ctrl Pts',(-58.0277545560001,45.6748763311635,12.));
#91775=CARTESIAN_POINT('Ctrl Pts',(-58.0015847497838,45.6680556685494,12.));
#91776=CARTESIAN_POINT('Ctrl Pts',(-57.975456163507,45.6612202069927,12.));
#91777=CARTESIAN_POINT('Ctrl Pts',(-57.9493688714249,45.6543700146689,12.));
#91778=CARTESIAN_POINT('Ctrl Pts',(-57.923322948432,45.6475051605542,12.));
#91779=CARTESIAN_POINT('Ctrl Pts',(-57.8973184699037,45.6406257142385,12.));
#91780=CARTESIAN_POINT('Ctrl Pts',(-57.8713555115232,45.6337317457253,12.));
#91781=CARTESIAN_POINT('Ctrl Pts',(-57.8454341491236,45.6268233252543,12.));
#91782=CARTESIAN_POINT('Ctrl Pts',(-57.819554458484,45.619900523078,12.));
#91783=CARTESIAN_POINT('Ctrl Pts',(-57.7937165153379,45.6129634094677,12.));
#91784=CARTESIAN_POINT('Ctrl Pts',(-57.7679203954735,45.6060120548199,12.));
#91785=CARTESIAN_POINT('Ctrl Pts',(-57.7421661748022,45.5990465297341,12.));
#91786=CARTESIAN_POINT('Ctrl Pts',(-57.7164539294316,45.5920669050988,12.));
#91787=CARTESIAN_POINT('Ctrl Pts',(-57.6907837357425,45.5850732521902,12.));
#91788=CARTESIAN_POINT('Ctrl Pts',(-57.6651556704249,45.5780656427172,12.));
#91789=CARTESIAN_POINT('Ctrl Pts',(-57.6395698104416,45.5710441487683,12.));
#91790=CARTESIAN_POINT('Ctrl Pts',(-57.6140262330048,45.5640088427819,12.));
#91791=CARTESIAN_POINT('Ctrl Pts',(-57.5885250155432,45.5569597975096,12.));
#91792=CARTESIAN_POINT('Ctrl Pts',(-57.5630662356671,45.5498970859829,12.));
#91793=CARTESIAN_POINT('Ctrl Pts',(-57.5376499711338,45.5428207814832,12.));
#91794=CARTESIAN_POINT('Ctrl Pts',(-57.5122762998732,45.5357309575603,12.));
#91795=CARTESIAN_POINT('Ctrl Pts',(-57.4869453000055,45.5286276880479,12.));
#91796=CARTESIAN_POINT('Ctrl Pts',(-57.4616570498566,45.5215110470825,12.));
#91797=CARTESIAN_POINT('Ctrl Pts',(-57.4364116279708,45.5143811091209,12.));
#91798=CARTESIAN_POINT('Ctrl Pts',(-57.4112091131193,45.5072379489637,12.));
#91799=CARTESIAN_POINT('Ctrl Pts',(-57.3860495843043,45.5000816417516,12.));
#91800=CARTESIAN_POINT('Ctrl Pts',(-57.360933120758,45.4929122629576,12.));
#91801=CARTESIAN_POINT('Ctrl Pts',(-57.3358598019391,45.4857298883826,12.));
#91802=CARTESIAN_POINT('Ctrl Pts',(-57.3108297075262,45.4785345941505,12.));
#91803=CARTESIAN_POINT('Ctrl Pts',(-57.2858429174056,45.4713264567059,12.));
#91804=CARTESIAN_POINT('Ctrl Pts',(-57.2608995116727,45.4641055528138,12.));
#91805=CARTESIAN_POINT('Ctrl Pts',(-57.2359995706441,45.4568719595639,12.));
#91806=CARTESIAN_POINT('Ctrl Pts',(-57.2111431748629,45.4496257543759,12.));
#91807=CARTESIAN_POINT('Ctrl Pts',(-57.1863304051011,45.4423670150035,12.));
#91808=CARTESIAN_POINT('Ctrl Pts',(-57.1615613423586,45.4350958195434,12.));
#91809=CARTESIAN_POINT('Ctrl Pts',(-57.1368360678629,45.4278122464387,12.));
#91810=CARTESIAN_POINT('Ctrl Pts',(-57.1121546630776,45.4205163744778,12.));
#91811=CARTESIAN_POINT('Ctrl Pts',(-57.0875172097048,45.4132082827945,12.));
#91812=CARTESIAN_POINT('Ctrl Pts',(-57.0629237896848,45.4058880508693,12.));
#91813=CARTESIAN_POINT('Ctrl Pts',(-57.0383744851917,45.3985557585316,12.));
#91814=CARTESIAN_POINT('Ctrl Pts',(-57.0138693786287,45.3912114859625,12.));
#91815=CARTESIAN_POINT('Ctrl Pts',(-56.9894085526383,45.3838553136957,12.));
#91816=CARTESIAN_POINT('Ctrl Pts',(-56.9649920901079,45.3764873226202,12.));
#91817=CARTESIAN_POINT('Ctrl Pts',(-56.9406200741714,45.3691075939827,12.));
#91818=CARTESIAN_POINT('Ctrl Pts',(-56.916292588208,45.3617162093918,12.));
#91819=CARTESIAN_POINT('Ctrl Pts',(-56.8920097158371,45.3543132508234,12.));
#91820=CARTESIAN_POINT('Ctrl Pts',(-56.8677715409266,45.3468988006202,12.));
#91821=CARTESIAN_POINT('Ctrl Pts',(-56.8435781475982,45.3394729414932,12.));
#91822=CARTESIAN_POINT('Ctrl Pts',(-56.8194296202293,45.3320357565241,12.));
#91823=CARTESIAN_POINT('Ctrl Pts',(-56.7953260434521,45.3245873291682,12.));
#91824=CARTESIAN_POINT('Ctrl Pts',(-56.771267502148,45.3171277432592,12.));
#91825=CARTESIAN_POINT('Ctrl Pts',(-56.747254081454,45.3096570830107,12.));
#91826=CARTESIAN_POINT('Ctrl Pts',(-56.7232858667697,45.3021754330169,12.));
#91827=CARTESIAN_POINT('Ctrl Pts',(-56.6993629437596,45.2946828782557,12.));
#91828=CARTESIAN_POINT('Ctrl Pts',(-56.6754853983535,45.2871795040912,12.));
#91829=CARTESIAN_POINT('Ctrl Pts',(-56.6516533167398,45.2796653962796,12.));
#91830=CARTESIAN_POINT('Ctrl Pts',(-56.6278667853716,45.2721406409706,12.));
#91831=CARTESIAN_POINT('Ctrl Pts',(-56.604125890975,45.2646053247094,12.));
#91832=CARTESIAN_POINT('Ctrl Pts',(-56.5804307205507,45.2570595344382,12.));
#91833=CARTESIAN_POINT('Ctrl Pts',(-56.5567813613752,45.2495033574997,12.));
#91834=CARTESIAN_POINT('Ctrl Pts',(-56.533177900995,45.2419368816423,12.));
#91835=CARTESIAN_POINT('Ctrl Pts',(-56.5096204272299,45.2343601950222,12.));
#91836=CARTESIAN_POINT('Ctrl Pts',(-56.4861090281819,45.2267733862046,12.));
#91837=CARTESIAN_POINT('Ctrl Pts',(-56.4626437922385,45.2191765441666,12.));
#91838=CARTESIAN_POINT('Ctrl Pts',(-56.4392248080733,45.2115697583002,12.));
#91839=CARTESIAN_POINT('Ctrl Pts',(-56.4158521646412,45.2039531184172,12.));
#91840=CARTESIAN_POINT('Ctrl Pts',(-56.3925259511804,45.1963267147527,12.));
#91841=CARTESIAN_POINT('Ctrl Pts',(-56.3692462572228,45.1886906379664,12.));
#91842=CARTESIAN_POINT('Ctrl Pts',(-56.3460131725962,45.1810449791451,12.));
#91843=CARTESIAN_POINT('Ctrl Pts',(-56.3228267874265,45.1733898298062,12.));
#91844=CARTESIAN_POINT('Ctrl Pts',(-56.2996871921321,45.1657252819018,12.));
#91845=CARTESIAN_POINT('Ctrl Pts',(-56.2765944774252,45.158051427823,12.));
#91846=CARTESIAN_POINT('Ctrl Pts',(-56.2535487343227,45.150368360401,12.));
#91847=CARTESIAN_POINT('Ctrl Pts',(-56.2305500541491,45.1426761729107,12.));
#91848=CARTESIAN_POINT('Ctrl Pts',(-56.2075985285391,45.1349749590736,12.));
#91849=CARTESIAN_POINT('Ctrl Pts',(-56.1846942494321,45.1272648130627,12.));
#91850=CARTESIAN_POINT('Ctrl Pts',(-56.1618373090729,45.119545829506,12.));
#91851=CARTESIAN_POINT('Ctrl Pts',(-56.1390278000226,45.1118181034888,12.));
#91852=CARTESIAN_POINT('Ctrl Pts',(-56.1162658151621,45.1040817305563,12.));
#91853=CARTESIAN_POINT('Ctrl Pts',(-56.0935514476945,45.0963368067177,12.));
#91854=CARTESIAN_POINT('Ctrl Pts',(-56.070884791141,45.0885834284513,12.));
#91855=CARTESIAN_POINT('Ctrl Pts',(-56.0482659393412,45.0808216927082,12.));
#91856=CARTESIAN_POINT('Ctrl Pts',(-56.025694986463,45.0730516969142,12.));
#91857=CARTESIAN_POINT('Ctrl Pts',(-56.0031720270074,45.0652735389729,12.));
#91858=CARTESIAN_POINT('Ctrl Pts',(-55.9806971558099,45.0574873172696,12.));
#91859=CARTESIAN_POINT('Ctrl Pts',(-55.958270468037,45.0496931306766,12.));
#91860=CARTESIAN_POINT('Ctrl Pts',(-55.9358920591861,45.041891078557,12.));
#91861=CARTESIAN_POINT('Ctrl Pts',(-55.9135620250977,45.0340812607676,12.));
#91862=CARTESIAN_POINT('Ctrl Pts',(-55.8912804619588,45.0262637776623,12.));
#91863=CARTESIAN_POINT('Ctrl Pts',(-55.8690474663058,45.0184387300968,12.));
#91864=CARTESIAN_POINT('Ctrl Pts',(-55.8468631350195,45.0106062194325,12.));
#91865=CARTESIAN_POINT('Ctrl Pts',(-55.8247275653257,45.002766347541,12.));
#91866=CARTESIAN_POINT('Ctrl Pts',(-55.8026408548078,44.9949192168073,12.));
#91867=CARTESIAN_POINT('Ctrl Pts',(-55.7806031014093,44.9870649301333,12.));
#91868=CARTESIAN_POINT('Ctrl Pts',(-55.7586144034376,44.979203590942,12.));
#91869=CARTESIAN_POINT('Ctrl Pts',(-55.7366748595582,44.9713353031827,12.));
#91870=CARTESIAN_POINT('Ctrl Pts',(-55.7147845687969,44.9634601713352,12.));
#91871=CARTESIAN_POINT('Ctrl Pts',(-55.6929436305522,44.9555783004133,12.));
#91872=CARTESIAN_POINT('Ctrl Pts',(-55.671152144599,44.9476897959694,12.));
#91873=CARTESIAN_POINT('Ctrl Pts',(-55.6494102110922,44.9397947640996,12.));
#91874=CARTESIAN_POINT('Ctrl Pts',(-55.6277179305604,44.9318933114483,12.));
#91875=CARTESIAN_POINT('Ctrl Pts',(-55.6060754039089,44.9239855452119,12.));
#91876=CARTESIAN_POINT('Ctrl Pts',(-55.5844827324315,44.9160715731425,12.));
#91877=CARTESIAN_POINT('Ctrl Pts',(-55.5629400178136,44.9081515035525,12.));
#91878=CARTESIAN_POINT('Ctrl Pts',(-55.541447362135,44.9002254453192,12.));
#91879=CARTESIAN_POINT('Ctrl Pts',(-55.5200048678648,44.8922935078905,12.));
#91880=CARTESIAN_POINT('Ctrl Pts',(-55.4986126378676,44.8843558012903,12.));
#91881=CARTESIAN_POINT('Ctrl Pts',(-55.4772707754139,44.8764124361218,12.));
#91882=CARTESIAN_POINT('Ctrl Pts',(-55.4559793841838,44.8684635235727,12.));
#91883=CARTESIAN_POINT('Ctrl Pts',(-55.4347385682697,44.8605091754208,12.));
#91884=CARTESIAN_POINT('Ctrl Pts',(-55.4135484321706,44.8525495040397,12.));
#91885=CARTESIAN_POINT('Ctrl Pts',(-55.3924090808002,44.8445846224034,12.));
#91886=CARTESIAN_POINT('Ctrl Pts',(-55.3713206194962,44.8366146440896,12.));
#91887=CARTESIAN_POINT('Ctrl Pts',(-55.350283154023,44.8286396832849,12.));
#91888=CARTESIAN_POINT('Ctrl Pts',(-55.3292967905726,44.8206598547889,12.));
#91889=CARTESIAN_POINT('Ctrl Pts',(-55.3083616357605,44.812675274021,12.));
#91890=CARTESIAN_POINT('Ctrl Pts',(-55.287477796635,44.8046860570245,12.));
#91891=CARTESIAN_POINT('Ctrl Pts',(-55.2666453806883,44.7966923204741,12.));
#91892=CARTESIAN_POINT('Ctrl Pts',(-55.2458644958617,44.7886941816823,12.));
#91893=CARTESIAN_POINT('Ctrl Pts',(-55.2251352505475,44.7806917586077,12.));
#91894=CARTESIAN_POINT('Ctrl Pts',(-55.2044577535866,44.7726851698619,12.));
#91895=CARTESIAN_POINT('Ctrl Pts',(-55.1838321142779,44.7646745347109,12.));
#91896=CARTESIAN_POINT('Ctrl Pts',(-55.1632584423815,44.7566599730773,12.));
#91897=CARTESIAN_POINT('Ctrl Pts',(-55.14273684812,44.748641605542,12.));
#91898=CARTESIAN_POINT('Ctrl Pts',(-55.1222674421743,44.740619553348,12.));
#91899=CARTESIAN_POINT('Ctrl Pts',(-55.1018503356796,44.7325939384035,12.));
#91900=CARTESIAN_POINT('Ctrl Pts',(-55.0814856402496,44.7245648832979,12.));
#91901=CARTESIAN_POINT('Ctrl Pts',(-55.0611734679894,44.7165325113159,12.));
#91902=CARTESIAN_POINT('Ctrl Pts',(-55.0409139315078,44.7084969464513,12.));
#91903=CARTESIAN_POINT('Ctrl Pts',(-55.0207071439237,44.7004583134249,12.));
#91904=CARTESIAN_POINT('Ctrl Pts',(-55.0005532188667,44.6924167376869,12.));
#91905=CARTESIAN_POINT('Ctrl Pts',(-54.9804522704686,44.6843723454,12.));
#91906=CARTESIAN_POINT('Ctrl Pts',(-54.9604044133501,44.6763252634258,12.));
#91907=CARTESIAN_POINT('Ctrl Pts',(-54.9404097626077,44.6682756193147,12.));
#91908=CARTESIAN_POINT('Ctrl Pts',(-54.9204684337822,44.6602235412836,12.));
#91909=CARTESIAN_POINT('Ctrl Pts',(-54.9005805428969,44.6521691582533,12.));
#91910=CARTESIAN_POINT('Ctrl Pts',(-54.8807462065164,44.6441125999063,12.));
#91911=CARTESIAN_POINT('Ctrl Pts',(-54.860965541796,44.6360539967392,12.));
#91912=CARTESIAN_POINT('Ctrl Pts',(-54.8412386665276,44.6279934801169,12.));
#91913=CARTESIAN_POINT('Ctrl Pts',(-54.8215656991837,44.6199311823293,12.));
#91914=CARTESIAN_POINT('Ctrl Pts',(-54.8019467588278,44.6118672364906,12.));
#91915=CARTESIAN_POINT('Ctrl Pts',(-54.7823819650149,44.6038017764309,12.));
#91916=CARTESIAN_POINT('Ctrl Pts',(-54.7628714377037,44.5957349366059,12.));
#91917=CARTESIAN_POINT('Ctrl Pts',(-54.7434152971267,44.5876668519661,12.));
#91918=CARTESIAN_POINT('Ctrl Pts',(-54.7240136637717,44.5795976579454,12.));
#91919=CARTESIAN_POINT('Ctrl Pts',(-54.7046666586754,44.5715274907619,12.));
#91920=CARTESIAN_POINT('Ctrl Pts',(-54.6853744036751,44.5634564876863,12.));
#91921=CARTESIAN_POINT('Ctrl Pts',(-54.6661370216252,44.5553847872721,12.));
#91922=CARTESIAN_POINT('Ctrl Pts',(-54.6469546367408,44.5473125297311,12.));
#91923=CARTESIAN_POINT('Ctrl Pts',(-54.6278273743587,44.5392398566802,12.));
#91924=CARTESIAN_POINT('Ctrl Pts',(-54.6087553602914,44.5311669104515,12.));
#91925=CARTESIAN_POINT('Ctrl Pts',(-54.5897387202815,44.5230938335167,12.));
#91926=CARTESIAN_POINT('Ctrl Pts',(-54.5707775794412,44.5150207678988,12.));
#91927=CARTESIAN_POINT('Ctrl Pts',(-54.5518720616016,44.5069478544945,12.));
#91928=CARTESIAN_POINT('Ctrl Pts',(-54.5330222905438,44.4988752343715,12.));
#91929=CARTESIAN_POINT('Ctrl Pts',(-54.5142283914684,44.4908030503209,12.));
#91930=CARTESIAN_POINT('Ctrl Pts',(-54.4954904921938,44.482731448127,12.));
#91931=CARTESIAN_POINT('Ctrl Pts',(-54.4768087248854,44.4746605784056,12.));
#91932=CARTESIAN_POINT('Ctrl Pts',(-54.4581832262072,44.4665905967701,12.));
#91933=CARTESIAN_POINT('Ctrl Pts',(-54.4396141337008,44.4585216599933,12.));
#91934=CARTESIAN_POINT('Ctrl Pts',(-54.4211015825959,44.4504539226336,12.));
#91935=CARTESIAN_POINT('Ctrl Pts',(-54.4026457030316,44.442387534098,12.));
#91936=CARTESIAN_POINT('Ctrl Pts',(-54.3842466156151,44.4343226339555,12.));
#91937=CARTESIAN_POINT('Ctrl Pts',(-54.3659044357064,44.4262593564664,12.));
#91938=CARTESIAN_POINT('Ctrl Pts',(-54.347619281931,44.4181978395814,12.));
#91939=CARTESIAN_POINT('Ctrl Pts',(-54.3293912830237,44.4101382321834,12.));
#91940=CARTESIAN_POINT('Ctrl Pts',(-54.3112205860776,44.4020807028144,12.));
#91941=CARTESIAN_POINT('Ctrl Pts',(-54.2931073621661,44.3940254456427,12.));
#91942=CARTESIAN_POINT('Ctrl Pts',(-54.2750517888695,44.3859726620288,12.));
#91943=CARTESIAN_POINT('Ctrl Pts',(-54.2570540336536,44.3779225430461,12.));
#91944=CARTESIAN_POINT('Ctrl Pts',(-54.2391142386354,44.369875253351,12.));
#91945=CARTESIAN_POINT('Ctrl Pts',(-54.2212325005847,44.3618309103245,12.));
#91946=CARTESIAN_POINT('Ctrl Pts',(-54.203408870162,44.3537895823819,12.));
#91947=CARTESIAN_POINT('Ctrl Pts',(-54.1891964684439,44.3473589597468,12.));
#91948=CARTESIAN_POINT('Ctrl Pts',(-54.1785633257456,44.3425373700829,12.));
#91949=CARTESIAN_POINT('Ctrl Pts',(-54.1714861895278,44.3393235891014,12.));
#91950=CARTESIAN_POINT('Ctrl Pts',(-54.1679505278134,44.3377168516418,12.));
#91951=CARTESIAN_POINT('Ctrl Pts',(-59.3276657444392,44.5696260757792,-1.11022302462516E-15));
#91952=CARTESIAN_POINT('Ctrl Pts',(-59.3276657444392,44.5696260757792,4.));
#91953=CARTESIAN_POINT('Ctrl Pts',(-59.3276657444392,44.5696260757792,8.));
#91954=CARTESIAN_POINT('Ctrl Pts',(-59.3276657444392,44.5696260757792,12.));
#91955=CARTESIAN_POINT('Ctrl Pts',(-59.3806648691719,44.6658822400933,-1.11022302462516E-15));
#91956=CARTESIAN_POINT('Ctrl Pts',(-59.3806648691719,44.6658822400933,4.));
#91957=CARTESIAN_POINT('Ctrl Pts',(-59.3806648691719,44.6658822400933,8.));
#91958=CARTESIAN_POINT('Ctrl Pts',(-59.3806648691719,44.6658822400933,12.));
#91959=CARTESIAN_POINT('Ctrl Pts',(-59.4154499491518,44.8655383388341,-1.03713949455603E-15));
#91960=CARTESIAN_POINT('Ctrl Pts',(-59.4154499491518,44.8655383388341,4.));
#91961=CARTESIAN_POINT('Ctrl Pts',(-59.4154499491518,44.8655383388341,7.99999999999999));
#91962=CARTESIAN_POINT('Ctrl Pts',(-59.4154499491518,44.8655383388341,12.));
#91963=CARTESIAN_POINT('Ctrl Pts',(-59.3374774995081,45.047980595232,-8.63611844427577E-16));
#91964=CARTESIAN_POINT('Ctrl Pts',(-59.3374774995081,45.047980595232,4.));
#91965=CARTESIAN_POINT('Ctrl Pts',(-59.3374774995081,45.0479805952321,8.00000000000001));
#91966=CARTESIAN_POINT('Ctrl Pts',(-59.3374774995081,45.0479805952321,12.));
#91967=CARTESIAN_POINT('Ctrl Pts',(-59.2875729049565,45.1135644683452,-7.79957864199761E-16));
#91968=CARTESIAN_POINT('Ctrl Pts',(-59.2875729049565,45.1135644683452,4.));
#91969=CARTESIAN_POINT('Ctrl Pts',(-59.2875729049565,45.1135644683452,8.));
#91970=CARTESIAN_POINT('Ctrl Pts',(-59.2875729049565,45.1135644683452,12.));
#91971=CARTESIAN_POINT('',(-59.3276657444392,44.5696260757792,2.77555756156289E-16));
#91972=CARTESIAN_POINT('',(-59.2875729049561,45.1135644683449,2.77555756156289E-16));
#91973=CARTESIAN_POINT('Ctrl Pts',(-59.3276657444392,44.5696260757792,-3.21795698712167E-17));
#91974=CARTESIAN_POINT('Ctrl Pts',(-59.3806648691719,44.6658822400933,-3.2179569871217E-17));
#91975=CARTESIAN_POINT('Ctrl Pts',(-59.4005420577319,44.7799714393737,9.58244731114085E-18));
#91976=CARTESIAN_POINT('Ctrl Pts',(-59.3836004611086,44.8884397921749,8.41425445128705E-17));
#91977=CARTESIAN_POINT('Ctrl Pts',(-59.3708942636411,44.9697910567758,1.40062617414167E-16));
#91978=CARTESIAN_POINT('Ctrl Pts',(-59.3374774995081,45.047980595232,2.14431610326361E-16));
#91979=CARTESIAN_POINT('Ctrl Pts',(-59.2875729049565,45.1135644683452,2.98085590554179E-16));
#91980=CARTESIAN_POINT('',(-59.2875729049561,45.1135644683449,12.));
#91981=CARTESIAN_POINT('Ctrl Pts',(-59.2875729049565,45.1135644683452,-7.79957864199761E-16));
#91982=CARTESIAN_POINT('Ctrl Pts',(-59.2875729049565,45.1135644683452,4.));
#91983=CARTESIAN_POINT('Ctrl Pts',(-59.2875729049565,45.1135644683452,8.));
#91984=CARTESIAN_POINT('Ctrl Pts',(-59.2875729049565,45.1135644683452,12.));
#91985=CARTESIAN_POINT('',(-59.3276657444392,44.5696260757792,12.));
#91986=CARTESIAN_POINT('Ctrl Pts',(-59.2875729049565,45.1135644683452,12.));
#91987=CARTESIAN_POINT('Ctrl Pts',(-59.3374774995081,45.0479805952321,12.));
#91988=CARTESIAN_POINT('Ctrl Pts',(-59.3708942636412,44.9697910567758,12.));
#91989=CARTESIAN_POINT('Ctrl Pts',(-59.3836004611086,44.8884397921749,12.));
#91990=CARTESIAN_POINT('Ctrl Pts',(-59.4005420577319,44.7799714393738,12.));
#91991=CARTESIAN_POINT('Ctrl Pts',(-59.3806648691719,44.6658822400933,12.));
#91992=CARTESIAN_POINT('Ctrl Pts',(-59.3276657444392,44.5696260757792,12.));
#91993=CARTESIAN_POINT('Ctrl Pts',(-59.3276657444392,44.5696260757792,12.));
#91994=CARTESIAN_POINT('Ctrl Pts',(-59.3276657444392,44.5696260757792,8.));
#91995=CARTESIAN_POINT('Ctrl Pts',(-59.3276657444392,44.5696260757792,4.));
#91996=CARTESIAN_POINT('Ctrl Pts',(-59.3276657444392,44.5696260757792,-1.11022302462516E-15));
#91997=CARTESIAN_POINT('Origin',(-2.97443977737815E-10,2.28111678886296E-10,
0.));
#91998=CARTESIAN_POINT('Origin',(-2.97443977737815E-10,2.28111678886296E-10,
12.));
#91999=CARTESIAN_POINT('Origin',(-2.97443977737815E-10,2.28111678886296E-10,
0.));
#92000=CARTESIAN_POINT('Ctrl Pts',(-54.7233670476849,50.5529731960876,0.));
#92001=CARTESIAN_POINT('Ctrl Pts',(-54.7233670476849,50.5529731960876,4.));
#92002=CARTESIAN_POINT('Ctrl Pts',(-54.7233670476849,50.5529731960876,8.));
#92003=CARTESIAN_POINT('Ctrl Pts',(-54.7233670476849,50.5529731960876,12.));
#92004=CARTESIAN_POINT('Ctrl Pts',(-54.6488048279283,50.6336864649947,0.));
#92005=CARTESIAN_POINT('Ctrl Pts',(-54.6488048279283,50.6336864649947,4.));
#92006=CARTESIAN_POINT('Ctrl Pts',(-54.6488048279283,50.6336864649947,8.));
#92007=CARTESIAN_POINT('Ctrl Pts',(-54.6488048279283,50.6336864649947,12.));
#92008=CARTESIAN_POINT('Ctrl Pts',(-54.4703879751555,50.7298112257545,0.));
#92009=CARTESIAN_POINT('Ctrl Pts',(-54.4703879751555,50.7298112257545,4.00000000000001));
#92010=CARTESIAN_POINT('Ctrl Pts',(-54.4703879751555,50.7298112257545,8.));
#92011=CARTESIAN_POINT('Ctrl Pts',(-54.4703879751555,50.7298112257545,12.));
#92012=CARTESIAN_POINT('Ctrl Pts',(-54.2726521137411,50.7135202769403,0.));
#92013=CARTESIAN_POINT('Ctrl Pts',(-54.2726521137411,50.7135202769403,4.));
#92014=CARTESIAN_POINT('Ctrl Pts',(-54.2726521137411,50.7135202769403,8.));
#92015=CARTESIAN_POINT('Ctrl Pts',(-54.2726521137411,50.7135202769403,12.));
#92016=CARTESIAN_POINT('Ctrl Pts',(-54.1946543499979,50.6869108458687,0.));
#92017=CARTESIAN_POINT('Ctrl Pts',(-54.1946543499979,50.6869108458687,4.));
#92018=CARTESIAN_POINT('Ctrl Pts',(-54.1946543499979,50.6869108458687,8.));
#92019=CARTESIAN_POINT('Ctrl Pts',(-54.1946543499979,50.6869108458687,12.));
#92020=CARTESIAN_POINT('',(-54.7233670476849,50.5529731960876,0.));
#92021=CARTESIAN_POINT('',(-54.1946543499978,50.6869108458688,0.));
#92022=CARTESIAN_POINT('Ctrl Pts',(-54.7233670476849,50.5529731960876,1.38777878078145E-16));
#92023=CARTESIAN_POINT('Ctrl Pts',(-54.6488048279283,50.6336864649947,1.38777878078144E-16));
#92024=CARTESIAN_POINT('Ctrl Pts',(-54.5468523406296,50.6886148997146,1.38777878078145E-16));
#92025=CARTESIAN_POINT('Ctrl Pts',(-54.4385916056111,50.7068361639613,1.38777878078145E-16));
#92026=CARTESIAN_POINT('Ctrl Pts',(-54.3573960543472,50.7205021121464,1.38777878078145E-16));
#92027=CARTESIAN_POINT('Ctrl Pts',(-54.2726521137411,50.7135202769403,1.38777878078144E-16));
#92028=CARTESIAN_POINT('Ctrl Pts',(-54.1946543499979,50.6869108458687,1.38777878078145E-16));
#92029=CARTESIAN_POINT('',(-54.1946543499978,50.6869108458688,12.));
#92030=CARTESIAN_POINT('Ctrl Pts',(-54.1946543499979,50.6869108458687,0.));
#92031=CARTESIAN_POINT('Ctrl Pts',(-54.1946543499979,50.6869108458687,4.));
#92032=CARTESIAN_POINT('Ctrl Pts',(-54.1946543499979,50.6869108458687,8.));
#92033=CARTESIAN_POINT('Ctrl Pts',(-54.1946543499979,50.6869108458687,12.));
#92034=CARTESIAN_POINT('',(-54.7233670476849,50.5529731960876,12.));
#92035=CARTESIAN_POINT('Ctrl Pts',(-54.1946543499979,50.6869108458687,12.));
#92036=CARTESIAN_POINT('Ctrl Pts',(-54.2726521137411,50.7135202769403,12.));
#92037=CARTESIAN_POINT('Ctrl Pts',(-54.3573960543472,50.7205021121464,12.));
#92038=CARTESIAN_POINT('Ctrl Pts',(-54.4385916056111,50.7068361639613,12.));
#92039=CARTESIAN_POINT('Ctrl Pts',(-54.5468523406296,50.6886148997146,12.));
#92040=CARTESIAN_POINT('Ctrl Pts',(-54.6488048279283,50.6336864649947,12.));
#92041=CARTESIAN_POINT('Ctrl Pts',(-54.7233670476849,50.5529731960876,12.));
#92042=CARTESIAN_POINT('Ctrl Pts',(-54.7233670476849,50.5529731960876,12.));
#92043=CARTESIAN_POINT('Ctrl Pts',(-54.7233670476849,50.5529731960876,8.));
#92044=CARTESIAN_POINT('Ctrl Pts',(-54.7233670476849,50.5529731960876,4.));
#92045=CARTESIAN_POINT('Ctrl Pts',(-54.7233670476849,50.5529731960876,0.));
#92046=CARTESIAN_POINT('Ctrl Pts',(-50.0975384783634,48.8900464144686,0.));
#92047=CARTESIAN_POINT('Ctrl Pts',(-50.0975384783634,48.8900464144686,12.));
#92048=CARTESIAN_POINT('Ctrl Pts',(-50.1009206494209,48.8919551910299,0.));
#92049=CARTESIAN_POINT('Ctrl Pts',(-50.1009206494209,48.8919551910299,12.));
#92050=CARTESIAN_POINT('Ctrl Pts',(-50.1076907555303,48.8957735556681,0.));
#92051=CARTESIAN_POINT('Ctrl Pts',(-50.1076907555303,48.8957735556681,12.));
#92052=CARTESIAN_POINT('Ctrl Pts',(-50.1178632066821,48.9015035371772,0.));
#92053=CARTESIAN_POINT('Ctrl Pts',(-50.1178632066821,48.9015035371772,12.));
#92054=CARTESIAN_POINT('Ctrl Pts',(-50.1314610602286,48.9091483817797,0.));
#92055=CARTESIAN_POINT('Ctrl Pts',(-50.1314610602286,48.9091483817797,12.));
#92056=CARTESIAN_POINT('Ctrl Pts',(-50.148516018447,48.9187125417897,0.));
#92057=CARTESIAN_POINT('Ctrl Pts',(-50.148516018447,48.9187125417897,12.));
#92058=CARTESIAN_POINT('Ctrl Pts',(-50.1656286003943,48.9282847698237,0.));
#92059=CARTESIAN_POINT('Ctrl Pts',(-50.1656286003943,48.9282847698237,12.));
#92060=CARTESIAN_POINT('Ctrl Pts',(-50.1827987615659,48.9378649933116,0.));
#92061=CARTESIAN_POINT('Ctrl Pts',(-50.1827987615659,48.9378649933116,12.));
#92062=CARTESIAN_POINT('Ctrl Pts',(-50.2000264157903,48.9474530868847,0.));
#92063=CARTESIAN_POINT('Ctrl Pts',(-50.2000264157903,48.9474530868847,12.));
#92064=CARTESIAN_POINT('Ctrl Pts',(-50.2173114358423,48.9570488741273,0.));
#92065=CARTESIAN_POINT('Ctrl Pts',(-50.2173114358423,48.9570488741273,12.));
#92066=CARTESIAN_POINT('Ctrl Pts',(-50.2346536715465,48.9666521500969,0.));
#92067=CARTESIAN_POINT('Ctrl Pts',(-50.2346536715465,48.9666521500969,12.));
#92068=CARTESIAN_POINT('Ctrl Pts',(-50.252052963548,48.9762626987227,0.));
#92069=CARTESIAN_POINT('Ctrl Pts',(-50.252052963548,48.9762626987227,12.));
#92070=CARTESIAN_POINT('Ctrl Pts',(-50.2695091583473,48.9858803116649,0.));
#92071=CARTESIAN_POINT('Ctrl Pts',(-50.2695091583473,48.9858803116649,12.));
#92072=CARTESIAN_POINT('Ctrl Pts',(-50.2870221241003,48.9955048082028,0.));
#92073=CARTESIAN_POINT('Ctrl Pts',(-50.2870221241003,48.9955048082028,12.));
#92074=CARTESIAN_POINT('Ctrl Pts',(-50.3045917455383,49.0051360288002,0.));
#92075=CARTESIAN_POINT('Ctrl Pts',(-50.3045917455383,49.0051360288002,12.));
#92076=CARTESIAN_POINT('Ctrl Pts',(-50.3222179165102,49.0147738256925,0.));
#92077=CARTESIAN_POINT('Ctrl Pts',(-50.3222179165102,49.0147738256925,12.));
#92078=CARTESIAN_POINT('Ctrl Pts',(-50.3399005337967,49.0244180550759,0.));
#92079=CARTESIAN_POINT('Ctrl Pts',(-50.3399005337967,49.0244180550759,12.));
#92080=CARTESIAN_POINT('Ctrl Pts',(-50.3576394894136,49.034068567401,0.));
#92081=CARTESIAN_POINT('Ctrl Pts',(-50.3576394894136,49.034068567401,12.));
#92082=CARTESIAN_POINT('Ctrl Pts',(-50.3754346667389,49.0437252024868,0.));
#92083=CARTESIAN_POINT('Ctrl Pts',(-50.3754346667389,49.0437252024868,12.));
#92084=CARTESIAN_POINT('Ctrl Pts',(-50.393285944528,49.0533877945771,0.));
#92085=CARTESIAN_POINT('Ctrl Pts',(-50.393285944528,49.0533877945771,12.));
#92086=CARTESIAN_POINT('Ctrl Pts',(-50.4111931994264,49.0630561755082,0.));
#92087=CARTESIAN_POINT('Ctrl Pts',(-50.4111931994264,49.0630561755082,12.));
#92088=CARTESIAN_POINT('Ctrl Pts',(-50.4291563088528,49.0727301783477,0.));
#92089=CARTESIAN_POINT('Ctrl Pts',(-50.4291563088528,49.0727301783477,12.));
#92090=CARTESIAN_POINT('Ctrl Pts',(-50.4471751542717,49.0824096415339,0.));
#92091=CARTESIAN_POINT('Ctrl Pts',(-50.4471751542717,49.0824096415339,12.));
#92092=CARTESIAN_POINT('Ctrl Pts',(-50.465249621057,49.0920944086973,0.));
#92093=CARTESIAN_POINT('Ctrl Pts',(-50.465249621057,49.0920944086973,12.));
#92094=CARTESIAN_POINT('Ctrl Pts',(-50.4833795969296,49.1017843266782,0.));
#92095=CARTESIAN_POINT('Ctrl Pts',(-50.4833795969296,49.1017843266782,12.));
#92096=CARTESIAN_POINT('Ctrl Pts',(-50.5015649708742,49.1114792441573,0.));
#92097=CARTESIAN_POINT('Ctrl Pts',(-50.5015649708742,49.1114792441573,12.));
#92098=CARTESIAN_POINT('Ctrl Pts',(-50.5198056318111,49.1211790099817,0.));
#92099=CARTESIAN_POINT('Ctrl Pts',(-50.5198056318111,49.1211790099817,12.));
#92100=CARTESIAN_POINT('Ctrl Pts',(-50.5381014674822,49.1308834717645,0.));
#92101=CARTESIAN_POINT('Ctrl Pts',(-50.5381014674822,49.1308834717645,12.));
#92102=CARTESIAN_POINT('Ctrl Pts',(-50.5564523650406,49.1405924766169,0.));
#92103=CARTESIAN_POINT('Ctrl Pts',(-50.5564523650406,49.1405924766169,12.));
#92104=CARTESIAN_POINT('Ctrl Pts',(-50.5748582115575,49.1503058717831,0.));
#92105=CARTESIAN_POINT('Ctrl Pts',(-50.5748582115575,49.1503058717831,12.));
#92106=CARTESIAN_POINT('Ctrl Pts',(-50.593318894516,49.1600235052613,0.));
#92107=CARTESIAN_POINT('Ctrl Pts',(-50.593318894516,49.1600235052613,12.));
#92108=CARTESIAN_POINT('Ctrl Pts',(-50.6118343023937,49.1697452265473,0.));
#92109=CARTESIAN_POINT('Ctrl Pts',(-50.6118343023937,49.1697452265473,12.));
#92110=CARTESIAN_POINT('Ctrl Pts',(-50.6304043248796,49.1794708869074,0.));
#92111=CARTESIAN_POINT('Ctrl Pts',(-50.6304043248796,49.1794708869074,12.));
#92112=CARTESIAN_POINT('Ctrl Pts',(-50.6490288525639,49.1892003389743,0.));
#92113=CARTESIAN_POINT('Ctrl Pts',(-50.6490288525639,49.1892003389743,12.));
#92114=CARTESIAN_POINT('Ctrl Pts',(-50.6677077767427,49.1989334364991,0.));
#92115=CARTESIAN_POINT('Ctrl Pts',(-50.6677077767427,49.1989334364991,12.));
#92116=CARTESIAN_POINT('Ctrl Pts',(-50.6864409891905,49.2086700340625,0.));
#92117=CARTESIAN_POINT('Ctrl Pts',(-50.6864409891905,49.2086700340625,12.));
#92118=CARTESIAN_POINT('Ctrl Pts',(-50.7052283818941,49.218409986748,0.));
#92119=CARTESIAN_POINT('Ctrl Pts',(-50.7052283818941,49.218409986748,12.));
#92120=CARTESIAN_POINT('Ctrl Pts',(-50.7240698470698,49.2281531501569,0.));
#92121=CARTESIAN_POINT('Ctrl Pts',(-50.7240698470698,49.2281531501569,12.));
#92122=CARTESIAN_POINT('Ctrl Pts',(-50.7429652772816,49.2378993805482,0.));
#92123=CARTESIAN_POINT('Ctrl Pts',(-50.7429652772816,49.2378993805482,12.));
#92124=CARTESIAN_POINT('Ctrl Pts',(-50.7619145655207,49.2476485349373,0.));
#92125=CARTESIAN_POINT('Ctrl Pts',(-50.7619145655207,49.2476485349373,12.));
#92126=CARTESIAN_POINT('Ctrl Pts',(-50.7809176052954,49.2574004712122,0.));
#92127=CARTESIAN_POINT('Ctrl Pts',(-50.7809176052954,49.2574004712122,12.));
#92128=CARTESIAN_POINT('Ctrl Pts',(-50.7999742907111,49.2671550482415,0.));
#92129=CARTESIAN_POINT('Ctrl Pts',(-50.7999742907111,49.2671550482415,12.));
#92130=CARTESIAN_POINT('Ctrl Pts',(-50.8190845164319,49.2769121258144,0.));
#92131=CARTESIAN_POINT('Ctrl Pts',(-50.8190845164319,49.2769121258144,12.));
#92132=CARTESIAN_POINT('Ctrl Pts',(-50.8382481776392,49.2866715645828,0.));
#92133=CARTESIAN_POINT('Ctrl Pts',(-50.8382481776392,49.2866715645828,12.));
#92134=CARTESIAN_POINT('Ctrl Pts',(-50.8574651699877,49.2964332260043,0.));
#92135=CARTESIAN_POINT('Ctrl Pts',(-50.8574651699877,49.2964332260043,12.));
#92136=CARTESIAN_POINT('Ctrl Pts',(-50.8767353895509,49.3061969722798,0.));
#92137=CARTESIAN_POINT('Ctrl Pts',(-50.8767353895509,49.3061969722798,12.));
#92138=CARTESIAN_POINT('Ctrl Pts',(-50.8960587327869,49.3159626663129,0.));
#92139=CARTESIAN_POINT('Ctrl Pts',(-50.8960587327869,49.3159626663129,12.));
#92140=CARTESIAN_POINT('Ctrl Pts',(-50.9154350965681,49.325730171735,0.));
#92141=CARTESIAN_POINT('Ctrl Pts',(-50.9154350965681,49.325730171735,12.));
#92142=CARTESIAN_POINT('Ctrl Pts',(-50.9348643781928,49.3354993529163,0.));
#92143=CARTESIAN_POINT('Ctrl Pts',(-50.9348643781928,49.3354993529163,12.));
#92144=CARTESIAN_POINT('Ctrl Pts',(-50.9543464753974,49.3452700749804,0.));
#92145=CARTESIAN_POINT('Ctrl Pts',(-50.9543464753974,49.3452700749804,12.));
#92146=CARTESIAN_POINT('Ctrl Pts',(-50.9738812863636,49.3550422038221,0.));
#92147=CARTESIAN_POINT('Ctrl Pts',(-50.9738812863636,49.3550422038221,12.));
#92148=CARTESIAN_POINT('Ctrl Pts',(-50.9934687097179,49.3648156061049,0.));
#92149=CARTESIAN_POINT('Ctrl Pts',(-50.9934687097179,49.3648156061049,12.));
#92150=CARTESIAN_POINT('Ctrl Pts',(-51.0131086445268,49.3745901492428,0.));
#92151=CARTESIAN_POINT('Ctrl Pts',(-51.0131086445268,49.3745901492428,12.));
#92152=CARTESIAN_POINT('Ctrl Pts',(-51.0328009902857,49.3843657013851,0.));
#92153=CARTESIAN_POINT('Ctrl Pts',(-51.0328009902857,49.3843657013851,12.));
#92154=CARTESIAN_POINT('Ctrl Pts',(-51.0525456469072,49.3941421314014,0.));
#92155=CARTESIAN_POINT('Ctrl Pts',(-51.0525456469072,49.3941421314014,12.));
#92156=CARTESIAN_POINT('Ctrl Pts',(-51.0723425146987,49.4039193088635,0.));
#92157=CARTESIAN_POINT('Ctrl Pts',(-51.0723425146987,49.4039193088635,12.));
#92158=CARTESIAN_POINT('Ctrl Pts',(-51.0921914943663,49.4136971040428,0.));
#92159=CARTESIAN_POINT('Ctrl Pts',(-51.0921914943663,49.4136971040428,12.));
#92160=CARTESIAN_POINT('Ctrl Pts',(-51.1120924870196,49.4234753879071,0.));
#92161=CARTESIAN_POINT('Ctrl Pts',(-51.1120924870196,49.4234753879071,12.));
#92162=CARTESIAN_POINT('Ctrl Pts',(-51.1320453941702,49.4332540321178,0.));
#92163=CARTESIAN_POINT('Ctrl Pts',(-51.1320453941702,49.4332540321178,12.));
#92164=CARTESIAN_POINT('Ctrl Pts',(-51.1520501177291,49.4430329090288,0.));
#92165=CARTESIAN_POINT('Ctrl Pts',(-51.1520501177291,49.4430329090288,12.));
#92166=CARTESIAN_POINT('Ctrl Pts',(-51.1721065599972,49.4528118916833,0.));
#92167=CARTESIAN_POINT('Ctrl Pts',(-51.1721065599972,49.4528118916833,12.));
#92168=CARTESIAN_POINT('Ctrl Pts',(-51.1922146236686,49.4625908538076,0.));
#92169=CARTESIAN_POINT('Ctrl Pts',(-51.1922146236686,49.4625908538076,12.));
#92170=CARTESIAN_POINT('Ctrl Pts',(-51.2123742118288,49.4723696698022,0.));
#92171=CARTESIAN_POINT('Ctrl Pts',(-51.2123742118288,49.4723696698022,12.));
#92172=CARTESIAN_POINT('Ctrl Pts',(-51.2325852279507,49.4821482147357,0.));
#92173=CARTESIAN_POINT('Ctrl Pts',(-51.2325852279507,49.4821482147357,12.));
#92174=CARTESIAN_POINT('Ctrl Pts',(-51.2528475758841,49.4919263643357,0.));
#92175=CARTESIAN_POINT('Ctrl Pts',(-51.2528475758841,49.4919263643357,12.));
#92176=CARTESIAN_POINT('Ctrl Pts',(-51.2731611598465,49.5017039949841,0.));
#92177=CARTESIAN_POINT('Ctrl Pts',(-51.2731611598465,49.5017039949841,12.));
#92178=CARTESIAN_POINT('Ctrl Pts',(-51.2935258844278,49.5114809837111,0.));
#92179=CARTESIAN_POINT('Ctrl Pts',(-51.2935258844278,49.5114809837111,12.));
#92180=CARTESIAN_POINT('Ctrl Pts',(-51.3139416545903,49.5212572081901,0.));
#92181=CARTESIAN_POINT('Ctrl Pts',(-51.3139416545903,49.5212572081901,12.));
#92182=CARTESIAN_POINT('Ctrl Pts',(-51.3344083756659,49.5310325467334,0.));
#92183=CARTESIAN_POINT('Ctrl Pts',(-51.3344083756659,49.5310325467334,12.));
#92184=CARTESIAN_POINT('Ctrl Pts',(-51.354925953347,49.5408068782871,0.));
#92185=CARTESIAN_POINT('Ctrl Pts',(-51.354925953347,49.5408068782871,12.));
#92186=CARTESIAN_POINT('Ctrl Pts',(-51.3754942936796,49.5505800824268,0.));
#92187=CARTESIAN_POINT('Ctrl Pts',(-51.3754942936796,49.5505800824268,12.));
#92188=CARTESIAN_POINT('Ctrl Pts',(-51.3961133030688,49.5603520393514,0.));
#92189=CARTESIAN_POINT('Ctrl Pts',(-51.3961133030688,49.5603520393514,12.));
#92190=CARTESIAN_POINT('Ctrl Pts',(-51.4167828882765,49.5701226298779,0.));
#92191=CARTESIAN_POINT('Ctrl Pts',(-51.4167828882765,49.5701226298779,12.));
#92192=CARTESIAN_POINT('Ctrl Pts',(-51.4375029564191,49.579891735436,0.));
#92193=CARTESIAN_POINT('Ctrl Pts',(-51.4375029564191,49.579891735436,12.));
#92194=CARTESIAN_POINT('Ctrl Pts',(-51.4582734149562,49.5896592380634,0.));
#92195=CARTESIAN_POINT('Ctrl Pts',(-51.4582734149562,49.5896592380634,12.));
#92196=CARTESIAN_POINT('Ctrl Pts',(-51.4790941716859,49.5994250204003,0.));
#92197=CARTESIAN_POINT('Ctrl Pts',(-51.4790941716859,49.5994250204003,12.));
#92198=CARTESIAN_POINT('Ctrl Pts',(-51.4999651347496,49.609188965684,0.));
#92199=CARTESIAN_POINT('Ctrl Pts',(-51.4999651347496,49.609188965684,12.));
#92200=CARTESIAN_POINT('Ctrl Pts',(-51.5208862126303,49.6189509577441,0.));
#92201=CARTESIAN_POINT('Ctrl Pts',(-51.5208862126303,49.6189509577441,12.));
#92202=CARTESIAN_POINT('Ctrl Pts',(-51.5418573141494,49.6287108809975,0.));
#92203=CARTESIAN_POINT('Ctrl Pts',(-51.5418573141494,49.6287108809975,12.));
#92204=CARTESIAN_POINT('Ctrl Pts',(-51.5628783484556,49.6384686204443,0.));
#92205=CARTESIAN_POINT('Ctrl Pts',(-51.5628783484556,49.6384686204443,12.));
#92206=CARTESIAN_POINT('Ctrl Pts',(-51.5839492250218,49.6482240616627,0.));
#92207=CARTESIAN_POINT('Ctrl Pts',(-51.5839492250218,49.6482240616627,12.));
#92208=CARTESIAN_POINT('Ctrl Pts',(-51.6050698536525,49.6579770908063,0.));
#92209=CARTESIAN_POINT('Ctrl Pts',(-51.6050698536525,49.6579770908063,12.));
#92210=CARTESIAN_POINT('Ctrl Pts',(-51.6262401444799,49.6677275945975,0.));
#92211=CARTESIAN_POINT('Ctrl Pts',(-51.6262401444799,49.6677275945975,12.));
#92212=CARTESIAN_POINT('Ctrl Pts',(-51.6474600079611,49.6774754603235,0.));
#92213=CARTESIAN_POINT('Ctrl Pts',(-51.6474600079611,49.6774754603235,12.));
#92214=CARTESIAN_POINT('Ctrl Pts',(-51.6687293548656,49.6872205758314,0.));
#92215=CARTESIAN_POINT('Ctrl Pts',(-51.6687293548656,49.6872205758314,12.));
#92216=CARTESIAN_POINT('Ctrl Pts',(-51.6900480962744,49.6969628295236,0.));
#92217=CARTESIAN_POINT('Ctrl Pts',(-51.6900480962744,49.6969628295236,12.));
#92218=CARTESIAN_POINT('Ctrl Pts',(-51.7114161435848,49.7067021103534,0.));
#92219=CARTESIAN_POINT('Ctrl Pts',(-51.7114161435848,49.7067021103534,12.));
#92220=CARTESIAN_POINT('Ctrl Pts',(-51.7328334085084,49.7164383078206,0.));
#92221=CARTESIAN_POINT('Ctrl Pts',(-51.7328334085084,49.7164383078206,12.));
#92222=CARTESIAN_POINT('Ctrl Pts',(-51.754299803068,49.7261713119672,0.));
#92223=CARTESIAN_POINT('Ctrl Pts',(-51.754299803068,49.7261713119672,12.));
#92224=CARTESIAN_POINT('Ctrl Pts',(-51.7758152395857,49.7359010133741,0.));
#92225=CARTESIAN_POINT('Ctrl Pts',(-51.7758152395857,49.7359010133741,12.));
#92226=CARTESIAN_POINT('Ctrl Pts',(-51.7973796306826,49.7456273031555,0.));
#92227=CARTESIAN_POINT('Ctrl Pts',(-51.7973796306826,49.7456273031555,12.));
#92228=CARTESIAN_POINT('Ctrl Pts',(-51.8189928892841,49.7553500729563,0.));
#92229=CARTESIAN_POINT('Ctrl Pts',(-51.8189928892841,49.7553500729563,12.));
#92230=CARTESIAN_POINT('Ctrl Pts',(-51.8406549286177,49.7650692149464,0.));
#92231=CARTESIAN_POINT('Ctrl Pts',(-51.8406549286177,49.7650692149464,12.));
#92232=CARTESIAN_POINT('Ctrl Pts',(-51.8623656622092,49.7747846218177,0.));
#92233=CARTESIAN_POINT('Ctrl Pts',(-51.8623656622092,49.7747846218177,12.));
#92234=CARTESIAN_POINT('Ctrl Pts',(-51.8841250038716,49.78449618678,0.));
#92235=CARTESIAN_POINT('Ctrl Pts',(-51.8841250038716,49.78449618678,12.));
#92236=CARTESIAN_POINT('Ctrl Pts',(-51.9059328677051,49.7942038035568,0.));
#92237=CARTESIAN_POINT('Ctrl Pts',(-51.9059328677051,49.7942038035568,12.));
#92238=CARTESIAN_POINT('Ctrl Pts',(-51.9277891681014,49.8039073663808,0.));
#92239=CARTESIAN_POINT('Ctrl Pts',(-51.9277891681014,49.8039073663808,12.));
#92240=CARTESIAN_POINT('Ctrl Pts',(-51.9496938197418,49.8136067699896,0.));
#92241=CARTESIAN_POINT('Ctrl Pts',(-51.9496938197418,49.8136067699896,12.));
#92242=CARTESIAN_POINT('Ctrl Pts',(-51.9716467375938,49.8233019096224,0.));
#92243=CARTESIAN_POINT('Ctrl Pts',(-51.9716467375938,49.8233019096224,12.));
#92244=CARTESIAN_POINT('Ctrl Pts',(-51.9936478369008,49.8329926810172,0.));
#92245=CARTESIAN_POINT('Ctrl Pts',(-51.9936478369008,49.8329926810172,12.));
#92246=CARTESIAN_POINT('Ctrl Pts',(-52.015697033182,49.8426789804068,0.));
#92247=CARTESIAN_POINT('Ctrl Pts',(-52.015697033182,49.8426789804068,12.));
#92248=CARTESIAN_POINT('Ctrl Pts',(-52.0377942422373,49.8523607045146,0.));
#92249=CARTESIAN_POINT('Ctrl Pts',(-52.0377942422373,49.8523607045146,12.));
#92250=CARTESIAN_POINT('Ctrl Pts',(-52.059939380145,49.8620377505498,0.));
#92251=CARTESIAN_POINT('Ctrl Pts',(-52.059939380145,49.8620377505498,12.));
#92252=CARTESIAN_POINT('Ctrl Pts',(-52.0821323632588,49.871710016205,0.));
#92253=CARTESIAN_POINT('Ctrl Pts',(-52.0821323632588,49.871710016205,12.));
#92254=CARTESIAN_POINT('Ctrl Pts',(-52.1043731081968,49.8813773996523,0.));
#92255=CARTESIAN_POINT('Ctrl Pts',(-52.1043731081968,49.8813773996523,12.));
#92256=CARTESIAN_POINT('Ctrl Pts',(-52.1266615318414,49.8910397995404,0.));
#92257=CARTESIAN_POINT('Ctrl Pts',(-52.1266615318414,49.8910397995404,12.));
#92258=CARTESIAN_POINT('Ctrl Pts',(-52.1489975513449,49.90069711499,0.));
#92259=CARTESIAN_POINT('Ctrl Pts',(-52.1489975513449,49.90069711499,12.));
#92260=CARTESIAN_POINT('Ctrl Pts',(-52.1713810841277,49.9103492455904,0.));
#92261=CARTESIAN_POINT('Ctrl Pts',(-52.1713810841277,49.9103492455904,12.));
#92262=CARTESIAN_POINT('Ctrl Pts',(-52.1938120478752,49.919996091396,0.));
#92263=CARTESIAN_POINT('Ctrl Pts',(-52.1938120478752,49.919996091396,12.));
#92264=CARTESIAN_POINT('Ctrl Pts',(-52.2162903605272,49.9296375529241,0.));
#92265=CARTESIAN_POINT('Ctrl Pts',(-52.2162903605272,49.9296375529241,12.));
#92266=CARTESIAN_POINT('Ctrl Pts',(-52.238815940277,49.9392735311507,0.));
#92267=CARTESIAN_POINT('Ctrl Pts',(-52.238815940277,49.9392735311507,12.));
#92268=CARTESIAN_POINT('Ctrl Pts',(-52.2613887055773,49.9489039275064,0.));
#92269=CARTESIAN_POINT('Ctrl Pts',(-52.2613887055773,49.9489039275064,12.));
#92270=CARTESIAN_POINT('Ctrl Pts',(-52.2840085751385,49.9585286438734,0.));
#92271=CARTESIAN_POINT('Ctrl Pts',(-52.2840085751385,49.9585286438734,12.));
#92272=CARTESIAN_POINT('Ctrl Pts',(-52.3066754679265,49.9681475825824,0.));
#92273=CARTESIAN_POINT('Ctrl Pts',(-52.3066754679265,49.9681475825824,12.));
#92274=CARTESIAN_POINT('Ctrl Pts',(-52.3293893031524,49.9777606464103,0.));
#92275=CARTESIAN_POINT('Ctrl Pts',(-52.3293893031524,49.9777606464103,12.));
#92276=CARTESIAN_POINT('Ctrl Pts',(-52.3521500002711,49.9873677385769,0.));
#92277=CARTESIAN_POINT('Ctrl Pts',(-52.3521500002711,49.9873677385769,12.));
#92278=CARTESIAN_POINT('Ctrl Pts',(-52.3749574789865,49.9969687627402,0.));
#92279=CARTESIAN_POINT('Ctrl Pts',(-52.3749574789865,49.9969687627402,12.));
#92280=CARTESIAN_POINT('Ctrl Pts',(-52.3978116592505,50.0065636229934,0.));
#92281=CARTESIAN_POINT('Ctrl Pts',(-52.3978116592505,50.0065636229934,12.));
#92282=CARTESIAN_POINT('Ctrl Pts',(-52.420712461261,50.0161522238619,0.));
#92283=CARTESIAN_POINT('Ctrl Pts',(-52.420712461261,50.0161522238619,12.));
#92284=CARTESIAN_POINT('Ctrl Pts',(-52.4436598054523,50.0257344703008,0.));
#92285=CARTESIAN_POINT('Ctrl Pts',(-52.4436598054523,50.0257344703008,12.));
#92286=CARTESIAN_POINT('Ctrl Pts',(-52.4666536124926,50.0353102676933,0.));
#92287=CARTESIAN_POINT('Ctrl Pts',(-52.4666536124926,50.0353102676933,12.));
#92288=CARTESIAN_POINT('Ctrl Pts',(-52.4896938032896,50.0448795218453,0.));
#92289=CARTESIAN_POINT('Ctrl Pts',(-52.4896938032896,50.0448795218453,12.));
#92290=CARTESIAN_POINT('Ctrl Pts',(-52.5127802989903,50.0544421389824,0.));
#92291=CARTESIAN_POINT('Ctrl Pts',(-52.5127802989903,50.0544421389824,12.));
#92292=CARTESIAN_POINT('Ctrl Pts',(-52.5359130209789,50.0639980257477,0.));
#92293=CARTESIAN_POINT('Ctrl Pts',(-52.5359130209789,50.0639980257477,12.));
#92294=CARTESIAN_POINT('Ctrl Pts',(-52.5590918908691,50.0735470891996,0.));
#92295=CARTESIAN_POINT('Ctrl Pts',(-52.5590918908691,50.0735470891996,12.));
#92296=CARTESIAN_POINT('Ctrl Pts',(-52.5823168304981,50.0830892368095,0.));
#92297=CARTESIAN_POINT('Ctrl Pts',(-52.5823168304981,50.0830892368095,12.));
#92298=CARTESIAN_POINT('Ctrl Pts',(-52.6055877619338,50.0926243764569,0.));
#92299=CARTESIAN_POINT('Ctrl Pts',(-52.6055877619338,50.0926243764569,12.));
#92300=CARTESIAN_POINT('Ctrl Pts',(-52.6289046074743,50.1021524164261,0.));
#92301=CARTESIAN_POINT('Ctrl Pts',(-52.6289046074743,50.1021524164261,12.));
#92302=CARTESIAN_POINT('Ctrl Pts',(-52.6522672896462,50.1116732654041,0.));
#92303=CARTESIAN_POINT('Ctrl Pts',(-52.6522672896462,50.1116732654041,12.));
#92304=CARTESIAN_POINT('Ctrl Pts',(-52.6756757311979,50.1211868324781,0.));
#92305=CARTESIAN_POINT('Ctrl Pts',(-52.6756757311979,50.1211868324781,12.));
#92306=CARTESIAN_POINT('Ctrl Pts',(-52.6991298550928,50.1306930271343,0.));
#92307=CARTESIAN_POINT('Ctrl Pts',(-52.6991298550928,50.1306930271343,12.));
#92308=CARTESIAN_POINT('Ctrl Pts',(-52.7226295845156,50.1401917592532,0.));
#92309=CARTESIAN_POINT('Ctrl Pts',(-52.7226295845156,50.1401917592532,12.));
#92310=CARTESIAN_POINT('Ctrl Pts',(-52.7461748428733,50.1496829391068,0.));
#92311=CARTESIAN_POINT('Ctrl Pts',(-52.7461748428733,50.1496829391068,12.));
#92312=CARTESIAN_POINT('Ctrl Pts',(-52.769765553794,50.1591664773561,0.));
#92313=CARTESIAN_POINT('Ctrl Pts',(-52.769765553794,50.1591664773561,12.));
#92314=CARTESIAN_POINT('Ctrl Pts',(-52.793401641121,50.1686422850493,0.));
#92315=CARTESIAN_POINT('Ctrl Pts',(-52.793401641121,50.1686422850493,12.));
#92316=CARTESIAN_POINT('Ctrl Pts',(-52.8170830289052,50.1781102736215,0.));
#92317=CARTESIAN_POINT('Ctrl Pts',(-52.8170830289052,50.1781102736215,12.));
#92318=CARTESIAN_POINT('Ctrl Pts',(-52.8408096414101,50.1875703548893,0.));
#92319=CARTESIAN_POINT('Ctrl Pts',(-52.8408096414101,50.1875703548893,12.));
#92320=CARTESIAN_POINT('Ctrl Pts',(-52.8645814031137,50.1970224410476,0.));
#92321=CARTESIAN_POINT('Ctrl Pts',(-52.8645814031137,50.1970224410476,12.));
#92322=CARTESIAN_POINT('Ctrl Pts',(-52.8883982387068,50.2064664446663,0.));
#92323=CARTESIAN_POINT('Ctrl Pts',(-52.8883982387068,50.2064664446663,12.));
#92324=CARTESIAN_POINT('Ctrl Pts',(-52.9122600730882,50.2159022786876,0.));
#92325=CARTESIAN_POINT('Ctrl Pts',(-52.9122600730882,50.2159022786876,12.));
#92326=CARTESIAN_POINT('Ctrl Pts',(-52.9361668313539,50.2253298564237,0.));
#92327=CARTESIAN_POINT('Ctrl Pts',(-52.9361668313539,50.2253298564237,12.));
#92328=CARTESIAN_POINT('Ctrl Pts',(-52.9601184388027,50.2347490915553,0.));
#92329=CARTESIAN_POINT('Ctrl Pts',(-52.9601184388027,50.2347490915553,12.));
#92330=CARTESIAN_POINT('Ctrl Pts',(-52.9841148209404,50.2441598981286,0.));
#92331=CARTESIAN_POINT('Ctrl Pts',(-52.9841148209404,50.2441598981286,12.));
#92332=CARTESIAN_POINT('Ctrl Pts',(-53.0081559034802,50.2535621905553,0.));
#92333=CARTESIAN_POINT('Ctrl Pts',(-53.0081559034802,50.2535621905553,12.));
#92334=CARTESIAN_POINT('Ctrl Pts',(-53.0322416123404,50.262955883611,0.));
#92335=CARTESIAN_POINT('Ctrl Pts',(-53.0322416123404,50.262955883611,12.));
#92336=CARTESIAN_POINT('Ctrl Pts',(-53.0563718736361,50.272340892437,0.));
#92337=CARTESIAN_POINT('Ctrl Pts',(-53.0563718736361,50.272340892437,12.));
#92338=CARTESIAN_POINT('Ctrl Pts',(-53.0805466136791,50.2817171325354,0.));
#92339=CARTESIAN_POINT('Ctrl Pts',(-53.0805466136791,50.2817171325354,12.));
#92340=CARTESIAN_POINT('Ctrl Pts',(-53.1047657589806,50.2910845197615,0.));
#92341=CARTESIAN_POINT('Ctrl Pts',(-53.1047657589806,50.2910845197615,12.));
#92342=CARTESIAN_POINT('Ctrl Pts',(-53.1290292362482,50.3004429703188,0.));
#92343=CARTESIAN_POINT('Ctrl Pts',(-53.1290292362482,50.3004429703188,12.));
#92344=CARTESIAN_POINT('Ctrl Pts',(-53.153336972382,50.3097924007535,0.));
#92345=CARTESIAN_POINT('Ctrl Pts',(-53.153336972382,50.3097924007535,12.));
#92346=CARTESIAN_POINT('Ctrl Pts',(-53.1776888944622,50.3191327279497,0.));
#92347=CARTESIAN_POINT('Ctrl Pts',(-53.1776888944622,50.3191327279497,12.));
#92348=CARTESIAN_POINT('Ctrl Pts',(-53.202084929748,50.3284638691285,0.));
#92349=CARTESIAN_POINT('Ctrl Pts',(-53.202084929748,50.3284638691285,12.));
#92350=CARTESIAN_POINT('Ctrl Pts',(-53.2265250056896,50.3377857418522,0.));
#92351=CARTESIAN_POINT('Ctrl Pts',(-53.2265250056896,50.3377857418522,12.));
#92352=CARTESIAN_POINT('Ctrl Pts',(-53.2510090499341,50.3470982640293,0.));
#92353=CARTESIAN_POINT('Ctrl Pts',(-53.2510090499341,50.3470982640293,12.));
#92354=CARTESIAN_POINT('Ctrl Pts',(-53.2755369903291,50.3564013539198,0.));
#92355=CARTESIAN_POINT('Ctrl Pts',(-53.2755369903291,50.3564013539198,12.));
#92356=CARTESIAN_POINT('Ctrl Pts',(-53.3001087549222,50.3656949301423,0.));
#92357=CARTESIAN_POINT('Ctrl Pts',(-53.3001087549222,50.3656949301423,12.));
#92358=CARTESIAN_POINT('Ctrl Pts',(-53.3247242719575,50.3749789116777,0.));
#92359=CARTESIAN_POINT('Ctrl Pts',(-53.3247242719575,50.3749789116777,12.));
#92360=CARTESIAN_POINT('Ctrl Pts',(-53.3493834698685,50.384253217845,0.));
#92361=CARTESIAN_POINT('Ctrl Pts',(-53.3493834698685,50.384253217845,12.));
#92362=CARTESIAN_POINT('Ctrl Pts',(-53.3740862772673,50.393517768283,0.));
#92363=CARTESIAN_POINT('Ctrl Pts',(-53.3740862772673,50.393517768283,12.));
#92364=CARTESIAN_POINT('Ctrl Pts',(-53.3988326229308,50.4027724829296,0.));
#92365=CARTESIAN_POINT('Ctrl Pts',(-53.3988326229308,50.4027724829296,12.));
#92366=CARTESIAN_POINT('Ctrl Pts',(-53.4236224357846,50.4120172820054,0.));
#92367=CARTESIAN_POINT('Ctrl Pts',(-53.4236224357846,50.4120172820054,12.));
#92368=CARTESIAN_POINT('Ctrl Pts',(-53.4484556448787,50.4212520859924,0.));
#92369=CARTESIAN_POINT('Ctrl Pts',(-53.4484556448787,50.4212520859924,12.));
#92370=CARTESIAN_POINT('Ctrl Pts',(-53.4733321794199,50.4304768156677,0.));
#92371=CARTESIAN_POINT('Ctrl Pts',(-53.4733321794199,50.4304768156677,12.));
#92372=CARTESIAN_POINT('Ctrl Pts',(-53.4982519688032,50.4396913921389,0.));
#92373=CARTESIAN_POINT('Ctrl Pts',(-53.4982519688032,50.4396913921389,12.));
#92374=CARTESIAN_POINT('Ctrl Pts',(-53.5232149426415,50.4488957368841,0.));
#92375=CARTESIAN_POINT('Ctrl Pts',(-53.5232149426415,50.4488957368841,12.));
#92376=CARTESIAN_POINT('Ctrl Pts',(-53.5482210307864,50.4580897717835,0.));
#92377=CARTESIAN_POINT('Ctrl Pts',(-53.5482210307864,50.4580897717835,12.));
#92378=CARTESIAN_POINT('Ctrl Pts',(-53.5732701633603,50.4672734191749,0.));
#92379=CARTESIAN_POINT('Ctrl Pts',(-53.5732701633603,50.4672734191749,12.));
#92380=CARTESIAN_POINT('Ctrl Pts',(-53.5983622707231,50.4764466018064,0.));
#92381=CARTESIAN_POINT('Ctrl Pts',(-53.5983622707231,50.4764466018064,12.));
#92382=CARTESIAN_POINT('Ctrl Pts',(-53.6234972834055,50.4856092427309,0.));
#92383=CARTESIAN_POINT('Ctrl Pts',(-53.6234972834055,50.4856092427309,12.));
#92384=CARTESIAN_POINT('Ctrl Pts',(-53.6486751320434,50.4947612652147,0.));
#92385=CARTESIAN_POINT('Ctrl Pts',(-53.6486751320434,50.4947612652147,12.));
#92386=CARTESIAN_POINT('Ctrl Pts',(-53.6738957473158,50.5039025926531,0.));
#92387=CARTESIAN_POINT('Ctrl Pts',(-53.6738957473158,50.5039025926531,12.));
#92388=CARTESIAN_POINT('Ctrl Pts',(-53.6991590598551,50.5130331484563,0.));
#92389=CARTESIAN_POINT('Ctrl Pts',(-53.6991590598551,50.5130331484563,12.));
#92390=CARTESIAN_POINT('Ctrl Pts',(-53.7244650002382,50.5221528560427,0.));
#92391=CARTESIAN_POINT('Ctrl Pts',(-53.7244650002382,50.5221528560427,12.));
#92392=CARTESIAN_POINT('Ctrl Pts',(-53.7498134991714,50.5312616390789,0.));
#92393=CARTESIAN_POINT('Ctrl Pts',(-53.7498134991714,50.5312616390789,12.));
#92394=CARTESIAN_POINT('Ctrl Pts',(-53.7752044876313,50.5403594216706,0.));
#92395=CARTESIAN_POINT('Ctrl Pts',(-53.7752044876313,50.5403594216706,12.));
#92396=CARTESIAN_POINT('Ctrl Pts',(-53.8006378970198,50.5494461285762,0.));
#92397=CARTESIAN_POINT('Ctrl Pts',(-53.8006378970198,50.5494461285762,12.));
#92398=CARTESIAN_POINT('Ctrl Pts',(-53.8261136593064,50.5585216854082,0.));
#92399=CARTESIAN_POINT('Ctrl Pts',(-53.8261136593064,50.5585216854082,12.));
#92400=CARTESIAN_POINT('Ctrl Pts',(-53.8516317071783,50.567586018852,0.));
#92401=CARTESIAN_POINT('Ctrl Pts',(-53.8516317071783,50.567586018852,12.));
#92402=CARTESIAN_POINT('Ctrl Pts',(-53.8771919737007,50.5766390561861,0.));
#92403=CARTESIAN_POINT('Ctrl Pts',(-53.8771919737007,50.5766390561861,12.));
#92404=CARTESIAN_POINT('Ctrl Pts',(-53.9027943919814,50.5856807248133,0.));
#92405=CARTESIAN_POINT('Ctrl Pts',(-53.9027943919814,50.5856807248133,12.));
#92406=CARTESIAN_POINT('Ctrl Pts',(-53.9284388947996,50.5947109517476,0.));
#92407=CARTESIAN_POINT('Ctrl Pts',(-53.9284388947996,50.5947109517476,12.));
#92408=CARTESIAN_POINT('Ctrl Pts',(-53.9541254143131,50.603729663215,0.));
#92409=CARTESIAN_POINT('Ctrl Pts',(-53.9541254143131,50.603729663215,12.));
#92410=CARTESIAN_POINT('Ctrl Pts',(-53.9798538815561,50.6127367839738,0.));
#92411=CARTESIAN_POINT('Ctrl Pts',(-53.9798538815561,50.6127367839738,12.));
#92412=CARTESIAN_POINT('Ctrl Pts',(-54.0056242268443,50.6217322378686,0.));
#92413=CARTESIAN_POINT('Ctrl Pts',(-54.0056242268443,50.6217322378686,12.));
#92414=CARTESIAN_POINT('Ctrl Pts',(-54.0314363806751,50.630715949059,0.));
#92415=CARTESIAN_POINT('Ctrl Pts',(-54.0314363806751,50.630715949059,12.));
#92416=CARTESIAN_POINT('Ctrl Pts',(-54.0572902745101,50.6396878430961,0.));
#92417=CARTESIAN_POINT('Ctrl Pts',(-54.0572902745101,50.6396878430961,12.));
#92418=CARTESIAN_POINT('Ctrl Pts',(-54.0831858415182,50.6486478479459,0.));
#92419=CARTESIAN_POINT('Ctrl Pts',(-54.0831858415182,50.6486478479459,12.));
#92420=CARTESIAN_POINT('Ctrl Pts',(-54.1091230175319,50.657595895318,0.));
#92421=CARTESIAN_POINT('Ctrl Pts',(-54.1091230175319,50.657595895318,12.));
#92422=CARTESIAN_POINT('Ctrl Pts',(-54.1351017412722,50.6665319209798,0.));
#92423=CARTESIAN_POINT('Ctrl Pts',(-54.1351017412722,50.6665319209798,12.));
#92424=CARTESIAN_POINT('Ctrl Pts',(-54.1611219522299,50.6754558618218,0.));
#92425=CARTESIAN_POINT('Ctrl Pts',(-54.1611219522299,50.6754558618218,12.));
#92426=CARTESIAN_POINT('Ctrl Pts',(-54.1871835889908,50.6843676535428,0.));
#92427=CARTESIAN_POINT('Ctrl Pts',(-54.1871835889908,50.6843676535428,12.));
#92428=CARTESIAN_POINT('Ctrl Pts',(-54.2132865872968,50.6932672279758,0.));
#92429=CARTESIAN_POINT('Ctrl Pts',(-54.2132865872968,50.6932672279758,12.));
#92430=CARTESIAN_POINT('Ctrl Pts',(-54.2394308784093,50.7021545108369,0.));
#92431=CARTESIAN_POINT('Ctrl Pts',(-54.2394308784093,50.7021545108369,12.));
#92432=CARTESIAN_POINT('Ctrl Pts',(-54.2656163868258,50.7110294185832,0.));
#92433=CARTESIAN_POINT('Ctrl Pts',(-54.2656163868258,50.7110294185832,12.));
#92434=CARTESIAN_POINT('Ctrl Pts',(-54.2918430335414,50.7198918629632,0.));
#92435=CARTESIAN_POINT('Ctrl Pts',(-54.2918430335414,50.7198918629632,12.));
#92436=CARTESIAN_POINT('Ctrl Pts',(-54.3181107400862,50.7287417566296,0.));
#92437=CARTESIAN_POINT('Ctrl Pts',(-54.3181107400862,50.7287417566296,12.));
#92438=CARTESIAN_POINT('Ctrl Pts',(-54.344419432416,50.7375790185988,0.));
#92439=CARTESIAN_POINT('Ctrl Pts',(-54.344419432416,50.7375790185988,12.));
#92440=CARTESIAN_POINT('Ctrl Pts',(-54.3707690445679,50.7464035792846,0.));
#92441=CARTESIAN_POINT('Ctrl Pts',(-54.3707690445679,50.7464035792846,12.));
#92442=CARTESIAN_POINT('Ctrl Pts',(-54.3971595231285,50.7552153869224,0.));
#92443=CARTESIAN_POINT('Ctrl Pts',(-54.3971595231285,50.7552153869224,12.));
#92444=CARTESIAN_POINT('Ctrl Pts',(-54.4235908287188,50.7640144089601,0.));
#92445=CARTESIAN_POINT('Ctrl Pts',(-54.4235908287188,50.7640144089601,12.));
#92446=CARTESIAN_POINT('Ctrl Pts',(-54.4500629335867,50.772800626886,0.));
#92447=CARTESIAN_POINT('Ctrl Pts',(-54.4500629335867,50.772800626886,12.));
#92448=CARTESIAN_POINT('Ctrl Pts',(-54.4712732428597,50.7798193515479,0.));
#92449=CARTESIAN_POINT('Ctrl Pts',(-54.4712732428597,50.7798193515479,12.));
#92450=CARTESIAN_POINT('Ctrl Pts',(-54.4871993224549,50.7850776288567,0.));
#92451=CARTESIAN_POINT('Ctrl Pts',(-54.4871993224549,50.7850776288567,12.));
#92452=CARTESIAN_POINT('Ctrl Pts',(-54.4978248630284,50.7885805844191,0.));
#92453=CARTESIAN_POINT('Ctrl Pts',(-54.4978248630284,50.7885805844191,12.));
#92454=CARTESIAN_POINT('Ctrl Pts',(-54.5031396718592,50.7903314215393,0.));
#92455=CARTESIAN_POINT('Ctrl Pts',(-54.5031396718592,50.7903314215393,12.));
#92456=CARTESIAN_POINT('',(-50.0975384783634,48.8900464144686,0.));
#92457=CARTESIAN_POINT('Ctrl Pts',(-50.0975384783634,48.8900464144686,0.));
#92458=CARTESIAN_POINT('Ctrl Pts',(-50.1009206494209,48.8919551910299,0.));
#92459=CARTESIAN_POINT('Ctrl Pts',(-50.1076907555303,48.8957735556681,0.));
#92460=CARTESIAN_POINT('Ctrl Pts',(-50.1178632066821,48.9015035371772,0.));
#92461=CARTESIAN_POINT('Ctrl Pts',(-50.1314610602286,48.9091483817797,0.));
#92462=CARTESIAN_POINT('Ctrl Pts',(-50.148516018447,48.9187125417897,0.));
#92463=CARTESIAN_POINT('Ctrl Pts',(-50.1656286003943,48.9282847698237,0.));
#92464=CARTESIAN_POINT('Ctrl Pts',(-50.1827987615659,48.9378649933116,0.));
#92465=CARTESIAN_POINT('Ctrl Pts',(-50.2000264157903,48.9474530868847,0.));
#92466=CARTESIAN_POINT('Ctrl Pts',(-50.2173114358423,48.9570488741273,0.));
#92467=CARTESIAN_POINT('Ctrl Pts',(-50.2346536715465,48.9666521500969,0.));
#92468=CARTESIAN_POINT('Ctrl Pts',(-50.252052963548,48.9762626987227,0.));
#92469=CARTESIAN_POINT('Ctrl Pts',(-50.2695091583473,48.9858803116649,0.));
#92470=CARTESIAN_POINT('Ctrl Pts',(-50.2870221241003,48.9955048082028,0.));
#92471=CARTESIAN_POINT('Ctrl Pts',(-50.3045917455383,49.0051360288002,0.));
#92472=CARTESIAN_POINT('Ctrl Pts',(-50.3222179165102,49.0147738256925,0.));
#92473=CARTESIAN_POINT('Ctrl Pts',(-50.3399005337967,49.0244180550759,0.));
#92474=CARTESIAN_POINT('Ctrl Pts',(-50.3576394894136,49.034068567401,0.));
#92475=CARTESIAN_POINT('Ctrl Pts',(-50.3754346667389,49.0437252024868,0.));
#92476=CARTESIAN_POINT('Ctrl Pts',(-50.393285944528,49.0533877945771,0.));
#92477=CARTESIAN_POINT('Ctrl Pts',(-50.4111931994264,49.0630561755082,0.));
#92478=CARTESIAN_POINT('Ctrl Pts',(-50.4291563088528,49.0727301783477,0.));
#92479=CARTESIAN_POINT('Ctrl Pts',(-50.4471751542717,49.0824096415339,0.));
#92480=CARTESIAN_POINT('Ctrl Pts',(-50.465249621057,49.0920944086973,0.));
#92481=CARTESIAN_POINT('Ctrl Pts',(-50.4833795969296,49.1017843266782,0.));
#92482=CARTESIAN_POINT('Ctrl Pts',(-50.5015649708742,49.1114792441573,0.));
#92483=CARTESIAN_POINT('Ctrl Pts',(-50.5198056318111,49.1211790099817,0.));
#92484=CARTESIAN_POINT('Ctrl Pts',(-50.5381014674822,49.1308834717645,0.));
#92485=CARTESIAN_POINT('Ctrl Pts',(-50.5564523650406,49.1405924766169,0.));
#92486=CARTESIAN_POINT('Ctrl Pts',(-50.5748582115575,49.1503058717831,0.));
#92487=CARTESIAN_POINT('Ctrl Pts',(-50.593318894516,49.1600235052613,0.));
#92488=CARTESIAN_POINT('Ctrl Pts',(-50.6118343023937,49.1697452265473,0.));
#92489=CARTESIAN_POINT('Ctrl Pts',(-50.6304043248796,49.1794708869074,0.));
#92490=CARTESIAN_POINT('Ctrl Pts',(-50.6490288525639,49.1892003389743,0.));
#92491=CARTESIAN_POINT('Ctrl Pts',(-50.6677077767427,49.1989334364991,0.));
#92492=CARTESIAN_POINT('Ctrl Pts',(-50.6864409891905,49.2086700340625,0.));
#92493=CARTESIAN_POINT('Ctrl Pts',(-50.7052283818941,49.218409986748,0.));
#92494=CARTESIAN_POINT('Ctrl Pts',(-50.7240698470698,49.2281531501569,0.));
#92495=CARTESIAN_POINT('Ctrl Pts',(-50.7429652772816,49.2378993805482,0.));
#92496=CARTESIAN_POINT('Ctrl Pts',(-50.7619145655207,49.2476485349373,0.));
#92497=CARTESIAN_POINT('Ctrl Pts',(-50.7809176052954,49.2574004712122,0.));
#92498=CARTESIAN_POINT('Ctrl Pts',(-50.7999742907111,49.2671550482415,0.));
#92499=CARTESIAN_POINT('Ctrl Pts',(-50.8190845164319,49.2769121258144,0.));
#92500=CARTESIAN_POINT('Ctrl Pts',(-50.8382481776392,49.2866715645828,0.));
#92501=CARTESIAN_POINT('Ctrl Pts',(-50.8574651699877,49.2964332260043,0.));
#92502=CARTESIAN_POINT('Ctrl Pts',(-50.8767353895509,49.3061969722798,0.));
#92503=CARTESIAN_POINT('Ctrl Pts',(-50.8960587327869,49.3159626663129,0.));
#92504=CARTESIAN_POINT('Ctrl Pts',(-50.9154350965681,49.325730171735,0.));
#92505=CARTESIAN_POINT('Ctrl Pts',(-50.9348643781928,49.3354993529163,0.));
#92506=CARTESIAN_POINT('Ctrl Pts',(-50.9543464753974,49.3452700749804,0.));
#92507=CARTESIAN_POINT('Ctrl Pts',(-50.9738812863636,49.3550422038221,0.));
#92508=CARTESIAN_POINT('Ctrl Pts',(-50.9934687097179,49.3648156061049,0.));
#92509=CARTESIAN_POINT('Ctrl Pts',(-51.0131086445268,49.3745901492428,0.));
#92510=CARTESIAN_POINT('Ctrl Pts',(-51.0328009902857,49.3843657013851,0.));
#92511=CARTESIAN_POINT('Ctrl Pts',(-51.0525456469072,49.3941421314014,0.));
#92512=CARTESIAN_POINT('Ctrl Pts',(-51.0723425146987,49.4039193088635,0.));
#92513=CARTESIAN_POINT('Ctrl Pts',(-51.0921914943663,49.4136971040428,0.));
#92514=CARTESIAN_POINT('Ctrl Pts',(-51.1120924870196,49.4234753879071,0.));
#92515=CARTESIAN_POINT('Ctrl Pts',(-51.1320453941702,49.4332540321178,0.));
#92516=CARTESIAN_POINT('Ctrl Pts',(-51.1520501177291,49.4430329090288,0.));
#92517=CARTESIAN_POINT('Ctrl Pts',(-51.1721065599972,49.4528118916833,0.));
#92518=CARTESIAN_POINT('Ctrl Pts',(-51.1922146236686,49.4625908538076,0.));
#92519=CARTESIAN_POINT('Ctrl Pts',(-51.2123742118288,49.4723696698022,0.));
#92520=CARTESIAN_POINT('Ctrl Pts',(-51.2325852279507,49.4821482147357,0.));
#92521=CARTESIAN_POINT('Ctrl Pts',(-51.2528475758841,49.4919263643357,0.));
#92522=CARTESIAN_POINT('Ctrl Pts',(-51.2731611598465,49.5017039949841,0.));
#92523=CARTESIAN_POINT('Ctrl Pts',(-51.2935258844278,49.5114809837111,0.));
#92524=CARTESIAN_POINT('Ctrl Pts',(-51.3139416545903,49.5212572081901,0.));
#92525=CARTESIAN_POINT('Ctrl Pts',(-51.3344083756659,49.5310325467334,0.));
#92526=CARTESIAN_POINT('Ctrl Pts',(-51.354925953347,49.5408068782871,0.));
#92527=CARTESIAN_POINT('Ctrl Pts',(-51.3754942936796,49.5505800824268,0.));
#92528=CARTESIAN_POINT('Ctrl Pts',(-51.3961133030688,49.5603520393514,0.));
#92529=CARTESIAN_POINT('Ctrl Pts',(-51.4167828882765,49.5701226298779,0.));
#92530=CARTESIAN_POINT('Ctrl Pts',(-51.4375029564191,49.579891735436,0.));
#92531=CARTESIAN_POINT('Ctrl Pts',(-51.4582734149562,49.5896592380634,0.));
#92532=CARTESIAN_POINT('Ctrl Pts',(-51.4790941716859,49.5994250204003,0.));
#92533=CARTESIAN_POINT('Ctrl Pts',(-51.4999651347496,49.609188965684,0.));
#92534=CARTESIAN_POINT('Ctrl Pts',(-51.5208862126303,49.6189509577441,0.));
#92535=CARTESIAN_POINT('Ctrl Pts',(-51.5418573141494,49.6287108809975,0.));
#92536=CARTESIAN_POINT('Ctrl Pts',(-51.5628783484556,49.6384686204443,0.));
#92537=CARTESIAN_POINT('Ctrl Pts',(-51.5839492250218,49.6482240616627,0.));
#92538=CARTESIAN_POINT('Ctrl Pts',(-51.6050698536525,49.6579770908063,0.));
#92539=CARTESIAN_POINT('Ctrl Pts',(-51.6262401444799,49.6677275945975,0.));
#92540=CARTESIAN_POINT('Ctrl Pts',(-51.6474600079611,49.6774754603235,0.));
#92541=CARTESIAN_POINT('Ctrl Pts',(-51.6687293548656,49.6872205758314,0.));
#92542=CARTESIAN_POINT('Ctrl Pts',(-51.6900480962744,49.6969628295236,0.));
#92543=CARTESIAN_POINT('Ctrl Pts',(-51.7114161435848,49.7067021103534,0.));
#92544=CARTESIAN_POINT('Ctrl Pts',(-51.7328334085084,49.7164383078206,0.));
#92545=CARTESIAN_POINT('Ctrl Pts',(-51.754299803068,49.7261713119672,0.));
#92546=CARTESIAN_POINT('Ctrl Pts',(-51.7758152395857,49.7359010133741,0.));
#92547=CARTESIAN_POINT('Ctrl Pts',(-51.7973796306826,49.7456273031555,0.));
#92548=CARTESIAN_POINT('Ctrl Pts',(-51.8189928892841,49.7553500729563,0.));
#92549=CARTESIAN_POINT('Ctrl Pts',(-51.8406549286177,49.7650692149464,0.));
#92550=CARTESIAN_POINT('Ctrl Pts',(-51.8623656622092,49.7747846218177,0.));
#92551=CARTESIAN_POINT('Ctrl Pts',(-51.8841250038716,49.78449618678,0.));
#92552=CARTESIAN_POINT('Ctrl Pts',(-51.9059328677051,49.7942038035568,0.));
#92553=CARTESIAN_POINT('Ctrl Pts',(-51.9277891681014,49.8039073663808,0.));
#92554=CARTESIAN_POINT('Ctrl Pts',(-51.9496938197418,49.8136067699896,0.));
#92555=CARTESIAN_POINT('Ctrl Pts',(-51.9716467375938,49.8233019096224,0.));
#92556=CARTESIAN_POINT('Ctrl Pts',(-51.9936478369008,49.8329926810172,0.));
#92557=CARTESIAN_POINT('Ctrl Pts',(-52.015697033182,49.8426789804068,0.));
#92558=CARTESIAN_POINT('Ctrl Pts',(-52.0377942422373,49.8523607045146,0.));
#92559=CARTESIAN_POINT('Ctrl Pts',(-52.059939380145,49.8620377505498,0.));
#92560=CARTESIAN_POINT('Ctrl Pts',(-52.0821323632588,49.871710016205,0.));
#92561=CARTESIAN_POINT('Ctrl Pts',(-52.1043731081968,49.8813773996523,0.));
#92562=CARTESIAN_POINT('Ctrl Pts',(-52.1266615318414,49.8910397995404,0.));
#92563=CARTESIAN_POINT('Ctrl Pts',(-52.1489975513449,49.90069711499,0.));
#92564=CARTESIAN_POINT('Ctrl Pts',(-52.1713810841277,49.9103492455904,0.));
#92565=CARTESIAN_POINT('Ctrl Pts',(-52.1938120478752,49.919996091396,0.));
#92566=CARTESIAN_POINT('Ctrl Pts',(-52.2162903605272,49.9296375529241,0.));
#92567=CARTESIAN_POINT('Ctrl Pts',(-52.238815940277,49.9392735311507,0.));
#92568=CARTESIAN_POINT('Ctrl Pts',(-52.2613887055773,49.9489039275064,0.));
#92569=CARTESIAN_POINT('Ctrl Pts',(-52.2840085751385,49.9585286438734,0.));
#92570=CARTESIAN_POINT('Ctrl Pts',(-52.3066754679265,49.9681475825824,0.));
#92571=CARTESIAN_POINT('Ctrl Pts',(-52.3293893031524,49.9777606464103,0.));
#92572=CARTESIAN_POINT('Ctrl Pts',(-52.3521500002711,49.9873677385769,0.));
#92573=CARTESIAN_POINT('Ctrl Pts',(-52.3749574789865,49.9969687627402,0.));
#92574=CARTESIAN_POINT('Ctrl Pts',(-52.3978116592505,50.0065636229934,0.));
#92575=CARTESIAN_POINT('Ctrl Pts',(-52.420712461261,50.0161522238619,0.));
#92576=CARTESIAN_POINT('Ctrl Pts',(-52.4436598054523,50.0257344703008,0.));
#92577=CARTESIAN_POINT('Ctrl Pts',(-52.4666536124926,50.0353102676933,0.));
#92578=CARTESIAN_POINT('Ctrl Pts',(-52.4896938032896,50.0448795218453,0.));
#92579=CARTESIAN_POINT('Ctrl Pts',(-52.5127802989903,50.0544421389824,0.));
#92580=CARTESIAN_POINT('Ctrl Pts',(-52.5359130209789,50.0639980257477,0.));
#92581=CARTESIAN_POINT('Ctrl Pts',(-52.5590918908691,50.0735470891996,0.));
#92582=CARTESIAN_POINT('Ctrl Pts',(-52.5823168304981,50.0830892368095,0.));
#92583=CARTESIAN_POINT('Ctrl Pts',(-52.6055877619338,50.0926243764569,0.));
#92584=CARTESIAN_POINT('Ctrl Pts',(-52.6289046074743,50.1021524164261,0.));
#92585=CARTESIAN_POINT('Ctrl Pts',(-52.6522672896462,50.1116732654041,0.));
#92586=CARTESIAN_POINT('Ctrl Pts',(-52.6756757311979,50.1211868324781,0.));
#92587=CARTESIAN_POINT('Ctrl Pts',(-52.6991298550928,50.1306930271343,0.));
#92588=CARTESIAN_POINT('Ctrl Pts',(-52.7226295845156,50.1401917592532,0.));
#92589=CARTESIAN_POINT('Ctrl Pts',(-52.7461748428733,50.1496829391068,0.));
#92590=CARTESIAN_POINT('Ctrl Pts',(-52.769765553794,50.1591664773561,0.));
#92591=CARTESIAN_POINT('Ctrl Pts',(-52.793401641121,50.1686422850493,0.));
#92592=CARTESIAN_POINT('Ctrl Pts',(-52.8170830289052,50.1781102736215,0.));
#92593=CARTESIAN_POINT('Ctrl Pts',(-52.8408096414101,50.1875703548893,0.));
#92594=CARTESIAN_POINT('Ctrl Pts',(-52.8645814031137,50.1970224410476,0.));
#92595=CARTESIAN_POINT('Ctrl Pts',(-52.8883982387068,50.2064664446663,0.));
#92596=CARTESIAN_POINT('Ctrl Pts',(-52.9122600730882,50.2159022786876,0.));
#92597=CARTESIAN_POINT('Ctrl Pts',(-52.9361668313539,50.2253298564237,0.));
#92598=CARTESIAN_POINT('Ctrl Pts',(-52.9601184388027,50.2347490915553,0.));
#92599=CARTESIAN_POINT('Ctrl Pts',(-52.9841148209404,50.2441598981286,0.));
#92600=CARTESIAN_POINT('Ctrl Pts',(-53.0081559034802,50.2535621905553,0.));
#92601=CARTESIAN_POINT('Ctrl Pts',(-53.0322416123404,50.262955883611,0.));
#92602=CARTESIAN_POINT('Ctrl Pts',(-53.0563718736361,50.272340892437,0.));
#92603=CARTESIAN_POINT('Ctrl Pts',(-53.0805466136791,50.2817171325354,0.));
#92604=CARTESIAN_POINT('Ctrl Pts',(-53.1047657589806,50.2910845197615,0.));
#92605=CARTESIAN_POINT('Ctrl Pts',(-53.1290292362482,50.3004429703188,0.));
#92606=CARTESIAN_POINT('Ctrl Pts',(-53.153336972382,50.3097924007535,0.));
#92607=CARTESIAN_POINT('Ctrl Pts',(-53.1776888944622,50.3191327279497,0.));
#92608=CARTESIAN_POINT('Ctrl Pts',(-53.202084929748,50.3284638691285,0.));
#92609=CARTESIAN_POINT('Ctrl Pts',(-53.2265250056896,50.3377857418522,0.));
#92610=CARTESIAN_POINT('Ctrl Pts',(-53.2510090499341,50.3470982640293,0.));
#92611=CARTESIAN_POINT('Ctrl Pts',(-53.2755369903291,50.3564013539198,0.));
#92612=CARTESIAN_POINT('Ctrl Pts',(-53.3001087549222,50.3656949301423,0.));
#92613=CARTESIAN_POINT('Ctrl Pts',(-53.3247242719575,50.3749789116777,0.));
#92614=CARTESIAN_POINT('Ctrl Pts',(-53.3493834698685,50.384253217845,0.));
#92615=CARTESIAN_POINT('Ctrl Pts',(-53.3740862772673,50.393517768283,0.));
#92616=CARTESIAN_POINT('Ctrl Pts',(-53.3988326229308,50.4027724829296,0.));
#92617=CARTESIAN_POINT('Ctrl Pts',(-53.4236224357846,50.4120172820054,0.));
#92618=CARTESIAN_POINT('Ctrl Pts',(-53.4484556448787,50.4212520859924,0.));
#92619=CARTESIAN_POINT('Ctrl Pts',(-53.4733321794199,50.4304768156677,0.));
#92620=CARTESIAN_POINT('Ctrl Pts',(-53.4982519688032,50.4396913921389,0.));
#92621=CARTESIAN_POINT('Ctrl Pts',(-53.5232149426415,50.4488957368841,0.));
#92622=CARTESIAN_POINT('Ctrl Pts',(-53.5482210307864,50.4580897717835,0.));
#92623=CARTESIAN_POINT('Ctrl Pts',(-53.5732701633603,50.4672734191749,0.));
#92624=CARTESIAN_POINT('Ctrl Pts',(-53.5983622707231,50.4764466018064,0.));
#92625=CARTESIAN_POINT('Ctrl Pts',(-53.6234972834055,50.4856092427309,0.));
#92626=CARTESIAN_POINT('Ctrl Pts',(-53.6486751320434,50.4947612652147,0.));
#92627=CARTESIAN_POINT('Ctrl Pts',(-53.6738957473158,50.5039025926531,0.));
#92628=CARTESIAN_POINT('Ctrl Pts',(-53.6991590598551,50.5130331484563,0.));
#92629=CARTESIAN_POINT('Ctrl Pts',(-53.7244650002382,50.5221528560427,0.));
#92630=CARTESIAN_POINT('Ctrl Pts',(-53.7498134991714,50.5312616390789,0.));
#92631=CARTESIAN_POINT('Ctrl Pts',(-53.7752044876313,50.5403594216706,0.));
#92632=CARTESIAN_POINT('Ctrl Pts',(-53.8006378970198,50.5494461285762,0.));
#92633=CARTESIAN_POINT('Ctrl Pts',(-53.8261136593064,50.5585216854082,0.));
#92634=CARTESIAN_POINT('Ctrl Pts',(-53.8516317071783,50.567586018852,0.));
#92635=CARTESIAN_POINT('Ctrl Pts',(-53.8771919737007,50.5766390561861,0.));
#92636=CARTESIAN_POINT('Ctrl Pts',(-53.9027943919814,50.5856807248133,0.));
#92637=CARTESIAN_POINT('Ctrl Pts',(-53.9284388947996,50.5947109517476,0.));
#92638=CARTESIAN_POINT('Ctrl Pts',(-53.9541254143131,50.603729663215,0.));
#92639=CARTESIAN_POINT('Ctrl Pts',(-53.9798538815561,50.6127367839738,0.));
#92640=CARTESIAN_POINT('Ctrl Pts',(-54.0056242268443,50.6217322378686,0.));
#92641=CARTESIAN_POINT('Ctrl Pts',(-54.0314363806751,50.630715949059,0.));
#92642=CARTESIAN_POINT('Ctrl Pts',(-54.0572902745101,50.6396878430961,0.));
#92643=CARTESIAN_POINT('Ctrl Pts',(-54.0831858415182,50.6486478479459,0.));
#92644=CARTESIAN_POINT('Ctrl Pts',(-54.1091230175319,50.657595895318,0.));
#92645=CARTESIAN_POINT('Ctrl Pts',(-54.1351017412722,50.6665319209798,0.));
#92646=CARTESIAN_POINT('Ctrl Pts',(-54.1574061041882,50.6741814675382,0.));
#92647=CARTESIAN_POINT('Ctrl Pts',(-54.1745287898577,50.6800396668659,0.));
#92648=CARTESIAN_POINT('Ctrl Pts',(-54.1864514381924,50.6841118861803,0.));
#92649=CARTESIAN_POINT('Ctrl Pts',(-54.1931619277295,50.6864016965603,0.));
#92650=CARTESIAN_POINT('Ctrl Pts',(-54.1946543499978,50.6869108458688,0.));
#92651=CARTESIAN_POINT('',(-50.0975384783634,48.8900464144686,12.));
#92652=CARTESIAN_POINT('',(-50.0975384783634,48.8900464144686,0.));
#92653=CARTESIAN_POINT('Ctrl Pts',(-54.1946543499978,50.6869108458688,12.));
#92654=CARTESIAN_POINT('Ctrl Pts',(-54.1931619277295,50.6864016965603,12.));
#92655=CARTESIAN_POINT('Ctrl Pts',(-54.1864514381924,50.6841118861803,12.));
#92656=CARTESIAN_POINT('Ctrl Pts',(-54.1745287898577,50.6800396668659,12.));
#92657=CARTESIAN_POINT('Ctrl Pts',(-54.1574061041882,50.6741814675382,12.));
#92658=CARTESIAN_POINT('Ctrl Pts',(-54.1351017412722,50.6665319209798,12.));
#92659=CARTESIAN_POINT('Ctrl Pts',(-54.1091230175319,50.657595895318,12.));
#92660=CARTESIAN_POINT('Ctrl Pts',(-54.0831858415182,50.6486478479459,12.));
#92661=CARTESIAN_POINT('Ctrl Pts',(-54.0572902745101,50.6396878430961,12.));
#92662=CARTESIAN_POINT('Ctrl Pts',(-54.0314363806751,50.630715949059,12.));
#92663=CARTESIAN_POINT('Ctrl Pts',(-54.0056242268443,50.6217322378686,12.));
#92664=CARTESIAN_POINT('Ctrl Pts',(-53.9798538815561,50.6127367839738,12.));
#92665=CARTESIAN_POINT('Ctrl Pts',(-53.9541254143131,50.603729663215,12.));
#92666=CARTESIAN_POINT('Ctrl Pts',(-53.9284388947996,50.5947109517476,12.));
#92667=CARTESIAN_POINT('Ctrl Pts',(-53.9027943919814,50.5856807248133,12.));
#92668=CARTESIAN_POINT('Ctrl Pts',(-53.8771919737007,50.5766390561861,12.));
#92669=CARTESIAN_POINT('Ctrl Pts',(-53.8516317071783,50.567586018852,12.));
#92670=CARTESIAN_POINT('Ctrl Pts',(-53.8261136593064,50.5585216854082,12.));
#92671=CARTESIAN_POINT('Ctrl Pts',(-53.8006378970198,50.5494461285762,12.));
#92672=CARTESIAN_POINT('Ctrl Pts',(-53.7752044876313,50.5403594216706,12.));
#92673=CARTESIAN_POINT('Ctrl Pts',(-53.7498134991714,50.5312616390789,12.));
#92674=CARTESIAN_POINT('Ctrl Pts',(-53.7244650002382,50.5221528560427,12.));
#92675=CARTESIAN_POINT('Ctrl Pts',(-53.6991590598551,50.5130331484563,12.));
#92676=CARTESIAN_POINT('Ctrl Pts',(-53.6738957473158,50.5039025926531,12.));
#92677=CARTESIAN_POINT('Ctrl Pts',(-53.6486751320434,50.4947612652147,12.));
#92678=CARTESIAN_POINT('Ctrl Pts',(-53.6234972834055,50.4856092427309,12.));
#92679=CARTESIAN_POINT('Ctrl Pts',(-53.5983622707231,50.4764466018064,12.));
#92680=CARTESIAN_POINT('Ctrl Pts',(-53.5732701633603,50.4672734191749,12.));
#92681=CARTESIAN_POINT('Ctrl Pts',(-53.5482210307864,50.4580897717835,12.));
#92682=CARTESIAN_POINT('Ctrl Pts',(-53.5232149426415,50.4488957368841,12.));
#92683=CARTESIAN_POINT('Ctrl Pts',(-53.4982519688032,50.4396913921389,12.));
#92684=CARTESIAN_POINT('Ctrl Pts',(-53.4733321794199,50.4304768156677,12.));
#92685=CARTESIAN_POINT('Ctrl Pts',(-53.4484556448787,50.4212520859924,12.));
#92686=CARTESIAN_POINT('Ctrl Pts',(-53.4236224357846,50.4120172820054,12.));
#92687=CARTESIAN_POINT('Ctrl Pts',(-53.3988326229308,50.4027724829296,12.));
#92688=CARTESIAN_POINT('Ctrl Pts',(-53.3740862772673,50.393517768283,12.));
#92689=CARTESIAN_POINT('Ctrl Pts',(-53.3493834698685,50.384253217845,12.));
#92690=CARTESIAN_POINT('Ctrl Pts',(-53.3247242719575,50.3749789116777,12.));
#92691=CARTESIAN_POINT('Ctrl Pts',(-53.3001087549222,50.3656949301423,12.));
#92692=CARTESIAN_POINT('Ctrl Pts',(-53.2755369903291,50.3564013539198,12.));
#92693=CARTESIAN_POINT('Ctrl Pts',(-53.2510090499341,50.3470982640293,12.));
#92694=CARTESIAN_POINT('Ctrl Pts',(-53.2265250056896,50.3377857418522,12.));
#92695=CARTESIAN_POINT('Ctrl Pts',(-53.202084929748,50.3284638691285,12.));
#92696=CARTESIAN_POINT('Ctrl Pts',(-53.1776888944622,50.3191327279497,12.));
#92697=CARTESIAN_POINT('Ctrl Pts',(-53.153336972382,50.3097924007535,12.));
#92698=CARTESIAN_POINT('Ctrl Pts',(-53.1290292362482,50.3004429703188,12.));
#92699=CARTESIAN_POINT('Ctrl Pts',(-53.1047657589806,50.2910845197615,12.));
#92700=CARTESIAN_POINT('Ctrl Pts',(-53.0805466136791,50.2817171325354,12.));
#92701=CARTESIAN_POINT('Ctrl Pts',(-53.0563718736361,50.272340892437,12.));
#92702=CARTESIAN_POINT('Ctrl Pts',(-53.0322416123404,50.262955883611,12.));
#92703=CARTESIAN_POINT('Ctrl Pts',(-53.0081559034802,50.2535621905553,12.));
#92704=CARTESIAN_POINT('Ctrl Pts',(-52.9841148209404,50.2441598981286,12.));
#92705=CARTESIAN_POINT('Ctrl Pts',(-52.9601184388027,50.2347490915553,12.));
#92706=CARTESIAN_POINT('Ctrl Pts',(-52.9361668313539,50.2253298564237,12.));
#92707=CARTESIAN_POINT('Ctrl Pts',(-52.9122600730882,50.2159022786876,12.));
#92708=CARTESIAN_POINT('Ctrl Pts',(-52.8883982387068,50.2064664446663,12.));
#92709=CARTESIAN_POINT('Ctrl Pts',(-52.8645814031137,50.1970224410476,12.));
#92710=CARTESIAN_POINT('Ctrl Pts',(-52.8408096414101,50.1875703548893,12.));
#92711=CARTESIAN_POINT('Ctrl Pts',(-52.8170830289052,50.1781102736215,12.));
#92712=CARTESIAN_POINT('Ctrl Pts',(-52.793401641121,50.1686422850493,12.));
#92713=CARTESIAN_POINT('Ctrl Pts',(-52.769765553794,50.1591664773561,12.));
#92714=CARTESIAN_POINT('Ctrl Pts',(-52.7461748428733,50.1496829391068,12.));
#92715=CARTESIAN_POINT('Ctrl Pts',(-52.7226295845156,50.1401917592532,12.));
#92716=CARTESIAN_POINT('Ctrl Pts',(-52.6991298550928,50.1306930271343,12.));
#92717=CARTESIAN_POINT('Ctrl Pts',(-52.6756757311979,50.1211868324781,12.));
#92718=CARTESIAN_POINT('Ctrl Pts',(-52.6522672896462,50.1116732654041,12.));
#92719=CARTESIAN_POINT('Ctrl Pts',(-52.6289046074743,50.1021524164261,12.));
#92720=CARTESIAN_POINT('Ctrl Pts',(-52.6055877619338,50.0926243764569,12.));
#92721=CARTESIAN_POINT('Ctrl Pts',(-52.5823168304981,50.0830892368095,12.));
#92722=CARTESIAN_POINT('Ctrl Pts',(-52.5590918908691,50.0735470891996,12.));
#92723=CARTESIAN_POINT('Ctrl Pts',(-52.5359130209789,50.0639980257477,12.));
#92724=CARTESIAN_POINT('Ctrl Pts',(-52.5127802989903,50.0544421389824,12.));
#92725=CARTESIAN_POINT('Ctrl Pts',(-52.4896938032896,50.0448795218453,12.));
#92726=CARTESIAN_POINT('Ctrl Pts',(-52.4666536124926,50.0353102676933,12.));
#92727=CARTESIAN_POINT('Ctrl Pts',(-52.4436598054523,50.0257344703008,12.));
#92728=CARTESIAN_POINT('Ctrl Pts',(-52.420712461261,50.0161522238619,12.));
#92729=CARTESIAN_POINT('Ctrl Pts',(-52.3978116592505,50.0065636229934,12.));
#92730=CARTESIAN_POINT('Ctrl Pts',(-52.3749574789865,49.9969687627402,12.));
#92731=CARTESIAN_POINT('Ctrl Pts',(-52.3521500002711,49.9873677385769,12.));
#92732=CARTESIAN_POINT('Ctrl Pts',(-52.3293893031524,49.9777606464103,12.));
#92733=CARTESIAN_POINT('Ctrl Pts',(-52.3066754679265,49.9681475825824,12.));
#92734=CARTESIAN_POINT('Ctrl Pts',(-52.2840085751385,49.9585286438734,12.));
#92735=CARTESIAN_POINT('Ctrl Pts',(-52.2613887055773,49.9489039275064,12.));
#92736=CARTESIAN_POINT('Ctrl Pts',(-52.238815940277,49.9392735311507,12.));
#92737=CARTESIAN_POINT('Ctrl Pts',(-52.2162903605272,49.9296375529241,12.));
#92738=CARTESIAN_POINT('Ctrl Pts',(-52.1938120478752,49.919996091396,12.));
#92739=CARTESIAN_POINT('Ctrl Pts',(-52.1713810841277,49.9103492455904,12.));
#92740=CARTESIAN_POINT('Ctrl Pts',(-52.1489975513449,49.90069711499,12.));
#92741=CARTESIAN_POINT('Ctrl Pts',(-52.1266615318414,49.8910397995404,12.));
#92742=CARTESIAN_POINT('Ctrl Pts',(-52.1043731081968,49.8813773996523,12.));
#92743=CARTESIAN_POINT('Ctrl Pts',(-52.0821323632588,49.871710016205,12.));
#92744=CARTESIAN_POINT('Ctrl Pts',(-52.059939380145,49.8620377505498,12.));
#92745=CARTESIAN_POINT('Ctrl Pts',(-52.0377942422373,49.8523607045146,12.));
#92746=CARTESIAN_POINT('Ctrl Pts',(-52.015697033182,49.8426789804068,12.));
#92747=CARTESIAN_POINT('Ctrl Pts',(-51.9936478369008,49.8329926810172,12.));
#92748=CARTESIAN_POINT('Ctrl Pts',(-51.9716467375938,49.8233019096224,12.));
#92749=CARTESIAN_POINT('Ctrl Pts',(-51.9496938197418,49.8136067699896,12.));
#92750=CARTESIAN_POINT('Ctrl Pts',(-51.9277891681014,49.8039073663808,12.));
#92751=CARTESIAN_POINT('Ctrl Pts',(-51.9059328677051,49.7942038035568,12.));
#92752=CARTESIAN_POINT('Ctrl Pts',(-51.8841250038716,49.78449618678,12.));
#92753=CARTESIAN_POINT('Ctrl Pts',(-51.8623656622092,49.7747846218177,12.));
#92754=CARTESIAN_POINT('Ctrl Pts',(-51.8406549286177,49.7650692149464,12.));
#92755=CARTESIAN_POINT('Ctrl Pts',(-51.8189928892841,49.7553500729563,12.));
#92756=CARTESIAN_POINT('Ctrl Pts',(-51.7973796306826,49.7456273031555,12.));
#92757=CARTESIAN_POINT('Ctrl Pts',(-51.7758152395857,49.7359010133741,12.));
#92758=CARTESIAN_POINT('Ctrl Pts',(-51.754299803068,49.7261713119672,12.));
#92759=CARTESIAN_POINT('Ctrl Pts',(-51.7328334085084,49.7164383078206,12.));
#92760=CARTESIAN_POINT('Ctrl Pts',(-51.7114161435848,49.7067021103534,12.));
#92761=CARTESIAN_POINT('Ctrl Pts',(-51.6900480962744,49.6969628295236,12.));
#92762=CARTESIAN_POINT('Ctrl Pts',(-51.6687293548656,49.6872205758314,12.));
#92763=CARTESIAN_POINT('Ctrl Pts',(-51.6474600079611,49.6774754603235,12.));
#92764=CARTESIAN_POINT('Ctrl Pts',(-51.6262401444799,49.6677275945975,12.));
#92765=CARTESIAN_POINT('Ctrl Pts',(-51.6050698536525,49.6579770908063,12.));
#92766=CARTESIAN_POINT('Ctrl Pts',(-51.5839492250218,49.6482240616627,12.));
#92767=CARTESIAN_POINT('Ctrl Pts',(-51.5628783484556,49.6384686204443,12.));
#92768=CARTESIAN_POINT('Ctrl Pts',(-51.5418573141494,49.6287108809975,12.));
#92769=CARTESIAN_POINT('Ctrl Pts',(-51.5208862126303,49.6189509577441,12.));
#92770=CARTESIAN_POINT('Ctrl Pts',(-51.4999651347496,49.609188965684,12.));
#92771=CARTESIAN_POINT('Ctrl Pts',(-51.4790941716859,49.5994250204003,12.));
#92772=CARTESIAN_POINT('Ctrl Pts',(-51.4582734149562,49.5896592380634,12.));
#92773=CARTESIAN_POINT('Ctrl Pts',(-51.4375029564191,49.579891735436,12.));
#92774=CARTESIAN_POINT('Ctrl Pts',(-51.4167828882765,49.5701226298779,12.));
#92775=CARTESIAN_POINT('Ctrl Pts',(-51.3961133030688,49.5603520393514,12.));
#92776=CARTESIAN_POINT('Ctrl Pts',(-51.3754942936796,49.5505800824268,12.));
#92777=CARTESIAN_POINT('Ctrl Pts',(-51.354925953347,49.5408068782871,12.));
#92778=CARTESIAN_POINT('Ctrl Pts',(-51.3344083756659,49.5310325467334,12.));
#92779=CARTESIAN_POINT('Ctrl Pts',(-51.3139416545903,49.5212572081901,12.));
#92780=CARTESIAN_POINT('Ctrl Pts',(-51.2935258844278,49.5114809837111,12.));
#92781=CARTESIAN_POINT('Ctrl Pts',(-51.2731611598465,49.5017039949841,12.));
#92782=CARTESIAN_POINT('Ctrl Pts',(-51.2528475758841,49.4919263643357,12.));
#92783=CARTESIAN_POINT('Ctrl Pts',(-51.2325852279507,49.4821482147357,12.));
#92784=CARTESIAN_POINT('Ctrl Pts',(-51.2123742118288,49.4723696698022,12.));
#92785=CARTESIAN_POINT('Ctrl Pts',(-51.1922146236686,49.4625908538076,12.));
#92786=CARTESIAN_POINT('Ctrl Pts',(-51.1721065599972,49.4528118916833,12.));
#92787=CARTESIAN_POINT('Ctrl Pts',(-51.1520501177291,49.4430329090288,12.));
#92788=CARTESIAN_POINT('Ctrl Pts',(-51.1320453941702,49.4332540321178,12.));
#92789=CARTESIAN_POINT('Ctrl Pts',(-51.1120924870196,49.4234753879071,12.));
#92790=CARTESIAN_POINT('Ctrl Pts',(-51.0921914943663,49.4136971040428,12.));
#92791=CARTESIAN_POINT('Ctrl Pts',(-51.0723425146987,49.4039193088635,12.));
#92792=CARTESIAN_POINT('Ctrl Pts',(-51.0525456469072,49.3941421314014,12.));
#92793=CARTESIAN_POINT('Ctrl Pts',(-51.0328009902857,49.3843657013851,12.));
#92794=CARTESIAN_POINT('Ctrl Pts',(-51.0131086445268,49.3745901492428,12.));
#92795=CARTESIAN_POINT('Ctrl Pts',(-50.9934687097179,49.3648156061049,12.));
#92796=CARTESIAN_POINT('Ctrl Pts',(-50.9738812863636,49.3550422038221,12.));
#92797=CARTESIAN_POINT('Ctrl Pts',(-50.9543464753974,49.3452700749804,12.));
#92798=CARTESIAN_POINT('Ctrl Pts',(-50.9348643781928,49.3354993529163,12.));
#92799=CARTESIAN_POINT('Ctrl Pts',(-50.9154350965681,49.325730171735,12.));
#92800=CARTESIAN_POINT('Ctrl Pts',(-50.8960587327869,49.3159626663129,12.));
#92801=CARTESIAN_POINT('Ctrl Pts',(-50.8767353895509,49.3061969722798,12.));
#92802=CARTESIAN_POINT('Ctrl Pts',(-50.8574651699877,49.2964332260043,12.));
#92803=CARTESIAN_POINT('Ctrl Pts',(-50.8382481776392,49.2866715645828,12.));
#92804=CARTESIAN_POINT('Ctrl Pts',(-50.8190845164319,49.2769121258144,12.));
#92805=CARTESIAN_POINT('Ctrl Pts',(-50.7999742907111,49.2671550482415,12.));
#92806=CARTESIAN_POINT('Ctrl Pts',(-50.7809176052954,49.2574004712122,12.));
#92807=CARTESIAN_POINT('Ctrl Pts',(-50.7619145655207,49.2476485349373,12.));
#92808=CARTESIAN_POINT('Ctrl Pts',(-50.7429652772816,49.2378993805482,12.));
#92809=CARTESIAN_POINT('Ctrl Pts',(-50.7240698470698,49.2281531501569,12.));
#92810=CARTESIAN_POINT('Ctrl Pts',(-50.7052283818941,49.218409986748,12.));
#92811=CARTESIAN_POINT('Ctrl Pts',(-50.6864409891905,49.2086700340625,12.));
#92812=CARTESIAN_POINT('Ctrl Pts',(-50.6677077767427,49.1989334364991,12.));
#92813=CARTESIAN_POINT('Ctrl Pts',(-50.6490288525639,49.1892003389743,12.));
#92814=CARTESIAN_POINT('Ctrl Pts',(-50.6304043248796,49.1794708869074,12.));
#92815=CARTESIAN_POINT('Ctrl Pts',(-50.6118343023937,49.1697452265473,12.));
#92816=CARTESIAN_POINT('Ctrl Pts',(-50.593318894516,49.1600235052613,12.));
#92817=CARTESIAN_POINT('Ctrl Pts',(-50.5748582115575,49.1503058717831,12.));
#92818=CARTESIAN_POINT('Ctrl Pts',(-50.5564523650406,49.1405924766169,12.));
#92819=CARTESIAN_POINT('Ctrl Pts',(-50.5381014674822,49.1308834717645,12.));
#92820=CARTESIAN_POINT('Ctrl Pts',(-50.5198056318111,49.1211790099817,12.));
#92821=CARTESIAN_POINT('Ctrl Pts',(-50.5015649708742,49.1114792441573,12.));
#92822=CARTESIAN_POINT('Ctrl Pts',(-50.4833795969296,49.1017843266782,12.));
#92823=CARTESIAN_POINT('Ctrl Pts',(-50.465249621057,49.0920944086973,12.));
#92824=CARTESIAN_POINT('Ctrl Pts',(-50.4471751542717,49.0824096415339,12.));
#92825=CARTESIAN_POINT('Ctrl Pts',(-50.4291563088528,49.0727301783477,12.));
#92826=CARTESIAN_POINT('Ctrl Pts',(-50.4111931994264,49.0630561755082,12.));
#92827=CARTESIAN_POINT('Ctrl Pts',(-50.393285944528,49.0533877945771,12.));
#92828=CARTESIAN_POINT('Ctrl Pts',(-50.3754346667389,49.0437252024868,12.));
#92829=CARTESIAN_POINT('Ctrl Pts',(-50.3576394894136,49.034068567401,12.));
#92830=CARTESIAN_POINT('Ctrl Pts',(-50.3399005337967,49.0244180550759,12.));
#92831=CARTESIAN_POINT('Ctrl Pts',(-50.3222179165102,49.0147738256925,12.));
#92832=CARTESIAN_POINT('Ctrl Pts',(-50.3045917455383,49.0051360288002,12.));
#92833=CARTESIAN_POINT('Ctrl Pts',(-50.2870221241003,48.9955048082028,12.));
#92834=CARTESIAN_POINT('Ctrl Pts',(-50.2695091583473,48.9858803116649,12.));
#92835=CARTESIAN_POINT('Ctrl Pts',(-50.252052963548,48.9762626987227,12.));
#92836=CARTESIAN_POINT('Ctrl Pts',(-50.2346536715465,48.9666521500969,12.));
#92837=CARTESIAN_POINT('Ctrl Pts',(-50.2173114358423,48.9570488741273,12.));
#92838=CARTESIAN_POINT('Ctrl Pts',(-50.2000264157903,48.9474530868847,12.));
#92839=CARTESIAN_POINT('Ctrl Pts',(-50.1827987615659,48.9378649933116,12.));
#92840=CARTESIAN_POINT('Ctrl Pts',(-50.1656286003943,48.9282847698237,12.));
#92841=CARTESIAN_POINT('Ctrl Pts',(-50.148516018447,48.9187125417897,12.));
#92842=CARTESIAN_POINT('Ctrl Pts',(-50.1314610602286,48.9091483817797,12.));
#92843=CARTESIAN_POINT('Ctrl Pts',(-50.1178632066821,48.9015035371772,12.));
#92844=CARTESIAN_POINT('Ctrl Pts',(-50.1076907555303,48.8957735556681,12.));
#92845=CARTESIAN_POINT('Ctrl Pts',(-50.1009206494209,48.8919551910299,12.));
#92846=CARTESIAN_POINT('Ctrl Pts',(-50.0975384783634,48.8900464144686,12.));
#92847=CARTESIAN_POINT('Ctrl Pts',(-55.2174072001495,49.5707719660639,-5.55111512312578E-16));
#92848=CARTESIAN_POINT('Ctrl Pts',(-55.2174072001495,49.5707719660639,4.));
#92849=CARTESIAN_POINT('Ctrl Pts',(-55.2174072001495,49.5707719660639,8.));
#92850=CARTESIAN_POINT('Ctrl Pts',(-55.2174072001495,49.5707719660639,12.));
#92851=CARTESIAN_POINT('Ctrl Pts',(-55.2618153697169,49.6712810246933,-5.55111512312578E-16));
#92852=CARTESIAN_POINT('Ctrl Pts',(-55.2618153697169,49.6712810246933,4.));
#92853=CARTESIAN_POINT('Ctrl Pts',(-55.2618153697169,49.6712810246933,8.));
#92854=CARTESIAN_POINT('Ctrl Pts',(-55.2618153697169,49.6712810246933,12.));
#92855=CARTESIAN_POINT('Ctrl Pts',(-55.2790667815473,49.8732090625342,-5.55111512312578E-16));
#92856=CARTESIAN_POINT('Ctrl Pts',(-55.2790667815473,49.8732090625342,4.));
#92857=CARTESIAN_POINT('Ctrl Pts',(-55.2790667815473,49.8732090625342,7.99999999999999));
#92858=CARTESIAN_POINT('Ctrl Pts',(-55.2790667815473,49.8732090625342,12.));
#92859=CARTESIAN_POINT('Ctrl Pts',(-55.1854902750885,50.0481613529516,-5.55111512312578E-16));
#92860=CARTESIAN_POINT('Ctrl Pts',(-55.1854902750885,50.0481613529516,4.));
#92861=CARTESIAN_POINT('Ctrl Pts',(-55.1854902750885,50.0481613529516,8.00000000000001));
#92862=CARTESIAN_POINT('Ctrl Pts',(-55.1854902750885,50.0481613529516,12.));
#92863=CARTESIAN_POINT('Ctrl Pts',(-55.1300595714123,50.1091461876225,-5.55111512312578E-16));
#92864=CARTESIAN_POINT('Ctrl Pts',(-55.1300595714123,50.1091461876225,4.));
#92865=CARTESIAN_POINT('Ctrl Pts',(-55.1300595714123,50.1091461876225,8.));
#92866=CARTESIAN_POINT('Ctrl Pts',(-55.1300595714123,50.1091461876225,12.));
#92867=CARTESIAN_POINT('',(-55.2174072001495,49.5707719660639,-2.77555756156289E-16));
#92868=CARTESIAN_POINT('',(-55.1300595714124,50.1091461876225,2.77555756156289E-16));
#92869=CARTESIAN_POINT('Ctrl Pts',(-55.2174072001495,49.5707719660639,-5.55111512312578E-16));
#92870=CARTESIAN_POINT('Ctrl Pts',(-55.2618153697169,49.6712810246933,-5.55111512312578E-16));
#92871=CARTESIAN_POINT('Ctrl Pts',(-55.2716733193343,49.7866684748881,-5.55111512312578E-16));
#92872=CARTESIAN_POINT('Ctrl Pts',(-55.2453425609388,49.8932475177609,-5.55111512312578E-16));
#92873=CARTESIAN_POINT('Ctrl Pts',(-55.2255944921423,49.9731817999155,-5.55111512312578E-16));
#92874=CARTESIAN_POINT('Ctrl Pts',(-55.1854902750885,50.0481613529516,-5.55111512312578E-16));
#92875=CARTESIAN_POINT('Ctrl Pts',(-55.1300595714123,50.1091461876225,-5.55111512312578E-16));
#92876=CARTESIAN_POINT('',(-55.1300595714124,50.1091461876225,12.));
#92877=CARTESIAN_POINT('Ctrl Pts',(-55.1300595714123,50.1091461876225,-5.55111512312578E-16));
#92878=CARTESIAN_POINT('Ctrl Pts',(-55.1300595714123,50.1091461876225,4.));
#92879=CARTESIAN_POINT('Ctrl Pts',(-55.1300595714123,50.1091461876225,8.));
#92880=CARTESIAN_POINT('Ctrl Pts',(-55.1300595714123,50.1091461876225,12.));
#92881=CARTESIAN_POINT('',(-55.2174072001495,49.5707719660639,12.));
#92882=CARTESIAN_POINT('Ctrl Pts',(-55.1300595714123,50.1091461876225,12.));
#92883=CARTESIAN_POINT('Ctrl Pts',(-55.1854902750885,50.0481613529516,12.));
#92884=CARTESIAN_POINT('Ctrl Pts',(-55.2255944921423,49.9731817999155,12.));
#92885=CARTESIAN_POINT('Ctrl Pts',(-55.2453425609388,49.8932475177609,12.));
#92886=CARTESIAN_POINT('Ctrl Pts',(-55.2716733193343,49.7866684748881,12.));
#92887=CARTESIAN_POINT('Ctrl Pts',(-55.2618153697169,49.6712810246933,12.));
#92888=CARTESIAN_POINT('Ctrl Pts',(-55.2174072001495,49.5707719660639,12.));
#92889=CARTESIAN_POINT('Ctrl Pts',(-55.2174072001495,49.5707719660639,12.));
#92890=CARTESIAN_POINT('Ctrl Pts',(-55.2174072001495,49.5707719660639,8.));
#92891=CARTESIAN_POINT('Ctrl Pts',(-55.2174072001495,49.5707719660639,4.));
#92892=CARTESIAN_POINT('Ctrl Pts',(-55.2174072001495,49.5707719660639,-5.55111512312578E-16));
#92893=CARTESIAN_POINT('Origin',(-2.7643087079898E-10,2.53167595884892E-10,
0.));
#92894=CARTESIAN_POINT('Origin',(-2.7643087079898E-10,2.53167595884892E-10,
12.));
#92895=CARTESIAN_POINT('Origin',(-2.7643087079898E-10,2.53167595884892E-10,
0.));
#92896=CARTESIAN_POINT('Ctrl Pts',(-50.1091461876247,55.1300595714104,0.));
#92897=CARTESIAN_POINT('Ctrl Pts',(-50.1091461876247,55.1300595714104,4.));
#92898=CARTESIAN_POINT('Ctrl Pts',(-50.1091461876247,55.1300595714104,8.));
#92899=CARTESIAN_POINT('Ctrl Pts',(-50.1091461876247,55.1300595714104,12.));
#92900=CARTESIAN_POINT('Ctrl Pts',(-50.0278330747241,55.2039671763175,0.));
#92901=CARTESIAN_POINT('Ctrl Pts',(-50.0278330747241,55.2039671763175,4.));
#92902=CARTESIAN_POINT('Ctrl Pts',(-50.027833074724,55.2039671763175,8.));
#92903=CARTESIAN_POINT('Ctrl Pts',(-50.027833074724,55.2039671763175,12.));
#92904=CARTESIAN_POINT('Ctrl Pts',(-49.8417173275619,55.2841761056302,0.));
#92905=CARTESIAN_POINT('Ctrl Pts',(-49.8417173275619,55.2841761056302,4.00000000000001));
#92906=CARTESIAN_POINT('Ctrl Pts',(-49.8417173275619,55.2841761056302,8.));
#92907=CARTESIAN_POINT('Ctrl Pts',(-49.8417173275619,55.2841761056302,12.));
#92908=CARTESIAN_POINT('Ctrl Pts',(-49.6461537600013,55.2507133273147,0.));
#92909=CARTESIAN_POINT('Ctrl Pts',(-49.6461537600013,55.2507133273147,4.));
#92910=CARTESIAN_POINT('Ctrl Pts',(-49.6461537600013,55.2507133273147,8.));
#92911=CARTESIAN_POINT('Ctrl Pts',(-49.6461537600013,55.2507133273147,12.));
#92912=CARTESIAN_POINT('Ctrl Pts',(-49.5707719660265,55.2174072001301,0.));
#92913=CARTESIAN_POINT('Ctrl Pts',(-49.5707719660265,55.2174072001301,4.));
#92914=CARTESIAN_POINT('Ctrl Pts',(-49.5707719660265,55.2174072001302,8.));
#92915=CARTESIAN_POINT('Ctrl Pts',(-49.5707719660265,55.2174072001302,12.));
#92916=CARTESIAN_POINT('',(-50.1091461876247,55.1300595714104,0.));
#92917=CARTESIAN_POINT('',(-49.5707719660265,55.2174072001301,0.));
#92918=CARTESIAN_POINT('Ctrl Pts',(-50.1091461876247,55.1300595714104,0.));
#92919=CARTESIAN_POINT('Ctrl Pts',(-50.0278330747241,55.2039671763175,0.));
#92920=CARTESIAN_POINT('Ctrl Pts',(-49.9214812192028,55.2498008502105,0.));
#92921=CARTESIAN_POINT('Ctrl Pts',(-49.8120443611025,55.2585172318167,0.));
#92922=CARTESIAN_POINT('Ctrl Pts',(-49.7299667175273,55.2650545180213,0.));
#92923=CARTESIAN_POINT('Ctrl Pts',(-49.6461537600013,55.2507133273147,0.));
#92924=CARTESIAN_POINT('Ctrl Pts',(-49.5707719660265,55.2174072001301,0.));
#92925=CARTESIAN_POINT('',(-49.5707719660265,55.2174072001301,12.));
#92926=CARTESIAN_POINT('Ctrl Pts',(-49.5707719660265,55.2174072001301,0.));
#92927=CARTESIAN_POINT('Ctrl Pts',(-49.5707719660265,55.2174072001301,4.));
#92928=CARTESIAN_POINT('Ctrl Pts',(-49.5707719660265,55.2174072001302,8.));
#92929=CARTESIAN_POINT('Ctrl Pts',(-49.5707719660265,55.2174072001302,12.));
#92930=CARTESIAN_POINT('',(-50.1091461876247,55.1300595714104,12.));
#92931=CARTESIAN_POINT('Ctrl Pts',(-49.5707719660265,55.2174072001302,12.));
#92932=CARTESIAN_POINT('Ctrl Pts',(-49.6461537600013,55.2507133273147,12.));
#92933=CARTESIAN_POINT('Ctrl Pts',(-49.7299667175272,55.2650545180214,12.));
#92934=CARTESIAN_POINT('Ctrl Pts',(-49.8120443611025,55.2585172318167,12.));
#92935=CARTESIAN_POINT('Ctrl Pts',(-49.9214812192028,55.2498008502105,12.));
#92936=CARTESIAN_POINT('Ctrl Pts',(-50.027833074724,55.2039671763175,12.));
#92937=CARTESIAN_POINT('Ctrl Pts',(-50.1091461876247,55.1300595714104,12.));
#92938=CARTESIAN_POINT('Ctrl Pts',(-50.1091461876247,55.1300595714104,12.));
#92939=CARTESIAN_POINT('Ctrl Pts',(-50.1091461876247,55.1300595714104,8.));
#92940=CARTESIAN_POINT('Ctrl Pts',(-50.1091461876247,55.1300595714104,4.));
#92941=CARTESIAN_POINT('Ctrl Pts',(-50.1091461876247,55.1300595714104,0.));
#92942=CARTESIAN_POINT('Ctrl Pts',(-45.6458539113724,53.0702932034641,0.));
#92943=CARTESIAN_POINT('Ctrl Pts',(-45.6458539113724,53.0702932034641,12.));
#92944=CARTESIAN_POINT('Ctrl Pts',(-45.6490568514089,53.0724894921849,0.));
#92945=CARTESIAN_POINT('Ctrl Pts',(-45.6490568514089,53.0724894921849,12.));
#92946=CARTESIAN_POINT('Ctrl Pts',(-45.6554684028145,53.0768833804193,0.));
#92947=CARTESIAN_POINT('Ctrl Pts',(-45.6554684028145,53.0768833804193,12.));
#92948=CARTESIAN_POINT('Ctrl Pts',(-45.6651027439241,53.0834781451546,0.));
#92949=CARTESIAN_POINT('Ctrl Pts',(-45.6651027439241,53.0834781451546,12.));
#92950=CARTESIAN_POINT('Ctrl Pts',(-45.6779825614231,53.0922790298409,0.));
#92951=CARTESIAN_POINT('Ctrl Pts',(-45.6779825614231,53.0922790298409,12.));
#92952=CARTESIAN_POINT('Ctrl Pts',(-45.694139048907,53.1032932328857,0.));
#92953=CARTESIAN_POINT('Ctrl Pts',(-45.694139048907,53.1032932328857,12.));
#92954=CARTESIAN_POINT('Ctrl Pts',(-45.7103522376696,53.114320495492,0.));
#92955=CARTESIAN_POINT('Ctrl Pts',(-45.7103522376696,53.114320495492,12.));
#92956=CARTESIAN_POINT('Ctrl Pts',(-45.7266220897003,53.1253607414872,0.));
#92957=CARTESIAN_POINT('Ctrl Pts',(-45.7266220897003,53.1253607414872,12.));
#92958=CARTESIAN_POINT('Ctrl Pts',(-45.7429485300823,53.1364138384693,0.));
#92959=CARTESIAN_POINT('Ctrl Pts',(-45.7429485300823,53.1364138384693,12.));
#92960=CARTESIAN_POINT('Ctrl Pts',(-45.7593314474501,53.1474795996053,0.));
#92961=CARTESIAN_POINT('Ctrl Pts',(-45.7593314474501,53.1474795996053,12.));
#92962=CARTESIAN_POINT('Ctrl Pts',(-45.7757707100618,53.1585578076444,0.));
#92963=CARTESIAN_POINT('Ctrl Pts',(-45.7757707100618,53.1585578076444,12.));
#92964=CARTESIAN_POINT('Ctrl Pts',(-45.7922661780005,53.1696482334487,0.));
#92965=CARTESIAN_POINT('Ctrl Pts',(-45.7922661780005,53.1696482334487,12.));
#92966=CARTESIAN_POINT('Ctrl Pts',(-45.808817716509,53.1807506560933,0.));
#92967=CARTESIAN_POINT('Ctrl Pts',(-45.808817716509,53.1807506560933,12.));
#92968=CARTESIAN_POINT('Ctrl Pts',(-45.8254252099957,53.1918648840541,0.));
#92969=CARTESIAN_POINT('Ctrl Pts',(-45.8254252099957,53.1918648840541,12.));
#92970=CARTESIAN_POINT('Ctrl Pts',(-45.8420885575349,53.2029907483557,0.));
#92971=CARTESIAN_POINT('Ctrl Pts',(-45.8420885575349,53.2029907483557,12.));
#92972=CARTESIAN_POINT('Ctrl Pts',(-45.8588076662582,53.2141280925439,0.));
#92973=CARTESIAN_POINT('Ctrl Pts',(-45.8588076662582,53.2141280925439,12.));
#92974=CARTESIAN_POINT('Ctrl Pts',(-45.8755824458723,53.2252767643662,0.));
#92975=CARTESIAN_POINT('Ctrl Pts',(-45.8755824458723,53.2252767643662,12.));
#92976=CARTESIAN_POINT('Ctrl Pts',(-45.892412801838,53.2364366054306,0.));
#92977=CARTESIAN_POINT('Ctrl Pts',(-45.892412801838,53.2364366054306,12.));
#92978=CARTESIAN_POINT('Ctrl Pts',(-45.9092986319377,53.2476074460017,0.));
#92979=CARTESIAN_POINT('Ctrl Pts',(-45.9092986319377,53.2476074460017,12.));
#92980=CARTESIAN_POINT('Ctrl Pts',(-45.9262398298349,53.2587891103866,0.));
#92981=CARTESIAN_POINT('Ctrl Pts',(-45.9262398298349,53.2587891103866,12.));
#92982=CARTESIAN_POINT('Ctrl Pts',(-45.9432362873008,53.2699814203105,0.));
#92983=CARTESIAN_POINT('Ctrl Pts',(-45.9432362873008,53.2699814203105,12.));
#92984=CARTESIAN_POINT('Ctrl Pts',(-45.9602878967698,53.2811841987926,0.));
#92985=CARTESIAN_POINT('Ctrl Pts',(-45.9602878967698,53.2811841987926,12.));
#92986=CARTESIAN_POINT('Ctrl Pts',(-45.9773945542384,53.292397274555,0.));
#92987=CARTESIAN_POINT('Ctrl Pts',(-45.9773945542384,53.292397274555,12.));
#92988=CARTESIAN_POINT('Ctrl Pts',(-45.9945561591453,53.3036204818329,0.));
#92989=CARTESIAN_POINT('Ctrl Pts',(-45.9945561591453,53.3036204818329,12.));
#92990=CARTESIAN_POINT('Ctrl Pts',(-46.0117726129873,53.3148536582635,0.));
#92991=CARTESIAN_POINT('Ctrl Pts',(-46.0117726129873,53.3148536582635,12.));
#92992=CARTESIAN_POINT('Ctrl Pts',(-46.02904381836,53.326096643428,0.));
#92993=CARTESIAN_POINT('Ctrl Pts',(-46.02904381836,53.326096643428,12.));
#92994=CARTESIAN_POINT('Ctrl Pts',(-46.0463696777801,53.3373492770671,0.));
#92995=CARTESIAN_POINT('Ctrl Pts',(-46.0463696777801,53.3373492770671,12.));
#92996=CARTESIAN_POINT('Ctrl Pts',(-46.0637500926982,53.3486113975901,0.));
#92997=CARTESIAN_POINT('Ctrl Pts',(-46.0637500926982,53.3486113975901,12.));
#92998=CARTESIAN_POINT('Ctrl Pts',(-46.0811849640218,53.3598828428546,0.));
#92999=CARTESIAN_POINT('Ctrl Pts',(-46.0811849640218,53.3598828428546,12.));
#93000=CARTESIAN_POINT('Ctrl Pts',(-46.0986741925656,53.3711634508437,0.));
#93001=CARTESIAN_POINT('Ctrl Pts',(-46.0986741925656,53.3711634508437,12.));
#93002=CARTESIAN_POINT('Ctrl Pts',(-46.1162176794884,53.3824530603276,0.));
#93003=CARTESIAN_POINT('Ctrl Pts',(-46.1162176794884,53.3824530603276,12.));
#93004=CARTESIAN_POINT('Ctrl Pts',(-46.1338153268097,53.3937515116549,0.));
#93005=CARTESIAN_POINT('Ctrl Pts',(-46.1338153268097,53.3937515116549,12.));
#93006=CARTESIAN_POINT('Ctrl Pts',(-46.1514670376012,53.4050586470436,0.));
#93007=CARTESIAN_POINT('Ctrl Pts',(-46.1514670376012,53.4050586470436,12.));
#93008=CARTESIAN_POINT('Ctrl Pts',(-46.1691727157134,53.4163743101517,0.));
#93009=CARTESIAN_POINT('Ctrl Pts',(-46.1691727157134,53.4163743101517,12.));
#93010=CARTESIAN_POINT('Ctrl Pts',(-46.1869322656024,53.4276983458125,0.));
#93011=CARTESIAN_POINT('Ctrl Pts',(-46.1869322656024,53.4276983458125,12.));
#93012=CARTESIAN_POINT('Ctrl Pts',(-46.2047455921286,53.4390305997274,0.));
#93013=CARTESIAN_POINT('Ctrl Pts',(-46.2047455921286,53.4390305997274,12.));
#93014=CARTESIAN_POINT('Ctrl Pts',(-46.2226126003202,53.4503709181178,0.));
#93015=CARTESIAN_POINT('Ctrl Pts',(-46.2226126003202,53.4503709181178,12.));
#93016=CARTESIAN_POINT('Ctrl Pts',(-46.2405331953889,53.4617191477402,0.));
#93017=CARTESIAN_POINT('Ctrl Pts',(-46.2405331953889,53.4617191477402,12.));
#93018=CARTESIAN_POINT('Ctrl Pts',(-46.2585072828353,53.4730751360371,0.));
#93019=CARTESIAN_POINT('Ctrl Pts',(-46.2585072828353,53.4730751360371,12.));
#93020=CARTESIAN_POINT('Ctrl Pts',(-46.2765347685198,53.4844387312414,0.));
#93021=CARTESIAN_POINT('Ctrl Pts',(-46.2765347685198,53.4844387312414,12.));
#93022=CARTESIAN_POINT('Ctrl Pts',(-46.2946155587417,53.4958097825006,0.));
#93023=CARTESIAN_POINT('Ctrl Pts',(-46.2946155587417,53.4958097825006,12.));
#93024=CARTESIAN_POINT('Ctrl Pts',(-46.3127495603098,53.5071881399911,0.));
#93025=CARTESIAN_POINT('Ctrl Pts',(-46.3127495603098,53.5071881399911,12.));
#93026=CARTESIAN_POINT('Ctrl Pts',(-46.3309366805093,53.5185736548548,0.));
#93027=CARTESIAN_POINT('Ctrl Pts',(-46.3309366805093,53.5185736548548,12.));
#93028=CARTESIAN_POINT('Ctrl Pts',(-46.3491768270655,53.5299661791385,0.));
#93029=CARTESIAN_POINT('Ctrl Pts',(-46.3491768270655,53.5299661791385,12.));
#93030=CARTESIAN_POINT('Ctrl Pts',(-46.3674699081046,53.5413655657327,0.));
#93031=CARTESIAN_POINT('Ctrl Pts',(-46.3674699081046,53.5413655657327,12.));
#93032=CARTESIAN_POINT('Ctrl Pts',(-46.3858158321059,53.5527716683047,0.));
#93033=CARTESIAN_POINT('Ctrl Pts',(-46.3858158321059,53.5527716683047,12.));
#93034=CARTESIAN_POINT('Ctrl Pts',(-46.4042145078701,53.5641843412559,0.));
#93035=CARTESIAN_POINT('Ctrl Pts',(-46.4042145078701,53.5641843412559,12.));
#93036=CARTESIAN_POINT('Ctrl Pts',(-46.4226658445474,53.5756034397481,0.));
#93037=CARTESIAN_POINT('Ctrl Pts',(-46.4226658445474,53.5756034397481,12.));
#93038=CARTESIAN_POINT('Ctrl Pts',(-46.4411697516478,53.5870288197166,0.));
#93039=CARTESIAN_POINT('Ctrl Pts',(-46.4411697516478,53.5870288197166,12.));
#93040=CARTESIAN_POINT('Ctrl Pts',(-46.459726139052,53.5984603378855,0.));
#93041=CARTESIAN_POINT('Ctrl Pts',(-46.459726139052,53.5984603378855,12.));
#93042=CARTESIAN_POINT('Ctrl Pts',(-46.4783349170173,53.6098978517859,0.));
#93043=CARTESIAN_POINT('Ctrl Pts',(-46.4783349170173,53.6098978517859,12.));
#93044=CARTESIAN_POINT('Ctrl Pts',(-46.496995996177,53.6213412197533,0.));
#93045=CARTESIAN_POINT('Ctrl Pts',(-46.496995996177,53.6213412197533,12.));
#93046=CARTESIAN_POINT('Ctrl Pts',(-46.5157092875373,53.6327903009094,0.));
#93047=CARTESIAN_POINT('Ctrl Pts',(-46.5157092875373,53.6327903009094,12.));
#93048=CARTESIAN_POINT('Ctrl Pts',(-46.5344747024676,53.6442449551455,0.));
#93049=CARTESIAN_POINT('Ctrl Pts',(-46.5344747024676,53.6442449551455,12.));
#93050=CARTESIAN_POINT('Ctrl Pts',(-46.5532921526901,53.6557050431071,0.));
#93051=CARTESIAN_POINT('Ctrl Pts',(-46.5532921526901,53.6557050431071,12.));
#93052=CARTESIAN_POINT('Ctrl Pts',(-46.5721615502591,53.6671704261737,0.));
#93053=CARTESIAN_POINT('Ctrl Pts',(-46.5721615502591,53.6671704261737,12.));
#93054=CARTESIAN_POINT('Ctrl Pts',(-46.5910828075653,53.678640966456,0.));
#93055=CARTESIAN_POINT('Ctrl Pts',(-46.5910828075653,53.678640966456,12.));
#93056=CARTESIAN_POINT('Ctrl Pts',(-46.6100558373402,53.6901165267941,0.));
#93057=CARTESIAN_POINT('Ctrl Pts',(-46.6100558373402,53.6901165267941,12.));
#93058=CARTESIAN_POINT('Ctrl Pts',(-46.6290805526559,53.701596970754,0.));
#93059=CARTESIAN_POINT('Ctrl Pts',(-46.6290805526559,53.701596970754,12.));
#93060=CARTESIAN_POINT('Ctrl Pts',(-46.6481568669216,53.7130821626263,0.));
#93061=CARTESIAN_POINT('Ctrl Pts',(-46.6481568669216,53.7130821626263,12.));
#93062=CARTESIAN_POINT('Ctrl Pts',(-46.6672846938752,53.7245719674222,0.));
#93063=CARTESIAN_POINT('Ctrl Pts',(-46.6672846938752,53.7245719674222,12.));
#93064=CARTESIAN_POINT('Ctrl Pts',(-46.6864639475863,53.7360662508677,0.));
#93065=CARTESIAN_POINT('Ctrl Pts',(-46.6864639475863,53.7360662508677,12.));
#93066=CARTESIAN_POINT('Ctrl Pts',(-46.7056945424559,53.7475648793948,0.));
#93067=CARTESIAN_POINT('Ctrl Pts',(-46.7056945424559,53.7475648793948,12.));
#93068=CARTESIAN_POINT('Ctrl Pts',(-46.724976393213,53.7590677201344,0.));
#93069=CARTESIAN_POINT('Ctrl Pts',(-46.724976393213,53.7590677201344,12.));
#93070=CARTESIAN_POINT('Ctrl Pts',(-46.7443094149041,53.770574640907,0.));
#93071=CARTESIAN_POINT('Ctrl Pts',(-46.7443094149041,53.770574640907,12.));
#93072=CARTESIAN_POINT('Ctrl Pts',(-46.7636935228851,53.7820855102169,0.));
#93073=CARTESIAN_POINT('Ctrl Pts',(-46.7636935228851,53.7820855102169,12.));
#93074=CARTESIAN_POINT('Ctrl Pts',(-46.7831286328268,53.7936001972468,0.));
#93075=CARTESIAN_POINT('Ctrl Pts',(-46.7831286328268,53.7936001972468,12.));
#93076=CARTESIAN_POINT('Ctrl Pts',(-46.8026146607144,53.8051185718524,0.));
#93077=CARTESIAN_POINT('Ctrl Pts',(-46.8026146607144,53.8051185718524,12.));
#93078=CARTESIAN_POINT('Ctrl Pts',(-46.8221515228459,53.8166405045582,0.));
#93079=CARTESIAN_POINT('Ctrl Pts',(-46.8221515228459,53.8166405045582,12.));
#93080=CARTESIAN_POINT('Ctrl Pts',(-46.8417391358231,53.8281658665517,0.));
#93081=CARTESIAN_POINT('Ctrl Pts',(-46.8417391358231,53.8281658665517,12.));
#93082=CARTESIAN_POINT('Ctrl Pts',(-46.8613774165452,53.8396945296777,0.));
#93083=CARTESIAN_POINT('Ctrl Pts',(-46.8613774165452,53.8396945296777,12.));
#93084=CARTESIAN_POINT('Ctrl Pts',(-46.8810662822147,53.851226366434,0.));
#93085=CARTESIAN_POINT('Ctrl Pts',(-46.8810662822147,53.851226366434,12.));
#93086=CARTESIAN_POINT('Ctrl Pts',(-46.900805650336,53.8627612499648,0.));
#93087=CARTESIAN_POINT('Ctrl Pts',(-46.900805650336,53.8627612499648,12.));
#93088=CARTESIAN_POINT('Ctrl Pts',(-46.9205954387128,53.8742990540557,0.));
#93089=CARTESIAN_POINT('Ctrl Pts',(-46.9205954387128,53.8742990540557,12.));
#93090=CARTESIAN_POINT('Ctrl Pts',(-46.9404355654381,53.8858396531277,0.));
#93091=CARTESIAN_POINT('Ctrl Pts',(-46.9404355654381,53.8858396531277,12.));
#93092=CARTESIAN_POINT('Ctrl Pts',(-46.9603259488894,53.8973829222317,0.));
#93093=CARTESIAN_POINT('Ctrl Pts',(-46.9603259488894,53.8973829222317,12.));
#93094=CARTESIAN_POINT('Ctrl Pts',(-46.9802665077342,53.9089287370435,0.));
#93095=CARTESIAN_POINT('Ctrl Pts',(-46.9802665077342,53.9089287370435,12.));
#93096=CARTESIAN_POINT('Ctrl Pts',(-47.0002571609286,53.9204769738583,0.));
#93097=CARTESIAN_POINT('Ctrl Pts',(-47.0002571609286,53.9204769738583,12.));
#93098=CARTESIAN_POINT('Ctrl Pts',(-47.0202978277148,53.9320275095864,0.));
#93099=CARTESIAN_POINT('Ctrl Pts',(-47.0202978277148,53.9320275095864,12.));
#93100=CARTESIAN_POINT('Ctrl Pts',(-47.04038842761,53.9435802217468,0.));
#93101=CARTESIAN_POINT('Ctrl Pts',(-47.04038842761,53.9435802217468,12.));
#93102=CARTESIAN_POINT('Ctrl Pts',(-47.0605288804042,53.9551349884637,0.));
#93103=CARTESIAN_POINT('Ctrl Pts',(-47.0605288804042,53.9551349884637,12.));
#93104=CARTESIAN_POINT('Ctrl Pts',(-47.0807191061674,53.9666916884624,0.));
#93105=CARTESIAN_POINT('Ctrl Pts',(-47.0807191061674,53.9666916884624,12.));
#93106=CARTESIAN_POINT('Ctrl Pts',(-47.1009590252466,53.9782502010642,0.));
#93107=CARTESIAN_POINT('Ctrl Pts',(-47.1009590252466,53.9782502010642,12.));
#93108=CARTESIAN_POINT('Ctrl Pts',(-47.1212485582632,53.9898104061809,0.));
#93109=CARTESIAN_POINT('Ctrl Pts',(-47.1212485582632,53.9898104061809,12.));
#93110=CARTESIAN_POINT('Ctrl Pts',(-47.1415876261012,54.0013721843094,0.));
#93111=CARTESIAN_POINT('Ctrl Pts',(-47.1415876261012,54.0013721843094,12.));
#93112=CARTESIAN_POINT('Ctrl Pts',(-47.161976149906,54.0129354165269,0.));
#93113=CARTESIAN_POINT('Ctrl Pts',(-47.161976149906,54.0129354165269,12.));
#93114=CARTESIAN_POINT('Ctrl Pts',(-47.1824140510906,54.0244999844872,0.));
#93115=CARTESIAN_POINT('Ctrl Pts',(-47.1824140510906,54.0244999844872,12.));
#93116=CARTESIAN_POINT('Ctrl Pts',(-47.2029012513334,54.0360657704156,0.));
#93117=CARTESIAN_POINT('Ctrl Pts',(-47.2029012513334,54.0360657704156,12.));
#93118=CARTESIAN_POINT('Ctrl Pts',(-47.2234376725752,54.047632657105,0.));
#93119=CARTESIAN_POINT('Ctrl Pts',(-47.2234376725752,54.047632657105,12.));
#93120=CARTESIAN_POINT('Ctrl Pts',(-47.2440232370085,54.0592005279108,0.));
#93121=CARTESIAN_POINT('Ctrl Pts',(-47.2440232370085,54.0592005279108,12.));
#93122=CARTESIAN_POINT('Ctrl Pts',(-47.2646578670767,54.0707692667461,0.));
#93123=CARTESIAN_POINT('Ctrl Pts',(-47.2646578670767,54.0707692667461,12.));
#93124=CARTESIAN_POINT('Ctrl Pts',(-47.2853414854805,54.082338758079,0.));
#93125=CARTESIAN_POINT('Ctrl Pts',(-47.2853414854805,54.082338758079,12.));
#93126=CARTESIAN_POINT('Ctrl Pts',(-47.3060740151754,54.093908886927,0.));
#93127=CARTESIAN_POINT('Ctrl Pts',(-47.3060740151754,54.093908886927,12.));
#93128=CARTESIAN_POINT('Ctrl Pts',(-47.326855379369,54.1054795388538,0.));
#93129=CARTESIAN_POINT('Ctrl Pts',(-47.326855379369,54.1054795388538,12.));
#93130=CARTESIAN_POINT('Ctrl Pts',(-47.3476855015095,54.1170505999637,0.));
#93131=CARTESIAN_POINT('Ctrl Pts',(-47.3476855015095,54.1170505999637,12.));
#93132=CARTESIAN_POINT('Ctrl Pts',(-47.3685643052867,54.128621956898,0.));
#93133=CARTESIAN_POINT('Ctrl Pts',(-47.3685643052867,54.128621956898,12.));
#93134=CARTESIAN_POINT('Ctrl Pts',(-47.3894917146361,54.1401934968306,0.));
#93135=CARTESIAN_POINT('Ctrl Pts',(-47.3894917146361,54.1401934968306,12.));
#93136=CARTESIAN_POINT('Ctrl Pts',(-47.4104676537381,54.1517651074638,0.));
#93137=CARTESIAN_POINT('Ctrl Pts',(-47.4104676537381,54.1517651074638,12.));
#93138=CARTESIAN_POINT('Ctrl Pts',(-47.4314920470142,54.163336677024,0.));
#93139=CARTESIAN_POINT('Ctrl Pts',(-47.4314920470142,54.163336677024,12.));
#93140=CARTESIAN_POINT('Ctrl Pts',(-47.4525648191173,54.1749080942593,0.));
#93141=CARTESIAN_POINT('Ctrl Pts',(-47.4525648191173,54.1749080942593,12.));
#93142=CARTESIAN_POINT('Ctrl Pts',(-47.473685894932,54.1864792484343,0.));
#93143=CARTESIAN_POINT('Ctrl Pts',(-47.473685894932,54.1864792484343,12.));
#93144=CARTESIAN_POINT('Ctrl Pts',(-47.4948551995799,54.1980500293267,0.));
#93145=CARTESIAN_POINT('Ctrl Pts',(-47.4948551995799,54.1980500293267,12.));
#93146=CARTESIAN_POINT('Ctrl Pts',(-47.5160726584172,54.2096203272228,0.));
#93147=CARTESIAN_POINT('Ctrl Pts',(-47.5160726584172,54.2096203272228,12.));
#93148=CARTESIAN_POINT('Ctrl Pts',(-47.5373381970328,54.221190032914,0.));
#93149=CARTESIAN_POINT('Ctrl Pts',(-47.5373381970328,54.221190032914,12.));
#93150=CARTESIAN_POINT('Ctrl Pts',(-47.5586517412368,54.232759037693,0.));
#93151=CARTESIAN_POINT('Ctrl Pts',(-47.5586517412368,54.232759037693,12.));
#93152=CARTESIAN_POINT('Ctrl Pts',(-47.5800132170614,54.2443272333498,0.));
#93153=CARTESIAN_POINT('Ctrl Pts',(-47.5800132170614,54.2443272333498,12.));
#93154=CARTESIAN_POINT('Ctrl Pts',(-47.6014225507664,54.2558945121684,0.));
#93155=CARTESIAN_POINT('Ctrl Pts',(-47.6014225507664,54.2558945121684,12.));
#93156=CARTESIAN_POINT('Ctrl Pts',(-47.6228796688376,54.2674607669227,0.));
#93157=CARTESIAN_POINT('Ctrl Pts',(-47.6228796688376,54.2674607669227,12.));
#93158=CARTESIAN_POINT('Ctrl Pts',(-47.6443844979846,54.2790258908736,0.));
#93159=CARTESIAN_POINT('Ctrl Pts',(-47.6443844979846,54.2790258908736,12.));
#93160=CARTESIAN_POINT('Ctrl Pts',(-47.6659369651299,54.2905897777647,0.));
#93161=CARTESIAN_POINT('Ctrl Pts',(-47.6659369651299,54.2905897777647,12.));
#93162=CARTESIAN_POINT('Ctrl Pts',(-47.6875369974086,54.3021523218188,0.));
#93163=CARTESIAN_POINT('Ctrl Pts',(-47.6875369974086,54.3021523218188,12.));
#93164=CARTESIAN_POINT('Ctrl Pts',(-47.7091845221747,54.3137134177345,0.));
#93165=CARTESIAN_POINT('Ctrl Pts',(-47.7091845221747,54.3137134177345,12.));
#93166=CARTESIAN_POINT('Ctrl Pts',(-47.7308794669994,54.3252729606824,0.));
#93167=CARTESIAN_POINT('Ctrl Pts',(-47.7308794669994,54.3252729606824,12.));
#93168=CARTESIAN_POINT('Ctrl Pts',(-47.7526217596694,54.3368308463023,0.));
#93169=CARTESIAN_POINT('Ctrl Pts',(-47.7526217596694,54.3368308463023,12.));
#93170=CARTESIAN_POINT('Ctrl Pts',(-47.7744113281768,54.3483869706998,0.));
#93171=CARTESIAN_POINT('Ctrl Pts',(-47.7744113281768,54.3483869706998,12.));
#93172=CARTESIAN_POINT('Ctrl Pts',(-47.7962481007179,54.3599412304431,0.));
#93173=CARTESIAN_POINT('Ctrl Pts',(-47.7962481007179,54.3599412304431,12.));
#93174=CARTESIAN_POINT('Ctrl Pts',(-47.8181320056988,54.3714935225585,0.));
#93175=CARTESIAN_POINT('Ctrl Pts',(-47.8181320056988,54.3714935225585,12.));
#93176=CARTESIAN_POINT('Ctrl Pts',(-47.8400629717352,54.3830437445275,0.));
#93177=CARTESIAN_POINT('Ctrl Pts',(-47.8400629717352,54.3830437445275,12.));
#93178=CARTESIAN_POINT('Ctrl Pts',(-47.8620409276495,54.3945917942835,0.));
#93179=CARTESIAN_POINT('Ctrl Pts',(-47.8620409276495,54.3945917942835,12.));
#93180=CARTESIAN_POINT('Ctrl Pts',(-47.8840658024626,54.4061375702088,0.));
#93181=CARTESIAN_POINT('Ctrl Pts',(-47.8840658024626,54.4061375702088,12.));
#93182=CARTESIAN_POINT('Ctrl Pts',(-47.9061375253909,54.4176809711324,0.));
#93183=CARTESIAN_POINT('Ctrl Pts',(-47.9061375253909,54.4176809711324,12.));
#93184=CARTESIAN_POINT('Ctrl Pts',(-47.9282560258528,54.4292218963253,0.));
#93185=CARTESIAN_POINT('Ctrl Pts',(-47.9282560258528,54.4292218963253,12.));
#93186=CARTESIAN_POINT('Ctrl Pts',(-47.9504212334681,54.4407602454974,0.));
#93187=CARTESIAN_POINT('Ctrl Pts',(-47.9504212334681,54.4407602454974,12.));
#93188=CARTESIAN_POINT('Ctrl Pts',(-47.972633078057,54.4522959187952,0.));
#93189=CARTESIAN_POINT('Ctrl Pts',(-47.972633078057,54.4522959187952,12.));
#93190=CARTESIAN_POINT('Ctrl Pts',(-47.9948914896316,54.4638288167991,0.));
#93191=CARTESIAN_POINT('Ctrl Pts',(-47.9948914896316,54.4638288167991,12.));
#93192=CARTESIAN_POINT('Ctrl Pts',(-48.0171963983912,54.4753588405202,0.));
#93193=CARTESIAN_POINT('Ctrl Pts',(-48.0171963983912,54.4753588405202,12.));
#93194=CARTESIAN_POINT('Ctrl Pts',(-48.039547734729,54.4868858913961,0.));
#93195=CARTESIAN_POINT('Ctrl Pts',(-48.039547734729,54.4868858913961,12.));
#93196=CARTESIAN_POINT('Ctrl Pts',(-48.0619454292321,54.4984098712883,0.));
#93197=CARTESIAN_POINT('Ctrl Pts',(-48.0619454292321,54.4984098712883,12.));
#93198=CARTESIAN_POINT('Ctrl Pts',(-48.0843894126807,54.5099306824788,0.));
#93199=CARTESIAN_POINT('Ctrl Pts',(-48.0843894126807,54.5099306824788,12.));
#93200=CARTESIAN_POINT('Ctrl Pts',(-48.1068796160406,54.5214482276679,0.));
#93201=CARTESIAN_POINT('Ctrl Pts',(-48.1068796160406,54.5214482276679,12.));
#93202=CARTESIAN_POINT('Ctrl Pts',(-48.1294159704571,54.5329624099719,0.));
#93203=CARTESIAN_POINT('Ctrl Pts',(-48.1294159704571,54.5329624099719,12.));
#93204=CARTESIAN_POINT('Ctrl Pts',(-48.1519984072617,54.5444731329196,0.));
#93205=CARTESIAN_POINT('Ctrl Pts',(-48.1519984072617,54.5444731329196,12.));
#93206=CARTESIAN_POINT('Ctrl Pts',(-48.1746268579732,54.5559803004487,0.));
#93207=CARTESIAN_POINT('Ctrl Pts',(-48.1746268579732,54.5559803004487,12.));
#93208=CARTESIAN_POINT('Ctrl Pts',(-48.1973012542966,54.5674838169041,0.));
#93209=CARTESIAN_POINT('Ctrl Pts',(-48.1973012542966,54.5674838169041,12.));
#93210=CARTESIAN_POINT('Ctrl Pts',(-48.2200215281178,54.5789835870348,0.));
#93211=CARTESIAN_POINT('Ctrl Pts',(-48.2200215281178,54.5789835870348,12.));
#93212=CARTESIAN_POINT('Ctrl Pts',(-48.2427876114955,54.5904795159936,0.));
#93213=CARTESIAN_POINT('Ctrl Pts',(-48.2427876114955,54.5904795159936,12.));
#93214=CARTESIAN_POINT('Ctrl Pts',(-48.2655994366672,54.6019715093319,0.));
#93215=CARTESIAN_POINT('Ctrl Pts',(-48.2655994366672,54.6019715093319,12.));
#93216=CARTESIAN_POINT('Ctrl Pts',(-48.288456936051,54.6134594729964,0.));
#93217=CARTESIAN_POINT('Ctrl Pts',(-48.288456936051,54.6134594729964,12.));
#93218=CARTESIAN_POINT('Ctrl Pts',(-48.3113600422443,54.6249433133262,0.));
#93219=CARTESIAN_POINT('Ctrl Pts',(-48.3113600422443,54.6249433133262,12.));
#93220=CARTESIAN_POINT('Ctrl Pts',(-48.3343086880192,54.636422937049,0.));
#93221=CARTESIAN_POINT('Ctrl Pts',(-48.3343086880192,54.636422937049,12.));
#93222=CARTESIAN_POINT('Ctrl Pts',(-48.3573028063122,54.647898251279,0.));
#93223=CARTESIAN_POINT('Ctrl Pts',(-48.3573028063122,54.647898251279,12.));
#93224=CARTESIAN_POINT('Ctrl Pts',(-48.3803423302294,54.6593691635143,0.));
#93225=CARTESIAN_POINT('Ctrl Pts',(-48.3803423302294,54.6593691635143,12.));
#93226=CARTESIAN_POINT('Ctrl Pts',(-48.4034271930516,54.6708355816359,0.));
#93227=CARTESIAN_POINT('Ctrl Pts',(-48.4034271930516,54.6708355816359,12.));
#93228=CARTESIAN_POINT('Ctrl Pts',(-48.4265573282342,54.6822974139065,0.));
#93229=CARTESIAN_POINT('Ctrl Pts',(-48.4265573282342,54.6822974139065,12.));
#93230=CARTESIAN_POINT('Ctrl Pts',(-48.4497326694051,54.6937545689694,0.));
#93231=CARTESIAN_POINT('Ctrl Pts',(-48.4497326694051,54.6937545689694,12.));
#93232=CARTESIAN_POINT('Ctrl Pts',(-48.4729531503565,54.7052069558493,0.));
#93233=CARTESIAN_POINT('Ctrl Pts',(-48.4729531503565,54.7052069558493,12.));
#93234=CARTESIAN_POINT('Ctrl Pts',(-48.4962187050452,54.7166544839475,0.));
#93235=CARTESIAN_POINT('Ctrl Pts',(-48.4962187050452,54.7166544839475,12.));
#93236=CARTESIAN_POINT('Ctrl Pts',(-48.5195292675955,54.7280970630346,0.));
#93237=CARTESIAN_POINT('Ctrl Pts',(-48.5195292675955,54.7280970630346,12.));
#93238=CARTESIAN_POINT('Ctrl Pts',(-48.5428847722974,54.7395346032451,0.));
#93239=CARTESIAN_POINT('Ctrl Pts',(-48.5428847722974,54.7395346032451,12.));
#93240=CARTESIAN_POINT('Ctrl Pts',(-48.5662851536027,54.7509670150716,0.));
#93241=CARTESIAN_POINT('Ctrl Pts',(-48.5662851536027,54.7509670150716,12.));
#93242=CARTESIAN_POINT('Ctrl Pts',(-48.5897303461131,54.7623942093591,0.));
#93243=CARTESIAN_POINT('Ctrl Pts',(-48.5897303461131,54.7623942093591,12.));
#93244=CARTESIAN_POINT('Ctrl Pts',(-48.6132202845792,54.773816097304,0.));
#93245=CARTESIAN_POINT('Ctrl Pts',(-48.6132202845792,54.773816097304,12.));
#93246=CARTESIAN_POINT('Ctrl Pts',(-48.6367549039121,54.7852325904591,0.));
#93247=CARTESIAN_POINT('Ctrl Pts',(-48.6367549039121,54.7852325904591,12.));
#93248=CARTESIAN_POINT('Ctrl Pts',(-48.6603341391891,54.7966436007395,0.));
#93249=CARTESIAN_POINT('Ctrl Pts',(-48.6603341391891,54.7966436007395,12.));
#93250=CARTESIAN_POINT('Ctrl Pts',(-48.6839579256565,54.8080490404274,0.));
#93251=CARTESIAN_POINT('Ctrl Pts',(-48.6839579256565,54.8080490404274,12.));
#93252=CARTESIAN_POINT('Ctrl Pts',(-48.7076261987284,54.8194488221803,0.));
#93253=CARTESIAN_POINT('Ctrl Pts',(-48.7076261987284,54.8194488221803,12.));
#93254=CARTESIAN_POINT('Ctrl Pts',(-48.7313388939834,54.8308428590333,0.));
#93255=CARTESIAN_POINT('Ctrl Pts',(-48.7313388939834,54.8308428590333,12.));
#93256=CARTESIAN_POINT('Ctrl Pts',(-48.755095947159,54.8422310643752,0.));
#93257=CARTESIAN_POINT('Ctrl Pts',(-48.755095947159,54.8422310643752,12.));
#93258=CARTESIAN_POINT('Ctrl Pts',(-48.7788972941431,54.8536133519285,0.));
#93259=CARTESIAN_POINT('Ctrl Pts',(-48.7788972941431,54.8536133519285,12.));
#93260=CARTESIAN_POINT('Ctrl Pts',(-48.8027428709613,54.8649896357284,0.));
#93261=CARTESIAN_POINT('Ctrl Pts',(-48.8027428709613,54.8649896357284,12.));
#93262=CARTESIAN_POINT('Ctrl Pts',(-48.8266326137629,54.8763598301045,0.));
#93263=CARTESIAN_POINT('Ctrl Pts',(-48.8266326137629,54.8763598301045,12.));
#93264=CARTESIAN_POINT('Ctrl Pts',(-48.8505664587985,54.8877238496576,0.));
#93265=CARTESIAN_POINT('Ctrl Pts',(-48.8505664587985,54.8877238496576,12.));
#93266=CARTESIAN_POINT('Ctrl Pts',(-48.8745443424488,54.8990816092964,0.));
#93267=CARTESIAN_POINT('Ctrl Pts',(-48.8745443424488,54.8990816092964,12.));
#93268=CARTESIAN_POINT('Ctrl Pts',(-48.8985662012535,54.910433024275,0.));
#93269=CARTESIAN_POINT('Ctrl Pts',(-48.8985662012535,54.910433024275,12.));
#93270=CARTESIAN_POINT('Ctrl Pts',(-48.922631971937,54.9217780102357,0.));
#93271=CARTESIAN_POINT('Ctrl Pts',(-48.922631971937,54.9217780102357,12.));
#93272=CARTESIAN_POINT('Ctrl Pts',(-48.9467415914266,54.933116483242,0.));
#93273=CARTESIAN_POINT('Ctrl Pts',(-48.9467415914266,54.933116483242,12.));
#93274=CARTESIAN_POINT('Ctrl Pts',(-48.9708949968789,54.9444483598372,0.));
#93275=CARTESIAN_POINT('Ctrl Pts',(-48.9708949968789,54.9444483598372,12.));
#93276=CARTESIAN_POINT('Ctrl Pts',(-48.995092125652,54.9557735569936,0.));
#93277=CARTESIAN_POINT('Ctrl Pts',(-48.995092125652,54.9557735569936,12.));
#93278=CARTESIAN_POINT('Ctrl Pts',(-49.0193329152475,54.9670919920024,0.));
#93279=CARTESIAN_POINT('Ctrl Pts',(-49.0193329152475,54.9670919920024,12.));
#93280=CARTESIAN_POINT('Ctrl Pts',(-49.0436173032527,54.9784035823764,0.));
#93281=CARTESIAN_POINT('Ctrl Pts',(-49.0436173032527,54.9784035823764,12.));
#93282=CARTESIAN_POINT('Ctrl Pts',(-49.0679452272871,54.9897082457606,0.));
#93283=CARTESIAN_POINT('Ctrl Pts',(-49.0679452272871,54.9897082457606,12.));
#93284=CARTESIAN_POINT('Ctrl Pts',(-49.0923166249222,55.0010058998111,0.));
#93285=CARTESIAN_POINT('Ctrl Pts',(-49.0923166249222,55.0010058998111,12.));
#93286=CARTESIAN_POINT('Ctrl Pts',(-49.1167314336737,55.0122964621868,0.));
#93287=CARTESIAN_POINT('Ctrl Pts',(-49.1167314336737,55.0122964621868,12.));
#93288=CARTESIAN_POINT('Ctrl Pts',(-49.1411895911646,55.0235798508056,0.));
#93289=CARTESIAN_POINT('Ctrl Pts',(-49.1411895911646,55.0235798508056,12.));
#93290=CARTESIAN_POINT('Ctrl Pts',(-49.1656910352484,55.0348559840461,0.));
#93291=CARTESIAN_POINT('Ctrl Pts',(-49.1656910352484,55.0348559840461,12.));
#93292=CARTESIAN_POINT('Ctrl Pts',(-49.1902357041462,55.0461247809745,0.));
#93293=CARTESIAN_POINT('Ctrl Pts',(-49.1902357041462,55.0461247809745,12.));
#93294=CARTESIAN_POINT('Ctrl Pts',(-49.2148235365694,55.0573861615569,0.));
#93295=CARTESIAN_POINT('Ctrl Pts',(-49.2148235365694,55.0573861615569,12.));
#93296=CARTESIAN_POINT('Ctrl Pts',(-49.2394544718513,55.0686400468911,0.));
#93297=CARTESIAN_POINT('Ctrl Pts',(-49.2394544718513,55.0686400468911,12.));
#93298=CARTESIAN_POINT('Ctrl Pts',(-49.2641284496496,55.0798863586986,0.));
#93299=CARTESIAN_POINT('Ctrl Pts',(-49.2641284496496,55.0798863586986,12.));
#93300=CARTESIAN_POINT('Ctrl Pts',(-49.2888454096544,55.0911250188282,0.));
#93301=CARTESIAN_POINT('Ctrl Pts',(-49.2888454096544,55.0911250188282,12.));
#93302=CARTESIAN_POINT('Ctrl Pts',(-49.3136052912614,55.1023559487133,0.));
#93303=CARTESIAN_POINT('Ctrl Pts',(-49.3136052912614,55.1023559487133,12.));
#93304=CARTESIAN_POINT('Ctrl Pts',(-49.3384080333166,55.1135790689475,0.));
#93305=CARTESIAN_POINT('Ctrl Pts',(-49.3384080333166,55.1135790689475,12.));
#93306=CARTESIAN_POINT('Ctrl Pts',(-49.3632535736744,55.1247942985649,0.));
#93307=CARTESIAN_POINT('Ctrl Pts',(-49.3632535736744,55.1247942985649,12.));
#93308=CARTESIAN_POINT('Ctrl Pts',(-49.3881418495529,55.1360015556262,0.));
#93309=CARTESIAN_POINT('Ctrl Pts',(-49.3881418495529,55.1360015556262,12.));
#93310=CARTESIAN_POINT('Ctrl Pts',(-49.413072798324,55.1472007585223,0.));
#93311=CARTESIAN_POINT('Ctrl Pts',(-49.413072798324,55.1472007585223,12.));
#93312=CARTESIAN_POINT('Ctrl Pts',(-49.4380463581989,55.158391827114,0.));
#93313=CARTESIAN_POINT('Ctrl Pts',(-49.4380463581989,55.158391827114,12.));
#93314=CARTESIAN_POINT('Ctrl Pts',(-49.4630624688787,55.1695746838168,0.));
#93315=CARTESIAN_POINT('Ctrl Pts',(-49.4630624688787,55.1695746838168,12.));
#93316=CARTESIAN_POINT('Ctrl Pts',(-49.4881210723921,55.1807492550073,0.));
#93317=CARTESIAN_POINT('Ctrl Pts',(-49.4881210723921,55.1807492550073,12.));
#93318=CARTESIAN_POINT('Ctrl Pts',(-49.5132221132916,55.1919154713569,0.));
#93319=CARTESIAN_POINT('Ctrl Pts',(-49.5132221132916,55.1919154713569,12.));
#93320=CARTESIAN_POINT('Ctrl Pts',(-49.5383655367987,55.2030732647222,0.));
#93321=CARTESIAN_POINT('Ctrl Pts',(-49.5383655367987,55.2030732647222,12.));
#93322=CARTESIAN_POINT('Ctrl Pts',(-49.5635512873368,55.2142225656943,0.));
#93323=CARTESIAN_POINT('Ctrl Pts',(-49.5635512873368,55.2142225656943,12.));
#93324=CARTESIAN_POINT('Ctrl Pts',(-49.5887793068337,55.225363300765,0.));
#93325=CARTESIAN_POINT('Ctrl Pts',(-49.5887793068337,55.225363300765,12.));
#93326=CARTESIAN_POINT('Ctrl Pts',(-49.6140495332865,55.2364953899423,0.));
#93327=CARTESIAN_POINT('Ctrl Pts',(-49.6140495332865,55.2364953899423,12.));
#93328=CARTESIAN_POINT('Ctrl Pts',(-49.6393618987614,55.2476187434204,0.));
#93329=CARTESIAN_POINT('Ctrl Pts',(-49.6393618987614,55.2476187434204,12.));
#93330=CARTESIAN_POINT('Ctrl Pts',(-49.6647163322457,55.2587332663982,0.));
#93331=CARTESIAN_POINT('Ctrl Pts',(-49.6647163322457,55.2587332663982,12.));
#93332=CARTESIAN_POINT('Ctrl Pts',(-49.690112763181,55.2698388650215,0.));
#93333=CARTESIAN_POINT('Ctrl Pts',(-49.690112763181,55.2698388650215,12.));
#93334=CARTESIAN_POINT('Ctrl Pts',(-49.7155511248629,55.2809354521616,0.));
#93335=CARTESIAN_POINT('Ctrl Pts',(-49.7155511248629,55.2809354521616,12.));
#93336=CARTESIAN_POINT('Ctrl Pts',(-49.7410313576444,55.292022952748,0.));
#93337=CARTESIAN_POINT('Ctrl Pts',(-49.7410313576444,55.292022952748,12.));
#93338=CARTESIAN_POINT('Ctrl Pts',(-49.7665534128269,55.3031013105578,0.));
#93339=CARTESIAN_POINT('Ctrl Pts',(-49.7665534128269,55.3031013105578,12.));
#93340=CARTESIAN_POINT('Ctrl Pts',(-49.7921172540185,55.3141704897307,0.));
#93341=CARTESIAN_POINT('Ctrl Pts',(-49.7921172540185,55.3141704897307,12.));
#93342=CARTESIAN_POINT('Ctrl Pts',(-49.817722855186,55.3252304694066,0.));
#93343=CARTESIAN_POINT('Ctrl Pts',(-49.817722855186,55.3252304694066,12.));
#93344=CARTESIAN_POINT('Ctrl Pts',(-49.8382407306675,55.3340710859607,0.));
#93345=CARTESIAN_POINT('Ctrl Pts',(-49.8382407306675,55.3340710859607,12.));
#93346=CARTESIAN_POINT('Ctrl Pts',(-49.8536479176573,55.340697403233,0.));
#93347=CARTESIAN_POINT('Ctrl Pts',(-49.8536479176573,55.340697403233,12.));
#93348=CARTESIAN_POINT('Ctrl Pts',(-49.8639277221471,55.3451131058727,0.));
#93349=CARTESIAN_POINT('Ctrl Pts',(-49.8639277221471,55.3451131058727,12.));
#93350=CARTESIAN_POINT('Ctrl Pts',(-49.8690697110161,55.3473204966403,0.));
#93351=CARTESIAN_POINT('Ctrl Pts',(-49.8690697110161,55.3473204966403,12.));
#93352=CARTESIAN_POINT('',(-45.6458539113724,53.0702932034641,0.));
#93353=CARTESIAN_POINT('Ctrl Pts',(-45.6458539113724,53.0702932034641,0.));
#93354=CARTESIAN_POINT('Ctrl Pts',(-45.6490568514089,53.0724894921849,0.));
#93355=CARTESIAN_POINT('Ctrl Pts',(-45.6554684028145,53.0768833804193,0.));
#93356=CARTESIAN_POINT('Ctrl Pts',(-45.6651027439241,53.0834781451546,0.));
#93357=CARTESIAN_POINT('Ctrl Pts',(-45.6779825614231,53.0922790298409,0.));
#93358=CARTESIAN_POINT('Ctrl Pts',(-45.694139048907,53.1032932328857,0.));
#93359=CARTESIAN_POINT('Ctrl Pts',(-45.7103522376696,53.114320495492,0.));
#93360=CARTESIAN_POINT('Ctrl Pts',(-45.7266220897003,53.1253607414872,0.));
#93361=CARTESIAN_POINT('Ctrl Pts',(-45.7429485300823,53.1364138384693,0.));
#93362=CARTESIAN_POINT('Ctrl Pts',(-45.7593314474501,53.1474795996053,0.));
#93363=CARTESIAN_POINT('Ctrl Pts',(-45.7757707100618,53.1585578076444,0.));
#93364=CARTESIAN_POINT('Ctrl Pts',(-45.7922661780005,53.1696482334487,0.));
#93365=CARTESIAN_POINT('Ctrl Pts',(-45.808817716509,53.1807506560933,0.));
#93366=CARTESIAN_POINT('Ctrl Pts',(-45.8254252099957,53.1918648840541,0.));
#93367=CARTESIAN_POINT('Ctrl Pts',(-45.8420885575349,53.2029907483557,0.));
#93368=CARTESIAN_POINT('Ctrl Pts',(-45.8588076662582,53.2141280925439,0.));
#93369=CARTESIAN_POINT('Ctrl Pts',(-45.8755824458723,53.2252767643662,0.));
#93370=CARTESIAN_POINT('Ctrl Pts',(-45.892412801838,53.2364366054306,0.));
#93371=CARTESIAN_POINT('Ctrl Pts',(-45.9092986319377,53.2476074460017,0.));
#93372=CARTESIAN_POINT('Ctrl Pts',(-45.9262398298349,53.2587891103866,0.));
#93373=CARTESIAN_POINT('Ctrl Pts',(-45.9432362873008,53.2699814203105,0.));
#93374=CARTESIAN_POINT('Ctrl Pts',(-45.9602878967698,53.2811841987926,0.));
#93375=CARTESIAN_POINT('Ctrl Pts',(-45.9773945542384,53.292397274555,0.));
#93376=CARTESIAN_POINT('Ctrl Pts',(-45.9945561591453,53.3036204818329,0.));
#93377=CARTESIAN_POINT('Ctrl Pts',(-46.0117726129873,53.3148536582635,0.));
#93378=CARTESIAN_POINT('Ctrl Pts',(-46.02904381836,53.326096643428,0.));
#93379=CARTESIAN_POINT('Ctrl Pts',(-46.0463696777801,53.3373492770671,0.));
#93380=CARTESIAN_POINT('Ctrl Pts',(-46.0637500926982,53.3486113975901,0.));
#93381=CARTESIAN_POINT('Ctrl Pts',(-46.0811849640218,53.3598828428546,0.));
#93382=CARTESIAN_POINT('Ctrl Pts',(-46.0986741925656,53.3711634508437,0.));
#93383=CARTESIAN_POINT('Ctrl Pts',(-46.1162176794884,53.3824530603276,0.));
#93384=CARTESIAN_POINT('Ctrl Pts',(-46.1338153268097,53.3937515116549,0.));
#93385=CARTESIAN_POINT('Ctrl Pts',(-46.1514670376012,53.4050586470436,0.));
#93386=CARTESIAN_POINT('Ctrl Pts',(-46.1691727157134,53.4163743101517,0.));
#93387=CARTESIAN_POINT('Ctrl Pts',(-46.1869322656024,53.4276983458125,0.));
#93388=CARTESIAN_POINT('Ctrl Pts',(-46.2047455921286,53.4390305997274,0.));
#93389=CARTESIAN_POINT('Ctrl Pts',(-46.2226126003202,53.4503709181178,0.));
#93390=CARTESIAN_POINT('Ctrl Pts',(-46.2405331953889,53.4617191477402,0.));
#93391=CARTESIAN_POINT('Ctrl Pts',(-46.2585072828353,53.4730751360371,0.));
#93392=CARTESIAN_POINT('Ctrl Pts',(-46.2765347685198,53.4844387312414,0.));
#93393=CARTESIAN_POINT('Ctrl Pts',(-46.2946155587417,53.4958097825006,0.));
#93394=CARTESIAN_POINT('Ctrl Pts',(-46.3127495603098,53.5071881399911,0.));
#93395=CARTESIAN_POINT('Ctrl Pts',(-46.3309366805093,53.5185736548548,0.));
#93396=CARTESIAN_POINT('Ctrl Pts',(-46.3491768270655,53.5299661791385,0.));
#93397=CARTESIAN_POINT('Ctrl Pts',(-46.3674699081046,53.5413655657327,0.));
#93398=CARTESIAN_POINT('Ctrl Pts',(-46.3858158321059,53.5527716683047,0.));
#93399=CARTESIAN_POINT('Ctrl Pts',(-46.4042145078701,53.5641843412559,0.));
#93400=CARTESIAN_POINT('Ctrl Pts',(-46.4226658445474,53.5756034397481,0.));
#93401=CARTESIAN_POINT('Ctrl Pts',(-46.4411697516478,53.5870288197166,0.));
#93402=CARTESIAN_POINT('Ctrl Pts',(-46.459726139052,53.5984603378855,0.));
#93403=CARTESIAN_POINT('Ctrl Pts',(-46.4783349170173,53.6098978517859,0.));
#93404=CARTESIAN_POINT('Ctrl Pts',(-46.496995996177,53.6213412197533,0.));
#93405=CARTESIAN_POINT('Ctrl Pts',(-46.5157092875373,53.6327903009094,0.));
#93406=CARTESIAN_POINT('Ctrl Pts',(-46.5344747024676,53.6442449551455,0.));
#93407=CARTESIAN_POINT('Ctrl Pts',(-46.5532921526901,53.6557050431071,0.));
#93408=CARTESIAN_POINT('Ctrl Pts',(-46.5721615502591,53.6671704261737,0.));
#93409=CARTESIAN_POINT('Ctrl Pts',(-46.5910828075653,53.678640966456,0.));
#93410=CARTESIAN_POINT('Ctrl Pts',(-46.6100558373402,53.6901165267941,0.));
#93411=CARTESIAN_POINT('Ctrl Pts',(-46.6290805526559,53.701596970754,0.));
#93412=CARTESIAN_POINT('Ctrl Pts',(-46.6481568669216,53.7130821626263,0.));
#93413=CARTESIAN_POINT('Ctrl Pts',(-46.6672846938752,53.7245719674222,0.));
#93414=CARTESIAN_POINT('Ctrl Pts',(-46.6864639475863,53.7360662508677,0.));
#93415=CARTESIAN_POINT('Ctrl Pts',(-46.7056945424559,53.7475648793948,0.));
#93416=CARTESIAN_POINT('Ctrl Pts',(-46.724976393213,53.7590677201344,0.));
#93417=CARTESIAN_POINT('Ctrl Pts',(-46.7443094149041,53.770574640907,0.));
#93418=CARTESIAN_POINT('Ctrl Pts',(-46.7636935228851,53.7820855102169,0.));
#93419=CARTESIAN_POINT('Ctrl Pts',(-46.7831286328268,53.7936001972468,0.));
#93420=CARTESIAN_POINT('Ctrl Pts',(-46.8026146607144,53.8051185718524,0.));
#93421=CARTESIAN_POINT('Ctrl Pts',(-46.8221515228459,53.8166405045582,0.));
#93422=CARTESIAN_POINT('Ctrl Pts',(-46.8417391358231,53.8281658665517,0.));
#93423=CARTESIAN_POINT('Ctrl Pts',(-46.8613774165452,53.8396945296777,0.));
#93424=CARTESIAN_POINT('Ctrl Pts',(-46.8810662822147,53.851226366434,0.));
#93425=CARTESIAN_POINT('Ctrl Pts',(-46.900805650336,53.8627612499648,0.));
#93426=CARTESIAN_POINT('Ctrl Pts',(-46.9205954387128,53.8742990540557,0.));
#93427=CARTESIAN_POINT('Ctrl Pts',(-46.9404355654381,53.8858396531277,0.));
#93428=CARTESIAN_POINT('Ctrl Pts',(-46.9603259488894,53.8973829222317,0.));
#93429=CARTESIAN_POINT('Ctrl Pts',(-46.9802665077342,53.9089287370435,0.));
#93430=CARTESIAN_POINT('Ctrl Pts',(-47.0002571609286,53.9204769738583,0.));
#93431=CARTESIAN_POINT('Ctrl Pts',(-47.0202978277148,53.9320275095864,0.));
#93432=CARTESIAN_POINT('Ctrl Pts',(-47.04038842761,53.9435802217468,0.));
#93433=CARTESIAN_POINT('Ctrl Pts',(-47.0605288804042,53.9551349884637,0.));
#93434=CARTESIAN_POINT('Ctrl Pts',(-47.0807191061674,53.9666916884624,0.));
#93435=CARTESIAN_POINT('Ctrl Pts',(-47.1009590252466,53.9782502010642,0.));
#93436=CARTESIAN_POINT('Ctrl Pts',(-47.1212485582632,53.9898104061809,0.));
#93437=CARTESIAN_POINT('Ctrl Pts',(-47.1415876261012,54.0013721843094,0.));
#93438=CARTESIAN_POINT('Ctrl Pts',(-47.161976149906,54.0129354165269,0.));
#93439=CARTESIAN_POINT('Ctrl Pts',(-47.1824140510906,54.0244999844872,0.));
#93440=CARTESIAN_POINT('Ctrl Pts',(-47.2029012513334,54.0360657704156,0.));
#93441=CARTESIAN_POINT('Ctrl Pts',(-47.2234376725752,54.047632657105,0.));
#93442=CARTESIAN_POINT('Ctrl Pts',(-47.2440232370085,54.0592005279108,0.));
#93443=CARTESIAN_POINT('Ctrl Pts',(-47.2646578670767,54.0707692667461,0.));
#93444=CARTESIAN_POINT('Ctrl Pts',(-47.2853414854805,54.082338758079,0.));
#93445=CARTESIAN_POINT('Ctrl Pts',(-47.3060740151754,54.093908886927,0.));
#93446=CARTESIAN_POINT('Ctrl Pts',(-47.326855379369,54.1054795388538,0.));
#93447=CARTESIAN_POINT('Ctrl Pts',(-47.3476855015095,54.1170505999637,0.));
#93448=CARTESIAN_POINT('Ctrl Pts',(-47.3685643052867,54.128621956898,0.));
#93449=CARTESIAN_POINT('Ctrl Pts',(-47.3894917146361,54.1401934968306,0.));
#93450=CARTESIAN_POINT('Ctrl Pts',(-47.4104676537381,54.1517651074638,0.));
#93451=CARTESIAN_POINT('Ctrl Pts',(-47.4314920470142,54.163336677024,0.));
#93452=CARTESIAN_POINT('Ctrl Pts',(-47.4525648191173,54.1749080942593,0.));
#93453=CARTESIAN_POINT('Ctrl Pts',(-47.473685894932,54.1864792484343,0.));
#93454=CARTESIAN_POINT('Ctrl Pts',(-47.4948551995799,54.1980500293267,0.));
#93455=CARTESIAN_POINT('Ctrl Pts',(-47.5160726584172,54.2096203272228,0.));
#93456=CARTESIAN_POINT('Ctrl Pts',(-47.5373381970328,54.221190032914,0.));
#93457=CARTESIAN_POINT('Ctrl Pts',(-47.5586517412368,54.232759037693,0.));
#93458=CARTESIAN_POINT('Ctrl Pts',(-47.5800132170614,54.2443272333498,0.));
#93459=CARTESIAN_POINT('Ctrl Pts',(-47.6014225507664,54.2558945121684,0.));
#93460=CARTESIAN_POINT('Ctrl Pts',(-47.6228796688376,54.2674607669227,0.));
#93461=CARTESIAN_POINT('Ctrl Pts',(-47.6443844979846,54.2790258908736,0.));
#93462=CARTESIAN_POINT('Ctrl Pts',(-47.6659369651299,54.2905897777647,0.));
#93463=CARTESIAN_POINT('Ctrl Pts',(-47.6875369974086,54.3021523218188,0.));
#93464=CARTESIAN_POINT('Ctrl Pts',(-47.7091845221747,54.3137134177345,0.));
#93465=CARTESIAN_POINT('Ctrl Pts',(-47.7308794669994,54.3252729606824,0.));
#93466=CARTESIAN_POINT('Ctrl Pts',(-47.7526217596694,54.3368308463023,0.));
#93467=CARTESIAN_POINT('Ctrl Pts',(-47.7744113281768,54.3483869706998,0.));
#93468=CARTESIAN_POINT('Ctrl Pts',(-47.7962481007179,54.3599412304431,0.));
#93469=CARTESIAN_POINT('Ctrl Pts',(-47.8181320056988,54.3714935225585,0.));
#93470=CARTESIAN_POINT('Ctrl Pts',(-47.8400629717352,54.3830437445275,0.));
#93471=CARTESIAN_POINT('Ctrl Pts',(-47.8620409276495,54.3945917942835,0.));
#93472=CARTESIAN_POINT('Ctrl Pts',(-47.8840658024626,54.4061375702088,0.));
#93473=CARTESIAN_POINT('Ctrl Pts',(-47.9061375253909,54.4176809711324,0.));
#93474=CARTESIAN_POINT('Ctrl Pts',(-47.9282560258528,54.4292218963253,0.));
#93475=CARTESIAN_POINT('Ctrl Pts',(-47.9504212334681,54.4407602454974,0.));
#93476=CARTESIAN_POINT('Ctrl Pts',(-47.972633078057,54.4522959187952,0.));
#93477=CARTESIAN_POINT('Ctrl Pts',(-47.9948914896316,54.4638288167991,0.));
#93478=CARTESIAN_POINT('Ctrl Pts',(-48.0171963983912,54.4753588405202,0.));
#93479=CARTESIAN_POINT('Ctrl Pts',(-48.039547734729,54.4868858913961,0.));
#93480=CARTESIAN_POINT('Ctrl Pts',(-48.0619454292321,54.4984098712883,0.));
#93481=CARTESIAN_POINT('Ctrl Pts',(-48.0843894126807,54.5099306824788,0.));
#93482=CARTESIAN_POINT('Ctrl Pts',(-48.1068796160406,54.5214482276679,0.));
#93483=CARTESIAN_POINT('Ctrl Pts',(-48.1294159704571,54.5329624099719,0.));
#93484=CARTESIAN_POINT('Ctrl Pts',(-48.1519984072617,54.5444731329196,0.));
#93485=CARTESIAN_POINT('Ctrl Pts',(-48.1746268579732,54.5559803004487,0.));
#93486=CARTESIAN_POINT('Ctrl Pts',(-48.1973012542966,54.5674838169041,0.));
#93487=CARTESIAN_POINT('Ctrl Pts',(-48.2200215281178,54.5789835870348,0.));
#93488=CARTESIAN_POINT('Ctrl Pts',(-48.2427876114955,54.5904795159936,0.));
#93489=CARTESIAN_POINT('Ctrl Pts',(-48.2655994366672,54.6019715093319,0.));
#93490=CARTESIAN_POINT('Ctrl Pts',(-48.288456936051,54.6134594729964,0.));
#93491=CARTESIAN_POINT('Ctrl Pts',(-48.3113600422443,54.6249433133262,0.));
#93492=CARTESIAN_POINT('Ctrl Pts',(-48.3343086880192,54.636422937049,0.));
#93493=CARTESIAN_POINT('Ctrl Pts',(-48.3573028063122,54.647898251279,0.));
#93494=CARTESIAN_POINT('Ctrl Pts',(-48.3803423302294,54.6593691635143,0.));
#93495=CARTESIAN_POINT('Ctrl Pts',(-48.4034271930516,54.6708355816359,0.));
#93496=CARTESIAN_POINT('Ctrl Pts',(-48.4265573282342,54.6822974139065,0.));
#93497=CARTESIAN_POINT('Ctrl Pts',(-48.4497326694051,54.6937545689694,0.));
#93498=CARTESIAN_POINT('Ctrl Pts',(-48.4729531503565,54.7052069558493,0.));
#93499=CARTESIAN_POINT('Ctrl Pts',(-48.4962187050452,54.7166544839475,0.));
#93500=CARTESIAN_POINT('Ctrl Pts',(-48.5195292675955,54.7280970630346,0.));
#93501=CARTESIAN_POINT('Ctrl Pts',(-48.5428847722974,54.7395346032451,0.));
#93502=CARTESIAN_POINT('Ctrl Pts',(-48.5662851536027,54.7509670150716,0.));
#93503=CARTESIAN_POINT('Ctrl Pts',(-48.5897303461131,54.7623942093591,0.));
#93504=CARTESIAN_POINT('Ctrl Pts',(-48.6132202845792,54.773816097304,0.));
#93505=CARTESIAN_POINT('Ctrl Pts',(-48.6367549039121,54.7852325904591,0.));
#93506=CARTESIAN_POINT('Ctrl Pts',(-48.6603341391891,54.7966436007395,0.));
#93507=CARTESIAN_POINT('Ctrl Pts',(-48.6839579256565,54.8080490404274,0.));
#93508=CARTESIAN_POINT('Ctrl Pts',(-48.7076261987284,54.8194488221803,0.));
#93509=CARTESIAN_POINT('Ctrl Pts',(-48.7313388939834,54.8308428590333,0.));
#93510=CARTESIAN_POINT('Ctrl Pts',(-48.755095947159,54.8422310643752,0.));
#93511=CARTESIAN_POINT('Ctrl Pts',(-48.7788972941431,54.8536133519285,0.));
#93512=CARTESIAN_POINT('Ctrl Pts',(-48.8027428709613,54.8649896357284,0.));
#93513=CARTESIAN_POINT('Ctrl Pts',(-48.8266326137629,54.8763598301045,0.));
#93514=CARTESIAN_POINT('Ctrl Pts',(-48.8505664587985,54.8877238496576,0.));
#93515=CARTESIAN_POINT('Ctrl Pts',(-48.8745443424488,54.8990816092964,0.));
#93516=CARTESIAN_POINT('Ctrl Pts',(-48.8985662012535,54.910433024275,0.));
#93517=CARTESIAN_POINT('Ctrl Pts',(-48.922631971937,54.9217780102357,0.));
#93518=CARTESIAN_POINT('Ctrl Pts',(-48.9467415914266,54.933116483242,0.));
#93519=CARTESIAN_POINT('Ctrl Pts',(-48.9708949968789,54.9444483598372,0.));
#93520=CARTESIAN_POINT('Ctrl Pts',(-48.995092125652,54.9557735569936,0.));
#93521=CARTESIAN_POINT('Ctrl Pts',(-49.0193329152475,54.9670919920024,0.));
#93522=CARTESIAN_POINT('Ctrl Pts',(-49.0436173032527,54.9784035823764,0.));
#93523=CARTESIAN_POINT('Ctrl Pts',(-49.0679452272871,54.9897082457606,0.));
#93524=CARTESIAN_POINT('Ctrl Pts',(-49.0923166249222,55.0010058998111,0.));
#93525=CARTESIAN_POINT('Ctrl Pts',(-49.1167314336737,55.0122964621868,0.));
#93526=CARTESIAN_POINT('Ctrl Pts',(-49.1411895911646,55.0235798508056,0.));
#93527=CARTESIAN_POINT('Ctrl Pts',(-49.1656910352484,55.0348559840461,0.));
#93528=CARTESIAN_POINT('Ctrl Pts',(-49.1902357041462,55.0461247809745,0.));
#93529=CARTESIAN_POINT('Ctrl Pts',(-49.2148235365694,55.0573861615569,0.));
#93530=CARTESIAN_POINT('Ctrl Pts',(-49.2394544718513,55.0686400468911,0.));
#93531=CARTESIAN_POINT('Ctrl Pts',(-49.2641284496496,55.0798863586986,0.));
#93532=CARTESIAN_POINT('Ctrl Pts',(-49.2888454096544,55.0911250188282,0.));
#93533=CARTESIAN_POINT('Ctrl Pts',(-49.3136052912614,55.1023559487133,0.));
#93534=CARTESIAN_POINT('Ctrl Pts',(-49.3384080333166,55.1135790689475,0.));
#93535=CARTESIAN_POINT('Ctrl Pts',(-49.3632535736744,55.1247942985649,0.));
#93536=CARTESIAN_POINT('Ctrl Pts',(-49.3881418495529,55.1360015556262,0.));
#93537=CARTESIAN_POINT('Ctrl Pts',(-49.413072798324,55.1472007585223,0.));
#93538=CARTESIAN_POINT('Ctrl Pts',(-49.4380463581989,55.158391827114,0.));
#93539=CARTESIAN_POINT('Ctrl Pts',(-49.4630624688787,55.1695746838168,0.));
#93540=CARTESIAN_POINT('Ctrl Pts',(-49.4881210723921,55.1807492550073,0.));
#93541=CARTESIAN_POINT('Ctrl Pts',(-49.5132221132916,55.1919154713569,0.));
#93542=CARTESIAN_POINT('Ctrl Pts',(-49.5347748994609,55.2014798623976,0.));
#93543=CARTESIAN_POINT('Ctrl Pts',(-49.5513218524283,55.2088081098956,0.));
#93544=CARTESIAN_POINT('Ctrl Pts',(-49.5628442141876,55.2139039604571,0.));
#93545=CARTESIAN_POINT('Ctrl Pts',(-49.5693295981616,55.2167699151171,0.));
#93546=CARTESIAN_POINT('Ctrl Pts',(-49.5707719660265,55.2174072001301,0.));
#93547=CARTESIAN_POINT('',(-45.6458539113724,53.0702932034641,12.));
#93548=CARTESIAN_POINT('',(-45.6458539113724,53.0702932034641,0.));
#93549=CARTESIAN_POINT('Ctrl Pts',(-49.5707719660265,55.2174072001301,12.));
#93550=CARTESIAN_POINT('Ctrl Pts',(-49.5693295981616,55.2167699151171,12.));
#93551=CARTESIAN_POINT('Ctrl Pts',(-49.5628442141876,55.2139039604571,12.));
#93552=CARTESIAN_POINT('Ctrl Pts',(-49.5513218524283,55.2088081098956,12.));
#93553=CARTESIAN_POINT('Ctrl Pts',(-49.5347748994609,55.2014798623976,12.));
#93554=CARTESIAN_POINT('Ctrl Pts',(-49.5132221132916,55.1919154713569,12.));
#93555=CARTESIAN_POINT('Ctrl Pts',(-49.4881210723921,55.1807492550073,12.));
#93556=CARTESIAN_POINT('Ctrl Pts',(-49.4630624688787,55.1695746838168,12.));
#93557=CARTESIAN_POINT('Ctrl Pts',(-49.4380463581989,55.158391827114,12.));
#93558=CARTESIAN_POINT('Ctrl Pts',(-49.413072798324,55.1472007585223,12.));
#93559=CARTESIAN_POINT('Ctrl Pts',(-49.3881418495529,55.1360015556262,12.));
#93560=CARTESIAN_POINT('Ctrl Pts',(-49.3632535736744,55.1247942985649,12.));
#93561=CARTESIAN_POINT('Ctrl Pts',(-49.3384080333166,55.1135790689475,12.));
#93562=CARTESIAN_POINT('Ctrl Pts',(-49.3136052912614,55.1023559487133,12.));
#93563=CARTESIAN_POINT('Ctrl Pts',(-49.2888454096544,55.0911250188282,12.));
#93564=CARTESIAN_POINT('Ctrl Pts',(-49.2641284496496,55.0798863586986,12.));
#93565=CARTESIAN_POINT('Ctrl Pts',(-49.2394544718513,55.0686400468911,12.));
#93566=CARTESIAN_POINT('Ctrl Pts',(-49.2148235365694,55.0573861615569,12.));
#93567=CARTESIAN_POINT('Ctrl Pts',(-49.1902357041462,55.0461247809745,12.));
#93568=CARTESIAN_POINT('Ctrl Pts',(-49.1656910352484,55.0348559840461,12.));
#93569=CARTESIAN_POINT('Ctrl Pts',(-49.1411895911646,55.0235798508056,12.));
#93570=CARTESIAN_POINT('Ctrl Pts',(-49.1167314336737,55.0122964621868,12.));
#93571=CARTESIAN_POINT('Ctrl Pts',(-49.0923166249222,55.0010058998111,12.));
#93572=CARTESIAN_POINT('Ctrl Pts',(-49.0679452272871,54.9897082457606,12.));
#93573=CARTESIAN_POINT('Ctrl Pts',(-49.0436173032527,54.9784035823764,12.));
#93574=CARTESIAN_POINT('Ctrl Pts',(-49.0193329152475,54.9670919920024,12.));
#93575=CARTESIAN_POINT('Ctrl Pts',(-48.995092125652,54.9557735569936,12.));
#93576=CARTESIAN_POINT('Ctrl Pts',(-48.9708949968789,54.9444483598372,12.));
#93577=CARTESIAN_POINT('Ctrl Pts',(-48.9467415914266,54.933116483242,12.));
#93578=CARTESIAN_POINT('Ctrl Pts',(-48.922631971937,54.9217780102357,12.));
#93579=CARTESIAN_POINT('Ctrl Pts',(-48.8985662012535,54.910433024275,12.));
#93580=CARTESIAN_POINT('Ctrl Pts',(-48.8745443424488,54.8990816092964,12.));
#93581=CARTESIAN_POINT('Ctrl Pts',(-48.8505664587985,54.8877238496576,12.));
#93582=CARTESIAN_POINT('Ctrl Pts',(-48.8266326137629,54.8763598301045,12.));
#93583=CARTESIAN_POINT('Ctrl Pts',(-48.8027428709613,54.8649896357284,12.));
#93584=CARTESIAN_POINT('Ctrl Pts',(-48.7788972941431,54.8536133519285,12.));
#93585=CARTESIAN_POINT('Ctrl Pts',(-48.755095947159,54.8422310643752,12.));
#93586=CARTESIAN_POINT('Ctrl Pts',(-48.7313388939834,54.8308428590333,12.));
#93587=CARTESIAN_POINT('Ctrl Pts',(-48.7076261987284,54.8194488221803,12.));
#93588=CARTESIAN_POINT('Ctrl Pts',(-48.6839579256565,54.8080490404274,12.));
#93589=CARTESIAN_POINT('Ctrl Pts',(-48.6603341391891,54.7966436007395,12.));
#93590=CARTESIAN_POINT('Ctrl Pts',(-48.6367549039121,54.7852325904591,12.));
#93591=CARTESIAN_POINT('Ctrl Pts',(-48.6132202845792,54.773816097304,12.));
#93592=CARTESIAN_POINT('Ctrl Pts',(-48.5897303461131,54.7623942093591,12.));
#93593=CARTESIAN_POINT('Ctrl Pts',(-48.5662851536027,54.7509670150716,12.));
#93594=CARTESIAN_POINT('Ctrl Pts',(-48.5428847722974,54.7395346032451,12.));
#93595=CARTESIAN_POINT('Ctrl Pts',(-48.5195292675955,54.7280970630346,12.));
#93596=CARTESIAN_POINT('Ctrl Pts',(-48.4962187050452,54.7166544839475,12.));
#93597=CARTESIAN_POINT('Ctrl Pts',(-48.4729531503565,54.7052069558493,12.));
#93598=CARTESIAN_POINT('Ctrl Pts',(-48.4497326694051,54.6937545689694,12.));
#93599=CARTESIAN_POINT('Ctrl Pts',(-48.4265573282342,54.6822974139065,12.));
#93600=CARTESIAN_POINT('Ctrl Pts',(-48.4034271930516,54.6708355816359,12.));
#93601=CARTESIAN_POINT('Ctrl Pts',(-48.3803423302294,54.6593691635143,12.));
#93602=CARTESIAN_POINT('Ctrl Pts',(-48.3573028063122,54.647898251279,12.));
#93603=CARTESIAN_POINT('Ctrl Pts',(-48.3343086880192,54.636422937049,12.));
#93604=CARTESIAN_POINT('Ctrl Pts',(-48.3113600422443,54.6249433133262,12.));
#93605=CARTESIAN_POINT('Ctrl Pts',(-48.288456936051,54.6134594729964,12.));
#93606=CARTESIAN_POINT('Ctrl Pts',(-48.2655994366672,54.6019715093319,12.));
#93607=CARTESIAN_POINT('Ctrl Pts',(-48.2427876114955,54.5904795159936,12.));
#93608=CARTESIAN_POINT('Ctrl Pts',(-48.2200215281178,54.5789835870348,12.));
#93609=CARTESIAN_POINT('Ctrl Pts',(-48.1973012542966,54.5674838169041,12.));
#93610=CARTESIAN_POINT('Ctrl Pts',(-48.1746268579732,54.5559803004487,12.));
#93611=CARTESIAN_POINT('Ctrl Pts',(-48.1519984072617,54.5444731329196,12.));
#93612=CARTESIAN_POINT('Ctrl Pts',(-48.1294159704571,54.5329624099719,12.));
#93613=CARTESIAN_POINT('Ctrl Pts',(-48.1068796160406,54.5214482276679,12.));
#93614=CARTESIAN_POINT('Ctrl Pts',(-48.0843894126807,54.5099306824788,12.));
#93615=CARTESIAN_POINT('Ctrl Pts',(-48.0619454292321,54.4984098712883,12.));
#93616=CARTESIAN_POINT('Ctrl Pts',(-48.039547734729,54.4868858913961,12.));
#93617=CARTESIAN_POINT('Ctrl Pts',(-48.0171963983912,54.4753588405202,12.));
#93618=CARTESIAN_POINT('Ctrl Pts',(-47.9948914896316,54.4638288167991,12.));
#93619=CARTESIAN_POINT('Ctrl Pts',(-47.972633078057,54.4522959187952,12.));
#93620=CARTESIAN_POINT('Ctrl Pts',(-47.9504212334681,54.4407602454974,12.));
#93621=CARTESIAN_POINT('Ctrl Pts',(-47.9282560258528,54.4292218963253,12.));
#93622=CARTESIAN_POINT('Ctrl Pts',(-47.9061375253909,54.4176809711324,12.));
#93623=CARTESIAN_POINT('Ctrl Pts',(-47.8840658024626,54.4061375702088,12.));
#93624=CARTESIAN_POINT('Ctrl Pts',(-47.8620409276495,54.3945917942835,12.));
#93625=CARTESIAN_POINT('Ctrl Pts',(-47.8400629717352,54.3830437445275,12.));
#93626=CARTESIAN_POINT('Ctrl Pts',(-47.8181320056988,54.3714935225585,12.));
#93627=CARTESIAN_POINT('Ctrl Pts',(-47.7962481007179,54.3599412304431,12.));
#93628=CARTESIAN_POINT('Ctrl Pts',(-47.7744113281768,54.3483869706998,12.));
#93629=CARTESIAN_POINT('Ctrl Pts',(-47.7526217596694,54.3368308463023,12.));
#93630=CARTESIAN_POINT('Ctrl Pts',(-47.7308794669994,54.3252729606824,12.));
#93631=CARTESIAN_POINT('Ctrl Pts',(-47.7091845221747,54.3137134177345,12.));
#93632=CARTESIAN_POINT('Ctrl Pts',(-47.6875369974086,54.3021523218188,12.));
#93633=CARTESIAN_POINT('Ctrl Pts',(-47.6659369651299,54.2905897777647,12.));
#93634=CARTESIAN_POINT('Ctrl Pts',(-47.6443844979846,54.2790258908736,12.));
#93635=CARTESIAN_POINT('Ctrl Pts',(-47.6228796688376,54.2674607669227,12.));
#93636=CARTESIAN_POINT('Ctrl Pts',(-47.6014225507664,54.2558945121684,12.));
#93637=CARTESIAN_POINT('Ctrl Pts',(-47.5800132170614,54.2443272333498,12.));
#93638=CARTESIAN_POINT('Ctrl Pts',(-47.5586517412368,54.232759037693,12.));
#93639=CARTESIAN_POINT('Ctrl Pts',(-47.5373381970328,54.221190032914,12.));
#93640=CARTESIAN_POINT('Ctrl Pts',(-47.5160726584172,54.2096203272228,12.));
#93641=CARTESIAN_POINT('Ctrl Pts',(-47.4948551995799,54.1980500293267,12.));
#93642=CARTESIAN_POINT('Ctrl Pts',(-47.473685894932,54.1864792484343,12.));
#93643=CARTESIAN_POINT('Ctrl Pts',(-47.4525648191173,54.1749080942593,12.));
#93644=CARTESIAN_POINT('Ctrl Pts',(-47.4314920470142,54.163336677024,12.));
#93645=CARTESIAN_POINT('Ctrl Pts',(-47.4104676537381,54.1517651074638,12.));
#93646=CARTESIAN_POINT('Ctrl Pts',(-47.3894917146361,54.1401934968306,12.));
#93647=CARTESIAN_POINT('Ctrl Pts',(-47.3685643052867,54.128621956898,12.));
#93648=CARTESIAN_POINT('Ctrl Pts',(-47.3476855015095,54.1170505999637,12.));
#93649=CARTESIAN_POINT('Ctrl Pts',(-47.326855379369,54.1054795388538,12.));
#93650=CARTESIAN_POINT('Ctrl Pts',(-47.3060740151754,54.093908886927,12.));
#93651=CARTESIAN_POINT('Ctrl Pts',(-47.2853414854805,54.082338758079,12.));
#93652=CARTESIAN_POINT('Ctrl Pts',(-47.2646578670767,54.0707692667461,12.));
#93653=CARTESIAN_POINT('Ctrl Pts',(-47.2440232370085,54.0592005279108,12.));
#93654=CARTESIAN_POINT('Ctrl Pts',(-47.2234376725752,54.047632657105,12.));
#93655=CARTESIAN_POINT('Ctrl Pts',(-47.2029012513334,54.0360657704156,12.));
#93656=CARTESIAN_POINT('Ctrl Pts',(-47.1824140510906,54.0244999844872,12.));
#93657=CARTESIAN_POINT('Ctrl Pts',(-47.161976149906,54.0129354165269,12.));
#93658=CARTESIAN_POINT('Ctrl Pts',(-47.1415876261012,54.0013721843094,12.));
#93659=CARTESIAN_POINT('Ctrl Pts',(-47.1212485582632,53.9898104061809,12.));
#93660=CARTESIAN_POINT('Ctrl Pts',(-47.1009590252466,53.9782502010642,12.));
#93661=CARTESIAN_POINT('Ctrl Pts',(-47.0807191061674,53.9666916884624,12.));
#93662=CARTESIAN_POINT('Ctrl Pts',(-47.0605288804042,53.9551349884637,12.));
#93663=CARTESIAN_POINT('Ctrl Pts',(-47.04038842761,53.9435802217468,12.));
#93664=CARTESIAN_POINT('Ctrl Pts',(-47.0202978277148,53.9320275095864,12.));
#93665=CARTESIAN_POINT('Ctrl Pts',(-47.0002571609286,53.9204769738583,12.));
#93666=CARTESIAN_POINT('Ctrl Pts',(-46.9802665077342,53.9089287370435,12.));
#93667=CARTESIAN_POINT('Ctrl Pts',(-46.9603259488894,53.8973829222317,12.));
#93668=CARTESIAN_POINT('Ctrl Pts',(-46.9404355654381,53.8858396531277,12.));
#93669=CARTESIAN_POINT('Ctrl Pts',(-46.9205954387128,53.8742990540557,12.));
#93670=CARTESIAN_POINT('Ctrl Pts',(-46.900805650336,53.8627612499648,12.));
#93671=CARTESIAN_POINT('Ctrl Pts',(-46.8810662822147,53.851226366434,12.));
#93672=CARTESIAN_POINT('Ctrl Pts',(-46.8613774165452,53.8396945296777,12.));
#93673=CARTESIAN_POINT('Ctrl Pts',(-46.8417391358231,53.8281658665517,12.));
#93674=CARTESIAN_POINT('Ctrl Pts',(-46.8221515228459,53.8166405045582,12.));
#93675=CARTESIAN_POINT('Ctrl Pts',(-46.8026146607144,53.8051185718524,12.));
#93676=CARTESIAN_POINT('Ctrl Pts',(-46.7831286328268,53.7936001972468,12.));
#93677=CARTESIAN_POINT('Ctrl Pts',(-46.7636935228851,53.7820855102169,12.));
#93678=CARTESIAN_POINT('Ctrl Pts',(-46.7443094149041,53.770574640907,12.));
#93679=CARTESIAN_POINT('Ctrl Pts',(-46.724976393213,53.7590677201344,12.));
#93680=CARTESIAN_POINT('Ctrl Pts',(-46.7056945424559,53.7475648793948,12.));
#93681=CARTESIAN_POINT('Ctrl Pts',(-46.6864639475863,53.7360662508677,12.));
#93682=CARTESIAN_POINT('Ctrl Pts',(-46.6672846938752,53.7245719674222,12.));
#93683=CARTESIAN_POINT('Ctrl Pts',(-46.6481568669216,53.7130821626263,12.));
#93684=CARTESIAN_POINT('Ctrl Pts',(-46.6290805526559,53.701596970754,12.));
#93685=CARTESIAN_POINT('Ctrl Pts',(-46.6100558373402,53.6901165267941,12.));
#93686=CARTESIAN_POINT('Ctrl Pts',(-46.5910828075653,53.678640966456,12.));
#93687=CARTESIAN_POINT('Ctrl Pts',(-46.5721615502591,53.6671704261737,12.));
#93688=CARTESIAN_POINT('Ctrl Pts',(-46.5532921526901,53.6557050431071,12.));
#93689=CARTESIAN_POINT('Ctrl Pts',(-46.5344747024676,53.6442449551455,12.));
#93690=CARTESIAN_POINT('Ctrl Pts',(-46.5157092875373,53.6327903009094,12.));
#93691=CARTESIAN_POINT('Ctrl Pts',(-46.496995996177,53.6213412197533,12.));
#93692=CARTESIAN_POINT('Ctrl Pts',(-46.4783349170173,53.6098978517859,12.));
#93693=CARTESIAN_POINT('Ctrl Pts',(-46.459726139052,53.5984603378855,12.));
#93694=CARTESIAN_POINT('Ctrl Pts',(-46.4411697516478,53.5870288197166,12.));
#93695=CARTESIAN_POINT('Ctrl Pts',(-46.4226658445474,53.5756034397481,12.));
#93696=CARTESIAN_POINT('Ctrl Pts',(-46.4042145078701,53.5641843412559,12.));
#93697=CARTESIAN_POINT('Ctrl Pts',(-46.3858158321059,53.5527716683047,12.));
#93698=CARTESIAN_POINT('Ctrl Pts',(-46.3674699081046,53.5413655657327,12.));
#93699=CARTESIAN_POINT('Ctrl Pts',(-46.3491768270655,53.5299661791385,12.));
#93700=CARTESIAN_POINT('Ctrl Pts',(-46.3309366805093,53.5185736548548,12.));
#93701=CARTESIAN_POINT('Ctrl Pts',(-46.3127495603098,53.5071881399911,12.));
#93702=CARTESIAN_POINT('Ctrl Pts',(-46.2946155587417,53.4958097825006,12.));
#93703=CARTESIAN_POINT('Ctrl Pts',(-46.2765347685198,53.4844387312414,12.));
#93704=CARTESIAN_POINT('Ctrl Pts',(-46.2585072828353,53.4730751360371,12.));
#93705=CARTESIAN_POINT('Ctrl Pts',(-46.2405331953889,53.4617191477402,12.));
#93706=CARTESIAN_POINT('Ctrl Pts',(-46.2226126003202,53.4503709181178,12.));
#93707=CARTESIAN_POINT('Ctrl Pts',(-46.2047455921286,53.4390305997274,12.));
#93708=CARTESIAN_POINT('Ctrl Pts',(-46.1869322656024,53.4276983458125,12.));
#93709=CARTESIAN_POINT('Ctrl Pts',(-46.1691727157134,53.4163743101517,12.));
#93710=CARTESIAN_POINT('Ctrl Pts',(-46.1514670376012,53.4050586470436,12.));
#93711=CARTESIAN_POINT('Ctrl Pts',(-46.1338153268097,53.3937515116549,12.));
#93712=CARTESIAN_POINT('Ctrl Pts',(-46.1162176794884,53.3824530603276,12.));
#93713=CARTESIAN_POINT('Ctrl Pts',(-46.0986741925656,53.3711634508437,12.));
#93714=CARTESIAN_POINT('Ctrl Pts',(-46.0811849640218,53.3598828428546,12.));
#93715=CARTESIAN_POINT('Ctrl Pts',(-46.0637500926982,53.3486113975901,12.));
#93716=CARTESIAN_POINT('Ctrl Pts',(-46.0463696777801,53.3373492770671,12.));
#93717=CARTESIAN_POINT('Ctrl Pts',(-46.02904381836,53.326096643428,12.));
#93718=CARTESIAN_POINT('Ctrl Pts',(-46.0117726129873,53.3148536582635,12.));
#93719=CARTESIAN_POINT('Ctrl Pts',(-45.9945561591453,53.3036204818329,12.));
#93720=CARTESIAN_POINT('Ctrl Pts',(-45.9773945542384,53.292397274555,12.));
#93721=CARTESIAN_POINT('Ctrl Pts',(-45.9602878967698,53.2811841987926,12.));
#93722=CARTESIAN_POINT('Ctrl Pts',(-45.9432362873008,53.2699814203105,12.));
#93723=CARTESIAN_POINT('Ctrl Pts',(-45.9262398298349,53.2587891103866,12.));
#93724=CARTESIAN_POINT('Ctrl Pts',(-45.9092986319377,53.2476074460017,12.));
#93725=CARTESIAN_POINT('Ctrl Pts',(-45.892412801838,53.2364366054306,12.));
#93726=CARTESIAN_POINT('Ctrl Pts',(-45.8755824458723,53.2252767643662,12.));
#93727=CARTESIAN_POINT('Ctrl Pts',(-45.8588076662582,53.2141280925439,12.));
#93728=CARTESIAN_POINT('Ctrl Pts',(-45.8420885575349,53.2029907483557,12.));
#93729=CARTESIAN_POINT('Ctrl Pts',(-45.8254252099957,53.1918648840541,12.));
#93730=CARTESIAN_POINT('Ctrl Pts',(-45.808817716509,53.1807506560933,12.));
#93731=CARTESIAN_POINT('Ctrl Pts',(-45.7922661780005,53.1696482334487,12.));
#93732=CARTESIAN_POINT('Ctrl Pts',(-45.7757707100618,53.1585578076444,12.));
#93733=CARTESIAN_POINT('Ctrl Pts',(-45.7593314474501,53.1474795996053,12.));
#93734=CARTESIAN_POINT('Ctrl Pts',(-45.7429485300823,53.1364138384693,12.));
#93735=CARTESIAN_POINT('Ctrl Pts',(-45.7266220897003,53.1253607414872,12.));
#93736=CARTESIAN_POINT('Ctrl Pts',(-45.7103522376696,53.114320495492,12.));
#93737=CARTESIAN_POINT('Ctrl Pts',(-45.694139048907,53.1032932328857,12.));
#93738=CARTESIAN_POINT('Ctrl Pts',(-45.6779825614231,53.0922790298409,12.));
#93739=CARTESIAN_POINT('Ctrl Pts',(-45.6651027439241,53.0834781451546,12.));
#93740=CARTESIAN_POINT('Ctrl Pts',(-45.6554684028145,53.0768833804193,12.));
#93741=CARTESIAN_POINT('Ctrl Pts',(-45.6490568514089,53.0724894921849,12.));
#93742=CARTESIAN_POINT('Ctrl Pts',(-45.6458539113724,53.0702932034641,12.));
#93743=CARTESIAN_POINT('Ctrl Pts',(-50.6869108458849,54.1946543500369,-5.55111512312578E-16));
#93744=CARTESIAN_POINT('Ctrl Pts',(-50.6869108458849,54.1946543500369,4.));
#93745=CARTESIAN_POINT('Ctrl Pts',(-50.6869108458849,54.194654350037,8.));
#93746=CARTESIAN_POINT('Ctrl Pts',(-50.6869108458849,54.194654350037,12.));
#93747=CARTESIAN_POINT('Ctrl Pts',(-50.7223900873019,54.2986513683563,-5.55111512312578E-16));
#93748=CARTESIAN_POINT('Ctrl Pts',(-50.7223900873019,54.2986513683563,4.));
#93749=CARTESIAN_POINT('Ctrl Pts',(-50.722390087302,54.2986513683564,8.));
#93750=CARTESIAN_POINT('Ctrl Pts',(-50.722390087302,54.2986513683564,12.));
#93751=CARTESIAN_POINT('Ctrl Pts',(-50.7219766588191,54.5013145669259,-5.55111512312578E-16));
#93752=CARTESIAN_POINT('Ctrl Pts',(-50.7219766588191,54.5013145669259,4.));
#93753=CARTESIAN_POINT('Ctrl Pts',(-50.7219766588192,54.501314566926,8.00000000000001));
#93754=CARTESIAN_POINT('Ctrl Pts',(-50.7219766588192,54.501314566926,12.));
#93755=CARTESIAN_POINT('Ctrl Pts',(-50.6135081477653,54.667445382869,-5.55111512312578E-16));
#93756=CARTESIAN_POINT('Ctrl Pts',(-50.6135081477653,54.667445382869,4.));
#93757=CARTESIAN_POINT('Ctrl Pts',(-50.6135081477653,54.6674453828691,8.));
#93758=CARTESIAN_POINT('Ctrl Pts',(-50.6135081477653,54.6674453828691,12.));
#93759=CARTESIAN_POINT('Ctrl Pts',(-50.5529731960896,54.7233670476822,-5.55111512312578E-16));
#93760=CARTESIAN_POINT('Ctrl Pts',(-50.5529731960896,54.7233670476822,4.));
#93761=CARTESIAN_POINT('Ctrl Pts',(-50.5529731960896,54.7233670476823,8.));
#93762=CARTESIAN_POINT('Ctrl Pts',(-50.5529731960896,54.7233670476823,12.));
#93763=CARTESIAN_POINT('',(-50.6869108458849,54.1946543500369,-2.77555756156289E-16));
#93764=CARTESIAN_POINT('',(-50.5529731960901,54.7233670476827,0.));
#93765=CARTESIAN_POINT('Ctrl Pts',(-50.6869108458849,54.1946543500369,-5.55111512312578E-16));
#93766=CARTESIAN_POINT('Ctrl Pts',(-50.7223900873019,54.2986513683563,-5.55111512312578E-16));
#93767=CARTESIAN_POINT('Ctrl Pts',(-50.7221538424546,54.4144589103961,-5.55111512312578E-16));
#93768=CARTESIAN_POINT('Ctrl Pts',(-50.6866343053392,54.51833751117,-5.55111512312578E-16));
#93769=CARTESIAN_POINT('Ctrl Pts',(-50.6599946525026,54.5962464617505,-5.55111512312578E-16));
#93770=CARTESIAN_POINT('Ctrl Pts',(-50.6135081477653,54.667445382869,-5.55111512312578E-16));
#93771=CARTESIAN_POINT('Ctrl Pts',(-50.5529731960896,54.7233670476822,-5.55111512312578E-16));
#93772=CARTESIAN_POINT('',(-50.55297319609,54.7233670476827,12.));
#93773=CARTESIAN_POINT('Ctrl Pts',(-50.5529731960896,54.7233670476822,-5.55111512312578E-16));
#93774=CARTESIAN_POINT('Ctrl Pts',(-50.5529731960896,54.7233670476822,4.));
#93775=CARTESIAN_POINT('Ctrl Pts',(-50.5529731960896,54.7233670476823,8.));
#93776=CARTESIAN_POINT('Ctrl Pts',(-50.5529731960896,54.7233670476823,12.));
#93777=CARTESIAN_POINT('',(-50.6869108458849,54.194654350037,12.));
#93778=CARTESIAN_POINT('Ctrl Pts',(-50.5529731960896,54.7233670476823,12.));
#93779=CARTESIAN_POINT('Ctrl Pts',(-50.6135081477653,54.6674453828691,12.));
#93780=CARTESIAN_POINT('Ctrl Pts',(-50.6599946525027,54.5962464617506,12.));
#93781=CARTESIAN_POINT('Ctrl Pts',(-50.6866343053393,54.5183375111701,12.));
#93782=CARTESIAN_POINT('Ctrl Pts',(-50.7221538424547,54.4144589103961,12.));
#93783=CARTESIAN_POINT('Ctrl Pts',(-50.722390087302,54.2986513683564,12.));
#93784=CARTESIAN_POINT('Ctrl Pts',(-50.6869108458849,54.194654350037,12.));
#93785=CARTESIAN_POINT('Ctrl Pts',(-50.6869108458849,54.194654350037,12.));
#93786=CARTESIAN_POINT('Ctrl Pts',(-50.6869108458849,54.194654350037,8.));
#93787=CARTESIAN_POINT('Ctrl Pts',(-50.6869108458849,54.1946543500369,4.));
#93788=CARTESIAN_POINT('Ctrl Pts',(-50.6869108458849,54.1946543500369,-5.55111512312578E-16));
#93789=CARTESIAN_POINT('Origin',(-2.53313958019842E-10,2.7629675461203E-10,
0.));
#93790=CARTESIAN_POINT('Origin',(-2.53313958019842E-10,2.7629675461203E-10,
12.));
#93791=CARTESIAN_POINT('Origin',(-2.53313958019842E-10,2.7629675461203E-10,
0.));
#93792=CARTESIAN_POINT('Ctrl Pts',(-45.1135644683471,59.2875729049545,-5.55111512312578E-16));
#93793=CARTESIAN_POINT('Ctrl Pts',(-45.1135644683471,59.2875729049545,4.));
#93794=CARTESIAN_POINT('Ctrl Pts',(-45.113564468347,59.2875729049545,8.));
#93795=CARTESIAN_POINT('Ctrl Pts',(-45.113564468347,59.2875729049545,12.));
#93796=CARTESIAN_POINT('Ctrl Pts',(-45.0261193041895,59.3541123643618,-5.55111512312578E-16));
#93797=CARTESIAN_POINT('Ctrl Pts',(-45.0261193041895,59.3541123643618,4.));
#93798=CARTESIAN_POINT('Ctrl Pts',(-45.0261193041895,59.3541123643618,8.));
#93799=CARTESIAN_POINT('Ctrl Pts',(-45.0261193041895,59.3541123643618,12.));
#93800=CARTESIAN_POINT('Ctrl Pts',(-44.8337211159574,59.4177951463802,-5.55111512312578E-16));
#93801=CARTESIAN_POINT('Ctrl Pts',(-44.8337211159574,59.4177951463802,4.));
#93802=CARTESIAN_POINT('Ctrl Pts',(-44.8337211159573,59.4177951463802,8.));
#93803=CARTESIAN_POINT('Ctrl Pts',(-44.8337211159573,59.4177951463802,12.));
#93804=CARTESIAN_POINT('Ctrl Pts',(-44.6418181989797,59.3674150879747,-5.55111512312578E-16));
#93805=CARTESIAN_POINT('Ctrl Pts',(-44.6418181989797,59.3674150879747,4.));
#93806=CARTESIAN_POINT('Ctrl Pts',(-44.6418181989796,59.3674150879747,8.00000000000001));
#93807=CARTESIAN_POINT('Ctrl Pts',(-44.6418181989796,59.3674150879747,12.));
#93808=CARTESIAN_POINT('Ctrl Pts',(-44.5696260757421,59.3276657444156,-5.55111512312578E-16));
#93809=CARTESIAN_POINT('Ctrl Pts',(-44.5696260757421,59.3276657444156,4.));
#93810=CARTESIAN_POINT('Ctrl Pts',(-44.5696260757421,59.3276657444156,8.));
#93811=CARTESIAN_POINT('Ctrl Pts',(-44.5696260757421,59.3276657444156,12.));
#93812=CARTESIAN_POINT('',(-45.1135644683471,59.2875729049545,0.));
#93813=CARTESIAN_POINT('',(-44.5696260757421,59.3276657444158,0.));
#93814=CARTESIAN_POINT('Ctrl Pts',(-45.1135644683471,59.2875729049545,-5.55111512312578E-16));
#93815=CARTESIAN_POINT('Ctrl Pts',(-45.0261193041895,59.3541123643618,-5.55111512312578E-16));
#93816=CARTESIAN_POINT('Ctrl Pts',(-44.9161774823426,59.3905025255151,-5.55111512312578E-16));
#93817=CARTESIAN_POINT('Ctrl Pts',(-44.8063973817216,59.3896476775505,-5.55111512312578E-16));
#93818=CARTESIAN_POINT('Ctrl Pts',(-44.7240623062559,59.389006541577,-5.55111512312578E-16));
#93819=CARTESIAN_POINT('Ctrl Pts',(-44.6418181989797,59.3674150879747,-5.55111512312578E-16));
#93820=CARTESIAN_POINT('Ctrl Pts',(-44.5696260757421,59.3276657444156,-5.55111512312578E-16));
#93821=CARTESIAN_POINT('',(-44.569626075742,59.3276657444158,12.));
#93822=CARTESIAN_POINT('Ctrl Pts',(-44.5696260757421,59.3276657444156,-5.55111512312578E-16));
#93823=CARTESIAN_POINT('Ctrl Pts',(-44.5696260757421,59.3276657444156,4.));
#93824=CARTESIAN_POINT('Ctrl Pts',(-44.5696260757421,59.3276657444156,8.));
#93825=CARTESIAN_POINT('Ctrl Pts',(-44.5696260757421,59.3276657444156,12.));
#93826=CARTESIAN_POINT('',(-45.113564468347,59.2875729049545,12.));
#93827=CARTESIAN_POINT('Ctrl Pts',(-44.5696260757421,59.3276657444156,12.));
#93828=CARTESIAN_POINT('Ctrl Pts',(-44.6418181989796,59.3674150879747,12.));
#93829=CARTESIAN_POINT('Ctrl Pts',(-44.7240623062558,59.3890065415771,12.));
#93830=CARTESIAN_POINT('Ctrl Pts',(-44.8063973817216,59.3896476775505,12.));
#93831=CARTESIAN_POINT('Ctrl Pts',(-44.9161774823425,59.3905025255152,12.));
#93832=CARTESIAN_POINT('Ctrl Pts',(-45.0261193041895,59.3541123643618,12.));
#93833=CARTESIAN_POINT('Ctrl Pts',(-45.113564468347,59.2875729049545,12.));
#93834=CARTESIAN_POINT('Ctrl Pts',(-45.113564468347,59.2875729049545,12.));
#93835=CARTESIAN_POINT('Ctrl Pts',(-45.113564468347,59.2875729049545,8.));
#93836=CARTESIAN_POINT('Ctrl Pts',(-45.1135644683471,59.2875729049545,4.));
#93837=CARTESIAN_POINT('Ctrl Pts',(-45.1135644683471,59.2875729049545,-5.55111512312578E-16));
#93838=CARTESIAN_POINT('Ctrl Pts',(-40.8467768343956,56.8466430164621,0.));
#93839=CARTESIAN_POINT('Ctrl Pts',(-40.8467768343956,56.8466430164621,12.));
#93840=CARTESIAN_POINT('Ctrl Pts',(-40.8497761671036,56.8491101022591,0.));
#93841=CARTESIAN_POINT('Ctrl Pts',(-40.8497761671036,56.8491101022591,12.));
#93842=CARTESIAN_POINT('Ctrl Pts',(-40.8557803680277,56.8540460739472,0.));
#93843=CARTESIAN_POINT('Ctrl Pts',(-40.8557803680277,56.8540460739472,12.));
#93844=CARTESIAN_POINT('Ctrl Pts',(-40.864803275942,56.8614554317668,0.));
#93845=CARTESIAN_POINT('Ctrl Pts',(-40.864803275942,56.8614554317668,12.));
#93846=CARTESIAN_POINT('Ctrl Pts',(-40.8768670342052,56.8713453764905,0.));
#93847=CARTESIAN_POINT('Ctrl Pts',(-40.8768670342052,56.8713453764905,12.));
#93848=CARTESIAN_POINT('Ctrl Pts',(-40.8920020903293,56.8837257978343,0.));
#93849=CARTESIAN_POINT('Ctrl Pts',(-40.8920020903293,56.8837257978343,12.));
#93850=CARTESIAN_POINT('Ctrl Pts',(-40.9071924937508,56.8961241708861,0.));
#93851=CARTESIAN_POINT('Ctrl Pts',(-40.9071924937508,56.8961241708861,12.));
#93852=CARTESIAN_POINT('Ctrl Pts',(-40.9224382132427,56.9085404164502,0.));
#93853=CARTESIAN_POINT('Ctrl Pts',(-40.9224382132427,56.9085404164502,12.));
#93854=CARTESIAN_POINT('Ctrl Pts',(-40.9377391857128,56.9209743960992,0.));
#93855=CARTESIAN_POINT('Ctrl Pts',(-40.9377391857128,56.9209743960992,12.));
#93856=CARTESIAN_POINT('Ctrl Pts',(-40.9530953165031,56.9334259140049,0.));
#93857=CARTESIAN_POINT('Ctrl Pts',(-40.9530953165031,56.9334259140049,12.));
#93858=CARTESIAN_POINT('Ctrl Pts',(-40.9685064933074,56.9458947422608,0.));
#93859=CARTESIAN_POINT('Ctrl Pts',(-40.9685064933074,56.9458947422608,12.));
#93860=CARTESIAN_POINT('Ctrl Pts',(-40.9839725967121,56.9583806404069,0.));
#93861=CARTESIAN_POINT('Ctrl Pts',(-40.9839725967121,56.9583806404069,12.));
#93862=CARTESIAN_POINT('Ctrl Pts',(-40.9994935117276,56.9708833766137,0.));
#93863=CARTESIAN_POINT('Ctrl Pts',(-40.9994935117276,56.9708833766137,12.));
#93864=CARTESIAN_POINT('Ctrl Pts',(-41.0150691398947,56.9834027500117,0.));
#93865=CARTESIAN_POINT('Ctrl Pts',(-41.0150691398947,56.9834027500117,12.));
#93866=CARTESIAN_POINT('Ctrl Pts',(-41.0306993953988,56.995938583472,0.));
#93867=CARTESIAN_POINT('Ctrl Pts',(-41.0306993953988,56.995938583472,12.));
#93868=CARTESIAN_POINT('Ctrl Pts',(-41.0463841993608,57.008490713042,0.));
#93869=CARTESIAN_POINT('Ctrl Pts',(-41.0463841993608,57.008490713042,12.));
#93870=CARTESIAN_POINT('Ctrl Pts',(-41.0621234751007,57.0210589791788,0.));
#93871=CARTESIAN_POINT('Ctrl Pts',(-41.0621234751007,57.0210589791788,12.));
#93872=CARTESIAN_POINT('Ctrl Pts',(-41.0779171422438,57.0336432158536,0.));
#93873=CARTESIAN_POINT('Ctrl Pts',(-41.0779171422438,57.0336432158536,12.));
#93874=CARTESIAN_POINT('Ctrl Pts',(-41.0937651137549,57.046243245068,0.));
#93875=CARTESIAN_POINT('Ctrl Pts',(-41.0937651137549,57.046243245068,12.));
#93876=CARTESIAN_POINT('Ctrl Pts',(-41.1096672990148,57.0588588825298,0.));
#93877=CARTESIAN_POINT('Ctrl Pts',(-41.1096672990148,57.0588588825298,12.));
#93878=CARTESIAN_POINT('Ctrl Pts',(-41.1256236057442,57.0714899412099,0.));
#93879=CARTESIAN_POINT('Ctrl Pts',(-41.1256236057442,57.0714899412099,12.));
#93880=CARTESIAN_POINT('Ctrl Pts',(-41.1416339422117,57.084136235426,0.));
#93881=CARTESIAN_POINT('Ctrl Pts',(-41.1416339422117,57.084136235426,12.));
#93882=CARTESIAN_POINT('Ctrl Pts',(-41.1576982197374,57.0967975854874,0.));
#93883=CARTESIAN_POINT('Ctrl Pts',(-41.1576982197374,57.0967975854874,12.));
#93884=CARTESIAN_POINT('Ctrl Pts',(-41.1738163525901,57.1094738174957,0.));
#93885=CARTESIAN_POINT('Ctrl Pts',(-41.1738163525901,57.1094738174957,12.));
#93886=CARTESIAN_POINT('Ctrl Pts',(-41.1899882567923,57.1221647611207,0.));
#93887=CARTESIAN_POINT('Ctrl Pts',(-41.1899882567923,57.1221647611207,12.));
#93888=CARTESIAN_POINT('Ctrl Pts',(-41.2062138492915,57.1348702480647,0.));
#93889=CARTESIAN_POINT('Ctrl Pts',(-41.2062138492915,57.1348702480647,12.));
#93890=CARTESIAN_POINT('Ctrl Pts',(-41.222493046943,57.147590110182,0.));
#93891=CARTESIAN_POINT('Ctrl Pts',(-41.222493046943,57.147590110182,12.));
#93892=CARTESIAN_POINT('Ctrl Pts',(-41.2388257656559,57.1603241779077,0.));
#93893=CARTESIAN_POINT('Ctrl Pts',(-41.2388257656559,57.1603241779077,12.));
#93894=CARTESIAN_POINT('Ctrl Pts',(-41.2552119208465,57.17307228108,0.));
#93895=CARTESIAN_POINT('Ctrl Pts',(-41.2552119208465,57.17307228108,12.));
#93896=CARTESIAN_POINT('Ctrl Pts',(-41.2716514278276,57.1858342496538,0.));
#93897=CARTESIAN_POINT('Ctrl Pts',(-41.2716514278276,57.1858342496538,12.));
#93898=CARTESIAN_POINT('Ctrl Pts',(-41.2881442021863,57.1986099143983,0.));
#93899=CARTESIAN_POINT('Ctrl Pts',(-41.2881442021863,57.1986099143983,12.));
#93900=CARTESIAN_POINT('Ctrl Pts',(-41.3046901602293,57.2113991077302,0.));
#93901=CARTESIAN_POINT('Ctrl Pts',(-41.3046901602293,57.2113991077302,12.));
#93902=CARTESIAN_POINT('Ctrl Pts',(-41.321289219149,57.2242016640198,0.));
#93903=CARTESIAN_POINT('Ctrl Pts',(-41.321289219149,57.2242016640198,12.));
#93904=CARTESIAN_POINT('Ctrl Pts',(-41.3379412967875,57.2370174191401,0.));
#93905=CARTESIAN_POINT('Ctrl Pts',(-41.3379412967875,57.2370174191401,12.));
#93906=CARTESIAN_POINT('Ctrl Pts',(-41.3546463114885,57.2498462101879,0.));
#93907=CARTESIAN_POINT('Ctrl Pts',(-41.3546463114885,57.2498462101879,12.));
#93908=CARTESIAN_POINT('Ctrl Pts',(-41.3714041819223,57.2626878751596,0.));
#93909=CARTESIAN_POINT('Ctrl Pts',(-41.3714041819223,57.2626878751596,12.));
#93910=CARTESIAN_POINT('Ctrl Pts',(-41.3882148268813,57.2755422525844,0.));
#93911=CARTESIAN_POINT('Ctrl Pts',(-41.3882148268813,57.2755422525844,12.));
#93912=CARTESIAN_POINT('Ctrl Pts',(-41.4050781652938,57.2884091815406,0.));
#93913=CARTESIAN_POINT('Ctrl Pts',(-41.4050781652938,57.2884091815406,12.));
#93914=CARTESIAN_POINT('Ctrl Pts',(-41.4219941163163,57.3012885018151,0.));
#93915=CARTESIAN_POINT('Ctrl Pts',(-41.4219941163163,57.3012885018151,12.));
#93916=CARTESIAN_POINT('Ctrl Pts',(-41.4389625993948,57.3141800540137,0.));
#93917=CARTESIAN_POINT('Ctrl Pts',(-41.4389625993948,57.3141800540137,12.));
#93918=CARTESIAN_POINT('Ctrl Pts',(-41.4559835343328,57.3270836796911,0.));
#93919=CARTESIAN_POINT('Ctrl Pts',(-41.4559835343328,57.3270836796911,12.));
#93920=CARTESIAN_POINT('Ctrl Pts',(-41.4730568413518,57.3399992214717,0.));
#93921=CARTESIAN_POINT('Ctrl Pts',(-41.4730568413518,57.3399992214717,12.));
#93922=CARTESIAN_POINT('Ctrl Pts',(-41.4901824410636,57.3529265229835,0.));
#93923=CARTESIAN_POINT('Ctrl Pts',(-41.4901824410636,57.3529265229835,12.));
#93924=CARTESIAN_POINT('Ctrl Pts',(-41.5073602544396,57.3658654287937,0.));
#93925=CARTESIAN_POINT('Ctrl Pts',(-41.5073602544396,57.3658654287937,12.));
#93926=CARTESIAN_POINT('Ctrl Pts',(-41.524590202777,57.3788157843454,0.));
#93927=CARTESIAN_POINT('Ctrl Pts',(-41.524590202777,57.3788157843454,12.));
#93928=CARTESIAN_POINT('Ctrl Pts',(-41.5418722076572,57.3917774358863,0.));
#93929=CARTESIAN_POINT('Ctrl Pts',(-41.5418722076572,57.3917774358863,12.));
#93930=CARTESIAN_POINT('Ctrl Pts',(-41.5592061909176,57.4047502304231,0.));
#93931=CARTESIAN_POINT('Ctrl Pts',(-41.5592061909176,57.4047502304231,12.));
#93932=CARTESIAN_POINT('Ctrl Pts',(-41.5765920746777,57.4177340157508,0.));
#93933=CARTESIAN_POINT('Ctrl Pts',(-41.5765920746777,57.4177340157508,12.));
#93934=CARTESIAN_POINT('Ctrl Pts',(-41.5940297813477,57.4307286404662,0.));
#93935=CARTESIAN_POINT('Ctrl Pts',(-41.5940297813477,57.4307286404662,12.));
#93936=CARTESIAN_POINT('Ctrl Pts',(-41.6115192336388,57.4437339539841,0.));
#93937=CARTESIAN_POINT('Ctrl Pts',(-41.6115192336388,57.4437339539841,12.));
#93938=CARTESIAN_POINT('Ctrl Pts',(-41.6290603545666,57.4567498065562,0.));
#93939=CARTESIAN_POINT('Ctrl Pts',(-41.6290603545666,57.4567498065562,12.));
#93940=CARTESIAN_POINT('Ctrl Pts',(-41.6466530674514,57.4697760492683,0.));
#93941=CARTESIAN_POINT('Ctrl Pts',(-41.6466530674514,57.4697760492683,12.));
#93942=CARTESIAN_POINT('Ctrl Pts',(-41.6642972959165,57.4828125340218,0.));
#93943=CARTESIAN_POINT('Ctrl Pts',(-41.6642972959165,57.4828125340218,12.));
#93944=CARTESIAN_POINT('Ctrl Pts',(-41.6819929638797,57.4958591135165,0.));
#93945=CARTESIAN_POINT('Ctrl Pts',(-41.6819929638797,57.4958591135165,12.));
#93946=CARTESIAN_POINT('Ctrl Pts',(-41.6997399955447,57.5089156412343,0.));
#93947=CARTESIAN_POINT('Ctrl Pts',(-41.6997399955447,57.5089156412343,12.));
#93948=CARTESIAN_POINT('Ctrl Pts',(-41.7175383153821,57.5219819714171,0.));
#93949=CARTESIAN_POINT('Ctrl Pts',(-41.7175383153821,57.5219819714171,12.));
#93950=CARTESIAN_POINT('Ctrl Pts',(-41.7353878481336,57.5350579590649,0.));
#93951=CARTESIAN_POINT('Ctrl Pts',(-41.7353878481336,57.5350579590649,12.));
#93952=CARTESIAN_POINT('Ctrl Pts',(-41.7532885188174,57.5481434599335,0.));
#93953=CARTESIAN_POINT('Ctrl Pts',(-41.7532885188174,57.5481434599335,12.));
#93954=CARTESIAN_POINT('Ctrl Pts',(-41.7712402527273,57.561238330532,0.));
#93955=CARTESIAN_POINT('Ctrl Pts',(-41.7712402527273,57.561238330532,12.));
#93956=CARTESIAN_POINT('Ctrl Pts',(-41.7892429754297,57.5743424281205,0.));
#93957=CARTESIAN_POINT('Ctrl Pts',(-41.7892429754297,57.5743424281205,12.));
#93958=CARTESIAN_POINT('Ctrl Pts',(-41.8072966127558,57.5874556107056,0.));
#93959=CARTESIAN_POINT('Ctrl Pts',(-41.8072966127558,57.5874556107056,12.));
#93960=CARTESIAN_POINT('Ctrl Pts',(-41.8254010908051,57.6005777370349,0.));
#93961=CARTESIAN_POINT('Ctrl Pts',(-41.8254010908051,57.6005777370349,12.));
#93962=CARTESIAN_POINT('Ctrl Pts',(-41.8435563359456,57.6137086665882,0.));
#93963=CARTESIAN_POINT('Ctrl Pts',(-41.8435563359456,57.6137086665882,12.));
#93964=CARTESIAN_POINT('Ctrl Pts',(-41.8617622748108,57.6268482595702,0.));
#93965=CARTESIAN_POINT('Ctrl Pts',(-41.8617622748108,57.6268482595702,12.));
#93966=CARTESIAN_POINT('Ctrl Pts',(-41.8800188342908,57.6399963769003,0.));
#93967=CARTESIAN_POINT('Ctrl Pts',(-41.8800188342908,57.6399963769003,12.));
#93968=CARTESIAN_POINT('Ctrl Pts',(-41.8983259415244,57.6531528802059,0.));
#93969=CARTESIAN_POINT('Ctrl Pts',(-41.8983259415244,57.6531528802059,12.));
#93970=CARTESIAN_POINT('Ctrl Pts',(-41.9166835239046,57.6663176318176,0.));
#93971=CARTESIAN_POINT('Ctrl Pts',(-41.9166835239046,57.6663176318176,12.));
#93972=CARTESIAN_POINT('Ctrl Pts',(-41.9350915090791,57.6794904947641,0.));
#93973=CARTESIAN_POINT('Ctrl Pts',(-41.9350915090791,57.6794904947641,12.));
#93974=CARTESIAN_POINT('Ctrl Pts',(-41.9535498249489,57.6926713327674,0.));
#93975=CARTESIAN_POINT('Ctrl Pts',(-41.9535498249489,57.6926713327674,12.));
#93976=CARTESIAN_POINT('Ctrl Pts',(-41.9720583996601,57.7058600102365,0.));
#93977=CARTESIAN_POINT('Ctrl Pts',(-41.9720583996601,57.7058600102365,12.));
#93978=CARTESIAN_POINT('Ctrl Pts',(-41.9906171615974,57.7190563922614,0.));
#93979=CARTESIAN_POINT('Ctrl Pts',(-41.9906171615974,57.7190563922614,12.));
#93980=CARTESIAN_POINT('Ctrl Pts',(-42.0092260393911,57.7322603446086,0.));
#93981=CARTESIAN_POINT('Ctrl Pts',(-42.0092260393911,57.7322603446086,12.));
#93982=CARTESIAN_POINT('Ctrl Pts',(-42.0278849619156,57.7454717337151,0.));
#93983=CARTESIAN_POINT('Ctrl Pts',(-42.0278849619156,57.7454717337151,12.));
#93984=CARTESIAN_POINT('Ctrl Pts',(-42.0465938582877,57.7586904266828,0.));
#93985=CARTESIAN_POINT('Ctrl Pts',(-42.0465938582877,57.7586904266828,12.));
#93986=CARTESIAN_POINT('Ctrl Pts',(-42.0653526578571,57.7719162912721,0.));
#93987=CARTESIAN_POINT('Ctrl Pts',(-42.0653526578571,57.7719162912721,12.));
#93988=CARTESIAN_POINT('Ctrl Pts',(-42.0841612902018,57.7851491958954,0.));
#93989=CARTESIAN_POINT('Ctrl Pts',(-42.0841612902018,57.7851491958954,12.));
#93990=CARTESIAN_POINT('Ctrl Pts',(-42.1030196851344,57.798389009613,0.));
#93991=CARTESIAN_POINT('Ctrl Pts',(-42.1030196851344,57.798389009613,12.));
#93992=CARTESIAN_POINT('Ctrl Pts',(-42.121927772701,57.8116356021274,0.));
#93993=CARTESIAN_POINT('Ctrl Pts',(-42.121927772701,57.8116356021274,12.));
#93994=CARTESIAN_POINT('Ctrl Pts',(-42.1408854831791,57.8248888437787,0.));
#93995=CARTESIAN_POINT('Ctrl Pts',(-42.1408854831791,57.8248888437787,12.));
#93996=CARTESIAN_POINT('Ctrl Pts',(-42.1598927470671,57.8381486055376,0.));
#93997=CARTESIAN_POINT('Ctrl Pts',(-42.1598927470671,57.8381486055376,12.));
#93998=CARTESIAN_POINT('Ctrl Pts',(-42.1789494950824,57.8514147590012,0.));
#93999=CARTESIAN_POINT('Ctrl Pts',(-42.1789494950824,57.8514147590012,12.));
#94000=CARTESIAN_POINT('Ctrl Pts',(-42.1980556581688,57.86468717639,0.));
#94001=CARTESIAN_POINT('Ctrl Pts',(-42.1980556581688,57.86468717639,12.));
#94002=CARTESIAN_POINT('Ctrl Pts',(-42.2172111674945,57.8779657305423,0.));
#94003=CARTESIAN_POINT('Ctrl Pts',(-42.2172111674945,57.8779657305423,12.));
#94004=CARTESIAN_POINT('Ctrl Pts',(-42.2364159544492,57.8912502949084,0.));
#94005=CARTESIAN_POINT('Ctrl Pts',(-42.2364159544492,57.8912502949084,12.));
#94006=CARTESIAN_POINT('Ctrl Pts',(-42.2556699506332,57.9045407435447,0.));
#94007=CARTESIAN_POINT('Ctrl Pts',(-42.2556699506332,57.9045407435447,12.));
#94008=CARTESIAN_POINT('Ctrl Pts',(-42.274973087857,57.9178369511084,0.));
#94009=CARTESIAN_POINT('Ctrl Pts',(-42.274973087857,57.9178369511084,12.));
#94010=CARTESIAN_POINT('Ctrl Pts',(-42.2943252981471,57.9311387928541,0.));
#94011=CARTESIAN_POINT('Ctrl Pts',(-42.2943252981471,57.9311387928541,12.));
#94012=CARTESIAN_POINT('Ctrl Pts',(-42.3137265137446,57.9444461446292,0.));
#94013=CARTESIAN_POINT('Ctrl Pts',(-42.3137265137446,57.9444461446292,12.));
#94014=CARTESIAN_POINT('Ctrl Pts',(-42.3331766671028,57.9577588828693,0.));
#94015=CARTESIAN_POINT('Ctrl Pts',(-42.3331766671028,57.9577588828693,12.));
#94016=CARTESIAN_POINT('Ctrl Pts',(-42.3526756908764,57.9710768845923,0.));
#94017=CARTESIAN_POINT('Ctrl Pts',(-42.3526756908764,57.9710768845923,12.));
#94018=CARTESIAN_POINT('Ctrl Pts',(-42.3722235179216,57.9844000273936,0.));
#94019=CARTESIAN_POINT('Ctrl Pts',(-42.3722235179216,57.9844000273936,12.));
#94020=CARTESIAN_POINT('Ctrl Pts',(-42.3918200813024,57.9977281894437,0.));
#94021=CARTESIAN_POINT('Ctrl Pts',(-42.3918200813024,57.9977281894437,12.));
#94022=CARTESIAN_POINT('Ctrl Pts',(-42.4114653142891,58.011061249483,0.));
#94023=CARTESIAN_POINT('Ctrl Pts',(-42.4114653142891,58.011061249483,12.));
#94024=CARTESIAN_POINT('Ctrl Pts',(-42.4311591503551,58.0243990868175,0.));
#94025=CARTESIAN_POINT('Ctrl Pts',(-42.4311591503551,58.0243990868175,12.));
#94026=CARTESIAN_POINT('Ctrl Pts',(-42.4509015231667,58.0377415813132,0.));
#94027=CARTESIAN_POINT('Ctrl Pts',(-42.4509015231667,58.0377415813132,12.));
#94028=CARTESIAN_POINT('Ctrl Pts',(-42.4706923665838,58.0510886133917,0.));
#94029=CARTESIAN_POINT('Ctrl Pts',(-42.4706923665838,58.0510886133917,12.));
#94030=CARTESIAN_POINT('Ctrl Pts',(-42.4905316146649,58.064440064027,0.));
#94031=CARTESIAN_POINT('Ctrl Pts',(-42.4905316146649,58.064440064027,12.));
#94032=CARTESIAN_POINT('Ctrl Pts',(-42.5104192016664,58.0777958147404,0.));
#94033=CARTESIAN_POINT('Ctrl Pts',(-42.5104192016664,58.0777958147404,12.));
#94034=CARTESIAN_POINT('Ctrl Pts',(-42.5303550620388,58.0911557475967,0.));
#94035=CARTESIAN_POINT('Ctrl Pts',(-42.5303550620388,58.0911557475967,12.));
#94036=CARTESIAN_POINT('Ctrl Pts',(-42.5503391304182,58.1045197452003,0.));
#94037=CARTESIAN_POINT('Ctrl Pts',(-42.5503391304182,58.1045197452003,12.));
#94038=CARTESIAN_POINT('Ctrl Pts',(-42.5703713416263,58.1178876906905,0.));
#94039=CARTESIAN_POINT('Ctrl Pts',(-42.5703713416263,58.1178876906905,12.));
#94040=CARTESIAN_POINT('Ctrl Pts',(-42.5904516306759,58.1312594677383,0.));
#94041=CARTESIAN_POINT('Ctrl Pts',(-42.5904516306759,58.1312594677383,12.));
#94042=CARTESIAN_POINT('Ctrl Pts',(-42.6105799327697,58.1446349605419,0.));
#94043=CARTESIAN_POINT('Ctrl Pts',(-42.6105799327697,58.1446349605419,12.));
#94044=CARTESIAN_POINT('Ctrl Pts',(-42.6307561832977,58.158014053823,0.));
#94045=CARTESIAN_POINT('Ctrl Pts',(-42.6307561832977,58.158014053823,12.));
#94046=CARTESIAN_POINT('Ctrl Pts',(-42.6509803178269,58.1713966328217,0.));
#94047=CARTESIAN_POINT('Ctrl Pts',(-42.6509803178269,58.1713966328217,12.));
#94048=CARTESIAN_POINT('Ctrl Pts',(-42.6712522721021,58.1847825832932,0.));
#94049=CARTESIAN_POINT('Ctrl Pts',(-42.6712522721021,58.1847825832932,12.));
#94050=CARTESIAN_POINT('Ctrl Pts',(-42.6915719820516,58.1981717915043,0.));
#94051=CARTESIAN_POINT('Ctrl Pts',(-42.6915719820516,58.1981717915043,12.));
#94052=CARTESIAN_POINT('Ctrl Pts',(-42.7119393837866,58.2115641442302,0.));
#94053=CARTESIAN_POINT('Ctrl Pts',(-42.7119393837866,58.2115641442302,12.));
#94054=CARTESIAN_POINT('Ctrl Pts',(-42.7323544135983,58.2249595287497,0.));
#94055=CARTESIAN_POINT('Ctrl Pts',(-42.7323544135983,58.2249595287497,12.));
#94056=CARTESIAN_POINT('Ctrl Pts',(-42.7528170079482,58.238357832842,0.));
#94057=CARTESIAN_POINT('Ctrl Pts',(-42.7528170079482,58.238357832842,12.));
#94058=CARTESIAN_POINT('Ctrl Pts',(-42.7733271034678,58.2517589447818,0.));
#94059=CARTESIAN_POINT('Ctrl Pts',(-42.7733271034678,58.2517589447818,12.));
#94060=CARTESIAN_POINT('Ctrl Pts',(-42.7938846369651,58.2651627533368,0.));
#94061=CARTESIAN_POINT('Ctrl Pts',(-42.7938846369651,58.2651627533368,12.));
#94062=CARTESIAN_POINT('Ctrl Pts',(-42.8144895454234,58.278569147764,0.));
#94063=CARTESIAN_POINT('Ctrl Pts',(-42.8144895454234,58.278569147764,12.));
#94064=CARTESIAN_POINT('Ctrl Pts',(-42.8351417659998,58.2919780178063,0.));
#94065=CARTESIAN_POINT('Ctrl Pts',(-42.8351417659998,58.2919780178063,12.));
#94066=CARTESIAN_POINT('Ctrl Pts',(-42.8558412360154,58.305389253689,0.));
#94067=CARTESIAN_POINT('Ctrl Pts',(-42.8558412360154,58.305389253689,12.));
#94068=CARTESIAN_POINT('Ctrl Pts',(-42.8765878929545,58.3188027461158,0.));
#94069=CARTESIAN_POINT('Ctrl Pts',(-42.8765878929545,58.3188027461158,12.));
#94070=CARTESIAN_POINT('Ctrl Pts',(-42.8973816744703,58.3322183862647,0.));
#94071=CARTESIAN_POINT('Ctrl Pts',(-42.8973816744703,58.3322183862647,12.));
#94072=CARTESIAN_POINT('Ctrl Pts',(-42.9182225183851,58.3456360657861,0.));
#94073=CARTESIAN_POINT('Ctrl Pts',(-42.9182225183851,58.3456360657861,12.));
#94074=CARTESIAN_POINT('Ctrl Pts',(-42.9391103626881,58.3590556767981,0.));
#94075=CARTESIAN_POINT('Ctrl Pts',(-42.9391103626881,58.3590556767981,12.));
#94076=CARTESIAN_POINT('Ctrl Pts',(-42.9600451455267,58.3724771118835,0.));
#94077=CARTESIAN_POINT('Ctrl Pts',(-42.9600451455267,58.3724771118835,12.));
#94078=CARTESIAN_POINT('Ctrl Pts',(-42.9810268052043,58.3859002640871,0.));
#94079=CARTESIAN_POINT('Ctrl Pts',(-42.9810268052043,58.3859002640871,12.));
#94080=CARTESIAN_POINT('Ctrl Pts',(-43.0020552801869,58.3993250269115,0.));
#94081=CARTESIAN_POINT('Ctrl Pts',(-43.0020552801869,58.3993250269115,12.));
#94082=CARTESIAN_POINT('Ctrl Pts',(-43.0231305091032,58.4127512943144,0.));
#94083=CARTESIAN_POINT('Ctrl Pts',(-43.0231305091032,58.4127512943144,12.));
#94084=CARTESIAN_POINT('Ctrl Pts',(-43.0442524307432,58.4261789607055,0.));
#94085=CARTESIAN_POINT('Ctrl Pts',(-43.0442524307432,58.4261789607055,12.));
#94086=CARTESIAN_POINT('Ctrl Pts',(-43.0654209840502,58.4396079209438,0.));
#94087=CARTESIAN_POINT('Ctrl Pts',(-43.0654209840502,58.4396079209438,12.));
#94088=CARTESIAN_POINT('Ctrl Pts',(-43.0866361081166,58.4530380703335,0.));
#94089=CARTESIAN_POINT('Ctrl Pts',(-43.0866361081166,58.4530380703335,12.));
#94090=CARTESIAN_POINT('Ctrl Pts',(-43.1078977421908,58.4664693046206,0.));
#94091=CARTESIAN_POINT('Ctrl Pts',(-43.1078977421908,58.4664693046206,12.));
#94092=CARTESIAN_POINT('Ctrl Pts',(-43.1292058256774,58.4799015199904,0.));
#94093=CARTESIAN_POINT('Ctrl Pts',(-43.1292058256774,58.4799015199904,12.));
#94094=CARTESIAN_POINT('Ctrl Pts',(-43.1505602981366,58.4933346130638,0.));
#94095=CARTESIAN_POINT('Ctrl Pts',(-43.1505602981366,58.4933346130638,12.));
#94096=CARTESIAN_POINT('Ctrl Pts',(-43.1719610992771,58.5067684808946,0.));
#94097=CARTESIAN_POINT('Ctrl Pts',(-43.1719610992771,58.5067684808946,12.));
#94098=CARTESIAN_POINT('Ctrl Pts',(-43.1934081689503,58.5202030209667,0.));
#94099=CARTESIAN_POINT('Ctrl Pts',(-43.1934081689503,58.5202030209667,12.));
#94100=CARTESIAN_POINT('Ctrl Pts',(-43.214901447157,58.5336381311911,0.));
#94101=CARTESIAN_POINT('Ctrl Pts',(-43.214901447157,58.5336381311911,12.));
#94102=CARTESIAN_POINT('Ctrl Pts',(-43.2364408740488,58.5470737099027,0.));
#94103=CARTESIAN_POINT('Ctrl Pts',(-43.2364408740488,58.5470737099027,12.));
#94104=CARTESIAN_POINT('Ctrl Pts',(-43.2580263899278,58.5605096558578,0.));
#94105=CARTESIAN_POINT('Ctrl Pts',(-43.2580263899278,58.5605096558578,12.));
#94106=CARTESIAN_POINT('Ctrl Pts',(-43.2796579352405,58.5739458682317,0.));
#94107=CARTESIAN_POINT('Ctrl Pts',(-43.2796579352405,58.5739458682317,12.));
#94108=CARTESIAN_POINT('Ctrl Pts',(-43.3013354505707,58.5873822466163,0.));
#94109=CARTESIAN_POINT('Ctrl Pts',(-43.3013354505707,58.5873822466163,12.));
#94110=CARTESIAN_POINT('Ctrl Pts',(-43.3230588766455,58.6008186910166,0.));
#94111=CARTESIAN_POINT('Ctrl Pts',(-43.3230588766455,58.6008186910166,12.));
#94112=CARTESIAN_POINT('Ctrl Pts',(-43.3448281543374,58.6142551018473,0.));
#94113=CARTESIAN_POINT('Ctrl Pts',(-43.3448281543374,58.6142551018473,12.));
#94114=CARTESIAN_POINT('Ctrl Pts',(-43.3666432246634,58.627691379929,0.));
#94115=CARTESIAN_POINT('Ctrl Pts',(-43.3666432246634,58.627691379929,12.));
#94116=CARTESIAN_POINT('Ctrl Pts',(-43.3885040287808,58.6411274264854,0.));
#94117=CARTESIAN_POINT('Ctrl Pts',(-43.3885040287808,58.6411274264854,12.));
#94118=CARTESIAN_POINT('Ctrl Pts',(-43.4104105079766,58.6545631431388,0.));
#94119=CARTESIAN_POINT('Ctrl Pts',(-43.4104105079766,58.6545631431388,12.));
#94120=CARTESIAN_POINT('Ctrl Pts',(-43.4323626036736,58.6679984319095,0.));
#94121=CARTESIAN_POINT('Ctrl Pts',(-43.4323626036736,58.6679984319095,12.));
#94122=CARTESIAN_POINT('Ctrl Pts',(-43.4543602574352,58.6814331952138,0.));
#94123=CARTESIAN_POINT('Ctrl Pts',(-43.4543602574352,58.6814331952138,12.));
#94124=CARTESIAN_POINT('Ctrl Pts',(-43.4764034109654,58.6948673358639,0.));
#94125=CARTESIAN_POINT('Ctrl Pts',(-43.4764034109654,58.6948673358639,12.));
#94126=CARTESIAN_POINT('Ctrl Pts',(-43.4984920061071,58.708300757066,0.));
#94127=CARTESIAN_POINT('Ctrl Pts',(-43.4984920061071,58.708300757066,12.));
#94128=CARTESIAN_POINT('Ctrl Pts',(-43.5206259848333,58.7217333624206,0.));
#94129=CARTESIAN_POINT('Ctrl Pts',(-43.5206259848333,58.7217333624206,12.));
#94130=CARTESIAN_POINT('Ctrl Pts',(-43.5428052892483,58.7351650559176,0.));
#94131=CARTESIAN_POINT('Ctrl Pts',(-43.5428052892483,58.7351650559176,12.));
#94132=CARTESIAN_POINT('Ctrl Pts',(-43.5650298615911,58.7485957419296,0.));
#94133=CARTESIAN_POINT('Ctrl Pts',(-43.5650298615911,58.7485957419296,12.));
#94134=CARTESIAN_POINT('Ctrl Pts',(-43.5872996442343,58.7620253252059,0.));
#94135=CARTESIAN_POINT('Ctrl Pts',(-43.5872996442343,58.7620253252059,12.));
#94136=CARTESIAN_POINT('Ctrl Pts',(-43.6096145796798,58.7754537108672,0.));
#94137=CARTESIAN_POINT('Ctrl Pts',(-43.6096145796798,58.7754537108672,12.));
#94138=CARTESIAN_POINT('Ctrl Pts',(-43.6319746105487,58.7888808043976,0.));
#94139=CARTESIAN_POINT('Ctrl Pts',(-43.6319746105487,58.7888808043976,12.));
#94140=CARTESIAN_POINT('Ctrl Pts',(-43.6543796795797,58.8023065116446,0.));
#94141=CARTESIAN_POINT('Ctrl Pts',(-43.6543796795797,58.8023065116446,12.));
#94142=CARTESIAN_POINT('Ctrl Pts',(-43.6768297296402,58.8157307388247,0.));
#94143=CARTESIAN_POINT('Ctrl Pts',(-43.6768297296402,58.8157307388247,12.));
#94144=CARTESIAN_POINT('Ctrl Pts',(-43.6993247037318,58.8291533925299,0.));
#94145=CARTESIAN_POINT('Ctrl Pts',(-43.6993247037318,58.8291533925299,12.));
#94146=CARTESIAN_POINT('Ctrl Pts',(-43.7218645449921,58.8425743797325,0.));
#94147=CARTESIAN_POINT('Ctrl Pts',(-43.7218645449921,58.8425743797325,12.));
#94148=CARTESIAN_POINT('Ctrl Pts',(-43.7444491966935,58.8559936077933,0.));
#94149=CARTESIAN_POINT('Ctrl Pts',(-43.7444491966935,58.8559936077933,12.));
#94150=CARTESIAN_POINT('Ctrl Pts',(-43.7670786022392,58.8694109844636,0.));
#94151=CARTESIAN_POINT('Ctrl Pts',(-43.7670786022392,58.8694109844636,12.));
#94152=CARTESIAN_POINT('Ctrl Pts',(-43.7897527051599,58.882826417861,0.));
#94153=CARTESIAN_POINT('Ctrl Pts',(-43.7897527051599,58.882826417861,12.));
#94154=CARTESIAN_POINT('Ctrl Pts',(-43.8124714491069,58.8962398164486,0.));
#94155=CARTESIAN_POINT('Ctrl Pts',(-43.8124714491069,58.8962398164486,12.));
#94156=CARTESIAN_POINT('Ctrl Pts',(-43.8352347778419,58.9096510890128,0.));
#94157=CARTESIAN_POINT('Ctrl Pts',(-43.8352347778419,58.9096510890128,12.));
#94158=CARTESIAN_POINT('Ctrl Pts',(-43.8580426352236,58.9230601446445,0.));
#94159=CARTESIAN_POINT('Ctrl Pts',(-43.8580426352236,58.9230601446445,12.));
#94160=CARTESIAN_POINT('Ctrl Pts',(-43.8808949651882,58.9364668927132,0.));
#94161=CARTESIAN_POINT('Ctrl Pts',(-43.8808949651882,58.9364668927132,12.));
#94162=CARTESIAN_POINT('Ctrl Pts',(-43.9037917117748,58.9498712429066,0.));
#94163=CARTESIAN_POINT('Ctrl Pts',(-43.9037917117748,58.9498712429066,12.));
#94164=CARTESIAN_POINT('Ctrl Pts',(-43.9267328191507,58.9632731052704,0.));
#94165=CARTESIAN_POINT('Ctrl Pts',(-43.9267328191507,58.9632731052704,12.));
#94166=CARTESIAN_POINT('Ctrl Pts',(-43.9497182316333,58.9766723902531,0.));
#94167=CARTESIAN_POINT('Ctrl Pts',(-43.9497182316333,58.9766723902531,12.));
#94168=CARTESIAN_POINT('Ctrl Pts',(-43.9727478937053,58.9900690087404,0.));
#94169=CARTESIAN_POINT('Ctrl Pts',(-43.9727478937053,58.9900690087404,12.));
#94170=CARTESIAN_POINT('Ctrl Pts',(-43.9958217500363,59.0034628721161,0.));
#94171=CARTESIAN_POINT('Ctrl Pts',(-43.9958217500363,59.0034628721161,12.));
#94172=CARTESIAN_POINT('Ctrl Pts',(-44.0189397454593,59.0168538922087,0.));
#94173=CARTESIAN_POINT('Ctrl Pts',(-44.0189397454593,59.0168538922087,12.));
#94174=CARTESIAN_POINT('Ctrl Pts',(-44.0421018249219,59.0302419811772,0.));
#94175=CARTESIAN_POINT('Ctrl Pts',(-44.0421018249219,59.0302419811772,12.));
#94176=CARTESIAN_POINT('Ctrl Pts',(-44.0653079334384,59.0436270514085,0.));
#94177=CARTESIAN_POINT('Ctrl Pts',(-44.0653079334384,59.0436270514085,12.));
#94178=CARTESIAN_POINT('Ctrl Pts',(-44.0885580160433,59.0570090154243,0.));
#94179=CARTESIAN_POINT('Ctrl Pts',(-44.0885580160433,59.0570090154243,12.));
#94180=CARTESIAN_POINT('Ctrl Pts',(-44.1118520177223,59.0703877857529,0.));
#94181=CARTESIAN_POINT('Ctrl Pts',(-44.1118520177223,59.0703877857529,12.));
#94182=CARTESIAN_POINT('Ctrl Pts',(-44.1351898834057,59.0837632749209,0.));
#94183=CARTESIAN_POINT('Ctrl Pts',(-44.1351898834057,59.0837632749209,12.));
#94184=CARTESIAN_POINT('Ctrl Pts',(-44.1585715581073,59.0971353957218,0.));
#94185=CARTESIAN_POINT('Ctrl Pts',(-44.1585715581073,59.0971353957218,12.));
#94186=CARTESIAN_POINT('Ctrl Pts',(-44.1819969870314,59.1105040614285,0.));
#94187=CARTESIAN_POINT('Ctrl Pts',(-44.1819969870314,59.1105040614285,12.));
#94188=CARTESIAN_POINT('Ctrl Pts',(-44.2054661156876,59.1238691860307,0.));
#94189=CARTESIAN_POINT('Ctrl Pts',(-44.2054661156876,59.1238691860307,12.));
#94190=CARTESIAN_POINT('Ctrl Pts',(-44.2289788899962,59.1372306844575,0.));
#94191=CARTESIAN_POINT('Ctrl Pts',(-44.2289788899962,59.1372306844575,12.));
#94192=CARTESIAN_POINT('Ctrl Pts',(-44.2525352563979,59.1505884728194,0.));
#94193=CARTESIAN_POINT('Ctrl Pts',(-44.2525352563979,59.1505884728194,12.));
#94194=CARTESIAN_POINT('Ctrl Pts',(-44.2761351616027,59.1639424678766,0.));
#94195=CARTESIAN_POINT('Ctrl Pts',(-44.2761351616027,59.1639424678766,12.));
#94196=CARTESIAN_POINT('Ctrl Pts',(-44.2997785523413,59.1772925865191,0.));
#94197=CARTESIAN_POINT('Ctrl Pts',(-44.2997785523413,59.1772925865191,12.));
#94198=CARTESIAN_POINT('Ctrl Pts',(-44.3234653750877,59.1906387451971,0.));
#94199=CARTESIAN_POINT('Ctrl Pts',(-44.3234653750877,59.1906387451971,12.));
#94200=CARTESIAN_POINT('Ctrl Pts',(-44.3471955758412,59.2039808594765,0.));
#94201=CARTESIAN_POINT('Ctrl Pts',(-44.3471955758412,59.2039808594765,12.));
#94202=CARTESIAN_POINT('Ctrl Pts',(-44.3709690997495,59.217318843283,0.));
#94203=CARTESIAN_POINT('Ctrl Pts',(-44.3709690997495,59.217318843283,12.));
#94204=CARTESIAN_POINT('Ctrl Pts',(-44.394785891411,59.2306526095175,0.));
#94205=CARTESIAN_POINT('Ctrl Pts',(-44.394785891411,59.2306526095175,12.));
#94206=CARTESIAN_POINT('Ctrl Pts',(-44.4186458955486,59.2439820714231,0.));
#94207=CARTESIAN_POINT('Ctrl Pts',(-44.4186458955486,59.2439820714231,12.));
#94208=CARTESIAN_POINT('Ctrl Pts',(-44.4425490575932,59.2573071437801,0.));
#94209=CARTESIAN_POINT('Ctrl Pts',(-44.4425490575932,59.2573071437801,12.));
#94210=CARTESIAN_POINT('Ctrl Pts',(-44.4664953242373,59.2706277440438,0.));
#94211=CARTESIAN_POINT('Ctrl Pts',(-44.4664953242373,59.2706277440438,12.));
#94212=CARTESIAN_POINT('Ctrl Pts',(-44.490484644147,59.2839437938187,0.));
#94213=CARTESIAN_POINT('Ctrl Pts',(-44.490484644147,59.2839437938187,12.));
#94214=CARTESIAN_POINT('Ctrl Pts',(-44.514516968128,59.2972552192072,0.));
#94215=CARTESIAN_POINT('Ctrl Pts',(-44.514516968128,59.2972552192072,12.));
#94216=CARTESIAN_POINT('Ctrl Pts',(-44.5385922475494,59.3105619475512,0.));
#94217=CARTESIAN_POINT('Ctrl Pts',(-44.5385922475494,59.3105619475512,12.));
#94218=CARTESIAN_POINT('Ctrl Pts',(-44.5627104330956,59.3238639048618,0.));
#94219=CARTESIAN_POINT('Ctrl Pts',(-44.5627104330956,59.3238639048618,12.));
#94220=CARTESIAN_POINT('Ctrl Pts',(-44.5868714733219,59.3371610128494,0.));
#94221=CARTESIAN_POINT('Ctrl Pts',(-44.5868714733219,59.3371610128494,12.));
#94222=CARTESIAN_POINT('Ctrl Pts',(-44.6110753134333,59.3504531864223,0.));
#94223=CARTESIAN_POINT('Ctrl Pts',(-44.6110753134333,59.3504531864223,12.));
#94224=CARTESIAN_POINT('Ctrl Pts',(-44.6353218935813,59.3637403301959,0.));
#94225=CARTESIAN_POINT('Ctrl Pts',(-44.6353218935813,59.3637403301959,12.));
#94226=CARTESIAN_POINT('Ctrl Pts',(-44.659611151286,59.3770223435405,0.));
#94227=CARTESIAN_POINT('Ctrl Pts',(-44.659611151286,59.3770223435405,12.));
#94228=CARTESIAN_POINT('Ctrl Pts',(-44.6839430244375,59.3902991268094,0.));
#94229=CARTESIAN_POINT('Ctrl Pts',(-44.6839430244375,59.3902991268094,12.));
#94230=CARTESIAN_POINT('Ctrl Pts',(-44.708317454179,59.403570587392,0.));
#94231=CARTESIAN_POINT('Ctrl Pts',(-44.708317454179,59.403570587392,12.));
#94232=CARTESIAN_POINT('Ctrl Pts',(-44.7327343876333,59.4168366453047,0.));
#94233=CARTESIAN_POINT('Ctrl Pts',(-44.7327343876333,59.4168366453047,12.));
#94234=CARTESIAN_POINT('Ctrl Pts',(-44.7571937811872,59.4300972402943,0.));
#94235=CARTESIAN_POINT('Ctrl Pts',(-44.7571937811872,59.4300972402943,12.));
#94236=CARTESIAN_POINT('Ctrl Pts',(-44.7816956017126,59.4433523334651,0.));
#94237=CARTESIAN_POINT('Ctrl Pts',(-44.7816956017126,59.4433523334651,12.));
#94238=CARTESIAN_POINT('Ctrl Pts',(-44.8062398250937,59.4566019017674,0.));
#94239=CARTESIAN_POINT('Ctrl Pts',(-44.8062398250937,59.4566019017674,12.));
#94240=CARTESIAN_POINT('Ctrl Pts',(-44.8259091133624,59.4671971277837,0.));
#94241=CARTESIAN_POINT('Ctrl Pts',(-44.8259091133624,59.4671971277837,12.));
#94242=CARTESIAN_POINT('Ctrl Pts',(-44.8406801497506,59.475141054744,0.));
#94243=CARTESIAN_POINT('Ctrl Pts',(-44.8406801497506,59.475141054744,12.));
#94244=CARTESIAN_POINT('Ctrl Pts',(-44.8505359826374,59.4804358982977,0.));
#94245=CARTESIAN_POINT('Ctrl Pts',(-44.8505359826374,59.4804358982977,12.));
#94246=CARTESIAN_POINT('Ctrl Pts',(-44.8554660179045,59.483083043136,0.));
#94247=CARTESIAN_POINT('Ctrl Pts',(-44.8554660179045,59.483083043136,12.));
#94248=CARTESIAN_POINT('',(-40.8467768343956,56.8466430164621,0.));
#94249=CARTESIAN_POINT('Ctrl Pts',(-40.8467768343956,56.8466430164621,0.));
#94250=CARTESIAN_POINT('Ctrl Pts',(-40.8497761671036,56.8491101022591,0.));
#94251=CARTESIAN_POINT('Ctrl Pts',(-40.8557803680277,56.8540460739472,0.));
#94252=CARTESIAN_POINT('Ctrl Pts',(-40.864803275942,56.8614554317668,0.));
#94253=CARTESIAN_POINT('Ctrl Pts',(-40.8768670342052,56.8713453764905,0.));
#94254=CARTESIAN_POINT('Ctrl Pts',(-40.8920020903293,56.8837257978343,0.));
#94255=CARTESIAN_POINT('Ctrl Pts',(-40.9071924937508,56.8961241708861,0.));
#94256=CARTESIAN_POINT('Ctrl Pts',(-40.9224382132427,56.9085404164502,0.));
#94257=CARTESIAN_POINT('Ctrl Pts',(-40.9377391857128,56.9209743960992,0.));
#94258=CARTESIAN_POINT('Ctrl Pts',(-40.9530953165031,56.9334259140049,0.));
#94259=CARTESIAN_POINT('Ctrl Pts',(-40.9685064933074,56.9458947422608,0.));
#94260=CARTESIAN_POINT('Ctrl Pts',(-40.9839725967121,56.9583806404069,0.));
#94261=CARTESIAN_POINT('Ctrl Pts',(-40.9994935117276,56.9708833766137,0.));
#94262=CARTESIAN_POINT('Ctrl Pts',(-41.0150691398947,56.9834027500117,0.));
#94263=CARTESIAN_POINT('Ctrl Pts',(-41.0306993953988,56.995938583472,0.));
#94264=CARTESIAN_POINT('Ctrl Pts',(-41.0463841993608,57.008490713042,0.));
#94265=CARTESIAN_POINT('Ctrl Pts',(-41.0621234751007,57.0210589791788,0.));
#94266=CARTESIAN_POINT('Ctrl Pts',(-41.0779171422438,57.0336432158536,0.));
#94267=CARTESIAN_POINT('Ctrl Pts',(-41.0937651137549,57.046243245068,0.));
#94268=CARTESIAN_POINT('Ctrl Pts',(-41.1096672990148,57.0588588825298,0.));
#94269=CARTESIAN_POINT('Ctrl Pts',(-41.1256236057442,57.0714899412099,0.));
#94270=CARTESIAN_POINT('Ctrl Pts',(-41.1416339422117,57.084136235426,0.));
#94271=CARTESIAN_POINT('Ctrl Pts',(-41.1576982197374,57.0967975854874,0.));
#94272=CARTESIAN_POINT('Ctrl Pts',(-41.1738163525901,57.1094738174957,0.));
#94273=CARTESIAN_POINT('Ctrl Pts',(-41.1899882567923,57.1221647611207,0.));
#94274=CARTESIAN_POINT('Ctrl Pts',(-41.2062138492915,57.1348702480647,0.));
#94275=CARTESIAN_POINT('Ctrl Pts',(-41.222493046943,57.147590110182,0.));
#94276=CARTESIAN_POINT('Ctrl Pts',(-41.2388257656559,57.1603241779077,0.));
#94277=CARTESIAN_POINT('Ctrl Pts',(-41.2552119208465,57.17307228108,0.));
#94278=CARTESIAN_POINT('Ctrl Pts',(-41.2716514278276,57.1858342496538,0.));
#94279=CARTESIAN_POINT('Ctrl Pts',(-41.2881442021863,57.1986099143983,0.));
#94280=CARTESIAN_POINT('Ctrl Pts',(-41.3046901602293,57.2113991077302,0.));
#94281=CARTESIAN_POINT('Ctrl Pts',(-41.321289219149,57.2242016640198,0.));
#94282=CARTESIAN_POINT('Ctrl Pts',(-41.3379412967875,57.2370174191401,0.));
#94283=CARTESIAN_POINT('Ctrl Pts',(-41.3546463114885,57.2498462101879,0.));
#94284=CARTESIAN_POINT('Ctrl Pts',(-41.3714041819223,57.2626878751596,0.));
#94285=CARTESIAN_POINT('Ctrl Pts',(-41.3882148268813,57.2755422525844,0.));
#94286=CARTESIAN_POINT('Ctrl Pts',(-41.4050781652938,57.2884091815406,0.));
#94287=CARTESIAN_POINT('Ctrl Pts',(-41.4219941163163,57.3012885018151,0.));
#94288=CARTESIAN_POINT('Ctrl Pts',(-41.4389625993948,57.3141800540137,0.));
#94289=CARTESIAN_POINT('Ctrl Pts',(-41.4559835343328,57.3270836796911,0.));
#94290=CARTESIAN_POINT('Ctrl Pts',(-41.4730568413518,57.3399992214717,0.));
#94291=CARTESIAN_POINT('Ctrl Pts',(-41.4901824410636,57.3529265229835,0.));
#94292=CARTESIAN_POINT('Ctrl Pts',(-41.5073602544396,57.3658654287937,0.));
#94293=CARTESIAN_POINT('Ctrl Pts',(-41.524590202777,57.3788157843454,0.));
#94294=CARTESIAN_POINT('Ctrl Pts',(-41.5418722076572,57.3917774358863,0.));
#94295=CARTESIAN_POINT('Ctrl Pts',(-41.5592061909176,57.4047502304231,0.));
#94296=CARTESIAN_POINT('Ctrl Pts',(-41.5765920746777,57.4177340157508,0.));
#94297=CARTESIAN_POINT('Ctrl Pts',(-41.5940297813477,57.4307286404662,0.));
#94298=CARTESIAN_POINT('Ctrl Pts',(-41.6115192336388,57.4437339539841,0.));
#94299=CARTESIAN_POINT('Ctrl Pts',(-41.6290603545666,57.4567498065562,0.));
#94300=CARTESIAN_POINT('Ctrl Pts',(-41.6466530674514,57.4697760492683,0.));
#94301=CARTESIAN_POINT('Ctrl Pts',(-41.6642972959165,57.4828125340218,0.));
#94302=CARTESIAN_POINT('Ctrl Pts',(-41.6819929638797,57.4958591135165,0.));
#94303=CARTESIAN_POINT('Ctrl Pts',(-41.6997399955447,57.5089156412343,0.));
#94304=CARTESIAN_POINT('Ctrl Pts',(-41.7175383153821,57.5219819714171,0.));
#94305=CARTESIAN_POINT('Ctrl Pts',(-41.7353878481336,57.5350579590649,0.));
#94306=CARTESIAN_POINT('Ctrl Pts',(-41.7532885188174,57.5481434599335,0.));
#94307=CARTESIAN_POINT('Ctrl Pts',(-41.7712402527273,57.561238330532,0.));
#94308=CARTESIAN_POINT('Ctrl Pts',(-41.7892429754297,57.5743424281205,0.));
#94309=CARTESIAN_POINT('Ctrl Pts',(-41.8072966127558,57.5874556107056,0.));
#94310=CARTESIAN_POINT('Ctrl Pts',(-41.8254010908051,57.6005777370349,0.));
#94311=CARTESIAN_POINT('Ctrl Pts',(-41.8435563359456,57.6137086665882,0.));
#94312=CARTESIAN_POINT('Ctrl Pts',(-41.8617622748108,57.6268482595702,0.));
#94313=CARTESIAN_POINT('Ctrl Pts',(-41.8800188342908,57.6399963769003,0.));
#94314=CARTESIAN_POINT('Ctrl Pts',(-41.8983259415244,57.6531528802059,0.));
#94315=CARTESIAN_POINT('Ctrl Pts',(-41.9166835239046,57.6663176318176,0.));
#94316=CARTESIAN_POINT('Ctrl Pts',(-41.9350915090791,57.6794904947641,0.));
#94317=CARTESIAN_POINT('Ctrl Pts',(-41.9535498249489,57.6926713327674,0.));
#94318=CARTESIAN_POINT('Ctrl Pts',(-41.9720583996601,57.7058600102365,0.));
#94319=CARTESIAN_POINT('Ctrl Pts',(-41.9906171615974,57.7190563922614,0.));
#94320=CARTESIAN_POINT('Ctrl Pts',(-42.0092260393911,57.7322603446086,0.));
#94321=CARTESIAN_POINT('Ctrl Pts',(-42.0278849619156,57.7454717337151,0.));
#94322=CARTESIAN_POINT('Ctrl Pts',(-42.0465938582877,57.7586904266828,0.));
#94323=CARTESIAN_POINT('Ctrl Pts',(-42.0653526578571,57.7719162912721,0.));
#94324=CARTESIAN_POINT('Ctrl Pts',(-42.0841612902018,57.7851491958954,0.));
#94325=CARTESIAN_POINT('Ctrl Pts',(-42.1030196851344,57.798389009613,0.));
#94326=CARTESIAN_POINT('Ctrl Pts',(-42.121927772701,57.8116356021274,0.));
#94327=CARTESIAN_POINT('Ctrl Pts',(-42.1408854831791,57.8248888437787,0.));
#94328=CARTESIAN_POINT('Ctrl Pts',(-42.1598927470671,57.8381486055376,0.));
#94329=CARTESIAN_POINT('Ctrl Pts',(-42.1789494950824,57.8514147590012,0.));
#94330=CARTESIAN_POINT('Ctrl Pts',(-42.1980556581688,57.86468717639,0.));
#94331=CARTESIAN_POINT('Ctrl Pts',(-42.2172111674945,57.8779657305423,0.));
#94332=CARTESIAN_POINT('Ctrl Pts',(-42.2364159544492,57.8912502949084,0.));
#94333=CARTESIAN_POINT('Ctrl Pts',(-42.2556699506332,57.9045407435447,0.));
#94334=CARTESIAN_POINT('Ctrl Pts',(-42.274973087857,57.9178369511084,0.));
#94335=CARTESIAN_POINT('Ctrl Pts',(-42.2943252981471,57.9311387928541,0.));
#94336=CARTESIAN_POINT('Ctrl Pts',(-42.3137265137446,57.9444461446292,0.));
#94337=CARTESIAN_POINT('Ctrl Pts',(-42.3331766671028,57.9577588828693,0.));
#94338=CARTESIAN_POINT('Ctrl Pts',(-42.3526756908764,57.9710768845923,0.));
#94339=CARTESIAN_POINT('Ctrl Pts',(-42.3722235179216,57.9844000273936,0.));
#94340=CARTESIAN_POINT('Ctrl Pts',(-42.3918200813024,57.9977281894437,0.));
#94341=CARTESIAN_POINT('Ctrl Pts',(-42.4114653142891,58.011061249483,0.));
#94342=CARTESIAN_POINT('Ctrl Pts',(-42.4311591503551,58.0243990868175,0.));
#94343=CARTESIAN_POINT('Ctrl Pts',(-42.4509015231667,58.0377415813132,0.));
#94344=CARTESIAN_POINT('Ctrl Pts',(-42.4706923665838,58.0510886133917,0.));
#94345=CARTESIAN_POINT('Ctrl Pts',(-42.4905316146649,58.064440064027,0.));
#94346=CARTESIAN_POINT('Ctrl Pts',(-42.5104192016664,58.0777958147404,0.));
#94347=CARTESIAN_POINT('Ctrl Pts',(-42.5303550620388,58.0911557475967,0.));
#94348=CARTESIAN_POINT('Ctrl Pts',(-42.5503391304182,58.1045197452003,0.));
#94349=CARTESIAN_POINT('Ctrl Pts',(-42.5703713416263,58.1178876906905,0.));
#94350=CARTESIAN_POINT('Ctrl Pts',(-42.5904516306759,58.1312594677383,0.));
#94351=CARTESIAN_POINT('Ctrl Pts',(-42.6105799327697,58.1446349605419,0.));
#94352=CARTESIAN_POINT('Ctrl Pts',(-42.6307561832977,58.158014053823,0.));
#94353=CARTESIAN_POINT('Ctrl Pts',(-42.6509803178269,58.1713966328217,0.));
#94354=CARTESIAN_POINT('Ctrl Pts',(-42.6712522721021,58.1847825832932,0.));
#94355=CARTESIAN_POINT('Ctrl Pts',(-42.6915719820516,58.1981717915043,0.));
#94356=CARTESIAN_POINT('Ctrl Pts',(-42.7119393837866,58.2115641442302,0.));
#94357=CARTESIAN_POINT('Ctrl Pts',(-42.7323544135983,58.2249595287497,0.));
#94358=CARTESIAN_POINT('Ctrl Pts',(-42.7528170079482,58.238357832842,0.));
#94359=CARTESIAN_POINT('Ctrl Pts',(-42.7733271034678,58.2517589447818,0.));
#94360=CARTESIAN_POINT('Ctrl Pts',(-42.7938846369651,58.2651627533368,0.));
#94361=CARTESIAN_POINT('Ctrl Pts',(-42.8144895454234,58.278569147764,0.));
#94362=CARTESIAN_POINT('Ctrl Pts',(-42.8351417659998,58.2919780178063,0.));
#94363=CARTESIAN_POINT('Ctrl Pts',(-42.8558412360154,58.305389253689,0.));
#94364=CARTESIAN_POINT('Ctrl Pts',(-42.8765878929545,58.3188027461158,0.));
#94365=CARTESIAN_POINT('Ctrl Pts',(-42.8973816744703,58.3322183862647,0.));
#94366=CARTESIAN_POINT('Ctrl Pts',(-42.9182225183851,58.3456360657861,0.));
#94367=CARTESIAN_POINT('Ctrl Pts',(-42.9391103626881,58.3590556767981,0.));
#94368=CARTESIAN_POINT('Ctrl Pts',(-42.9600451455267,58.3724771118835,0.));
#94369=CARTESIAN_POINT('Ctrl Pts',(-42.9810268052043,58.3859002640871,0.));
#94370=CARTESIAN_POINT('Ctrl Pts',(-43.0020552801869,58.3993250269115,0.));
#94371=CARTESIAN_POINT('Ctrl Pts',(-43.0231305091032,58.4127512943144,0.));
#94372=CARTESIAN_POINT('Ctrl Pts',(-43.0442524307432,58.4261789607055,0.));
#94373=CARTESIAN_POINT('Ctrl Pts',(-43.0654209840502,58.4396079209438,0.));
#94374=CARTESIAN_POINT('Ctrl Pts',(-43.0866361081166,58.4530380703335,0.));
#94375=CARTESIAN_POINT('Ctrl Pts',(-43.1078977421908,58.4664693046206,0.));
#94376=CARTESIAN_POINT('Ctrl Pts',(-43.1292058256774,58.4799015199904,0.));
#94377=CARTESIAN_POINT('Ctrl Pts',(-43.1505602981366,58.4933346130638,0.));
#94378=CARTESIAN_POINT('Ctrl Pts',(-43.1719610992771,58.5067684808946,0.));
#94379=CARTESIAN_POINT('Ctrl Pts',(-43.1934081689503,58.5202030209667,0.));
#94380=CARTESIAN_POINT('Ctrl Pts',(-43.214901447157,58.5336381311911,0.));
#94381=CARTESIAN_POINT('Ctrl Pts',(-43.2364408740488,58.5470737099027,0.));
#94382=CARTESIAN_POINT('Ctrl Pts',(-43.2580263899278,58.5605096558578,0.));
#94383=CARTESIAN_POINT('Ctrl Pts',(-43.2796579352405,58.5739458682317,0.));
#94384=CARTESIAN_POINT('Ctrl Pts',(-43.3013354505707,58.5873822466163,0.));
#94385=CARTESIAN_POINT('Ctrl Pts',(-43.3230588766455,58.6008186910166,0.));
#94386=CARTESIAN_POINT('Ctrl Pts',(-43.3448281543374,58.6142551018473,0.));
#94387=CARTESIAN_POINT('Ctrl Pts',(-43.3666432246634,58.627691379929,0.));
#94388=CARTESIAN_POINT('Ctrl Pts',(-43.3885040287808,58.6411274264854,0.));
#94389=CARTESIAN_POINT('Ctrl Pts',(-43.4104105079766,58.6545631431388,0.));
#94390=CARTESIAN_POINT('Ctrl Pts',(-43.4323626036736,58.6679984319095,0.));
#94391=CARTESIAN_POINT('Ctrl Pts',(-43.4543602574352,58.6814331952138,0.));
#94392=CARTESIAN_POINT('Ctrl Pts',(-43.4764034109654,58.6948673358639,0.));
#94393=CARTESIAN_POINT('Ctrl Pts',(-43.4984920061071,58.708300757066,0.));
#94394=CARTESIAN_POINT('Ctrl Pts',(-43.5206259848333,58.7217333624206,0.));
#94395=CARTESIAN_POINT('Ctrl Pts',(-43.5428052892483,58.7351650559176,0.));
#94396=CARTESIAN_POINT('Ctrl Pts',(-43.5650298615911,58.7485957419296,0.));
#94397=CARTESIAN_POINT('Ctrl Pts',(-43.5872996442343,58.7620253252059,0.));
#94398=CARTESIAN_POINT('Ctrl Pts',(-43.6096145796798,58.7754537108672,0.));
#94399=CARTESIAN_POINT('Ctrl Pts',(-43.6319746105487,58.7888808043976,0.));
#94400=CARTESIAN_POINT('Ctrl Pts',(-43.6543796795797,58.8023065116446,0.));
#94401=CARTESIAN_POINT('Ctrl Pts',(-43.6768297296402,58.8157307388247,0.));
#94402=CARTESIAN_POINT('Ctrl Pts',(-43.6993247037318,58.8291533925299,0.));
#94403=CARTESIAN_POINT('Ctrl Pts',(-43.7218645449921,58.8425743797325,0.));
#94404=CARTESIAN_POINT('Ctrl Pts',(-43.7444491966935,58.8559936077933,0.));
#94405=CARTESIAN_POINT('Ctrl Pts',(-43.7670786022392,58.8694109844636,0.));
#94406=CARTESIAN_POINT('Ctrl Pts',(-43.7897527051599,58.882826417861,0.));
#94407=CARTESIAN_POINT('Ctrl Pts',(-43.8124714491069,58.8962398164486,0.));
#94408=CARTESIAN_POINT('Ctrl Pts',(-43.8352347778419,58.9096510890128,0.));
#94409=CARTESIAN_POINT('Ctrl Pts',(-43.8580426352236,58.9230601446445,0.));
#94410=CARTESIAN_POINT('Ctrl Pts',(-43.8808949651882,58.9364668927132,0.));
#94411=CARTESIAN_POINT('Ctrl Pts',(-43.9037917117748,58.9498712429066,0.));
#94412=CARTESIAN_POINT('Ctrl Pts',(-43.9267328191507,58.9632731052704,0.));
#94413=CARTESIAN_POINT('Ctrl Pts',(-43.9497182316333,58.9766723902531,0.));
#94414=CARTESIAN_POINT('Ctrl Pts',(-43.9727478937053,58.9900690087404,0.));
#94415=CARTESIAN_POINT('Ctrl Pts',(-43.9958217500363,59.0034628721161,0.));
#94416=CARTESIAN_POINT('Ctrl Pts',(-44.0189397454593,59.0168538922087,0.));
#94417=CARTESIAN_POINT('Ctrl Pts',(-44.0421018249219,59.0302419811772,0.));
#94418=CARTESIAN_POINT('Ctrl Pts',(-44.0653079334384,59.0436270514085,0.));
#94419=CARTESIAN_POINT('Ctrl Pts',(-44.0885580160433,59.0570090154243,0.));
#94420=CARTESIAN_POINT('Ctrl Pts',(-44.1118520177223,59.0703877857529,0.));
#94421=CARTESIAN_POINT('Ctrl Pts',(-44.1351898834057,59.0837632749209,0.));
#94422=CARTESIAN_POINT('Ctrl Pts',(-44.1585715581073,59.0971353957218,0.));
#94423=CARTESIAN_POINT('Ctrl Pts',(-44.1819969870314,59.1105040614285,0.));
#94424=CARTESIAN_POINT('Ctrl Pts',(-44.2054661156876,59.1238691860307,0.));
#94425=CARTESIAN_POINT('Ctrl Pts',(-44.2289788899962,59.1372306844575,0.));
#94426=CARTESIAN_POINT('Ctrl Pts',(-44.2525352563979,59.1505884728194,0.));
#94427=CARTESIAN_POINT('Ctrl Pts',(-44.2761351616027,59.1639424678766,0.));
#94428=CARTESIAN_POINT('Ctrl Pts',(-44.2997785523413,59.1772925865191,0.));
#94429=CARTESIAN_POINT('Ctrl Pts',(-44.3234653750877,59.1906387451971,0.));
#94430=CARTESIAN_POINT('Ctrl Pts',(-44.3471955758412,59.2039808594765,0.));
#94431=CARTESIAN_POINT('Ctrl Pts',(-44.3709690997495,59.217318843283,0.));
#94432=CARTESIAN_POINT('Ctrl Pts',(-44.394785891411,59.2306526095175,0.));
#94433=CARTESIAN_POINT('Ctrl Pts',(-44.4186458955486,59.2439820714231,0.));
#94434=CARTESIAN_POINT('Ctrl Pts',(-44.4425490575932,59.2573071437801,0.));
#94435=CARTESIAN_POINT('Ctrl Pts',(-44.4664953242373,59.2706277440438,0.));
#94436=CARTESIAN_POINT('Ctrl Pts',(-44.490484644147,59.2839437938187,0.));
#94437=CARTESIAN_POINT('Ctrl Pts',(-44.514516968128,59.2972552192072,0.));
#94438=CARTESIAN_POINT('Ctrl Pts',(-44.5351541478336,59.3086616639392,0.));
#94439=CARTESIAN_POINT('Ctrl Pts',(-44.5509994357954,59.317404187219,0.));
#94440=CARTESIAN_POINT('Ctrl Pts',(-44.5620338188485,59.3234848865278,0.));
#94441=CARTESIAN_POINT('Ctrl Pts',(-44.5682447395713,59.3269051738222,0.));
#94442=CARTESIAN_POINT('Ctrl Pts',(-44.569626075742,59.3276657444158,0.));
#94443=CARTESIAN_POINT('',(-40.8467768343956,56.8466430164621,12.));
#94444=CARTESIAN_POINT('',(-40.8467768343956,56.8466430164621,0.));
#94445=CARTESIAN_POINT('Ctrl Pts',(-44.569626075742,59.3276657444158,12.));
#94446=CARTESIAN_POINT('Ctrl Pts',(-44.5682447395712,59.3269051738222,12.));
#94447=CARTESIAN_POINT('Ctrl Pts',(-44.5620338188485,59.3234848865278,12.));
#94448=CARTESIAN_POINT('Ctrl Pts',(-44.5509994357953,59.317404187219,12.));
#94449=CARTESIAN_POINT('Ctrl Pts',(-44.5351541478336,59.3086616639392,12.));
#94450=CARTESIAN_POINT('Ctrl Pts',(-44.514516968128,59.2972552192072,12.));
#94451=CARTESIAN_POINT('Ctrl Pts',(-44.490484644147,59.2839437938187,12.));
#94452=CARTESIAN_POINT('Ctrl Pts',(-44.4664953242373,59.2706277440438,12.));
#94453=CARTESIAN_POINT('Ctrl Pts',(-44.4425490575932,59.2573071437801,12.));
#94454=CARTESIAN_POINT('Ctrl Pts',(-44.4186458955486,59.2439820714231,12.));
#94455=CARTESIAN_POINT('Ctrl Pts',(-44.394785891411,59.2306526095175,12.));
#94456=CARTESIAN_POINT('Ctrl Pts',(-44.3709690997495,59.217318843283,12.));
#94457=CARTESIAN_POINT('Ctrl Pts',(-44.3471955758412,59.2039808594765,12.));
#94458=CARTESIAN_POINT('Ctrl Pts',(-44.3234653750877,59.1906387451971,12.));
#94459=CARTESIAN_POINT('Ctrl Pts',(-44.2997785523413,59.1772925865191,12.));
#94460=CARTESIAN_POINT('Ctrl Pts',(-44.2761351616027,59.1639424678766,12.));
#94461=CARTESIAN_POINT('Ctrl Pts',(-44.2525352563979,59.1505884728194,12.));
#94462=CARTESIAN_POINT('Ctrl Pts',(-44.2289788899962,59.1372306844575,12.));
#94463=CARTESIAN_POINT('Ctrl Pts',(-44.2054661156876,59.1238691860307,12.));
#94464=CARTESIAN_POINT('Ctrl Pts',(-44.1819969870314,59.1105040614285,12.));
#94465=CARTESIAN_POINT('Ctrl Pts',(-44.1585715581073,59.0971353957218,12.));
#94466=CARTESIAN_POINT('Ctrl Pts',(-44.1351898834057,59.0837632749209,12.));
#94467=CARTESIAN_POINT('Ctrl Pts',(-44.1118520177223,59.0703877857529,12.));
#94468=CARTESIAN_POINT('Ctrl Pts',(-44.0885580160433,59.0570090154243,12.));
#94469=CARTESIAN_POINT('Ctrl Pts',(-44.0653079334384,59.0436270514085,12.));
#94470=CARTESIAN_POINT('Ctrl Pts',(-44.0421018249219,59.0302419811772,12.));
#94471=CARTESIAN_POINT('Ctrl Pts',(-44.0189397454593,59.0168538922087,12.));
#94472=CARTESIAN_POINT('Ctrl Pts',(-43.9958217500363,59.0034628721161,12.));
#94473=CARTESIAN_POINT('Ctrl Pts',(-43.9727478937053,58.9900690087404,12.));
#94474=CARTESIAN_POINT('Ctrl Pts',(-43.9497182316333,58.9766723902531,12.));
#94475=CARTESIAN_POINT('Ctrl Pts',(-43.9267328191507,58.9632731052704,12.));
#94476=CARTESIAN_POINT('Ctrl Pts',(-43.9037917117748,58.9498712429066,12.));
#94477=CARTESIAN_POINT('Ctrl Pts',(-43.8808949651882,58.9364668927132,12.));
#94478=CARTESIAN_POINT('Ctrl Pts',(-43.8580426352236,58.9230601446445,12.));
#94479=CARTESIAN_POINT('Ctrl Pts',(-43.8352347778419,58.9096510890128,12.));
#94480=CARTESIAN_POINT('Ctrl Pts',(-43.8124714491069,58.8962398164486,12.));
#94481=CARTESIAN_POINT('Ctrl Pts',(-43.7897527051599,58.882826417861,12.));
#94482=CARTESIAN_POINT('Ctrl Pts',(-43.7670786022392,58.8694109844636,12.));
#94483=CARTESIAN_POINT('Ctrl Pts',(-43.7444491966935,58.8559936077933,12.));
#94484=CARTESIAN_POINT('Ctrl Pts',(-43.7218645449921,58.8425743797325,12.));
#94485=CARTESIAN_POINT('Ctrl Pts',(-43.6993247037318,58.8291533925299,12.));
#94486=CARTESIAN_POINT('Ctrl Pts',(-43.6768297296402,58.8157307388247,12.));
#94487=CARTESIAN_POINT('Ctrl Pts',(-43.6543796795797,58.8023065116446,12.));
#94488=CARTESIAN_POINT('Ctrl Pts',(-43.6319746105487,58.7888808043976,12.));
#94489=CARTESIAN_POINT('Ctrl Pts',(-43.6096145796798,58.7754537108672,12.));
#94490=CARTESIAN_POINT('Ctrl Pts',(-43.5872996442343,58.7620253252059,12.));
#94491=CARTESIAN_POINT('Ctrl Pts',(-43.5650298615911,58.7485957419296,12.));
#94492=CARTESIAN_POINT('Ctrl Pts',(-43.5428052892483,58.7351650559176,12.));
#94493=CARTESIAN_POINT('Ctrl Pts',(-43.5206259848333,58.7217333624206,12.));
#94494=CARTESIAN_POINT('Ctrl Pts',(-43.4984920061071,58.708300757066,12.));
#94495=CARTESIAN_POINT('Ctrl Pts',(-43.4764034109654,58.6948673358639,12.));
#94496=CARTESIAN_POINT('Ctrl Pts',(-43.4543602574352,58.6814331952138,12.));
#94497=CARTESIAN_POINT('Ctrl Pts',(-43.4323626036736,58.6679984319095,12.));
#94498=CARTESIAN_POINT('Ctrl Pts',(-43.4104105079766,58.6545631431388,12.));
#94499=CARTESIAN_POINT('Ctrl Pts',(-43.3885040287808,58.6411274264854,12.));
#94500=CARTESIAN_POINT('Ctrl Pts',(-43.3666432246634,58.627691379929,12.));
#94501=CARTESIAN_POINT('Ctrl Pts',(-43.3448281543374,58.6142551018473,12.));
#94502=CARTESIAN_POINT('Ctrl Pts',(-43.3230588766455,58.6008186910166,12.));
#94503=CARTESIAN_POINT('Ctrl Pts',(-43.3013354505707,58.5873822466163,12.));
#94504=CARTESIAN_POINT('Ctrl Pts',(-43.2796579352405,58.5739458682317,12.));
#94505=CARTESIAN_POINT('Ctrl Pts',(-43.2580263899278,58.5605096558578,12.));
#94506=CARTESIAN_POINT('Ctrl Pts',(-43.2364408740488,58.5470737099027,12.));
#94507=CARTESIAN_POINT('Ctrl Pts',(-43.214901447157,58.5336381311911,12.));
#94508=CARTESIAN_POINT('Ctrl Pts',(-43.1934081689503,58.5202030209667,12.));
#94509=CARTESIAN_POINT('Ctrl Pts',(-43.1719610992771,58.5067684808946,12.));
#94510=CARTESIAN_POINT('Ctrl Pts',(-43.1505602981366,58.4933346130638,12.));
#94511=CARTESIAN_POINT('Ctrl Pts',(-43.1292058256774,58.4799015199904,12.));
#94512=CARTESIAN_POINT('Ctrl Pts',(-43.1078977421908,58.4664693046206,12.));
#94513=CARTESIAN_POINT('Ctrl Pts',(-43.0866361081166,58.4530380703335,12.));
#94514=CARTESIAN_POINT('Ctrl Pts',(-43.0654209840502,58.4396079209438,12.));
#94515=CARTESIAN_POINT('Ctrl Pts',(-43.0442524307432,58.4261789607055,12.));
#94516=CARTESIAN_POINT('Ctrl Pts',(-43.0231305091032,58.4127512943144,12.));
#94517=CARTESIAN_POINT('Ctrl Pts',(-43.0020552801869,58.3993250269115,12.));
#94518=CARTESIAN_POINT('Ctrl Pts',(-42.9810268052043,58.3859002640871,12.));
#94519=CARTESIAN_POINT('Ctrl Pts',(-42.9600451455267,58.3724771118835,12.));
#94520=CARTESIAN_POINT('Ctrl Pts',(-42.9391103626881,58.3590556767981,12.));
#94521=CARTESIAN_POINT('Ctrl Pts',(-42.9182225183851,58.3456360657861,12.));
#94522=CARTESIAN_POINT('Ctrl Pts',(-42.8973816744703,58.3322183862647,12.));
#94523=CARTESIAN_POINT('Ctrl Pts',(-42.8765878929545,58.3188027461158,12.));
#94524=CARTESIAN_POINT('Ctrl Pts',(-42.8558412360154,58.305389253689,12.));
#94525=CARTESIAN_POINT('Ctrl Pts',(-42.8351417659998,58.2919780178063,12.));
#94526=CARTESIAN_POINT('Ctrl Pts',(-42.8144895454234,58.278569147764,12.));
#94527=CARTESIAN_POINT('Ctrl Pts',(-42.7938846369651,58.2651627533368,12.));
#94528=CARTESIAN_POINT('Ctrl Pts',(-42.7733271034678,58.2517589447818,12.));
#94529=CARTESIAN_POINT('Ctrl Pts',(-42.7528170079482,58.238357832842,12.));
#94530=CARTESIAN_POINT('Ctrl Pts',(-42.7323544135983,58.2249595287497,12.));
#94531=CARTESIAN_POINT('Ctrl Pts',(-42.7119393837866,58.2115641442302,12.));
#94532=CARTESIAN_POINT('Ctrl Pts',(-42.6915719820516,58.1981717915043,12.));
#94533=CARTESIAN_POINT('Ctrl Pts',(-42.6712522721021,58.1847825832932,12.));
#94534=CARTESIAN_POINT('Ctrl Pts',(-42.6509803178269,58.1713966328217,12.));
#94535=CARTESIAN_POINT('Ctrl Pts',(-42.6307561832977,58.158014053823,12.));
#94536=CARTESIAN_POINT('Ctrl Pts',(-42.6105799327697,58.1446349605419,12.));
#94537=CARTESIAN_POINT('Ctrl Pts',(-42.5904516306759,58.1312594677383,12.));
#94538=CARTESIAN_POINT('Ctrl Pts',(-42.5703713416263,58.1178876906905,12.));
#94539=CARTESIAN_POINT('Ctrl Pts',(-42.5503391304182,58.1045197452003,12.));
#94540=CARTESIAN_POINT('Ctrl Pts',(-42.5303550620388,58.0911557475967,12.));
#94541=CARTESIAN_POINT('Ctrl Pts',(-42.5104192016664,58.0777958147404,12.));
#94542=CARTESIAN_POINT('Ctrl Pts',(-42.4905316146649,58.064440064027,12.));
#94543=CARTESIAN_POINT('Ctrl Pts',(-42.4706923665838,58.0510886133917,12.));
#94544=CARTESIAN_POINT('Ctrl Pts',(-42.4509015231667,58.0377415813132,12.));
#94545=CARTESIAN_POINT('Ctrl Pts',(-42.4311591503551,58.0243990868175,12.));
#94546=CARTESIAN_POINT('Ctrl Pts',(-42.4114653142891,58.011061249483,12.));
#94547=CARTESIAN_POINT('Ctrl Pts',(-42.3918200813024,57.9977281894437,12.));
#94548=CARTESIAN_POINT('Ctrl Pts',(-42.3722235179216,57.9844000273936,12.));
#94549=CARTESIAN_POINT('Ctrl Pts',(-42.3526756908764,57.9710768845923,12.));
#94550=CARTESIAN_POINT('Ctrl Pts',(-42.3331766671028,57.9577588828693,12.));
#94551=CARTESIAN_POINT('Ctrl Pts',(-42.3137265137446,57.9444461446292,12.));
#94552=CARTESIAN_POINT('Ctrl Pts',(-42.2943252981471,57.9311387928541,12.));
#94553=CARTESIAN_POINT('Ctrl Pts',(-42.274973087857,57.9178369511084,12.));
#94554=CARTESIAN_POINT('Ctrl Pts',(-42.2556699506332,57.9045407435447,12.));
#94555=CARTESIAN_POINT('Ctrl Pts',(-42.2364159544492,57.8912502949084,12.));
#94556=CARTESIAN_POINT('Ctrl Pts',(-42.2172111674945,57.8779657305423,12.));
#94557=CARTESIAN_POINT('Ctrl Pts',(-42.1980556581688,57.86468717639,12.));
#94558=CARTESIAN_POINT('Ctrl Pts',(-42.1789494950824,57.8514147590012,12.));
#94559=CARTESIAN_POINT('Ctrl Pts',(-42.1598927470671,57.8381486055376,12.));
#94560=CARTESIAN_POINT('Ctrl Pts',(-42.1408854831791,57.8248888437787,12.));
#94561=CARTESIAN_POINT('Ctrl Pts',(-42.121927772701,57.8116356021274,12.));
#94562=CARTESIAN_POINT('Ctrl Pts',(-42.1030196851344,57.798389009613,12.));
#94563=CARTESIAN_POINT('Ctrl Pts',(-42.0841612902018,57.7851491958954,12.));
#94564=CARTESIAN_POINT('Ctrl Pts',(-42.0653526578571,57.7719162912721,12.));
#94565=CARTESIAN_POINT('Ctrl Pts',(-42.0465938582877,57.7586904266828,12.));
#94566=CARTESIAN_POINT('Ctrl Pts',(-42.0278849619156,57.7454717337151,12.));
#94567=CARTESIAN_POINT('Ctrl Pts',(-42.0092260393911,57.7322603446086,12.));
#94568=CARTESIAN_POINT('Ctrl Pts',(-41.9906171615974,57.7190563922614,12.));
#94569=CARTESIAN_POINT('Ctrl Pts',(-41.9720583996601,57.7058600102365,12.));
#94570=CARTESIAN_POINT('Ctrl Pts',(-41.9535498249489,57.6926713327674,12.));
#94571=CARTESIAN_POINT('Ctrl Pts',(-41.9350915090791,57.6794904947641,12.));
#94572=CARTESIAN_POINT('Ctrl Pts',(-41.9166835239046,57.6663176318176,12.));
#94573=CARTESIAN_POINT('Ctrl Pts',(-41.8983259415244,57.6531528802059,12.));
#94574=CARTESIAN_POINT('Ctrl Pts',(-41.8800188342908,57.6399963769003,12.));
#94575=CARTESIAN_POINT('Ctrl Pts',(-41.8617622748108,57.6268482595702,12.));
#94576=CARTESIAN_POINT('Ctrl Pts',(-41.8435563359456,57.6137086665882,12.));
#94577=CARTESIAN_POINT('Ctrl Pts',(-41.8254010908051,57.6005777370349,12.));
#94578=CARTESIAN_POINT('Ctrl Pts',(-41.8072966127558,57.5874556107056,12.));
#94579=CARTESIAN_POINT('Ctrl Pts',(-41.7892429754297,57.5743424281205,12.));
#94580=CARTESIAN_POINT('Ctrl Pts',(-41.7712402527273,57.561238330532,12.));
#94581=CARTESIAN_POINT('Ctrl Pts',(-41.7532885188174,57.5481434599335,12.));
#94582=CARTESIAN_POINT('Ctrl Pts',(-41.7353878481336,57.5350579590649,12.));
#94583=CARTESIAN_POINT('Ctrl Pts',(-41.7175383153821,57.5219819714171,12.));
#94584=CARTESIAN_POINT('Ctrl Pts',(-41.6997399955447,57.5089156412343,12.));
#94585=CARTESIAN_POINT('Ctrl Pts',(-41.6819929638797,57.4958591135165,12.));
#94586=CARTESIAN_POINT('Ctrl Pts',(-41.6642972959165,57.4828125340218,12.));
#94587=CARTESIAN_POINT('Ctrl Pts',(-41.6466530674514,57.4697760492683,12.));
#94588=CARTESIAN_POINT('Ctrl Pts',(-41.6290603545666,57.4567498065562,12.));
#94589=CARTESIAN_POINT('Ctrl Pts',(-41.6115192336388,57.4437339539841,12.));
#94590=CARTESIAN_POINT('Ctrl Pts',(-41.5940297813477,57.4307286404662,12.));
#94591=CARTESIAN_POINT('Ctrl Pts',(-41.5765920746777,57.4177340157508,12.));
#94592=CARTESIAN_POINT('Ctrl Pts',(-41.5592061909176,57.4047502304231,12.));
#94593=CARTESIAN_POINT('Ctrl Pts',(-41.5418722076572,57.3917774358863,12.));
#94594=CARTESIAN_POINT('Ctrl Pts',(-41.524590202777,57.3788157843454,12.));
#94595=CARTESIAN_POINT('Ctrl Pts',(-41.5073602544396,57.3658654287937,12.));
#94596=CARTESIAN_POINT('Ctrl Pts',(-41.4901824410636,57.3529265229835,12.));
#94597=CARTESIAN_POINT('Ctrl Pts',(-41.4730568413518,57.3399992214717,12.));
#94598=CARTESIAN_POINT('Ctrl Pts',(-41.4559835343328,57.3270836796911,12.));
#94599=CARTESIAN_POINT('Ctrl Pts',(-41.4389625993948,57.3141800540137,12.));
#94600=CARTESIAN_POINT('Ctrl Pts',(-41.4219941163163,57.3012885018151,12.));
#94601=CARTESIAN_POINT('Ctrl Pts',(-41.4050781652938,57.2884091815406,12.));
#94602=CARTESIAN_POINT('Ctrl Pts',(-41.3882148268813,57.2755422525844,12.));
#94603=CARTESIAN_POINT('Ctrl Pts',(-41.3714041819223,57.2626878751596,12.));
#94604=CARTESIAN_POINT('Ctrl Pts',(-41.3546463114885,57.2498462101879,12.));
#94605=CARTESIAN_POINT('Ctrl Pts',(-41.3379412967875,57.2370174191401,12.));
#94606=CARTESIAN_POINT('Ctrl Pts',(-41.321289219149,57.2242016640198,12.));
#94607=CARTESIAN_POINT('Ctrl Pts',(-41.3046901602293,57.2113991077302,12.));
#94608=CARTESIAN_POINT('Ctrl Pts',(-41.2881442021863,57.1986099143983,12.));
#94609=CARTESIAN_POINT('Ctrl Pts',(-41.2716514278276,57.1858342496538,12.));
#94610=CARTESIAN_POINT('Ctrl Pts',(-41.2552119208465,57.17307228108,12.));
#94611=CARTESIAN_POINT('Ctrl Pts',(-41.2388257656559,57.1603241779077,12.));
#94612=CARTESIAN_POINT('Ctrl Pts',(-41.222493046943,57.147590110182,12.));
#94613=CARTESIAN_POINT('Ctrl Pts',(-41.2062138492915,57.1348702480647,12.));
#94614=CARTESIAN_POINT('Ctrl Pts',(-41.1899882567923,57.1221647611207,12.));
#94615=CARTESIAN_POINT('Ctrl Pts',(-41.1738163525901,57.1094738174957,12.));
#94616=CARTESIAN_POINT('Ctrl Pts',(-41.1576982197374,57.0967975854874,12.));
#94617=CARTESIAN_POINT('Ctrl Pts',(-41.1416339422117,57.084136235426,12.));
#94618=CARTESIAN_POINT('Ctrl Pts',(-41.1256236057442,57.0714899412099,12.));
#94619=CARTESIAN_POINT('Ctrl Pts',(-41.1096672990148,57.0588588825298,12.));
#94620=CARTESIAN_POINT('Ctrl Pts',(-41.0937651137549,57.046243245068,12.));
#94621=CARTESIAN_POINT('Ctrl Pts',(-41.0779171422438,57.0336432158536,12.));
#94622=CARTESIAN_POINT('Ctrl Pts',(-41.0621234751007,57.0210589791788,12.));
#94623=CARTESIAN_POINT('Ctrl Pts',(-41.0463841993608,57.008490713042,12.));
#94624=CARTESIAN_POINT('Ctrl Pts',(-41.0306993953988,56.995938583472,12.));
#94625=CARTESIAN_POINT('Ctrl Pts',(-41.0150691398947,56.9834027500117,12.));
#94626=CARTESIAN_POINT('Ctrl Pts',(-40.9994935117276,56.9708833766137,12.));
#94627=CARTESIAN_POINT('Ctrl Pts',(-40.9839725967121,56.9583806404069,12.));
#94628=CARTESIAN_POINT('Ctrl Pts',(-40.9685064933074,56.9458947422608,12.));
#94629=CARTESIAN_POINT('Ctrl Pts',(-40.9530953165031,56.9334259140049,12.));
#94630=CARTESIAN_POINT('Ctrl Pts',(-40.9377391857128,56.9209743960992,12.));
#94631=CARTESIAN_POINT('Ctrl Pts',(-40.9224382132427,56.9085404164502,12.));
#94632=CARTESIAN_POINT('Ctrl Pts',(-40.9071924937508,56.8961241708861,12.));
#94633=CARTESIAN_POINT('Ctrl Pts',(-40.8920020903293,56.8837257978343,12.));
#94634=CARTESIAN_POINT('Ctrl Pts',(-40.8768670342052,56.8713453764905,12.));
#94635=CARTESIAN_POINT('Ctrl Pts',(-40.864803275942,56.8614554317668,12.));
#94636=CARTESIAN_POINT('Ctrl Pts',(-40.8557803680277,56.8540460739472,12.));
#94637=CARTESIAN_POINT('Ctrl Pts',(-40.8497761671036,56.8491101022591,12.));
#94638=CARTESIAN_POINT('Ctrl Pts',(-40.8467768343956,56.8466430164621,12.));
#94639=CARTESIAN_POINT('Ctrl Pts',(-45.7706564944896,58.4060826907797,-5.55111512312578E-16));
#94640=CARTESIAN_POINT('Ctrl Pts',(-45.7706564944896,58.4060826907797,4.));
#94641=CARTESIAN_POINT('Ctrl Pts',(-45.7706564944896,58.4060826907797,8.));
#94642=CARTESIAN_POINT('Ctrl Pts',(-45.7706564944896,58.4060826907797,12.));
#94643=CARTESIAN_POINT('Ctrl Pts',(-45.7969367893064,58.5127761886847,-5.55111512312578E-16));
#94644=CARTESIAN_POINT('Ctrl Pts',(-45.7969367893064,58.5127761886847,4.));
#94645=CARTESIAN_POINT('Ctrl Pts',(-45.7969367893064,58.5127761886847,8.00000000000001));
#94646=CARTESIAN_POINT('Ctrl Pts',(-45.7969367893064,58.5127761886847,12.));
#94647=CARTESIAN_POINT('Ctrl Pts',(-45.7788617791411,58.714632205056,-5.55111512312578E-16));
#94648=CARTESIAN_POINT('Ctrl Pts',(-45.7788617791411,58.714632205056,4.));
#94649=CARTESIAN_POINT('Ctrl Pts',(-45.7788617791411,58.714632205056,7.99999999999999));
#94650=CARTESIAN_POINT('Ctrl Pts',(-45.7788617791411,58.714632205056,12.));
#94651=CARTESIAN_POINT('Ctrl Pts',(-45.6563266621663,58.870677144318,-5.55111512312578E-16));
#94652=CARTESIAN_POINT('Ctrl Pts',(-45.6563266621663,58.870677144318,4.));
#94653=CARTESIAN_POINT('Ctrl Pts',(-45.6563266621663,58.870677144318,8.00000000000001));
#94654=CARTESIAN_POINT('Ctrl Pts',(-45.6563266621663,58.870677144318,12.));
#94655=CARTESIAN_POINT('Ctrl Pts',(-45.5911481700252,58.9211100416378,-5.55111512312578E-16));
#94656=CARTESIAN_POINT('Ctrl Pts',(-45.5911481700252,58.9211100416378,4.));
#94657=CARTESIAN_POINT('Ctrl Pts',(-45.5911481700252,58.9211100416378,8.));
#94658=CARTESIAN_POINT('Ctrl Pts',(-45.5911481700252,58.9211100416378,12.));
#94659=CARTESIAN_POINT('',(-45.7706564944896,58.4060826907797,2.77555756156289E-16));
#94660=CARTESIAN_POINT('',(-45.5911481700253,58.9211100416379,0.));
#94661=CARTESIAN_POINT('Ctrl Pts',(-45.7706564944896,58.4060826907797,-1.38777878078145E-16));
#94662=CARTESIAN_POINT('Ctrl Pts',(-45.7969367893064,58.5127761886847,-1.38777878078145E-16));
#94663=CARTESIAN_POINT('Ctrl Pts',(-45.7866082120691,58.628122483754,-1.38777878078144E-16));
#94664=CARTESIAN_POINT('Ctrl Pts',(-45.7421702122001,58.7285100597672,-1.38777878078145E-16));
#94665=CARTESIAN_POINT('Ctrl Pts',(-45.7088417122983,58.8038007417772,-1.38777878078145E-16));
#94666=CARTESIAN_POINT('Ctrl Pts',(-45.6563266621663,58.870677144318,-1.38777878078145E-16));
#94667=CARTESIAN_POINT('Ctrl Pts',(-45.5911481700252,58.9211100416378,-1.38777878078145E-16));
#94668=CARTESIAN_POINT('',(-45.5911481700253,58.9211100416379,12.));
#94669=CARTESIAN_POINT('Ctrl Pts',(-45.5911481700252,58.9211100416378,-5.55111512312578E-16));
#94670=CARTESIAN_POINT('Ctrl Pts',(-45.5911481700252,58.9211100416378,4.));
#94671=CARTESIAN_POINT('Ctrl Pts',(-45.5911481700252,58.9211100416378,8.));
#94672=CARTESIAN_POINT('Ctrl Pts',(-45.5911481700252,58.9211100416378,12.));
#94673=CARTESIAN_POINT('',(-45.7706564944896,58.4060826907797,12.));
#94674=CARTESIAN_POINT('Ctrl Pts',(-45.5911481700252,58.9211100416378,12.));
#94675=CARTESIAN_POINT('Ctrl Pts',(-45.6563266621663,58.870677144318,12.));
#94676=CARTESIAN_POINT('Ctrl Pts',(-45.7088417122983,58.8038007417772,12.));
#94677=CARTESIAN_POINT('Ctrl Pts',(-45.7421702122001,58.7285100597672,12.));
#94678=CARTESIAN_POINT('Ctrl Pts',(-45.7866082120691,58.628122483754,12.));
#94679=CARTESIAN_POINT('Ctrl Pts',(-45.7969367893064,58.5127761886847,12.));
#94680=CARTESIAN_POINT('Ctrl Pts',(-45.7706564944896,58.4060826907797,12.));
#94681=CARTESIAN_POINT('Ctrl Pts',(-45.7706564944896,58.4060826907797,12.));
#94682=CARTESIAN_POINT('Ctrl Pts',(-45.7706564944896,58.4060826907797,8.));
#94683=CARTESIAN_POINT('Ctrl Pts',(-45.7706564944896,58.4060826907797,4.));
#94684=CARTESIAN_POINT('Ctrl Pts',(-45.7706564944896,58.4060826907797,-5.55111512312578E-16));
#94685=CARTESIAN_POINT('Origin',(-2.28269173065022E-10,2.97323128204029E-10,
0.));
#94686=CARTESIAN_POINT('Origin',(-2.28269173065022E-10,2.97323128204029E-10,
12.));
#94687=CARTESIAN_POINT('Origin',(-2.28269173065022E-10,2.97323128204029E-10,
0.));
#94688=CARTESIAN_POINT('Ctrl Pts',(-39.7746412831503,62.9938720098766,-5.55111512312578E-16));
#94689=CARTESIAN_POINT('Ctrl Pts',(-39.7746412831503,62.9938720098766,4.));
#94690=CARTESIAN_POINT('Ctrl Pts',(-39.7746412831503,62.9938720098766,8.));
#94691=CARTESIAN_POINT('Ctrl Pts',(-39.7746412831503,62.9938720098766,12.));
#94692=CARTESIAN_POINT('Ctrl Pts',(-39.6817295782362,63.0525369183202,-5.55111512312578E-16));
#94693=CARTESIAN_POINT('Ctrl Pts',(-39.6817295782362,63.0525369183202,4.));
#94694=CARTESIAN_POINT('Ctrl Pts',(-39.6817295782362,63.0525369183202,8.));
#94695=CARTESIAN_POINT('Ctrl Pts',(-39.6817295782362,63.0525369183202,12.));
#94696=CARTESIAN_POINT('Ctrl Pts',(-39.4845131830972,63.0992090147607,-5.55111512312578E-16));
#94697=CARTESIAN_POINT('Ctrl Pts',(-39.4845131830972,63.0992090147607,4.));
#94698=CARTESIAN_POINT('Ctrl Pts',(-39.4845131830972,63.0992090147607,7.99999999999999));
#94699=CARTESIAN_POINT('Ctrl Pts',(-39.4845131830972,63.0992090147607,12.));
#94700=CARTESIAN_POINT('Ctrl Pts',(-39.2977314459988,63.0322949727905,-5.55111512312578E-16));
#94701=CARTESIAN_POINT('Ctrl Pts',(-39.2977314459988,63.0322949727905,4.));
#94702=CARTESIAN_POINT('Ctrl Pts',(-39.2977314459988,63.0322949727905,8.00000000000001));
#94703=CARTESIAN_POINT('Ctrl Pts',(-39.2977314459988,63.0322949727905,12.));
#94704=CARTESIAN_POINT('Ctrl Pts',(-39.2292784191472,62.9864049293631,-5.55111512312578E-16));
#94705=CARTESIAN_POINT('Ctrl Pts',(-39.2292784191472,62.9864049293631,4.));
#94706=CARTESIAN_POINT('Ctrl Pts',(-39.2292784191471,62.9864049293632,8.));
#94707=CARTESIAN_POINT('Ctrl Pts',(-39.2292784191471,62.9864049293632,12.));
#94708=CARTESIAN_POINT('',(-39.7746412831503,62.9938720098766,0.));
#94709=CARTESIAN_POINT('',(-39.2292784191471,62.9864049293634,0.));
#94710=CARTESIAN_POINT('Ctrl Pts',(-39.7746412831503,62.9938720098766,4.16333634234434E-16));
#94711=CARTESIAN_POINT('Ctrl Pts',(-39.6817295782362,63.0525369183202,4.16333634234433E-16));
#94712=CARTESIAN_POINT('Ctrl Pts',(-39.5690344952996,63.0792066877147,4.16333634234434E-16));
#94713=CARTESIAN_POINT('Ctrl Pts',(-39.4597466476417,63.0687871057915,4.16333634234434E-16));
#94714=CARTESIAN_POINT('Ctrl Pts',(-39.3777807618982,63.0609724193491,4.16333634234434E-16));
#94715=CARTESIAN_POINT('Ctrl Pts',(-39.2977314459988,63.0322949727905,4.16333634234433E-16));
#94716=CARTESIAN_POINT('Ctrl Pts',(-39.2292784191472,62.9864049293631,4.16333634234434E-16));
#94717=CARTESIAN_POINT('',(-39.229278419147,62.9864049293633,12.));
#94718=CARTESIAN_POINT('Ctrl Pts',(-39.2292784191472,62.9864049293631,-5.55111512312578E-16));
#94719=CARTESIAN_POINT('Ctrl Pts',(-39.2292784191472,62.9864049293631,4.));
#94720=CARTESIAN_POINT('Ctrl Pts',(-39.2292784191471,62.9864049293632,8.));
#94721=CARTESIAN_POINT('Ctrl Pts',(-39.2292784191471,62.9864049293632,12.));
#94722=CARTESIAN_POINT('',(-39.7746412831503,62.9938720098766,12.));
#94723=CARTESIAN_POINT('Ctrl Pts',(-39.2292784191471,62.9864049293632,12.));
#94724=CARTESIAN_POINT('Ctrl Pts',(-39.2977314459988,63.0322949727905,12.));
#94725=CARTESIAN_POINT('Ctrl Pts',(-39.3777807618981,63.0609724193492,12.));
#94726=CARTESIAN_POINT('Ctrl Pts',(-39.4597466476416,63.0687871057916,12.));
#94727=CARTESIAN_POINT('Ctrl Pts',(-39.5690344952996,63.0792066877148,12.));
#94728=CARTESIAN_POINT('Ctrl Pts',(-39.6817295782362,63.0525369183202,12.));
#94729=CARTESIAN_POINT('Ctrl Pts',(-39.7746412831503,62.9938720098766,12.));
#94730=CARTESIAN_POINT('Ctrl Pts',(-39.7746412831503,62.9938720098766,12.));
#94731=CARTESIAN_POINT('Ctrl Pts',(-39.7746412831503,62.9938720098766,8.));
#94732=CARTESIAN_POINT('Ctrl Pts',(-39.7746412831503,62.9938720098766,4.));
#94733=CARTESIAN_POINT('Ctrl Pts',(-39.7746412831503,62.9938720098766,-5.55111512312578E-16));
#94734=CARTESIAN_POINT('Ctrl Pts',(-35.7368311217509,60.1903555511633,0.));
#94735=CARTESIAN_POINT('Ctrl Pts',(-35.7368311217509,60.1903555511633,12.));
#94736=CARTESIAN_POINT('Ctrl Pts',(-35.7396040203973,60.1930746580239,0.));
#94737=CARTESIAN_POINT('Ctrl Pts',(-35.7396040203973,60.1930746580239,12.));
#94738=CARTESIAN_POINT('Ctrl Pts',(-35.7451551752456,60.1985151474406,0.));
#94739=CARTESIAN_POINT('Ctrl Pts',(-35.7451551752456,60.1985151474406,12.));
#94740=CARTESIAN_POINT('Ctrl Pts',(-35.7534979801871,60.2066827086579,0.));
#94741=CARTESIAN_POINT('Ctrl Pts',(-35.7534979801871,60.2066827086579,12.));
#94742=CARTESIAN_POINT('Ctrl Pts',(-35.7646538667299,60.2175864449678,0.));
#94743=CARTESIAN_POINT('Ctrl Pts',(-35.7646538667299,60.2175864449678,12.));
#94744=CARTESIAN_POINT('Ctrl Pts',(-35.7786523045782,60.2312388621286,0.));
#94745=CARTESIAN_POINT('Ctrl Pts',(-35.7786523045782,60.2312388621286,12.));
#94746=CARTESIAN_POINT('Ctrl Pts',(-35.7927043145164,60.2449139865206,0.));
#94747=CARTESIAN_POINT('Ctrl Pts',(-35.7927043145164,60.2449139865206,12.));
#94748=CARTESIAN_POINT('Ctrl Pts',(-35.8068098723386,60.2586117365278,0.));
#94749=CARTESIAN_POINT('Ctrl Pts',(-35.8068098723386,60.2586117365278,12.));
#94750=CARTESIAN_POINT('Ctrl Pts',(-35.8209689272574,60.2723319687507,0.));
#94751=CARTESIAN_POINT('Ctrl Pts',(-35.8209689272574,60.2723319687507,12.));
#94752=CARTESIAN_POINT('Ctrl Pts',(-35.8351814020424,60.2860744798563,0.));
#94753=CARTESIAN_POINT('Ctrl Pts',(-35.8351814020424,60.2860744798563,12.));
#94754=CARTESIAN_POINT('Ctrl Pts',(-35.8494472046783,60.2998390330173,0.));
#94755=CARTESIAN_POINT('Ctrl Pts',(-35.8494472046783,60.2998390330173,12.));
#94756=CARTESIAN_POINT('Ctrl Pts',(-35.8637662371635,60.313625378281,0.));
#94757=CARTESIAN_POINT('Ctrl Pts',(-35.8637662371635,60.313625378281,12.));
#94758=CARTESIAN_POINT('Ctrl Pts',(-35.878138405151,60.3274332746782,0.));
#94759=CARTESIAN_POINT('Ctrl Pts',(-35.878138405151,60.3274332746782,12.));
#94760=CARTESIAN_POINT('Ctrl Pts',(-35.8925636280632,60.3412625135223,0.));
#94761=CARTESIAN_POINT('Ctrl Pts',(-35.8925636280632,60.3412625135223,12.));
#94762=CARTESIAN_POINT('Ctrl Pts',(-35.9070418358501,60.3551129108794,0.));
#94763=CARTESIAN_POINT('Ctrl Pts',(-35.9070418358501,60.3551129108794,12.));
#94764=CARTESIAN_POINT('Ctrl Pts',(-35.9215729642219,60.368984296546,0.));
#94765=CARTESIAN_POINT('Ctrl Pts',(-35.9215729642219,60.368984296546,12.));
#94766=CARTESIAN_POINT('Ctrl Pts',(-35.9361569506955,60.3828765049031,0.));
#94767=CARTESIAN_POINT('Ctrl Pts',(-35.9361569506955,60.3828765049031,12.));
#94768=CARTESIAN_POINT('Ctrl Pts',(-35.9507937296726,60.3967893635487,0.));
#94769=CARTESIAN_POINT('Ctrl Pts',(-35.9507937296726,60.3967893635487,12.));
#94770=CARTESIAN_POINT('Ctrl Pts',(-35.9654832299627,60.4107226875759,0.));
#94771=CARTESIAN_POINT('Ctrl Pts',(-35.9654832299627,60.4107226875759,12.));
#94772=CARTESIAN_POINT('Ctrl Pts',(-35.9802253773534,60.4246762854961,0.));
#94773=CARTESIAN_POINT('Ctrl Pts',(-35.9802253773534,60.4246762854961,12.));
#94774=CARTESIAN_POINT('Ctrl Pts',(-35.9950200962175,60.438649962949,0.));
#94775=CARTESIAN_POINT('Ctrl Pts',(-35.9950200962175,60.438649962949,12.));
#94776=CARTESIAN_POINT('Ctrl Pts',(-36.0098673113556,60.452643526964,0.));
#94777=CARTESIAN_POINT('Ctrl Pts',(-36.0098673113556,60.452643526964,12.));
#94778=CARTESIAN_POINT('Ctrl Pts',(-36.0247669500867,60.4666567908053,0.));
#94779=CARTESIAN_POINT('Ctrl Pts',(-36.0247669500867,60.4666567908053,12.));
